#191893=CARTESIAN_POINT('Ctrl Pts',(10.3211590649999,11.6,1.33482139999999));
#191894=CARTESIAN_POINT('Ctrl Pts',(10.3199801189999,15.2,1.33480649299999));
#191895=CARTESIAN_POINT('Ctrl Pts',(10.3199801189999,11.6,1.33480649299999));
#191896=CARTESIAN_POINT('Ctrl Pts',(10.3188100709999,15.2,1.33479055299999));
#191897=CARTESIAN_POINT('Ctrl Pts',(10.3188100709999,11.6,1.33479055299999));
#191898=CARTESIAN_POINT('Ctrl Pts',(10.3176489429999,15.2,1.33477359499999));
#191899=CARTESIAN_POINT('Ctrl Pts',(10.3176489429999,11.6,1.33477359499999));
#191900=CARTESIAN_POINT('Ctrl Pts',(10.3164967599999,15.2,1.33475563599998));
#191901=CARTESIAN_POINT('Ctrl Pts',(10.3164967599999,11.6,1.33475563599998));
#191902=CARTESIAN_POINT('Ctrl Pts',(10.3153535459999,15.2,1.33473669599999));
#191903=CARTESIAN_POINT('Ctrl Pts',(10.3153535459999,11.6,1.33473669599998));
#191904=CARTESIAN_POINT('Ctrl Pts',(10.3142193239999,15.2,1.33471678699999));
#191905=CARTESIAN_POINT('Ctrl Pts',(10.3142193239999,11.6,1.33471678699998));
#191906=CARTESIAN_POINT('Ctrl Pts',(10.3130941179999,15.2,1.33469593099999));
#191907=CARTESIAN_POINT('Ctrl Pts',(10.3130941179999,11.6,1.33469593099999));
#191908=CARTESIAN_POINT('Ctrl Pts',(10.3119779519999,15.2,1.33467414199998));
#191909=CARTESIAN_POINT('Ctrl Pts',(10.3119779519999,11.6,1.33467414199998));
#191910=CARTESIAN_POINT('Ctrl Pts',(10.3108708509999,15.2,1.33465143799999));
#191911=CARTESIAN_POINT('Ctrl Pts',(10.3108708509999,11.6,1.33465143799999));
#191912=CARTESIAN_POINT('Ctrl Pts',(10.3097728379999,15.2,1.33462783699999));
#191913=CARTESIAN_POINT('Ctrl Pts',(10.3097728379999,11.6,1.33462783699999));
#191914=CARTESIAN_POINT('Ctrl Pts',(10.3086839379999,15.2,1.33460335699999));
#191915=CARTESIAN_POINT('Ctrl Pts',(10.3086839379999,11.6,1.33460335699999));
#191916=CARTESIAN_POINT('Ctrl Pts',(10.3076041749999,15.2,1.33457801399999));
#191917=CARTESIAN_POINT('Ctrl Pts',(10.3076041749999,11.6,1.33457801399999));
#191918=CARTESIAN_POINT('Ctrl Pts',(10.3065335739999,15.2,1.33455182699999));
#191919=CARTESIAN_POINT('Ctrl Pts',(10.3065335739999,11.6,1.33455182699999));
#191920=CARTESIAN_POINT('Ctrl Pts',(10.3054721599999,15.2,1.33452481299999));
#191921=CARTESIAN_POINT('Ctrl Pts',(10.3054721599999,11.6,1.33452481299999));
#191922=CARTESIAN_POINT('Ctrl Pts',(10.3044199559999,15.2,1.33449698899998));
#191923=CARTESIAN_POINT('Ctrl Pts',(10.3044199559999,11.6,1.33449698899998));
#191924=CARTESIAN_POINT('Ctrl Pts',(10.3033769899999,15.2,1.33446837399998));
#191925=CARTESIAN_POINT('Ctrl Pts',(10.3033769899999,11.6,1.33446837399998));
#191926=CARTESIAN_POINT('Ctrl Pts',(10.3023432839999,15.2,1.33443898699999));
#191927=CARTESIAN_POINT('Ctrl Pts',(10.3023432839999,11.6,1.33443898699999));
#191928=CARTESIAN_POINT('Ctrl Pts',(10.3013188639999,15.2,1.33440884399999));
#191929=CARTESIAN_POINT('Ctrl Pts',(10.3013188639999,11.6,1.33440884399999));
#191930=CARTESIAN_POINT('Ctrl Pts',(10.3003037569999,15.2,1.33437796599999));
#191931=CARTESIAN_POINT('Ctrl Pts',(10.3003037569999,11.6,1.33437796599999));
#191932=CARTESIAN_POINT('Ctrl Pts',(10.2992979849999,15.2,1.33434636899999));
#191933=CARTESIAN_POINT('Ctrl Pts',(10.2992979849999,11.6,1.33434636899999));
#191934=CARTESIAN_POINT('Ctrl Pts',(10.2983015759999,15.2,1.33431407099998));
#191935=CARTESIAN_POINT('Ctrl Pts',(10.2983015759999,11.6,1.33431407099998));
#191936=CARTESIAN_POINT('Ctrl Pts',(10.2973145539999,15.2,1.33428109299999));
#191937=CARTESIAN_POINT('Ctrl Pts',(10.2973145539999,11.6,1.33428109299999));
#191938=CARTESIAN_POINT('Ctrl Pts',(10.2963369469999,15.2,1.33424745299998));
#191939=CARTESIAN_POINT('Ctrl Pts',(10.2963369469999,11.6,1.33424745299998));
#191940=CARTESIAN_POINT('Ctrl Pts',(10.2953687779999,15.2,1.33421316799998));
#191941=CARTESIAN_POINT('Ctrl Pts',(10.2953687779999,11.6,1.33421316799998));
#191942=CARTESIAN_POINT('Ctrl Pts',(10.2944100739999,15.2,1.33417825799999));
#191943=CARTESIAN_POINT('Ctrl Pts',(10.2944100739999,11.6,1.33417825799999));
#191944=CARTESIAN_POINT('Ctrl Pts',(10.2934608629999,15.2,1.33414274199998));
#191945=CARTESIAN_POINT('Ctrl Pts',(10.2934608629999,11.6,1.33414274199998));
#191946=CARTESIAN_POINT('Ctrl Pts',(10.2925211679999,15.2,1.33410663999999));
#191947=CARTESIAN_POINT('Ctrl Pts',(10.2925211679999,11.6,1.33410663999999));
#191948=CARTESIAN_POINT('Ctrl Pts',(10.2915910169999,15.2,1.33406996999998));
#191949=CARTESIAN_POINT('Ctrl Pts',(10.2915910169999,11.6,1.33406996999998));
#191950=CARTESIAN_POINT('Ctrl Pts',(10.2906757369999,15.2,1.33403296599999));
#191951=CARTESIAN_POINT('Ctrl Pts',(10.2906757369999,11.6,1.33403296599999));
#191952=CARTESIAN_POINT('Ctrl Pts',(10.2899521419999,15.2,1.33400298799998));
#191953=CARTESIAN_POINT('Ctrl Pts',(10.2899521419999,11.6,1.33400298799998));
#191954=CARTESIAN_POINT('Ctrl Pts',(10.2894150039999,15.2,1.33398033399999));
#191955=CARTESIAN_POINT('Ctrl Pts',(10.2894150039999,11.6,1.33398033399999));
#191956=CARTESIAN_POINT('Ctrl Pts',(10.2890605209999,15.2,1.33396520799999));
#191957=CARTESIAN_POINT('Ctrl Pts',(10.2890605209999,11.6,1.33396520799998));
#191958=CARTESIAN_POINT('Ctrl Pts',(10.2888863229999,15.2,1.33395773199998));
#191959=CARTESIAN_POINT('Ctrl Pts',(10.2888863229999,11.6,1.33395773199998));
#191960=CARTESIAN_POINT('',(10.2888863229999,12.2,1.33395773199998));
#191961=CARTESIAN_POINT('',(10.2888863229999,15.2,1.33395773199998));
#191962=CARTESIAN_POINT('',(10.2888863229999,12.2,1.33395773199998));
#191963=CARTESIAN_POINT('Ctrl Pts',(11.4479048649999,12.2,1.09337742899998));
#191964=CARTESIAN_POINT('Ctrl Pts',(11.4471888789999,12.2,1.09364567099998));
#191965=CARTESIAN_POINT('Ctrl Pts',(11.4457572179999,12.2,1.09418172899999));
#191966=CARTESIAN_POINT('Ctrl Pts',(11.4436106639999,12.2,1.09498454299999));
#191967=CARTESIAN_POINT('Ctrl Pts',(11.4407504639999,12.2,1.09605241699999));
#191968=CARTESIAN_POINT('Ctrl Pts',(11.4371783349999,12.2,1.09738301699998));
#191969=CARTESIAN_POINT('Ctrl Pts',(11.4336093279999,12.2,1.09870937299998));
#191970=CARTESIAN_POINT('Ctrl Pts',(11.4300434449999,12.2,1.10003148899999));
#191971=CARTESIAN_POINT('Ctrl Pts',(11.4264806909999,12.2,1.10134936399998));
#191972=CARTESIAN_POINT('Ctrl Pts',(11.4229210689999,12.2,1.10266299899999));
#191973=CARTESIAN_POINT('Ctrl Pts',(11.4193645909999,12.2,1.10397239899998));
#191974=CARTESIAN_POINT('Ctrl Pts',(11.4158112619999,12.2,1.10527756499998));
#191975=CARTESIAN_POINT('Ctrl Pts',(11.4122610939999,12.2,1.10657849999999));
#191976=CARTESIAN_POINT('Ctrl Pts',(11.4087140989999,12.2,1.10787520999999));
#191977=CARTESIAN_POINT('Ctrl Pts',(11.4051702859999,12.2,1.10916769599998));
#191978=CARTESIAN_POINT('Ctrl Pts',(11.4016296639999,12.2,1.11045596299999));
#191979=CARTESIAN_POINT('Ctrl Pts',(11.3980922449999,12.2,1.11174001299998));
#191980=CARTESIAN_POINT('Ctrl Pts',(11.3945580339999,12.2,1.11301984899999));
#191981=CARTESIAN_POINT('Ctrl Pts',(11.3910270409999,12.2,1.11429547399998));
#191982=CARTESIAN_POINT('Ctrl Pts',(11.3874992709999,12.2,1.11556689099999));
#191983=CARTESIAN_POINT('Ctrl Pts',(11.3839747349999,12.2,1.11683410099999));
#191984=CARTESIAN_POINT('Ctrl Pts',(11.3804534399999,12.2,1.11809710599998));
#191985=CARTESIAN_POINT('Ctrl Pts',(11.3769353939999,12.2,1.11935591199999));
#191986=CARTESIAN_POINT('Ctrl Pts',(11.3734206059999,12.2,1.12061051999999));
#191987=CARTESIAN_POINT('Ctrl Pts',(11.3699090849999,12.2,1.12186093299998));
#191988=CARTESIAN_POINT('Ctrl Pts',(11.3664008399999,12.2,1.12310715499999));
#191989=CARTESIAN_POINT('Ctrl Pts',(11.3628958789999,12.2,1.12434918799998));
#191990=CARTESIAN_POINT('Ctrl Pts',(11.3593942139999,12.2,1.12558703499999));
#191991=CARTESIAN_POINT('Ctrl Pts',(11.3558958509999,12.2,1.12682069999999));
#191992=CARTESIAN_POINT('Ctrl Pts',(11.3524007989999,12.2,1.12805018499999));
#191993=CARTESIAN_POINT('Ctrl Pts',(11.3489090669999,12.2,1.12927549499998));
#191994=CARTESIAN_POINT('Ctrl Pts',(11.3454206639999,12.2,1.13049662999999));
#191995=CARTESIAN_POINT('Ctrl Pts',(11.3419355979999,12.2,1.13171359399999));
#191996=CARTESIAN_POINT('Ctrl Pts',(11.3384538779999,12.2,1.13292639099999));
#191997=CARTESIAN_POINT('Ctrl Pts',(11.3349755119999,12.2,1.13413502399998));
#191998=CARTESIAN_POINT('Ctrl Pts',(11.3315005099999,12.2,1.13533949399999));
#191999=CARTESIAN_POINT('Ctrl Pts',(11.3280288789999,12.2,1.13653980499999));
#192000=CARTESIAN_POINT('Ctrl Pts',(11.3245606299999,12.2,1.13773596199998));
#192001=CARTESIAN_POINT('Ctrl Pts',(11.3210957719999,12.2,1.13892796799998));
#192002=CARTESIAN_POINT('Ctrl Pts',(11.3176343119999,12.2,1.14011582299999));
#192003=CARTESIAN_POINT('Ctrl Pts',(11.3141762599999,12.2,1.14129953199999));
#192004=CARTESIAN_POINT('Ctrl Pts',(11.3107216239999,12.2,1.14247909899999));
#192005=CARTESIAN_POINT('Ctrl Pts',(11.3072704139999,12.2,1.14365452599999));
#192006=CARTESIAN_POINT('Ctrl Pts',(11.3038226389999,12.2,1.14482581599999));
#192007=CARTESIAN_POINT('Ctrl Pts',(11.3003783059999,12.2,1.14599297299999));
#192008=CARTESIAN_POINT('Ctrl Pts',(11.2969374249999,12.2,1.14715599999998));
#192009=CARTESIAN_POINT('Ctrl Pts',(11.2935000059999,12.2,1.14831489899998));
#192010=CARTESIAN_POINT('Ctrl Pts',(11.2900660559999,12.2,1.14946967499999));
#192011=CARTESIAN_POINT('Ctrl Pts',(11.2866355859999,12.2,1.15062032999999));
#192012=CARTESIAN_POINT('Ctrl Pts',(11.2832086039999,12.2,1.15176686799999));
#192013=CARTESIAN_POINT('Ctrl Pts',(11.2797851169999,12.2,1.15290929199999));
#192014=CARTESIAN_POINT('Ctrl Pts',(11.2763651379999,12.2,1.15404760499999));
#192015=CARTESIAN_POINT('Ctrl Pts',(11.2729486729999,12.2,1.15518180999999));
#192016=CARTESIAN_POINT('Ctrl Pts',(11.2695357319999,12.2,1.15631191099999));
#192017=CARTESIAN_POINT('Ctrl Pts',(11.2661263239999,12.2,1.15743791099999));
#192018=CARTESIAN_POINT('Ctrl Pts',(11.2627204589999,12.2,1.15855981299998));
#192019=CARTESIAN_POINT('Ctrl Pts',(11.2593181439999,12.2,1.15967762199999));
#192020=CARTESIAN_POINT('Ctrl Pts',(11.2559193889999,12.2,1.16079133899999));
#192021=CARTESIAN_POINT('Ctrl Pts',(11.2525242039999,12.2,1.16190096799999));
#192022=CARTESIAN_POINT('Ctrl Pts',(11.2491325969999,12.2,1.16300651299999));
#192023=CARTESIAN_POINT('Ctrl Pts',(11.2457445769999,12.2,1.16410797799999));
#192024=CARTESIAN_POINT('Ctrl Pts',(11.2423601539999,12.2,1.16520536499999));
#192025=CARTESIAN_POINT('Ctrl Pts',(11.2389793369999,12.2,1.16629867799999));
#192026=CARTESIAN_POINT('Ctrl Pts',(11.2356021349999,12.2,1.16738791999999));
#192027=CARTESIAN_POINT('Ctrl Pts',(11.2322285569999,12.2,1.16847309399999));
#192028=CARTESIAN_POINT('Ctrl Pts',(11.2288586119999,12.2,1.16955420599998));
#192029=CARTESIAN_POINT('Ctrl Pts',(11.2254923089999,12.2,1.17063125699998));
#192030=CARTESIAN_POINT('Ctrl Pts',(11.2221296589999,12.2,1.17170425099999));
#192031=CARTESIAN_POINT('Ctrl Pts',(11.2187706689999,12.2,1.17277319199999));
#192032=CARTESIAN_POINT('Ctrl Pts',(11.2154153489999,12.2,1.17383808299998));
#192033=CARTESIAN_POINT('Ctrl Pts',(11.2120637079999,12.2,1.17489892799998));
#192034=CARTESIAN_POINT('Ctrl Pts',(11.2087157559999,12.2,1.17595572999999));
#192035=CARTESIAN_POINT('Ctrl Pts',(11.2053715019999,12.2,1.17700849199998));
#192036=CARTESIAN_POINT('Ctrl Pts',(11.2020309559999,12.2,1.17805721999999));
#192037=CARTESIAN_POINT('Ctrl Pts',(11.1986941249999,12.2,1.17910191499998));
#192038=CARTESIAN_POINT('Ctrl Pts',(11.1953610209999,12.2,1.18014258099999));
#192039=CARTESIAN_POINT('Ctrl Pts',(11.1920316519999,12.2,1.18117922199998));
#192040=CARTESIAN_POINT('Ctrl Pts',(11.1887060269999,12.2,1.18221184299999));
#192041=CARTESIAN_POINT('Ctrl Pts',(11.1853841569999,12.2,1.18324044599999));
#192042=CARTESIAN_POINT('Ctrl Pts',(11.1820660499999,12.2,1.18426503499999));
#192043=CARTESIAN_POINT('Ctrl Pts',(11.1787517149999,12.2,1.18528561399998));
#192044=CARTESIAN_POINT('Ctrl Pts',(11.1754411629999,12.2,1.18630218499999));
#192045=CARTESIAN_POINT('Ctrl Pts',(11.1721344009999,12.2,1.18731475499999));
#192046=CARTESIAN_POINT('Ctrl Pts',(11.1688314409999,12.2,1.18832332399998));
#192047=CARTESIAN_POINT('Ctrl Pts',(11.1655322919999,12.2,1.18932789899999));
#192048=CARTESIAN_POINT('Ctrl Pts',(11.1622369629999,12.2,1.19032848099998));
#192049=CARTESIAN_POINT('Ctrl Pts',(11.1589454619999,12.2,1.19132507599998));
#192050=CARTESIAN_POINT('Ctrl Pts',(11.1556577999999,12.2,1.19231768599999));
#192051=CARTESIAN_POINT('Ctrl Pts',(11.1523739879999,12.2,1.19330631599999));
#192052=CARTESIAN_POINT('Ctrl Pts',(11.1490940329999,12.2,1.19429096899998));
#192053=CARTESIAN_POINT('Ctrl Pts',(11.1458179459999,12.2,1.19527164899999));
#192054=CARTESIAN_POINT('Ctrl Pts',(11.1425457349999,12.2,1.19624835999999));
#192055=CARTESIAN_POINT('Ctrl Pts',(11.1392774109999,12.2,1.19722110599998));
#192056=CARTESIAN_POINT('Ctrl Pts',(11.1360129839999,12.2,1.19818988999999));
#192057=CARTESIAN_POINT('Ctrl Pts',(11.1327524619999,12.2,1.19915471699999));
#192058=CARTESIAN_POINT('Ctrl Pts',(11.1294958549999,12.2,1.20011559099999));
#192059=CARTESIAN_POINT('Ctrl Pts',(11.1262431739999,12.2,1.20107251499999));
#192060=CARTESIAN_POINT('Ctrl Pts',(11.1229944269999,12.2,1.20202549299998));
#192061=CARTESIAN_POINT('Ctrl Pts',(11.1197496249999,12.2,1.20297452899999));
#192062=CARTESIAN_POINT('Ctrl Pts',(11.1165087779999,12.2,1.20391962699999));
#192063=CARTESIAN_POINT('Ctrl Pts',(11.1132718939999,12.2,1.20486079099999));
#192064=CARTESIAN_POINT('Ctrl Pts',(11.1100389819999,12.2,1.20579802499998));
#192065=CARTESIAN_POINT('Ctrl Pts',(11.1068100549999,12.2,1.20673133399999));
#192066=CARTESIAN_POINT('Ctrl Pts',(11.1035851209999,12.2,1.20766071999999));
#192067=CARTESIAN_POINT('Ctrl Pts',(11.1003641889999,12.2,1.20858618799998));
#192068=CARTESIAN_POINT('Ctrl Pts',(11.0971472699999,12.2,1.20950774199999));
#192069=CARTESIAN_POINT('Ctrl Pts',(11.0939343729999,12.2,1.21042538699998));
#192070=CARTESIAN_POINT('Ctrl Pts',(11.0907255089999,12.2,1.21133912599999));
#192071=CARTESIAN_POINT('Ctrl Pts',(11.0875206859999,12.2,1.21224896199998));
#192072=CARTESIAN_POINT('Ctrl Pts',(11.0843199139999,12.2,1.21315490199999));
#192073=CARTESIAN_POINT('Ctrl Pts',(11.0811232049999,12.2,1.21405694799999));
#192074=CARTESIAN_POINT('Ctrl Pts',(11.0779305669999,12.2,1.21495510399999));
#192075=CARTESIAN_POINT('Ctrl Pts',(11.0747420099999,12.2,1.21584937499998));
#192076=CARTESIAN_POINT('Ctrl Pts',(11.0715575449999,12.2,1.21673976599999));
#192077=CARTESIAN_POINT('Ctrl Pts',(11.0683771819999,12.2,1.21762627999999));
#192078=CARTESIAN_POINT('Ctrl Pts',(11.0652009289999,12.2,1.21850892099999));
#192079=CARTESIAN_POINT('Ctrl Pts',(11.0620287979999,12.2,1.21938769199998));
#192080=CARTESIAN_POINT('Ctrl Pts',(11.0588607969999,12.2,1.22026260099998));
#192081=CARTESIAN_POINT('Ctrl Pts',(11.0556969379999,12.2,1.22113364899999));
#192082=CARTESIAN_POINT('Ctrl Pts',(11.0525372299999,12.2,1.22200084099998));
#192083=CARTESIAN_POINT('Ctrl Pts',(11.0493816829999,12.2,1.22286418199999));
#192084=CARTESIAN_POINT('Ctrl Pts',(11.0462303079999,12.2,1.22372367599999));
#192085=CARTESIAN_POINT('Ctrl Pts',(11.0430831139999,12.2,1.22457932799998));
#192086=CARTESIAN_POINT('Ctrl Pts',(11.0399401109999,12.2,1.22543113999999));
#192087=CARTESIAN_POINT('Ctrl Pts',(11.0368013089999,12.2,1.22627911899999));
#192088=CARTESIAN_POINT('Ctrl Pts',(11.0336667189999,12.2,1.22712326699999));
#192089=CARTESIAN_POINT('Ctrl Pts',(11.0305363499999,12.2,1.22796359099999));
#192090=CARTESIAN_POINT('Ctrl Pts',(11.0274102129999,12.2,1.22880009299998));
#192091=CARTESIAN_POINT('Ctrl Pts',(11.0242883189999,12.2,1.22963277999999));
#192092=CARTESIAN_POINT('Ctrl Pts',(11.0211706759999,12.2,1.23046165299999));
#192093=CARTESIAN_POINT('Ctrl Pts',(11.0180572959999,12.2,1.23128671899998));
#192094=CARTESIAN_POINT('Ctrl Pts',(11.0149481889999,12.2,1.23210798199999));
#192095=CARTESIAN_POINT('Ctrl Pts',(11.0118433639999,12.2,1.23292544599999));
#192096=CARTESIAN_POINT('Ctrl Pts',(11.0087428319999,12.2,1.23373911599999));
#192097=CARTESIAN_POINT('Ctrl Pts',(11.0056466049999,12.2,1.23454899599999));
#192098=CARTESIAN_POINT('Ctrl Pts',(11.0025546899999,12.2,1.23535509099999));
#192099=CARTESIAN_POINT('Ctrl Pts',(10.9994670979999,12.2,1.23615740499998));
#192100=CARTESIAN_POINT('Ctrl Pts',(10.9963838419999,12.2,1.23695594399999));
#192101=CARTESIAN_POINT('Ctrl Pts',(10.9933049299999,12.2,1.23775071099999));
#192102=CARTESIAN_POINT('Ctrl Pts',(10.9902303719999,12.2,1.23854171099998));
#192103=CARTESIAN_POINT('Ctrl Pts',(10.9871601809999,12.2,1.23932894899998));
#192104=CARTESIAN_POINT('Ctrl Pts',(10.9840943639999,12.2,1.24011242999998));
#192105=CARTESIAN_POINT('Ctrl Pts',(10.9810329339999,12.2,1.24089215599998));
#192106=CARTESIAN_POINT('Ctrl Pts',(10.9779759009999,12.2,1.24166813599999));
#192107=CARTESIAN_POINT('Ctrl Pts',(10.9749232749999,12.2,1.24244037199999));
#192108=CARTESIAN_POINT('Ctrl Pts',(10.9718750649999,12.2,1.24320886799998));
#192109=CARTESIAN_POINT('Ctrl Pts',(10.9688312839999,12.2,1.24397363099999));
#192110=CARTESIAN_POINT('Ctrl Pts',(10.9657919419999,12.2,1.24473466399999));
#192111=CARTESIAN_POINT('Ctrl Pts',(10.9627570469999,12.2,1.24549197299999));
#192112=CARTESIAN_POINT('Ctrl Pts',(10.9597266129999,12.2,1.24624556199999));
#192113=CARTESIAN_POINT('Ctrl Pts',(10.9567006489999,12.2,1.24699543599998));
#192114=CARTESIAN_POINT('Ctrl Pts',(10.9536791659999,12.2,1.24774160099999));
#192115=CARTESIAN_POINT('Ctrl Pts',(10.9506621729999,12.2,1.24848405899999));
#192116=CARTESIAN_POINT('Ctrl Pts',(10.9476496829999,12.2,1.24922281699998));
#192117=CARTESIAN_POINT('Ctrl Pts',(10.9446417049999,12.2,1.24995787999998));
#192118=CARTESIAN_POINT('Ctrl Pts',(10.9416382509999,12.2,1.25068925199999));
#192119=CARTESIAN_POINT('Ctrl Pts',(10.9386393289999,12.2,1.25141693899999));
#192120=CARTESIAN_POINT('Ctrl Pts',(10.9356449539999,12.2,1.25214094399999));
#192121=CARTESIAN_POINT('Ctrl Pts',(10.9326551319999,12.2,1.25286127399999));
#192122=CARTESIAN_POINT('Ctrl Pts',(10.9296698779999,12.2,1.25357793199999));
#192123=CARTESIAN_POINT('Ctrl Pts',(10.9266891999999,12.2,1.25429092499999));
#192124=CARTESIAN_POINT('Ctrl Pts',(10.9237131089999,12.2,1.25500025699999));
#192125=CARTESIAN_POINT('Ctrl Pts',(10.9207416159999,12.2,1.25570593399999));
#192126=CARTESIAN_POINT('Ctrl Pts',(10.9177747329999,12.2,1.25640795999999));
#192127=CARTESIAN_POINT('Ctrl Pts',(10.9148124699999,12.2,1.25710633999998));
#192128=CARTESIAN_POINT('Ctrl Pts',(10.9118548369999,12.2,1.25780107899998));
#192129=CARTESIAN_POINT('Ctrl Pts',(10.9089018469999,12.2,1.25849218299999));
#192130=CARTESIAN_POINT('Ctrl Pts',(10.9059535079999,12.2,1.25917965599998));
#192131=CARTESIAN_POINT('Ctrl Pts',(10.9030098339999,12.2,1.25986350499999));
#192132=CARTESIAN_POINT('Ctrl Pts',(10.9000708339999,12.2,1.26054373299999));
#192133=CARTESIAN_POINT('Ctrl Pts',(10.8971365199999,12.2,1.26122034599998));
#192134=CARTESIAN_POINT('Ctrl Pts',(10.8942069009999,12.2,1.26189335099999));
#192135=CARTESIAN_POINT('Ctrl Pts',(10.8912819899999,12.2,1.26256274999998));
#192136=CARTESIAN_POINT('Ctrl Pts',(10.8883617979999,12.2,1.26322854999998));
#192137=CARTESIAN_POINT('Ctrl Pts',(10.8854463339999,12.2,1.26389075699999));
#192138=CARTESIAN_POINT('Ctrl Pts',(10.8825356119999,12.2,1.26454937599998));
#192139=CARTESIAN_POINT('Ctrl Pts',(10.8796296409999,12.2,1.26520441099998));
#192140=CARTESIAN_POINT('Ctrl Pts',(10.8767284329999,12.2,1.26585586799999));
#192141=CARTESIAN_POINT('Ctrl Pts',(10.8738319979999,12.2,1.26650375199999));
#192142=CARTESIAN_POINT('Ctrl Pts',(10.8709403489999,12.2,1.26714806999999));
#192143=CARTESIAN_POINT('Ctrl Pts',(10.8680534959999,12.2,1.26778882499998));
#192144=CARTESIAN_POINT('Ctrl Pts',(10.8651714489999,12.2,1.26842602399998));
#192145=CARTESIAN_POINT('Ctrl Pts',(10.8622942209999,12.2,1.26905967299999));
#192146=CARTESIAN_POINT('Ctrl Pts',(10.8594218239999,12.2,1.26968977599998));
#192147=CARTESIAN_POINT('Ctrl Pts',(10.8565542679999,12.2,1.27031633899998));
#192148=CARTESIAN_POINT('Ctrl Pts',(10.8536915629999,12.2,1.27093936699998));
#192149=CARTESIAN_POINT('Ctrl Pts',(10.8508337229999,12.2,1.27155886699999));
#192150=CARTESIAN_POINT('Ctrl Pts',(10.8479807569999,12.2,1.27217484299999));
#192151=CARTESIAN_POINT('Ctrl Pts',(10.8451326779999,12.2,1.27278730199999));
#192152=CARTESIAN_POINT('Ctrl Pts',(10.8422894959999,12.2,1.27339624799998));
#192153=CARTESIAN_POINT('Ctrl Pts',(10.8394512219999,12.2,1.27400168799999));
#192154=CARTESIAN_POINT('Ctrl Pts',(10.8366178699999,12.2,1.27460362699999));
#192155=CARTESIAN_POINT('Ctrl Pts',(10.8337894499999,12.2,1.27520206999999));
#192156=CARTESIAN_POINT('Ctrl Pts',(10.8309659719999,12.2,1.27579702399998));
#192157=CARTESIAN_POINT('Ctrl Pts',(10.8281474499999,12.2,1.27638849299998));
#192158=CARTESIAN_POINT('Ctrl Pts',(10.8253338939999,12.2,1.27697648499999));
#192159=CARTESIAN_POINT('Ctrl Pts',(10.8225253159999,12.2,1.27756100399999));
#192160=CARTESIAN_POINT('Ctrl Pts',(10.8197217269999,12.2,1.27814205699998));
#192161=CARTESIAN_POINT('Ctrl Pts',(10.8169231379999,12.2,1.27871964799999));
#192162=CARTESIAN_POINT('Ctrl Pts',(10.8141295629999,12.2,1.27929378499998));
#192163=CARTESIAN_POINT('Ctrl Pts',(10.8113410119999,12.2,1.27986447199998));
#192164=CARTESIAN_POINT('Ctrl Pts',(10.8085574969999,12.2,1.28043171599999));
#192165=CARTESIAN_POINT('Ctrl Pts',(10.8057790279999,12.2,1.28099552199998));
#192166=CARTESIAN_POINT('Ctrl Pts',(10.8030056189999,12.2,1.28155589599999));
#192167=CARTESIAN_POINT('Ctrl Pts',(10.8002372809999,12.2,1.28211284599999));
#192168=CARTESIAN_POINT('Ctrl Pts',(10.7974740259999,12.2,1.28266637499999));
#192169=CARTESIAN_POINT('Ctrl Pts',(10.7947158649999,12.2,1.28321648999998));
#192170=CARTESIAN_POINT('Ctrl Pts',(10.7919628099999,12.2,1.28376319699999));
#192171=CARTESIAN_POINT('Ctrl Pts',(10.7892148729999,12.2,1.28430650299999));
#192172=CARTESIAN_POINT('Ctrl Pts',(10.7864720659999,12.2,1.28484641299998));
#192173=CARTESIAN_POINT('Ctrl Pts',(10.7837344009999,12.2,1.28538293399998));
#192174=CARTESIAN_POINT('Ctrl Pts',(10.7810018879999,12.2,1.28591607099999));
#192175=CARTESIAN_POINT('Ctrl Pts',(10.7782745419999,12.2,1.28644583099998));
#192176=CARTESIAN_POINT('Ctrl Pts',(10.7755523729999,12.2,1.28697221799999));
#192177=CARTESIAN_POINT('Ctrl Pts',(10.7728353919999,12.2,1.28749524099999));
#192178=CARTESIAN_POINT('Ctrl Pts',(10.7701236149999,12.2,1.28801490499999));
#192179=CARTESIAN_POINT('Ctrl Pts',(10.7674170489999,12.2,1.28853121599999));
#192180=CARTESIAN_POINT('Ctrl Pts',(10.7647157089999,12.2,1.28904418099999));
#192181=CARTESIAN_POINT('Ctrl Pts',(10.7620196059999,12.2,1.28955380499999));
#192182=CARTESIAN_POINT('Ctrl Pts',(10.7593287539999,12.2,1.29006009499999));
#192183=CARTESIAN_POINT('Ctrl Pts',(10.7566431619999,12.2,1.29056305799998));
#192184=CARTESIAN_POINT('Ctrl Pts',(10.7539628449999,12.2,1.29106269999999));
#192185=CARTESIAN_POINT('Ctrl Pts',(10.7512878129999,12.2,1.29155902599999));
#192186=CARTESIAN_POINT('Ctrl Pts',(10.7486180789999,12.2,1.29205204399998));
#192187=CARTESIAN_POINT('Ctrl Pts',(10.7459536549999,12.2,1.29254175999999));
#192188=CARTESIAN_POINT('Ctrl Pts',(10.7432945539999,12.2,1.29302817899998));
#192189=CARTESIAN_POINT('Ctrl Pts',(10.7406407879999,12.2,1.29351130999999));
#192190=CARTESIAN_POINT('Ctrl Pts',(10.7379923689999,12.2,1.29399115799998));
#192191=CARTESIAN_POINT('Ctrl Pts',(10.7353493089999,12.2,1.29446772899998));
#192192=CARTESIAN_POINT('Ctrl Pts',(10.7327116219999,12.2,1.29494102999999));
#192193=CARTESIAN_POINT('Ctrl Pts',(10.7300793179999,12.2,1.29541106899998));
#192194=CARTESIAN_POINT('Ctrl Pts',(10.7274524109999,12.2,1.29587785099998));
#192195=CARTESIAN_POINT('Ctrl Pts',(10.7248309119999,12.2,1.29634138299998));
#192196=CARTESIAN_POINT('Ctrl Pts',(10.7222148359999,12.2,1.29680166999998));
#192197=CARTESIAN_POINT('Ctrl Pts',(10.7196041929999,12.2,1.29725872299999));
#192198=CARTESIAN_POINT('Ctrl Pts',(10.7169989959999,12.2,1.29771254499999));
#192199=CARTESIAN_POINT('Ctrl Pts',(10.7143992589999,12.2,1.29816314299998));
#192200=CARTESIAN_POINT('Ctrl Pts',(10.7118049929999,12.2,1.29861052499999));
#192201=CARTESIAN_POINT('Ctrl Pts',(10.7092162099999,12.2,1.29905469699999));
#192202=CARTESIAN_POINT('Ctrl Pts',(10.7066329249999,12.2,1.29949566599999));
#192203=CARTESIAN_POINT('Ctrl Pts',(10.7040551489999,12.2,1.29993343899999));
#192204=CARTESIAN_POINT('Ctrl Pts',(10.7014828959999,12.2,1.30036802199998));
#192205=CARTESIAN_POINT('Ctrl Pts',(10.6989161759999,12.2,1.30079942299998));
#192206=CARTESIAN_POINT('Ctrl Pts',(10.6963550049999,12.2,1.30122764799999));
#192207=CARTESIAN_POINT('Ctrl Pts',(10.6937993929999,12.2,1.30165270599999));
#192208=CARTESIAN_POINT('Ctrl Pts',(10.6912493539999,12.2,1.30207460099999));
#192209=CARTESIAN_POINT('Ctrl Pts',(10.6887049019999,12.2,1.30249334199998));
#192210=CARTESIAN_POINT('Ctrl Pts',(10.6861660479999,12.2,1.30290893499998));
#192211=CARTESIAN_POINT('Ctrl Pts',(10.6836328059999,12.2,1.30332138799998));
#192212=CARTESIAN_POINT('Ctrl Pts',(10.6811051889999,12.2,1.30373070699998));
#192213=CARTESIAN_POINT('Ctrl Pts',(10.6785832079999,12.2,1.30413689899999));
#192214=CARTESIAN_POINT('Ctrl Pts',(10.6760668779999,12.2,1.30453997299998));
#192215=CARTESIAN_POINT('Ctrl Pts',(10.6735562119999,12.2,1.30493993399998));
#192216=CARTESIAN_POINT('Ctrl Pts',(10.6710512209999,12.2,1.30533679099999));
#192217=CARTESIAN_POINT('Ctrl Pts',(10.6685519209999,12.2,1.30573054999998));
#192218=CARTESIAN_POINT('Ctrl Pts',(10.6660583229999,12.2,1.30612121799999));
#192219=CARTESIAN_POINT('Ctrl Pts',(10.6635704409999,12.2,1.30650880399998));
#192220=CARTESIAN_POINT('Ctrl Pts',(10.6610882879999,12.2,1.30689331299998));
#192221=CARTESIAN_POINT('Ctrl Pts',(10.6586118759999,12.2,1.30727475299999));
#192222=CARTESIAN_POINT('Ctrl Pts',(10.6561412199999,12.2,1.30765313299999));
#192223=CARTESIAN_POINT('Ctrl Pts',(10.6536763329999,12.2,1.30802845899999));
#192224=CARTESIAN_POINT('Ctrl Pts',(10.6512172259999,12.2,1.30840073799999));
#192225=CARTESIAN_POINT('Ctrl Pts',(10.6487639159999,12.2,1.30876997899998));
#192226=CARTESIAN_POINT('Ctrl Pts',(10.6463164129999,12.2,1.30913618899998));
#192227=CARTESIAN_POINT('Ctrl Pts',(10.6438747329999,12.2,1.30949937399999));
#192228=CARTESIAN_POINT('Ctrl Pts',(10.6414388879999,12.2,1.30985954199998));
#192229=CARTESIAN_POINT('Ctrl Pts',(10.6390088909999,12.2,1.31021670299999));
#192230=CARTESIAN_POINT('Ctrl Pts',(10.6365847569999,12.2,1.31057086099998));
#192231=CARTESIAN_POINT('Ctrl Pts',(10.6341664979999,12.2,1.31092202699998));
#192232=CARTESIAN_POINT('Ctrl Pts',(10.6317541279999,12.2,1.31127020699998));
#192233=CARTESIAN_POINT('Ctrl Pts',(10.6293476599999,12.2,1.31161540699999));
#192234=CARTESIAN_POINT('Ctrl Pts',(10.6269471099999,12.2,1.31195763899999));
#192235=CARTESIAN_POINT('Ctrl Pts',(10.6245524889999,12.2,1.31229690699998));
#192236=CARTESIAN_POINT('Ctrl Pts',(10.6221638119999,12.2,1.31263321999999));
#192237=CARTESIAN_POINT('Ctrl Pts',(10.6197810909999,12.2,1.31296658599998));
#192238=CARTESIAN_POINT('Ctrl Pts',(10.6174043419999,12.2,1.31329701299999));
#192239=CARTESIAN_POINT('Ctrl Pts',(10.6150335779999,12.2,1.31362450999998));
#192240=CARTESIAN_POINT('Ctrl Pts',(10.6126688119999,12.2,1.31394908099999));
#192241=CARTESIAN_POINT('Ctrl Pts',(10.6103100589999,12.2,1.31427073799999));
#192242=CARTESIAN_POINT('Ctrl Pts',(10.6079573329999,12.2,1.31458948699999));
#192243=CARTESIAN_POINT('Ctrl Pts',(10.6056106459999,12.2,1.31490533699999));
#192244=CARTESIAN_POINT('Ctrl Pts',(10.6032700129999,12.2,1.31521829699999));
#192245=CARTESIAN_POINT('Ctrl Pts',(10.6009354489999,12.2,1.31552837099999));
#192246=CARTESIAN_POINT('Ctrl Pts',(10.5986069669999,12.2,1.31583557099999));
#192247=CARTESIAN_POINT('Ctrl Pts',(10.5962845809999,12.2,1.31613990499998));
#192248=CARTESIAN_POINT('Ctrl Pts',(10.5935050499009,12.2,1.31650167378684));
#192249=CARTESIAN_POINT('Ctrl Pts',(10.5907347060494,12.2,1.31685916610655));
#192250=CARTESIAN_POINT('Ctrl Pts',(10.5879735759504,12.2,1.31721239989341));
#192251=CARTESIAN_POINT('Ctrl Pts',(10.5852216883489,12.2,1.31756139018143));
#192252=CARTESIAN_POINT('Ctrl Pts',(10.5824790749999,12.2,1.31790615499999));
#192253=CARTESIAN_POINT('Ctrl Pts',(10.5801997579999,12.2,1.31819064899998));
#192254=CARTESIAN_POINT('Ctrl Pts',(10.5779266509999,12.2,1.31847234299999));
#192255=CARTESIAN_POINT('Ctrl Pts',(10.5756597679999,12.2,1.31875124499999));
#192256=CARTESIAN_POINT('Ctrl Pts',(10.5733991249999,12.2,1.31902736299998));
#192257=CARTESIAN_POINT('Ctrl Pts',(10.5711447329999,12.2,1.31930070599998));
#192258=CARTESIAN_POINT('Ctrl Pts',(10.5688966099999,12.2,1.31957128299999));
#192259=CARTESIAN_POINT('Ctrl Pts',(10.5666547689999,12.2,1.31983910099999));
#192260=CARTESIAN_POINT('Ctrl Pts',(10.5644192249999,12.2,1.32010417099998));
#192261=CARTESIAN_POINT('Ctrl Pts',(10.5621899909999,12.2,1.32036649799999));
#192262=CARTESIAN_POINT('Ctrl Pts',(10.5599670829999,12.2,1.32062609399998));
#192263=CARTESIAN_POINT('Ctrl Pts',(10.5577505169999,12.2,1.32088296799999));
#192264=CARTESIAN_POINT('Ctrl Pts',(10.5555403039999,12.2,1.32113712699998));
#192265=CARTESIAN_POINT('Ctrl Pts',(10.5533364629999,12.2,1.32138857999998));
#192266=CARTESIAN_POINT('Ctrl Pts',(10.5511390059999,12.2,1.32163733699999));
#192267=CARTESIAN_POINT('Ctrl Pts',(10.5489479479999,12.2,1.32188340599999));
#192268=CARTESIAN_POINT('Ctrl Pts',(10.5467633059999,12.2,1.32212679499998));
#192269=CARTESIAN_POINT('Ctrl Pts',(10.5445850929999,12.2,1.32236751399998));
#192270=CARTESIAN_POINT('Ctrl Pts',(10.5424133229999,12.2,1.32260557299999));
#192271=CARTESIAN_POINT('Ctrl Pts',(10.5402480139999,12.2,1.32284097999999));
#192272=CARTESIAN_POINT('Ctrl Pts',(10.5380891789999,12.2,1.32307374399999));
#192273=CARTESIAN_POINT('Ctrl Pts',(10.5359368329999,12.2,1.32330387399998));
#192274=CARTESIAN_POINT('Ctrl Pts',(10.5337909929999,12.2,1.32353137899999));
#192275=CARTESIAN_POINT('Ctrl Pts',(10.5316516719999,12.2,1.32375626999998));
#192276=CARTESIAN_POINT('Ctrl Pts',(10.5295188859999,12.2,1.32397855399998));
#192277=CARTESIAN_POINT('Ctrl Pts',(10.5273926489999,12.2,1.32419824099999));
#192278=CARTESIAN_POINT('Ctrl Pts',(10.5252729789999,12.2,1.32441534099998));
#192279=CARTESIAN_POINT('Ctrl Pts',(10.5231598899999,12.2,1.32462986199998));
#192280=CARTESIAN_POINT('Ctrl Pts',(10.5210533959999,12.2,1.32484181499999));
#192281=CARTESIAN_POINT('Ctrl Pts',(10.5189535149999,12.2,1.32505120799999));
#192282=CARTESIAN_POINT('Ctrl Pts',(10.5168602599999,12.2,1.32525805099998));
#192283=CARTESIAN_POINT('Ctrl Pts',(10.5147736479999,12.2,1.32546235499999));
#192284=CARTESIAN_POINT('Ctrl Pts',(10.5126936939999,12.2,1.32566412699999));
#192285=CARTESIAN_POINT('Ctrl Pts',(10.5106204149999,12.2,1.32586337799999));
#192286=CARTESIAN_POINT('Ctrl Pts',(10.5085538239999,12.2,1.32606011699998));
#192287=CARTESIAN_POINT('Ctrl Pts',(10.5064939389999,12.2,1.32625435499999));
#192288=CARTESIAN_POINT('Ctrl Pts',(10.5044407749999,12.2,1.32644610099999));
#192289=CARTESIAN_POINT('Ctrl Pts',(10.5023943459999,12.2,1.32663536299999));
#192290=CARTESIAN_POINT('Ctrl Pts',(10.5003546709999,12.2,1.32682215399999));
#192291=CARTESIAN_POINT('Ctrl Pts',(10.4983217629999,12.2,1.32700648099998));
#192292=CARTESIAN_POINT('Ctrl Pts',(10.4962956399999,12.2,1.32718835599999));
#192293=CARTESIAN_POINT('Ctrl Pts',(10.4942763159999,12.2,1.32736778799998));
#192294=CARTESIAN_POINT('Ctrl Pts',(10.4922638099999,12.2,1.32754478599999));
#192295=CARTESIAN_POINT('Ctrl Pts',(10.4902581349999,12.2,1.32771936199998));
#192296=CARTESIAN_POINT('Ctrl Pts',(10.4882593079999,12.2,1.32789152599999));
#192297=CARTESIAN_POINT('Ctrl Pts',(10.4862673459999,12.2,1.32806128699999));
#192298=CARTESIAN_POINT('Ctrl Pts',(10.4842822649999,12.2,1.32822865399998));
#192299=CARTESIAN_POINT('Ctrl Pts',(10.4823040789999,12.2,1.32839363899999));
#192300=CARTESIAN_POINT('Ctrl Pts',(10.4803328079999,12.2,1.32855625199999));
#192301=CARTESIAN_POINT('Ctrl Pts',(10.4783684649999,12.2,1.32871650399998));
#192302=CARTESIAN_POINT('Ctrl Pts',(10.4764110689999,12.2,1.32887440299998));
#192303=CARTESIAN_POINT('Ctrl Pts',(10.4744606349999,12.2,1.32902996199999));
#192304=CARTESIAN_POINT('Ctrl Pts',(10.4725171799999,12.2,1.32918318999999));
#192305=CARTESIAN_POINT('Ctrl Pts',(10.4705807189999,12.2,1.32933409699998));
#192306=CARTESIAN_POINT('Ctrl Pts',(10.4686512709999,12.2,1.32948269499999));
#192307=CARTESIAN_POINT('Ctrl Pts',(10.4667288519999,12.2,1.32962899399999));
#192308=CARTESIAN_POINT('Ctrl Pts',(10.4648134769999,12.2,1.32977300399999));
#192309=CARTESIAN_POINT('Ctrl Pts',(10.4629051649999,12.2,1.32991473599999));
#192310=CARTESIAN_POINT('Ctrl Pts',(10.4610039309999,12.2,1.33005419999999));
#192311=CARTESIAN_POINT('Ctrl Pts',(10.4591097919999,12.2,1.33019140799998));
#192312=CARTESIAN_POINT('Ctrl Pts',(10.4572227669999,12.2,1.33032637099999));
#192313=CARTESIAN_POINT('Ctrl Pts',(10.4553428709999,12.2,1.33045909899999));
#192314=CARTESIAN_POINT('Ctrl Pts',(10.4534701199999,12.2,1.33058960299998));
#192315=CARTESIAN_POINT('Ctrl Pts',(10.4516045329999,12.2,1.33071789399999));
#192316=CARTESIAN_POINT('Ctrl Pts',(10.4497461279999,12.2,1.33084398299999));
#192317=CARTESIAN_POINT('Ctrl Pts',(10.4478949189999,12.2,1.33096787999999));
#192318=CARTESIAN_POINT('Ctrl Pts',(10.4460509249999,12.2,1.33108959799999));
#192319=CARTESIAN_POINT('Ctrl Pts',(10.4442141639999,12.2,1.33120914799999));
#192320=CARTESIAN_POINT('Ctrl Pts',(10.4423846519999,12.2,1.33132653899999));
#192321=CARTESIAN_POINT('Ctrl Pts',(10.4405624069999,12.2,1.33144178399998));
#192322=CARTESIAN_POINT('Ctrl Pts',(10.4387474469999,12.2,1.33155489399998));
#192323=CARTESIAN_POINT('Ctrl Pts',(10.4369397879999,12.2,1.33166588099999));
#192324=CARTESIAN_POINT('Ctrl Pts',(10.4351394479999,12.2,1.33177475499998));
#192325=CARTESIAN_POINT('Ctrl Pts',(10.4333464449999,12.2,1.33188152799999));
#192326=CARTESIAN_POINT('Ctrl Pts',(10.4315607969999,12.2,1.33198621299998));
#192327=CARTESIAN_POINT('Ctrl Pts',(10.4297825219999,12.2,1.33208881899999));
#192328=CARTESIAN_POINT('Ctrl Pts',(10.4280116349999,12.2,1.33218935899999));
#192329=CARTESIAN_POINT('Ctrl Pts',(10.4262481579999,12.2,1.33228784499998));
#192330=CARTESIAN_POINT('Ctrl Pts',(10.4244921049999,12.2,1.33238428799999));
#192331=CARTESIAN_POINT('Ctrl Pts',(10.4227434979999,12.2,1.33247869999999));
#192332=CARTESIAN_POINT('Ctrl Pts',(10.4210023509999,12.2,1.33257109199999));
#192333=CARTESIAN_POINT('Ctrl Pts',(10.4192686839999,12.2,1.33266147799999));
#192334=CARTESIAN_POINT('Ctrl Pts',(10.4175425149999,12.2,1.33274986699998));
#192335=CARTESIAN_POINT('Ctrl Pts',(10.4158238619999,12.2,1.33283627399999));
#192336=CARTESIAN_POINT('Ctrl Pts',(10.4141127429999,12.2,1.33292070899998));
#192337=CARTESIAN_POINT('Ctrl Pts',(10.4124091789999,12.2,1.33300318499999));
#192338=CARTESIAN_POINT('Ctrl Pts',(10.4107131829999,12.2,1.33308371299998));
#192339=CARTESIAN_POINT('Ctrl Pts',(10.4090247779999,12.2,1.33316230699998));
#192340=CARTESIAN_POINT('Ctrl Pts',(10.4073439809999,12.2,1.33323897699999));
#192341=CARTESIAN_POINT('Ctrl Pts',(10.4056708099999,12.2,1.33331373699999));
#192342=CARTESIAN_POINT('Ctrl Pts',(10.4040052849999,12.2,1.33338659999998));
#192343=CARTESIAN_POINT('Ctrl Pts',(10.4023474229999,12.2,1.33345757799999));
#192344=CARTESIAN_POINT('Ctrl Pts',(10.4006972429999,12.2,1.33352668099999));
#192345=CARTESIAN_POINT('Ctrl Pts',(10.3990547659999,12.2,1.33359392399999));
#192346=CARTESIAN_POINT('Ctrl Pts',(10.3974200079999,12.2,1.33365931999998));
#192347=CARTESIAN_POINT('Ctrl Pts',(10.3957929889999,12.2,1.33372287999999));
#192348=CARTESIAN_POINT('Ctrl Pts',(10.3941737289999,12.2,1.33378461799999));
#192349=CARTESIAN_POINT('Ctrl Pts',(10.3925622469999,12.2,1.33384454499998));
#192350=CARTESIAN_POINT('Ctrl Pts',(10.3909585599999,12.2,1.33390267699999));
#192351=CARTESIAN_POINT('Ctrl Pts',(10.3893626899999,12.2,1.33395902399998));
#192352=CARTESIAN_POINT('Ctrl Pts',(10.3877746539999,12.2,1.33401360099999));
#192353=CARTESIAN_POINT('Ctrl Pts',(10.3861944729999,12.2,1.33406641899999));
#192354=CARTESIAN_POINT('Ctrl Pts',(10.3846221649999,12.2,1.33411749199999));
#192355=CARTESIAN_POINT('Ctrl Pts',(10.3830577499999,12.2,1.33416683399998));
#192356=CARTESIAN_POINT('Ctrl Pts',(10.3815012489999,12.2,1.33421445799998));
#192357=CARTESIAN_POINT('Ctrl Pts',(10.3799526789999,12.2,1.33426037599999));
#192358=CARTESIAN_POINT('Ctrl Pts',(10.3784120619999,12.2,1.33430460199999));
#192359=CARTESIAN_POINT('Ctrl Pts',(10.3768794159999,12.2,1.33434714999999));
#192360=CARTESIAN_POINT('Ctrl Pts',(10.3753547629999,12.2,1.33438803399998));
#192361=CARTESIAN_POINT('Ctrl Pts',(10.3738381209999,12.2,1.33442726599998));
#192362=CARTESIAN_POINT('Ctrl Pts',(10.3723295099999,12.2,1.33446485899999));
#192363=CARTESIAN_POINT('Ctrl Pts',(10.3708289509999,12.2,1.33450082899999));
#192364=CARTESIAN_POINT('Ctrl Pts',(10.3693364639999,12.2,1.33453518899998));
#192365=CARTESIAN_POINT('Ctrl Pts',(10.3678520689999,12.2,1.33456795199999));
#192366=CARTESIAN_POINT('Ctrl Pts',(10.3663757859999,12.2,1.33459913299999));
#192367=CARTESIAN_POINT('Ctrl Pts',(10.3649076359999,12.2,1.33462874399998));
#192368=CARTESIAN_POINT('Ctrl Pts',(10.3634476389999,12.2,1.33465680099999));
#192369=CARTESIAN_POINT('Ctrl Pts',(10.3619958159999,12.2,1.33468331699999));
#192370=CARTESIAN_POINT('Ctrl Pts',(10.3605521859999,12.2,1.33470830799999));
#192371=CARTESIAN_POINT('Ctrl Pts',(10.3591167719999,12.2,1.33473178499999));
#192372=CARTESIAN_POINT('Ctrl Pts',(10.3576895929999,12.2,1.33475376599999));
#192373=CARTESIAN_POINT('Ctrl Pts',(10.3562706699999,12.2,1.33477426199998));
#192374=CARTESIAN_POINT('Ctrl Pts',(10.3548600249999,12.2,1.33479328899998));
#192375=CARTESIAN_POINT('Ctrl Pts',(10.3534576789999,12.2,1.33481086299998));
#192376=CARTESIAN_POINT('Ctrl Pts',(10.3520636509999,12.2,1.33482699499998));
#192377=CARTESIAN_POINT('Ctrl Pts',(10.3506779649999,12.2,1.33484170199999));
#192378=CARTESIAN_POINT('Ctrl Pts',(10.3493006389999,12.2,1.33485499899999));
#192379=CARTESIAN_POINT('Ctrl Pts',(10.3479316969999,12.2,1.33486689999998));
#192380=CARTESIAN_POINT('Ctrl Pts',(10.3465711599999,12.2,1.33487741899998));
#192381=CARTESIAN_POINT('Ctrl Pts',(10.3452190479999,12.2,1.33488657399999));
#192382=CARTESIAN_POINT('Ctrl Pts',(10.3438753839999,12.2,1.33489437599998));
#192383=CARTESIAN_POINT('Ctrl Pts',(10.3425401889999,12.2,1.33490084399998));
#192384=CARTESIAN_POINT('Ctrl Pts',(10.3412134849999,12.2,1.33490598999999));
#192385=CARTESIAN_POINT('Ctrl Pts',(10.3398952939999,12.2,1.33490982999998));
#192386=CARTESIAN_POINT('Ctrl Pts',(10.3385856379999,12.2,1.33491238099999));
#192387=CARTESIAN_POINT('Ctrl Pts',(10.3372845369999,12.2,1.33491365699999));
#192388=CARTESIAN_POINT('Ctrl Pts',(10.3359920159999,12.2,1.33491367299999));
#192389=CARTESIAN_POINT('Ctrl Pts',(10.3347080959999,12.2,1.33491244599998));
#192390=CARTESIAN_POINT('Ctrl Pts',(10.3334327989999,12.2,1.33490999099998));
#192391=CARTESIAN_POINT('Ctrl Pts',(10.3321661469999,12.2,1.33490632399999));
#192392=CARTESIAN_POINT('Ctrl Pts',(10.3309081639999,12.2,1.33490145999998));
#192393=CARTESIAN_POINT('Ctrl Pts',(10.3296588699999,12.2,1.33489541599999));
#192394=CARTESIAN_POINT('Ctrl Pts',(10.3284182899999,12.2,1.33488820699998));
#192395=CARTESIAN_POINT('Ctrl Pts',(10.3271864459999,12.2,1.33487984899999));
#192396=CARTESIAN_POINT('Ctrl Pts',(10.3259633609999,12.2,1.33487035899998));
#192397=CARTESIAN_POINT('Ctrl Pts',(10.3247490569999,12.2,1.33485975299998));
#192398=CARTESIAN_POINT('Ctrl Pts',(10.3235435579999,12.2,1.33484804699998));
#192399=CARTESIAN_POINT('Ctrl Pts',(10.3223468859999,12.2,1.33483525699999));
#192400=CARTESIAN_POINT('Ctrl Pts',(10.3211590649999,12.2,1.33482139999999));
#192401=CARTESIAN_POINT('Ctrl Pts',(10.3199801189999,12.2,1.33480649299999));
#192402=CARTESIAN_POINT('Ctrl Pts',(10.3188100709999,12.2,1.33479055299999));
#192403=CARTESIAN_POINT('Ctrl Pts',(10.3176489429999,12.2,1.33477359499999));
#192404=CARTESIAN_POINT('Ctrl Pts',(10.3164967599999,12.2,1.33475563599998));
#192405=CARTESIAN_POINT('Ctrl Pts',(10.3153535459999,12.2,1.33473669599999));
#192406=CARTESIAN_POINT('Ctrl Pts',(10.3142193239999,12.2,1.33471678699999));
#192407=CARTESIAN_POINT('Ctrl Pts',(10.3130941179999,12.2,1.33469593099999));
#192408=CARTESIAN_POINT('Ctrl Pts',(10.3119779519999,12.2,1.33467414199998));
#192409=CARTESIAN_POINT('Ctrl Pts',(10.3108708509999,12.2,1.33465143799999));
#192410=CARTESIAN_POINT('Ctrl Pts',(10.3097728379999,12.2,1.33462783699999));
#192411=CARTESIAN_POINT('Ctrl Pts',(10.3086839379999,12.2,1.33460335699999));
#192412=CARTESIAN_POINT('Ctrl Pts',(10.3076041749999,12.2,1.33457801399999));
#192413=CARTESIAN_POINT('Ctrl Pts',(10.3065335739999,12.2,1.33455182699999));
#192414=CARTESIAN_POINT('Ctrl Pts',(10.3054721599999,12.2,1.33452481299999));
#192415=CARTESIAN_POINT('Ctrl Pts',(10.3044199559999,12.2,1.33449698899998));
#192416=CARTESIAN_POINT('Ctrl Pts',(10.3033769899999,12.2,1.33446837399998));
#192417=CARTESIAN_POINT('Ctrl Pts',(10.3023432839999,12.2,1.33443898699999));
#192418=CARTESIAN_POINT('Ctrl Pts',(10.3013188639999,12.2,1.33440884399999));
#192419=CARTESIAN_POINT('Ctrl Pts',(10.3003037569999,12.2,1.33437796599999));
#192420=CARTESIAN_POINT('Ctrl Pts',(10.2992979849999,12.2,1.33434636899999));
#192421=CARTESIAN_POINT('Ctrl Pts',(10.2983015759999,12.2,1.33431407099998));
#192422=CARTESIAN_POINT('Ctrl Pts',(10.2973145539999,12.2,1.33428109299999));
#192423=CARTESIAN_POINT('Ctrl Pts',(10.2963369469999,12.2,1.33424745299998));
#192424=CARTESIAN_POINT('Ctrl Pts',(10.2953687779999,12.2,1.33421316799998));
#192425=CARTESIAN_POINT('Ctrl Pts',(10.2944100739999,12.2,1.33417825799999));
#192426=CARTESIAN_POINT('Ctrl Pts',(10.2934608629999,12.2,1.33414274199998));
#192427=CARTESIAN_POINT('Ctrl Pts',(10.2925211679999,12.2,1.33410663999999));
#192428=CARTESIAN_POINT('Ctrl Pts',(10.2915910169999,12.2,1.33406996999998));
#192429=CARTESIAN_POINT('Ctrl Pts',(10.2906757369999,12.2,1.33403296599999));
#192430=CARTESIAN_POINT('Ctrl Pts',(10.2899521419999,12.2,1.33400298799998));
#192431=CARTESIAN_POINT('Ctrl Pts',(10.2894150039999,12.2,1.33398033399999));
#192432=CARTESIAN_POINT('Ctrl Pts',(10.2890605199999,12.2,1.33396520799999));
#192433=CARTESIAN_POINT('Ctrl Pts',(10.2888863229999,12.2,1.33395773199998));
#192434=CARTESIAN_POINT('Ctrl Pts',(10.2888863229999,15.2,1.33395773199998));
#192435=CARTESIAN_POINT('Ctrl Pts',(10.2890605199999,15.2,1.33396520799999));
#192436=CARTESIAN_POINT('Ctrl Pts',(10.2894150039999,15.2,1.33398033399999));
#192437=CARTESIAN_POINT('Ctrl Pts',(10.2899521419999,15.2,1.33400298799998));
#192438=CARTESIAN_POINT('Ctrl Pts',(10.2906757369999,15.2,1.33403296599999));
#192439=CARTESIAN_POINT('Ctrl Pts',(10.2915910169999,15.2,1.33406996999998));
#192440=CARTESIAN_POINT('Ctrl Pts',(10.2925211679999,15.2,1.33410663999999));
#192441=CARTESIAN_POINT('Ctrl Pts',(10.2934608629999,15.2,1.33414274199998));
#192442=CARTESIAN_POINT('Ctrl Pts',(10.2944100739999,15.2,1.33417825799999));
#192443=CARTESIAN_POINT('Ctrl Pts',(10.2953687779999,15.2,1.33421316799998));
#192444=CARTESIAN_POINT('Ctrl Pts',(10.2963369469999,15.2,1.33424745299998));
#192445=CARTESIAN_POINT('Ctrl Pts',(10.2973145539999,15.2,1.33428109299999));
#192446=CARTESIAN_POINT('Ctrl Pts',(10.2983015759999,15.2,1.33431407099998));
#192447=CARTESIAN_POINT('Ctrl Pts',(10.2992979849999,15.2,1.33434636899999));
#192448=CARTESIAN_POINT('Ctrl Pts',(10.3003037569999,15.2,1.33437796599999));
#192449=CARTESIAN_POINT('Ctrl Pts',(10.3013188639999,15.2,1.33440884399999));
#192450=CARTESIAN_POINT('Ctrl Pts',(10.3023432839999,15.2,1.33443898699999));
#192451=CARTESIAN_POINT('Ctrl Pts',(10.3033769899999,15.2,1.33446837399998));
#192452=CARTESIAN_POINT('Ctrl Pts',(10.3044199559999,15.2,1.33449698899998));
#192453=CARTESIAN_POINT('Ctrl Pts',(10.3054721599999,15.2,1.33452481299999));
#192454=CARTESIAN_POINT('Ctrl Pts',(10.3065335739999,15.2,1.33455182699999));
#192455=CARTESIAN_POINT('Ctrl Pts',(10.3076041749999,15.2,1.33457801399999));
#192456=CARTESIAN_POINT('Ctrl Pts',(10.3086839379999,15.2,1.33460335699999));
#192457=CARTESIAN_POINT('Ctrl Pts',(10.3097728379999,15.2,1.33462783699999));
#192458=CARTESIAN_POINT('Ctrl Pts',(10.3108708509999,15.2,1.33465143799999));
#192459=CARTESIAN_POINT('Ctrl Pts',(10.3119779519999,15.2,1.33467414199998));
#192460=CARTESIAN_POINT('Ctrl Pts',(10.3130941179999,15.2,1.33469593099999));
#192461=CARTESIAN_POINT('Ctrl Pts',(10.3142193239999,15.2,1.33471678699999));
#192462=CARTESIAN_POINT('Ctrl Pts',(10.3153535459999,15.2,1.33473669599999));
#192463=CARTESIAN_POINT('Ctrl Pts',(10.3164967599999,15.2,1.33475563599998));
#192464=CARTESIAN_POINT('Ctrl Pts',(10.3176489429999,15.2,1.33477359499999));
#192465=CARTESIAN_POINT('Ctrl Pts',(10.3188100709999,15.2,1.33479055299999));
#192466=CARTESIAN_POINT('Ctrl Pts',(10.3199801189999,15.2,1.33480649299999));
#192467=CARTESIAN_POINT('Ctrl Pts',(10.3211590649999,15.2,1.33482139999999));
#192468=CARTESIAN_POINT('Ctrl Pts',(10.3223468859999,15.2,1.33483525699999));
#192469=CARTESIAN_POINT('Ctrl Pts',(10.3235435579999,15.2,1.33484804699998));
#192470=CARTESIAN_POINT('Ctrl Pts',(10.3247490569999,15.2,1.33485975299998));
#192471=CARTESIAN_POINT('Ctrl Pts',(10.3259633609999,15.2,1.33487035899998));
#192472=CARTESIAN_POINT('Ctrl Pts',(10.3271864459999,15.2,1.33487984899999));
#192473=CARTESIAN_POINT('Ctrl Pts',(10.3284182899999,15.2,1.33488820699998));
#192474=CARTESIAN_POINT('Ctrl Pts',(10.3296588699999,15.2,1.33489541599999));
#192475=CARTESIAN_POINT('Ctrl Pts',(10.3309081639999,15.2,1.33490145999998));
#192476=CARTESIAN_POINT('Ctrl Pts',(10.3321661469999,15.2,1.33490632399999));
#192477=CARTESIAN_POINT('Ctrl Pts',(10.3334327989999,15.2,1.33490999099998));
#192478=CARTESIAN_POINT('Ctrl Pts',(10.3347080959999,15.2,1.33491244599998));
#192479=CARTESIAN_POINT('Ctrl Pts',(10.3359920159999,15.2,1.33491367299999));
#192480=CARTESIAN_POINT('Ctrl Pts',(10.3372845369999,15.2,1.33491365699999));
#192481=CARTESIAN_POINT('Ctrl Pts',(10.3385856379999,15.2,1.33491238099999));
#192482=CARTESIAN_POINT('Ctrl Pts',(10.3398952939999,15.2,1.33490982999998));
#192483=CARTESIAN_POINT('Ctrl Pts',(10.3412134849999,15.2,1.33490598999999));
#192484=CARTESIAN_POINT('Ctrl Pts',(10.3425401889999,15.2,1.33490084399998));
#192485=CARTESIAN_POINT('Ctrl Pts',(10.3438753839999,15.2,1.33489437599998));
#192486=CARTESIAN_POINT('Ctrl Pts',(10.3452190479999,15.2,1.33488657399999));
#192487=CARTESIAN_POINT('Ctrl Pts',(10.3465711599999,15.2,1.33487741899998));
#192488=CARTESIAN_POINT('Ctrl Pts',(10.3479316969999,15.2,1.33486689999998));
#192489=CARTESIAN_POINT('Ctrl Pts',(10.3493006389999,15.2,1.33485499899999));
#192490=CARTESIAN_POINT('Ctrl Pts',(10.3506779649999,15.2,1.33484170199999));
#192491=CARTESIAN_POINT('Ctrl Pts',(10.3520636509999,15.2,1.33482699499998));
#192492=CARTESIAN_POINT('Ctrl Pts',(10.3534576789999,15.2,1.33481086299998));
#192493=CARTESIAN_POINT('Ctrl Pts',(10.3548600249999,15.2,1.33479328899998));
#192494=CARTESIAN_POINT('Ctrl Pts',(10.3562706699999,15.2,1.33477426199998));
#192495=CARTESIAN_POINT('Ctrl Pts',(10.3576895929999,15.2,1.33475376599999));
#192496=CARTESIAN_POINT('Ctrl Pts',(10.3591167719999,15.2,1.33473178499999));
#192497=CARTESIAN_POINT('Ctrl Pts',(10.3605521859999,15.2,1.33470830799999));
#192498=CARTESIAN_POINT('Ctrl Pts',(10.3619958159999,15.2,1.33468331699999));
#192499=CARTESIAN_POINT('Ctrl Pts',(10.3634476389999,15.2,1.33465680099999));
#192500=CARTESIAN_POINT('Ctrl Pts',(10.3649076359999,15.2,1.33462874399998));
#192501=CARTESIAN_POINT('Ctrl Pts',(10.3663757859999,15.2,1.33459913299999));
#192502=CARTESIAN_POINT('Ctrl Pts',(10.3678520689999,15.2,1.33456795199999));
#192503=CARTESIAN_POINT('Ctrl Pts',(10.3693364639999,15.2,1.33453518899998));
#192504=CARTESIAN_POINT('Ctrl Pts',(10.3708289509999,15.2,1.33450082899999));
#192505=CARTESIAN_POINT('Ctrl Pts',(10.3723295099999,15.2,1.33446485899999));
#192506=CARTESIAN_POINT('Ctrl Pts',(10.3738381209999,15.2,1.33442726599998));
#192507=CARTESIAN_POINT('Ctrl Pts',(10.3753547629999,15.2,1.33438803399998));
#192508=CARTESIAN_POINT('Ctrl Pts',(10.3768794159999,15.2,1.33434714999999));
#192509=CARTESIAN_POINT('Ctrl Pts',(10.3784120619999,15.2,1.33430460199999));
#192510=CARTESIAN_POINT('Ctrl Pts',(10.3799526789999,15.2,1.33426037599999));
#192511=CARTESIAN_POINT('Ctrl Pts',(10.3815012489999,15.2,1.33421445799998));
#192512=CARTESIAN_POINT('Ctrl Pts',(10.3830577499999,15.2,1.33416683399998));
#192513=CARTESIAN_POINT('Ctrl Pts',(10.3846221649999,15.2,1.33411749199999));
#192514=CARTESIAN_POINT('Ctrl Pts',(10.3861944729999,15.2,1.33406641899999));
#192515=CARTESIAN_POINT('Ctrl Pts',(10.3877746539999,15.2,1.33401360099999));
#192516=CARTESIAN_POINT('Ctrl Pts',(10.3893626899999,15.2,1.33395902399998));
#192517=CARTESIAN_POINT('Ctrl Pts',(10.3909585599999,15.2,1.33390267699999));
#192518=CARTESIAN_POINT('Ctrl Pts',(10.3925622469999,15.2,1.33384454499998));
#192519=CARTESIAN_POINT('Ctrl Pts',(10.3941737289999,15.2,1.33378461799999));
#192520=CARTESIAN_POINT('Ctrl Pts',(10.3957929889999,15.2,1.33372287999999));
#192521=CARTESIAN_POINT('Ctrl Pts',(10.3974200079999,15.2,1.33365931999998));
#192522=CARTESIAN_POINT('Ctrl Pts',(10.3990547659999,15.2,1.33359392399999));
#192523=CARTESIAN_POINT('Ctrl Pts',(10.4006972429999,15.2,1.33352668099999));
#192524=CARTESIAN_POINT('Ctrl Pts',(10.4023474229999,15.2,1.33345757799999));
#192525=CARTESIAN_POINT('Ctrl Pts',(10.4040052849999,15.2,1.33338659999998));
#192526=CARTESIAN_POINT('Ctrl Pts',(10.4056708099999,15.2,1.33331373699999));
#192527=CARTESIAN_POINT('Ctrl Pts',(10.4073439809999,15.2,1.33323897699999));
#192528=CARTESIAN_POINT('Ctrl Pts',(10.4090247779999,15.2,1.33316230699998));
#192529=CARTESIAN_POINT('Ctrl Pts',(10.4107131829999,15.2,1.33308371299998));
#192530=CARTESIAN_POINT('Ctrl Pts',(10.4124091789999,15.2,1.33300318499999));
#192531=CARTESIAN_POINT('Ctrl Pts',(10.4141127429999,15.2,1.33292070899998));
#192532=CARTESIAN_POINT('Ctrl Pts',(10.4158238619999,15.2,1.33283627399999));
#192533=CARTESIAN_POINT('Ctrl Pts',(10.4175425149999,15.2,1.33274986699998));
#192534=CARTESIAN_POINT('Ctrl Pts',(10.4192686839999,15.2,1.33266147799999));
#192535=CARTESIAN_POINT('Ctrl Pts',(10.4210023509999,15.2,1.33257109199999));
#192536=CARTESIAN_POINT('Ctrl Pts',(10.4227434979999,15.2,1.33247869999999));
#192537=CARTESIAN_POINT('Ctrl Pts',(10.4244921049999,15.2,1.33238428799999));
#192538=CARTESIAN_POINT('Ctrl Pts',(10.4262481579999,15.2,1.33228784499998));
#192539=CARTESIAN_POINT('Ctrl Pts',(10.4280116349999,15.2,1.33218935899999));
#192540=CARTESIAN_POINT('Ctrl Pts',(10.4297825219999,15.2,1.33208881899999));
#192541=CARTESIAN_POINT('Ctrl Pts',(10.4315607969999,15.2,1.33198621299998));
#192542=CARTESIAN_POINT('Ctrl Pts',(10.4333464449999,15.2,1.33188152799999));
#192543=CARTESIAN_POINT('Ctrl Pts',(10.4351394479999,15.2,1.33177475499998));
#192544=CARTESIAN_POINT('Ctrl Pts',(10.4369397879999,15.2,1.33166588099999));
#192545=CARTESIAN_POINT('Ctrl Pts',(10.4387474469999,15.2,1.33155489399998));
#192546=CARTESIAN_POINT('Ctrl Pts',(10.4405624069999,15.2,1.33144178399998));
#192547=CARTESIAN_POINT('Ctrl Pts',(10.4423846519999,15.2,1.33132653899999));
#192548=CARTESIAN_POINT('Ctrl Pts',(10.4442141639999,15.2,1.33120914799999));
#192549=CARTESIAN_POINT('Ctrl Pts',(10.4460509249999,15.2,1.33108959799999));
#192550=CARTESIAN_POINT('Ctrl Pts',(10.4478949189999,15.2,1.33096787999999));
#192551=CARTESIAN_POINT('Ctrl Pts',(10.4497461279999,15.2,1.33084398299999));
#192552=CARTESIAN_POINT('Ctrl Pts',(10.4516045329999,15.2,1.33071789399999));
#192553=CARTESIAN_POINT('Ctrl Pts',(10.4534701199999,15.2,1.33058960299998));
#192554=CARTESIAN_POINT('Ctrl Pts',(10.4553428709999,15.2,1.33045909899999));
#192555=CARTESIAN_POINT('Ctrl Pts',(10.4572227669999,15.2,1.33032637099999));
#192556=CARTESIAN_POINT('Ctrl Pts',(10.4591097919999,15.2,1.33019140799998));
#192557=CARTESIAN_POINT('Ctrl Pts',(10.4610039309999,15.2,1.33005419999999));
#192558=CARTESIAN_POINT('Ctrl Pts',(10.4629051649999,15.2,1.32991473599999));
#192559=CARTESIAN_POINT('Ctrl Pts',(10.4648134769999,15.2,1.32977300399999));
#192560=CARTESIAN_POINT('Ctrl Pts',(10.4667288519999,15.2,1.32962899399999));
#192561=CARTESIAN_POINT('Ctrl Pts',(10.4686512709999,15.2,1.32948269499999));
#192562=CARTESIAN_POINT('Ctrl Pts',(10.4705807189999,15.2,1.32933409699998));
#192563=CARTESIAN_POINT('Ctrl Pts',(10.4725171799999,15.2,1.32918318999999));
#192564=CARTESIAN_POINT('Ctrl Pts',(10.4744606349999,15.2,1.32902996199999));
#192565=CARTESIAN_POINT('Ctrl Pts',(10.4764110689999,15.2,1.32887440299998));
#192566=CARTESIAN_POINT('Ctrl Pts',(10.4783684649999,15.2,1.32871650399998));
#192567=CARTESIAN_POINT('Ctrl Pts',(10.4803328079999,15.2,1.32855625199999));
#192568=CARTESIAN_POINT('Ctrl Pts',(10.4823040789999,15.2,1.32839363899999));
#192569=CARTESIAN_POINT('Ctrl Pts',(10.4842822649999,15.2,1.32822865399998));
#192570=CARTESIAN_POINT('Ctrl Pts',(10.4862673459999,15.2,1.32806128699999));
#192571=CARTESIAN_POINT('Ctrl Pts',(10.4882593079999,15.2,1.32789152599999));
#192572=CARTESIAN_POINT('Ctrl Pts',(10.4902581349999,15.2,1.32771936199998));
#192573=CARTESIAN_POINT('Ctrl Pts',(10.4922638099999,15.2,1.32754478599999));
#192574=CARTESIAN_POINT('Ctrl Pts',(10.4942763159999,15.2,1.32736778799998));
#192575=CARTESIAN_POINT('Ctrl Pts',(10.4962956399999,15.2,1.32718835599999));
#192576=CARTESIAN_POINT('Ctrl Pts',(10.4983217629999,15.2,1.32700648099998));
#192577=CARTESIAN_POINT('Ctrl Pts',(10.5003546709999,15.2,1.32682215399999));
#192578=CARTESIAN_POINT('Ctrl Pts',(10.5023943459999,15.2,1.32663536299999));
#192579=CARTESIAN_POINT('Ctrl Pts',(10.5044407749999,15.2,1.32644610099999));
#192580=CARTESIAN_POINT('Ctrl Pts',(10.5064939389999,15.2,1.32625435499999));
#192581=CARTESIAN_POINT('Ctrl Pts',(10.5085538239999,15.2,1.32606011699998));
#192582=CARTESIAN_POINT('Ctrl Pts',(10.5106204149999,15.2,1.32586337799999));
#192583=CARTESIAN_POINT('Ctrl Pts',(10.5126936939999,15.2,1.32566412699999));
#192584=CARTESIAN_POINT('Ctrl Pts',(10.5147736479999,15.2,1.32546235499999));
#192585=CARTESIAN_POINT('Ctrl Pts',(10.5168602599999,15.2,1.32525805099998));
#192586=CARTESIAN_POINT('Ctrl Pts',(10.5189535149999,15.2,1.32505120799999));
#192587=CARTESIAN_POINT('Ctrl Pts',(10.5210533959999,15.2,1.32484181499999));
#192588=CARTESIAN_POINT('Ctrl Pts',(10.5231598899999,15.2,1.32462986199998));
#192589=CARTESIAN_POINT('Ctrl Pts',(10.5252729789999,15.2,1.32441534099998));
#192590=CARTESIAN_POINT('Ctrl Pts',(10.5273926489999,15.2,1.32419824099999));
#192591=CARTESIAN_POINT('Ctrl Pts',(10.5295188859999,15.2,1.32397855399998));
#192592=CARTESIAN_POINT('Ctrl Pts',(10.5316516719999,15.2,1.32375626999998));
#192593=CARTESIAN_POINT('Ctrl Pts',(10.5337909929999,15.2,1.32353137899999));
#192594=CARTESIAN_POINT('Ctrl Pts',(10.5359368329999,15.2,1.32330387399998));
#192595=CARTESIAN_POINT('Ctrl Pts',(10.5380891789999,15.2,1.32307374399999));
#192596=CARTESIAN_POINT('Ctrl Pts',(10.5402480139999,15.2,1.32284097999999));
#192597=CARTESIAN_POINT('Ctrl Pts',(10.5424133229999,15.2,1.32260557299999));
#192598=CARTESIAN_POINT('Ctrl Pts',(10.5445850929999,15.2,1.32236751399998));
#192599=CARTESIAN_POINT('Ctrl Pts',(10.5467633059999,15.2,1.32212679499998));
#192600=CARTESIAN_POINT('Ctrl Pts',(10.5489479479999,15.2,1.32188340599999));
#192601=CARTESIAN_POINT('Ctrl Pts',(10.5511390059999,15.2,1.32163733699999));
#192602=CARTESIAN_POINT('Ctrl Pts',(10.5533364629999,15.2,1.32138857999998));
#192603=CARTESIAN_POINT('Ctrl Pts',(10.5555403039999,15.2,1.32113712699998));
#192604=CARTESIAN_POINT('Ctrl Pts',(10.5577505169999,15.2,1.32088296799999));
#192605=CARTESIAN_POINT('Ctrl Pts',(10.5599670829999,15.2,1.32062609399998));
#192606=CARTESIAN_POINT('Ctrl Pts',(10.5621899909999,15.2,1.32036649799999));
#192607=CARTESIAN_POINT('Ctrl Pts',(10.5644192249999,15.2,1.32010417099998));
#192608=CARTESIAN_POINT('Ctrl Pts',(10.5666547689999,15.2,1.31983910099999));
#192609=CARTESIAN_POINT('Ctrl Pts',(10.5688966099999,15.2,1.31957128299999));
#192610=CARTESIAN_POINT('Ctrl Pts',(10.5711447329999,15.2,1.31930070599998));
#192611=CARTESIAN_POINT('Ctrl Pts',(10.5733991249999,15.2,1.31902736299998));
#192612=CARTESIAN_POINT('Ctrl Pts',(10.5756597679999,15.2,1.31875124499999));
#192613=CARTESIAN_POINT('Ctrl Pts',(10.5779266509999,15.2,1.31847234299999));
#192614=CARTESIAN_POINT('Ctrl Pts',(10.5801997579999,15.2,1.31819064899998));
#192615=CARTESIAN_POINT('Ctrl Pts',(10.5824790749999,15.2,1.31790615499999));
#192616=CARTESIAN_POINT('Ctrl Pts',(10.5852216883494,15.2,1.3175613901812));
#192617=CARTESIAN_POINT('Ctrl Pts',(10.5879735759502,15.2,1.31721239989353));
#192618=CARTESIAN_POINT('Ctrl Pts',(10.5907347060497,15.2,1.31685916610644));
#192619=CARTESIAN_POINT('Ctrl Pts',(10.5935050499004,15.2,1.31650167378707));
#192620=CARTESIAN_POINT('Ctrl Pts',(10.5962845809999,15.2,1.31613990499998));
#192621=CARTESIAN_POINT('Ctrl Pts',(10.5986069669999,15.2,1.31583557099999));
#192622=CARTESIAN_POINT('Ctrl Pts',(10.6009354489999,15.2,1.31552837099999));
#192623=CARTESIAN_POINT('Ctrl Pts',(10.6032700129999,15.2,1.31521829699999));
#192624=CARTESIAN_POINT('Ctrl Pts',(10.6056106459999,15.2,1.31490533699999));
#192625=CARTESIAN_POINT('Ctrl Pts',(10.6079573329999,15.2,1.31458948699999));
#192626=CARTESIAN_POINT('Ctrl Pts',(10.6103100589999,15.2,1.31427073799999));
#192627=CARTESIAN_POINT('Ctrl Pts',(10.6126688119999,15.2,1.31394908099999));
#192628=CARTESIAN_POINT('Ctrl Pts',(10.6150335779999,15.2,1.31362450999998));
#192629=CARTESIAN_POINT('Ctrl Pts',(10.6174043419999,15.2,1.31329701299999));
#192630=CARTESIAN_POINT('Ctrl Pts',(10.6197810909999,15.2,1.31296658599998));
#192631=CARTESIAN_POINT('Ctrl Pts',(10.6221638119999,15.2,1.31263321999999));
#192632=CARTESIAN_POINT('Ctrl Pts',(10.6245524889999,15.2,1.31229690699998));
#192633=CARTESIAN_POINT('Ctrl Pts',(10.6269471099999,15.2,1.31195763899999));
#192634=CARTESIAN_POINT('Ctrl Pts',(10.6293476599999,15.2,1.31161540699999));
#192635=CARTESIAN_POINT('Ctrl Pts',(10.6317541279999,15.2,1.31127020699998));
#192636=CARTESIAN_POINT('Ctrl Pts',(10.6341664979999,15.2,1.31092202699998));
#192637=CARTESIAN_POINT('Ctrl Pts',(10.6365847569999,15.2,1.31057086099998));
#192638=CARTESIAN_POINT('Ctrl Pts',(10.6390088909999,15.2,1.31021670299999));
#192639=CARTESIAN_POINT('Ctrl Pts',(10.6414388879999,15.2,1.30985954199998));
#192640=CARTESIAN_POINT('Ctrl Pts',(10.6438747329999,15.2,1.30949937399999));
#192641=CARTESIAN_POINT('Ctrl Pts',(10.6463164129999,15.2,1.30913618899998));
#192642=CARTESIAN_POINT('Ctrl Pts',(10.6487639159999,15.2,1.30876997899998));
#192643=CARTESIAN_POINT('Ctrl Pts',(10.6512172259999,15.2,1.30840073799999));
#192644=CARTESIAN_POINT('Ctrl Pts',(10.6536763329999,15.2,1.30802845899999));
#192645=CARTESIAN_POINT('Ctrl Pts',(10.6561412199999,15.2,1.30765313299999));
#192646=CARTESIAN_POINT('Ctrl Pts',(10.6586118759999,15.2,1.30727475299999));
#192647=CARTESIAN_POINT('Ctrl Pts',(10.6610882879999,15.2,1.30689331299998));
#192648=CARTESIAN_POINT('Ctrl Pts',(10.6635704409999,15.2,1.30650880399998));
#192649=CARTESIAN_POINT('Ctrl Pts',(10.6660583229999,15.2,1.30612121799999));
#192650=CARTESIAN_POINT('Ctrl Pts',(10.6685519209999,15.2,1.30573054999998));
#192651=CARTESIAN_POINT('Ctrl Pts',(10.6710512209999,15.2,1.30533679099999));
#192652=CARTESIAN_POINT('Ctrl Pts',(10.6735562119999,15.2,1.30493993399998));
#192653=CARTESIAN_POINT('Ctrl Pts',(10.6760668779999,15.2,1.30453997299998));
#192654=CARTESIAN_POINT('Ctrl Pts',(10.6785832079999,15.2,1.30413689899999));
#192655=CARTESIAN_POINT('Ctrl Pts',(10.6811051889999,15.2,1.30373070699998));
#192656=CARTESIAN_POINT('Ctrl Pts',(10.6836328059999,15.2,1.30332138799998));
#192657=CARTESIAN_POINT('Ctrl Pts',(10.6861660479999,15.2,1.30290893499998));
#192658=CARTESIAN_POINT('Ctrl Pts',(10.6887049019999,15.2,1.30249334199998));
#192659=CARTESIAN_POINT('Ctrl Pts',(10.6912493539999,15.2,1.30207460099999));
#192660=CARTESIAN_POINT('Ctrl Pts',(10.6937993929999,15.2,1.30165270599999));
#192661=CARTESIAN_POINT('Ctrl Pts',(10.6963550049999,15.2,1.30122764799999));
#192662=CARTESIAN_POINT('Ctrl Pts',(10.6989161759999,15.2,1.30079942299998));
#192663=CARTESIAN_POINT('Ctrl Pts',(10.7014828959999,15.2,1.30036802199998));
#192664=CARTESIAN_POINT('Ctrl Pts',(10.7040551489999,15.2,1.29993343899999));
#192665=CARTESIAN_POINT('Ctrl Pts',(10.7066329249999,15.2,1.29949566599999));
#192666=CARTESIAN_POINT('Ctrl Pts',(10.7092162099999,15.2,1.29905469699999));
#192667=CARTESIAN_POINT('Ctrl Pts',(10.7118049929999,15.2,1.29861052499999));
#192668=CARTESIAN_POINT('Ctrl Pts',(10.7143992589999,15.2,1.29816314299998));
#192669=CARTESIAN_POINT('Ctrl Pts',(10.7169989959999,15.2,1.29771254499999));
#192670=CARTESIAN_POINT('Ctrl Pts',(10.7196041929999,15.2,1.29725872299999));
#192671=CARTESIAN_POINT('Ctrl Pts',(10.7222148359999,15.2,1.29680166999998));
#192672=CARTESIAN_POINT('Ctrl Pts',(10.7248309119999,15.2,1.29634138299998));
#192673=CARTESIAN_POINT('Ctrl Pts',(10.7274524109999,15.2,1.29587785099998));
#192674=CARTESIAN_POINT('Ctrl Pts',(10.7300793179999,15.2,1.29541106899998));
#192675=CARTESIAN_POINT('Ctrl Pts',(10.7327116219999,15.2,1.29494102999999));
#192676=CARTESIAN_POINT('Ctrl Pts',(10.7353493089999,15.2,1.29446772899998));
#192677=CARTESIAN_POINT('Ctrl Pts',(10.7379923689999,15.2,1.29399115799998));
#192678=CARTESIAN_POINT('Ctrl Pts',(10.7406407879999,15.2,1.29351130999999));
#192679=CARTESIAN_POINT('Ctrl Pts',(10.7432945539999,15.2,1.29302817899998));
#192680=CARTESIAN_POINT('Ctrl Pts',(10.7459536549999,15.2,1.29254175999999));
#192681=CARTESIAN_POINT('Ctrl Pts',(10.7486180789999,15.2,1.29205204399998));
#192682=CARTESIAN_POINT('Ctrl Pts',(10.7512878129999,15.2,1.29155902599999));
#192683=CARTESIAN_POINT('Ctrl Pts',(10.7539628449999,15.2,1.29106269999999));
#192684=CARTESIAN_POINT('Ctrl Pts',(10.7566431619999,15.2,1.29056305799998));
#192685=CARTESIAN_POINT('Ctrl Pts',(10.7593287539999,15.2,1.29006009499999));
#192686=CARTESIAN_POINT('Ctrl Pts',(10.7620196059999,15.2,1.28955380499999));
#192687=CARTESIAN_POINT('Ctrl Pts',(10.7647157089999,15.2,1.28904418099999));
#192688=CARTESIAN_POINT('Ctrl Pts',(10.7674170489999,15.2,1.28853121599999));
#192689=CARTESIAN_POINT('Ctrl Pts',(10.7701236149999,15.2,1.28801490499999));
#192690=CARTESIAN_POINT('Ctrl Pts',(10.7728353919999,15.2,1.28749524099999));
#192691=CARTESIAN_POINT('Ctrl Pts',(10.7755523729999,15.2,1.28697221799999));
#192692=CARTESIAN_POINT('Ctrl Pts',(10.7782745419999,15.2,1.28644583099998));
#192693=CARTESIAN_POINT('Ctrl Pts',(10.7810018879999,15.2,1.28591607099999));
#192694=CARTESIAN_POINT('Ctrl Pts',(10.7837344009999,15.2,1.28538293399998));
#192695=CARTESIAN_POINT('Ctrl Pts',(10.7864720659999,15.2,1.28484641299998));
#192696=CARTESIAN_POINT('Ctrl Pts',(10.7892148729999,15.2,1.28430650299999));
#192697=CARTESIAN_POINT('Ctrl Pts',(10.7919628099999,15.2,1.28376319699999));
#192698=CARTESIAN_POINT('Ctrl Pts',(10.7947158649999,15.2,1.28321648999998));
#192699=CARTESIAN_POINT('Ctrl Pts',(10.7974740259999,15.2,1.28266637499999));
#192700=CARTESIAN_POINT('Ctrl Pts',(10.8002372809999,15.2,1.28211284599999));
#192701=CARTESIAN_POINT('Ctrl Pts',(10.8030056189999,15.2,1.28155589599999));
#192702=CARTESIAN_POINT('Ctrl Pts',(10.8057790279999,15.2,1.28099552199998));
#192703=CARTESIAN_POINT('Ctrl Pts',(10.8085574969999,15.2,1.28043171599999));
#192704=CARTESIAN_POINT('Ctrl Pts',(10.8113410119999,15.2,1.27986447199998));
#192705=CARTESIAN_POINT('Ctrl Pts',(10.8141295629999,15.2,1.27929378499998));
#192706=CARTESIAN_POINT('Ctrl Pts',(10.8169231379999,15.2,1.27871964799999));
#192707=CARTESIAN_POINT('Ctrl Pts',(10.8197217269999,15.2,1.27814205699998));
#192708=CARTESIAN_POINT('Ctrl Pts',(10.8225253159999,15.2,1.27756100399999));
#192709=CARTESIAN_POINT('Ctrl Pts',(10.8253338939999,15.2,1.27697648499999));
#192710=CARTESIAN_POINT('Ctrl Pts',(10.8281474499999,15.2,1.27638849299998));
#192711=CARTESIAN_POINT('Ctrl Pts',(10.8309659719999,15.2,1.27579702399998));
#192712=CARTESIAN_POINT('Ctrl Pts',(10.8337894499999,15.2,1.27520206999999));
#192713=CARTESIAN_POINT('Ctrl Pts',(10.8366178699999,15.2,1.27460362699999));
#192714=CARTESIAN_POINT('Ctrl Pts',(10.8394512219999,15.2,1.27400168799999));
#192715=CARTESIAN_POINT('Ctrl Pts',(10.8422894959999,15.2,1.27339624799998));
#192716=CARTESIAN_POINT('Ctrl Pts',(10.8451326779999,15.2,1.27278730199999));
#192717=CARTESIAN_POINT('Ctrl Pts',(10.8479807569999,15.2,1.27217484299999));
#192718=CARTESIAN_POINT('Ctrl Pts',(10.8508337229999,15.2,1.27155886699999));
#192719=CARTESIAN_POINT('Ctrl Pts',(10.8536915629999,15.2,1.27093936699998));
#192720=CARTESIAN_POINT('Ctrl Pts',(10.8565542679999,15.2,1.27031633899998));
#192721=CARTESIAN_POINT('Ctrl Pts',(10.8594218239999,15.2,1.26968977599998));
#192722=CARTESIAN_POINT('Ctrl Pts',(10.8622942209999,15.2,1.26905967299999));
#192723=CARTESIAN_POINT('Ctrl Pts',(10.8651714489999,15.2,1.26842602399998));
#192724=CARTESIAN_POINT('Ctrl Pts',(10.8680534959999,15.2,1.26778882499998));
#192725=CARTESIAN_POINT('Ctrl Pts',(10.8709403489999,15.2,1.26714806999999));
#192726=CARTESIAN_POINT('Ctrl Pts',(10.8738319979999,15.2,1.26650375199999));
#192727=CARTESIAN_POINT('Ctrl Pts',(10.8767284329999,15.2,1.26585586799999));
#192728=CARTESIAN_POINT('Ctrl Pts',(10.8796296409999,15.2,1.26520441099998));
#192729=CARTESIAN_POINT('Ctrl Pts',(10.8825356119999,15.2,1.26454937599998));
#192730=CARTESIAN_POINT('Ctrl Pts',(10.8854463339999,15.2,1.26389075699999));
#192731=CARTESIAN_POINT('Ctrl Pts',(10.8883617979999,15.2,1.26322854999998));
#192732=CARTESIAN_POINT('Ctrl Pts',(10.8912819899999,15.2,1.26256274999998));
#192733=CARTESIAN_POINT('Ctrl Pts',(10.8942069009999,15.2,1.26189335099999));
#192734=CARTESIAN_POINT('Ctrl Pts',(10.8971365199999,15.2,1.26122034599998));
#192735=CARTESIAN_POINT('Ctrl Pts',(10.9000708339999,15.2,1.26054373299999));
#192736=CARTESIAN_POINT('Ctrl Pts',(10.9030098339999,15.2,1.25986350499999));
#192737=CARTESIAN_POINT('Ctrl Pts',(10.9059535079999,15.2,1.25917965599998));
#192738=CARTESIAN_POINT('Ctrl Pts',(10.9089018469999,15.2,1.25849218299999));
#192739=CARTESIAN_POINT('Ctrl Pts',(10.9118548369999,15.2,1.25780107899998));
#192740=CARTESIAN_POINT('Ctrl Pts',(10.9148124699999,15.2,1.25710633999998));
#192741=CARTESIAN_POINT('Ctrl Pts',(10.9177747329999,15.2,1.25640795999999));
#192742=CARTESIAN_POINT('Ctrl Pts',(10.9207416159999,15.2,1.25570593399999));
#192743=CARTESIAN_POINT('Ctrl Pts',(10.9237131089999,15.2,1.25500025699999));
#192744=CARTESIAN_POINT('Ctrl Pts',(10.9266891999999,15.2,1.25429092499999));
#192745=CARTESIAN_POINT('Ctrl Pts',(10.9296698779999,15.2,1.25357793199999));
#192746=CARTESIAN_POINT('Ctrl Pts',(10.9326551319999,15.2,1.25286127399999));
#192747=CARTESIAN_POINT('Ctrl Pts',(10.9356449539999,15.2,1.25214094399999));
#192748=CARTESIAN_POINT('Ctrl Pts',(10.9386393289999,15.2,1.25141693899999));
#192749=CARTESIAN_POINT('Ctrl Pts',(10.9416382509999,15.2,1.25068925199999));
#192750=CARTESIAN_POINT('Ctrl Pts',(10.9446417049999,15.2,1.24995787999998));
#192751=CARTESIAN_POINT('Ctrl Pts',(10.9476496829999,15.2,1.24922281699998));
#192752=CARTESIAN_POINT('Ctrl Pts',(10.9506621729999,15.2,1.24848405899999));
#192753=CARTESIAN_POINT('Ctrl Pts',(10.9536791659999,15.2,1.24774160099999));
#192754=CARTESIAN_POINT('Ctrl Pts',(10.9567006489999,15.2,1.24699543599998));
#192755=CARTESIAN_POINT('Ctrl Pts',(10.9597266129999,15.2,1.24624556199999));
#192756=CARTESIAN_POINT('Ctrl Pts',(10.9627570469999,15.2,1.24549197299999));
#192757=CARTESIAN_POINT('Ctrl Pts',(10.9657919419999,15.2,1.24473466399999));
#192758=CARTESIAN_POINT('Ctrl Pts',(10.9688312839999,15.2,1.24397363099999));
#192759=CARTESIAN_POINT('Ctrl Pts',(10.9718750649999,15.2,1.24320886799998));
#192760=CARTESIAN_POINT('Ctrl Pts',(10.9749232749999,15.2,1.24244037199999));
#192761=CARTESIAN_POINT('Ctrl Pts',(10.9779759009999,15.2,1.24166813599999));
#192762=CARTESIAN_POINT('Ctrl Pts',(10.9810329339999,15.2,1.24089215599998));
#192763=CARTESIAN_POINT('Ctrl Pts',(10.9840943639999,15.2,1.24011242999998));
#192764=CARTESIAN_POINT('Ctrl Pts',(10.9871601809999,15.2,1.23932894899998));
#192765=CARTESIAN_POINT('Ctrl Pts',(10.9902303719999,15.2,1.23854171099998));
#192766=CARTESIAN_POINT('Ctrl Pts',(10.9933049299999,15.2,1.23775071099999));
#192767=CARTESIAN_POINT('Ctrl Pts',(10.9963838419999,15.2,1.23695594399999));
#192768=CARTESIAN_POINT('Ctrl Pts',(10.9994670979999,15.2,1.23615740499998));
#192769=CARTESIAN_POINT('Ctrl Pts',(11.0025546899999,15.2,1.23535509099999));
#192770=CARTESIAN_POINT('Ctrl Pts',(11.0056466049999,15.2,1.23454899599999));
#192771=CARTESIAN_POINT('Ctrl Pts',(11.0087428319999,15.2,1.23373911599999));
#192772=CARTESIAN_POINT('Ctrl Pts',(11.0118433639999,15.2,1.23292544599999));
#192773=CARTESIAN_POINT('Ctrl Pts',(11.0149481889999,15.2,1.23210798199999));
#192774=CARTESIAN_POINT('Ctrl Pts',(11.0180572959999,15.2,1.23128671899998));
#192775=CARTESIAN_POINT('Ctrl Pts',(11.0211706759999,15.2,1.23046165299999));
#192776=CARTESIAN_POINT('Ctrl Pts',(11.0242883189999,15.2,1.22963277999999));
#192777=CARTESIAN_POINT('Ctrl Pts',(11.0274102129999,15.2,1.22880009299998));
#192778=CARTESIAN_POINT('Ctrl Pts',(11.0305363499999,15.2,1.22796359099999));
#192779=CARTESIAN_POINT('Ctrl Pts',(11.0336667189999,15.2,1.22712326699999));
#192780=CARTESIAN_POINT('Ctrl Pts',(11.0368013089999,15.2,1.22627911899999));
#192781=CARTESIAN_POINT('Ctrl Pts',(11.0399401109999,15.2,1.22543113999999));
#192782=CARTESIAN_POINT('Ctrl Pts',(11.0430831139999,15.2,1.22457932799998));
#192783=CARTESIAN_POINT('Ctrl Pts',(11.0462303079999,15.2,1.22372367599999));
#192784=CARTESIAN_POINT('Ctrl Pts',(11.0493816829999,15.2,1.22286418199999));
#192785=CARTESIAN_POINT('Ctrl Pts',(11.0525372299999,15.2,1.22200084099998));
#192786=CARTESIAN_POINT('Ctrl Pts',(11.0556969379999,15.2,1.22113364899999));
#192787=CARTESIAN_POINT('Ctrl Pts',(11.0588607969999,15.2,1.22026260099998));
#192788=CARTESIAN_POINT('Ctrl Pts',(11.0620287979999,15.2,1.21938769199998));
#192789=CARTESIAN_POINT('Ctrl Pts',(11.0652009289999,15.2,1.21850892099999));
#192790=CARTESIAN_POINT('Ctrl Pts',(11.0683771819999,15.2,1.21762627999999));
#192791=CARTESIAN_POINT('Ctrl Pts',(11.0715575449999,15.2,1.21673976599999));
#192792=CARTESIAN_POINT('Ctrl Pts',(11.0747420099999,15.2,1.21584937499998));
#192793=CARTESIAN_POINT('Ctrl Pts',(11.0779305669999,15.2,1.21495510399999));
#192794=CARTESIAN_POINT('Ctrl Pts',(11.0811232049999,15.2,1.21405694799999));
#192795=CARTESIAN_POINT('Ctrl Pts',(11.0843199139999,15.2,1.21315490199999));
#192796=CARTESIAN_POINT('Ctrl Pts',(11.0875206859999,15.2,1.21224896199998));
#192797=CARTESIAN_POINT('Ctrl Pts',(11.0907255089999,15.2,1.21133912599999));
#192798=CARTESIAN_POINT('Ctrl Pts',(11.0939343729999,15.2,1.21042538699998));
#192799=CARTESIAN_POINT('Ctrl Pts',(11.0971472699999,15.2,1.20950774199999));
#192800=CARTESIAN_POINT('Ctrl Pts',(11.1003641889999,15.2,1.20858618799998));
#192801=CARTESIAN_POINT('Ctrl Pts',(11.1035851209999,15.2,1.20766071999999));
#192802=CARTESIAN_POINT('Ctrl Pts',(11.1068100549999,15.2,1.20673133399999));
#192803=CARTESIAN_POINT('Ctrl Pts',(11.1100389819999,15.2,1.20579802499998));
#192804=CARTESIAN_POINT('Ctrl Pts',(11.1132718939999,15.2,1.20486079099999));
#192805=CARTESIAN_POINT('Ctrl Pts',(11.1165087779999,15.2,1.20391962699999));
#192806=CARTESIAN_POINT('Ctrl Pts',(11.1197496249999,15.2,1.20297452899999));
#192807=CARTESIAN_POINT('Ctrl Pts',(11.1229944269999,15.2,1.20202549299998));
#192808=CARTESIAN_POINT('Ctrl Pts',(11.1262431739999,15.2,1.20107251499999));
#192809=CARTESIAN_POINT('Ctrl Pts',(11.1294958549999,15.2,1.20011559099999));
#192810=CARTESIAN_POINT('Ctrl Pts',(11.1327524619999,15.2,1.19915471699999));
#192811=CARTESIAN_POINT('Ctrl Pts',(11.1360129839999,15.2,1.19818988999999));
#192812=CARTESIAN_POINT('Ctrl Pts',(11.1392774109999,15.2,1.19722110599998));
#192813=CARTESIAN_POINT('Ctrl Pts',(11.1425457349999,15.2,1.19624835999999));
#192814=CARTESIAN_POINT('Ctrl Pts',(11.1458179459999,15.2,1.19527164899999));
#192815=CARTESIAN_POINT('Ctrl Pts',(11.1490940329999,15.2,1.19429096899998));
#192816=CARTESIAN_POINT('Ctrl Pts',(11.1523739879999,15.2,1.19330631599999));
#192817=CARTESIAN_POINT('Ctrl Pts',(11.1556577999999,15.2,1.19231768599999));
#192818=CARTESIAN_POINT('Ctrl Pts',(11.1589454619999,15.2,1.19132507599998));
#192819=CARTESIAN_POINT('Ctrl Pts',(11.1622369629999,15.2,1.19032848099998));
#192820=CARTESIAN_POINT('Ctrl Pts',(11.1655322919999,15.2,1.18932789899999));
#192821=CARTESIAN_POINT('Ctrl Pts',(11.1688314409999,15.2,1.18832332399998));
#192822=CARTESIAN_POINT('Ctrl Pts',(11.1721344009999,15.2,1.18731475499999));
#192823=CARTESIAN_POINT('Ctrl Pts',(11.1754411629999,15.2,1.18630218499999));
#192824=CARTESIAN_POINT('Ctrl Pts',(11.1787517149999,15.2,1.18528561399998));
#192825=CARTESIAN_POINT('Ctrl Pts',(11.1820660499999,15.2,1.18426503499999));
#192826=CARTESIAN_POINT('Ctrl Pts',(11.1853841569999,15.2,1.18324044599999));
#192827=CARTESIAN_POINT('Ctrl Pts',(11.1887060269999,15.2,1.18221184299999));
#192828=CARTESIAN_POINT('Ctrl Pts',(11.1920316519999,15.2,1.18117922199998));
#192829=CARTESIAN_POINT('Ctrl Pts',(11.1953610209999,15.2,1.18014258099999));
#192830=CARTESIAN_POINT('Ctrl Pts',(11.1986941249999,15.2,1.17910191499998));
#192831=CARTESIAN_POINT('Ctrl Pts',(11.2020309559999,15.2,1.17805721999999));
#192832=CARTESIAN_POINT('Ctrl Pts',(11.2053715019999,15.2,1.17700849199998));
#192833=CARTESIAN_POINT('Ctrl Pts',(11.2087157559999,15.2,1.17595572999999));
#192834=CARTESIAN_POINT('Ctrl Pts',(11.2120637079999,15.2,1.17489892799998));
#192835=CARTESIAN_POINT('Ctrl Pts',(11.2154153489999,15.2,1.17383808299998));
#192836=CARTESIAN_POINT('Ctrl Pts',(11.2187706689999,15.2,1.17277319199999));
#192837=CARTESIAN_POINT('Ctrl Pts',(11.2221296589999,15.2,1.17170425099999));
#192838=CARTESIAN_POINT('Ctrl Pts',(11.2254923089999,15.2,1.17063125699998));
#192839=CARTESIAN_POINT('Ctrl Pts',(11.2288586119999,15.2,1.16955420599998));
#192840=CARTESIAN_POINT('Ctrl Pts',(11.2322285569999,15.2,1.16847309399999));
#192841=CARTESIAN_POINT('Ctrl Pts',(11.2356021349999,15.2,1.16738791999999));
#192842=CARTESIAN_POINT('Ctrl Pts',(11.2389793369999,15.2,1.16629867799999));
#192843=CARTESIAN_POINT('Ctrl Pts',(11.2423601539999,15.2,1.16520536499999));
#192844=CARTESIAN_POINT('Ctrl Pts',(11.2457445769999,15.2,1.16410797799999));
#192845=CARTESIAN_POINT('Ctrl Pts',(11.2491325969999,15.2,1.16300651299999));
#192846=CARTESIAN_POINT('Ctrl Pts',(11.2525242039999,15.2,1.16190096799999));
#192847=CARTESIAN_POINT('Ctrl Pts',(11.2559193889999,15.2,1.16079133899999));
#192848=CARTESIAN_POINT('Ctrl Pts',(11.2593181439999,15.2,1.15967762199999));
#192849=CARTESIAN_POINT('Ctrl Pts',(11.2627204589999,15.2,1.15855981299998));
#192850=CARTESIAN_POINT('Ctrl Pts',(11.2661263239999,15.2,1.15743791099999));
#192851=CARTESIAN_POINT('Ctrl Pts',(11.2695357319999,15.2,1.15631191099999));
#192852=CARTESIAN_POINT('Ctrl Pts',(11.2729486729999,15.2,1.15518180999999));
#192853=CARTESIAN_POINT('Ctrl Pts',(11.2763651379999,15.2,1.15404760499999));
#192854=CARTESIAN_POINT('Ctrl Pts',(11.2797851169999,15.2,1.15290929199999));
#192855=CARTESIAN_POINT('Ctrl Pts',(11.2832086039999,15.2,1.15176686799999));
#192856=CARTESIAN_POINT('Ctrl Pts',(11.2866355859999,15.2,1.15062032999999));
#192857=CARTESIAN_POINT('Ctrl Pts',(11.2900660559999,15.2,1.14946967499999));
#192858=CARTESIAN_POINT('Ctrl Pts',(11.2935000059999,15.2,1.14831489899998));
#192859=CARTESIAN_POINT('Ctrl Pts',(11.2969374249999,15.2,1.14715599999998));
#192860=CARTESIAN_POINT('Ctrl Pts',(11.3003783059999,15.2,1.14599297299999));
#192861=CARTESIAN_POINT('Ctrl Pts',(11.3038226389999,15.2,1.14482581599999));
#192862=CARTESIAN_POINT('Ctrl Pts',(11.3072704139999,15.2,1.14365452599999));
#192863=CARTESIAN_POINT('Ctrl Pts',(11.3107216239999,15.2,1.14247909899999));
#192864=CARTESIAN_POINT('Ctrl Pts',(11.3141762599999,15.2,1.14129953199999));
#192865=CARTESIAN_POINT('Ctrl Pts',(11.3176343119999,15.2,1.14011582299999));
#192866=CARTESIAN_POINT('Ctrl Pts',(11.3210957719999,15.2,1.13892796799998));
#192867=CARTESIAN_POINT('Ctrl Pts',(11.3245606299999,15.2,1.13773596199998));
#192868=CARTESIAN_POINT('Ctrl Pts',(11.3280288789999,15.2,1.13653980499999));
#192869=CARTESIAN_POINT('Ctrl Pts',(11.3315005099999,15.2,1.13533949399999));
#192870=CARTESIAN_POINT('Ctrl Pts',(11.3349755119999,15.2,1.13413502399998));
#192871=CARTESIAN_POINT('Ctrl Pts',(11.3384538779999,15.2,1.13292639099999));
#192872=CARTESIAN_POINT('Ctrl Pts',(11.3419355979999,15.2,1.13171359399999));
#192873=CARTESIAN_POINT('Ctrl Pts',(11.3454206639999,15.2,1.13049662999999));
#192874=CARTESIAN_POINT('Ctrl Pts',(11.3489090669999,15.2,1.12927549499998));
#192875=CARTESIAN_POINT('Ctrl Pts',(11.3524007989999,15.2,1.12805018499999));
#192876=CARTESIAN_POINT('Ctrl Pts',(11.3558958509999,15.2,1.12682069999999));
#192877=CARTESIAN_POINT('Ctrl Pts',(11.3593942139999,15.2,1.12558703499999));
#192878=CARTESIAN_POINT('Ctrl Pts',(11.3628958789999,15.2,1.12434918799998));
#192879=CARTESIAN_POINT('Ctrl Pts',(11.3664008399999,15.2,1.12310715499999));
#192880=CARTESIAN_POINT('Ctrl Pts',(11.3699090849999,15.2,1.12186093299998));
#192881=CARTESIAN_POINT('Ctrl Pts',(11.3734206059999,15.2,1.12061051999999));
#192882=CARTESIAN_POINT('Ctrl Pts',(11.3769353939999,15.2,1.11935591199999));
#192883=CARTESIAN_POINT('Ctrl Pts',(11.3804534399999,15.2,1.11809710599998));
#192884=CARTESIAN_POINT('Ctrl Pts',(11.3839747349999,15.2,1.11683410099999));
#192885=CARTESIAN_POINT('Ctrl Pts',(11.3874992709999,15.2,1.11556689099999));
#192886=CARTESIAN_POINT('Ctrl Pts',(11.3910270409999,15.2,1.11429547399998));
#192887=CARTESIAN_POINT('Ctrl Pts',(11.3945580339999,15.2,1.11301984899999));
#192888=CARTESIAN_POINT('Ctrl Pts',(11.3980922449999,15.2,1.11174001299998));
#192889=CARTESIAN_POINT('Ctrl Pts',(11.4016296639999,15.2,1.11045596299999));
#192890=CARTESIAN_POINT('Ctrl Pts',(11.4051702859999,15.2,1.10916769599998));
#192891=CARTESIAN_POINT('Ctrl Pts',(11.4087140989999,15.2,1.10787520999999));
#192892=CARTESIAN_POINT('Ctrl Pts',(11.4122610939999,15.2,1.10657849999999));
#192893=CARTESIAN_POINT('Ctrl Pts',(11.4158112619999,15.2,1.10527756499998));
#192894=CARTESIAN_POINT('Ctrl Pts',(11.4193645909999,15.2,1.10397239899998));
#192895=CARTESIAN_POINT('Ctrl Pts',(11.4229210689999,15.2,1.10266299899999));
#192896=CARTESIAN_POINT('Ctrl Pts',(11.4264806909999,15.2,1.10134936399998));
#192897=CARTESIAN_POINT('Ctrl Pts',(11.4300434449999,15.2,1.10003148899999));
#192898=CARTESIAN_POINT('Ctrl Pts',(11.4336093279999,15.2,1.09870937299998));
#192899=CARTESIAN_POINT('Ctrl Pts',(11.4371783349999,15.2,1.09738301699998));
#192900=CARTESIAN_POINT('Ctrl Pts',(11.4407504639999,15.2,1.09605241699999));
#192901=CARTESIAN_POINT('Ctrl Pts',(11.4436106639999,15.2,1.09498454299999));
#192902=CARTESIAN_POINT('Ctrl Pts',(11.4457572179999,15.2,1.09418172899999));
#192903=CARTESIAN_POINT('Ctrl Pts',(11.4471888789999,15.2,1.09364567099998));
#192904=CARTESIAN_POINT('Ctrl Pts',(11.4479048649999,15.2,1.09337742899998));
#192905=CARTESIAN_POINT('Ctrl Pts',(10.3708900239999,15.2,0.292001928999985));
#192906=CARTESIAN_POINT('Ctrl Pts',(10.3708900239999,11.6,0.292001928999985));
#192907=CARTESIAN_POINT('Ctrl Pts',(10.3710632449999,15.2,0.292021795999986));
#192908=CARTESIAN_POINT('Ctrl Pts',(10.3710632449999,11.6,0.292021795999986));
#192909=CARTESIAN_POINT('Ctrl Pts',(10.3714157299999,15.2,0.292062309999985));
#192910=CARTESIAN_POINT('Ctrl Pts',(10.3714157299999,11.6,0.292062309999985));
#192911=CARTESIAN_POINT('Ctrl Pts',(10.3719497989999,15.2,0.292123961999984));
#192912=CARTESIAN_POINT('Ctrl Pts',(10.3719497989999,11.6,0.292123961999983));
#192913=CARTESIAN_POINT('Ctrl Pts',(10.3726691759999,15.2,0.292207547999985));
#192914=CARTESIAN_POINT('Ctrl Pts',(10.3726691759999,11.6,0.292207547999985));
#192915=CARTESIAN_POINT('Ctrl Pts',(10.3735789749999,15.2,0.292314179999984));
#192916=CARTESIAN_POINT('Ctrl Pts',(10.3735789749999,11.6,0.292314179999984));
#192917=CARTESIAN_POINT('Ctrl Pts',(10.3745034109999,15.2,0.292423468999985));
#192918=CARTESIAN_POINT('Ctrl Pts',(10.3745034109999,11.6,0.292423468999985));
#192919=CARTESIAN_POINT('Ctrl Pts',(10.3754371839999,15.2,0.292534811999987));
#192920=CARTESIAN_POINT('Ctrl Pts',(10.3754371839999,11.6,0.292534811999987));
#192921=CARTESIAN_POINT('Ctrl Pts',(10.3763802659999,15.2,0.292648223999983));
#192922=CARTESIAN_POINT('Ctrl Pts',(10.3763802659999,11.6,0.292648223999982));
#192923=CARTESIAN_POINT('Ctrl Pts',(10.3773326269999,15.2,0.292763717999982));
#192924=CARTESIAN_POINT('Ctrl Pts',(10.3773326269999,11.6,0.292763717999982));
#192925=CARTESIAN_POINT('Ctrl Pts',(10.3782942399999,15.2,0.292881309999986));
#192926=CARTESIAN_POINT('Ctrl Pts',(10.3782942399999,11.6,0.292881309999986));
#192927=CARTESIAN_POINT('Ctrl Pts',(10.3792650739999,15.2,0.293001014999987));
#192928=CARTESIAN_POINT('Ctrl Pts',(10.3792650739999,11.6,0.293001014999987));
#192929=CARTESIAN_POINT('Ctrl Pts',(10.3802451029999,15.2,0.293122846999987));
#192930=CARTESIAN_POINT('Ctrl Pts',(10.3802451029999,11.6,0.293122846999986));
#192931=CARTESIAN_POINT('Ctrl Pts',(10.3812342959999,15.2,0.293246819999986));
#192932=CARTESIAN_POINT('Ctrl Pts',(10.3812342959999,11.6,0.293246819999986));
#192933=CARTESIAN_POINT('Ctrl Pts',(10.3822326279999,15.2,0.293372949999986));
#192934=CARTESIAN_POINT('Ctrl Pts',(10.3822326279999,11.6,0.293372949999986));
#192935=CARTESIAN_POINT('Ctrl Pts',(10.3832400689999,15.2,0.293501248999988));
#192936=CARTESIAN_POINT('Ctrl Pts',(10.3832400689999,11.6,0.293501248999987));
#192937=CARTESIAN_POINT('Ctrl Pts',(10.3842565909999,15.2,0.293631731999984));
#192938=CARTESIAN_POINT('Ctrl Pts',(10.3842565909999,11.6,0.293631731999983));
#192939=CARTESIAN_POINT('Ctrl Pts',(10.3852821679999,15.2,0.293764413999984));
#192940=CARTESIAN_POINT('Ctrl Pts',(10.3852821679999,11.6,0.293764413999984));
#192941=CARTESIAN_POINT('Ctrl Pts',(10.3863167709999,15.2,0.293899307999985));
#192942=CARTESIAN_POINT('Ctrl Pts',(10.3863167709999,11.6,0.293899307999985));
#192943=CARTESIAN_POINT('Ctrl Pts',(10.3873603719999,15.2,0.294036427999984));
#192944=CARTESIAN_POINT('Ctrl Pts',(10.3873603719999,11.6,0.294036427999984));
#192945=CARTESIAN_POINT('Ctrl Pts',(10.3884129439999,15.2,0.294175786999986));
#192946=CARTESIAN_POINT('Ctrl Pts',(10.3884129439999,11.6,0.294175786999986));
#192947=CARTESIAN_POINT('Ctrl Pts',(10.3894744609999,15.2,0.294317400999984));
#192948=CARTESIAN_POINT('Ctrl Pts',(10.3894744609999,11.6,0.294317400999983));
#192949=CARTESIAN_POINT('Ctrl Pts',(10.3905448939999,15.2,0.294461282999983));
#192950=CARTESIAN_POINT('Ctrl Pts',(10.3905448939999,11.6,0.294461282999982));
#192951=CARTESIAN_POINT('Ctrl Pts',(10.3916242179999,15.2,0.294607444999984));
#192952=CARTESIAN_POINT('Ctrl Pts',(10.3916242179999,11.6,0.294607444999983));
#192953=CARTESIAN_POINT('Ctrl Pts',(10.3927124039999,15.2,0.294755900999988));
#192954=CARTESIAN_POINT('Ctrl Pts',(10.3927124039999,11.6,0.294755900999987));
#192955=CARTESIAN_POINT('Ctrl Pts',(10.3938094269999,15.2,0.294906666999988));
#192956=CARTESIAN_POINT('Ctrl Pts',(10.3938094269999,11.6,0.294906666999987));
#192957=CARTESIAN_POINT('Ctrl Pts',(10.3949152589999,15.2,0.295059752999984));
#192958=CARTESIAN_POINT('Ctrl Pts',(10.3949152589999,11.6,0.295059752999984));
#192959=CARTESIAN_POINT('Ctrl Pts',(10.3960298749999,15.2,0.295215173999988));
#192960=CARTESIAN_POINT('Ctrl Pts',(10.3960298749999,11.6,0.295215173999987));
#192961=CARTESIAN_POINT('Ctrl Pts',(10.3971532469999,15.2,0.295372941999985));
#192962=CARTESIAN_POINT('Ctrl Pts',(10.3971532469999,11.6,0.295372941999985));
#192963=CARTESIAN_POINT('Ctrl Pts',(10.3982853499999,15.2,0.295533071999987));
#192964=CARTESIAN_POINT('Ctrl Pts',(10.3982853499999,11.6,0.295533071999987));
#192965=CARTESIAN_POINT('Ctrl Pts',(10.3994261559999,15.2,0.295695575999986));
#192966=CARTESIAN_POINT('Ctrl Pts',(10.3994261559999,11.6,0.295695575999985));
#192967=CARTESIAN_POINT('Ctrl Pts',(10.4005756419999,15.2,0.295860467999987));
#192968=CARTESIAN_POINT('Ctrl Pts',(10.4005756419999,11.6,0.295860467999986));
#192969=CARTESIAN_POINT('Ctrl Pts',(10.4017337789999,15.2,0.296027758999986));
#192970=CARTESIAN_POINT('Ctrl Pts',(10.4017337789999,11.6,0.296027758999986));
#192971=CARTESIAN_POINT('Ctrl Pts',(10.4029005419999,15.2,0.296197463999985));
#192972=CARTESIAN_POINT('Ctrl Pts',(10.4029005419999,11.6,0.296197463999985));
#192973=CARTESIAN_POINT('Ctrl Pts',(10.4040759059999,15.2,0.296369593999986));
#192974=CARTESIAN_POINT('Ctrl Pts',(10.4040759059999,11.6,0.296369593999985));
#192975=CARTESIAN_POINT('Ctrl Pts',(10.4052598449999,15.2,0.296544161999983));
#192976=CARTESIAN_POINT('Ctrl Pts',(10.4052598449999,11.6,0.296544161999983));
#192977=CARTESIAN_POINT('Ctrl Pts',(10.4064523339999,15.2,0.296721180999988));
#192978=CARTESIAN_POINT('Ctrl Pts',(10.4064523339999,11.6,0.296721180999988));
#192979=CARTESIAN_POINT('Ctrl Pts',(10.4076533469999,15.2,0.296900664999988));
#192980=CARTESIAN_POINT('Ctrl Pts',(10.4076533469999,11.6,0.296900664999988));
#192981=CARTESIAN_POINT('Ctrl Pts',(10.4088628589999,15.2,0.297082624999985));
#192982=CARTESIAN_POINT('Ctrl Pts',(10.4088628589999,11.6,0.297082624999984));
#192983=CARTESIAN_POINT('Ctrl Pts',(10.4100808439999,15.2,0.297267072999983));
#192984=CARTESIAN_POINT('Ctrl Pts',(10.4100808439999,11.6,0.297267072999982));
#192985=CARTESIAN_POINT('Ctrl Pts',(10.4113072789999,15.2,0.297454021999983));
#192986=CARTESIAN_POINT('Ctrl Pts',(10.4113072789999,11.6,0.297454021999983));
#192987=CARTESIAN_POINT('Ctrl Pts',(10.4125421359999,15.2,0.297643483999988));
#192988=CARTESIAN_POINT('Ctrl Pts',(10.4125421359999,11.6,0.297643483999987));
#192989=CARTESIAN_POINT('Ctrl Pts',(10.4137853929999,15.2,0.297835471999988));
#192990=CARTESIAN_POINT('Ctrl Pts',(10.4137853929999,11.6,0.297835471999987));
#192991=CARTESIAN_POINT('Ctrl Pts',(10.4150370239999,15.2,0.298029997999985));
#192992=CARTESIAN_POINT('Ctrl Pts',(10.4150370239999,11.6,0.298029997999984));
#192993=CARTESIAN_POINT('Ctrl Pts',(10.4162970039999,15.2,0.298227073999984));
#192994=CARTESIAN_POINT('Ctrl Pts',(10.4162970039999,11.6,0.298227073999983));
#192995=CARTESIAN_POINT('Ctrl Pts',(10.4175653089999,15.2,0.298426710999986));
#192996=CARTESIAN_POINT('Ctrl Pts',(10.4175653089999,11.6,0.298426710999986));
#192997=CARTESIAN_POINT('Ctrl Pts',(10.4188419149999,15.2,0.298628921999988));
#192998=CARTESIAN_POINT('Ctrl Pts',(10.4188419149999,11.6,0.298628921999988));
#192999=CARTESIAN_POINT('Ctrl Pts',(10.4201267969999,15.2,0.298833718999987));
#193000=CARTESIAN_POINT('Ctrl Pts',(10.4201267969999,11.6,0.298833718999986));
#193001=CARTESIAN_POINT('Ctrl Pts',(10.4214199299999,15.2,0.299041113999987));
#193002=CARTESIAN_POINT('Ctrl Pts',(10.4214199299999,11.6,0.299041113999987));
#193003=CARTESIAN_POINT('Ctrl Pts',(10.4227212909999,15.2,0.299251117999986));
#193004=CARTESIAN_POINT('Ctrl Pts',(10.4227212909999,11.6,0.299251117999985));
#193005=CARTESIAN_POINT('Ctrl Pts',(10.4240308559999,15.2,0.299463742999984));
#193006=CARTESIAN_POINT('Ctrl Pts',(10.4240308559999,11.6,0.299463742999983));
#193007=CARTESIAN_POINT('Ctrl Pts',(10.4253486009999,15.2,0.299679001999986));
#193008=CARTESIAN_POINT('Ctrl Pts',(10.4253486009999,11.6,0.299679001999986));
#193009=CARTESIAN_POINT('Ctrl Pts',(10.4266745019999,15.2,0.299896902999985));
#193010=CARTESIAN_POINT('Ctrl Pts',(10.4266745019999,11.6,0.299896902999985));
#193011=CARTESIAN_POINT('Ctrl Pts',(10.4280085349999,15.2,0.300117460999987));
#193012=CARTESIAN_POINT('Ctrl Pts',(10.4280085349999,11.6,0.300117460999986));
#193013=CARTESIAN_POINT('Ctrl Pts',(10.4293506769999,15.2,0.300340685999987));
#193014=CARTESIAN_POINT('Ctrl Pts',(10.4293506769999,11.6,0.300340685999986));
#193015=CARTESIAN_POINT('Ctrl Pts',(10.4307009019999,15.2,0.300566589999987));
#193016=CARTESIAN_POINT('Ctrl Pts',(10.4307009019999,11.6,0.300566589999986));
#193017=CARTESIAN_POINT('Ctrl Pts',(10.4320591909999,15.2,0.300795183999987));
#193018=CARTESIAN_POINT('Ctrl Pts',(10.4320591909999,11.6,0.300795183999986));
#193019=CARTESIAN_POINT('Ctrl Pts',(10.4334255159999,15.2,0.301026479999984));
#193020=CARTESIAN_POINT('Ctrl Pts',(10.4334255159999,11.6,0.301026479999984));
#193021=CARTESIAN_POINT('Ctrl Pts',(10.4347998569999,15.2,0.301260487999984));
#193022=CARTESIAN_POINT('Ctrl Pts',(10.4347998569999,11.6,0.301260487999983));
#193023=CARTESIAN_POINT('Ctrl Pts',(10.4361821889999,15.2,0.301497219999987));
#193024=CARTESIAN_POINT('Ctrl Pts',(10.4361821889999,11.6,0.301497219999986));
#193025=CARTESIAN_POINT('Ctrl Pts',(10.4375724899999,15.2,0.301736685999985));
#193026=CARTESIAN_POINT('Ctrl Pts',(10.4375724899999,11.6,0.301736685999984));
#193027=CARTESIAN_POINT('Ctrl Pts',(10.4389707379999,15.2,0.301978897999984));
#193028=CARTESIAN_POINT('Ctrl Pts',(10.4389707379999,11.6,0.301978897999983));
#193029=CARTESIAN_POINT('Ctrl Pts',(10.4403769079999,15.2,0.302223867999984));
#193030=CARTESIAN_POINT('Ctrl Pts',(10.4403769079999,11.6,0.302223867999984));
#193031=CARTESIAN_POINT('Ctrl Pts',(10.4417909759999,15.2,0.302471604999983));
#193032=CARTESIAN_POINT('Ctrl Pts',(10.4417909759999,11.6,0.302471604999983));
#193033=CARTESIAN_POINT('Ctrl Pts',(10.4432129229999,15.2,0.302722120999985));
#193034=CARTESIAN_POINT('Ctrl Pts',(10.4432129229999,11.6,0.302722120999985));
#193035=CARTESIAN_POINT('Ctrl Pts',(10.4446427239999,15.2,0.302975425999983));
#193036=CARTESIAN_POINT('Ctrl Pts',(10.4446427239999,11.6,0.302975425999982));
#193037=CARTESIAN_POINT('Ctrl Pts',(10.4460803579999,15.2,0.303231530999986));
#193038=CARTESIAN_POINT('Ctrl Pts',(10.4460803579999,11.6,0.303231530999985));
#193039=CARTESIAN_POINT('Ctrl Pts',(10.4475257999999,15.2,0.303490447999986));
#193040=CARTESIAN_POINT('Ctrl Pts',(10.4475257999999,11.6,0.303490447999985));
#193041=CARTESIAN_POINT('Ctrl Pts',(10.4489790289999,15.2,0.303752186999984));
#193042=CARTESIAN_POINT('Ctrl Pts',(10.4489790289999,11.6,0.303752186999983));
#193043=CARTESIAN_POINT('Ctrl Pts',(10.4504400239999,15.2,0.304016756999985));
#193044=CARTESIAN_POINT('Ctrl Pts',(10.4504400239999,11.6,0.304016756999985));
#193045=CARTESIAN_POINT('Ctrl Pts',(10.4519087609999,15.2,0.304284169999987));
#193046=CARTESIAN_POINT('Ctrl Pts',(10.4519087609999,11.6,0.304284169999986));
#193047=CARTESIAN_POINT('Ctrl Pts',(10.4533852189999,15.2,0.304554435999984));
#193048=CARTESIAN_POINT('Ctrl Pts',(10.4533852189999,11.6,0.304554435999984));
#193049=CARTESIAN_POINT('Ctrl Pts',(10.4548693739999,15.2,0.304827565999983));
#193050=CARTESIAN_POINT('Ctrl Pts',(10.4548693739999,11.6,0.304827565999983));
#193051=CARTESIAN_POINT('Ctrl Pts',(10.4563612069999,15.2,0.305103569999985));
#193052=CARTESIAN_POINT('Ctrl Pts',(10.4563612069999,11.6,0.305103569999984));
#193053=CARTESIAN_POINT('Ctrl Pts',(10.4578606949999,15.2,0.305382457999985));
#193054=CARTESIAN_POINT('Ctrl Pts',(10.4578606949999,11.6,0.305382457999985));
#193055=CARTESIAN_POINT('Ctrl Pts',(10.4593678149999,15.2,0.305664240999985));
#193056=CARTESIAN_POINT('Ctrl Pts',(10.4593678149999,11.6,0.305664240999985));
#193057=CARTESIAN_POINT('Ctrl Pts',(10.4608825449999,15.2,0.305948927999986));
#193058=CARTESIAN_POINT('Ctrl Pts',(10.4608825449999,11.6,0.305948927999986));
#193059=CARTESIAN_POINT('Ctrl Pts',(10.4624048659999,15.2,0.306236530999984));
#193060=CARTESIAN_POINT('Ctrl Pts',(10.4624048659999,11.6,0.306236530999983));
#193061=CARTESIAN_POINT('Ctrl Pts',(10.4639347549999,15.2,0.306527058999984));
#193062=CARTESIAN_POINT('Ctrl Pts',(10.4639347549999,11.6,0.306527058999983));
#193063=CARTESIAN_POINT('Ctrl Pts',(10.4654721899999,15.2,0.306820520999986));
#193064=CARTESIAN_POINT('Ctrl Pts',(10.4654721899999,11.6,0.306820520999986));
#193065=CARTESIAN_POINT('Ctrl Pts',(10.4670171509999,15.2,0.307116928999989));
#193066=CARTESIAN_POINT('Ctrl Pts',(10.4670171509999,11.6,0.307116928999988));
#193067=CARTESIAN_POINT('Ctrl Pts',(10.4685696139999,15.2,0.307416291999987));
#193068=CARTESIAN_POINT('Ctrl Pts',(10.4685696139999,11.6,0.307416291999986));
#193069=CARTESIAN_POINT('Ctrl Pts',(10.4701295609999,15.2,0.307718619999986));
#193070=CARTESIAN_POINT('Ctrl Pts',(10.4701295609999,11.6,0.307718619999986));
#193071=CARTESIAN_POINT('Ctrl Pts',(10.4716969689999,15.2,0.308023921999983));
#193072=CARTESIAN_POINT('Ctrl Pts',(10.4716969689999,11.6,0.308023921999982));
#193073=CARTESIAN_POINT('Ctrl Pts',(10.4732718189999,15.2,0.308332208999986));
#193074=CARTESIAN_POINT('Ctrl Pts',(10.4732718189999,11.6,0.308332208999986));
#193075=CARTESIAN_POINT('Ctrl Pts',(10.4748540859999,15.2,0.308643490999985));
#193076=CARTESIAN_POINT('Ctrl Pts',(10.4748540859999,11.6,0.308643490999984));
#193077=CARTESIAN_POINT('Ctrl Pts',(10.4764437519999,15.2,0.308957776999983));
#193078=CARTESIAN_POINT('Ctrl Pts',(10.4764437519999,11.6,0.308957776999983));
#193079=CARTESIAN_POINT('Ctrl Pts',(10.4780407969999,15.2,0.309275076999986));
#193080=CARTESIAN_POINT('Ctrl Pts',(10.4780407969999,11.6,0.309275076999986));
#193081=CARTESIAN_POINT('Ctrl Pts',(10.4796451969999,15.2,0.309595398999987));
#193082=CARTESIAN_POINT('Ctrl Pts',(10.4796451969999,11.6,0.309595398999986));
#193083=CARTESIAN_POINT('Ctrl Pts',(10.4812569339999,15.2,0.309918754999985));
#193084=CARTESIAN_POINT('Ctrl Pts',(10.4812569339999,11.6,0.309918754999984));
#193085=CARTESIAN_POINT('Ctrl Pts',(10.4828759869999,15.2,0.310245152999986));
#193086=CARTESIAN_POINT('Ctrl Pts',(10.4828759869999,11.6,0.310245152999986));
#193087=CARTESIAN_POINT('Ctrl Pts',(10.4845023339999,15.2,0.310574602999987));
#193088=CARTESIAN_POINT('Ctrl Pts',(10.4845023339999,11.6,0.310574602999986));
#193089=CARTESIAN_POINT('Ctrl Pts',(10.4861359559999,15.2,0.310907112999987));
#193090=CARTESIAN_POINT('Ctrl Pts',(10.4861359559999,11.6,0.310907112999987));
#193091=CARTESIAN_POINT('Ctrl Pts',(10.4877768319999,15.2,0.311242694999985));
#193092=CARTESIAN_POINT('Ctrl Pts',(10.4877768319999,11.6,0.311242694999984));
#193093=CARTESIAN_POINT('Ctrl Pts',(10.4894249419999,15.2,0.311581356999984));
#193094=CARTESIAN_POINT('Ctrl Pts',(10.4894249419999,11.6,0.311581356999983));
#193095=CARTESIAN_POINT('Ctrl Pts',(10.4910802659999,15.2,0.311923107999985));
#193096=CARTESIAN_POINT('Ctrl Pts',(10.4910802659999,11.6,0.311923107999985));
#193097=CARTESIAN_POINT('Ctrl Pts',(10.4927427829999,15.2,0.312267955999985));
#193098=CARTESIAN_POINT('Ctrl Pts',(10.4927427829999,11.6,0.312267955999985));
#193099=CARTESIAN_POINT('Ctrl Pts',(10.4944124729999,15.2,0.312615912999985));
#193100=CARTESIAN_POINT('Ctrl Pts',(10.4944124729999,11.6,0.312615912999985));
#193101=CARTESIAN_POINT('Ctrl Pts',(10.4960893159999,15.2,0.312966985999985));
#193102=CARTESIAN_POINT('Ctrl Pts',(10.4960893159999,11.6,0.312966985999985));
#193103=CARTESIAN_POINT('Ctrl Pts',(10.4977732919999,15.2,0.313321184999986));
#193104=CARTESIAN_POINT('Ctrl Pts',(10.4977732919999,11.6,0.313321184999986));
#193105=CARTESIAN_POINT('Ctrl Pts',(10.4994643819999,15.2,0.313678519999985));
#193106=CARTESIAN_POINT('Ctrl Pts',(10.4994643819999,11.6,0.313678519999984));
#193107=CARTESIAN_POINT('Ctrl Pts',(10.5011625649999,15.2,0.314038996999986));
#193108=CARTESIAN_POINT('Ctrl Pts',(10.5011625649999,11.6,0.314038996999985));
#193109=CARTESIAN_POINT('Ctrl Pts',(10.5028678219999,15.2,0.314402627999986));
#193110=CARTESIAN_POINT('Ctrl Pts',(10.5028678219999,11.6,0.314402627999985));
#193111=CARTESIAN_POINT('Ctrl Pts',(10.5045801319999,15.2,0.314769419999985));
#193112=CARTESIAN_POINT('Ctrl Pts',(10.5045801319999,11.6,0.314769419999985));
#193113=CARTESIAN_POINT('Ctrl Pts',(10.5062994779999,15.2,0.315139381999985));
#193114=CARTESIAN_POINT('Ctrl Pts',(10.5062994779999,11.6,0.315139381999984));
#193115=CARTESIAN_POINT('Ctrl Pts',(10.5080258379999,15.2,0.315512523999986));
#193116=CARTESIAN_POINT('Ctrl Pts',(10.5080258379999,11.6,0.315512523999985));
#193117=CARTESIAN_POINT('Ctrl Pts',(10.5097591929999,15.2,0.315888853999984));
#193118=CARTESIAN_POINT('Ctrl Pts',(10.5097591929999,11.6,0.315888853999983));
#193119=CARTESIAN_POINT('Ctrl Pts',(10.5114995239999,15.2,0.316268379999984));
#193120=CARTESIAN_POINT('Ctrl Pts',(10.5114995239999,11.6,0.316268379999984));
#193121=CARTESIAN_POINT('Ctrl Pts',(10.5132468119999,15.2,0.316651112999988));
#193122=CARTESIAN_POINT('Ctrl Pts',(10.5132468119999,11.6,0.316651112999988));
#193123=CARTESIAN_POINT('Ctrl Pts',(10.5150010359999,15.2,0.317037058999983));
#193124=CARTESIAN_POINT('Ctrl Pts',(10.5150010359999,11.6,0.317037058999982));
#193125=CARTESIAN_POINT('Ctrl Pts',(10.5167621799999,15.2,0.317426227999986));
#193126=CARTESIAN_POINT('Ctrl Pts',(10.5167621799999,11.6,0.317426227999986));
#193127=CARTESIAN_POINT('Ctrl Pts',(10.5185302209999,15.2,0.317818628999986));
#193128=CARTESIAN_POINT('Ctrl Pts',(10.5185302209999,11.6,0.317818628999986));
#193129=CARTESIAN_POINT('Ctrl Pts',(10.5203051419999,15.2,0.318214267999988));
#193130=CARTESIAN_POINT('Ctrl Pts',(10.5203051419999,11.6,0.318214267999987));
#193131=CARTESIAN_POINT('Ctrl Pts',(10.5220869239999,15.2,0.318613156999987));
#193132=CARTESIAN_POINT('Ctrl Pts',(10.5220869239999,11.6,0.318613156999987));
#193133=CARTESIAN_POINT('Ctrl Pts',(10.5238755469999,15.2,0.319015301999985));
#193134=CARTESIAN_POINT('Ctrl Pts',(10.5238755469999,11.6,0.319015301999985));
#193135=CARTESIAN_POINT('Ctrl Pts',(10.5256709929999,15.2,0.319420711999987));
#193136=CARTESIAN_POINT('Ctrl Pts',(10.5256709929999,11.6,0.319420711999987));
#193137=CARTESIAN_POINT('Ctrl Pts',(10.5274732429999,15.2,0.319829395999989));
#193138=CARTESIAN_POINT('Ctrl Pts',(10.5274732429999,11.6,0.319829395999988));
#193139=CARTESIAN_POINT('Ctrl Pts',(10.5292822789999,15.2,0.320241360999987));
#193140=CARTESIAN_POINT('Ctrl Pts',(10.5292822789999,11.6,0.320241360999986));
#193141=CARTESIAN_POINT('Ctrl Pts',(10.5310980799999,15.2,0.320656615999986));
#193142=CARTESIAN_POINT('Ctrl Pts',(10.5310980799999,11.6,0.320656615999985));
#193143=CARTESIAN_POINT('Ctrl Pts',(10.5329206289999,15.2,0.321075169999983));
#193144=CARTESIAN_POINT('Ctrl Pts',(10.5329206289999,11.6,0.321075169999982));
#193145=CARTESIAN_POINT('Ctrl Pts',(10.5347499079999,15.2,0.321497028999986));
#193146=CARTESIAN_POINT('Ctrl Pts',(10.5347499079999,11.6,0.321497028999986));
#193147=CARTESIAN_POINT('Ctrl Pts',(10.5365858959999,15.2,0.321922202999985));
#193148=CARTESIAN_POINT('Ctrl Pts',(10.5365858959999,11.6,0.321922202999984));
#193149=CARTESIAN_POINT('Ctrl Pts',(10.5384285769999,15.2,0.322350700999987));
#193150=CARTESIAN_POINT('Ctrl Pts',(10.5384285769999,11.6,0.322350700999987));
#193151=CARTESIAN_POINT('Ctrl Pts',(10.5402779309999,15.2,0.322782526999985));
#193152=CARTESIAN_POINT('Ctrl Pts',(10.5402779309999,11.6,0.322782526999985));
#193153=CARTESIAN_POINT('Ctrl Pts',(10.5421339399999,15.2,0.323217693999984));
#193154=CARTESIAN_POINT('Ctrl Pts',(10.5421339399999,11.6,0.323217693999984));
#193155=CARTESIAN_POINT('Ctrl Pts',(10.5439965859999,15.2,0.323656206999985));
#193156=CARTESIAN_POINT('Ctrl Pts',(10.5439965859999,11.6,0.323656206999984));
#193157=CARTESIAN_POINT('Ctrl Pts',(10.5458658509999,15.2,0.324098074999988));
#193158=CARTESIAN_POINT('Ctrl Pts',(10.5458658509999,11.6,0.324098074999987));
#193159=CARTESIAN_POINT('Ctrl Pts',(10.5477417169999,15.2,0.324543303999985));
#193160=CARTESIAN_POINT('Ctrl Pts',(10.5477417169999,11.6,0.324543303999984));
#193161=CARTESIAN_POINT('Ctrl Pts',(10.5496241639999,15.2,0.324991904999985));
#193162=CARTESIAN_POINT('Ctrl Pts',(10.5496241639999,11.6,0.324991904999985));
#193163=CARTESIAN_POINT('Ctrl Pts',(10.5515131759999,15.2,0.325443883999985));
#193164=CARTESIAN_POINT('Ctrl Pts',(10.5515131759999,11.6,0.325443883999985));
#193165=CARTESIAN_POINT('Ctrl Pts',(10.5534087349999,15.2,0.325899248999986));
#193166=CARTESIAN_POINT('Ctrl Pts',(10.5534087349999,11.6,0.325899248999985));
#193167=CARTESIAN_POINT('Ctrl Pts',(10.5553108209999,15.2,0.326358006999987));
#193168=CARTESIAN_POINT('Ctrl Pts',(10.5553108209999,11.6,0.326358006999987));
#193169=CARTESIAN_POINT('Ctrl Pts',(10.5572194179999,15.2,0.326820166999986));
#193170=CARTESIAN_POINT('Ctrl Pts',(10.5572194179999,11.6,0.326820166999986));
#193171=CARTESIAN_POINT('Ctrl Pts',(10.5591345069999,15.2,0.327285735999983));
#193172=CARTESIAN_POINT('Ctrl Pts',(10.5591345069999,11.6,0.327285735999982));
#193173=CARTESIAN_POINT('Ctrl Pts',(10.5610560699999,15.2,0.327754721999987));
#193174=CARTESIAN_POINT('Ctrl Pts',(10.5610560699999,11.6,0.327754721999986));
#193175=CARTESIAN_POINT('Ctrl Pts',(10.5629840909999,15.2,0.328227131999985));
#193176=CARTESIAN_POINT('Ctrl Pts',(10.5629840909999,11.6,0.328227131999985));
#193177=CARTESIAN_POINT('Ctrl Pts',(10.5649185509999,15.2,0.328702973999988));
#193178=CARTESIAN_POINT('Ctrl Pts',(10.5649185509999,11.6,0.328702973999988));
#193179=CARTESIAN_POINT('Ctrl Pts',(10.5668594319999,15.2,0.329182255999987));
#193180=CARTESIAN_POINT('Ctrl Pts',(10.5668594319999,11.6,0.329182255999986));
#193181=CARTESIAN_POINT('Ctrl Pts',(10.5688067179999,15.2,0.329664984999987));
#193182=CARTESIAN_POINT('Ctrl Pts',(10.5688067179999,11.6,0.329664984999986));
#193183=CARTESIAN_POINT('Ctrl Pts',(10.5707603889999,15.2,0.330151168999984));
#193184=CARTESIAN_POINT('Ctrl Pts',(10.5707603889999,11.6,0.330151168999983));
#193185=CARTESIAN_POINT('Ctrl Pts',(10.5727204309999,15.2,0.330640813999987));
#193186=CARTESIAN_POINT('Ctrl Pts',(10.5727204309999,11.6,0.330640813999987));
#193187=CARTESIAN_POINT('Ctrl Pts',(10.5746868229999,15.2,0.331133928999985));
#193188=CARTESIAN_POINT('Ctrl Pts',(10.5746868229999,11.6,0.331133928999984));
#193189=CARTESIAN_POINT('Ctrl Pts',(10.5766595509999,15.2,0.331630518999986));
#193190=CARTESIAN_POINT('Ctrl Pts',(10.5766595509999,11.6,0.331630518999985));
#193191=CARTESIAN_POINT('Ctrl Pts',(10.5786385939999,15.2,0.332130593999986));
#193192=CARTESIAN_POINT('Ctrl Pts',(10.5786385939999,11.6,0.332130593999986));
#193193=CARTESIAN_POINT('Ctrl Pts',(10.5806239379999,15.2,0.332634160999987));
#193194=CARTESIAN_POINT('Ctrl Pts',(10.5806239379999,11.6,0.332634160999987));
#193195=CARTESIAN_POINT('Ctrl Pts',(10.5826155629999,15.2,0.333141224999984));
#193196=CARTESIAN_POINT('Ctrl Pts',(10.5826155629999,11.6,0.333141224999984));
#193197=CARTESIAN_POINT('Ctrl Pts',(10.5846134539999,15.2,0.333651795999987));
#193198=CARTESIAN_POINT('Ctrl Pts',(10.5846134539999,11.6,0.333651795999987));
#193199=CARTESIAN_POINT('Ctrl Pts',(10.5866175939999,15.2,0.334165879999984));
#193200=CARTESIAN_POINT('Ctrl Pts',(10.5866175939999,11.6,0.334165879999983));
#193201=CARTESIAN_POINT('Ctrl Pts',(10.5886279639999,15.2,0.334683481999987));
#193202=CARTESIAN_POINT('Ctrl Pts',(10.5886279639999,11.6,0.334683481999986));
#193203=CARTESIAN_POINT('Ctrl Pts',(10.5906445489999,15.2,0.335204612999984));
#193204=CARTESIAN_POINT('Ctrl Pts',(10.5906445489999,11.6,0.335204612999984));
#193205=CARTESIAN_POINT('Ctrl Pts',(10.5926673309999,15.2,0.335729276999985));
#193206=CARTESIAN_POINT('Ctrl Pts',(10.5926673309999,11.6,0.335729276999985));
#193207=CARTESIAN_POINT('Ctrl Pts',(10.5946962929999,15.2,0.336257483999987));
#193208=CARTESIAN_POINT('Ctrl Pts',(10.5946962929999,11.6,0.336257483999986));
#193209=CARTESIAN_POINT('Ctrl Pts',(10.5967314189999,15.2,0.336789236999984));
#193210=CARTESIAN_POINT('Ctrl Pts',(10.5967314189999,11.6,0.336789236999983));
#193211=CARTESIAN_POINT('Ctrl Pts',(10.5987726909999,15.2,0.337324546999986));
#193212=CARTESIAN_POINT('Ctrl Pts',(10.5987726909999,11.6,0.337324546999986));
#193213=CARTESIAN_POINT('Ctrl Pts',(10.6008200939999,15.2,0.337863417999986));
#193214=CARTESIAN_POINT('Ctrl Pts',(10.6008200939999,11.6,0.337863417999986));
#193215=CARTESIAN_POINT('Ctrl Pts',(10.6028736079999,15.2,0.338405857999984));
#193216=CARTESIAN_POINT('Ctrl Pts',(10.6028736079999,11.6,0.338405857999983));
#193217=CARTESIAN_POINT('Ctrl Pts',(10.6049332199999,15.2,0.338951874999989));
#193218=CARTESIAN_POINT('Ctrl Pts',(10.6049332199999,11.6,0.338951874999988));
#193219=CARTESIAN_POINT('Ctrl Pts',(10.6069989119999,15.2,0.339501473999988));
#193220=CARTESIAN_POINT('Ctrl Pts',(10.6069989119999,11.6,0.339501473999988));
#193221=CARTESIAN_POINT('Ctrl Pts',(10.6090706669999,15.2,0.340054661999982));
#193222=CARTESIAN_POINT('Ctrl Pts',(10.6090706669999,11.6,0.340054661999982));
#193223=CARTESIAN_POINT('Ctrl Pts',(10.6111484689999,15.2,0.340611447999986));
#193224=CARTESIAN_POINT('Ctrl Pts',(10.6111484689999,11.6,0.340611447999985));
#193225=CARTESIAN_POINT('Ctrl Pts',(10.6132323019999,15.2,0.341171835999985));
#193226=CARTESIAN_POINT('Ctrl Pts',(10.6132323019999,11.6,0.341171835999984));
#193227=CARTESIAN_POINT('Ctrl Pts',(10.6153221469999,15.2,0.341735832999985));
#193228=CARTESIAN_POINT('Ctrl Pts',(10.6153221469999,11.6,0.341735832999985));
#193229=CARTESIAN_POINT('Ctrl Pts',(10.6174179919999,15.2,0.342303447999988));
#193230=CARTESIAN_POINT('Ctrl Pts',(10.6174179919999,11.6,0.342303447999987));
#193231=CARTESIAN_POINT('Ctrl Pts',(10.6195198169999,15.2,0.342874684999988));
#193232=CARTESIAN_POINT('Ctrl Pts',(10.6195198169999,11.6,0.342874684999987));
#193233=CARTESIAN_POINT('Ctrl Pts',(10.6216276069999,15.2,0.343449551999986));
#193234=CARTESIAN_POINT('Ctrl Pts',(10.6216276069999,11.6,0.343449551999985));
#193235=CARTESIAN_POINT('Ctrl Pts',(10.6237413459999,15.2,0.344028055999988));
#193236=CARTESIAN_POINT('Ctrl Pts',(10.6237413459999,11.6,0.344028055999987));
#193237=CARTESIAN_POINT('Ctrl Pts',(10.6258610179999,15.2,0.344610201999984));
#193238=CARTESIAN_POINT('Ctrl Pts',(10.6258610179999,11.6,0.344610201999984));
#193239=CARTESIAN_POINT('Ctrl Pts',(10.6279866059999,15.2,0.345195998999985));
#193240=CARTESIAN_POINT('Ctrl Pts',(10.6279866059999,11.6,0.345195998999985));
#193241=CARTESIAN_POINT('Ctrl Pts',(10.6301180949999,15.2,0.345785449999987));
#193242=CARTESIAN_POINT('Ctrl Pts',(10.6301180949999,11.6,0.345785449999986));
#193243=CARTESIAN_POINT('Ctrl Pts',(10.6322554669999,15.2,0.346378564999985));
#193244=CARTESIAN_POINT('Ctrl Pts',(10.6322554669999,11.6,0.346378564999985));
#193245=CARTESIAN_POINT('Ctrl Pts',(10.6343987089999,15.2,0.346975346999985));
#193246=CARTESIAN_POINT('Ctrl Pts',(10.6343987089999,11.6,0.346975346999984));
#193247=CARTESIAN_POINT('Ctrl Pts',(10.6365478019999,15.2,0.347575804999987));
#193248=CARTESIAN_POINT('Ctrl Pts',(10.6365478019999,11.6,0.347575804999986));
#193249=CARTESIAN_POINT('Ctrl Pts',(10.6387027319999,15.2,0.348179944999987));
#193250=CARTESIAN_POINT('Ctrl Pts',(10.6387027319999,11.6,0.348179944999986));
#193251=CARTESIAN_POINT('Ctrl Pts',(10.6408634829999,15.2,0.348787772999986));
#193252=CARTESIAN_POINT('Ctrl Pts',(10.6408634829999,11.6,0.348787772999985));
#193253=CARTESIAN_POINT('Ctrl Pts',(10.6430300389999,15.2,0.349399293999983));
#193254=CARTESIAN_POINT('Ctrl Pts',(10.6430300389999,11.6,0.349399293999983));
#193255=CARTESIAN_POINT('Ctrl Pts',(10.6452023819999,15.2,0.350014516999986));
#193256=CARTESIAN_POINT('Ctrl Pts',(10.6452023819999,11.6,0.350014516999985));
#193257=CARTESIAN_POINT('Ctrl Pts',(10.6473805009999,15.2,0.350633446999984));
#193258=CARTESIAN_POINT('Ctrl Pts',(10.6473805009999,11.6,0.350633446999983));
#193259=CARTESIAN_POINT('Ctrl Pts',(10.6495643749999,15.2,0.351256088999987));
#193260=CARTESIAN_POINT('Ctrl Pts',(10.6495643749999,11.6,0.351256088999987));
#193261=CARTESIAN_POINT('Ctrl Pts',(10.6517539929999,15.2,0.351882449999987));
#193262=CARTESIAN_POINT('Ctrl Pts',(10.6517539929999,11.6,0.351882449999987));
#193263=CARTESIAN_POINT('Ctrl Pts',(10.6539493359999,15.2,0.352512536999985));
#193264=CARTESIAN_POINT('Ctrl Pts',(10.6539493359999,11.6,0.352512536999984));
#193265=CARTESIAN_POINT('Ctrl Pts',(10.6561503909999,15.2,0.353146354999985));
#193266=CARTESIAN_POINT('Ctrl Pts',(10.6561503909999,11.6,0.353146354999984));
#193267=CARTESIAN_POINT('Ctrl Pts',(10.6583571409999,15.2,0.353783909999983));
#193268=CARTESIAN_POINT('Ctrl Pts',(10.6583571409999,11.6,0.353783909999982));
#193269=CARTESIAN_POINT('Ctrl Pts',(10.6605695709999,15.2,0.354425208999984));
#193270=CARTESIAN_POINT('Ctrl Pts',(10.6605695709999,11.6,0.354425208999984));
#193271=CARTESIAN_POINT('Ctrl Pts',(10.6627876639999,15.2,0.355070257999985));
#193272=CARTESIAN_POINT('Ctrl Pts',(10.6627876639999,11.6,0.355070257999985));
#193273=CARTESIAN_POINT('Ctrl Pts',(10.6650114069999,15.2,0.355719062999986));
#193274=CARTESIAN_POINT('Ctrl Pts',(10.6650114069999,11.6,0.355719062999986));
#193275=CARTESIAN_POINT('Ctrl Pts',(10.6672407829999,15.2,0.356371629999988));
#193276=CARTESIAN_POINT('Ctrl Pts',(10.6672407829999,11.6,0.356371629999987));
#193277=CARTESIAN_POINT('Ctrl Pts',(10.6694757779999,15.2,0.357027963999985));
#193278=CARTESIAN_POINT('Ctrl Pts',(10.6694757779999,11.6,0.357027963999985));
#193279=CARTESIAN_POINT('Ctrl Pts',(10.6717163759999,15.2,0.357688071999984));
#193280=CARTESIAN_POINT('Ctrl Pts',(10.6717163759999,11.6,0.357688071999984));
#193281=CARTESIAN_POINT('Ctrl Pts',(10.6739625609999,15.2,0.358351958999985));
#193282=CARTESIAN_POINT('Ctrl Pts',(10.6739625609999,11.6,0.358351958999985));
#193283=CARTESIAN_POINT('Ctrl Pts',(10.6762143189999,15.2,0.359019631999988));
#193284=CARTESIAN_POINT('Ctrl Pts',(10.6762143189999,11.6,0.359019631999988));
#193285=CARTESIAN_POINT('Ctrl Pts',(10.6784716349999,15.2,0.359691095999985));
#193286=CARTESIAN_POINT('Ctrl Pts',(10.6784716349999,11.6,0.359691095999985));
#193287=CARTESIAN_POINT('Ctrl Pts',(10.6807344929999,15.2,0.360366356999986));
#193288=CARTESIAN_POINT('Ctrl Pts',(10.6807344929999,11.6,0.360366356999986));
#193289=CARTESIAN_POINT('Ctrl Pts',(10.6830028779999,15.2,0.361045420999986));
#193290=CARTESIAN_POINT('Ctrl Pts',(10.6830028779999,11.6,0.361045420999985));
#193291=CARTESIAN_POINT('Ctrl Pts',(10.6852767759999,15.2,0.361728292999985));
#193292=CARTESIAN_POINT('Ctrl Pts',(10.6852767759999,11.6,0.361728292999985));
#193293=CARTESIAN_POINT('Ctrl Pts',(10.6875561699999,15.2,0.362414979999985));
#193294=CARTESIAN_POINT('Ctrl Pts',(10.6875561699999,11.6,0.362414979999985));
#193295=CARTESIAN_POINT('Ctrl Pts',(10.6898410479999,15.2,0.363105487999986));
#193296=CARTESIAN_POINT('Ctrl Pts',(10.6898410479999,11.6,0.363105487999986));
#193297=CARTESIAN_POINT('Ctrl Pts',(10.6921313919999,15.2,0.363799819999984));
#193298=CARTESIAN_POINT('Ctrl Pts',(10.6921313919999,11.6,0.363799819999983));
#193299=CARTESIAN_POINT('Ctrl Pts',(10.6944271889999,15.2,0.364497984999983));
#193300=CARTESIAN_POINT('Ctrl Pts',(10.6944271889999,11.6,0.364497984999983));
#193301=CARTESIAN_POINT('Ctrl Pts',(10.6967284239999,15.2,0.365199985999984));
#193302=CARTESIAN_POINT('Ctrl Pts',(10.6967284239999,11.6,0.365199985999984));
#193303=CARTESIAN_POINT('Ctrl Pts',(10.6990350819999,15.2,0.365905829999988));
#193304=CARTESIAN_POINT('Ctrl Pts',(10.6990350819999,11.6,0.365905829999988));
#193305=CARTESIAN_POINT('Ctrl Pts',(10.7013471479999,15.2,0.366615522999982));
#193306=CARTESIAN_POINT('Ctrl Pts',(10.7013471479999,11.6,0.366615522999982));
#193307=CARTESIAN_POINT('Ctrl Pts',(10.7036646069999,15.2,0.367329069999984));
#193308=CARTESIAN_POINT('Ctrl Pts',(10.7036646069999,11.6,0.367329069999984));
#193309=CARTESIAN_POINT('Ctrl Pts',(10.7059874449999,15.2,0.368046474999986));
#193310=CARTESIAN_POINT('Ctrl Pts',(10.7059874449999,11.6,0.368046474999985));
#193311=CARTESIAN_POINT('Ctrl Pts',(10.7083156469999,15.2,0.368767745999987));
#193312=CARTESIAN_POINT('Ctrl Pts',(10.7083156469999,11.6,0.368767745999987));
#193313=CARTESIAN_POINT('Ctrl Pts',(10.7106491999999,15.2,0.369492886999985));
#193314=CARTESIAN_POINT('Ctrl Pts',(10.7106491999999,11.6,0.369492886999984));
#193315=CARTESIAN_POINT('Ctrl Pts',(10.7129880859999,15.2,0.370221903999983));
#193316=CARTESIAN_POINT('Ctrl Pts',(10.7129880859999,11.6,0.370221903999983));
#193317=CARTESIAN_POINT('Ctrl Pts',(10.7153322929999,15.2,0.370954801999983));
#193318=CARTESIAN_POINT('Ctrl Pts',(10.7153322929999,11.6,0.370954801999983));
#193319=CARTESIAN_POINT('Ctrl Pts',(10.7176818059999,15.2,0.371691585999985));
#193320=CARTESIAN_POINT('Ctrl Pts',(10.7176818059999,11.6,0.371691585999984));
#193321=CARTESIAN_POINT('Ctrl Pts',(10.7200366109999,15.2,0.372432262999984));
#193322=CARTESIAN_POINT('Ctrl Pts',(10.7200366109999,11.6,0.372432262999984));
#193323=CARTESIAN_POINT('Ctrl Pts',(10.7223966929999,15.2,0.373176837999987));
#193324=CARTESIAN_POINT('Ctrl Pts',(10.7223966929999,11.6,0.373176837999986));
#193325=CARTESIAN_POINT('Ctrl Pts',(10.7247620369999,15.2,0.373925313999983));
#193326=CARTESIAN_POINT('Ctrl Pts',(10.7247620369999,11.6,0.373925313999983));
#193327=CARTESIAN_POINT('Ctrl Pts',(10.7271326309999,15.2,0.374677699999988));
#193328=CARTESIAN_POINT('Ctrl Pts',(10.7271326309999,11.6,0.374677699999987));
#193329=CARTESIAN_POINT('Ctrl Pts',(10.7295084569999,15.2,0.375433997999988));
#193330=CARTESIAN_POINT('Ctrl Pts',(10.7295084569999,11.6,0.375433997999987));
#193331=CARTESIAN_POINT('Ctrl Pts',(10.7318895039999,15.2,0.376194214999988));
#193332=CARTESIAN_POINT('Ctrl Pts',(10.7318895039999,11.6,0.376194214999987));
#193333=CARTESIAN_POINT('Ctrl Pts',(10.7342757559999,15.2,0.376958354999988));
#193334=CARTESIAN_POINT('Ctrl Pts',(10.7342757559999,11.6,0.376958354999987));
#193335=CARTESIAN_POINT('Ctrl Pts',(10.7366671989999,15.2,0.377726424999985));
#193336=CARTESIAN_POINT('Ctrl Pts',(10.7366671989999,11.6,0.377726424999984));
#193337=CARTESIAN_POINT('Ctrl Pts',(10.7390638199999,15.2,0.378498429999983));
#193338=CARTESIAN_POINT('Ctrl Pts',(10.7390638199999,11.6,0.378498429999982));
#193339=CARTESIAN_POINT('Ctrl Pts',(10.7414656029999,15.2,0.379274372999987));
#193340=CARTESIAN_POINT('Ctrl Pts',(10.7414656029999,11.6,0.379274372999987));
#193341=CARTESIAN_POINT('Ctrl Pts',(10.7438725369999,15.2,0.380054260999985));
#193342=CARTESIAN_POINT('Ctrl Pts',(10.7438725369999,11.6,0.380054260999984));
#193343=CARTESIAN_POINT('Ctrl Pts',(10.7462846039999,15.2,0.380838097999985));
#193344=CARTESIAN_POINT('Ctrl Pts',(10.7462846039999,11.6,0.380838097999984));
#193345=CARTESIAN_POINT('Ctrl Pts',(10.7487017909999,15.2,0.381625889999988));
#193346=CARTESIAN_POINT('Ctrl Pts',(10.7487017909999,11.6,0.381625889999988));
#193347=CARTESIAN_POINT('Ctrl Pts',(10.7511240869999,15.2,0.382417640999986));
#193348=CARTESIAN_POINT('Ctrl Pts',(10.7511240869999,11.6,0.382417640999985));
#193349=CARTESIAN_POINT('Ctrl Pts',(10.7535514749999,15.2,0.383213357999987));
#193350=CARTESIAN_POINT('Ctrl Pts',(10.7535514749999,11.6,0.383213357999987));
#193351=CARTESIAN_POINT('Ctrl Pts',(10.7559839419999,15.2,0.384013043999989));
#193352=CARTESIAN_POINT('Ctrl Pts',(10.7559839419999,11.6,0.384013043999988));
#193353=CARTESIAN_POINT('Ctrl Pts',(10.7584214739999,15.2,0.384816704999986));
#193354=CARTESIAN_POINT('Ctrl Pts',(10.7584214739999,11.6,0.384816704999986));
#193355=CARTESIAN_POINT('Ctrl Pts',(10.7608640569999,15.2,0.385624345999984));
#193356=CARTESIAN_POINT('Ctrl Pts',(10.7608640569999,11.6,0.385624345999984));
#193357=CARTESIAN_POINT('Ctrl Pts',(10.7633116769999,15.2,0.386435971999983));
#193358=CARTESIAN_POINT('Ctrl Pts',(10.7633116769999,11.6,0.386435971999983));
#193359=CARTESIAN_POINT('Ctrl Pts',(10.7657643219999,15.2,0.387251585999984));
#193360=CARTESIAN_POINT('Ctrl Pts',(10.7657643219999,11.6,0.387251585999983));
#193361=CARTESIAN_POINT('Ctrl Pts',(10.7682219759999,15.2,0.388071195999986));
#193362=CARTESIAN_POINT('Ctrl Pts',(10.7682219759999,11.6,0.388071195999986));
#193363=CARTESIAN_POINT('Ctrl Pts',(10.7706846259999,15.2,0.388894804999986));
#193364=CARTESIAN_POINT('Ctrl Pts',(10.7706846259999,11.6,0.388894804999986));
#193365=CARTESIAN_POINT('Ctrl Pts',(10.7731522589999,15.2,0.389722418999985));
#193366=CARTESIAN_POINT('Ctrl Pts',(10.7731522589999,11.6,0.389722418999984));
#193367=CARTESIAN_POINT('Ctrl Pts',(10.7756248599999,15.2,0.390554039999986));
#193368=CARTESIAN_POINT('Ctrl Pts',(10.7756248599999,11.6,0.390554039999986));
#193369=CARTESIAN_POINT('Ctrl Pts',(10.7781024159999,15.2,0.391389675999987));
#193370=CARTESIAN_POINT('Ctrl Pts',(10.7781024159999,11.6,0.391389675999986));
#193371=CARTESIAN_POINT('Ctrl Pts',(10.7805849149999,15.2,0.392229330999987));
#193372=CARTESIAN_POINT('Ctrl Pts',(10.7805849149999,11.6,0.392229330999986));
#193373=CARTESIAN_POINT('Ctrl Pts',(10.7830723399999,15.2,0.393073009999987));
#193374=CARTESIAN_POINT('Ctrl Pts',(10.7830723399999,11.6,0.393073009999986));
#193375=CARTESIAN_POINT('Ctrl Pts',(10.7855646809999,15.2,0.393920716999983));
#193376=CARTESIAN_POINT('Ctrl Pts',(10.7855646809999,11.6,0.393920716999982));
#193377=CARTESIAN_POINT('Ctrl Pts',(10.7880619219999,15.2,0.394772455999988));
#193378=CARTESIAN_POINT('Ctrl Pts',(10.7880619219999,11.6,0.394772455999987));
#193379=CARTESIAN_POINT('Ctrl Pts',(10.7905640509999,15.2,0.395628232999985));
#193380=CARTESIAN_POINT('Ctrl Pts',(10.7905640509999,11.6,0.395628232999985));
#193381=CARTESIAN_POINT('Ctrl Pts',(10.7930710549999,15.2,0.396488051999988));
#193382=CARTESIAN_POINT('Ctrl Pts',(10.7930710549999,11.6,0.396488051999988));
#193383=CARTESIAN_POINT('Ctrl Pts',(10.7955829179999,15.2,0.397351917999984));
#193384=CARTESIAN_POINT('Ctrl Pts',(10.7955829179999,11.6,0.397351917999984));
#193385=CARTESIAN_POINT('Ctrl Pts',(10.7980996289999,15.2,0.398219834999987));
#193386=CARTESIAN_POINT('Ctrl Pts',(10.7980996289999,11.6,0.398219834999986));
#193387=CARTESIAN_POINT('Ctrl Pts',(10.8006211739999,15.2,0.399091808999987));
#193388=CARTESIAN_POINT('Ctrl Pts',(10.8006211739999,11.6,0.399091808999987));
#193389=CARTESIAN_POINT('Ctrl Pts',(10.8031475389999,15.2,0.399967843999987));
#193390=CARTESIAN_POINT('Ctrl Pts',(10.8031475389999,11.6,0.399967843999986));
#193391=CARTESIAN_POINT('Ctrl Pts',(10.8056787119999,15.2,0.400847942999984));
#193392=CARTESIAN_POINT('Ctrl Pts',(10.8056787119999,11.6,0.400847942999984));
#193393=CARTESIAN_POINT('Ctrl Pts',(10.8082146789999,15.2,0.401732112999986));
#193394=CARTESIAN_POINT('Ctrl Pts',(10.8082146789999,11.6,0.401732112999986));
#193395=CARTESIAN_POINT('Ctrl Pts',(10.8107554269999,15.2,0.402620356999983));
#193396=CARTESIAN_POINT('Ctrl Pts',(10.8107554269999,11.6,0.402620356999983));
#193397=CARTESIAN_POINT('Ctrl Pts',(10.8133009429999,15.2,0.403512679999984));
#193398=CARTESIAN_POINT('Ctrl Pts',(10.8133009429999,11.6,0.403512679999984));
#193399=CARTESIAN_POINT('Ctrl Pts',(10.8158512129999,15.2,0.404409085999986));
#193400=CARTESIAN_POINT('Ctrl Pts',(10.8158512129999,11.6,0.404409085999986));
#193401=CARTESIAN_POINT('Ctrl Pts',(10.8184062239999,15.2,0.405309579999984));
#193402=CARTESIAN_POINT('Ctrl Pts',(10.8184062239999,11.6,0.405309579999984));
#193403=CARTESIAN_POINT('Ctrl Pts',(10.8209659639999,15.2,0.406214165999987));
#193404=CARTESIAN_POINT('Ctrl Pts',(10.8209659639999,11.6,0.406214165999987));
#193405=CARTESIAN_POINT('Ctrl Pts',(10.8235304189999,15.2,0.407122848999983));
#193406=CARTESIAN_POINT('Ctrl Pts',(10.8235304189999,11.6,0.407122848999983));
#193407=CARTESIAN_POINT('Ctrl Pts',(10.8260995769999,15.2,0.408035632999986));
#193408=CARTESIAN_POINT('Ctrl Pts',(10.8260995769999,11.6,0.408035632999985));
#193409=CARTESIAN_POINT('Ctrl Pts',(10.8286734229999,15.2,0.408952522999986));
#193410=CARTESIAN_POINT('Ctrl Pts',(10.8286734229999,11.6,0.408952522999985));
#193411=CARTESIAN_POINT('Ctrl Pts',(10.8312519469999,15.2,0.409873522999984));
#193412=CARTESIAN_POINT('Ctrl Pts',(10.8312519469999,11.6,0.409873522999983));
#193413=CARTESIAN_POINT('Ctrl Pts',(10.8338351319999,15.2,0.410798634999985));
#193414=CARTESIAN_POINT('Ctrl Pts',(10.8338351319999,11.6,0.410798634999984));
#193415=CARTESIAN_POINT('Ctrl Pts',(10.8364229689999,15.2,0.411727866999985));
#193416=CARTESIAN_POINT('Ctrl Pts',(10.8364229689999,11.6,0.411727866999984));
#193417=CARTESIAN_POINT('Ctrl Pts',(10.8390154429999,15.2,0.412661221999984));
#193418=CARTESIAN_POINT('Ctrl Pts',(10.8390154429999,11.6,0.412661221999983));
#193419=CARTESIAN_POINT('Ctrl Pts',(10.8416125419999,15.2,0.413598703999987));
#193420=CARTESIAN_POINT('Ctrl Pts',(10.8416125419999,11.6,0.413598703999986));
#193421=CARTESIAN_POINT('Ctrl Pts',(10.8442142529999,15.2,0.414540315999985));
#193422=CARTESIAN_POINT('Ctrl Pts',(10.8442142529999,11.6,0.414540315999985));
#193423=CARTESIAN_POINT('Ctrl Pts',(10.8468205619999,15.2,0.415486064999988));
#193424=CARTESIAN_POINT('Ctrl Pts',(10.8468205619999,11.6,0.415486064999988));
#193425=CARTESIAN_POINT('Ctrl Pts',(10.8494314579999,15.2,0.416435953999983));
#193426=CARTESIAN_POINT('Ctrl Pts',(10.8494314579999,11.6,0.416435953999982));
#193427=CARTESIAN_POINT('Ctrl Pts',(10.8520469269999,15.2,0.417389984999983));
#193428=CARTESIAN_POINT('Ctrl Pts',(10.8520469269999,11.6,0.417389984999982));
#193429=CARTESIAN_POINT('Ctrl Pts',(10.8546669569999,15.2,0.418348164999984));
#193430=CARTESIAN_POINT('Ctrl Pts',(10.8546669569999,11.6,0.418348164999984));
#193431=CARTESIAN_POINT('Ctrl Pts',(10.8572915349999,15.2,0.419310497999987));
#193432=CARTESIAN_POINT('Ctrl Pts',(10.8572915349999,11.6,0.419310497999987));
#193433=CARTESIAN_POINT('Ctrl Pts',(10.8599206479999,15.2,0.420276986999983));
#193434=CARTESIAN_POINT('Ctrl Pts',(10.8599206479999,11.6,0.420276986999983));
#193435=CARTESIAN_POINT('Ctrl Pts',(10.8625542849999,15.2,0.421247635999986));
#193436=CARTESIAN_POINT('Ctrl Pts',(10.8625542849999,11.6,0.421247635999986));
#193437=CARTESIAN_POINT('Ctrl Pts',(10.8651924309999,15.2,0.422222449999987));
#193438=CARTESIAN_POINT('Ctrl Pts',(10.8651924309999,11.6,0.422222449999987));
#193439=CARTESIAN_POINT('Ctrl Pts',(10.8678350749999,15.2,0.423201432999987));
#193440=CARTESIAN_POINT('Ctrl Pts',(10.8678350749999,11.6,0.423201432999986));
#193441=CARTESIAN_POINT('Ctrl Pts',(10.8704822049999,15.2,0.424184587999985));
#193442=CARTESIAN_POINT('Ctrl Pts',(10.8704822049999,11.6,0.424184587999985));
#193443=CARTESIAN_POINT('Ctrl Pts',(10.8731338059999,15.2,0.425171920999983));
#193444=CARTESIAN_POINT('Ctrl Pts',(10.8731338059999,11.6,0.425171920999982));
#193445=CARTESIAN_POINT('Ctrl Pts',(10.8757898679999,15.2,0.426163433999989));
#193446=CARTESIAN_POINT('Ctrl Pts',(10.8757898679999,11.6,0.426163433999988));
#193447=CARTESIAN_POINT('Ctrl Pts',(10.8784503779999,15.2,0.427159131999986));
#193448=CARTESIAN_POINT('Ctrl Pts',(10.8784503779999,11.6,0.427159131999985));
#193449=CARTESIAN_POINT('Ctrl Pts',(10.8811153219999,15.2,0.428159017999987));
#193450=CARTESIAN_POINT('Ctrl Pts',(10.8811153219999,11.6,0.428159017999987));
#193451=CARTESIAN_POINT('Ctrl Pts',(10.8837846889999,15.2,0.429163097999985));
#193452=CARTESIAN_POINT('Ctrl Pts',(10.8837846889999,11.6,0.429163097999985));
#193453=CARTESIAN_POINT('Ctrl Pts',(10.8864584659999,15.2,0.430171373999984));
#193454=CARTESIAN_POINT('Ctrl Pts',(10.8864584659999,11.6,0.430171373999983));
#193455=CARTESIAN_POINT('Ctrl Pts',(10.8891366429999,15.2,0.431183849999983));
#193456=CARTESIAN_POINT('Ctrl Pts',(10.8891366429999,11.6,0.431183849999983));
#193457=CARTESIAN_POINT('Ctrl Pts',(10.8918192029999,15.2,0.432200530999989));
#193458=CARTESIAN_POINT('Ctrl Pts',(10.8918192029999,11.6,0.432200530999988));
#193459=CARTESIAN_POINT('Ctrl Pts',(10.8945061379999,15.2,0.433221420999987));
#193460=CARTESIAN_POINT('Ctrl Pts',(10.8945061379999,11.6,0.433221420999987));
#193461=CARTESIAN_POINT('Ctrl Pts',(10.8971974329999,15.2,0.434246522999988));
#193462=CARTESIAN_POINT('Ctrl Pts',(10.8971974329999,11.6,0.434246522999988));
#193463=CARTESIAN_POINT('Ctrl Pts',(10.8998930779999,15.2,0.435275839999987));
#193464=CARTESIAN_POINT('Ctrl Pts',(10.8998930779999,11.6,0.435275839999986));
#193465=CARTESIAN_POINT('Ctrl Pts',(10.9025930589999,15.2,0.436309378999984));
#193466=CARTESIAN_POINT('Ctrl Pts',(10.9025930589999,11.6,0.436309378999983));
#193467=CARTESIAN_POINT('Ctrl Pts',(10.9052973639999,15.2,0.437347140999984));
#193468=CARTESIAN_POINT('Ctrl Pts',(10.9052973639999,11.6,0.437347140999984));
#193469=CARTESIAN_POINT('Ctrl Pts',(10.9080059809999,15.2,0.438389129999983));
#193470=CARTESIAN_POINT('Ctrl Pts',(10.9080059809999,11.6,0.438389129999983));
#193471=CARTESIAN_POINT('Ctrl Pts',(10.9107188979999,15.2,0.439435350999986));
#193472=CARTESIAN_POINT('Ctrl Pts',(10.9107188979999,11.6,0.439435350999986));
#193473=CARTESIAN_POINT('Ctrl Pts',(10.9134361039999,15.2,0.440485805999984));
#193474=CARTESIAN_POINT('Ctrl Pts',(10.9134361039999,11.6,0.440485805999983));
#193475=CARTESIAN_POINT('Ctrl Pts',(10.9161575839999,15.2,0.441540500999986));
#193476=CARTESIAN_POINT('Ctrl Pts',(10.9161575839999,11.6,0.441540500999986));
#193477=CARTESIAN_POINT('Ctrl Pts',(10.9188833299999,15.2,0.442599438999984));
#193478=CARTESIAN_POINT('Ctrl Pts',(10.9188833299999,11.6,0.442599438999984));
#193479=CARTESIAN_POINT('Ctrl Pts',(10.9216133259999,15.2,0.443662621999987));
#193480=CARTESIAN_POINT('Ctrl Pts',(10.9216133259999,11.6,0.443662621999987));
#193481=CARTESIAN_POINT('Ctrl Pts',(10.9243475619999,15.2,0.444730056999987));
#193482=CARTESIAN_POINT('Ctrl Pts',(10.9243475619999,11.6,0.444730056999986));
#193483=CARTESIAN_POINT('Ctrl Pts',(10.9270860269999,15.2,0.445801742999983));
#193484=CARTESIAN_POINT('Ctrl Pts',(10.9270860269999,11.6,0.445801742999982));
#193485=CARTESIAN_POINT('Ctrl Pts',(10.9298287059999,15.2,0.446877687999985));
#193486=CARTESIAN_POINT('Ctrl Pts',(10.9298287059999,11.6,0.446877687999984));
#193487=CARTESIAN_POINT('Ctrl Pts',(10.9325755889999,15.2,0.447957893999984));
#193488=CARTESIAN_POINT('Ctrl Pts',(10.9325755889999,11.6,0.447957893999984));
#193489=CARTESIAN_POINT('Ctrl Pts',(10.9353266639999,15.2,0.449042364999985));
#193490=CARTESIAN_POINT('Ctrl Pts',(10.9353266639999,11.6,0.449042364999985));
#193491=CARTESIAN_POINT('Ctrl Pts',(10.9380819189999,15.2,0.450131101999984));
#193492=CARTESIAN_POINT('Ctrl Pts',(10.9380819189999,11.6,0.450131101999984));
#193493=CARTESIAN_POINT('Ctrl Pts',(10.9408413419999,15.2,0.451224112999986));
#193494=CARTESIAN_POINT('Ctrl Pts',(10.9408413419999,11.6,0.451224112999986));
#193495=CARTESIAN_POINT('Ctrl Pts',(10.9436049209999,15.2,0.452321397999986));
#193496=CARTESIAN_POINT('Ctrl Pts',(10.9436049209999,11.6,0.452321397999986));
#193497=CARTESIAN_POINT('Ctrl Pts',(10.9463726449999,15.2,0.453422962999985));
#193498=CARTESIAN_POINT('Ctrl Pts',(10.9463726449999,11.6,0.453422962999985));
#193499=CARTESIAN_POINT('Ctrl Pts',(10.9491445009999,15.2,0.454528808999988));
#193500=CARTESIAN_POINT('Ctrl Pts',(10.9491445009999,11.6,0.454528808999987));
#193501=CARTESIAN_POINT('Ctrl Pts',(10.9519204779999,15.2,0.455638941999985));
#193502=CARTESIAN_POINT('Ctrl Pts',(10.9519204779999,11.6,0.455638941999985));
#193503=CARTESIAN_POINT('Ctrl Pts',(10.9547005639999,15.2,0.456753363999987));
#193504=CARTESIAN_POINT('Ctrl Pts',(10.9547005639999,11.6,0.456753363999986));
#193505=CARTESIAN_POINT('Ctrl Pts',(10.9574847479999,15.2,0.457872078999984));
#193506=CARTESIAN_POINT('Ctrl Pts',(10.9574847479999,11.6,0.457872078999983));
#193507=CARTESIAN_POINT('Ctrl Pts',(10.9602730159999,15.2,0.458995089999985));
#193508=CARTESIAN_POINT('Ctrl Pts',(10.9602730159999,11.6,0.458995089999985));
#193509=CARTESIAN_POINT('Ctrl Pts',(10.9630653589999,15.2,0.460122401999987));
#193510=CARTESIAN_POINT('Ctrl Pts',(10.9630653589999,11.6,0.460122401999987));
#193511=CARTESIAN_POINT('Ctrl Pts',(10.9658617639999,15.2,0.461254016999986));
#193512=CARTESIAN_POINT('Ctrl Pts',(10.9658617639999,11.6,0.461254016999985));
#193513=CARTESIAN_POINT('Ctrl Pts',(10.9686622189999,15.2,0.462389937999985));
#193514=CARTESIAN_POINT('Ctrl Pts',(10.9686622189999,11.6,0.462389937999985));
#193515=CARTESIAN_POINT('Ctrl Pts',(10.9714667139999,15.2,0.463530168999986));
#193516=CARTESIAN_POINT('Ctrl Pts',(10.9714667139999,11.6,0.463530168999986));
#193517=CARTESIAN_POINT('Ctrl Pts',(10.9742752359999,15.2,0.464674713999984));
#193518=CARTESIAN_POINT('Ctrl Pts',(10.9742752359999,11.6,0.464674713999984));
#193519=CARTESIAN_POINT('Ctrl Pts',(10.9770877739999,15.2,0.465823574999984));
#193520=CARTESIAN_POINT('Ctrl Pts',(10.9770877739999,11.6,0.465823574999984));
#193521=CARTESIAN_POINT('Ctrl Pts',(10.9799043159999,15.2,0.466976757999986));
#193522=CARTESIAN_POINT('Ctrl Pts',(10.9799043159999,11.6,0.466976757999986));
#193523=CARTESIAN_POINT('Ctrl Pts',(10.9827248519999,15.2,0.468134262999986));
#193524=CARTESIAN_POINT('Ctrl Pts',(10.9827248519999,11.6,0.468134262999986));
#193525=CARTESIAN_POINT('Ctrl Pts',(10.9855493679999,15.2,0.469296094999985));
#193526=CARTESIAN_POINT('Ctrl Pts',(10.9855493679999,11.6,0.469296094999984));
#193527=CARTESIAN_POINT('Ctrl Pts',(10.9883778529999,15.2,0.470462257999986));
#193528=CARTESIAN_POINT('Ctrl Pts',(10.9883778529999,11.6,0.470462257999986));
#193529=CARTESIAN_POINT('Ctrl Pts',(10.9912102979999,15.2,0.471632752999986));
#193530=CARTESIAN_POINT('Ctrl Pts',(10.9912102979999,11.6,0.471632752999986));
#193531=CARTESIAN_POINT('Ctrl Pts',(10.9940466899999,15.2,0.472807584999986));
#193532=CARTESIAN_POINT('Ctrl Pts',(10.9940466899999,11.6,0.472807584999985));
#193533=CARTESIAN_POINT('Ctrl Pts',(10.9968870169999,15.2,0.473986756999984));
#193534=CARTESIAN_POINT('Ctrl Pts',(10.9968870169999,11.6,0.473986756999984));
#193535=CARTESIAN_POINT('Ctrl Pts',(10.9997312679999,15.2,0.475170272999983));
#193536=CARTESIAN_POINT('Ctrl Pts',(10.9997312679999,11.6,0.475170272999982));
#193537=CARTESIAN_POINT('Ctrl Pts',(11.0025794309999,15.2,0.476358134999986));
#193538=CARTESIAN_POINT('Ctrl Pts',(11.0025794309999,11.6,0.476358134999985));
#193539=CARTESIAN_POINT('Ctrl Pts',(11.0054314969999,15.2,0.477550345999984));
#193540=CARTESIAN_POINT('Ctrl Pts',(11.0054314969999,11.6,0.477550345999984));
#193541=CARTESIAN_POINT('Ctrl Pts',(11.0082874519999,15.2,0.478746909999987));
#193542=CARTESIAN_POINT('Ctrl Pts',(11.0082874519999,11.6,0.478746909999987));
#193543=CARTESIAN_POINT('Ctrl Pts',(11.0111472859999,15.2,0.479947829999983));
#193544=CARTESIAN_POINT('Ctrl Pts',(11.0111472859999,11.6,0.479947829999982));
#193545=CARTESIAN_POINT('Ctrl Pts',(11.0140109889999,15.2,0.481153109999983));
#193546=CARTESIAN_POINT('Ctrl Pts',(11.0140109889999,11.6,0.481153109999983));
#193547=CARTESIAN_POINT('Ctrl Pts',(11.0168785469999,15.2,0.482362750999985));
#193548=CARTESIAN_POINT('Ctrl Pts',(11.0168785469999,11.6,0.482362750999985));
#193549=CARTESIAN_POINT('Ctrl Pts',(11.0197499499999,15.2,0.483576758999984));
#193550=CARTESIAN_POINT('Ctrl Pts',(11.0197499499999,11.6,0.483576758999984));
#193551=CARTESIAN_POINT('Ctrl Pts',(11.0226251869999,15.2,0.484795133999985));
#193552=CARTESIAN_POINT('Ctrl Pts',(11.0226251869999,11.6,0.484795133999984));
#193553=CARTESIAN_POINT('Ctrl Pts',(11.0255042469999,15.2,0.486017880999987));
#193554=CARTESIAN_POINT('Ctrl Pts',(11.0255042469999,11.6,0.486017880999987));
#193555=CARTESIAN_POINT('Ctrl Pts',(11.0283871179999,15.2,0.487245001999987));
#193556=CARTESIAN_POINT('Ctrl Pts',(11.0283871179999,11.6,0.487245001999987));
#193557=CARTESIAN_POINT('Ctrl Pts',(11.0312737899999,15.2,0.488476501999986));
#193558=CARTESIAN_POINT('Ctrl Pts',(11.0312737899999,11.6,0.488476501999985));
#193559=CARTESIAN_POINT('Ctrl Pts',(11.0341642509999,15.2,0.489712382999983));
#193560=CARTESIAN_POINT('Ctrl Pts',(11.0341642509999,11.6,0.489712382999982));
#193561=CARTESIAN_POINT('Ctrl Pts',(11.0370584909999,15.2,0.490952646999983));
#193562=CARTESIAN_POINT('Ctrl Pts',(11.0370584909999,11.6,0.490952646999982));
#193563=CARTESIAN_POINT('Ctrl Pts',(11.0399564969999,15.2,0.492197297999986));
#193564=CARTESIAN_POINT('Ctrl Pts',(11.0399564969999,11.6,0.492197297999985));
#193565=CARTESIAN_POINT('Ctrl Pts',(11.0428582599999,15.2,0.493446338999988));
#193566=CARTESIAN_POINT('Ctrl Pts',(11.0428582599999,11.6,0.493446338999987));
#193567=CARTESIAN_POINT('Ctrl Pts',(11.0457637679999,15.2,0.494699771999985));
#193568=CARTESIAN_POINT('Ctrl Pts',(11.0457637679999,11.6,0.494699771999984));
#193569=CARTESIAN_POINT('Ctrl Pts',(11.0486730089999,15.2,0.495957601999986));
#193570=CARTESIAN_POINT('Ctrl Pts',(11.0486730089999,11.6,0.495957601999985));
#193571=CARTESIAN_POINT('Ctrl Pts',(11.0515859739999,15.2,0.497219829999986));
#193572=CARTESIAN_POINT('Ctrl Pts',(11.0515859739999,11.6,0.497219829999986));
#193573=CARTESIAN_POINT('Ctrl Pts',(11.0545026509999,15.2,0.498486459999987));
#193574=CARTESIAN_POINT('Ctrl Pts',(11.0545026509999,11.6,0.498486459999987));
#193575=CARTESIAN_POINT('Ctrl Pts',(11.0574230279999,15.2,0.499757494999984));
#193576=CARTESIAN_POINT('Ctrl Pts',(11.0574230279999,11.6,0.499757494999983));
#193577=CARTESIAN_POINT('Ctrl Pts',(11.0603470969999,15.2,0.501032936999986));
#193578=CARTESIAN_POINT('Ctrl Pts',(11.0603470969999,11.6,0.501032936999985));
#193579=CARTESIAN_POINT('Ctrl Pts',(11.0632748429999,15.2,0.502312789999984));
#193580=CARTESIAN_POINT('Ctrl Pts',(11.0632748429999,11.6,0.502312789999983));
#193581=CARTESIAN_POINT('Ctrl Pts',(11.0662062589999,15.2,0.503597055999983));
#193582=CARTESIAN_POINT('Ctrl Pts',(11.0662062589999,11.6,0.503597055999982));
#193583=CARTESIAN_POINT('Ctrl Pts',(11.0691413309999,15.2,0.504885737999987));
#193584=CARTESIAN_POINT('Ctrl Pts',(11.0691413309999,11.6,0.504885737999987));
#193585=CARTESIAN_POINT('Ctrl Pts',(11.0720800509999,15.2,0.506178839999984));
#193586=CARTESIAN_POINT('Ctrl Pts',(11.0720800509999,11.6,0.506178839999984));
#193587=CARTESIAN_POINT('Ctrl Pts',(11.0750224069999,15.2,0.507476362999988));
#193588=CARTESIAN_POINT('Ctrl Pts',(11.0750224069999,11.6,0.507476362999987));
#193589=CARTESIAN_POINT('Ctrl Pts',(11.0779683879999,15.2,0.508778310999984));
#193590=CARTESIAN_POINT('Ctrl Pts',(11.0779683879999,11.6,0.508778310999984));
#193591=CARTESIAN_POINT('Ctrl Pts',(11.0809179819999,15.2,0.510084686999988));
#193592=CARTESIAN_POINT('Ctrl Pts',(11.0809179819999,11.6,0.510084686999987));
#193593=CARTESIAN_POINT('Ctrl Pts',(11.0838711809999,15.2,0.511395492999984));
#193594=CARTESIAN_POINT('Ctrl Pts',(11.0838711809999,11.6,0.511395492999984));
#193595=CARTESIAN_POINT('Ctrl Pts',(11.0868279709999,15.2,0.512710731999988));
#193596=CARTESIAN_POINT('Ctrl Pts',(11.0868279709999,11.6,0.512710731999988));
#193597=CARTESIAN_POINT('Ctrl Pts',(11.0897883439999,15.2,0.514030406999986));
#193598=CARTESIAN_POINT('Ctrl Pts',(11.0897883439999,11.6,0.514030406999985));
#193599=CARTESIAN_POINT('Ctrl Pts',(11.0927522879999,15.2,0.515354519999986));
#193600=CARTESIAN_POINT('Ctrl Pts',(11.0927522879999,11.6,0.515354519999986));
#193601=CARTESIAN_POINT('Ctrl Pts',(11.0957197919999,15.2,0.516683075999986));
#193602=CARTESIAN_POINT('Ctrl Pts',(11.0957197919999,11.6,0.516683075999986));
#193603=CARTESIAN_POINT('Ctrl Pts',(11.0986908469999,15.2,0.518016075999985));
#193604=CARTESIAN_POINT('Ctrl Pts',(11.0986908469999,11.6,0.518016075999985));
#193605=CARTESIAN_POINT('Ctrl Pts',(11.1016654419999,15.2,0.519353521999988));
#193606=CARTESIAN_POINT('Ctrl Pts',(11.1016654419999,11.6,0.519353521999987));
#193607=CARTESIAN_POINT('Ctrl Pts',(11.1046435639999,15.2,0.520695417999986));
#193608=CARTESIAN_POINT('Ctrl Pts',(11.1046435639999,11.6,0.520695417999985));
#193609=CARTESIAN_POINT('Ctrl Pts',(11.1076252049999,15.2,0.522041765999983));
#193610=CARTESIAN_POINT('Ctrl Pts',(11.1076252049999,11.6,0.522041765999983));
#193611=CARTESIAN_POINT('Ctrl Pts',(11.1106103519999,15.2,0.523392568999985));
#193612=CARTESIAN_POINT('Ctrl Pts',(11.1106103519999,11.6,0.523392568999985));
#193613=CARTESIAN_POINT('Ctrl Pts',(11.1135989969999,15.2,0.524747829999987));
#193614=CARTESIAN_POINT('Ctrl Pts',(11.1135989969999,11.6,0.524747829999987));
#193615=CARTESIAN_POINT('Ctrl Pts',(11.1165911289999,15.2,0.526107550999986));
#193616=CARTESIAN_POINT('Ctrl Pts',(11.1165911289999,11.6,0.526107550999985));
#193617=CARTESIAN_POINT('Ctrl Pts',(11.1195867359999,15.2,0.527471733999985));
#193618=CARTESIAN_POINT('Ctrl Pts',(11.1195867359999,11.6,0.527471733999984));
#193619=CARTESIAN_POINT('Ctrl Pts',(11.1225858069999,15.2,0.528840383999984));
#193620=CARTESIAN_POINT('Ctrl Pts',(11.1225858069999,11.6,0.528840383999984));
#193621=CARTESIAN_POINT('Ctrl Pts',(11.1255883349999,15.2,0.530213501999985));
#193622=CARTESIAN_POINT('Ctrl Pts',(11.1255883349999,11.6,0.530213501999985));
#193623=CARTESIAN_POINT('Ctrl Pts',(11.1285943059999,15.2,0.531591089999988));
#193624=CARTESIAN_POINT('Ctrl Pts',(11.1285943059999,11.6,0.531591089999987));
#193625=CARTESIAN_POINT('Ctrl Pts',(11.1316037109999,15.2,0.532973150999982));
#193626=CARTESIAN_POINT('Ctrl Pts',(11.1316037109999,11.6,0.532973150999982));
#193627=CARTESIAN_POINT('Ctrl Pts',(11.1346165399999,15.2,0.534359688999988));
#193628=CARTESIAN_POINT('Ctrl Pts',(11.1346165399999,11.6,0.534359688999988));
#193629=CARTESIAN_POINT('Ctrl Pts',(11.1376327809999,15.2,0.535750703999986));
#193630=CARTESIAN_POINT('Ctrl Pts',(11.1376327809999,11.6,0.535750703999986));
#193631=CARTESIAN_POINT('Ctrl Pts',(11.1406524249999,15.2,0.537146200999987));
#193632=CARTESIAN_POINT('Ctrl Pts',(11.1406524249999,11.6,0.537146200999987));
#193633=CARTESIAN_POINT('Ctrl Pts',(11.1436754609999,15.2,0.538546180999986));
#193634=CARTESIAN_POINT('Ctrl Pts',(11.1436754609999,11.6,0.538546180999985));
#193635=CARTESIAN_POINT('Ctrl Pts',(11.1467018789999,15.2,0.539950646999987));
#193636=CARTESIAN_POINT('Ctrl Pts',(11.1467018789999,11.6,0.539950646999987));
#193637=CARTESIAN_POINT('Ctrl Pts',(11.1497316689999,15.2,0.541359601999982));
#193638=CARTESIAN_POINT('Ctrl Pts',(11.1497316689999,11.6,0.541359601999982));
#193639=CARTESIAN_POINT('Ctrl Pts',(11.1527648199999,15.2,0.542773047999985));
#193640=CARTESIAN_POINT('Ctrl Pts',(11.1527648199999,11.6,0.542773047999984));
#193641=CARTESIAN_POINT('Ctrl Pts',(11.1558013209999,15.2,0.544190986999986));
#193642=CARTESIAN_POINT('Ctrl Pts',(11.1558013209999,11.6,0.544190986999986));
#193643=CARTESIAN_POINT('Ctrl Pts',(11.1588411629999,15.2,0.545613420999986));
#193644=CARTESIAN_POINT('Ctrl Pts',(11.1588411629999,11.6,0.545613420999986));
#193645=CARTESIAN_POINT('Ctrl Pts',(11.1618843359999,15.2,0.547040353999986));
#193646=CARTESIAN_POINT('Ctrl Pts',(11.1618843359999,11.6,0.547040353999985));
#193647=CARTESIAN_POINT('Ctrl Pts',(11.1649308279999,15.2,0.548471788999985));
#193648=CARTESIAN_POINT('Ctrl Pts',(11.1649308279999,11.6,0.548471788999984));
#193649=CARTESIAN_POINT('Ctrl Pts',(11.1679806309999,15.2,0.549907724999983));
#193650=CARTESIAN_POINT('Ctrl Pts',(11.1679806309999,11.6,0.549907724999982));
#193651=CARTESIAN_POINT('Ctrl Pts',(11.1710337319999,15.2,0.551348167999985));
#193652=CARTESIAN_POINT('Ctrl Pts',(11.1710337319999,11.6,0.551348167999985));
#193653=CARTESIAN_POINT('Ctrl Pts',(11.1740901229999,15.2,0.552793118999984));
#193654=CARTESIAN_POINT('Ctrl Pts',(11.1740901229999,11.6,0.552793118999983));
#193655=CARTESIAN_POINT('Ctrl Pts',(11.1771497949999,15.2,0.554242579999986));
#193656=CARTESIAN_POINT('Ctrl Pts',(11.1771497949999,11.6,0.554242579999986));
#193657=CARTESIAN_POINT('Ctrl Pts',(11.1802127339999,15.2,0.555696553999985));
#193658=CARTESIAN_POINT('Ctrl Pts',(11.1802127339999,11.6,0.555696553999984));
#193659=CARTESIAN_POINT('Ctrl Pts',(11.1832789319999,15.2,0.557155042999984));
#193660=CARTESIAN_POINT('Ctrl Pts',(11.1832789319999,11.6,0.557155042999983));
#193661=CARTESIAN_POINT('Ctrl Pts',(11.1863483789999,15.2,0.558618048999988));
#193662=CARTESIAN_POINT('Ctrl Pts',(11.1863483789999,11.6,0.558618048999988));
#193663=CARTESIAN_POINT('Ctrl Pts',(11.1894210649999,15.2,0.560085574999984));
#193664=CARTESIAN_POINT('Ctrl Pts',(11.1894210649999,11.6,0.560085574999984));
#193665=CARTESIAN_POINT('Ctrl Pts',(11.1924969799999,15.2,0.561557623999986));
#193666=CARTESIAN_POINT('Ctrl Pts',(11.1924969799999,11.6,0.561557623999986));
#193667=CARTESIAN_POINT('Ctrl Pts',(11.1955761109999,15.2,0.563034195999985));
#193668=CARTESIAN_POINT('Ctrl Pts',(11.1955761109999,11.6,0.563034195999985));
#193669=CARTESIAN_POINT('Ctrl Pts',(11.1986584539999,15.2,0.564515295999986));
#193670=CARTESIAN_POINT('Ctrl Pts',(11.1986584539999,11.6,0.564515295999985));
#193671=CARTESIAN_POINT('Ctrl Pts',(11.2017439929999,15.2,0.566000923999983));
#193672=CARTESIAN_POINT('Ctrl Pts',(11.2017439929999,11.6,0.566000923999983));
#193673=CARTESIAN_POINT('Ctrl Pts',(11.2048327209999,15.2,0.567491083999982));
#193674=CARTESIAN_POINT('Ctrl Pts',(11.2048327209999,11.6,0.567491083999982));
#193675=CARTESIAN_POINT('Ctrl Pts',(11.2079246269999,15.2,0.568985776999984));
#193676=CARTESIAN_POINT('Ctrl Pts',(11.2079246269999,11.6,0.568985776999984));
#193677=CARTESIAN_POINT('Ctrl Pts',(11.2110197019999,15.2,0.570485004999988));
#193678=CARTESIAN_POINT('Ctrl Pts',(11.2110197019999,11.6,0.570485004999987));
#193679=CARTESIAN_POINT('Ctrl Pts',(11.2141179349999,15.2,0.571988772999985));
#193680=CARTESIAN_POINT('Ctrl Pts',(11.2141179349999,11.6,0.571988772999985));
#193681=CARTESIAN_POINT('Ctrl Pts',(11.2172193169999,15.2,0.573497079999985));
#193682=CARTESIAN_POINT('Ctrl Pts',(11.2172193169999,11.6,0.573497079999985));
#193683=CARTESIAN_POINT('Ctrl Pts',(11.2203238359999,15.2,0.575009928999983));
#193684=CARTESIAN_POINT('Ctrl Pts',(11.2203238359999,11.6,0.575009928999983));
#193685=CARTESIAN_POINT('Ctrl Pts',(11.2234314849999,15.2,0.576527321999984));
#193686=CARTESIAN_POINT('Ctrl Pts',(11.2234314849999,11.6,0.576527321999984));
#193687=CARTESIAN_POINT('Ctrl Pts',(11.2265422519999,15.2,0.578049263999985));
#193688=CARTESIAN_POINT('Ctrl Pts',(11.2265422519999,11.6,0.578049263999984));
#193689=CARTESIAN_POINT('Ctrl Pts',(11.2296561279999,15.2,0.579575753999984));
#193690=CARTESIAN_POINT('Ctrl Pts',(11.2296561279999,11.6,0.579575753999983));
#193691=CARTESIAN_POINT('Ctrl Pts',(11.2327731029999,15.2,0.581106793999986));
#193692=CARTESIAN_POINT('Ctrl Pts',(11.2327731029999,11.6,0.581106793999985));
#193693=CARTESIAN_POINT('Ctrl Pts',(11.2358931669999,15.2,0.582642387999983));
#193694=CARTESIAN_POINT('Ctrl Pts',(11.2358931669999,11.6,0.582642387999983));
#193695=CARTESIAN_POINT('Ctrl Pts',(11.2390163099999,15.2,0.584182537999984));
#193696=CARTESIAN_POINT('Ctrl Pts',(11.2390163099999,11.6,0.584182537999984));
#193697=CARTESIAN_POINT('Ctrl Pts',(11.2421425229999,15.2,0.585727244999985));
#193698=CARTESIAN_POINT('Ctrl Pts',(11.2421425229999,11.6,0.585727244999985));
#193699=CARTESIAN_POINT('Ctrl Pts',(11.2452717949999,15.2,0.587276511999986));
#193700=CARTESIAN_POINT('Ctrl Pts',(11.2452717949999,11.6,0.587276511999985));
#193701=CARTESIAN_POINT('Ctrl Pts',(11.2484041159999,15.2,0.588830339999986));
#193702=CARTESIAN_POINT('Ctrl Pts',(11.2484041159999,11.6,0.588830339999986));
#193703=CARTESIAN_POINT('Ctrl Pts',(11.2515394779999,15.2,0.590388731999987));
#193704=CARTESIAN_POINT('Ctrl Pts',(11.2515394779999,11.6,0.590388731999986));
#193705=CARTESIAN_POINT('Ctrl Pts',(11.2546778709999,15.2,0.591951689999988));
#193706=CARTESIAN_POINT('Ctrl Pts',(11.2546778709999,11.6,0.591951689999987));
#193707=CARTESIAN_POINT('Ctrl Pts',(11.2578192829999,15.2,0.593519215999985));
#193708=CARTESIAN_POINT('Ctrl Pts',(11.2578192829999,11.6,0.593519215999984));
#193709=CARTESIAN_POINT('Ctrl Pts',(11.2609637079999,15.2,0.595091311999987));
#193710=CARTESIAN_POINT('Ctrl Pts',(11.2609637079999,11.6,0.595091311999986));
#193711=CARTESIAN_POINT('Ctrl Pts',(11.2641111319999,15.2,0.596667980999985));
#193712=CARTESIAN_POINT('Ctrl Pts',(11.2641111319999,11.6,0.596667980999985));
#193713=CARTESIAN_POINT('Ctrl Pts',(11.2672615479999,15.2,0.598249222999985));
#193714=CARTESIAN_POINT('Ctrl Pts',(11.2672615479999,11.6,0.598249222999984));
#193715=CARTESIAN_POINT('Ctrl Pts',(11.2704149449999,15.2,0.599835040999985));
#193716=CARTESIAN_POINT('Ctrl Pts',(11.2704149449999,11.6,0.599835040999985));
#193717=CARTESIAN_POINT('Ctrl Pts',(11.2735713159999,15.2,0.601425437999983));
#193718=CARTESIAN_POINT('Ctrl Pts',(11.2735713159999,11.6,0.601425437999982));
#193719=CARTESIAN_POINT('Ctrl Pts',(11.2767306479999,15.2,0.603020413999986));
#193720=CARTESIAN_POINT('Ctrl Pts',(11.2767306479999,11.6,0.603020413999986));
#193721=CARTESIAN_POINT('Ctrl Pts',(11.2798929329999,15.2,0.604619971999987));
#193722=CARTESIAN_POINT('Ctrl Pts',(11.2798929329999,11.6,0.604619971999986));
#193723=CARTESIAN_POINT('Ctrl Pts',(11.2830581619999,15.2,0.606224114999985));
#193724=CARTESIAN_POINT('Ctrl Pts',(11.2830581619999,11.6,0.606224114999984));
#193725=CARTESIAN_POINT('Ctrl Pts',(11.2862263229999,15.2,0.607832843999985));
#193726=CARTESIAN_POINT('Ctrl Pts',(11.2862263229999,11.6,0.607832843999984));
#193727=CARTESIAN_POINT('Ctrl Pts',(11.2893974099999,15.2,0.609446159999987));
#193728=CARTESIAN_POINT('Ctrl Pts',(11.2893974099999,11.6,0.609446159999986));
#193729=CARTESIAN_POINT('Ctrl Pts',(11.2925714099999,15.2,0.611064066999987));
#193730=CARTESIAN_POINT('Ctrl Pts',(11.2925714099999,11.6,0.611064066999986));
#193731=CARTESIAN_POINT('Ctrl Pts',(11.2957483149999,15.2,0.612686564999985));
#193732=CARTESIAN_POINT('Ctrl Pts',(11.2957483149999,11.6,0.612686564999984));
#193733=CARTESIAN_POINT('Ctrl Pts',(11.2989281149999,15.2,0.614313657999985));
#193734=CARTESIAN_POINT('Ctrl Pts',(11.2989281149999,11.6,0.614313657999985));
#193735=CARTESIAN_POINT('Ctrl Pts',(11.3021108019999,15.2,0.615945344999984));
#193736=CARTESIAN_POINT('Ctrl Pts',(11.3021108019999,11.6,0.615945344999984));
#193737=CARTESIAN_POINT('Ctrl Pts',(11.3052963649999,15.2,0.617581629999986));
#193738=CARTESIAN_POINT('Ctrl Pts',(11.3052963649999,11.6,0.617581629999985));
#193739=CARTESIAN_POINT('Ctrl Pts',(11.3084847949999,15.2,0.619222514999986));
#193740=CARTESIAN_POINT('Ctrl Pts',(11.3084847949999,11.6,0.619222514999986));
#193741=CARTESIAN_POINT('Ctrl Pts',(11.3116760819999,15.2,0.620868000999986));
#193742=CARTESIAN_POINT('Ctrl Pts',(11.3116760819999,11.6,0.620868000999985));
#193743=CARTESIAN_POINT('Ctrl Pts',(11.3148702169999,15.2,0.622518089999984));
#193744=CARTESIAN_POINT('Ctrl Pts',(11.3148702169999,11.6,0.622518089999983));
#193745=CARTESIAN_POINT('Ctrl Pts',(11.3180671909999,15.2,0.624172784999986));
#193746=CARTESIAN_POINT('Ctrl Pts',(11.3180671909999,11.6,0.624172784999985));
#193747=CARTESIAN_POINT('Ctrl Pts',(11.3212669929999,15.2,0.625832085999987));
#193748=CARTESIAN_POINT('Ctrl Pts',(11.3212669929999,11.6,0.625832085999986));
#193749=CARTESIAN_POINT('Ctrl Pts',(11.3244696159999,15.2,0.627495995999983));
#193750=CARTESIAN_POINT('Ctrl Pts',(11.3244696159999,11.6,0.627495995999982));
#193751=CARTESIAN_POINT('Ctrl Pts',(11.3276750489999,15.2,0.629164515999987));
#193752=CARTESIAN_POINT('Ctrl Pts',(11.3276750489999,11.6,0.629164515999987));
#193753=CARTESIAN_POINT('Ctrl Pts',(11.3308832819999,15.2,0.630837647999982));
#193754=CARTESIAN_POINT('Ctrl Pts',(11.3308832819999,11.6,0.630837647999982));
#193755=CARTESIAN_POINT('Ctrl Pts',(11.3340943069999,15.2,0.632515394999986));
#193756=CARTESIAN_POINT('Ctrl Pts',(11.3340943069999,11.6,0.632515394999986));
#193757=CARTESIAN_POINT('Ctrl Pts',(11.3373081149999,15.2,0.634197756999986));
#193758=CARTESIAN_POINT('Ctrl Pts',(11.3373081149999,11.6,0.634197756999985));
#193759=CARTESIAN_POINT('Ctrl Pts',(11.3405246939999,15.2,0.635884737999985));
#193760=CARTESIAN_POINT('Ctrl Pts',(11.3405246939999,11.6,0.635884737999985));
#193761=CARTESIAN_POINT('Ctrl Pts',(11.3437440379999,15.2,0.637576336999985));
#193762=CARTESIAN_POINT('Ctrl Pts',(11.3437440379999,11.6,0.637576336999985));
#193763=CARTESIAN_POINT('Ctrl Pts',(11.3469661359999,15.2,0.639272557999986));
#193764=CARTESIAN_POINT('Ctrl Pts',(11.3469661359999,11.6,0.639272557999985));
#193765=CARTESIAN_POINT('Ctrl Pts',(11.3501909789999,15.2,0.640973401999982));
#193766=CARTESIAN_POINT('Ctrl Pts',(11.3501909789999,11.6,0.640973401999982));
#193767=CARTESIAN_POINT('Ctrl Pts',(11.3534185569999,15.2,0.642678869999984));
#193768=CARTESIAN_POINT('Ctrl Pts',(11.3534185569999,11.6,0.642678869999984));
#193769=CARTESIAN_POINT('Ctrl Pts',(11.3566488609999,15.2,0.644388963999987));
#193770=CARTESIAN_POINT('Ctrl Pts',(11.3566488609999,11.6,0.644388963999986));
#193771=CARTESIAN_POINT('Ctrl Pts',(11.3598818839999,15.2,0.646103686999986));
#193772=CARTESIAN_POINT('Ctrl Pts',(11.3598818839999,11.6,0.646103686999985));
#193773=CARTESIAN_POINT('Ctrl Pts',(11.3631176139999,15.2,0.647823038999986));
#193774=CARTESIAN_POINT('Ctrl Pts',(11.3631176139999,11.6,0.647823038999986));
#193775=CARTESIAN_POINT('Ctrl Pts',(11.3663560419999,15.2,0.649547022999983));
#193776=CARTESIAN_POINT('Ctrl Pts',(11.3663560419999,11.6,0.649547022999983));
#193777=CARTESIAN_POINT('Ctrl Pts',(11.3695971609999,15.2,0.651275639999986));
#193778=CARTESIAN_POINT('Ctrl Pts',(11.3695971609999,11.6,0.651275639999986));
#193779=CARTESIAN_POINT('Ctrl Pts',(11.3728409599999,15.2,0.653008890999986));
#193780=CARTESIAN_POINT('Ctrl Pts',(11.3728409599999,11.6,0.653008890999986));
#193781=CARTESIAN_POINT('Ctrl Pts',(11.3760874289999,15.2,0.654746779999984));
#193782=CARTESIAN_POINT('Ctrl Pts',(11.3760874289999,11.6,0.654746779999984));
#193783=CARTESIAN_POINT('Ctrl Pts',(11.3793365599999,15.2,0.656489305999983));
#193784=CARTESIAN_POINT('Ctrl Pts',(11.3793365599999,11.6,0.656489305999983));
#193785=CARTESIAN_POINT('Ctrl Pts',(11.3825883449999,15.2,0.658236471999984));
#193786=CARTESIAN_POINT('Ctrl Pts',(11.3825883449999,11.6,0.658236471999984));
#193787=CARTESIAN_POINT('Ctrl Pts',(11.3858427729999,15.2,0.659988279999983));
#193788=CARTESIAN_POINT('Ctrl Pts',(11.3858427729999,11.6,0.659988279999983));
#193789=CARTESIAN_POINT('Ctrl Pts',(11.3890998339999,15.2,0.661744729999985));
#193790=CARTESIAN_POINT('Ctrl Pts',(11.3890998339999,11.6,0.661744729999984));
#193791=CARTESIAN_POINT('Ctrl Pts',(11.3923595219999,15.2,0.663505825999984));
#193792=CARTESIAN_POINT('Ctrl Pts',(11.3923595219999,11.6,0.663505825999983));
#193793=CARTESIAN_POINT('Ctrl Pts',(11.3956218269999,15.2,0.665271566999985));
#193794=CARTESIAN_POINT('Ctrl Pts',(11.3956218269999,11.6,0.665271566999985));
#193795=CARTESIAN_POINT('Ctrl Pts',(11.3988867389999,15.2,0.667041954999985));
#193796=CARTESIAN_POINT('Ctrl Pts',(11.3988867389999,11.6,0.667041954999985));
#193797=CARTESIAN_POINT('Ctrl Pts',(11.4021542499999,15.2,0.668816992999983));
#193798=CARTESIAN_POINT('Ctrl Pts',(11.4021542499999,11.6,0.668816992999983));
#193799=CARTESIAN_POINT('Ctrl Pts',(11.4054243509999,15.2,0.670596681999989));
#193800=CARTESIAN_POINT('Ctrl Pts',(11.4054243509999,11.6,0.670596681999988));
#193801=CARTESIAN_POINT('Ctrl Pts',(11.4086970319999,15.2,0.672381023999984));
#193802=CARTESIAN_POINT('Ctrl Pts',(11.4086970319999,11.6,0.672381023999983));
#193803=CARTESIAN_POINT('Ctrl Pts',(11.4119722829999,15.2,0.674170018999987));
#193804=CARTESIAN_POINT('Ctrl Pts',(11.4119722829999,11.6,0.674170018999986));
#193805=CARTESIAN_POINT('Ctrl Pts',(11.4152500959999,15.2,0.675963670999984));
#193806=CARTESIAN_POINT('Ctrl Pts',(11.4152500959999,11.6,0.675963670999983));
#193807=CARTESIAN_POINT('Ctrl Pts',(11.4185304599999,15.2,0.677761978999989));
#193808=CARTESIAN_POINT('Ctrl Pts',(11.4185304599999,11.6,0.677761978999988));
#193809=CARTESIAN_POINT('Ctrl Pts',(11.4218133689999,15.2,0.679564945999989));
#193810=CARTESIAN_POINT('Ctrl Pts',(11.4218133689999,11.6,0.679564945999988));
#193811=CARTESIAN_POINT('Ctrl Pts',(11.4250988109999,15.2,0.681372573999983));
#193812=CARTESIAN_POINT('Ctrl Pts',(11.4250988109999,11.6,0.681372573999983));
#193813=CARTESIAN_POINT('Ctrl Pts',(11.4283867809999,15.2,0.683184862999986));
#193814=CARTESIAN_POINT('Ctrl Pts',(11.4283867809999,11.6,0.683184862999985));
#193815=CARTESIAN_POINT('Ctrl Pts',(11.4316772699999,15.2,0.685001813999988));
#193816=CARTESIAN_POINT('Ctrl Pts',(11.4316772699999,11.6,0.685001813999988));
#193817=CARTESIAN_POINT('Ctrl Pts',(11.4349702679999,15.2,0.686823429999985));
#193818=CARTESIAN_POINT('Ctrl Pts',(11.4349702679999,11.6,0.686823429999985));
#193819=CARTESIAN_POINT('Ctrl Pts',(11.4382657689999,15.2,0.688649711999982));
#193820=CARTESIAN_POINT('Ctrl Pts',(11.4382657689999,11.6,0.688649711999982));
#193821=CARTESIAN_POINT('Ctrl Pts',(11.4415637619999,15.2,0.690480658999988));
#193822=CARTESIAN_POINT('Ctrl Pts',(11.4415637619999,11.6,0.690480658999987));
#193823=CARTESIAN_POINT('Ctrl Pts',(11.4448642379999,15.2,0.692316276999985));
#193824=CARTESIAN_POINT('Ctrl Pts',(11.4448642379999,11.6,0.692316276999984));
#193825=CARTESIAN_POINT('Ctrl Pts',(11.4481671859999,15.2,0.694156563999986));
#193826=CARTESIAN_POINT('Ctrl Pts',(11.4481671859999,11.6,0.694156563999985));
#193827=CARTESIAN_POINT('Ctrl Pts',(11.4514725939999,15.2,0.696001523999983));
#193828=CARTESIAN_POINT('Ctrl Pts',(11.4514725939999,11.6,0.696001523999982));
#193829=CARTESIAN_POINT('Ctrl Pts',(11.4547804519999,15.2,0.697851158999985));
#193830=CARTESIAN_POINT('Ctrl Pts',(11.4547804519999,11.6,0.697851158999984));
#193831=CARTESIAN_POINT('Ctrl Pts',(11.4580907499999,15.2,0.699705468999987));
#193832=CARTESIAN_POINT('Ctrl Pts',(11.4580907499999,11.6,0.699705468999987));
#193833=CARTESIAN_POINT('Ctrl Pts',(11.4614034809999,15.2,0.701564455999986));
#193834=CARTESIAN_POINT('Ctrl Pts',(11.4614034809999,11.6,0.701564455999985));
#193835=CARTESIAN_POINT('Ctrl Pts',(11.4647186369999,15.2,0.703428121999985));
#193836=CARTESIAN_POINT('Ctrl Pts',(11.4647186369999,11.6,0.703428121999985));
#193837=CARTESIAN_POINT('Ctrl Pts',(11.4680362159999,15.2,0.705296463999985));
#193838=CARTESIAN_POINT('Ctrl Pts',(11.4680362159999,11.6,0.705296463999984));
#193839=CARTESIAN_POINT('Ctrl Pts',(11.4713562149999,15.2,0.707169484999985));
#193840=CARTESIAN_POINT('Ctrl Pts',(11.4713562149999,11.6,0.707169484999985));
#193841=CARTESIAN_POINT('Ctrl Pts',(11.4740141479999,15.2,0.708671645999988));
#193842=CARTESIAN_POINT('Ctrl Pts',(11.4740141479999,11.6,0.708671645999987));
#193843=CARTESIAN_POINT('Ctrl Pts',(11.4760086869999,15.2,0.709800371999982));
#193844=CARTESIAN_POINT('Ctrl Pts',(11.4760086869999,11.6,0.709800371999982));
#193845=CARTESIAN_POINT('Ctrl Pts',(11.4773388639999,15.2,0.710553791999988));
#193846=CARTESIAN_POINT('Ctrl Pts',(11.4773388639999,11.6,0.710553791999988));
#193847=CARTESIAN_POINT('Ctrl Pts',(11.4780040719999,15.2,0.710930734999984));
#193848=CARTESIAN_POINT('Ctrl Pts',(11.4780040719999,11.6,0.710930734999983));
#193849=CARTESIAN_POINT('Ctrl Pts',(10.3708900239999,15.2,0.292001928999985));
#193850=CARTESIAN_POINT('Ctrl Pts',(10.3726650375455,15.2,0.29220550820869));
#193851=CARTESIAN_POINT('Ctrl Pts',(10.3744962441107,15.2,0.292420934685804));
#193852=CARTESIAN_POINT('Ctrl Pts',(10.3763825855683,15.2,0.292648744500014));
#193853=CARTESIAN_POINT('Ctrl Pts',(10.3782780239178,15.2,0.2928776529283));
#193854=CARTESIAN_POINT('Ctrl Pts',(10.3802291370813,15.2,0.293119061022276));
#193855=CARTESIAN_POINT('Ctrl Pts',(10.3822349054607,15.2,0.293373492299609));
#193856=CARTESIAN_POINT('Ctrl Pts',(10.3845749682966,15.2,0.293670328755164));
#193857=CARTESIAN_POINT('Ctrl Pts',(10.38698942021,15.2,0.29398488688512));
#193858=CARTESIAN_POINT('Ctrl Pts',(10.3894766898008,15.2,0.294317967960511));
#193859=CARTESIAN_POINT('Ctrl Pts',(10.3916086354134,15.2,0.294603466058474));
#193860=CARTESIAN_POINT('Ctrl Pts',(10.3937940804213,15.2,0.294902569521762));
#193861=CARTESIAN_POINT('Ctrl Pts',(10.3960320642415,15.2,0.295215760805294));
#193862=CARTESIAN_POINT('Ctrl Pts',(10.39864304506,15.2,0.295581150593409));
#193863=CARTESIAN_POINT('Ctrl Pts',(10.4013255344682,15.2,0.295965719960752));
#193864=CARTESIAN_POINT('Ctrl Pts',(10.404078049501,15.2,0.296370203462173));
#193865=CARTESIAN_POINT('Ctrl Pts',(10.4064373483761,15.2,0.296716903646738));
#193866=CARTESIAN_POINT('Ctrl Pts',(10.4088480966947,15.2,0.297078237171211));
#193867=CARTESIAN_POINT('Ctrl Pts',(10.4113093847881,15.2,0.297454650294742));
#193868=CARTESIAN_POINT('Ctrl Pts',(10.4137706726579,15.2,0.297831063384081));
#193869=CARTESIAN_POINT('Ctrl Pts',(10.4162825002596,15.2,0.298222558514745));
#193870=CARTESIAN_POINT('Ctrl Pts',(10.4188439839998,15.2,0.298629568499958));
#193871=CARTESIAN_POINT('Ctrl Pts',(10.4214054677401,15.2,0.299036578485171));
#193872=CARTESIAN_POINT('Ctrl Pts',(10.4240166046342,15.2,0.299459106077529));
#193873=CARTESIAN_POINT('Ctrl Pts',(10.426676534751,15.2,0.299897567165915));
#193874=CARTESIAN_POINT('Ctrl Pts',(10.4293364651094,15.2,0.300336028294128));
#193875=CARTESIAN_POINT('Ctrl Pts',(10.4320451858385,15.2,0.3007904271745));
#193876=CARTESIAN_POINT('Ctrl Pts',(10.4348018550753,15.2,0.301261169034604));
#193877=CARTESIAN_POINT('Ctrl Pts',(10.4375585240618,15.2,0.301731910851949));
#193878=CARTESIAN_POINT('Ctrl Pts',(10.4403631424584,15.2,0.302218995524499));
#193879=CARTESIAN_POINT('Ctrl Pts',(10.4432148865345,15.2,0.302722818258519));
#193880=CARTESIAN_POINT('Ctrl Pts',(10.4460666306106,15.2,0.303226640992539));
#193881=CARTESIAN_POINT('Ctrl Pts',(10.4489654999236,15.2,0.303747202499338));
#193882=CARTESIAN_POINT('Ctrl Pts',(10.4519106910645,15.2,0.304284883229058));
#193883=CARTESIAN_POINT('Ctrl Pts',(10.454855882473,15.2,0.304822564007616));
#193884=CARTESIAN_POINT('Ctrl Pts',(10.457847395379,15.2,0.30537736525496));
#193885=CARTESIAN_POINT('Ctrl Pts',(10.4608844430476,15.2,0.305949657037339));
#193886=CARTESIAN_POINT('Ctrl Pts',(10.4639214904403,15.2,0.306521948767735));
#193887=CARTESIAN_POINT('Ctrl Pts',(10.4670040750655,15.2,0.307111731904449));
#193888=CARTESIAN_POINT('Ctrl Pts',(10.4701314264538,15.2,0.307719363549812));
#193889=CARTESIAN_POINT('Ctrl Pts',(10.4732587778421,15.2,0.308326995195175));
#193890=CARTESIAN_POINT('Ctrl Pts',(10.4764308974185,15.2,0.30895247778913));
#193891=CARTESIAN_POINT('Ctrl Pts',(10.4796470310498,15.2,0.309596157431617));
#193892=CARTESIAN_POINT('Ctrl Pts',(10.4828631649731,15.2,0.310239837132572));
#193893=CARTESIAN_POINT('Ctrl Pts',(10.4861233150853,15.2,0.310901714860778));
#193894=CARTESIAN_POINT('Ctrl Pts',(10.4894267458516,15.2,0.311582129315788));
#193895=CARTESIAN_POINT('Ctrl Pts',(10.4927301763179,15.2,0.312262543708994));
#193896=CARTESIAN_POINT('Ctrl Pts',(10.4960768859061,15.2,0.312961492114412));
#193897=CARTESIAN_POINT('Ctrl Pts',(10.4994661554514,15.2,0.313679305589152));
#193898=CARTESIAN_POINT('Ctrl Pts',(10.5045500597695,15.2,0.314756025801263));
#193899=CARTESIAN_POINT('Ctrl Pts',(10.5097297184083,15.2,0.315875189777522));
#193900=CARTESIAN_POINT('Ctrl Pts',(10.5150027656016,15.2,0.317037864666682));
#193901=CARTESIAN_POINT('Ctrl Pts',(10.5185181307164,15.2,0.317812981329863));
#193902=CARTESIAN_POINT('Ctrl Pts',(10.5220750012849,15.2,0.318607435192985));
#193903=CARTESIAN_POINT('Ctrl Pts',(10.5256726944004,15.2,0.319421530572026));
#193904=CARTESIAN_POINT('Ctrl Pts',(10.5292703871891,15.2,0.320235625877121));
#193905=CARTESIAN_POINT('Ctrl Pts',(10.5329089033351,15.2,0.321069360902435));
#193906=CARTESIAN_POINT('Ctrl Pts',(10.5365875692182,15.2,0.321923033958673));
#193907=CARTESIAN_POINT('Ctrl Pts',(10.5408793463046,15.2,0.322918985909312));
#193908=CARTESIAN_POINT('Ctrl Pts',(10.5452257733782,15.2,0.32394207156903));
#193909=CARTESIAN_POINT('Ctrl Pts',(10.5496258056443,15.2,0.324992749614784));
#193910=CARTESIAN_POINT('Ctrl Pts',(10.5533972616766,15.2,0.325893330750115));
#193911=CARTESIAN_POINT('Ctrl Pts',(10.5572081035156,15.2,0.326814180788589));
#193912=CARTESIAN_POINT('Ctrl Pts',(10.5610576844766,15.2,0.327755578008712));
#193913=CARTESIAN_POINT('Ctrl Pts',(10.5649072654377,15.2,0.328696975228835));
#193914=CARTESIAN_POINT('Ctrl Pts',(10.5687955874054,15.2,0.32965892028309));
#193915=CARTESIAN_POINT('Ctrl Pts',(10.5727220183444,15.2,0.330641681413143));
#193916=CARTESIAN_POINT('Ctrl Pts',(10.57664844964,15.2,0.331624442632464));
#193917=CARTESIAN_POINT('Ctrl Pts',(10.5806129884488,15.2,0.332628018379362));
#193918=CARTESIAN_POINT('Ctrl Pts',(10.5846150166694,15.2,0.333652674353308));
#193919=CARTESIAN_POINT('Ctrl Pts',(10.5879500396414,15.2,0.334506554191987));
#193920=CARTESIAN_POINT('Ctrl Pts',(10.5913110962726,15.2,0.335375069576351));
#193921=CARTESIAN_POINT('Ctrl Pts',(10.5946978335402,15.2,0.336258370451084));
#193922=CARTESIAN_POINT('Ctrl Pts',(10.598084571177,15.2,0.337141671422097));
#193923=CARTESIAN_POINT('Ctrl Pts',(10.6014969886578,15.2,0.33803975623175));
#193924=CARTESIAN_POINT('Ctrl Pts',(10.6049347395586,15.2,0.338952770397199));
#193925=CARTESIAN_POINT('Ctrl Pts',(10.6083724904593,15.2,0.339865784562648));
#193926=CARTESIAN_POINT('Ctrl Pts',(10.6118355735781,15.2,0.340793726400022));
#193927=CARTESIAN_POINT('Ctrl Pts',(10.6153236465284,15.2,0.341736737348865));
#193928=CARTESIAN_POINT('Ctrl Pts',(10.6195093342969,15.2,0.34286835054915));
#193929=CARTESIAN_POINT('Ctrl Pts',(10.6237310072045,15.2,0.344021663537506));
#193930=CARTESIAN_POINT('Ctrl Pts',(10.6279880816889,15.2,0.345196912686388));
#193931=CARTESIAN_POINT('Ctrl Pts',(10.6329546680074,15.2,0.34656803653329));
#193932=CARTESIAN_POINT('Ctrl Pts',(10.6379694394394,15.2,0.347969016672691));
#193933=CARTESIAN_POINT('Ctrl Pts',(10.6430314853886,15.2,0.349400219347995));
#193934=CARTESIAN_POINT('Ctrl Pts',(10.6466472327203,15.2,0.350422507036886));
#193935=CARTESIAN_POINT('Ctrl Pts',(10.6502871008117,15.2,0.351460214759748));
#193936=CARTESIAN_POINT('Ctrl Pts',(10.6539507637271,15.2,0.35251346968949));
#193937=CARTESIAN_POINT('Ctrl Pts',(10.6576144266425,15.2,0.353566724619232));
#193938=CARTESIAN_POINT('Ctrl Pts',(10.6613018846863,15.2,0.354635525991042));
#193939=CARTESIAN_POINT('Ctrl Pts',(10.6650128150323,15.2,0.355720003420784));
#193940=CARTESIAN_POINT('Ctrl Pts',(10.670950303505,15.2,0.35745516728473));
#193941=CARTESIAN_POINT('Ctrl Pts',(10.676947882173,15.2,0.359230456968549));
#193942=CARTESIAN_POINT('Ctrl Pts',(10.6830042559775,15.2,0.361046372942483));
#193943=CARTESIAN_POINT('Ctrl Pts',(10.6867894896568,15.2,0.362181320441656));
#193944=CARTESIAN_POINT('Ctrl Pts',(10.690597690334,15.2,0.363332138263453));
#193945=CARTESIAN_POINT('Ctrl Pts',(10.6944285482495,15.2,0.364498943957065));
#193946=CARTESIAN_POINT('Ctrl Pts',(10.6990255779986,15.2,0.365899110865708));
#193947=CARTESIAN_POINT('Ctrl Pts',(10.7036552325434,15.2,0.367322300760531));
#193948=CARTESIAN_POINT('Ctrl Pts',(10.7083169852164,15.2,0.368768713674277));
#193949=CARTESIAN_POINT('Ctrl Pts',(10.7122017784753,15.2,0.369974057571991));
#193950=CARTESIAN_POINT('Ctrl Pts',(10.7161088597494,15.2,0.37119552690207));
#193951=CARTESIAN_POINT('Ctrl Pts',(10.720037929736,15.2,0.37243323732139));
#193952=CARTESIAN_POINT('Ctrl Pts',(10.7239670001508,15.2,0.37367094787562));
#193953=CARTESIAN_POINT('Ctrl Pts',(10.7279180576654,15.2,0.374924897346244));
#193954=CARTESIAN_POINT('Ctrl Pts',(10.7318908047469,15.2,0.376195195608797));
#193955=CARTESIAN_POINT('Ctrl Pts',(10.7350690025854,15.2,0.377211434274224));
#193956=CARTESIAN_POINT('Ctrl Pts',(10.7382610807822,15.2,0.378238137886603));
#193957=CARTESIAN_POINT('Ctrl Pts',(10.7414668906937,15.2,0.379275359225652));
#193958=CARTESIAN_POINT('Ctrl Pts',(10.7462756051243,15.2,0.380831191092906));
#193959=CARTESIAN_POINT('Ctrl Pts',(10.7511152114962,15.2,0.382410689796956));
#193960=CARTESIAN_POINT('Ctrl Pts',(10.7559852079846,15.2,0.384014037654331));
#193961=CARTESIAN_POINT('Ctrl Pts',(10.7592318726051,15.2,0.385082936323006));
#193962=CARTESIAN_POINT('Ctrl Pts',(10.7624920433078,15.2,0.38616243504294));
#193963=CARTESIAN_POINT('Ctrl Pts',(10.7657655745426,15.2,0.387252585047496));
#193964=CARTESIAN_POINT('Ctrl Pts',(10.7690391053314,15.2,0.38834273490352));
#193965=CARTESIAN_POINT('Ctrl Pts',(10.7723259951077,15.2,0.389443538258318));
#193966=CARTESIAN_POINT('Ctrl Pts',(10.7756260982794,15.2,0.390555043555383));
#193967=CARTESIAN_POINT('Ctrl Pts',(10.7789262019008,15.2,0.391666549003891));
#193968=CARTESIAN_POINT('Ctrl Pts',(10.7822395196787,15.2,0.392788760491325));
#193969=CARTESIAN_POINT('Ctrl Pts',(10.7855659063053,15.2,0.393921725109331));
#193970=CARTESIAN_POINT('Ctrl Pts',(10.7888922924786,15.2,0.395054689572969));
#193971=CARTESIAN_POINT('Ctrl Pts',(10.7922317484244,15.2,0.396198408117783));
#193972=CARTESIAN_POINT('Ctrl Pts',(10.7955841294268,15.2,0.397352930577851));
#193973=CARTESIAN_POINT('Ctrl Pts',(10.798936510886,15.2,0.398507453195223));
#193974=CARTESIAN_POINT('Ctrl Pts',(10.8023018184777,15.2,0.399672780759046));
#193975=CARTESIAN_POINT('Ctrl Pts',(10.8056799105105,15.2,0.400848960717413));
#193976=CARTESIAN_POINT('Ctrl Pts',(10.8099025253214,15.2,0.402319185585244));
#193977=CARTESIAN_POINT('Ctrl Pts',(10.8141451158166,15.2,0.403806369147529));
#193978=CARTESIAN_POINT('Ctrl Pts',(10.8184074065121,15.2,0.405310603106756));
#193979=CARTESIAN_POINT('Ctrl Pts',(10.8218172387897,15.2,0.406513990175762));
#193980=CARTESIAN_POINT('Ctrl Pts',(10.8252396803287,15.2,0.407728290050905));
#193981=CARTESIAN_POINT('Ctrl Pts',(10.82867459188,15.2,0.40895355028295));
#193982=CARTESIAN_POINT('Ctrl Pts',(10.8321095038992,15.2,0.410178810681938));
#193983=CARTESIAN_POINT('Ctrl Pts',(10.8355568850952,15.2,0.411415028613229));
#193984=CARTESIAN_POINT('Ctrl Pts',(10.8390165992439,15.2,0.412662253742459));
#193985=CARTESIAN_POINT('Ctrl Pts',(10.8424763129213,15.2,0.413909478701755));
#193986=CARTESIAN_POINT('Ctrl Pts',(10.8459483590941,15.2,0.415167708938981));
#193987=CARTESIAN_POINT('Ctrl Pts',(10.8494326006969,15.2,0.416436989334086));
#193988=CARTESIAN_POINT('Ctrl Pts',(10.8529168427744,15.2,0.41770626990213));
#193989=CARTESIAN_POINT('Ctrl Pts',(10.8564132802198,15.2,0.418986601104559));
#193990=CARTESIAN_POINT('Ctrl Pts',(10.8599217789666,15.2,0.42027802700827));
#193991=CARTESIAN_POINT('Ctrl Pts',(10.8634302777133,15.2,0.421569452911981));
#193992=CARTESIAN_POINT('Ctrl Pts',(10.8669508372309,15.2,0.422871973497555));
#193993=CARTESIAN_POINT('Ctrl Pts',(10.8704833233691,15.2,0.424185632681398));
#193994=CARTESIAN_POINT('Ctrl Pts',(10.8748989303199,15.2,0.425827706392724));
#193995=CARTESIAN_POINT('Ctrl Pts',(10.8793331730265,15.2,0.427487183231485));
#193996=CARTESIAN_POINT('Ctrl Pts',(10.8837857909425,15.2,0.429164146797266));
#193997=CARTESIAN_POINT('Ctrl Pts',(10.8873478858576,15.2,0.430505717869237));
#193998=CARTESIAN_POINT('Ctrl Pts',(10.8909217425684,15.2,0.431858478925605));
#193999=CARTESIAN_POINT('Ctrl Pts',(10.8945072280416,15.2,0.433222473999939));
#194000=CARTESIAN_POINT('Ctrl Pts',(10.8980927135147,15.2,0.434586469074274));
#194001=CARTESIAN_POINT('Ctrl Pts',(10.9016898290587,15.2,0.435961696741592));
#194002=CARTESIAN_POINT('Ctrl Pts',(10.9052984425899,15.2,0.437348197984971));
#194003=CARTESIAN_POINT('Ctrl Pts',(10.9098092087663,15.2,0.43908132425583));
#194004=CARTESIAN_POINT('Ctrl Pts',(10.9143379425911,15.2,0.44083206546284));
#194005=CARTESIAN_POINT('Ctrl Pts',(10.9188843919552,15.2,0.442600500060302));
#194006=CARTESIAN_POINT('Ctrl Pts',(10.9225215520412,15.2,0.444015247969582));
#194007=CARTESIAN_POINT('Ctrl Pts',(10.926170050006,15.2,0.445441318854928));
#194008=CARTESIAN_POINT('Ctrl Pts',(10.9298297569832,15.2,0.446878753266602));
#194009=CARTESIAN_POINT('Ctrl Pts',(10.9334894639605,15.2,0.448316187678278));
#194010=CARTESIAN_POINT('Ctrl Pts',(10.9371603813529,15.2,0.449764984041275));
#194011=CARTESIAN_POINT('Ctrl Pts',(10.9408423816103,15.2,0.45122518178869));
#194012=CARTESIAN_POINT('Ctrl Pts',(10.9454448811794,15.2,0.45305042867453));
#194013=CARTESIAN_POINT('Ctrl Pts',(10.9500646984447,15.2,0.454893489216396));
#194014=CARTESIAN_POINT('Ctrl Pts',(10.9547015878684,15.2,0.456754436998201));
#194015=CARTESIAN_POINT('Ctrl Pts',(10.9584111000139,15.2,0.458243195467058));
#194016=CARTESIAN_POINT('Ctrl Pts',(10.9621315375354,15.2,0.45974340237033));
#194017=CARTESIAN_POINT('Ctrl Pts',(10.9658627765166,15.2,0.46125509350827));
#194018=CARTESIAN_POINT('Ctrl Pts',(10.9695940154977,15.2,0.462766784646209));
#194019=CARTESIAN_POINT('Ctrl Pts',(10.9733360566467,15.2,0.464289959282709));
#194020=CARTESIAN_POINT('Ctrl Pts',(10.9770887756301,15.2,0.465824655700869));
#194021=CARTESIAN_POINT('Ctrl Pts',(10.9817796741037,15.2,0.467743026119018));
#194022=CARTESIAN_POINT('Ctrl Pts',(10.9864872562776,15.2,0.469679397765223));
#194023=CARTESIAN_POINT('Ctrl Pts',(10.9912112853761,15.2,0.471633837488921));
#194024=CARTESIAN_POINT('Ctrl Pts',(10.994990508346,15.2,0.473197389140058));
#194025=CARTESIAN_POINT('Ctrl Pts',(10.9987802556102,15.2,0.474772506657516));
#194026=CARTESIAN_POINT('Ctrl Pts',(11.0025804067057,15.2,0.476359222257194));
#194027=CARTESIAN_POINT('Ctrl Pts',(11.0063805583189,15.2,0.477945938073063));
#194028=CARTESIAN_POINT('Ctrl Pts',(11.0101911138653,15.2,0.479544252743684));
#194029=CARTESIAN_POINT('Ctrl Pts',(11.014011953408,15.2,0.481154200554837));
#194030=CARTESIAN_POINT('Ctrl Pts',(11.0187880025759,15.2,0.483166635209101));
#194031=CARTESIAN_POINT('Ctrl Pts',(11.0235801178886,15.2,0.485197245672002));
#194032=CARTESIAN_POINT('Ctrl Pts',(11.0283880688621,15.2,0.487246096992937));
#194033=CARTESIAN_POINT('Ctrl Pts',(11.0331960193116,15.2,0.489294948090548));
#194034=CARTESIAN_POINT('Ctrl Pts',(11.0380198053124,15.2,0.491362041494871));
#194035=CARTESIAN_POINT('Ctrl Pts',(11.0428591956169,15.2,0.493447436752176));
#194036=CARTESIAN_POINT('Ctrl Pts',(11.047698586449,15.2,0.495532832236788));
#194037=CARTESIAN_POINT('Ctrl Pts',(11.0525535802363,15.2,0.497636531907216));
#194038=CARTESIAN_POINT('Ctrl Pts',(11.0574239503045,15.2,0.499758596489045));
#194039=CARTESIAN_POINT('Ctrl Pts',(11.0613202465714,15.2,0.50145624824703));
#194040=CARTESIAN_POINT('Ctrl Pts',(11.0652263825158,15.2,0.503165653263345));
#194041=CARTESIAN_POINT('Ctrl Pts',(11.0691422429692,15.2,0.504886842976115));
#194042=CARTESIAN_POINT('Ctrl Pts',(11.0730581028892,15.2,0.506608032454372));
#194043=CARTESIAN_POINT('Ctrl Pts',(11.0769836887681,15.2,0.508341006089075));
#194044=CARTESIAN_POINT('Ctrl Pts',(11.0809188825565,15.2,0.510085794223005));
#194045=CARTESIAN_POINT('Ctrl Pts',(11.0848540768811,15.2,0.511830582594661));
#194046=CARTESIAN_POINT('Ctrl Pts',(11.0887988802455,15.2,0.513587184286891));
#194047=CARTESIAN_POINT('Ctrl Pts',(11.0927531780166,15.2,0.515355630716602));
#194048=CARTESIAN_POINT('Ctrl Pts',(11.097696049961,15.2,0.517566188633265));
#194049=CARTESIAN_POINT('Ctrl Pts',(11.1026537596467,15.2,0.519795253490901));
#194050=CARTESIAN_POINT('Ctrl Pts',(11.1076260815443,15.2,0.522042879751165));
#194051=CARTESIAN_POINT('Ctrl Pts',(11.1135928676047,15.2,0.524740031165488));
#194052=CARTESIAN_POINT('Ctrl Pts',(11.1195806986001,15.2,0.527463913042928));
#194053=CARTESIAN_POINT('Ctrl Pts',(11.1255891954642,15.2,0.530214619358469));
#194054=CARTESIAN_POINT('Ctrl Pts',(11.1295948604041,15.2,0.5320484237354));
#194055=CARTESIAN_POINT('Ctrl Pts',(11.1336097096201,15.2,0.533894149516556));
#194056=CARTESIAN_POINT('Ctrl Pts',(11.1376336320623,15.2,0.535751824618584));
#194057=CARTESIAN_POINT('Ctrl Pts',(11.1426635348408,15.2,0.538073918369565));
#194058=CARTESIAN_POINT('Ctrl Pts',(11.1477076159057,15.2,0.540414683626949));
#194059=CARTESIAN_POINT('Ctrl Pts',(11.1527656581038,15.2,0.542774171523905));
#194060=CARTESIAN_POINT('Ctrl Pts',(11.1568120915315,15.2,0.544661761687159));
#194061=CARTESIAN_POINT('Ctrl Pts',(11.1608674602089,15.2,0.54656133336473));
#194062=CARTESIAN_POINT('Ctrl Pts',(11.1649316553761,15.2,0.548472914152112));
#194063=CARTESIAN_POINT('Ctrl Pts',(11.168995851097,15.2,0.550384495199946));
#194064=CARTESIAN_POINT('Ctrl Pts',(11.1730688724662,15.2,0.55230808468256));
#194065=CARTESIAN_POINT('Ctrl Pts',(11.1771506121337,15.2,0.554243708399956));
#194066=CARTESIAN_POINT('Ctrl Pts',(11.1822527864399,15.2,0.556663237914836));
#194067=CARTESIAN_POINT('Ctrl Pts',(11.1873685805938,15.2,0.559101570438957));
#194068=CARTESIAN_POINT('Ctrl Pts',(11.1924977846704,15.2,0.561558755076914));
#194069=CARTESIAN_POINT('Ctrl Pts',(11.1955753070045,15.2,0.563033065806122));
#194070=CARTESIAN_POINT('Ctrl Pts',(11.1986576579149,15.2,0.564514162982364));
#194071=CARTESIAN_POINT('Ctrl Pts',(11.2017447905532,15.2,0.566002057137232));
#194072=CARTESIAN_POINT('Ctrl Pts',(11.2058609672172,15.2,0.56798591592029));
#194073=CARTESIAN_POINT('Ctrl Pts',(11.2099856463879,15.2,0.569981857509243));
#194074=CARTESIAN_POINT('Ctrl Pts',(11.2141187215492,15.2,0.571989907454961));
#194075=CARTESIAN_POINT('Ctrl Pts',(11.2182517972736,15.2,0.573997957674276));
#194076=CARTESIAN_POINT('Ctrl Pts',(11.2223932680549,15.2,0.576018112850739));
#194077=CARTESIAN_POINT('Ctrl Pts',(11.2265430292444,15.2,0.578050401026323));
#194078=CARTESIAN_POINT('Ctrl Pts',(11.2296553498538,15.2,0.579574617019562));
#194079=CARTESIAN_POINT('Ctrl Pts',(11.2327723341463,15.2,0.581105654914132));
#194080=CARTESIAN_POINT('Ctrl Pts',(11.2358939367554,15.2,0.582643526990209));
#194081=CARTESIAN_POINT('Ctrl Pts',(11.2390155393645,15.2,0.584181399066286));
#194082=CARTESIAN_POINT('Ctrl Pts',(11.2421417612895,15.2,0.585726104487905));
#194083=CARTESIAN_POINT('Ctrl Pts',(11.2452725569254,15.2,0.587277652097601));
#194084=CARTESIAN_POINT('Ctrl Pts',(11.2494469514857,15.2,0.589346382431773));
#194085=CARTESIAN_POINT('Ctrl Pts',(11.2536294794081,15.2,0.591427276953513));
#194086=CARTESIAN_POINT('Ctrl Pts',(11.2578200365259,15.2,0.593520358679495));
#194087=CARTESIAN_POINT('Ctrl Pts',(11.2609629540788,15.2,0.59509016983139));
#194088=CARTESIAN_POINT('Ctrl Pts',(11.2641103876363,15.2,0.59666683680169));
#194089=CARTESIAN_POINT('Ctrl Pts',(11.2672622932861,15.2,0.598250367001377));
#194090=CARTESIAN_POINT('Ctrl Pts',(11.2714648339617,15.2,0.60036174050507));
#194091=CARTESIAN_POINT('Ctrl Pts',(11.2756753271309,15.2,0.602485317171043));
#194092=CARTESIAN_POINT('Ctrl Pts',(11.2798936682852,15.2,0.604621117884072));
#194093=CARTESIAN_POINT('Ctrl Pts',(11.2830574248694,15.2,0.606222968782597));
#194094=CARTESIAN_POINT('Ctrl Pts',(11.2862255958965,15.2,0.607831696166409));
#194095=CARTESIAN_POINT('Ctrl Pts',(11.2893981389832,15.2,0.609447308068814));
#194096=CARTESIAN_POINT('Ctrl Pts',(11.2925706814935,15.2,0.611062919677716));
#194097=CARTESIAN_POINT('Ctrl Pts',(11.2957475944786,15.2,0.612685416652924));
#194098=CARTESIAN_POINT('Ctrl Pts',(11.2989288370717,15.2,0.614314806719324));
#194099=CARTESIAN_POINT('Ctrl Pts',(11.3031704936699,15.2,0.616487326709188));
#194100=CARTESIAN_POINT('Ctrl Pts',(11.3074198466527,15.2,0.618672101302142));
#194101=CARTESIAN_POINT('Ctrl Pts',(11.3116767933039,15.2,0.62086915139906));
#194102=CARTESIAN_POINT('Ctrl Pts',(11.3148695040173,15.2,0.622516939345932));
#194103=CARTESIAN_POINT('Ctrl Pts',(11.3180664866986,15.2,0.624171632686409));
#194104=CARTESIAN_POINT('Ctrl Pts',(11.3212676989145,15.2,0.625833238595509));
#194105=CARTESIAN_POINT('Ctrl Pts',(11.3244689105487,15.2,0.62749484420275));
#194106=CARTESIAN_POINT('Ctrl Pts',(11.3276743522767,15.2,0.62916336240053));
#194107=CARTESIAN_POINT('Ctrl Pts',(11.3308839806126,15.2,0.63083880204916));
#194108=CARTESIAN_POINT('Ctrl Pts',(11.3340936089485,15.2,0.632514241697791));
#194109=CARTESIAN_POINT('Ctrl Pts',(11.337307424884,15.2,0.634196602661629));
#194110=CARTESIAN_POINT('Ctrl Pts',(11.3405253855591,15.2,0.635885892725854));
#194111=CARTESIAN_POINT('Ctrl Pts',(11.3448159995977,15.2,0.638138279375857));
#194112=CARTESIAN_POINT('Ctrl Pts',(11.3491139843876,15.2,0.640402984712273));
#194113=CARTESIAN_POINT('Ctrl Pts',(11.3534192378127,15.2,0.642680026135979));
#194114=CARTESIAN_POINT('Ctrl Pts',(11.3566481786147,15.2,0.644387807591567));
#194115=CARTESIAN_POINT('Ctrl Pts',(11.3598812104179,15.2,0.646102528940771));
#194116=CARTESIAN_POINT('Ctrl Pts',(11.3631182892223,15.2,0.647824197358602));
#194117=CARTESIAN_POINT('Ctrl Pts',(11.3685134191907,15.2,0.650693643991859));
#194118=CARTESIAN_POINT('Ctrl Pts',(11.3739197946772,15.2,0.653582388915906));
#194119=CARTESIAN_POINT('Ctrl Pts',(11.3793372227663,15.2,0.65649046561123));
#194120=CARTESIAN_POINT('Ctrl Pts',(11.3825876804465,15.2,0.658235312072198));
#194121=CARTESIAN_POINT('Ctrl Pts',(11.3858421171195,15.2,0.659987118460131));
#194122=CARTESIAN_POINT('Ctrl Pts',(11.3891004914269,15.2,0.661745891841689));
#194123=CARTESIAN_POINT('Ctrl Pts',(11.3945311144834,15.2,0.664677180384938));
#194124=CARTESIAN_POINT('Ctrl Pts',(11.3999726797678,15.2,0.667627819647947));
#194125=CARTESIAN_POINT('Ctrl Pts',(11.4054249967131,15.2,0.670597845621758));
#194126=CARTESIAN_POINT('Ctrl Pts',(11.4086963867614,15.2,0.672379861141297));
#194127=CARTESIAN_POINT('Ctrl Pts',(11.4119716465893,15.2,0.674168855272206));
#194128=CARTESIAN_POINT('Ctrl Pts',(11.415250734426,15.2,0.67596483538082));
#194129=CARTESIAN_POINT('Ctrl Pts',(11.4185298222628,15.2,0.677760815489433));
#194130=CARTESIAN_POINT('Ctrl Pts',(11.4218127380273,15.2,0.679563780979161));
#194131=CARTESIAN_POINT('Ctrl Pts',(11.4250994433249,15.2,0.681373739455673));
#194132=CARTESIAN_POINT('Ctrl Pts',(11.4283861486225,15.2,0.683183697932186));
#194133=CARTESIAN_POINT('Ctrl Pts',(11.4316766450363,15.2,0.685000647549539));
#194134=CARTESIAN_POINT('Ctrl Pts',(11.4349708937083,15.2,0.686824596483266));
#194135=CARTESIAN_POINT('Ctrl Pts',(11.4382651423802,15.2,0.688648545416993));
#194136=CARTESIAN_POINT('Ctrl Pts',(11.4415631447104,15.2,0.690479491583784));
#194137=CARTESIAN_POINT('Ctrl Pts',(11.4448648556318,15.2,0.692317444099715));
#194138=CARTESIAN_POINT('Ctrl Pts',(11.4481665665531,15.2,0.694155396615647));
#194139=CARTESIAN_POINT('Ctrl Pts',(11.4514719840484,15.2,0.696000354800605));
#194140=CARTESIAN_POINT('Ctrl Pts',(11.4547810613847,15.2,0.697852327408362));
#194141=CARTESIAN_POINT('Ctrl Pts',(11.4580901387211,15.2,0.69970430001612));
#194142=CARTESIAN_POINT('Ctrl Pts',(11.4614028748479,15.2,0.701563286711907));
#194143=CARTESIAN_POINT('Ctrl Pts',(11.4647192420186,15.2,0.703429290643153));
#194144=CARTESIAN_POINT('Ctrl Pts',(11.4691410653145,15.2,0.705917296110807));
#194145=CARTESIAN_POINT('Ctrl Pts',(11.4735693507915,15.2,0.7084177809819));
#194146=CARTESIAN_POINT('Ctrl Pts',(11.4780040719999,15.2,0.710930734999984));
#194147=CARTESIAN_POINT('Ctrl Pts',(10.3708900239999,12.2,0.292001928999985));
#194148=CARTESIAN_POINT('Ctrl Pts',(10.3726650375455,12.2,0.29220550820869));
#194149=CARTESIAN_POINT('Ctrl Pts',(10.3744962441107,12.2,0.292420934685804));
#194150=CARTESIAN_POINT('Ctrl Pts',(10.3763825855683,12.2,0.292648744500013));
#194151=CARTESIAN_POINT('Ctrl Pts',(10.3782780239178,12.2,0.2928776529283));
#194152=CARTESIAN_POINT('Ctrl Pts',(10.3802291370813,12.2,0.293119061022275));
#194153=CARTESIAN_POINT('Ctrl Pts',(10.3822349054607,12.2,0.293373492299608));
#194154=CARTESIAN_POINT('Ctrl Pts',(10.3845749682966,12.2,0.293670328755164));
#194155=CARTESIAN_POINT('Ctrl Pts',(10.38698942021,12.2,0.29398488688512));
#194156=CARTESIAN_POINT('Ctrl Pts',(10.3894766898008,12.2,0.29431796796051));
#194157=CARTESIAN_POINT('Ctrl Pts',(10.3916086354134,12.2,0.294603466058474));
#194158=CARTESIAN_POINT('Ctrl Pts',(10.3937940804213,12.2,0.294902569521762));
#194159=CARTESIAN_POINT('Ctrl Pts',(10.3960320642415,12.2,0.295215760805293));
#194160=CARTESIAN_POINT('Ctrl Pts',(10.39864304506,12.2,0.295581150593408));
#194161=CARTESIAN_POINT('Ctrl Pts',(10.4013255344682,12.2,0.295965719960751));
#194162=CARTESIAN_POINT('Ctrl Pts',(10.404078049501,12.2,0.296370203462172));
#194163=CARTESIAN_POINT('Ctrl Pts',(10.4064373483761,12.2,0.296716903646737));
#194164=CARTESIAN_POINT('Ctrl Pts',(10.4088480966947,12.2,0.29707823717121));
#194165=CARTESIAN_POINT('Ctrl Pts',(10.4113093847881,12.2,0.297454650294741));
#194166=CARTESIAN_POINT('Ctrl Pts',(10.4137706726579,12.2,0.297831063384081));
#194167=CARTESIAN_POINT('Ctrl Pts',(10.4162825002596,12.2,0.298222558514745));
#194168=CARTESIAN_POINT('Ctrl Pts',(10.4188439839998,12.2,0.298629568499958));
#194169=CARTESIAN_POINT('Ctrl Pts',(10.4214054677401,12.2,0.299036578485171));
#194170=CARTESIAN_POINT('Ctrl Pts',(10.4240166046342,12.2,0.299459106077528));
#194171=CARTESIAN_POINT('Ctrl Pts',(10.426676534751,12.2,0.299897567165915));
#194172=CARTESIAN_POINT('Ctrl Pts',(10.429779786715,12.2,0.300409105128917));
#194173=CARTESIAN_POINT('Ctrl Pts',(10.4329494469773,12.2,0.300942337035746));
#194174=CARTESIAN_POINT('Ctrl Pts',(10.4361841812499,12.2,0.301497903516621));
#194175=CARTESIAN_POINT('Ctrl Pts',(10.4389568104824,12.2,0.301974103332653));
#194176=CARTESIAN_POINT('Ctrl Pts',(10.4417772507362,12.2,0.302466714036415));
#194177=CARTESIAN_POINT('Ctrl Pts',(10.4446446819393,12.2,0.30297612595905));
#194178=CARTESIAN_POINT('Ctrl Pts',(10.4475121134028,12.2,0.303485537927957));
#194179=CARTESIAN_POINT('Ctrl Pts',(10.4504265340331,12.2,0.304011754270072));
#194180=CARTESIAN_POINT('Ctrl Pts',(10.4533871436142,12.2,0.304555152050855));
#194181=CARTESIAN_POINT('Ctrl Pts',(10.4563477529265,12.2,0.305098549782279));
#194182=CARTESIAN_POINT('Ctrl Pts',(10.4593545518565,12.2,0.30565912976856));
#194183=CARTESIAN_POINT('Ctrl Pts',(10.4624067580096,12.2,0.306237262250217));
#194184=CARTESIAN_POINT('Ctrl Pts',(10.4654589641627,12.2,0.306815394731874));
#194185=CARTESIAN_POINT('Ctrl Pts',(10.4685565750616,12.2,0.307411077481327));
#194186=CARTESIAN_POINT('Ctrl Pts',(10.4716988292788,12.2,0.308024668208254));
#194187=CARTESIAN_POINT('Ctrl Pts',(10.4748410837814,12.2,0.308638258990916));
#194188=CARTESIAN_POINT('Ctrl Pts',(10.478027976748,12.2,0.309269760050793));
#194189=CARTESIAN_POINT('Ctrl Pts',(10.4812587633437,12.2,0.309919515587448));
#194190=CARTESIAN_POINT('Ctrl Pts',(10.484489549646,12.2,0.310569271065084));
#194191=CARTESIAN_POINT('Ctrl Pts',(10.4877642267818,12.2,0.311237281638716));
#194192=CARTESIAN_POINT('Ctrl Pts',(10.4910820642597,12.2,0.311923882283599));
#194193=CARTESIAN_POINT('Ctrl Pts',(10.4943999017377,12.2,0.312610482928481));
#194194=CARTESIAN_POINT('Ctrl Pts',(10.4977608967567,12.2,0.3133156758627));
#194195=CARTESIAN_POINT('Ctrl Pts',(10.5011643332979,12.2,0.314039785418901));
#194196=CARTESIAN_POINT('Ctrl Pts',(10.5045677701482,12.2,0.314763895040875));
#194197=CARTESIAN_POINT('Ctrl Pts',(10.5080136477538,12.2,0.315506921331853));
#194198=CARTESIAN_POINT('Ctrl Pts',(10.5115012636134,12.2,0.316269181791375));
#194199=CARTESIAN_POINT('Ctrl Pts',(10.5149888791561,12.2,0.31703144218166));
#194200=CARTESIAN_POINT('Ctrl Pts',(10.5185182327559,12.2,0.317812935846945));
#194201=CARTESIAN_POINT('Ctrl Pts',(10.5220886344613,12.2,0.318613971068692));
#194202=CARTESIAN_POINT('Ctrl Pts',(10.5256590361667,12.2,0.319415006290438));
#194203=CARTESIAN_POINT('Ctrl Pts',(10.5292704866605,12.2,0.320235581935627));
#194204=CARTESIAN_POINT('Ctrl Pts',(10.532922311276,12.2,0.321075996237563));
#194205=CARTESIAN_POINT('Ctrl Pts',(10.5365741358916,12.2,0.321916410539499));
#194206=CARTESIAN_POINT('Ctrl Pts',(10.5402663324814,12.2,0.32277666341235));
#194207=CARTESIAN_POINT('Ctrl Pts',(10.5439982403431,12.2,0.323657045628992));
#194208=CARTESIAN_POINT('Ctrl Pts',(10.5477301485438,12.2,0.324537427925602));
#194209=CARTESIAN_POINT('Ctrl Pts',(10.55150176864,12.2,0.325437938149148));
#194210=CARTESIAN_POINT('Ctrl Pts',(10.5553124489327,12.2,0.32635885753356));
#194211=CARTESIAN_POINT('Ctrl Pts',(10.5597582420884,12.2,0.327433263356567));
#194212=CARTESIAN_POINT('Ctrl Pts',(10.5642572009667,12.2,0.328535448838623));
#194213=CARTESIAN_POINT('Ctrl Pts',(10.5688083138747,12.2,0.329665848627676));
#194214=CARTESIAN_POINT('Ctrl Pts',(10.5720591090114,12.2,0.330473277098718));
#194215=CARTESIAN_POINT('Ctrl Pts',(10.5753365152977,12.2,0.33129509770841));
#194216=CARTESIAN_POINT('Ctrl Pts',(10.5786401687678,12.2,0.332131466873889));
#194217=CARTESIAN_POINT('Ctrl Pts',(10.5819438222378,12.2,0.332967836039368));
#194218=CARTESIAN_POINT('Ctrl Pts',(10.5852737236279,12.2,0.333818752173959));
#194219=CARTESIAN_POINT('Ctrl Pts',(10.5886295173354,12.2,0.334684364091183));
#194220=CARTESIAN_POINT('Ctrl Pts',(10.5919853110429,12.2,0.335549976008407));
#194221=CARTESIAN_POINT('Ctrl Pts',(10.5953669967508,12.2,0.336430285558935));
#194222=CARTESIAN_POINT('Ctrl Pts',(10.5987742234855,12.2,0.337325437224829));
#194223=CARTESIAN_POINT('Ctrl Pts',(10.6021814502203,12.2,0.338220588890723));
#194224=CARTESIAN_POINT('Ctrl Pts',(10.6056142165808,12.2,0.339130582162553));
#194225=CARTESIAN_POINT('Ctrl Pts',(10.6090721785239,12.2,0.340055561397878));
#194226=CARTESIAN_POINT('Ctrl Pts',(10.612530140467,12.2,0.340980540633203));
#194227=CARTESIAN_POINT('Ctrl Pts',(10.6160132978765,12.2,0.341920504778467));
#194228=CARTESIAN_POINT('Ctrl Pts',(10.6195213082396,12.2,0.342875592491096));
#194229=CARTESIAN_POINT('Ctrl Pts',(10.6230293186027,12.2,0.343830680203724));
#194230=CARTESIAN_POINT('Ctrl Pts',(10.6265621837777,12.2,0.344800893372168));
#194231=CARTESIAN_POINT('Ctrl Pts',(10.6301195657916,12.2,0.345786365941613));
#194232=CARTESIAN_POINT('Ctrl Pts',(10.6336769478055,12.2,0.346771838511057));
#194233=CARTESIAN_POINT('Ctrl Pts',(10.6372588474132,12.2,0.347772571140291));
#194234=CARTESIAN_POINT('Ctrl Pts',(10.6408649342352,12.2,0.348788696283835));
#194235=CARTESIAN_POINT('Ctrl Pts',(10.6444710210572,12.2,0.349804821427379));
#194236=CARTESIAN_POINT('Ctrl Pts',(10.6481012925933,12.2,0.35083634071771));
#194237=CARTESIAN_POINT('Ctrl Pts',(10.651755424539,12.2,0.351883381551851));
#194238=CARTESIAN_POINT('Ctrl Pts',(10.6561403827145,12.2,0.353139830507171));
#194239=CARTESIAN_POINT('Ctrl Pts',(10.6605596987789,12.2,0.354418630552376));
#194240=CARTESIAN_POINT('Ctrl Pts',(10.6650128150323,12.2,0.355720003420783));
#194241=CARTESIAN_POINT('Ctrl Pts',(10.6702081175976,12.2,0.357238271846064));
#194242=CARTESIAN_POINT('Ctrl Pts',(10.6754494275741,12.2,0.35878726088698));
#194243=CARTESIAN_POINT('Ctrl Pts',(10.6807358750053,12.2,0.360367307815519));
#194244=CARTESIAN_POINT('Ctrl Pts',(10.684511908826,12.2,0.361495912746902));
#194245=CARTESIAN_POINT('Ctrl Pts',(10.6883109732599,12.2,0.3626403632751));
#194246=CARTESIAN_POINT('Ctrl Pts',(10.6921327554833,12.2,0.363800778275934));
#194247=CARTESIAN_POINT('Ctrl Pts',(10.6959545377067,12.2,0.364961193276767));
#194248=CARTESIAN_POINT('Ctrl Pts',(10.6997990398407,12.2,0.366137573777189));
#194249=CARTESIAN_POINT('Ctrl Pts',(10.7036659519946,12.2,0.367330034611361));
#194250=CARTESIAN_POINT('Ctrl Pts',(10.7075328641485,12.2,0.368522495445535));
#194251=CARTESIAN_POINT('Ctrl Pts',(10.711422188446,12.2,0.369731037763199));
#194252=CARTESIAN_POINT('Ctrl Pts',(10.7153336199624,12.2,0.37095577365884));
#194253=CARTESIAN_POINT('Ctrl Pts',(10.7192450514787,12.2,0.372180509554481));
#194254=CARTESIAN_POINT('Ctrl Pts',(10.7231785915877,12.2,0.373421440913062));
#194255=CARTESIAN_POINT('Ctrl Pts',(10.7271339395756,12.2,0.374678678206065));
#194256=CARTESIAN_POINT('Ctrl Pts',(10.7302982177072,12.2,0.375684467958244));
#194257=CARTESIAN_POINT('Ctrl Pts',(10.7334764524204,12.2,0.376700691622952));
#194258=CARTESIAN_POINT('Ctrl Pts',(10.7366684932141,12.2,0.377727408649442));
#194259=CARTESIAN_POINT('Ctrl Pts',(10.7398605344427,12.2,0.378754125815822));
#194260=CARTESIAN_POINT('Ctrl Pts',(10.743066382813,12.2,0.379791333552787));
#194261=CARTESIAN_POINT('Ctrl Pts',(10.7462858844838,12.2,0.380839086885371));
#194262=CARTESIAN_POINT('Ctrl Pts',(10.749505385716,12.2,0.381886840075198));
#194263=CARTESIAN_POINT('Ctrl Pts',(10.7527385438064,12.2,0.382945139131294));
#194264=CARTESIAN_POINT('Ctrl Pts',(10.7559852079846,12.2,0.384014037654331));
#194265=CARTESIAN_POINT('Ctrl Pts',(10.7592318726051,12.2,0.385082936323006));
#194266=CARTESIAN_POINT('Ctrl Pts',(10.7624920433078,12.2,0.38616243504294));
#194267=CARTESIAN_POINT('Ctrl Pts',(10.7657655745426,12.2,0.387252585047496));
#194268=CARTESIAN_POINT('Ctrl Pts',(10.7690391053314,12.2,0.388342734903519));
#194269=CARTESIAN_POINT('Ctrl Pts',(10.7723259951077,12.2,0.389443538258318));
#194270=CARTESIAN_POINT('Ctrl Pts',(10.7756260982794,12.2,0.390555043555382));
#194271=CARTESIAN_POINT('Ctrl Pts',(10.7789262019008,12.2,0.39166654900389));
#194272=CARTESIAN_POINT('Ctrl Pts',(10.7822395196787,12.2,0.392788760491324));
#194273=CARTESIAN_POINT('Ctrl Pts',(10.7855659063053,12.2,0.39392172510933));
#194274=CARTESIAN_POINT('Ctrl Pts',(10.7888922924786,12.2,0.395054689572968));
#194275=CARTESIAN_POINT('Ctrl Pts',(10.7922317484244,12.2,0.396198408117784));
#194276=CARTESIAN_POINT('Ctrl Pts',(10.7955841294268,12.2,0.397352930577852));
#194277=CARTESIAN_POINT('Ctrl Pts',(10.798936510886,12.2,0.398507453195224));
#194278=CARTESIAN_POINT('Ctrl Pts',(10.8023018184777,12.2,0.399672780759045));
#194279=CARTESIAN_POINT('Ctrl Pts',(10.8056799105105,12.2,0.400848960717412));
#194280=CARTESIAN_POINT('Ctrl Pts',(10.8090580020831,12.2,0.402025140515525));
#194281=CARTESIAN_POINT('Ctrl Pts',(10.8124488787035,12.2,0.403212174061467));
#194282=CARTESIAN_POINT('Ctrl Pts',(10.8158523977018,12.2,0.404410107795754));
#194283=CARTESIAN_POINT('Ctrl Pts',(10.8192559171637,12.2,0.405608041693259));
#194284=CARTESIAN_POINT('Ctrl Pts',(10.8226720809103,12.2,0.406816876258458));
#194285=CARTESIAN_POINT('Ctrl Pts',(10.8261007490416,12.2,0.408036659491605));
#194286=CARTESIAN_POINT('Ctrl Pts',(10.8295294171729,12.2,0.409256442724752));
#194287=CARTESIAN_POINT('Ctrl Pts',(10.8329705894834,12.2,0.410487172836951));
#194288=CARTESIAN_POINT('Ctrl Pts',(10.8364241288396,12.2,0.411728897961302));
#194289=CARTESIAN_POINT('Ctrl Pts',(10.8398776677252,12.2,0.412970622916468));
#194290=CARTESIAN_POINT('Ctrl Pts',(10.8433435737133,12.2,0.414223341143917));
#194291=CARTESIAN_POINT('Ctrl Pts',(10.8468217087225,12.2,0.41548709999075));
#194292=CARTESIAN_POINT('Ctrl Pts',(10.8502998442056,12.2,0.41675085900977));
#194293=CARTESIAN_POINT('Ctrl Pts',(10.8537902098138,12.2,0.418025655425087));
#194294=CARTESIAN_POINT('Ctrl Pts',(10.8572926693392,12.2,0.419311537218523));
#194295=CARTESIAN_POINT('Ctrl Pts',(10.8607951283875,12.2,0.420597418836759));
#194296=CARTESIAN_POINT('Ctrl Pts',(10.8643096819758,12.2,0.42189438352578));
#194297=CARTESIAN_POINT('Ctrl Pts',(10.8678361961867,12.2,0.423202475918111));
#194298=CARTESIAN_POINT('Ctrl Pts',(10.8713627108781,12.2,0.424510568488671));
#194299=CARTESIAN_POINT('Ctrl Pts',(10.8749011853905,12.2,0.425829789244775));
#194300=CARTESIAN_POINT('Ctrl Pts',(10.8784514870401,12.2,0.427160179218054));
#194301=CARTESIAN_POINT('Ctrl Pts',(10.8820017882061,12.2,0.428490569010066));
#194302=CARTESIAN_POINT('Ctrl Pts',(10.885563915548,12.2,0.429832129409109));
#194303=CARTESIAN_POINT('Ctrl Pts',(10.8891377385328,12.2,0.431184901131124));
#194304=CARTESIAN_POINT('Ctrl Pts',(10.8927115620046,12.2,0.432537673037453));
#194305=CARTESIAN_POINT('Ctrl Pts',(10.8962970795584,12.2,0.433901657709012));
#194306=CARTESIAN_POINT('Ctrl Pts',(10.8998941623107,12.2,0.435276895562474));
#194307=CARTESIAN_POINT('Ctrl Pts',(10.903491244573,12.2,0.436652133228559));
#194308=CARTESIAN_POINT('Ctrl Pts',(10.9070998892519,12.2,0.438038624931487));
#194309=CARTESIAN_POINT('Ctrl Pts',(10.9107199696913,12.2,0.439436409330509));
#194310=CARTESIAN_POINT('Ctrl Pts',(10.9152450706106,12.2,0.441183639972123));
#194311=CARTESIAN_POINT('Ctrl Pts',(10.9197880365582,12.2,0.442948518389949));
#194312=CARTESIAN_POINT('Ctrl Pts',(10.9243486189184,12.2,0.444731119708467));
#194313=CARTESIAN_POINT('Ctrl Pts',(10.9279970850054,12.2,0.446157200841003));
#194314=CARTESIAN_POINT('Ctrl Pts',(10.931656823766,12.2,0.447594625763789));
#194315=CARTESIAN_POINT('Ctrl Pts',(10.9353277093001,12.2,0.449043431676821));
#194316=CARTESIAN_POINT('Ctrl Pts',(10.938998594334,12.2,0.450492237392454));
#194317=CARTESIAN_POINT('Ctrl Pts',(10.9426806255991,12.2,0.451952425403687));
#194318=CARTESIAN_POINT('Ctrl Pts',(10.9463736774807,12.2,0.453424033078131));
#194319=CARTESIAN_POINT('Ctrl Pts',(10.9500667298655,12.2,0.454895640953082));
#194320=CARTESIAN_POINT('Ctrl Pts',(10.95377080242,12.2,0.456378668612243));
#194321=CARTESIAN_POINT('Ctrl Pts',(10.9574857693454,12.2,0.45787315313889));
#194322=CARTESIAN_POINT('Ctrl Pts',(10.9612007357646,12.2,0.459367637461913));
#194323=CARTESIAN_POINT('Ctrl Pts',(10.964926596615,12.2,0.460873580265958));
#194324=CARTESIAN_POINT('Ctrl Pts',(10.968663228364,12.2,0.462391015251845));
#194325=CARTESIAN_POINT('Ctrl Pts',(10.9723998606221,12.2,0.463908450444482));
#194326=CARTESIAN_POINT('Ctrl Pts',(10.9761472635951,12.2,0.465437379513202));
#194327=CARTESIAN_POINT('Ctrl Pts',(10.9799053144666,12.2,0.466977838541603));
#194328=CARTESIAN_POINT('Ctrl Pts',(10.9836633653381,12.2,0.468518297570005));
#194329=CARTESIAN_POINT('Ctrl Pts',(10.9874320618913,12.2,0.470070285624747));
#194330=CARTESIAN_POINT('Ctrl Pts',(10.9912112853761,12.2,0.471633837488919));
#194331=CARTESIAN_POINT('Ctrl Pts',(10.994990508346,12.2,0.473197389140057));
#194332=CARTESIAN_POINT('Ctrl Pts',(10.9987802556102,12.2,0.474772506657516));
#194333=CARTESIAN_POINT('Ctrl Pts',(11.0025804067057,12.2,0.476359222257194));
#194334=CARTESIAN_POINT('Ctrl Pts',(11.0063805583189,12.2,0.477945938073062));
#194335=CARTESIAN_POINT('Ctrl Pts',(11.0101911138653,12.2,0.479544252743683));
#194336=CARTESIAN_POINT('Ctrl Pts',(11.014011953408,12.2,0.481154200554837));
#194337=CARTESIAN_POINT('Ctrl Pts',(11.0187880025759,12.2,0.483166635209101));
#194338=CARTESIAN_POINT('Ctrl Pts',(11.0235801178886,12.2,0.485197245672001));
#194339=CARTESIAN_POINT('Ctrl Pts',(11.0283880688621,12.2,0.487246096992937));
#194340=CARTESIAN_POINT('Ctrl Pts',(11.0322344293265,12.2,0.48888517791569));
#194341=CARTESIAN_POINT('Ctrl Pts',(11.0360909250208,12.2,0.490535934007757));
#194342=CARTESIAN_POINT('Ctrl Pts',(11.0399574362223,12.2,0.492198395490474));
#194343=CARTESIAN_POINT('Ctrl Pts',(11.0438239479505,12.2,0.493860857199702));
#194344=CARTESIAN_POINT('Ctrl Pts',(11.0477004757558,12.2,0.495535024951953));
#194345=CARTESIAN_POINT('Ctrl Pts',(11.0515869026353,12.2,0.497220930767254));
#194346=CARTESIAN_POINT('Ctrl Pts',(11.0554733289853,12.2,0.49890683635285));
#194347=CARTESIAN_POINT('Ctrl Pts',(11.059369653609,12.2,0.500604480314707));
#194348=CARTESIAN_POINT('Ctrl Pts',(11.0632757601223,12.2,0.502313893118637));
#194349=CARTESIAN_POINT('Ctrl Pts',(11.0671818671679,12.2,0.504023306155474));
#194350=CARTESIAN_POINT('Ctrl Pts',(11.0710977566781,12.2,0.505744488255535));
#194351=CARTESIAN_POINT('Ctrl Pts',(11.0750233138113,12.2,0.507477469493138));
#194352=CARTESIAN_POINT('Ctrl Pts',(11.0789488704095,12.2,0.509210450494623));
#194353=CARTESIAN_POINT('Ctrl Pts',(11.0828840924951,12.2,0.510955231381379));
#194354=CARTESIAN_POINT('Ctrl Pts',(11.0868288663942,12.2,0.512711840848114));
#194355=CARTESIAN_POINT('Ctrl Pts',(11.0907736408308,12.2,0.514468450554187));
#194356=CARTESIAN_POINT('Ctrl Pts',(11.0947279667574,12.2,0.516236889897792));
#194357=CARTESIAN_POINT('Ctrl Pts',(11.0986917323074,12.2,0.518017187662257));
#194358=CARTESIAN_POINT('Ctrl Pts',(11.1026554973173,12.2,0.519797485184156));
#194359=CARTESIAN_POINT('Ctrl Pts',(11.10662869908,12.2,0.521589640343834));
#194360=CARTESIAN_POINT('Ctrl Pts',(11.1106112258971,12.2,0.523393683229892));
#194361=CARTESIAN_POINT('Ctrl Pts',(11.1145937532567,12.2,0.525197726361749));
#194362=CARTESIAN_POINT('Ctrl Pts',(11.1185856064668,12.2,0.527013655557412));
#194363=CARTESIAN_POINT('Ctrl Pts',(11.1225866715188,12.2,0.528841501157811));
#194364=CARTESIAN_POINT('Ctrl Pts',(11.1265877360256,12.2,0.530669346509165));
#194365=CARTESIAN_POINT('Ctrl Pts',(11.1305980138639,12.2,0.532509105863678));
#194366=CARTESIAN_POINT('Ctrl Pts',(11.1346173923677,12.2,0.534360807988857));
#194367=CARTESIAN_POINT('Ctrl Pts',(11.1386367714192,12.2,0.536212510366331));
#194368=CARTESIAN_POINT('Ctrl Pts',(11.1426652509226,12.2,0.538076154854329));
#194369=CARTESIAN_POINT('Ctrl Pts',(11.1467027219943,12.2,0.539951769242885));
#194370=CARTESIAN_POINT('Ctrl Pts',(11.1497308250231,12.2,0.541358479906526));
#194371=CARTESIAN_POINT('Ctrl Pts',(11.1527639856271,12.2,0.542771924060498));
#194372=CARTESIAN_POINT('Ctrl Pts',(11.1558021562388,12.2,0.544192110765316));
#194373=CARTESIAN_POINT('Ctrl Pts',(11.1588403268505,12.2,0.545612297470135));
#194374=CARTESIAN_POINT('Ctrl Pts',(11.1618835088623,12.2,0.547039228496462));
#194375=CARTESIAN_POINT('Ctrl Pts',(11.1649316553761,12.2,0.548472914152111));
#194376=CARTESIAN_POINT('Ctrl Pts',(11.1679798018899,12.2,0.54990659980776));
#194377=CARTESIAN_POINT('Ctrl Pts',(11.1710329121117,12.2,0.551347040037955));
#194378=CARTESIAN_POINT('Ctrl Pts',(11.1740909425416,12.2,0.552794246192785));
#194379=CARTESIAN_POINT('Ctrl Pts',(11.177148973527,12.2,0.554241452610524));
#194380=CARTESIAN_POINT('Ctrl Pts',(11.1802119228055,12.2,0.555695424655167));
#194381=CARTESIAN_POINT('Ctrl Pts',(11.1832797449187,12.2,0.557156172576721));
#194382=CARTESIAN_POINT('Ctrl Pts',(11.1863475664746,12.2,0.558616920232907));
#194383=CARTESIAN_POINT('Ctrl Pts',(11.1894202623362,12.2,0.560084444347706));
#194384=CARTESIAN_POINT('Ctrl Pts',(11.1924977846704,12.2,0.561558755076913));
#194385=CARTESIAN_POINT('Ctrl Pts',(11.1955753070045,12.2,0.563033065806121));
#194386=CARTESIAN_POINT('Ctrl Pts',(11.1986576579149,12.2,0.564514162982363));
#194387=CARTESIAN_POINT('Ctrl Pts',(11.2017447905532,12.2,0.566002057137232));
#194388=CARTESIAN_POINT('Ctrl Pts',(11.2058609672172,12.2,0.567985915920289));
#194389=CARTESIAN_POINT('Ctrl Pts',(11.2099856463879,12.2,0.569981857509243));
#194390=CARTESIAN_POINT('Ctrl Pts',(11.2141187215492,12.2,0.571989907454961));
#194391=CARTESIAN_POINT('Ctrl Pts',(11.217218528624,12.2,0.573495945256245));
#194392=CARTESIAN_POINT('Ctrl Pts',(11.2203230576252,12.2,0.575008791642777));
#194393=CARTESIAN_POINT('Ctrl Pts',(11.2234322652027,12.2,0.576528459531231));
#194394=CARTESIAN_POINT('Ctrl Pts',(11.2265414722154,12.2,0.578048127143612));
#194395=CARTESIAN_POINT('Ctrl Pts',(11.2296553571436,12.2,0.579574615508317));
#194396=CARTESIAN_POINT('Ctrl Pts',(11.2327738758533,12.2,0.581107932780002));
#194397=CARTESIAN_POINT('Ctrl Pts',(11.235892394563,12.2,0.582641250051688));
#194398=CARTESIAN_POINT('Ctrl Pts',(11.2390155465875,12.2,0.584181398040953));
#194399=CARTESIAN_POINT('Ctrl Pts',(11.2421432880992,12.2,0.585728385152007));
#194400=CARTESIAN_POINT('Ctrl Pts',(11.245271029611,12.2,0.587275372263061));
#194401=CARTESIAN_POINT('Ctrl Pts',(11.2484033592639,12.2,0.588829198389968));
#194402=CARTESIAN_POINT('Ctrl Pts',(11.2515402357332,12.2,0.590389873499935));
#194403=CARTESIAN_POINT('Ctrl Pts',(11.2546771122026,12.2,0.591950548609903));
#194404=CARTESIAN_POINT('Ctrl Pts',(11.2578185339551,12.2,0.593518072486248));
#194405=CARTESIAN_POINT('Ctrl Pts',(11.2609644574654,12.2,0.595092455053444));
#194406=CARTESIAN_POINT('Ctrl Pts',(11.2641103809757,12.2,0.59666683762064));
#194407=CARTESIAN_POINT('Ctrl Pts',(11.2672608046304,12.2,0.598248077771908));
#194408=CARTESIAN_POINT('Ctrl Pts',(11.2704156878396,12.2,0.599836185417745));
#194409=CARTESIAN_POINT('Ctrl Pts',(11.2735705710487,12.2,0.601424293063581));
#194410=CARTESIAN_POINT('Ctrl Pts',(11.2767299122758,12.2,0.603019267276549));
#194411=CARTESIAN_POINT('Ctrl Pts',(11.2798936682852,12.2,0.604621117884072));
#194412=CARTESIAN_POINT('Ctrl Pts',(11.2830574248694,12.2,0.606222968782597));
#194413=CARTESIAN_POINT('Ctrl Pts',(11.2862255958965,12.2,0.607831696166409));
#194414=CARTESIAN_POINT('Ctrl Pts',(11.2893981389832,12.2,0.609447308068814));
#194415=CARTESIAN_POINT('Ctrl Pts',(11.2936281954715,12.2,0.611601456782849));
#194416=CARTESIAN_POINT('Ctrl Pts',(11.2978660221283,12.2,0.613767846150855));
#194417=CARTESIAN_POINT('Ctrl Pts',(11.3021115206696,12.2,0.615946494305279));
#194418=CARTESIAN_POINT('Ctrl Pts',(11.3052956447202,12.2,0.617580480495307));
#194419=CARTESIAN_POINT('Ctrl Pts',(11.3084840831705,12.2,0.619221363751534));
#194420=CARTESIAN_POINT('Ctrl Pts',(11.3116767933039,12.2,0.62086915139906));
#194421=CARTESIAN_POINT('Ctrl Pts',(11.3148695040173,12.2,0.622516939345933));
#194422=CARTESIAN_POINT('Ctrl Pts',(11.3180664866986,12.2,0.624171632686409));
#194423=CARTESIAN_POINT('Ctrl Pts',(11.3212676989145,12.2,0.625833238595508));
#194424=CARTESIAN_POINT('Ctrl Pts',(11.3244689105487,12.2,0.627494844202749));
#194425=CARTESIAN_POINT('Ctrl Pts',(11.3276743522767,12.2,0.629163362400529));
#194426=CARTESIAN_POINT('Ctrl Pts',(11.3308839806126,12.2,0.63083880204916));
#194427=CARTESIAN_POINT('Ctrl Pts',(11.3340936089485,12.2,0.632514241697791));
#194428=CARTESIAN_POINT('Ctrl Pts',(11.337307424884,12.2,0.634196602661628));
#194429=CARTESIAN_POINT('Ctrl Pts',(11.3405253855591,12.2,0.635885892725853));
#194430=CARTESIAN_POINT('Ctrl Pts',(11.3437433462342,12.2,0.637575182790078));
#194431=CARTESIAN_POINT('Ctrl Pts',(11.3469654531671,12.2,0.639271401945137));
#194432=CARTESIAN_POINT('Ctrl Pts',(11.3501916627582,12.2,0.640974558008262));
#194433=CARTESIAN_POINT('Ctrl Pts',(11.3534178723494,12.2,0.642677714071387));
#194434=CARTESIAN_POINT('Ctrl Pts',(11.3566481849153,12.2,0.644387806525886));
#194435=CARTESIAN_POINT('Ctrl Pts',(11.3598825604224,12.2,0.646104844087896));
#194436=CARTESIAN_POINT('Ctrl Pts',(11.3631169359296,12.2,0.647821881649906));
#194437=CARTESIAN_POINT('Ctrl Pts',(11.3663553722123,12.2,0.649545863958999));
#194438=CARTESIAN_POINT('Ctrl Pts',(11.369597830381,12.2,0.651276798190114));
#194439=CARTESIAN_POINT('Ctrl Pts',(11.3728402885497,12.2,0.653007732421228));
#194440=CARTESIAN_POINT('Ctrl Pts',(11.3760867656766,12.2,0.654745619467243));
#194441=CARTESIAN_POINT('Ctrl Pts',(11.3793372227663,12.2,0.65649046561123));
#194442=CARTESIAN_POINT('Ctrl Pts',(11.3825876804465,12.2,0.658235312072197));
#194443=CARTESIAN_POINT('Ctrl Pts',(11.3858421171195,12.2,0.659987118460131));
#194444=CARTESIAN_POINT('Ctrl Pts',(11.3891004914269,12.2,0.661745891841688));
#194445=CARTESIAN_POINT('Ctrl Pts',(11.3934449895169,12.2,0.664090922484581));
#194446=CARTESIAN_POINT('Ctrl Pts',(11.3977964905477,12.2,0.666448337592532));
#194447=CARTESIAN_POINT('Ctrl Pts',(11.4021548971354,12.2,0.668818155564653));
#194448=CARTESIAN_POINT('Ctrl Pts',(11.4054237022246,12.2,0.670595519124467));
#194449=CARTESIAN_POINT('Ctrl Pts',(11.4086963915885,12.2,0.672379859213161));
#194450=CARTESIAN_POINT('Ctrl Pts',(11.411972922841,12.2,0.674171182861762));
#194451=CARTESIAN_POINT('Ctrl Pts',(11.4152494540936,12.2,0.675962506510362));
#194452=CARTESIAN_POINT('Ctrl Pts',(11.4185298269205,12.2,0.67776081332294));
#194453=CARTESIAN_POINT('Ctrl Pts',(11.4218140015923,12.2,0.679566110839722));
#194454=CARTESIAN_POINT('Ctrl Pts',(11.4261929015525,12.2,0.681973174414073));
#194455=CARTESIAN_POINT('Ctrl Pts',(11.4305785617466,12.2,0.684392664350729));
#194456=CARTESIAN_POINT('Ctrl Pts',(11.4349708937083,12.2,0.686824596483265));
#194457=CARTESIAN_POINT('Ctrl Pts',(11.4382651423802,12.2,0.688648545416993));
#194458=CARTESIAN_POINT('Ctrl Pts',(11.4415631447104,12.2,0.690479491583783));
#194459=CARTESIAN_POINT('Ctrl Pts',(11.4448648556318,12.2,0.692317444099715));
#194460=CARTESIAN_POINT('Ctrl Pts',(11.4481665665531,12.2,0.694155396615647));
#194461=CARTESIAN_POINT('Ctrl Pts',(11.4514719840484,12.2,0.696000354800609));
#194462=CARTESIAN_POINT('Ctrl Pts',(11.4547810613847,12.2,0.697852327408367));
#194463=CARTESIAN_POINT('Ctrl Pts',(11.4580901387211,12.2,0.699704300016125));
#194464=CARTESIAN_POINT('Ctrl Pts',(11.4614028748479,12.2,0.701563286711908));
#194465=CARTESIAN_POINT('Ctrl Pts',(11.4647192420186,12.2,0.703429290643153));
#194466=CARTESIAN_POINT('Ctrl Pts',(11.4691410653145,12.2,0.705917296110806));
#194467=CARTESIAN_POINT('Ctrl Pts',(11.4735693507915,12.2,0.7084177809819));
#194468=CARTESIAN_POINT('Ctrl Pts',(11.4780040719999,12.2,0.710930734999983));
#194469=CARTESIAN_POINT('Origin',(-5.66257110645729E-14,15.2,-1.77635683940025E-14));
#194470=CARTESIAN_POINT('',(10.2237731090076,15.2,1.76496130733463));
#194471=CARTESIAN_POINT('',(10.2237731090076,12.2,1.76496130733463));
#194472=CARTESIAN_POINT('',(10.2237731089999,15.2,1.76496130699999));
#194473=CARTESIAN_POINT('Origin',(-5.66257110645729E-14,12.2,-1.77635683940025E-14));
#194474=CARTESIAN_POINT('Origin',(-5.66257110645729E-14,15.2,-1.77635683940025E-14));
#194475=CARTESIAN_POINT('Origin',(-5.66257110645729E-14,15.2,-1.77635683940025E-14));
#194476=CARTESIAN_POINT('',(11.2599985479999,15.2,2.33718477899998));
#194477=CARTESIAN_POINT('',(11.1757778679999,15.2,2.71145515299998));
#194478=CARTESIAN_POINT('Origin',(-5.66257110645729E-14,15.2,-1.77635683940025E-14));
#194479=CARTESIAN_POINT('',(11.1757778679999,12.2,2.71145515299998));
#194480=CARTESIAN_POINT('',(11.1757778679999,15.2,2.71145515299998));
#194481=CARTESIAN_POINT('',(11.2599985479999,12.2,2.33718477899998));
#194482=CARTESIAN_POINT('Origin',(-5.66257110645729E-14,12.2,-1.77635683940025E-14));
#194483=CARTESIAN_POINT('',(11.2599985479999,15.2,2.33718477899998));
#194484=CARTESIAN_POINT('Ctrl Pts',(10.2237731089999,15.2,1.76496130799999));
#194485=CARTESIAN_POINT('Ctrl Pts',(10.2237731089999,11.6,1.76496130799999));
#194486=CARTESIAN_POINT('Ctrl Pts',(10.2239417409999,15.2,1.76500562399998));
#194487=CARTESIAN_POINT('Ctrl Pts',(10.2239417409999,11.6,1.76500562399998));
#194488=CARTESIAN_POINT('Ctrl Pts',(10.2242848729999,15.2,1.76509588899998));
#194489=CARTESIAN_POINT('Ctrl Pts',(10.2242848729999,11.6,1.76509588899998));
#194490=CARTESIAN_POINT('Ctrl Pts',(10.2248047309999,15.2,1.76523291899999));
#194491=CARTESIAN_POINT('Ctrl Pts',(10.2248047309999,11.6,1.76523291899999));
#194492=CARTESIAN_POINT('Ctrl Pts',(10.2255048889999,15.2,1.76541803299999));
#194493=CARTESIAN_POINT('Ctrl Pts',(10.2255048889999,11.6,1.76541803299999));
#194494=CARTESIAN_POINT('Ctrl Pts',(10.2263902529999,15.2,1.76565305799999));
#194495=CARTESIAN_POINT('Ctrl Pts',(10.2263902529999,11.6,1.76565305799999));
#194496=CARTESIAN_POINT('Ctrl Pts',(10.2272897259999,15.2,1.76589279499999));
#194497=CARTESIAN_POINT('Ctrl Pts',(10.2272897259999,11.6,1.76589279499999));
#194498=CARTESIAN_POINT('Ctrl Pts',(10.2281981499999,15.2,1.76613589499999));
#194499=CARTESIAN_POINT('Ctrl Pts',(10.2281981499999,11.6,1.76613589499999));
#194500=CARTESIAN_POINT('Ctrl Pts',(10.2291154919999,15.2,1.76638236599999));
#194501=CARTESIAN_POINT('Ctrl Pts',(10.2291154919999,11.6,1.76638236599999));
#194502=CARTESIAN_POINT('Ctrl Pts',(10.2300417219999,15.2,1.76663221999998));
#194503=CARTESIAN_POINT('Ctrl Pts',(10.2300417219999,11.6,1.76663221999998));
#194504=CARTESIAN_POINT('Ctrl Pts',(10.2309768119999,15.2,1.76688546699999));
#194505=CARTESIAN_POINT('Ctrl Pts',(10.2309768119999,11.6,1.76688546699999));
#194506=CARTESIAN_POINT('Ctrl Pts',(10.2319207289999,15.2,1.76714211799998));
#194507=CARTESIAN_POINT('Ctrl Pts',(10.2319207289999,11.6,1.76714211799998));
#194508=CARTESIAN_POINT('Ctrl Pts',(10.2328734439999,15.2,1.76740218199999));
#194509=CARTESIAN_POINT('Ctrl Pts',(10.2328734439999,11.6,1.76740218199999));
#194510=CARTESIAN_POINT('Ctrl Pts',(10.2338349259999,15.2,1.76766566999999));
#194511=CARTESIAN_POINT('Ctrl Pts',(10.2338349259999,11.6,1.76766566999999));
#194512=CARTESIAN_POINT('Ctrl Pts',(10.2348051459999,15.2,1.76793259399998));
#194513=CARTESIAN_POINT('Ctrl Pts',(10.2348051459999,11.6,1.76793259399998));
#194514=CARTESIAN_POINT('Ctrl Pts',(10.2357840739999,15.2,1.76820296099998));
#194515=CARTESIAN_POINT('Ctrl Pts',(10.2357840739999,11.6,1.76820296099998));
#194516=CARTESIAN_POINT('Ctrl Pts',(10.2367716789999,15.2,1.76847678099998));
#194517=CARTESIAN_POINT('Ctrl Pts',(10.2367716789999,11.6,1.76847678099998));
#194518=CARTESIAN_POINT('Ctrl Pts',(10.2377679339999,15.2,1.76875406799998));
#194519=CARTESIAN_POINT('Ctrl Pts',(10.2377679339999,11.6,1.76875406799998));
#194520=CARTESIAN_POINT('Ctrl Pts',(10.2387728089999,15.2,1.76903482699998));
#194521=CARTESIAN_POINT('Ctrl Pts',(10.2387728089999,11.6,1.76903482699998));
#194522=CARTESIAN_POINT('Ctrl Pts',(10.2397862729999,15.2,1.76931907099998));
#194523=CARTESIAN_POINT('Ctrl Pts',(10.2397862729999,11.6,1.76931907099998));
#194524=CARTESIAN_POINT('Ctrl Pts',(10.2408082999999,15.2,1.76960680999999));
#194525=CARTESIAN_POINT('Ctrl Pts',(10.2408082999999,11.6,1.76960680999999));
#194526=CARTESIAN_POINT('Ctrl Pts',(10.2418388579999,15.2,1.76989805099999));
#194527=CARTESIAN_POINT('Ctrl Pts',(10.2418388579999,11.6,1.76989805099998));
#194528=CARTESIAN_POINT('Ctrl Pts',(10.2428779189999,15.2,1.77019280699998));
#194529=CARTESIAN_POINT('Ctrl Pts',(10.2428779189999,11.6,1.77019280699998));
#194530=CARTESIAN_POINT('Ctrl Pts',(10.2439254559999,15.2,1.77049108599999));
#194531=CARTESIAN_POINT('Ctrl Pts',(10.2439254559999,11.6,1.77049108599999));
#194532=CARTESIAN_POINT('Ctrl Pts',(10.2449814379999,15.2,1.77079289599999));
#194533=CARTESIAN_POINT('Ctrl Pts',(10.2449814379999,11.6,1.77079289599999));
#194534=CARTESIAN_POINT('Ctrl Pts',(10.2460458399999,15.2,1.77109824999999));
#194535=CARTESIAN_POINT('Ctrl Pts',(10.2460458399999,11.6,1.77109824999999));
#194536=CARTESIAN_POINT('Ctrl Pts',(10.2471186289999,15.2,1.77140715399998));
#194537=CARTESIAN_POINT('Ctrl Pts',(10.2471186289999,11.6,1.77140715399998));
#194538=CARTESIAN_POINT('Ctrl Pts',(10.2481997809999,15.2,1.77171961899999));
#194539=CARTESIAN_POINT('Ctrl Pts',(10.2481997809999,11.6,1.77171961899999));
#194540=CARTESIAN_POINT('Ctrl Pts',(10.2492892659999,15.2,1.77203565399998));
#194541=CARTESIAN_POINT('Ctrl Pts',(10.2492892659999,11.6,1.77203565399998));
#194542=CARTESIAN_POINT('Ctrl Pts',(10.2503870569999,15.2,1.77235526999999));
#194543=CARTESIAN_POINT('Ctrl Pts',(10.2503870569999,11.6,1.77235526999999));
#194544=CARTESIAN_POINT('Ctrl Pts',(10.2514931249999,15.2,1.77267847299999));
#194545=CARTESIAN_POINT('Ctrl Pts',(10.2514931249999,11.6,1.77267847299999));
#194546=CARTESIAN_POINT('Ctrl Pts',(10.2526074429999,15.2,1.77300527499999));
#194547=CARTESIAN_POINT('Ctrl Pts',(10.2526074429999,11.6,1.77300527499999));
#194548=CARTESIAN_POINT('Ctrl Pts',(10.2537299839999,15.2,1.77333568399999));
#194549=CARTESIAN_POINT('Ctrl Pts',(10.2537299839999,11.6,1.77333568399999));
#194550=CARTESIAN_POINT('Ctrl Pts',(10.2548607199999,15.2,1.77366970799998));
#194551=CARTESIAN_POINT('Ctrl Pts',(10.2548607199999,11.6,1.77366970799998));
#194552=CARTESIAN_POINT('Ctrl Pts',(10.2559996249999,15.2,1.77400735799999));
#194553=CARTESIAN_POINT('Ctrl Pts',(10.2559996249999,11.6,1.77400735799999));
#194554=CARTESIAN_POINT('Ctrl Pts',(10.2571466689999,15.2,1.77434864199999));
#194555=CARTESIAN_POINT('Ctrl Pts',(10.2571466689999,11.6,1.77434864199998));
#194556=CARTESIAN_POINT('Ctrl Pts',(10.2583018279999,15.2,1.77469356899998));
#194557=CARTESIAN_POINT('Ctrl Pts',(10.2583018279999,11.6,1.77469356899998));
#194558=CARTESIAN_POINT('Ctrl Pts',(10.2594650729999,15.2,1.77504214699999));
#194559=CARTESIAN_POINT('Ctrl Pts',(10.2594650729999,11.6,1.77504214699999));
#194560=CARTESIAN_POINT('Ctrl Pts',(10.2606363769999,15.2,1.77539438599998));
#194561=CARTESIAN_POINT('Ctrl Pts',(10.2606363769999,11.6,1.77539438599998));
#194562=CARTESIAN_POINT('Ctrl Pts',(10.2618157169999,15.2,1.77575029399998));
#194563=CARTESIAN_POINT('Ctrl Pts',(10.2618157169999,11.6,1.77575029399998));
#194564=CARTESIAN_POINT('Ctrl Pts',(10.2630030619999,15.2,1.77610988099998));
#194565=CARTESIAN_POINT('Ctrl Pts',(10.2630030619999,11.6,1.77610988099998));
#194566=CARTESIAN_POINT('Ctrl Pts',(10.2641983869999,15.2,1.77647315299998));
#194567=CARTESIAN_POINT('Ctrl Pts',(10.2641983869999,11.6,1.77647315299998));
#194568=CARTESIAN_POINT('Ctrl Pts',(10.2654016659999,15.2,1.77684012099999));
#194569=CARTESIAN_POINT('Ctrl Pts',(10.2654016659999,11.6,1.77684012099998));
#194570=CARTESIAN_POINT('Ctrl Pts',(10.2666128729999,15.2,1.77721079199999));
#194571=CARTESIAN_POINT('Ctrl Pts',(10.2666128729999,11.6,1.77721079199999));
#194572=CARTESIAN_POINT('Ctrl Pts',(10.2678319819999,15.2,1.77758517599999));
#194573=CARTESIAN_POINT('Ctrl Pts',(10.2678319819999,11.6,1.77758517599999));
#194574=CARTESIAN_POINT('Ctrl Pts',(10.2690589659999,15.2,1.77796327999999));
#194575=CARTESIAN_POINT('Ctrl Pts',(10.2690589659999,11.6,1.77796327999999));
#194576=CARTESIAN_POINT('Ctrl Pts',(10.2702937999999,15.2,1.77834511299999));
#194577=CARTESIAN_POINT('Ctrl Pts',(10.2702937999999,11.6,1.77834511299999));
#194578=CARTESIAN_POINT('Ctrl Pts',(10.2715364579999,15.2,1.77873068299998));
#194579=CARTESIAN_POINT('Ctrl Pts',(10.2715364579999,11.6,1.77873068299998));
#194580=CARTESIAN_POINT('Ctrl Pts',(10.2727869139999,15.2,1.77911999899999));
#194581=CARTESIAN_POINT('Ctrl Pts',(10.2727869139999,11.6,1.77911999899999));
#194582=CARTESIAN_POINT('Ctrl Pts',(10.2740451429999,15.2,1.77951306799998));
#194583=CARTESIAN_POINT('Ctrl Pts',(10.2740451429999,11.6,1.77951306799998));
#194584=CARTESIAN_POINT('Ctrl Pts',(10.2753111179999,15.2,1.77990989899998));
#194585=CARTESIAN_POINT('Ctrl Pts',(10.2753111179999,11.6,1.77990989899998));
#194586=CARTESIAN_POINT('Ctrl Pts',(10.2765848159999,15.2,1.78031050099999));
#194587=CARTESIAN_POINT('Ctrl Pts',(10.2765848159999,11.6,1.78031050099999));
#194588=CARTESIAN_POINT('Ctrl Pts',(10.2778662099999,15.2,1.78071487999999));
#194589=CARTESIAN_POINT('Ctrl Pts',(10.2778662099999,11.6,1.78071487999999));
#194590=CARTESIAN_POINT('Ctrl Pts',(10.2791552759999,15.2,1.78112304599999));
#194591=CARTESIAN_POINT('Ctrl Pts',(10.2791552759999,11.6,1.78112304599999));
#194592=CARTESIAN_POINT('Ctrl Pts',(10.2804519869999,15.2,1.78153500599999));
#194593=CARTESIAN_POINT('Ctrl Pts',(10.2804519869999,11.6,1.78153500599999));
#194594=CARTESIAN_POINT('Ctrl Pts',(10.2817563209999,15.2,1.78195076799998));
#194595=CARTESIAN_POINT('Ctrl Pts',(10.2817563209999,11.6,1.78195076799998));
#194596=CARTESIAN_POINT('Ctrl Pts',(10.2830682509999,15.2,1.78237033999999));
#194597=CARTESIAN_POINT('Ctrl Pts',(10.2830682509999,11.6,1.78237033999999));
#194598=CARTESIAN_POINT('Ctrl Pts',(10.2843877529999,15.2,1.78279372899999));
#194599=CARTESIAN_POINT('Ctrl Pts',(10.2843877529999,11.6,1.78279372899999));
#194600=CARTESIAN_POINT('Ctrl Pts',(10.2857148029999,15.2,1.78322094399999));
#194601=CARTESIAN_POINT('Ctrl Pts',(10.2857148029999,11.6,1.78322094399999));
#194602=CARTESIAN_POINT('Ctrl Pts',(10.2870493749999,15.2,1.78365199299999));
#194603=CARTESIAN_POINT('Ctrl Pts',(10.2870493749999,11.6,1.78365199299999));
#194604=CARTESIAN_POINT('Ctrl Pts',(10.2883914449999,15.2,1.78408688299998));
#194605=CARTESIAN_POINT('Ctrl Pts',(10.2883914449999,11.6,1.78408688299998));
#194606=CARTESIAN_POINT('Ctrl Pts',(10.2897409889999,15.2,1.78452562099999));
#194607=CARTESIAN_POINT('Ctrl Pts',(10.2897409889999,11.6,1.78452562099999));
#194608=CARTESIAN_POINT('Ctrl Pts',(10.2910979839999,15.2,1.78496821599999));
#194609=CARTESIAN_POINT('Ctrl Pts',(10.2910979839999,11.6,1.78496821599999));
#194610=CARTESIAN_POINT('Ctrl Pts',(10.2924624019999,15.2,1.78541467399999));
#194611=CARTESIAN_POINT('Ctrl Pts',(10.2924624019999,11.6,1.78541467399999));
#194612=CARTESIAN_POINT('Ctrl Pts',(10.2938342229999,15.2,1.78586500399998));
#194613=CARTESIAN_POINT('Ctrl Pts',(10.2938342229999,11.6,1.78586500399998));
#194614=CARTESIAN_POINT('Ctrl Pts',(10.2952134229999,15.2,1.78631921299999));
#194615=CARTESIAN_POINT('Ctrl Pts',(10.2952134229999,11.6,1.78631921299999));
#194616=CARTESIAN_POINT('Ctrl Pts',(10.2965999749999,15.2,1.78677730799999));
#194617=CARTESIAN_POINT('Ctrl Pts',(10.2965999749999,11.6,1.78677730799999));
#194618=CARTESIAN_POINT('Ctrl Pts',(10.2979938569999,15.2,1.78723929699999));
#194619=CARTESIAN_POINT('Ctrl Pts',(10.2979938569999,11.6,1.78723929699998));
#194620=CARTESIAN_POINT('Ctrl Pts',(10.2993950459999,15.2,1.78770518799999));
#194621=CARTESIAN_POINT('Ctrl Pts',(10.2993950459999,11.6,1.78770518799999));
#194622=CARTESIAN_POINT('Ctrl Pts',(10.3008035169999,15.2,1.78817498699999));
#194623=CARTESIAN_POINT('Ctrl Pts',(10.3008035169999,11.6,1.78817498699999));
#194624=CARTESIAN_POINT('Ctrl Pts',(10.3022192479999,15.2,1.78864870099999));
#194625=CARTESIAN_POINT('Ctrl Pts',(10.3022192479999,11.6,1.78864870099999));
#194626=CARTESIAN_POINT('Ctrl Pts',(10.3036422139999,15.2,1.78912633799999));
#194627=CARTESIAN_POINT('Ctrl Pts',(10.3036422139999,11.6,1.78912633799999));
#194628=CARTESIAN_POINT('Ctrl Pts',(10.3050723929999,15.2,1.78960790499998));
#194629=CARTESIAN_POINT('Ctrl Pts',(10.3050723929999,11.6,1.78960790499998));
#194630=CARTESIAN_POINT('Ctrl Pts',(10.3065097609999,15.2,1.79009340899999));
#194631=CARTESIAN_POINT('Ctrl Pts',(10.3065097609999,11.6,1.79009340899999));
#194632=CARTESIAN_POINT('Ctrl Pts',(10.3079542959999,15.2,1.79058285899998));
#194633=CARTESIAN_POINT('Ctrl Pts',(10.3079542959999,11.6,1.79058285899998));
#194634=CARTESIAN_POINT('Ctrl Pts',(10.3094059739999,15.2,1.79107625799999));
#194635=CARTESIAN_POINT('Ctrl Pts',(10.3094059739999,11.6,1.79107625799999));
#194636=CARTESIAN_POINT('Ctrl Pts',(10.3108647719999,15.2,1.79157361699998));
#194637=CARTESIAN_POINT('Ctrl Pts',(10.3108647719999,11.6,1.79157361699998));
#194638=CARTESIAN_POINT('Ctrl Pts',(10.3123306679999,15.2,1.79207494199999));
#194639=CARTESIAN_POINT('Ctrl Pts',(10.3123306679999,11.6,1.79207494199999));
#194640=CARTESIAN_POINT('Ctrl Pts',(10.3138036379999,15.2,1.79258023699999));
#194641=CARTESIAN_POINT('Ctrl Pts',(10.3138036379999,11.6,1.79258023699999));
#194642=CARTESIAN_POINT('Ctrl Pts',(10.3152836599999,15.2,1.79308951299999));
#194643=CARTESIAN_POINT('Ctrl Pts',(10.3152836599999,11.6,1.79308951299999));
#194644=CARTESIAN_POINT('Ctrl Pts',(10.3167707109999,15.2,1.79360277499998));
#194645=CARTESIAN_POINT('Ctrl Pts',(10.3167707109999,11.6,1.79360277499998));
#194646=CARTESIAN_POINT('Ctrl Pts',(10.3182647709999,15.2,1.79412002899999));
#194647=CARTESIAN_POINT('Ctrl Pts',(10.3182647709999,11.6,1.79412002899999));
#194648=CARTESIAN_POINT('Ctrl Pts',(10.3197658129999,15.2,1.79464128299998));
#194649=CARTESIAN_POINT('Ctrl Pts',(10.3197658129999,11.6,1.79464128299998));
#194650=CARTESIAN_POINT('Ctrl Pts',(10.3212738189999,15.2,1.79516654399999));
#194651=CARTESIAN_POINT('Ctrl Pts',(10.3212738189999,11.6,1.79516654399999));
#194652=CARTESIAN_POINT('Ctrl Pts',(10.3227887639999,15.2,1.79569581799999));
#194653=CARTESIAN_POINT('Ctrl Pts',(10.3227887639999,11.6,1.79569581799999));
#194654=CARTESIAN_POINT('Ctrl Pts',(10.3243106259999,15.2,1.79622911099999));
#194655=CARTESIAN_POINT('Ctrl Pts',(10.3243106259999,11.6,1.79622911099999));
#194656=CARTESIAN_POINT('Ctrl Pts',(10.3258393839999,15.2,1.79676642999999));
#194657=CARTESIAN_POINT('Ctrl Pts',(10.3258393839999,11.6,1.79676642999999));
#194658=CARTESIAN_POINT('Ctrl Pts',(10.3273750169999,15.2,1.79730778399998));
#194659=CARTESIAN_POINT('Ctrl Pts',(10.3273750169999,11.6,1.79730778399998));
#194660=CARTESIAN_POINT('Ctrl Pts',(10.3289175009999,15.2,1.79785317599999));
#194661=CARTESIAN_POINT('Ctrl Pts',(10.3289175009999,11.6,1.79785317599999));
#194662=CARTESIAN_POINT('Ctrl Pts',(10.3304668139999,15.2,1.79840261399999));
#194663=CARTESIAN_POINT('Ctrl Pts',(10.3304668139999,11.6,1.79840261399998));
#194664=CARTESIAN_POINT('Ctrl Pts',(10.3320229349999,15.2,1.79895610499999));
#194665=CARTESIAN_POINT('Ctrl Pts',(10.3320229349999,11.6,1.79895610499999));
#194666=CARTESIAN_POINT('Ctrl Pts',(10.3335858439999,15.2,1.79951365499999));
#194667=CARTESIAN_POINT('Ctrl Pts',(10.3335858439999,11.6,1.79951365499999));
#194668=CARTESIAN_POINT('Ctrl Pts',(10.3351555169999,15.2,1.80007527099999));
#194669=CARTESIAN_POINT('Ctrl Pts',(10.3351555169999,11.6,1.80007527099999));
#194670=CARTESIAN_POINT('Ctrl Pts',(10.3367319329999,15.2,1.80064095699999));
#194671=CARTESIAN_POINT('Ctrl Pts',(10.3367319329999,11.6,1.80064095699999));
#194672=CARTESIAN_POINT('Ctrl Pts',(10.3383150709999,15.2,1.80121072199999));
#194673=CARTESIAN_POINT('Ctrl Pts',(10.3383150709999,11.6,1.80121072199999));
#194674=CARTESIAN_POINT('Ctrl Pts',(10.3399049089999,15.2,1.80178457099998));
#194675=CARTESIAN_POINT('Ctrl Pts',(10.3399049089999,11.6,1.80178457099998));
#194676=CARTESIAN_POINT('Ctrl Pts',(10.3415014269999,15.2,1.80236251099998));
#194677=CARTESIAN_POINT('Ctrl Pts',(10.3415014269999,11.6,1.80236251099998));
#194678=CARTESIAN_POINT('Ctrl Pts',(10.3431046029999,15.2,1.80294454799999));
#194679=CARTESIAN_POINT('Ctrl Pts',(10.3431046029999,11.6,1.80294454799998));
#194680=CARTESIAN_POINT('Ctrl Pts',(10.3447144149999,15.2,1.80353068699999));
#194681=CARTESIAN_POINT('Ctrl Pts',(10.3447144149999,11.6,1.80353068699999));
#194682=CARTESIAN_POINT('Ctrl Pts',(10.3463308429999,15.2,1.80412093599998));
#194683=CARTESIAN_POINT('Ctrl Pts',(10.3463308429999,11.6,1.80412093599998));
#194684=CARTESIAN_POINT('Ctrl Pts',(10.3479538659999,15.2,1.80471529999998));
#194685=CARTESIAN_POINT('Ctrl Pts',(10.3479538659999,11.6,1.80471529999998));
#194686=CARTESIAN_POINT('Ctrl Pts',(10.3495834629999,15.2,1.80531378499999));
#194687=CARTESIAN_POINT('Ctrl Pts',(10.3495834629999,11.6,1.80531378499999));
#194688=CARTESIAN_POINT('Ctrl Pts',(10.3512196119999,15.2,1.80591639799998));
#194689=CARTESIAN_POINT('Ctrl Pts',(10.3512196119999,11.6,1.80591639799998));
#194690=CARTESIAN_POINT('Ctrl Pts',(10.3528622949999,15.2,1.80652314399998));
#194691=CARTESIAN_POINT('Ctrl Pts',(10.3528622949999,11.6,1.80652314399998));
#194692=CARTESIAN_POINT('Ctrl Pts',(10.3545114879999,15.2,1.80713402899999));
#194693=CARTESIAN_POINT('Ctrl Pts',(10.3545114879999,11.6,1.80713402899999));
#194694=CARTESIAN_POINT('Ctrl Pts',(10.3561671729999,15.2,1.80774905899999));
#194695=CARTESIAN_POINT('Ctrl Pts',(10.3561671729999,11.6,1.80774905899999));
#194696=CARTESIAN_POINT('Ctrl Pts',(10.3578293269999,15.2,1.80836824099998));
#194697=CARTESIAN_POINT('Ctrl Pts',(10.3578293269999,11.6,1.80836824099998));
#194698=CARTESIAN_POINT('Ctrl Pts',(10.3594979319999,15.2,1.80899157899999));
#194699=CARTESIAN_POINT('Ctrl Pts',(10.3594979319999,11.6,1.80899157899999));
#194700=CARTESIAN_POINT('Ctrl Pts',(10.3611729669999,15.2,1.80961908099999));
#194701=CARTESIAN_POINT('Ctrl Pts',(10.3611729669999,11.6,1.80961908099999));
#194702=CARTESIAN_POINT('Ctrl Pts',(10.3628544089999,15.2,1.81025075099999));
#194703=CARTESIAN_POINT('Ctrl Pts',(10.3628544089999,11.6,1.81025075099999));
#194704=CARTESIAN_POINT('Ctrl Pts',(10.3645422419999,15.2,1.81088659599999));
#194705=CARTESIAN_POINT('Ctrl Pts',(10.3645422419999,11.6,1.81088659599998));
#194706=CARTESIAN_POINT('Ctrl Pts',(10.3662364429999,15.2,1.81152661999999));
#194707=CARTESIAN_POINT('Ctrl Pts',(10.3662364429999,11.6,1.81152661999999));
#194708=CARTESIAN_POINT('Ctrl Pts',(10.3679369919999,15.2,1.81217083099999));
#194709=CARTESIAN_POINT('Ctrl Pts',(10.3679369919999,11.6,1.81217083099999));
#194710=CARTESIAN_POINT('Ctrl Pts',(10.3696438709999,15.2,1.81281923299998));
#194711=CARTESIAN_POINT('Ctrl Pts',(10.3696438709999,11.6,1.81281923299998));
#194712=CARTESIAN_POINT('Ctrl Pts',(10.3713570579999,15.2,1.81347183299998));
#194713=CARTESIAN_POINT('Ctrl Pts',(10.3713570579999,11.6,1.81347183299998));
#194714=CARTESIAN_POINT('Ctrl Pts',(10.3730765319999,15.2,1.81412863499999));
#194715=CARTESIAN_POINT('Ctrl Pts',(10.3730765319999,11.6,1.81412863499998));
#194716=CARTESIAN_POINT('Ctrl Pts',(10.3748022759999,15.2,1.81478964499998));
#194717=CARTESIAN_POINT('Ctrl Pts',(10.3748022759999,11.6,1.81478964499998));
#194718=CARTESIAN_POINT('Ctrl Pts',(10.3765342689999,15.2,1.81545486999998));
#194719=CARTESIAN_POINT('Ctrl Pts',(10.3765342689999,11.6,1.81545486999998));
#194720=CARTESIAN_POINT('Ctrl Pts',(10.3782724909999,15.2,1.81612431399999));
#194721=CARTESIAN_POINT('Ctrl Pts',(10.3782724909999,11.6,1.81612431399999));
#194722=CARTESIAN_POINT('Ctrl Pts',(10.3800169229999,15.2,1.81679798299998));
#194723=CARTESIAN_POINT('Ctrl Pts',(10.3800169229999,11.6,1.81679798299998));
#194724=CARTESIAN_POINT('Ctrl Pts',(10.3817675449999,15.2,1.81747588299999));
#194725=CARTESIAN_POINT('Ctrl Pts',(10.3817675449999,11.6,1.81747588299999));
#194726=CARTESIAN_POINT('Ctrl Pts',(10.3835243379999,15.2,1.81815801799999));
#194727=CARTESIAN_POINT('Ctrl Pts',(10.3835243379999,11.6,1.81815801799999));
#194728=CARTESIAN_POINT('Ctrl Pts',(10.3852872809999,15.2,1.81884439299999));
#194729=CARTESIAN_POINT('Ctrl Pts',(10.3852872809999,11.6,1.81884439299999));
#194730=CARTESIAN_POINT('Ctrl Pts',(10.3870563549999,15.2,1.81953501599999));
#194731=CARTESIAN_POINT('Ctrl Pts',(10.3870563549999,11.6,1.81953501599999));
#194732=CARTESIAN_POINT('Ctrl Pts',(10.3888315429999,15.2,1.82022989099998));
#194733=CARTESIAN_POINT('Ctrl Pts',(10.3888315429999,11.6,1.82022989099998));
#194734=CARTESIAN_POINT('Ctrl Pts',(10.3906128229999,15.2,1.82092902299999));
#194735=CARTESIAN_POINT('Ctrl Pts',(10.3906128229999,11.6,1.82092902299999));
#194736=CARTESIAN_POINT('Ctrl Pts',(10.3924001779999,15.2,1.82163241699998));
#194737=CARTESIAN_POINT('Ctrl Pts',(10.3924001779999,11.6,1.82163241699998));
#194738=CARTESIAN_POINT('Ctrl Pts',(10.3941935869999,15.2,1.82234007799998));
#194739=CARTESIAN_POINT('Ctrl Pts',(10.3941935869999,11.6,1.82234007799998));
#194740=CARTESIAN_POINT('Ctrl Pts',(10.3959930309999,15.2,1.82305201299998));
#194741=CARTESIAN_POINT('Ctrl Pts',(10.3959930309999,11.6,1.82305201299998));
#194742=CARTESIAN_POINT('Ctrl Pts',(10.3977984929999,15.2,1.82376822499998));
#194743=CARTESIAN_POINT('Ctrl Pts',(10.3977984929999,11.6,1.82376822499998));
#194744=CARTESIAN_POINT('Ctrl Pts',(10.3996099509999,15.2,1.82448872199998));
#194745=CARTESIAN_POINT('Ctrl Pts',(10.3996099509999,11.6,1.82448872199998));
#194746=CARTESIAN_POINT('Ctrl Pts',(10.4014273889999,15.2,1.82521350599998));
#194747=CARTESIAN_POINT('Ctrl Pts',(10.4014273889999,11.6,1.82521350599998));
#194748=CARTESIAN_POINT('Ctrl Pts',(10.4032507859999,15.2,1.82594258299998));
#194749=CARTESIAN_POINT('Ctrl Pts',(10.4032507859999,11.6,1.82594258299998));
#194750=CARTESIAN_POINT('Ctrl Pts',(10.4050801249999,15.2,1.82667595899999));
#194751=CARTESIAN_POINT('Ctrl Pts',(10.4050801249999,11.6,1.82667595899999));
#194752=CARTESIAN_POINT('Ctrl Pts',(10.4069153869999,15.2,1.82741363799999));
#194753=CARTESIAN_POINT('Ctrl Pts',(10.4069153869999,11.6,1.82741363799999));
#194754=CARTESIAN_POINT('Ctrl Pts',(10.4087565519999,15.2,1.82815562599998));
#194755=CARTESIAN_POINT('Ctrl Pts',(10.4087565519999,11.6,1.82815562599998));
#194756=CARTESIAN_POINT('Ctrl Pts',(10.4106036029999,15.2,1.82890192799999));
#194757=CARTESIAN_POINT('Ctrl Pts',(10.4106036029999,11.6,1.82890192799999));
#194758=CARTESIAN_POINT('Ctrl Pts',(10.4124565199999,15.2,1.82965254699999));
#194759=CARTESIAN_POINT('Ctrl Pts',(10.4124565199999,11.6,1.82965254699999));
#194760=CARTESIAN_POINT('Ctrl Pts',(10.4143152849999,15.2,1.83040748999999));
#194761=CARTESIAN_POINT('Ctrl Pts',(10.4143152849999,11.6,1.83040748999999));
#194762=CARTESIAN_POINT('Ctrl Pts',(10.4161798809999,15.2,1.83116676099999));
#194763=CARTESIAN_POINT('Ctrl Pts',(10.4161798809999,11.6,1.83116676099999));
#194764=CARTESIAN_POINT('Ctrl Pts',(10.4180502869999,15.2,1.83193036499999));
#194765=CARTESIAN_POINT('Ctrl Pts',(10.4180502869999,11.6,1.83193036499999));
#194766=CARTESIAN_POINT('Ctrl Pts',(10.4199264869999,15.2,1.83269830799999));
#194767=CARTESIAN_POINT('Ctrl Pts',(10.4199264869999,11.6,1.83269830799999));
#194768=CARTESIAN_POINT('Ctrl Pts',(10.4218084619999,15.2,1.83347059299999));
#194769=CARTESIAN_POINT('Ctrl Pts',(10.4218084619999,11.6,1.83347059299999));
#194770=CARTESIAN_POINT('Ctrl Pts',(10.4236961939999,15.2,1.83424722499999));
#194771=CARTESIAN_POINT('Ctrl Pts',(10.4236961939999,11.6,1.83424722499998));
#194772=CARTESIAN_POINT('Ctrl Pts',(10.4255896649999,15.2,1.83502820899998));
#194773=CARTESIAN_POINT('Ctrl Pts',(10.4255896649999,11.6,1.83502820899998));
#194774=CARTESIAN_POINT('Ctrl Pts',(10.4274888559999,15.2,1.83581354999999));
#194775=CARTESIAN_POINT('Ctrl Pts',(10.4274888559999,11.6,1.83581354999998));
#194776=CARTESIAN_POINT('Ctrl Pts',(10.4293937499999,15.2,1.83660325299998));
#194777=CARTESIAN_POINT('Ctrl Pts',(10.4293937499999,11.6,1.83660325299998));
#194778=CARTESIAN_POINT('Ctrl Pts',(10.4313043289999,15.2,1.83739732299999));
#194779=CARTESIAN_POINT('Ctrl Pts',(10.4313043289999,11.6,1.83739732299998));
#194780=CARTESIAN_POINT('Ctrl Pts',(10.4332205739999,15.2,1.83819576399999));
#194781=CARTESIAN_POINT('Ctrl Pts',(10.4332205739999,11.6,1.83819576399999));
#194782=CARTESIAN_POINT('Ctrl Pts',(10.4351424679999,15.2,1.83899857999998));
#194783=CARTESIAN_POINT('Ctrl Pts',(10.4351424679999,11.6,1.83899857999998));
#194784=CARTESIAN_POINT('Ctrl Pts',(10.4370699929999,15.2,1.83980577599999));
#194785=CARTESIAN_POINT('Ctrl Pts',(10.4370699929999,11.6,1.83980577599998));
#194786=CARTESIAN_POINT('Ctrl Pts',(10.4390031319999,15.2,1.84061735699999));
#194787=CARTESIAN_POINT('Ctrl Pts',(10.4390031319999,11.6,1.84061735699998));
#194788=CARTESIAN_POINT('Ctrl Pts',(10.4409418659999,15.2,1.84143332699998));
#194789=CARTESIAN_POINT('Ctrl Pts',(10.4409418659999,11.6,1.84143332699998));
#194790=CARTESIAN_POINT('Ctrl Pts',(10.4428861799999,15.2,1.84225368999998));
#194791=CARTESIAN_POINT('Ctrl Pts',(10.4428861799999,11.6,1.84225368999998));
#194792=CARTESIAN_POINT('Ctrl Pts',(10.4448360519999,15.2,1.84307845199998));
#194793=CARTESIAN_POINT('Ctrl Pts',(10.4448360519999,11.6,1.84307845199998));
#194794=CARTESIAN_POINT('Ctrl Pts',(10.4467914679999,15.2,1.84390761799999));
#194795=CARTESIAN_POINT('Ctrl Pts',(10.4467914679999,11.6,1.84390761799999));
#194796=CARTESIAN_POINT('Ctrl Pts',(10.4487524099999,15.2,1.84474118999999));
#194797=CARTESIAN_POINT('Ctrl Pts',(10.4487524099999,11.6,1.84474118999999));
#194798=CARTESIAN_POINT('Ctrl Pts',(10.4507188599999,15.2,1.84557917299998));
#194799=CARTESIAN_POINT('Ctrl Pts',(10.4507188599999,11.6,1.84557917299998));
#194800=CARTESIAN_POINT('Ctrl Pts',(10.4526908009999,15.2,1.84642157199999));
#194801=CARTESIAN_POINT('Ctrl Pts',(10.4526908009999,11.6,1.84642157199999));
#194802=CARTESIAN_POINT('Ctrl Pts',(10.4546682149999,15.2,1.84726839199998));
#194803=CARTESIAN_POINT('Ctrl Pts',(10.4546682149999,11.6,1.84726839199998));
#194804=CARTESIAN_POINT('Ctrl Pts',(10.4566510849999,15.2,1.84811963699998));
#194805=CARTESIAN_POINT('Ctrl Pts',(10.4566510849999,11.6,1.84811963699998));
#194806=CARTESIAN_POINT('Ctrl Pts',(10.4586393939999,15.2,1.84897530999999));
#194807=CARTESIAN_POINT('Ctrl Pts',(10.4586393939999,11.6,1.84897530999998));
#194808=CARTESIAN_POINT('Ctrl Pts',(10.4606331249999,15.2,1.84983541599999));
#194809=CARTESIAN_POINT('Ctrl Pts',(10.4606331249999,11.6,1.84983541599998));
#194810=CARTESIAN_POINT('Ctrl Pts',(10.4626322619999,15.2,1.85069995999998));
#194811=CARTESIAN_POINT('Ctrl Pts',(10.4626322619999,11.6,1.85069995999998));
#194812=CARTESIAN_POINT('Ctrl Pts',(10.4646367859999,15.2,1.85156894599999));
#194813=CARTESIAN_POINT('Ctrl Pts',(10.4646367859999,11.6,1.85156894599999));
#194814=CARTESIAN_POINT('Ctrl Pts',(10.4666466809999,15.2,1.85244237799999));
#194815=CARTESIAN_POINT('Ctrl Pts',(10.4666466809999,11.6,1.85244237799999));
#194816=CARTESIAN_POINT('Ctrl Pts',(10.4686619289999,15.2,1.85332025999998));
#194817=CARTESIAN_POINT('Ctrl Pts',(10.4686619289999,11.6,1.85332025999998));
#194818=CARTESIAN_POINT('Ctrl Pts',(10.4706825139999,15.2,1.85420259599999));
#194819=CARTESIAN_POINT('Ctrl Pts',(10.4706825139999,11.6,1.85420259599998));
#194820=CARTESIAN_POINT('Ctrl Pts',(10.4727084189999,15.2,1.85508938999998));
#194821=CARTESIAN_POINT('Ctrl Pts',(10.4727084189999,11.6,1.85508938999998));
#194822=CARTESIAN_POINT('Ctrl Pts',(10.4747396279999,15.2,1.85598064699999));
#194823=CARTESIAN_POINT('Ctrl Pts',(10.4747396279999,11.6,1.85598064699999));
#194824=CARTESIAN_POINT('Ctrl Pts',(10.4767761229999,15.2,1.85687637099999));
#194825=CARTESIAN_POINT('Ctrl Pts',(10.4767761229999,11.6,1.85687637099999));
#194826=CARTESIAN_POINT('Ctrl Pts',(10.4788178879999,15.2,1.85777656499999));
#194827=CARTESIAN_POINT('Ctrl Pts',(10.4788178879999,11.6,1.85777656499999));
#194828=CARTESIAN_POINT('Ctrl Pts',(10.4808649049999,15.2,1.85868123499999));
#194829=CARTESIAN_POINT('Ctrl Pts',(10.4808649049999,11.6,1.85868123499999));
#194830=CARTESIAN_POINT('Ctrl Pts',(10.4829171589999,15.2,1.85959038199998));
#194831=CARTESIAN_POINT('Ctrl Pts',(10.4829171589999,11.6,1.85959038199998));
#194832=CARTESIAN_POINT('Ctrl Pts',(10.4849746339999,15.2,1.86050401299998));
#194833=CARTESIAN_POINT('Ctrl Pts',(10.4849746339999,11.6,1.86050401299998));
#194834=CARTESIAN_POINT('Ctrl Pts',(10.4870373119999,15.2,1.86142212899998));
#194835=CARTESIAN_POINT('Ctrl Pts',(10.4870373119999,11.6,1.86142212899998));
#194836=CARTESIAN_POINT('Ctrl Pts',(10.4891051769999,15.2,1.86234473799999));
#194837=CARTESIAN_POINT('Ctrl Pts',(10.4891051769999,11.6,1.86234473799999));
#194838=CARTESIAN_POINT('Ctrl Pts',(10.4911782119999,15.2,1.86327183999999));
#194839=CARTESIAN_POINT('Ctrl Pts',(10.4911782119999,11.6,1.86327183999999));
#194840=CARTESIAN_POINT('Ctrl Pts',(10.4932564019999,15.2,1.86420344099998));
#194841=CARTESIAN_POINT('Ctrl Pts',(10.4932564019999,11.6,1.86420344099998));
#194842=CARTESIAN_POINT('Ctrl Pts',(10.4953397299999,15.2,1.86513954399999));
#194843=CARTESIAN_POINT('Ctrl Pts',(10.4953397299999,11.6,1.86513954399999));
#194844=CARTESIAN_POINT('Ctrl Pts',(10.4974281779999,15.2,1.86608015299999));
#194845=CARTESIAN_POINT('Ctrl Pts',(10.4974281779999,11.6,1.86608015299999));
#194846=CARTESIAN_POINT('Ctrl Pts',(10.4995217329999,15.2,1.86702527299999));
#194847=CARTESIAN_POINT('Ctrl Pts',(10.4995217329999,11.6,1.86702527299999));
#194848=CARTESIAN_POINT('Ctrl Pts',(10.5016203769999,15.2,1.86797490599998));
#194849=CARTESIAN_POINT('Ctrl Pts',(10.5016203769999,11.6,1.86797490599998));
#194850=CARTESIAN_POINT('Ctrl Pts',(10.5037240939999,15.2,1.86892905699999));
#194851=CARTESIAN_POINT('Ctrl Pts',(10.5037240939999,11.6,1.86892905699999));
#194852=CARTESIAN_POINT('Ctrl Pts',(10.5058328669999,15.2,1.86988772999999));
#194853=CARTESIAN_POINT('Ctrl Pts',(10.5058328669999,11.6,1.86988772999999));
#194854=CARTESIAN_POINT('Ctrl Pts',(10.5079466819999,15.2,1.87085092699999));
#194855=CARTESIAN_POINT('Ctrl Pts',(10.5079466819999,11.6,1.87085092699998));
#194856=CARTESIAN_POINT('Ctrl Pts',(10.5100655219999,15.2,1.87181865399999));
#194857=CARTESIAN_POINT('Ctrl Pts',(10.5100655219999,11.6,1.87181865399999));
#194858=CARTESIAN_POINT('Ctrl Pts',(10.5121893699999,15.2,1.87279091299999));
#194859=CARTESIAN_POINT('Ctrl Pts',(10.5121893699999,11.6,1.87279091299999));
#194860=CARTESIAN_POINT('Ctrl Pts',(10.5143182119999,15.2,1.87376770899998));
#194861=CARTESIAN_POINT('Ctrl Pts',(10.5143182119999,11.6,1.87376770899998));
#194862=CARTESIAN_POINT('Ctrl Pts',(10.5164520309999,15.2,1.87474904399998));
#194863=CARTESIAN_POINT('Ctrl Pts',(10.5164520309999,11.6,1.87474904399998));
#194864=CARTESIAN_POINT('Ctrl Pts',(10.5185908099999,15.2,1.87573492299999));
#194865=CARTESIAN_POINT('Ctrl Pts',(10.5185908099999,11.6,1.87573492299998));
#194866=CARTESIAN_POINT('Ctrl Pts',(10.5207345359999,15.2,1.87672534899999));
#194867=CARTESIAN_POINT('Ctrl Pts',(10.5207345359999,11.6,1.87672534899999));
#194868=CARTESIAN_POINT('Ctrl Pts',(10.5228831919999,15.2,1.87772032599999));
#194869=CARTESIAN_POINT('Ctrl Pts',(10.5228831919999,11.6,1.87772032599998));
#194870=CARTESIAN_POINT('Ctrl Pts',(10.5250367609999,15.2,1.87871985699998));
#194871=CARTESIAN_POINT('Ctrl Pts',(10.5250367609999,11.6,1.87871985699998));
#194872=CARTESIAN_POINT('Ctrl Pts',(10.5271952289999,15.2,1.87972394599999));
#194873=CARTESIAN_POINT('Ctrl Pts',(10.5271952289999,11.6,1.87972394599999));
#194874=CARTESIAN_POINT('Ctrl Pts',(10.5293585799999,15.2,1.88073259699999));
#194875=CARTESIAN_POINT('Ctrl Pts',(10.5293585799999,11.6,1.88073259699999));
#194876=CARTESIAN_POINT('Ctrl Pts',(10.5315267989999,15.2,1.88174581299998));
#194877=CARTESIAN_POINT('Ctrl Pts',(10.5315267989999,11.6,1.88174581299998));
#194878=CARTESIAN_POINT('Ctrl Pts',(10.5336998689999,15.2,1.88276359699998));
#194879=CARTESIAN_POINT('Ctrl Pts',(10.5336998689999,11.6,1.88276359699998));
#194880=CARTESIAN_POINT('Ctrl Pts',(10.5358777749999,15.2,1.88378595299998));
#194881=CARTESIAN_POINT('Ctrl Pts',(10.5358777749999,11.6,1.88378595299998));
#194882=CARTESIAN_POINT('Ctrl Pts',(10.5380605019999,15.2,1.88481288399998));
#194883=CARTESIAN_POINT('Ctrl Pts',(10.5380605019999,11.6,1.88481288399998));
#194884=CARTESIAN_POINT('Ctrl Pts',(10.5402480349999,15.2,1.88584439399999));
#194885=CARTESIAN_POINT('Ctrl Pts',(10.5402480349999,11.6,1.88584439399999));
#194886=CARTESIAN_POINT('Ctrl Pts',(10.5424403579999,15.2,1.88688048699999));
#194887=CARTESIAN_POINT('Ctrl Pts',(10.5424403579999,11.6,1.88688048699999));
#194888=CARTESIAN_POINT('Ctrl Pts',(10.5446374549999,15.2,1.88792116499998));
#194889=CARTESIAN_POINT('Ctrl Pts',(10.5446374549999,11.6,1.88792116499998));
#194890=CARTESIAN_POINT('Ctrl Pts',(10.5468393119999,15.2,1.88896643199998));
#194891=CARTESIAN_POINT('Ctrl Pts',(10.5468393119999,11.6,1.88896643199998));
#194892=CARTESIAN_POINT('Ctrl Pts',(10.5490459129999,15.2,1.89001629099999));
#194893=CARTESIAN_POINT('Ctrl Pts',(10.5490459129999,11.6,1.89001629099998));
#194894=CARTESIAN_POINT('Ctrl Pts',(10.5512572439999,15.2,1.89107074599999));
#194895=CARTESIAN_POINT('Ctrl Pts',(10.5512572439999,11.6,1.89107074599998));
#194896=CARTESIAN_POINT('Ctrl Pts',(10.5534732879999,15.2,1.89212979899999));
#194897=CARTESIAN_POINT('Ctrl Pts',(10.5534732879999,11.6,1.89212979899999));
#194898=CARTESIAN_POINT('Ctrl Pts',(10.5556940319999,15.2,1.89319345599999));
#194899=CARTESIAN_POINT('Ctrl Pts',(10.5556940319999,11.6,1.89319345599999));
#194900=CARTESIAN_POINT('Ctrl Pts',(10.5579194589999,15.2,1.89426171699999));
#194901=CARTESIAN_POINT('Ctrl Pts',(10.5579194589999,11.6,1.89426171699999));
#194902=CARTESIAN_POINT('Ctrl Pts',(10.5601495539999,15.2,1.89533458699998));
#194903=CARTESIAN_POINT('Ctrl Pts',(10.5601495539999,11.6,1.89533458699998));
#194904=CARTESIAN_POINT('Ctrl Pts',(10.5623843029999,15.2,1.89641206899998));
#194905=CARTESIAN_POINT('Ctrl Pts',(10.5623843029999,11.6,1.89641206899998));
#194906=CARTESIAN_POINT('Ctrl Pts',(10.5646236909999,15.2,1.89749416699998));
#194907=CARTESIAN_POINT('Ctrl Pts',(10.5646236909999,11.6,1.89749416699998));
#194908=CARTESIAN_POINT('Ctrl Pts',(10.5668677029999,15.2,1.89858088199998));
#194909=CARTESIAN_POINT('Ctrl Pts',(10.5668677029999,11.6,1.89858088199998));
#194910=CARTESIAN_POINT('Ctrl Pts',(10.5691163239999,15.2,1.89967221899999));
#194911=CARTESIAN_POINT('Ctrl Pts',(10.5691163239999,11.6,1.89967221899999));
#194912=CARTESIAN_POINT('Ctrl Pts',(10.5713695389999,15.2,1.90076818199998));
#194913=CARTESIAN_POINT('Ctrl Pts',(10.5713695389999,11.6,1.90076818199998));
#194914=CARTESIAN_POINT('Ctrl Pts',(10.5736273329999,15.2,1.90186877199999));
#194915=CARTESIAN_POINT('Ctrl Pts',(10.5736273329999,11.6,1.90186877199999));
#194916=CARTESIAN_POINT('Ctrl Pts',(10.5758896919999,15.2,1.90297399199999));
#194917=CARTESIAN_POINT('Ctrl Pts',(10.5758896919999,11.6,1.90297399199999));
#194918=CARTESIAN_POINT('Ctrl Pts',(10.5781565999999,15.2,1.90408384699999));
#194919=CARTESIAN_POINT('Ctrl Pts',(10.5781565999999,11.6,1.90408384699999));
#194920=CARTESIAN_POINT('Ctrl Pts',(10.5804280449999,15.2,1.90519833799998));
#194921=CARTESIAN_POINT('Ctrl Pts',(10.5804280449999,11.6,1.90519833799998));
#194922=CARTESIAN_POINT('Ctrl Pts',(10.5827040089999,15.2,1.90631746999999));
#194923=CARTESIAN_POINT('Ctrl Pts',(10.5827040089999,11.6,1.90631746999998));
#194924=CARTESIAN_POINT('Ctrl Pts',(10.5849844789999,15.2,1.90744124499998));
#194925=CARTESIAN_POINT('Ctrl Pts',(10.5849844789999,11.6,1.90744124499998));
#194926=CARTESIAN_POINT('Ctrl Pts',(10.5872694409999,15.2,1.90856966699998));
#194927=CARTESIAN_POINT('Ctrl Pts',(10.5872694409999,11.6,1.90856966699998));
#194928=CARTESIAN_POINT('Ctrl Pts',(10.5895588789999,15.2,1.90970273699998));
#194929=CARTESIAN_POINT('Ctrl Pts',(10.5895588789999,11.6,1.90970273699998));
#194930=CARTESIAN_POINT('Ctrl Pts',(10.5918527799999,15.2,1.91084046099999));
#194931=CARTESIAN_POINT('Ctrl Pts',(10.5918527799999,11.6,1.91084046099998));
#194932=CARTESIAN_POINT('Ctrl Pts',(10.5941511279999,15.2,1.91198283799999));
#194933=CARTESIAN_POINT('Ctrl Pts',(10.5941511279999,11.6,1.91198283799999));
#194934=CARTESIAN_POINT('Ctrl Pts',(10.5964539099999,15.2,1.91312987399999));
#194935=CARTESIAN_POINT('Ctrl Pts',(10.5964539099999,11.6,1.91312987399999));
#194936=CARTESIAN_POINT('Ctrl Pts',(10.5987611109999,15.2,1.91428157099998));
#194937=CARTESIAN_POINT('Ctrl Pts',(10.5987611109999,11.6,1.91428157099998));
#194938=CARTESIAN_POINT('Ctrl Pts',(10.6010727169999,15.2,1.91543793199999));
#194939=CARTESIAN_POINT('Ctrl Pts',(10.6010727169999,11.6,1.91543793199999));
#194940=CARTESIAN_POINT('Ctrl Pts',(10.6033887129999,15.2,1.91659895999999));
#194941=CARTESIAN_POINT('Ctrl Pts',(10.6033887129999,11.6,1.91659895999999));
#194942=CARTESIAN_POINT('Ctrl Pts',(10.6057090859999,15.2,1.91776465699999));
#194943=CARTESIAN_POINT('Ctrl Pts',(10.6057090859999,11.6,1.91776465699998));
#194944=CARTESIAN_POINT('Ctrl Pts',(10.6080338189999,15.2,1.91893502699998));
#194945=CARTESIAN_POINT('Ctrl Pts',(10.6080338189999,11.6,1.91893502699998));
#194946=CARTESIAN_POINT('Ctrl Pts',(10.6103629009999,15.2,1.92011007299998));
#194947=CARTESIAN_POINT('Ctrl Pts',(10.6103629009999,11.6,1.92011007299998));
#194948=CARTESIAN_POINT('Ctrl Pts',(10.6126963159999,15.2,1.92128979699998));
#194949=CARTESIAN_POINT('Ctrl Pts',(10.6126963159999,11.6,1.92128979699998));
#194950=CARTESIAN_POINT('Ctrl Pts',(10.6150340509999,15.2,1.92247420199998));
#194951=CARTESIAN_POINT('Ctrl Pts',(10.6150340509999,11.6,1.92247420199998));
#194952=CARTESIAN_POINT('Ctrl Pts',(10.6173760899999,15.2,1.92366328999999));
#194953=CARTESIAN_POINT('Ctrl Pts',(10.6173760899999,11.6,1.92366328999999));
#194954=CARTESIAN_POINT('Ctrl Pts',(10.6197224209999,15.2,1.92485706499999));
#194955=CARTESIAN_POINT('Ctrl Pts',(10.6197224209999,11.6,1.92485706499998));
#194956=CARTESIAN_POINT('Ctrl Pts',(10.6220730289999,15.2,1.92605552899999));
#194957=CARTESIAN_POINT('Ctrl Pts',(10.6220730289999,11.6,1.92605552899999));
#194958=CARTESIAN_POINT('Ctrl Pts',(10.6244279009999,15.2,1.92725868499998));
#194959=CARTESIAN_POINT('Ctrl Pts',(10.6244279009999,11.6,1.92725868499998));
#194960=CARTESIAN_POINT('Ctrl Pts',(10.6267870199999,15.2,1.92846653699998));
#194961=CARTESIAN_POINT('Ctrl Pts',(10.6267870199999,11.6,1.92846653699998));
#194962=CARTESIAN_POINT('Ctrl Pts',(10.6291503759999,15.2,1.92967908499998));
#194963=CARTESIAN_POINT('Ctrl Pts',(10.6291503759999,11.6,1.92967908499998));
#194964=CARTESIAN_POINT('Ctrl Pts',(10.6315179529999,15.2,1.93089633399998));
#194965=CARTESIAN_POINT('Ctrl Pts',(10.6315179529999,11.6,1.93089633399998));
#194966=CARTESIAN_POINT('Ctrl Pts',(10.6338897369999,15.2,1.93211828599999));
#194967=CARTESIAN_POINT('Ctrl Pts',(10.6338897369999,11.6,1.93211828599999));
#194968=CARTESIAN_POINT('Ctrl Pts',(10.6362657159999,15.2,1.93334494299998));
#194969=CARTESIAN_POINT('Ctrl Pts',(10.6362657159999,11.6,1.93334494299998));
#194970=CARTESIAN_POINT('Ctrl Pts',(10.6386458729999,15.2,1.93457630799998));
#194971=CARTESIAN_POINT('Ctrl Pts',(10.6386458729999,11.6,1.93457630799998));
#194972=CARTESIAN_POINT('Ctrl Pts',(10.6410301979999,15.2,1.93581238299998));
#194973=CARTESIAN_POINT('Ctrl Pts',(10.6410301979999,11.6,1.93581238299998));
#194974=CARTESIAN_POINT('Ctrl Pts',(10.6434186729999,15.2,1.93705317299999));
#194975=CARTESIAN_POINT('Ctrl Pts',(10.6434186729999,11.6,1.93705317299999));
#194976=CARTESIAN_POINT('Ctrl Pts',(10.6458112889999,15.2,1.93829867799999));
#194977=CARTESIAN_POINT('Ctrl Pts',(10.6458112889999,11.6,1.93829867799999));
#194978=CARTESIAN_POINT('Ctrl Pts',(10.6482080289999,15.2,1.93954890099999));
#194979=CARTESIAN_POINT('Ctrl Pts',(10.6482080289999,11.6,1.93954890099999));
#194980=CARTESIAN_POINT('Ctrl Pts',(10.6506088799999,15.2,1.94080384499999));
#194981=CARTESIAN_POINT('Ctrl Pts',(10.6506088799999,11.6,1.94080384499998));
#194982=CARTESIAN_POINT('Ctrl Pts',(10.6530138299999,15.2,1.94206351299998));
#194983=CARTESIAN_POINT('Ctrl Pts',(10.6530138299999,11.6,1.94206351299998));
#194984=CARTESIAN_POINT('Ctrl Pts',(10.6554228629999,15.2,1.94332790599999));
#194985=CARTESIAN_POINT('Ctrl Pts',(10.6554228629999,11.6,1.94332790599998));
#194986=CARTESIAN_POINT('Ctrl Pts',(10.6578359679999,15.2,1.94459702899998));
#194987=CARTESIAN_POINT('Ctrl Pts',(10.6578359679999,11.6,1.94459702899998));
#194988=CARTESIAN_POINT('Ctrl Pts',(10.6602531299999,15.2,1.94587088299999));
#194989=CARTESIAN_POINT('Ctrl Pts',(10.6602531299999,11.6,1.94587088299999));
#194990=CARTESIAN_POINT('Ctrl Pts',(10.6626743349999,15.2,1.94714946999999));
#194991=CARTESIAN_POINT('Ctrl Pts',(10.6626743349999,11.6,1.94714946999999));
#194992=CARTESIAN_POINT('Ctrl Pts',(10.6650995699999,15.2,1.94843279199999));
#194993=CARTESIAN_POINT('Ctrl Pts',(10.6650995699999,11.6,1.94843279199999));
#194994=CARTESIAN_POINT('Ctrl Pts',(10.6675288229999,15.2,1.94972085299999));
#194995=CARTESIAN_POINT('Ctrl Pts',(10.6675288229999,11.6,1.94972085299998));
#194996=CARTESIAN_POINT('Ctrl Pts',(10.6699620789999,15.2,1.95101365499998));
#194997=CARTESIAN_POINT('Ctrl Pts',(10.6699620789999,11.6,1.95101365499998));
#194998=CARTESIAN_POINT('Ctrl Pts',(10.6723993259999,15.2,1.95231119999999));
#194999=CARTESIAN_POINT('Ctrl Pts',(10.6723993259999,11.6,1.95231119999998));
#195000=CARTESIAN_POINT('Ctrl Pts',(10.6748405499999,15.2,1.95361349199999));
#195001=CARTESIAN_POINT('Ctrl Pts',(10.6748405499999,11.6,1.95361349199999));
#195002=CARTESIAN_POINT('Ctrl Pts',(10.6772857359999,15.2,1.95492052999999));
#195003=CARTESIAN_POINT('Ctrl Pts',(10.6772857359999,11.6,1.95492052999999));
#195004=CARTESIAN_POINT('Ctrl Pts',(10.6797348739999,15.2,1.95623231899999));
#195005=CARTESIAN_POINT('Ctrl Pts',(10.6797348739999,11.6,1.95623231899999));
#195006=CARTESIAN_POINT('Ctrl Pts',(10.6821879489999,15.2,1.95754885999999));
#195007=CARTESIAN_POINT('Ctrl Pts',(10.6821879489999,11.6,1.95754885999999));
#195008=CARTESIAN_POINT('Ctrl Pts',(10.6846449469999,15.2,1.95887015699999));
#195009=CARTESIAN_POINT('Ctrl Pts',(10.6846449469999,11.6,1.95887015699999));
#195010=CARTESIAN_POINT('Ctrl Pts',(10.6871058569999,15.2,1.96019620999999));
#195011=CARTESIAN_POINT('Ctrl Pts',(10.6871058569999,11.6,1.96019620999999));
#195012=CARTESIAN_POINT('Ctrl Pts',(10.6895706639999,15.2,1.96152702399999));
#195013=CARTESIAN_POINT('Ctrl Pts',(10.6895706639999,11.6,1.96152702399999));
#195014=CARTESIAN_POINT('Ctrl Pts',(10.6920393549999,15.2,1.96286259899999));
#195015=CARTESIAN_POINT('Ctrl Pts',(10.6920393549999,11.6,1.96286259899999));
#195016=CARTESIAN_POINT('Ctrl Pts',(10.6945119189999,15.2,1.96420293799999));
#195017=CARTESIAN_POINT('Ctrl Pts',(10.6945119189999,11.6,1.96420293799999));
#195018=CARTESIAN_POINT('Ctrl Pts',(10.6969883409999,15.2,1.96554804299998));
#195019=CARTESIAN_POINT('Ctrl Pts',(10.6969883409999,11.6,1.96554804299998));
#195020=CARTESIAN_POINT('Ctrl Pts',(10.6994686089999,15.2,1.96689791799999));
#195021=CARTESIAN_POINT('Ctrl Pts',(10.6994686089999,11.6,1.96689791799999));
#195022=CARTESIAN_POINT('Ctrl Pts',(10.7019527089999,15.2,1.96825256199999));
#195023=CARTESIAN_POINT('Ctrl Pts',(10.7019527089999,11.6,1.96825256199999));
#195024=CARTESIAN_POINT('Ctrl Pts',(10.7044406279999,15.2,1.96961197999999));
#195025=CARTESIAN_POINT('Ctrl Pts',(10.7044406279999,11.6,1.96961197999999));
#195026=CARTESIAN_POINT('Ctrl Pts',(10.7069323549999,15.2,1.97097617399999));
#195027=CARTESIAN_POINT('Ctrl Pts',(10.7069323549999,11.6,1.97097617399998));
#195028=CARTESIAN_POINT('Ctrl Pts',(10.7094278759999,15.2,1.97234514399999));
#195029=CARTESIAN_POINT('Ctrl Pts',(10.7094278759999,11.6,1.97234514399998));
#195030=CARTESIAN_POINT('Ctrl Pts',(10.7119271769999,15.2,1.97371889399999));
#195031=CARTESIAN_POINT('Ctrl Pts',(10.7119271769999,11.6,1.97371889399998));
#195032=CARTESIAN_POINT('Ctrl Pts',(10.7144302479999,15.2,1.97509742499999));
#195033=CARTESIAN_POINT('Ctrl Pts',(10.7144302479999,11.6,1.97509742499998));
#195034=CARTESIAN_POINT('Ctrl Pts',(10.7169370719999,15.2,1.97648073999999));
#195035=CARTESIAN_POINT('Ctrl Pts',(10.7169370719999,11.6,1.97648073999999));
#195036=CARTESIAN_POINT('Ctrl Pts',(10.7194476399999,15.2,1.97786884199999));
#195037=CARTESIAN_POINT('Ctrl Pts',(10.7194476399999,11.6,1.97786884199999));
#195038=CARTESIAN_POINT('Ctrl Pts',(10.7219619379999,15.2,1.97926173099999));
#195039=CARTESIAN_POINT('Ctrl Pts',(10.7219619379999,11.6,1.97926173099999));
#195040=CARTESIAN_POINT('Ctrl Pts',(10.7244799519999,15.2,1.98065940999999));
#195041=CARTESIAN_POINT('Ctrl Pts',(10.7244799519999,11.6,1.98065940999998));
#195042=CARTESIAN_POINT('Ctrl Pts',(10.7270016709999,15.2,1.98206188099999));
#195043=CARTESIAN_POINT('Ctrl Pts',(10.7270016709999,11.6,1.98206188099999));
#195044=CARTESIAN_POINT('Ctrl Pts',(10.7295270829999,15.2,1.98346914599998));
#195045=CARTESIAN_POINT('Ctrl Pts',(10.7295270829999,11.6,1.98346914599998));
#195046=CARTESIAN_POINT('Ctrl Pts',(10.7320561729999,15.2,1.98488120799999));
#195047=CARTESIAN_POINT('Ctrl Pts',(10.7320561729999,11.6,1.98488120799999));
#195048=CARTESIAN_POINT('Ctrl Pts',(10.7345889299999,15.2,1.98629806799998));
#195049=CARTESIAN_POINT('Ctrl Pts',(10.7345889299999,11.6,1.98629806799998));
#195050=CARTESIAN_POINT('Ctrl Pts',(10.7371253409999,15.2,1.98771972799999));
#195051=CARTESIAN_POINT('Ctrl Pts',(10.7371253409999,11.6,1.98771972799999));
#195052=CARTESIAN_POINT('Ctrl Pts',(10.7396653929999,15.2,1.98914618999999));
#195053=CARTESIAN_POINT('Ctrl Pts',(10.7396653929999,11.6,1.98914618999999));
#195054=CARTESIAN_POINT('Ctrl Pts',(10.7422090749999,15.2,1.99057745699998));
#195055=CARTESIAN_POINT('Ctrl Pts',(10.7422090749999,11.6,1.99057745699998));
#195056=CARTESIAN_POINT('Ctrl Pts',(10.7447563729999,15.2,1.99201352999999));
#195057=CARTESIAN_POINT('Ctrl Pts',(10.7447563729999,11.6,1.99201352999998));
#195058=CARTESIAN_POINT('Ctrl Pts',(10.7473072759999,15.2,1.99345441099998));
#195059=CARTESIAN_POINT('Ctrl Pts',(10.7473072759999,11.6,1.99345441099998));
#195060=CARTESIAN_POINT('Ctrl Pts',(10.7498617699999,15.2,1.99490010199999));
#195061=CARTESIAN_POINT('Ctrl Pts',(10.7498617699999,11.6,1.99490010199999));
#195062=CARTESIAN_POINT('Ctrl Pts',(10.7524198429999,15.2,1.99635060499999));
#195063=CARTESIAN_POINT('Ctrl Pts',(10.7524198429999,11.6,1.99635060499999));
#195064=CARTESIAN_POINT('Ctrl Pts',(10.7549814829999,15.2,1.99780592199998));
#195065=CARTESIAN_POINT('Ctrl Pts',(10.7549814829999,11.6,1.99780592199998));
#195066=CARTESIAN_POINT('Ctrl Pts',(10.7575466779999,15.2,1.99926605499999));
#195067=CARTESIAN_POINT('Ctrl Pts',(10.7575466779999,11.6,1.99926605499999));
#195068=CARTESIAN_POINT('Ctrl Pts',(10.7601154139999,15.2,2.00073100599999));
#195069=CARTESIAN_POINT('Ctrl Pts',(10.7601154139999,11.6,2.00073100599999));
#195070=CARTESIAN_POINT('Ctrl Pts',(10.7626876819999,15.2,2.00220077599999));
#195071=CARTESIAN_POINT('Ctrl Pts',(10.7626876819999,11.6,2.00220077599999));
#195072=CARTESIAN_POINT('Ctrl Pts',(10.7652634659999,15.2,2.00367536799999));
#195073=CARTESIAN_POINT('Ctrl Pts',(10.7652634659999,11.6,2.00367536799999));
#195074=CARTESIAN_POINT('Ctrl Pts',(10.7678427559999,15.2,2.00515478299998));
#195075=CARTESIAN_POINT('Ctrl Pts',(10.7678427559999,11.6,2.00515478299998));
#195076=CARTESIAN_POINT('Ctrl Pts',(10.7704255389999,15.2,2.00663902299999));
#195077=CARTESIAN_POINT('Ctrl Pts',(10.7704255389999,11.6,2.00663902299999));
#195078=CARTESIAN_POINT('Ctrl Pts',(10.7730118039999,15.2,2.00812809099999));
#195079=CARTESIAN_POINT('Ctrl Pts',(10.7730118039999,11.6,2.00812809099999));
#195080=CARTESIAN_POINT('Ctrl Pts',(10.7756015359999,15.2,2.00962198699999));
#195081=CARTESIAN_POINT('Ctrl Pts',(10.7756015359999,11.6,2.00962198699999));
#195082=CARTESIAN_POINT('Ctrl Pts',(10.7781947259999,15.2,2.01112071299999));
#195083=CARTESIAN_POINT('Ctrl Pts',(10.7781947259999,11.6,2.01112071299998));
#195084=CARTESIAN_POINT('Ctrl Pts',(10.7807913609999,15.2,2.01262427099998));
#195085=CARTESIAN_POINT('Ctrl Pts',(10.7807913609999,11.6,2.01262427099998));
#195086=CARTESIAN_POINT('Ctrl Pts',(10.7833914279999,15.2,2.01413266499999));
#195087=CARTESIAN_POINT('Ctrl Pts',(10.7833914279999,11.6,2.01413266499999));
#195088=CARTESIAN_POINT('Ctrl Pts',(10.7859949149999,15.2,2.01564589299998));
#195089=CARTESIAN_POINT('Ctrl Pts',(10.7859949149999,11.6,2.01564589299998));
#195090=CARTESIAN_POINT('Ctrl Pts',(10.7886018119999,15.2,2.01716395899998));
#195091=CARTESIAN_POINT('Ctrl Pts',(10.7886018119999,11.6,2.01716395899998));
#195092=CARTESIAN_POINT('Ctrl Pts',(10.7912121039999,15.2,2.01868686499999));
#195093=CARTESIAN_POINT('Ctrl Pts',(10.7912121039999,11.6,2.01868686499999));
#195094=CARTESIAN_POINT('Ctrl Pts',(10.7938257809999,15.2,2.02021461199998));
#195095=CARTESIAN_POINT('Ctrl Pts',(10.7938257809999,11.6,2.02021461199998));
#195096=CARTESIAN_POINT('Ctrl Pts',(10.7964428309999,15.2,2.02174720099999));
#195097=CARTESIAN_POINT('Ctrl Pts',(10.7964428309999,11.6,2.02174720099999));
#195098=CARTESIAN_POINT('Ctrl Pts',(10.7990632409999,15.2,2.02328463499999));
#195099=CARTESIAN_POINT('Ctrl Pts',(10.7990632409999,11.6,2.02328463499999));
#195100=CARTESIAN_POINT('Ctrl Pts',(10.8016870009999,15.2,2.02482691399998));
#195101=CARTESIAN_POINT('Ctrl Pts',(10.8016870009999,11.6,2.02482691399998));
#195102=CARTESIAN_POINT('Ctrl Pts',(10.8043140959999,15.2,2.02637404199999));
#195103=CARTESIAN_POINT('Ctrl Pts',(10.8043140959999,11.6,2.02637404199998));
#195104=CARTESIAN_POINT('Ctrl Pts',(10.8069445179999,15.2,2.02792601899999));
#195105=CARTESIAN_POINT('Ctrl Pts',(10.8069445179999,11.6,2.02792601899999));
#195106=CARTESIAN_POINT('Ctrl Pts',(10.8095782509999,15.2,2.02948284699998));
#195107=CARTESIAN_POINT('Ctrl Pts',(10.8095782509999,11.6,2.02948284699998));
#195108=CARTESIAN_POINT('Ctrl Pts',(10.8122152859999,15.2,2.03104452799999));
#195109=CARTESIAN_POINT('Ctrl Pts',(10.8122152859999,11.6,2.03104452799999));
#195110=CARTESIAN_POINT('Ctrl Pts',(10.8148556109999,15.2,2.03261106299998));
#195111=CARTESIAN_POINT('Ctrl Pts',(10.8148556109999,11.6,2.03261106299998));
#195112=CARTESIAN_POINT('Ctrl Pts',(10.8174992139999,15.2,2.03418245299999));
#195113=CARTESIAN_POINT('Ctrl Pts',(10.8174992139999,11.6,2.03418245299999));
#195114=CARTESIAN_POINT('Ctrl Pts',(10.8201460829999,15.2,2.03575870199999));
#195115=CARTESIAN_POINT('Ctrl Pts',(10.8201460829999,11.6,2.03575870199999));
#195116=CARTESIAN_POINT('Ctrl Pts',(10.8227962069999,15.2,2.03733980899999));
#195117=CARTESIAN_POINT('Ctrl Pts',(10.8227962069999,11.6,2.03733980899999));
#195118=CARTESIAN_POINT('Ctrl Pts',(10.8254495719999,15.2,2.03892577599999));
#195119=CARTESIAN_POINT('Ctrl Pts',(10.8254495719999,11.6,2.03892577599999));
#195120=CARTESIAN_POINT('Ctrl Pts',(10.8281061699999,15.2,2.04051660499998));
#195121=CARTESIAN_POINT('Ctrl Pts',(10.8281061699999,11.6,2.04051660499998));
#195122=CARTESIAN_POINT('Ctrl Pts',(10.8307659859999,15.2,2.04211229899999));
#195123=CARTESIAN_POINT('Ctrl Pts',(10.8307659859999,11.6,2.04211229899998));
#195124=CARTESIAN_POINT('Ctrl Pts',(10.8334290109999,15.2,2.04371285799999));
#195125=CARTESIAN_POINT('Ctrl Pts',(10.8334290109999,11.6,2.04371285799999));
#195126=CARTESIAN_POINT('Ctrl Pts',(10.8360952309999,15.2,2.04531828299999));
#195127=CARTESIAN_POINT('Ctrl Pts',(10.8360952309999,11.6,2.04531828299999));
#195128=CARTESIAN_POINT('Ctrl Pts',(10.8387646369999,15.2,2.04692857699999));
#195129=CARTESIAN_POINT('Ctrl Pts',(10.8387646369999,11.6,2.04692857699999));
#195130=CARTESIAN_POINT('Ctrl Pts',(10.8414372149999,15.2,2.04854373999999));
#195131=CARTESIAN_POINT('Ctrl Pts',(10.8414372149999,11.6,2.04854373999999));
#195132=CARTESIAN_POINT('Ctrl Pts',(10.8441129549999,15.2,2.05016377399998));
#195133=CARTESIAN_POINT('Ctrl Pts',(10.8441129549999,11.6,2.05016377399998));
#195134=CARTESIAN_POINT('Ctrl Pts',(10.8467918459999,15.2,2.05178867999999));
#195135=CARTESIAN_POINT('Ctrl Pts',(10.8467918459999,11.6,2.05178867999999));
#195136=CARTESIAN_POINT('Ctrl Pts',(10.8494738749999,15.2,2.05341846099998));
#195137=CARTESIAN_POINT('Ctrl Pts',(10.8494738749999,11.6,2.05341846099998));
#195138=CARTESIAN_POINT('Ctrl Pts',(10.8521590309999,15.2,2.05505311699998));
#195139=CARTESIAN_POINT('Ctrl Pts',(10.8521590309999,11.6,2.05505311699998));
#195140=CARTESIAN_POINT('Ctrl Pts',(10.8548473029999,15.2,2.05669265099999));
#195141=CARTESIAN_POINT('Ctrl Pts',(10.8548473029999,11.6,2.05669265099999));
#195142=CARTESIAN_POINT('Ctrl Pts',(10.8575386799999,15.2,2.05833706299998));
#195143=CARTESIAN_POINT('Ctrl Pts',(10.8575386799999,11.6,2.05833706299998));
#195144=CARTESIAN_POINT('Ctrl Pts',(10.8602331499999,15.2,2.05998635399999));
#195145=CARTESIAN_POINT('Ctrl Pts',(10.8602331499999,11.6,2.05998635399998));
#195146=CARTESIAN_POINT('Ctrl Pts',(10.8629307009999,15.2,2.06164052599998));
#195147=CARTESIAN_POINT('Ctrl Pts',(10.8629307009999,11.6,2.06164052599998));
#195148=CARTESIAN_POINT('Ctrl Pts',(10.8656313229999,15.2,2.06329958099999));
#195149=CARTESIAN_POINT('Ctrl Pts',(10.8656313229999,11.6,2.06329958099999));
#195150=CARTESIAN_POINT('Ctrl Pts',(10.8683350049999,15.2,2.06496351899998));
#195151=CARTESIAN_POINT('Ctrl Pts',(10.8683350049999,11.6,2.06496351899998));
#195152=CARTESIAN_POINT('Ctrl Pts',(10.8710417329999,15.2,2.06663234299999));
#195153=CARTESIAN_POINT('Ctrl Pts',(10.8710417329999,11.6,2.06663234299999));
#195154=CARTESIAN_POINT('Ctrl Pts',(10.8737514979999,15.2,2.06830605399999));
#195155=CARTESIAN_POINT('Ctrl Pts',(10.8737514979999,11.6,2.06830605399999));
#195156=CARTESIAN_POINT('Ctrl Pts',(10.8764642889999,15.2,2.06998465199999));
#195157=CARTESIAN_POINT('Ctrl Pts',(10.8764642889999,11.6,2.06998465199998));
#195158=CARTESIAN_POINT('Ctrl Pts',(10.8791800939999,15.2,2.07166813999998));
#195159=CARTESIAN_POINT('Ctrl Pts',(10.8791800939999,11.6,2.07166813999998));
#195160=CARTESIAN_POINT('Ctrl Pts',(10.8818989019999,15.2,2.07335651799998));
#195161=CARTESIAN_POINT('Ctrl Pts',(10.8818989019999,11.6,2.07335651799998));
#195162=CARTESIAN_POINT('Ctrl Pts',(10.8846207019999,15.2,2.07504978699999));
#195163=CARTESIAN_POINT('Ctrl Pts',(10.8846207019999,11.6,2.07504978699998));
#195164=CARTESIAN_POINT('Ctrl Pts',(10.8873454819999,15.2,2.07674795099999));
#195165=CARTESIAN_POINT('Ctrl Pts',(10.8873454819999,11.6,2.07674795099999));
#195166=CARTESIAN_POINT('Ctrl Pts',(10.8900732309999,15.2,2.07845100799998));
#195167=CARTESIAN_POINT('Ctrl Pts',(10.8900732309999,11.6,2.07845100799998));
#195168=CARTESIAN_POINT('Ctrl Pts',(10.8928039389999,15.2,2.08015895999999));
#195169=CARTESIAN_POINT('Ctrl Pts',(10.8928039389999,11.6,2.08015895999999));
#195170=CARTESIAN_POINT('Ctrl Pts',(10.8955375949999,15.2,2.08187180999999));
#195171=CARTESIAN_POINT('Ctrl Pts',(10.8955375949999,11.6,2.08187180999999));
#195172=CARTESIAN_POINT('Ctrl Pts',(10.8982741869999,15.2,2.08358955799998));
#195173=CARTESIAN_POINT('Ctrl Pts',(10.8982741869999,11.6,2.08358955799998));
#195174=CARTESIAN_POINT('Ctrl Pts',(10.9010137039999,15.2,2.08531220599999));
#195175=CARTESIAN_POINT('Ctrl Pts',(10.9010137039999,11.6,2.08531220599998));
#195176=CARTESIAN_POINT('Ctrl Pts',(10.9037561339999,15.2,2.08703975299999));
#195177=CARTESIAN_POINT('Ctrl Pts',(10.9037561339999,11.6,2.08703975299999));
#195178=CARTESIAN_POINT('Ctrl Pts',(10.9065014689999,15.2,2.08877220199998));
#195179=CARTESIAN_POINT('Ctrl Pts',(10.9065014689999,11.6,2.08877220199998));
#195180=CARTESIAN_POINT('Ctrl Pts',(10.9092496959999,15.2,2.09050955499999));
#195181=CARTESIAN_POINT('Ctrl Pts',(10.9092496959999,11.6,2.09050955499999));
#195182=CARTESIAN_POINT('Ctrl Pts',(10.9120008039999,15.2,2.09225181199999));
#195183=CARTESIAN_POINT('Ctrl Pts',(10.9120008039999,11.6,2.09225181199999));
#195184=CARTESIAN_POINT('Ctrl Pts',(10.9147547819999,15.2,2.09399897299999));
#195185=CARTESIAN_POINT('Ctrl Pts',(10.9147547819999,11.6,2.09399897299999));
#195186=CARTESIAN_POINT('Ctrl Pts',(10.9175116189999,15.2,2.09575104199998));
#195187=CARTESIAN_POINT('Ctrl Pts',(10.9175116189999,11.6,2.09575104199998));
#195188=CARTESIAN_POINT('Ctrl Pts',(10.9202713059999,15.2,2.09750801799998));
#195189=CARTESIAN_POINT('Ctrl Pts',(10.9202713059999,11.6,2.09750801799998));
#195190=CARTESIAN_POINT('Ctrl Pts',(10.9230338299999,15.2,2.09926990299998));
#195191=CARTESIAN_POINT('Ctrl Pts',(10.9230338299999,11.6,2.09926990299998));
#195192=CARTESIAN_POINT('Ctrl Pts',(10.9257991809999,15.2,2.10103669699999));
#195193=CARTESIAN_POINT('Ctrl Pts',(10.9257991809999,11.6,2.10103669699999));
#195194=CARTESIAN_POINT('Ctrl Pts',(10.9285673489999,15.2,2.10280840299998));
#195195=CARTESIAN_POINT('Ctrl Pts',(10.9285673489999,11.6,2.10280840299998));
#195196=CARTESIAN_POINT('Ctrl Pts',(10.9313383209999,15.2,2.10458502099999));
#195197=CARTESIAN_POINT('Ctrl Pts',(10.9313383209999,11.6,2.10458502099998));
#195198=CARTESIAN_POINT('Ctrl Pts',(10.9341120879999,15.2,2.10636655199998));
#195199=CARTESIAN_POINT('Ctrl Pts',(10.9341120879999,11.6,2.10636655199998));
#195200=CARTESIAN_POINT('Ctrl Pts',(10.9368886379999,15.2,2.10815299699998));
#195201=CARTESIAN_POINT('Ctrl Pts',(10.9368886379999,11.6,2.10815299699998));
#195202=CARTESIAN_POINT('Ctrl Pts',(10.9396679609999,15.2,2.10994435799998));
#195203=CARTESIAN_POINT('Ctrl Pts',(10.9396679609999,11.6,2.10994435799998));
#195204=CARTESIAN_POINT('Ctrl Pts',(10.9424500479999,15.2,2.11174063499998));
#195205=CARTESIAN_POINT('Ctrl Pts',(10.9424500479999,11.6,2.11174063499998));
#195206=CARTESIAN_POINT('Ctrl Pts',(10.9452348849999,15.2,2.11354182899999));
#195207=CARTESIAN_POINT('Ctrl Pts',(10.9452348849999,11.6,2.11354182899999));
#195208=CARTESIAN_POINT('Ctrl Pts',(10.9480224639999,15.2,2.11534794299999));
#195209=CARTESIAN_POINT('Ctrl Pts',(10.9480224639999,11.6,2.11534794299999));
#195210=CARTESIAN_POINT('Ctrl Pts',(10.9508127719999,15.2,2.11715897599999));
#195211=CARTESIAN_POINT('Ctrl Pts',(10.9508127719999,11.6,2.11715897599999));
#195212=CARTESIAN_POINT('Ctrl Pts',(10.9536057999999,15.2,2.11897492899999));
#195213=CARTESIAN_POINT('Ctrl Pts',(10.9536057999999,11.6,2.11897492899999));
#195214=CARTESIAN_POINT('Ctrl Pts',(10.9564015379999,15.2,2.12079580299998));
#195215=CARTESIAN_POINT('Ctrl Pts',(10.9564015379999,11.6,2.12079580299998));
#195216=CARTESIAN_POINT('Ctrl Pts',(10.9591999729999,15.2,2.12262160099999));
#195217=CARTESIAN_POINT('Ctrl Pts',(10.9591999729999,11.6,2.12262160099998));
#195218=CARTESIAN_POINT('Ctrl Pts',(10.9620010959999,15.2,2.12445232199999));
#195219=CARTESIAN_POINT('Ctrl Pts',(10.9620010959999,11.6,2.12445232199999));
#195220=CARTESIAN_POINT('Ctrl Pts',(10.9648048959999,15.2,2.12628796699999));
#195221=CARTESIAN_POINT('Ctrl Pts',(10.9648048959999,11.6,2.12628796699999));
#195222=CARTESIAN_POINT('Ctrl Pts',(10.9676113639999,15.2,2.12812853899999));
#195223=CARTESIAN_POINT('Ctrl Pts',(10.9676113639999,11.6,2.12812853899999));
#195224=CARTESIAN_POINT('Ctrl Pts',(10.9704204879999,15.2,2.12997403599998));
#195225=CARTESIAN_POINT('Ctrl Pts',(10.9704204879999,11.6,2.12997403599998));
#195226=CARTESIAN_POINT('Ctrl Pts',(10.9732322569999,15.2,2.13182446099998));
#195227=CARTESIAN_POINT('Ctrl Pts',(10.9732322569999,11.6,2.13182446099998));
#195228=CARTESIAN_POINT('Ctrl Pts',(10.9760466609999,15.2,2.13367981399998));
#195229=CARTESIAN_POINT('Ctrl Pts',(10.9760466609999,11.6,2.13367981399998));
#195230=CARTESIAN_POINT('Ctrl Pts',(10.9788636899999,15.2,2.13554009799998));
#195231=CARTESIAN_POINT('Ctrl Pts',(10.9788636899999,11.6,2.13554009799998));
#195232=CARTESIAN_POINT('Ctrl Pts',(10.9816833339999,15.2,2.13740531099999));
#195233=CARTESIAN_POINT('Ctrl Pts',(10.9816833339999,11.6,2.13740531099999));
#195234=CARTESIAN_POINT('Ctrl Pts',(10.9845055819999,15.2,2.13927545499998));
#195235=CARTESIAN_POINT('Ctrl Pts',(10.9845055819999,11.6,2.13927545499998));
#195236=CARTESIAN_POINT('Ctrl Pts',(10.9873304239999,15.2,2.14115053199999));
#195237=CARTESIAN_POINT('Ctrl Pts',(10.9873304239999,11.6,2.14115053199999));
#195238=CARTESIAN_POINT('Ctrl Pts',(10.9901578469999,15.2,2.14303053999998));
#195239=CARTESIAN_POINT('Ctrl Pts',(10.9901578469999,11.6,2.14303053999998));
#195240=CARTESIAN_POINT('Ctrl Pts',(10.9929878449999,15.2,2.14491548299999));
#195241=CARTESIAN_POINT('Ctrl Pts',(10.9929878449999,11.6,2.14491548299998));
#195242=CARTESIAN_POINT('Ctrl Pts',(10.9958204049999,15.2,2.14680536099999));
#195243=CARTESIAN_POINT('Ctrl Pts',(10.9958204049999,11.6,2.14680536099999));
#195244=CARTESIAN_POINT('Ctrl Pts',(10.9986555149999,15.2,2.14870017399999));
#195245=CARTESIAN_POINT('Ctrl Pts',(10.9986555149999,11.6,2.14870017399999));
#195246=CARTESIAN_POINT('Ctrl Pts',(11.0014931689999,15.2,2.15059992399999));
#195247=CARTESIAN_POINT('Ctrl Pts',(11.0014931689999,11.6,2.15059992399999));
#195248=CARTESIAN_POINT('Ctrl Pts',(11.0043333539999,15.2,2.15250460999998));
#195249=CARTESIAN_POINT('Ctrl Pts',(11.0043333539999,11.6,2.15250460999998));
#195250=CARTESIAN_POINT('Ctrl Pts',(11.0071760609999,15.2,2.15441423599998));
#195251=CARTESIAN_POINT('Ctrl Pts',(11.0071760609999,11.6,2.15441423599998));
#195252=CARTESIAN_POINT('Ctrl Pts',(11.0100212779999,15.2,2.15632879999998));
#195253=CARTESIAN_POINT('Ctrl Pts',(11.0100212779999,11.6,2.15632879999998));
#195254=CARTESIAN_POINT('Ctrl Pts',(11.0128689959999,15.2,2.15824830299999));
#195255=CARTESIAN_POINT('Ctrl Pts',(11.0128689959999,11.6,2.15824830299999));
#195256=CARTESIAN_POINT('Ctrl Pts',(11.0157192049999,15.2,2.16017274699999));
#195257=CARTESIAN_POINT('Ctrl Pts',(11.0157192049999,11.6,2.16017274699999));
#195258=CARTESIAN_POINT('Ctrl Pts',(11.0185718939999,15.2,2.16210213199998));
#195259=CARTESIAN_POINT('Ctrl Pts',(11.0185718939999,11.6,2.16210213199998));
#195260=CARTESIAN_POINT('Ctrl Pts',(11.0214270539999,15.2,2.16403645899998));
#195261=CARTESIAN_POINT('Ctrl Pts',(11.0214270539999,11.6,2.16403645899998));
#195262=CARTESIAN_POINT('Ctrl Pts',(11.0242846729999,15.2,2.16597572899999));
#195263=CARTESIAN_POINT('Ctrl Pts',(11.0242846729999,11.6,2.16597572899999));
#195264=CARTESIAN_POINT('Ctrl Pts',(11.0271447429999,15.2,2.16791994299999));
#195265=CARTESIAN_POINT('Ctrl Pts',(11.0271447429999,11.6,2.16791994299998));
#195266=CARTESIAN_POINT('Ctrl Pts',(11.0300072519999,15.2,2.16986909999999));
#195267=CARTESIAN_POINT('Ctrl Pts',(11.0300072519999,11.6,2.16986909999999));
#195268=CARTESIAN_POINT('Ctrl Pts',(11.0328721909999,15.2,2.17182320299999));
#195269=CARTESIAN_POINT('Ctrl Pts',(11.0328721909999,11.6,2.17182320299999));
#195270=CARTESIAN_POINT('Ctrl Pts',(11.0357395489999,15.2,2.17378225199999));
#195271=CARTESIAN_POINT('Ctrl Pts',(11.0357395489999,11.6,2.17378225199999));
#195272=CARTESIAN_POINT('Ctrl Pts',(11.0386093189999,15.2,2.17574624799999));
#195273=CARTESIAN_POINT('Ctrl Pts',(11.0386093189999,11.6,2.17574624799999));
#195274=CARTESIAN_POINT('Ctrl Pts',(11.0414814859999,15.2,2.17771519099998));
#195275=CARTESIAN_POINT('Ctrl Pts',(11.0414814859999,11.6,2.17771519099998));
#195276=CARTESIAN_POINT('Ctrl Pts',(11.0443560429999,15.2,2.17968908099999));
#195277=CARTESIAN_POINT('Ctrl Pts',(11.0443560429999,11.6,2.17968908099999));
#195278=CARTESIAN_POINT('Ctrl Pts',(11.0472329809999,15.2,2.18166791999999));
#195279=CARTESIAN_POINT('Ctrl Pts',(11.0472329809999,11.6,2.18166791999999));
#195280=CARTESIAN_POINT('Ctrl Pts',(11.0501122879999,15.2,2.18365170899999));
#195281=CARTESIAN_POINT('Ctrl Pts',(11.0501122879999,11.6,2.18365170899998));
#195282=CARTESIAN_POINT('Ctrl Pts',(11.0529939539999,15.2,2.18564044699999));
#195283=CARTESIAN_POINT('Ctrl Pts',(11.0529939539999,11.6,2.18564044699999));
#195284=CARTESIAN_POINT('Ctrl Pts',(11.0558779689999,15.2,2.18763413699998));
#195285=CARTESIAN_POINT('Ctrl Pts',(11.0558779689999,11.6,2.18763413699998));
#195286=CARTESIAN_POINT('Ctrl Pts',(11.0587643239999,15.2,2.18963277699999));
#195287=CARTESIAN_POINT('Ctrl Pts',(11.0587643239999,11.6,2.18963277699999));
#195288=CARTESIAN_POINT('Ctrl Pts',(11.0616530089999,15.2,2.19163636999999));
#195289=CARTESIAN_POINT('Ctrl Pts',(11.0616530089999,11.6,2.19163636999998));
#195290=CARTESIAN_POINT('Ctrl Pts',(11.0645440139999,15.2,2.19364491499999));
#195291=CARTESIAN_POINT('Ctrl Pts',(11.0645440139999,11.6,2.19364491499999));
#195292=CARTESIAN_POINT('Ctrl Pts',(11.0674373299999,15.2,2.19565841299998));
#195293=CARTESIAN_POINT('Ctrl Pts',(11.0674373299999,11.6,2.19565841299998));
#195294=CARTESIAN_POINT('Ctrl Pts',(11.0703329449999,15.2,2.19767686499999));
#195295=CARTESIAN_POINT('Ctrl Pts',(11.0703329449999,11.6,2.19767686499999));
#195296=CARTESIAN_POINT('Ctrl Pts',(11.0732308509999,15.2,2.19970027199999));
#195297=CARTESIAN_POINT('Ctrl Pts',(11.0732308509999,11.6,2.19970027199999));
#195298=CARTESIAN_POINT('Ctrl Pts',(11.0761310369999,15.2,2.20172863399998));
#195299=CARTESIAN_POINT('Ctrl Pts',(11.0761310369999,11.6,2.20172863399998));
#195300=CARTESIAN_POINT('Ctrl Pts',(11.0790334939999,15.2,2.20376195199998));
#195301=CARTESIAN_POINT('Ctrl Pts',(11.0790334939999,11.6,2.20376195199998));
#195302=CARTESIAN_POINT('Ctrl Pts',(11.0819382109999,15.2,2.20580022499998));
#195303=CARTESIAN_POINT('Ctrl Pts',(11.0819382109999,11.6,2.20580022499998));
#195304=CARTESIAN_POINT('Ctrl Pts',(11.0848451789999,15.2,2.20784345599998));
#195305=CARTESIAN_POINT('Ctrl Pts',(11.0848451789999,11.6,2.20784345599998));
#195306=CARTESIAN_POINT('Ctrl Pts',(11.0877543899999,15.2,2.20989164299999));
#195307=CARTESIAN_POINT('Ctrl Pts',(11.0877543899999,11.6,2.20989164299999));
#195308=CARTESIAN_POINT('Ctrl Pts',(11.0906658309999,15.2,2.21194478999998));
#195309=CARTESIAN_POINT('Ctrl Pts',(11.0906658309999,11.6,2.21194478999998));
#195310=CARTESIAN_POINT('Ctrl Pts',(11.0935794949999,15.2,2.21400289499998));
#195311=CARTESIAN_POINT('Ctrl Pts',(11.0935794949999,11.6,2.21400289499998));
#195312=CARTESIAN_POINT('Ctrl Pts',(11.0964953709999,15.2,2.21606595799999));
#195313=CARTESIAN_POINT('Ctrl Pts',(11.0964953709999,11.6,2.21606595799999));
#195314=CARTESIAN_POINT('Ctrl Pts',(11.0994134489999,15.2,2.21813398099998));
#195315=CARTESIAN_POINT('Ctrl Pts',(11.0994134489999,11.6,2.21813398099998));
#195316=CARTESIAN_POINT('Ctrl Pts',(11.1023337189999,15.2,2.22020696299999));
#195317=CARTESIAN_POINT('Ctrl Pts',(11.1023337189999,11.6,2.22020696299999));
#195318=CARTESIAN_POINT('Ctrl Pts',(11.1052561719999,15.2,2.22228490799999));
#195319=CARTESIAN_POINT('Ctrl Pts',(11.1052561719999,11.6,2.22228490799999));
#195320=CARTESIAN_POINT('Ctrl Pts',(11.1081808009999,15.2,2.22436781199999));
#195321=CARTESIAN_POINT('Ctrl Pts',(11.1081808009999,11.6,2.22436781199999));
#195322=CARTESIAN_POINT('Ctrl Pts',(11.1111075909999,15.2,2.22645567899999));
#195323=CARTESIAN_POINT('Ctrl Pts',(11.1111075909999,11.6,2.22645567899999));
#195324=CARTESIAN_POINT('Ctrl Pts',(11.1140365369999,15.2,2.22854850799999));
#195325=CARTESIAN_POINT('Ctrl Pts',(11.1140365369999,11.6,2.22854850799999));
#195326=CARTESIAN_POINT('Ctrl Pts',(11.1169676269999,15.2,2.23064629899998));
#195327=CARTESIAN_POINT('Ctrl Pts',(11.1169676269999,11.6,2.23064629899998));
#195328=CARTESIAN_POINT('Ctrl Pts',(11.1199008519999,15.2,2.23274905299998));
#195329=CARTESIAN_POINT('Ctrl Pts',(11.1199008519999,11.6,2.23274905299998));
#195330=CARTESIAN_POINT('Ctrl Pts',(11.1228362039999,15.2,2.23485677099998));
#195331=CARTESIAN_POINT('Ctrl Pts',(11.1228362039999,11.6,2.23485677099998));
#195332=CARTESIAN_POINT('Ctrl Pts',(11.1257736699999,15.2,2.23696945299999));
#195333=CARTESIAN_POINT('Ctrl Pts',(11.1257736699999,11.6,2.23696945299999));
#195334=CARTESIAN_POINT('Ctrl Pts',(11.1287132429999,15.2,2.23908709899999));
#195335=CARTESIAN_POINT('Ctrl Pts',(11.1287132429999,11.6,2.23908709899999));
#195336=CARTESIAN_POINT('Ctrl Pts',(11.1316549139999,15.2,2.24120970899999));
#195337=CARTESIAN_POINT('Ctrl Pts',(11.1316549139999,11.6,2.24120970899999));
#195338=CARTESIAN_POINT('Ctrl Pts',(11.1345986719999,15.2,2.24333728499999));
#195339=CARTESIAN_POINT('Ctrl Pts',(11.1345986719999,11.6,2.24333728499999));
#195340=CARTESIAN_POINT('Ctrl Pts',(11.1375445069999,15.2,2.24546982699998));
#195341=CARTESIAN_POINT('Ctrl Pts',(11.1375445069999,11.6,2.24546982699998));
#195342=CARTESIAN_POINT('Ctrl Pts',(11.1404924099999,15.2,2.24760733499998));
#195343=CARTESIAN_POINT('Ctrl Pts',(11.1404924099999,11.6,2.24760733499998));
#195344=CARTESIAN_POINT('Ctrl Pts',(11.1434423739999,15.2,2.24974980999999));
#195345=CARTESIAN_POINT('Ctrl Pts',(11.1434423739999,11.6,2.24974980999999));
#195346=CARTESIAN_POINT('Ctrl Pts',(11.1463943869999,15.2,2.25189725099999));
#195347=CARTESIAN_POINT('Ctrl Pts',(11.1463943869999,11.6,2.25189725099999));
#195348=CARTESIAN_POINT('Ctrl Pts',(11.1493484399999,15.2,2.25404965899999));
#195349=CARTESIAN_POINT('Ctrl Pts',(11.1493484399999,11.6,2.25404965899999));
#195350=CARTESIAN_POINT('Ctrl Pts',(11.1523045239999,15.2,2.25620703599999));
#195351=CARTESIAN_POINT('Ctrl Pts',(11.1523045239999,11.6,2.25620703599999));
#195352=CARTESIAN_POINT('Ctrl Pts',(11.1552626289999,15.2,2.25836937999999));
#195353=CARTESIAN_POINT('Ctrl Pts',(11.1552626289999,11.6,2.25836937999999));
#195354=CARTESIAN_POINT('Ctrl Pts',(11.1582227479999,15.2,2.26053669299999));
#195355=CARTESIAN_POINT('Ctrl Pts',(11.1582227479999,11.6,2.26053669299999));
#195356=CARTESIAN_POINT('Ctrl Pts',(11.1611848689999,15.2,2.26270897399999));
#195357=CARTESIAN_POINT('Ctrl Pts',(11.1611848689999,11.6,2.26270897399999));
#195358=CARTESIAN_POINT('Ctrl Pts',(11.1641489819999,15.2,2.26488622499998));
#195359=CARTESIAN_POINT('Ctrl Pts',(11.1641489819999,11.6,2.26488622499998));
#195360=CARTESIAN_POINT('Ctrl Pts',(11.1671150809999,15.2,2.26706844399999));
#195361=CARTESIAN_POINT('Ctrl Pts',(11.1671150809999,11.6,2.26706844399999));
#195362=CARTESIAN_POINT('Ctrl Pts',(11.1700831519999,15.2,2.26925563399998));
#195363=CARTESIAN_POINT('Ctrl Pts',(11.1700831519999,11.6,2.26925563399998));
#195364=CARTESIAN_POINT('Ctrl Pts',(11.1730531909999,15.2,2.27144779399998));
#195365=CARTESIAN_POINT('Ctrl Pts',(11.1730531909999,11.6,2.27144779399998));
#195366=CARTESIAN_POINT('Ctrl Pts',(11.1760251839999,15.2,2.27364492299999));
#195367=CARTESIAN_POINT('Ctrl Pts',(11.1760251839999,11.6,2.27364492299999));
#195368=CARTESIAN_POINT('Ctrl Pts',(11.1789991259999,15.2,2.27584702399998));
#195369=CARTESIAN_POINT('Ctrl Pts',(11.1789991259999,11.6,2.27584702399998));
#195370=CARTESIAN_POINT('Ctrl Pts',(11.1819750049999,15.2,2.27805409499998));
#195371=CARTESIAN_POINT('Ctrl Pts',(11.1819750049999,11.6,2.27805409499998));
#195372=CARTESIAN_POINT('Ctrl Pts',(11.1849528119999,15.2,2.28026613799999));
#195373=CARTESIAN_POINT('Ctrl Pts',(11.1849528119999,11.6,2.28026613799999));
#195374=CARTESIAN_POINT('Ctrl Pts',(11.1879325399999,15.2,2.28248315199998));
#195375=CARTESIAN_POINT('Ctrl Pts',(11.1879325399999,11.6,2.28248315199998));
#195376=CARTESIAN_POINT('Ctrl Pts',(11.1909141789999,15.2,2.28470513899998));
#195377=CARTESIAN_POINT('Ctrl Pts',(11.1909141789999,11.6,2.28470513899998));
#195378=CARTESIAN_POINT('Ctrl Pts',(11.1938977179999,15.2,2.28693209699999));
#195379=CARTESIAN_POINT('Ctrl Pts',(11.1938977179999,11.6,2.28693209699998));
#195380=CARTESIAN_POINT('Ctrl Pts',(11.1968831489999,15.2,2.28916402699999));
#195381=CARTESIAN_POINT('Ctrl Pts',(11.1968831489999,11.6,2.28916402699999));
#195382=CARTESIAN_POINT('Ctrl Pts',(11.1998704629999,15.2,2.29140092999998));
#195383=CARTESIAN_POINT('Ctrl Pts',(11.1998704629999,11.6,2.29140092999998));
#195384=CARTESIAN_POINT('Ctrl Pts',(11.2028596489999,15.2,2.29364280599999));
#195385=CARTESIAN_POINT('Ctrl Pts',(11.2028596489999,11.6,2.29364280599999));
#195386=CARTESIAN_POINT('Ctrl Pts',(11.2058506979999,15.2,2.29588965499998));
#195387=CARTESIAN_POINT('Ctrl Pts',(11.2058506979999,11.6,2.29588965499998));
#195388=CARTESIAN_POINT('Ctrl Pts',(11.2088436019999,15.2,2.29814147699999));
#195389=CARTESIAN_POINT('Ctrl Pts',(11.2088436019999,11.6,2.29814147699999));
#195390=CARTESIAN_POINT('Ctrl Pts',(11.2118383509999,15.2,2.30039827199999));
#195391=CARTESIAN_POINT('Ctrl Pts',(11.2118383509999,11.6,2.30039827199999));
#195392=CARTESIAN_POINT('Ctrl Pts',(11.2148349389999,15.2,2.30266004199999));
#195393=CARTESIAN_POINT('Ctrl Pts',(11.2148349389999,11.6,2.30266004199999));
#195394=CARTESIAN_POINT('Ctrl Pts',(11.2178333559999,15.2,2.30492678499999));
#195395=CARTESIAN_POINT('Ctrl Pts',(11.2178333559999,11.6,2.30492678499999));
#195396=CARTESIAN_POINT('Ctrl Pts',(11.2208335929999,15.2,2.30719850199999));
#195397=CARTESIAN_POINT('Ctrl Pts',(11.2208335929999,11.6,2.30719850199998));
#195398=CARTESIAN_POINT('Ctrl Pts',(11.2238356439999,15.2,2.30947519299999));
#195399=CARTESIAN_POINT('Ctrl Pts',(11.2238356439999,11.6,2.30947519299999));
#195400=CARTESIAN_POINT('Ctrl Pts',(11.2268394979999,15.2,2.31175685899998));
#195401=CARTESIAN_POINT('Ctrl Pts',(11.2268394979999,11.6,2.31175685899998));
#195402=CARTESIAN_POINT('Ctrl Pts',(11.2298451429999,15.2,2.31404349899998));
#195403=CARTESIAN_POINT('Ctrl Pts',(11.2298451429999,11.6,2.31404349899998));
#195404=CARTESIAN_POINT('Ctrl Pts',(11.2328525719999,15.2,2.31633511299998));
#195405=CARTESIAN_POINT('Ctrl Pts',(11.2328525719999,11.6,2.31633511299998));
#195406=CARTESIAN_POINT('Ctrl Pts',(11.2358617709999,15.2,2.31863170299999));
#195407=CARTESIAN_POINT('Ctrl Pts',(11.2358617709999,11.6,2.31863170299999));
#195408=CARTESIAN_POINT('Ctrl Pts',(11.2388727289999,15.2,2.32093326799999));
#195409=CARTESIAN_POINT('Ctrl Pts',(11.2388727289999,11.6,2.32093326799998));
#195410=CARTESIAN_POINT('Ctrl Pts',(11.2418854369999,15.2,2.32323980799999));
#195411=CARTESIAN_POINT('Ctrl Pts',(11.2418854369999,11.6,2.32323980799999));
#195412=CARTESIAN_POINT('Ctrl Pts',(11.2448998869999,15.2,2.32555132399999));
#195413=CARTESIAN_POINT('Ctrl Pts',(11.2448998869999,11.6,2.32555132399999));
#195414=CARTESIAN_POINT('Ctrl Pts',(11.2479160729999,15.2,2.32786781599998));
#195415=CARTESIAN_POINT('Ctrl Pts',(11.2479160729999,11.6,2.32786781599998));
#195416=CARTESIAN_POINT('Ctrl Pts',(11.2509339899999,15.2,2.33018928199999));
#195417=CARTESIAN_POINT('Ctrl Pts',(11.2509339899999,11.6,2.33018928199999));
#195418=CARTESIAN_POINT('Ctrl Pts',(11.2539536379999,15.2,2.33251572499999));
#195419=CARTESIAN_POINT('Ctrl Pts',(11.2539536379999,11.6,2.33251572499999));
#195420=CARTESIAN_POINT('Ctrl Pts',(11.2563707379999,15.2,2.33438085799999));
#195421=CARTESIAN_POINT('Ctrl Pts',(11.2563707379999,11.6,2.33438085799999));
#195422=CARTESIAN_POINT('Ctrl Pts',(11.2581843409999,15.2,2.33578194799998));
#195423=CARTESIAN_POINT('Ctrl Pts',(11.2581843409999,11.6,2.33578194799998));
#195424=CARTESIAN_POINT('Ctrl Pts',(11.2593937549999,15.2,2.33671700299999));
#195425=CARTESIAN_POINT('Ctrl Pts',(11.2593937549999,11.6,2.33671700299999));
#195426=CARTESIAN_POINT('Ctrl Pts',(11.2599985479999,15.2,2.33718477899998));
#195427=CARTESIAN_POINT('Ctrl Pts',(11.2599985479999,11.6,2.33718477899998));
#195428=CARTESIAN_POINT('Ctrl Pts',(10.2237731089999,15.2,1.76496130799999));
#195429=CARTESIAN_POINT('Ctrl Pts',(10.2255010835344,15.2,1.76541541469069));
#195430=CARTESIAN_POINT('Ctrl Pts',(10.227282994496,15.2,1.76588926687173));
#195431=CARTESIAN_POINT('Ctrl Pts',(10.2291177138156,15.2,1.76638321167919));
#195432=CARTESIAN_POINT('Ctrl Pts',(10.2309612810791,15.2,1.76687953853818));
#195433=CARTESIAN_POINT('Ctrl Pts',(10.2328581800569,15.2,1.76739616235299));
#195434=CARTESIAN_POINT('Ctrl Pts',(10.2348073231802,15.2,1.76793345482698));
#195435=CARTESIAN_POINT('Ctrl Pts',(10.2367564661265,15.2,1.76847074725216));
#195436=CARTESIAN_POINT('Ctrl Pts',(10.2387578528578,15.2,1.76902870390431));
#195437=CARTESIAN_POINT('Ctrl Pts',(10.2408104327832,15.2,1.76960768554995));
#195438=CARTESIAN_POINT('Ctrl Pts',(10.2428630127086,15.2,1.77018666719558));
#195439=CARTESIAN_POINT('Ctrl Pts',(10.2449667829652,15.2,1.77078667349933));
#195440=CARTESIAN_POINT('Ctrl Pts',(10.2471207194916,15.2,1.77140804417322));
#195441=CARTESIAN_POINT('Ctrl Pts',(10.2492746562137,15.2,1.77202941490356));
#195442=CARTESIAN_POINT('Ctrl Pts',(10.251478760386,15.2,1.77267215322636));
#195443=CARTESIAN_POINT('Ctrl Pts',(10.2537320330121,15.2,1.77333658784738));
#195444=CARTESIAN_POINT('Ctrl Pts',(10.256360850769,15.2,1.77411176148137));
#195445=CARTESIAN_POINT('Ctrl Pts',(10.2590565910528,15.2,1.77491646793701));
#195446=CARTESIAN_POINT('Ctrl Pts',(10.261817718071,15.2,1.77575121364745));
#195447=CARTESIAN_POINT('Ctrl Pts',(10.2641843986488,15.2,1.77646671005425));
#195448=CARTESIAN_POINT('Ctrl Pts',(10.2665991148725,15.2,1.77720427386484));
#195449=CARTESIAN_POINT('Ctrl Pts',(10.2690609287599,15.2,1.77796421232445));
#195450=CARTESIAN_POINT('Ctrl Pts',(10.2715227424237,15.2,1.77872415071503));
#195451=CARTESIAN_POINT('Ctrl Pts',(10.2740316523571,15.2,1.77950646297585));
#195452=CARTESIAN_POINT('Ctrl Pts',(10.276586740026,15.2,1.78031144528365));
#195453=CARTESIAN_POINT('Ctrl Pts',(10.2791418276949,15.2,1.78111642759145));
#195454=CARTESIAN_POINT('Ctrl Pts',(10.281743092104,15.2,1.78194408006059));
#195455=CARTESIAN_POINT('Ctrl Pts',(10.2843896398392,15.2,1.78279468544535));
#195456=CARTESIAN_POINT('Ctrl Pts',(10.2870361878147,15.2,1.78364529090738));
#195457=CARTESIAN_POINT('Ctrl Pts',(10.2897280175293,15.2,1.78451885269724));
#195458=CARTESIAN_POINT('Ctrl Pts',(10.2924642530148,15.2,1.78541564208104));
#195459=CARTESIAN_POINT('Ctrl Pts',(10.2952004882518,15.2,1.78631243138337));
#195460=CARTESIAN_POINT('Ctrl Pts',(10.2979811341463,15.2,1.78723245159305));
#195461=CARTESIAN_POINT('Ctrl Pts',(10.300805332129,15.2,1.7881759658098));
#195462=CARTESIAN_POINT('Ctrl Pts',(10.3036295301116,15.2,1.78911948002654));
#195463=CARTESIAN_POINT('Ctrl Pts',(10.3064972817074,15.2,1.79008648852474));
#195464=CARTESIAN_POINT('Ctrl Pts',(10.3094077538498,15.2,1.79107724790438));
#195465=CARTESIAN_POINT('Ctrl Pts',(10.3123182259922,15.2,1.79206800728402));
#195466=CARTESIAN_POINT('Ctrl Pts',(10.3152714181101,15.2,1.79308251966779));
#195467=CARTESIAN_POINT('Ctrl Pts',(10.3182665162484,15.2,1.79412102887842));
#195468=CARTESIAN_POINT('Ctrl Pts',(10.3212616146588,15.2,1.79515953818338));
#195469=CARTESIAN_POINT('Ctrl Pts',(10.3242986165983,15.2,1.79622204662399));
#195470=CARTESIAN_POINT('Ctrl Pts',(10.3273767299345,15.2,1.79730879360094));
#195471=CARTESIAN_POINT('Ctrl Pts',(10.3304548429911,15.2,1.79839554047917));
#195472=CARTESIAN_POINT('Ctrl Pts',(10.3335740630194,15.2,1.79950652453049));
#195473=CARTESIAN_POINT('Ctrl Pts',(10.3367336133195,15.2,1.80064197665483));
#195474=CARTESIAN_POINT('Ctrl Pts',(10.3398931636196,15.2,1.80177742877918));
#195475=CARTESIAN_POINT('Ctrl Pts',(10.3430930440172,15.2,1.80293735075722));
#195476=CARTESIAN_POINT('Ctrl Pts',(10.3463324913968,15.2,1.80412196462916));
#195477=CARTESIAN_POINT('Ctrl Pts',(10.3495719390707,15.2,1.8053065786087));
#195478=CARTESIAN_POINT('Ctrl Pts',(10.3528509547067,15.2,1.8065158840573));
#195479=CARTESIAN_POINT('Ctrl Pts',(10.3561687904725,15.2,1.80775009704231));
#195480=CARTESIAN_POINT('Ctrl Pts',(10.359486625937,15.2,1.80898430991522));
#195481=CARTESIAN_POINT('Ctrl Pts',(10.3628432832897,15.2,1.81024343075692));
#195482=CARTESIAN_POINT('Ctrl Pts',(10.366238030015,15.2,1.81152766671603));
#195483=CARTESIAN_POINT('Ctrl Pts',(10.3696327767403,15.2,1.81281190267514));
#195484=CARTESIAN_POINT('Ctrl Pts',(10.3730656142586,15.2,1.81412125483802));
#195485=CARTESIAN_POINT('Ctrl Pts',(10.37653582588,15.2,1.81545592462113));
#195486=CARTESIAN_POINT('Ctrl Pts',(10.3800060378165,15.2,1.81679059452548));
#195487=CARTESIAN_POINT('Ctrl Pts',(10.3835136246788,15.2,1.81815058024617));
#195488=CARTESIAN_POINT('Ctrl Pts',(10.3870578838012,15.2,1.81953607914237));
#195489=CARTESIAN_POINT('Ctrl Pts',(10.3906021426016,15.2,1.82092157791272));
#195490=CARTESIAN_POINT('Ctrl Pts',(10.3941830753479,15.2,1.8223325864188));
#195491=CARTESIAN_POINT('Ctrl Pts',(10.3977999920499,15.2,1.82376929619994));
#195492=CARTESIAN_POINT('Ctrl Pts',(10.4014169087518,15.2,1.82520600598107));
#195493=CARTESIAN_POINT('Ctrl Pts',(10.4050698101533,15.2,1.82666841365391));
#195494=CARTESIAN_POINT('Ctrl Pts',(10.4087580231182,15.2,1.82815670433936));
#195495=CARTESIAN_POINT('Ctrl Pts',(10.4124462364181,15.2,1.82964499516));
#195496=CARTESIAN_POINT('Ctrl Pts',(10.416169759044,15.2,1.83115916493211));
#195497=CARTESIAN_POINT('Ctrl Pts',(10.4199279311679,15.2,1.8326993936845));
#195498=CARTESIAN_POINT('Ctrl Pts',(10.4230597411004,15.2,1.83398291757487));
#195499=CARTESIAN_POINT('Ctrl Pts',(10.4262156133916,15.2,1.83528453345442));
#195500=CARTESIAN_POINT('Ctrl Pts',(10.4293951716574,15.2,1.83660434491424));
#195501=CARTESIAN_POINT('Ctrl Pts',(10.4325747295767,15.2,1.8379241562302));
#195502=CARTESIAN_POINT('Ctrl Pts',(10.4357779722426,15.2,1.83926216116631));
#195503=CARTESIAN_POINT('Ctrl Pts',(10.4390045303612,15.2,1.84061845407254));
#195504=CARTESIAN_POINT('Ctrl Pts',(10.4422310888315,15.2,1.8419747471266));
#195505=CARTESIAN_POINT('Ctrl Pts',(10.4454809623459,15.2,1.8433493293748));
#195506=CARTESIAN_POINT('Ctrl Pts',(10.4487537865801,15.2,1.84474229256775));
#195507=CARTESIAN_POINT('Ctrl Pts',(10.4520266108144,15.2,1.84613525576069));
#195508=CARTESIAN_POINT('Ctrl Pts',(10.4553223845839,15.2,1.8475466014861));
#195509=CARTESIAN_POINT('Ctrl Pts',(10.4586407491231,15.2,1.84897641808402));
#195510=CARTESIAN_POINT('Ctrl Pts',(10.4619591136623,15.2,1.85040623468195));
#195511=CARTESIAN_POINT('Ctrl Pts',(10.4653000711479,15.2,1.8518545245162));
#195512=CARTESIAN_POINT('Ctrl Pts',(10.4686632630217,15.2,1.85332137340412));
#195513=CARTESIAN_POINT('Ctrl Pts',(10.4720264548956,15.2,1.85478822229204));
#195514=CARTESIAN_POINT('Ctrl Pts',(10.4754118847616,15.2,1.85627363004155));
#195515=CARTESIAN_POINT('Ctrl Pts',(10.4788192008022,15.2,1.85777768386002));
#195516=CARTESIAN_POINT('Ctrl Pts',(10.4835894433332,15.2,1.85988335923867));
#195517=CARTESIAN_POINT('Ctrl Pts',(10.4884025857108,15.2,1.86202557789432));
#195518=CARTESIAN_POINT('Ctrl Pts',(10.4932576867185,15.2,1.86420456661017));
#195519=CARTESIAN_POINT('Ctrl Pts',(10.4974192016519,15.2,1.86607227112682));
#195520=CARTESIAN_POINT('Ctrl Pts',(10.5016115419829,15.2,1.86796699033299));
#195521=CARTESIAN_POINT('Ctrl Pts',(10.5058341272449,15.2,1.86988886092864));
#195522=CARTESIAN_POINT('Ctrl Pts',(10.5093529484243,15.2,1.87149041981655));
#195523=CARTESIAN_POINT('Ctrl Pts',(10.5128927747652,15.2,1.87311083441943));
#195524=CARTESIAN_POINT('Ctrl Pts',(10.5164532710313,15.2,1.87475017998238));
#195525=CARTESIAN_POINT('Ctrl Pts',(10.5207258663954,15.2,1.87671739458644));
#195526=CARTESIAN_POINT('Ctrl Pts',(10.5250282293371,15.2,1.87871187060489));
#195527=CARTESIAN_POINT('Ctrl Pts',(10.5293597965111,15.2,1.88073373802956));
#195528=CARTESIAN_POINT('Ctrl Pts',(10.5329694359539,15.2,1.88241862761134));
#195529=CARTESIAN_POINT('Ctrl Pts',(10.5365993542464,15.2,1.88412253659281));
#195530=CARTESIAN_POINT('Ctrl Pts',(10.5402492320225,15.2,1.88584553950791));
#195531=CARTESIAN_POINT('Ctrl Pts',(10.5438991097986,15.2,1.887568542423));
#195532=CARTESIAN_POINT('Ctrl Pts',(10.5475689445887,15.2,1.88931063802));
#195533=CARTESIAN_POINT('Ctrl Pts',(10.551258421855,15.2,1.89107189532888));
#195534=CARTESIAN_POINT('Ctrl Pts',(10.5549478991213,15.2,1.89283315263777));
#195535=CARTESIAN_POINT('Ctrl Pts',(10.5586570170905,15.2,1.89461357251113));
#195536=CARTESIAN_POINT('Ctrl Pts',(10.5623854625062,15.2,1.89641322285736));
#195537=CARTESIAN_POINT('Ctrl Pts',(10.5661139079218,15.2,1.89821287320358));
#195538=CARTESIAN_POINT('Ctrl Pts',(10.5698616819046,15.2,1.90003175384195));
#195539=CARTESIAN_POINT('Ctrl Pts',(10.573628473987,15.2,1.9018699293965));
#195540=CARTESIAN_POINT('Ctrl Pts',(10.5766419078171,15.2,1.90334046992029));
#195541=CARTESIAN_POINT('Ctrl Pts',(10.5796675144474,15.2,1.90482335915971));
#195542=CARTESIAN_POINT('Ctrl Pts',(10.5827051359324,15.2,1.90631863098364));
#195543=CARTESIAN_POINT('Ctrl Pts',(10.5865021625817,15.2,1.9081877206617));
#195544=CARTESIAN_POINT('Ctrl Pts',(10.5903179639277,15.2,1.91007615824236));
#195545=CARTESIAN_POINT('Ctrl Pts',(10.5941522369848,15.2,1.91198400296616));
#195546=CARTESIAN_POINT('Ctrl Pts',(10.5972196551796,15.2,1.91351027862042));
#195547=CARTESIAN_POINT('Ctrl Pts',(10.6002988962174,15.2,1.9150489769342));
#195548=CARTESIAN_POINT('Ctrl Pts',(10.603389806964,15.2,1.91660012713992));
#195549=CARTESIAN_POINT('Ctrl Pts',(10.6064807181317,15.2,1.91815127755698));
#195550=CARTESIAN_POINT('Ctrl Pts',(10.6095832977116,15.2,1.91971488102687));
#195551=CARTESIAN_POINT('Ctrl Pts',(10.6126973964268,15.2,1.92129096747037));
#195552=CARTESIAN_POINT('Ctrl Pts',(10.6158114947177,15.2,1.92286705369913));
#195553=CARTESIAN_POINT('Ctrl Pts',(10.6189371099674,15.2,1.92445562162032));
#195554=CARTESIAN_POINT('Ctrl Pts',(10.6220740947102,15.2,1.9260567018775));
#195555=CARTESIAN_POINT('Ctrl Pts',(10.6267795724656,15.2,1.9284583225905));
#195556=CARTESIAN_POINT('Ctrl Pts',(10.6315106270658,15.2,1.93088809770698));
#195557=CARTESIAN_POINT('Ctrl Pts',(10.6362667610767,15.2,1.93334612025953));
#195558=CARTESIAN_POINT('Ctrl Pts',(10.6402302054377,15.2,1.93539447205175));
#195559=CARTESIAN_POINT('Ctrl Pts',(10.6442110659086,15.2,1.9374624416227));
#195560=CARTESIAN_POINT('Ctrl Pts',(10.6482090562353,15.2,1.93955008097688));
#195561=CARTESIAN_POINT('Ctrl Pts',(10.6514074490196,15.2,1.94122019273328));
#195562=CARTESIAN_POINT('Ctrl Pts',(10.6546168056938,15.2,1.9429028934992));
#195563=CARTESIAN_POINT('Ctrl Pts',(10.6578369822582,15.2,1.94459821175827));
#195564=CARTESIAN_POINT('Ctrl Pts',(10.6610571588226,15.2,1.94629353001733));
#195565=CARTESIAN_POINT('Ctrl Pts',(10.6642881529605,15.2,1.94800146288064));
#195566=CARTESIAN_POINT('Ctrl Pts',(10.6675298243049,15.2,1.94972203853126));
#195567=CARTESIAN_POINT('Ctrl Pts',(10.6715819128229,15.2,1.95187275774288));
#195568=CARTESIAN_POINT('Ctrl Pts',(10.6756506826844,15.2,1.9540432316316));
#195569=CARTESIAN_POINT('Ctrl Pts',(10.6797358577239,15.2,1.95623350673846));
#195570=CARTESIAN_POINT('Ctrl Pts',(10.6830039982898,15.2,1.95798572711043));
#195571=CARTESIAN_POINT('Ctrl Pts',(10.686282637504,15.2,1.95975062134473));
#195572=CARTESIAN_POINT('Ctrl Pts',(10.6895716350166,15.2,1.96152821427493));
#195573=CARTESIAN_POINT('Ctrl Pts',(10.6928606325291,15.2,1.96330580720514));
#195574=CARTESIAN_POINT('Ctrl Pts',(10.6961599902013,15.2,1.96509609760628));
#195575=CARTESIAN_POINT('Ctrl Pts',(10.6994695675494,15.2,1.96689911059474));
#195576=CARTESIAN_POINT('Ctrl Pts',(10.7036065385581,15.2,1.96915287646182));
#195577=CARTESIAN_POINT('Ctrl Pts',(10.7077594778936,15.2,1.97142652144045));
#195578=CARTESIAN_POINT('Ctrl Pts',(10.7119281188963,15.2,1.97372008896661));
#195579=CARTESIAN_POINT('Ctrl Pts',(10.7152630322437,15.2,1.97555494328754));
#195580=CARTESIAN_POINT('Ctrl Pts',(10.7186079935643,15.2,1.97740254944576));
#195581=CARTESIAN_POINT('Ctrl Pts',(10.7219628670249,15.2,1.9792629284916));
#195582=CARTESIAN_POINT('Ctrl Pts',(10.7253177404855,15.2,1.98112330753744));
#195583=CARTESIAN_POINT('Ctrl Pts',(10.7286825267667,15.2,1.98299645954587));
#195584=CARTESIAN_POINT('Ctrl Pts',(10.732057090285,15.2,1.98488240781663));
#195585=CARTESIAN_POINT('Ctrl Pts',(10.7362752939931,15.2,1.98723984276964));
#195586=CARTESIAN_POINT('Ctrl Pts',(10.7405087750363,15.2,1.98961727000487));
#195587=CARTESIAN_POINT('Ctrl Pts',(10.7447572736692,15.2,1.99201473168635));
#195588=CARTESIAN_POINT('Ctrl Pts',(10.7481560731312,15.2,1.99393270134512));
#195589=CARTESIAN_POINT('Ctrl Pts',(10.7515644829914,15.2,1.99586349233844));
#195590=CARTESIAN_POINT('Ctrl Pts',(10.7549823717332,15.2,1.99780712599993));
#195591=CARTESIAN_POINT('Ctrl Pts',(10.7584002604751,15.2,1.99975075966142));
#195592=CARTESIAN_POINT('Ctrl Pts',(10.7618276281264,15.2,2.00170723580496));
#195593=CARTESIAN_POINT('Ctrl Pts',(10.7652643430368,15.2,2.00367657408026));
#195594=CARTESIAN_POINT('Ctrl Pts',(10.768701057479,15.2,2.00564591208724));
#195595=CARTESIAN_POINT('Ctrl Pts',(10.7721471206199,15.2,2.0076281130971));
#195596=CARTESIAN_POINT('Ctrl Pts',(10.7756024004642,15.2,2.00962319449858));
#195597=CARTESIAN_POINT('Ctrl Pts',(10.7790576807793,15.2,2.01161827617189));
#195598=CARTESIAN_POINT('Ctrl Pts',(10.7825221798915,15.2,2.01362623970223));
#195599=CARTESIAN_POINT('Ctrl Pts',(10.7859957680262,15.2,2.01564710281369));
#195600=CARTESIAN_POINT('Ctrl Pts',(10.7903377529579,15.2,2.01817318156534));
#195601=CARTESIAN_POINT('Ctrl Pts',(10.7946939390982,15.2,2.02071941883954));
#195602=CARTESIAN_POINT('Ctrl Pts',(10.7990640790299,15.2,2.02328584661897));
#195603=CARTESIAN_POINT('Ctrl Pts',(10.8043082467573,15.2,2.02636555984238));
#195604=CARTESIAN_POINT('Ctrl Pts',(10.8095725046703,15.2,2.02947435145939));
#195605=CARTESIAN_POINT('Ctrl Pts',(10.8148564305023,15.2,2.03261227677636));
#195606=CARTESIAN_POINT('Ctrl Pts',(10.8183790475637,15.2,2.03470422689267));
#195607=CARTESIAN_POINT('Ctrl Pts',(10.8219104058475,15.2,2.03680912705869));
#195608=CARTESIAN_POINT('Ctrl Pts',(10.8254503796128,15.2,2.03892699116201));
#195609=CARTESIAN_POINT('Ctrl Pts',(10.8289903538604,15.2,2.04104485555388));
#195610=CARTESIAN_POINT('Ctrl Pts',(10.8325389445422,15.2,2.04317568727476));
#195611=CARTESIAN_POINT('Ctrl Pts',(10.8360960274582,15.2,2.04531950022493));
#195612=CARTESIAN_POINT('Ctrl Pts',(10.8396531103743,15.2,2.0474633131751));
#195613=CARTESIAN_POINT('Ctrl Pts',(10.843218685572,15.2,2.04962010746013));
#195614=CARTESIAN_POINT('Ctrl Pts',(10.8467926311009,15.2,2.0517898990797));
#195615=CARTESIAN_POINT('Ctrl Pts',(10.8512600622817,15.2,2.05450213816072));
#195616=CARTESIAN_POINT('Ctrl Pts',(10.8557405708641,15.2,2.05723468808047));
#195617=CARTESIAN_POINT('Ctrl Pts',(10.8602339196788,15.2,2.05998757388986));
#195618=CARTESIAN_POINT('Ctrl Pts',(10.8638285993184,15.2,2.06218988289744));
#195619=CARTESIAN_POINT('Ctrl Pts',(10.8674314978142,15.2,2.06440520789794));
#195620=CARTESIAN_POINT('Ctrl Pts',(10.8710424922332,15.2,2.0666335647416));
#195621=CARTESIAN_POINT('Ctrl Pts',(10.8746534866523,15.2,2.06886192158526));
#195622=CARTESIAN_POINT('Ctrl Pts',(10.8782725796639,15.2,2.07110330940823));
#195623=CARTESIAN_POINT('Ctrl Pts',(10.8818996505846,15.2,2.07335774114354));
#195624=CARTESIAN_POINT('Ctrl Pts',(10.8873402564715,15.2,2.07673938843934));
#195625=CARTESIAN_POINT('Ctrl Pts',(10.8927988116549,15.2,2.08015038720294));
#195626=CARTESIAN_POINT('Ctrl Pts',(10.8982749185401,15.2,2.08359078316256));
#195627=CARTESIAN_POINT('Ctrl Pts',(10.9019256562977,15.2,2.0858843803648));
#195628=CARTESIAN_POINT('Ctrl Pts',(10.9055841938399,15.2,2.08819104081164));
#195629=CARTESIAN_POINT('Ctrl Pts',(10.9092504156505,15.2,2.09051078062066));
#195630=CARTESIAN_POINT('Ctrl Pts',(10.9147497491157,15.2,2.0939903908083));
#195631=CARTESIAN_POINT('Ctrl Pts',(10.9202663680979,15.2,2.09749942469599));
#195632=CARTESIAN_POINT('Ctrl Pts',(10.9257998857603,15.2,2.10103792531731));
#195633=CARTESIAN_POINT('Ctrl Pts',(10.9294888970325,15.2,2.10339692541012));
#195634=CARTESIAN_POINT('Ctrl Pts',(10.933185416981,15.2,2.10576902187315));
#195635=CARTESIAN_POINT('Ctrl Pts',(10.9368893309555,15.2,2.1081542257884));
#195636=CARTESIAN_POINT('Ctrl Pts',(10.9405932454347,15.2,2.11053943002863));
#195637=CARTESIAN_POINT('Ctrl Pts',(10.9443045562731,15.2,2.11293774149825));
#195638=CARTESIAN_POINT('Ctrl Pts',(10.9480231465873,15.2,2.11534917296386));
#195639=CARTESIAN_POINT('Ctrl Pts',(10.9526713842268,15.2,2.11836346213159));
#195640=CARTESIAN_POINT('Ctrl Pts',(10.9573309977969,15.2,2.12139824793951));
#195641=CARTESIAN_POINT('Ctrl Pts',(10.9620017658088,15.2,2.12445355337135));
#195642=CARTESIAN_POINT('Ctrl Pts',(10.9666725338207,15.2,2.12750885880319));
#195643=CARTESIAN_POINT('Ctrl Pts',(10.9713544584184,15.2,2.13058468287549));
#195644=CARTESIAN_POINT('Ctrl Pts',(10.9760473178638,15.2,2.13368104711328));
#195645=CARTESIAN_POINT('Ctrl Pts',(10.9798016051131,15.2,2.13615813830101));
#195646=CARTESIAN_POINT('Ctrl Pts',(10.9835628936977,15.2,2.13864837468981));
#195647=CARTESIAN_POINT('Ctrl Pts',(10.9873310690003,15.2,2.14115176459541));
#195648=CARTESIAN_POINT('Ctrl Pts',(10.9901572006056,15.2,2.14302930710988));
#195649=CARTESIAN_POINT('Ctrl Pts',(10.9929872077135,15.2,2.14491424879229));
#195650=CARTESIAN_POINT('Ctrl Pts',(10.9958210420017,15.2,2.14680659440055));
#195651=CARTESIAN_POINT('Ctrl Pts',(10.9986548762898,15.2,2.14869894000881));
#195652=CARTESIAN_POINT('Ctrl Pts',(11.0014925388342,15.2,2.15059868852115));
#195653=CARTESIAN_POINT('Ctrl Pts',(11.0043339838555,15.2,2.15250584453418));
#195654=CARTESIAN_POINT('Ctrl Pts',(11.0071754293929,15.2,2.15441300089368));
#195655=CARTESIAN_POINT('Ctrl Pts',(11.0100206563231,15.2,2.1563275647886));
#195656=CARTESIAN_POINT('Ctrl Pts',(11.0128696193627,15.2,2.15824953865226));
#195657=CARTESIAN_POINT('Ctrl Pts',(11.0166682358861,15.2,2.16081216988856));
#195658=CARTESIAN_POINT('Ctrl Pts',(11.0204734941615,15.2,2.16338797565092));
#195659=CARTESIAN_POINT('Ctrl Pts',(11.024285285405,15.2,2.16597696477174));
#195660=CARTESIAN_POINT('Ctrl Pts',(11.0271441289675,15.2,2.16791870670055));
#195661=CARTESIAN_POINT('Ctrl Pts',(11.0300066474401,15.2,2.16986786306232));
#195662=CARTESIAN_POINT('Ctrl Pts',(11.0328727952288,15.2,2.17182443912979));
#195663=CARTESIAN_POINT('Ctrl Pts',(11.0357389430174,15.2,2.17378101519726));
#195664=CARTESIAN_POINT('Ctrl Pts',(11.0386087216284,15.2,2.17574501082614));
#195665=CARTESIAN_POINT('Ctrl Pts',(11.0414820828569,15.2,2.17771642733684));
#195666=CARTESIAN_POINT('Ctrl Pts',(11.0453132315094,15.2,2.18034498292319));
#195667=CARTESIAN_POINT('Ctrl Pts',(11.049150754771,15.2,2.18298673275803));
#195668=CARTESIAN_POINT('Ctrl Pts',(11.0529945412583,15.2,2.18564168495826));
#195669=CARTESIAN_POINT('Ctrl Pts',(11.0558773808618,15.2,2.18763289892758));
#195670=CARTESIAN_POINT('Ctrl Pts',(11.0587637445903,15.2,2.1896315388716));
#195671=CARTESIAN_POINT('Ctrl Pts',(11.0616535886933,15.2,2.19163760779806));
#195672=CARTESIAN_POINT('Ctrl Pts',(11.0645434327964,15.2,2.19364367672452));
#195673=CARTESIAN_POINT('Ctrl Pts',(11.0674367574171,15.2,2.19565717378234));
#195674=CARTESIAN_POINT('Ctrl Pts',(11.0703335171645,15.2,2.19767810335068));
#195675=CARTESIAN_POINT('Ctrl Pts',(11.0732302769119,15.2,2.19969903291901));
#195676=CARTESIAN_POINT('Ctrl Pts',(11.0761304723229,15.2,2.20172739483113));
#195677=CARTESIAN_POINT('Ctrl Pts',(11.0790340583836,15.2,2.20376319033947));
#195678=CARTESIAN_POINT('Ctrl Pts',(11.0819376449718,15.2,2.20579898621764));
#195679=CARTESIAN_POINT('Ctrl Pts',(11.0848446225943,15.2,2.20784221601461));
#195680=CARTESIAN_POINT('Ctrl Pts',(11.0877549481844,15.2,2.20989288339699));
#195681=CARTESIAN_POINT('Ctrl Pts',(11.0926054901296,15.2,2.2133106618709));
#195682=CARTESIAN_POINT('Ctrl Pts',(11.0974653306805,15.2,2.21674909830068));
#195683=CARTESIAN_POINT('Ctrl Pts',(11.1023342654034,15.2,2.22020820413573));
#195684=CARTESIAN_POINT('Ctrl Pts',(11.1052556261311,15.2,2.22228366756135));
#195685=CARTESIAN_POINT('Ctrl Pts',(11.1081802630752,15.2,2.22436657185321));
#195686=CARTESIAN_POINT('Ctrl Pts',(11.1111081302608,15.2,2.22645691973624));
#195687=CARTESIAN_POINT('Ctrl Pts',(11.1140359974464,15.2,2.22854726761927));
#195688=CARTESIAN_POINT('Ctrl Pts',(11.1169670961792,15.2,2.23064505801875));
#195689=CARTESIAN_POINT('Ctrl Pts',(11.1199013837109,15.2,2.23275029399352));
#195690=CARTESIAN_POINT('Ctrl Pts',(11.1228356712426,15.2,2.23485552996828));
#195691=CARTESIAN_POINT('Ctrl Pts',(11.1257731464074,15.2,2.23696821199878));
#195692=CARTESIAN_POINT('Ctrl Pts',(11.1287137674806,15.2,2.23908834001468));
#195693=CARTESIAN_POINT('Ctrl Pts',(11.1316543885538,15.2,2.24120846803057));
#195694=CARTESIAN_POINT('Ctrl Pts',(11.1345981554694,15.2,2.24333604331223));
#195695=CARTESIAN_POINT('Ctrl Pts',(11.1375450236954,15.2,2.24547106827567));
#195696=CARTESIAN_POINT('Ctrl Pts',(11.1404918919214,15.2,2.24760609323912));
#195697=CARTESIAN_POINT('Ctrl Pts',(11.1434418642139,15.2,2.24974856774373));
#195698=CARTESIAN_POINT('Ctrl Pts',(11.1463948963562,15.2,2.25189849228959));
#195699=CARTESIAN_POINT('Ctrl Pts',(11.1503322729035,15.2,2.25476505861112));
#195700=CARTESIAN_POINT('Ctrl Pts',(11.1542750895084,15.2,2.25764487213383));
#195701=CARTESIAN_POINT('Ctrl Pts',(11.1582232485193,15.2,2.26053793502691));
#195702=CARTESIAN_POINT('Ctrl Pts',(11.1611843675085,15.2,2.26270773199963));
#195703=CARTESIAN_POINT('Ctrl Pts',(11.1641484899249,15.2,2.26488498220077));
#195704=CARTESIAN_POINT('Ctrl Pts',(11.1671155740806,15.2,2.26706968671462));
#195705=CARTESIAN_POINT('Ctrl Pts',(11.1700826582362,15.2,2.26925439122848));
#195706=CARTESIAN_POINT('Ctrl Pts',(11.1730527041842,15.2,2.27144655075754));
#195707=CARTESIAN_POINT('Ctrl Pts',(11.1760256708676,15.2,2.27364616571863));
#195708=CARTESIAN_POINT('Ctrl Pts',(11.178998637551,15.2,2.27584578067973));
#195709=CARTESIAN_POINT('Ctrl Pts',(11.1819745248925,15.2,2.278052851832));
#195710=CARTESIAN_POINT('Ctrl Pts',(11.1849532915756,15.2,2.28026738029217));
#195711=CARTESIAN_POINT('Ctrl Pts',(11.188924980847,15.2,2.28322008517394));
#195712=CARTESIAN_POINT('Ctrl Pts',(11.192901790612,15.2,2.28618604801213));
#195713=CARTESIAN_POINT('Ctrl Pts',(11.196883619736,15.2,2.28916527024364));
#195714=CARTESIAN_POINT('Ctrl Pts',(11.1998699913077,15.2,2.29139968671431));
#195715=CARTESIAN_POINT('Ctrl Pts',(11.2028591860757,15.2,2.29364156281944));
#195716=CARTESIAN_POINT('Ctrl Pts',(11.2058511617305,15.2,2.29589089824789));
#195717=CARTESIAN_POINT('Ctrl Pts',(11.2088431373854,15.2,2.29814023367635));
#195718=CARTESIAN_POINT('Ctrl Pts',(11.2118378943324,15.2,2.30039702865285));
#195719=CARTESIAN_POINT('Ctrl Pts',(11.2148353959316,15.2,2.30266128502826));
#195720=CARTESIAN_POINT('Ctrl Pts',(11.2178328975308,15.2,2.30492554140367));
#195721=CARTESIAN_POINT('Ctrl Pts',(11.2208331426548,15.2,2.30719725782024));
#195722=CARTESIAN_POINT('Ctrl Pts',(11.223836094087,15.2,2.30947643623641));
#195723=CARTESIAN_POINT('Ctrl Pts',(11.2268390460647,15.2,2.31175561506664));
#195724=CARTESIAN_POINT('Ctrl Pts',(11.2298447017849,15.2,2.31404225509897));
#195725=CARTESIAN_POINT('Ctrl Pts',(11.2328530151807,15.2,2.31633635747505));
#195726=CARTESIAN_POINT('Ctrl Pts',(11.2358613280301,15.2,2.31863045943438));
#195727=CARTESIAN_POINT('Ctrl Pts',(11.2388722946416,15.2,2.32093202436442));
#195728=CARTESIAN_POINT('Ctrl Pts',(11.2418858730997,15.2,2.32324105243841));
#195729=CARTESIAN_POINT('Ctrl Pts',(11.2448994515577,15.2,2.32555008051241));
#195730=CARTESIAN_POINT('Ctrl Pts',(11.2479156408273,15.2,2.32786657206639));
#195731=CARTESIAN_POINT('Ctrl Pts',(11.2509344230443,15.2,2.33019052644606));
#195732=CARTESIAN_POINT('Ctrl Pts',(11.2539532052613,15.2,2.33251448082574));
#195733=CARTESIAN_POINT('Ctrl Pts',(11.2569745824506,15.2,2.3348458985751));
#195734=CARTESIAN_POINT('Ctrl Pts',(11.2599985479999,15.2,2.33718477899998));
#195735=CARTESIAN_POINT('Ctrl Pts',(10.2237731089999,12.2,1.76496130799999));
#195736=CARTESIAN_POINT('Ctrl Pts',(10.2255010835344,12.2,1.76541541469069));
#195737=CARTESIAN_POINT('Ctrl Pts',(10.227282994496,12.2,1.76588926687173));
#195738=CARTESIAN_POINT('Ctrl Pts',(10.2291177138156,12.2,1.76638321167919));
#195739=CARTESIAN_POINT('Ctrl Pts',(10.2309612810791,12.2,1.76687953853818));
#195740=CARTESIAN_POINT('Ctrl Pts',(10.2328581800569,12.2,1.76739616235299));
#195741=CARTESIAN_POINT('Ctrl Pts',(10.2348073231802,12.2,1.76793345482698));
#195742=CARTESIAN_POINT('Ctrl Pts',(10.2367564661264,12.2,1.76847074725216));
#195743=CARTESIAN_POINT('Ctrl Pts',(10.2387578528578,12.2,1.76902870390432));
#195744=CARTESIAN_POINT('Ctrl Pts',(10.2408104327832,12.2,1.76960768554995));
#195745=CARTESIAN_POINT('Ctrl Pts',(10.2428630127086,12.2,1.77018666719558));
#195746=CARTESIAN_POINT('Ctrl Pts',(10.2449667829652,12.2,1.77078667349933));
#195747=CARTESIAN_POINT('Ctrl Pts',(10.2471207194916,12.2,1.77140804417322));
#195748=CARTESIAN_POINT('Ctrl Pts',(10.2492746562137,12.2,1.77202941490356));
#195749=CARTESIAN_POINT('Ctrl Pts',(10.251478760386,12.2,1.77267215322635));
#195750=CARTESIAN_POINT('Ctrl Pts',(10.2537320330121,12.2,1.77333658784738));
#195751=CARTESIAN_POINT('Ctrl Pts',(10.256360850769,12.2,1.77411176148137));
#195752=CARTESIAN_POINT('Ctrl Pts',(10.2590565910528,12.2,1.77491646793701));
#195753=CARTESIAN_POINT('Ctrl Pts',(10.261817718071,12.2,1.77575121364745));
#195754=CARTESIAN_POINT('Ctrl Pts',(10.2641843986488,12.2,1.77646671005425));
#195755=CARTESIAN_POINT('Ctrl Pts',(10.2665991148725,12.2,1.77720427386484));
#195756=CARTESIAN_POINT('Ctrl Pts',(10.2690609287599,12.2,1.77796421232445));
#195757=CARTESIAN_POINT('Ctrl Pts',(10.2715227424237,12.2,1.77872415071503));
#195758=CARTESIAN_POINT('Ctrl Pts',(10.2740316523571,12.2,1.77950646297585));
#195759=CARTESIAN_POINT('Ctrl Pts',(10.276586740026,12.2,1.78031144528364));
#195760=CARTESIAN_POINT('Ctrl Pts',(10.2791418276949,12.2,1.78111642759144));
#195761=CARTESIAN_POINT('Ctrl Pts',(10.281743092104,12.2,1.78194408006059));
#195762=CARTESIAN_POINT('Ctrl Pts',(10.2843896398392,12.2,1.78279468544535));
#195763=CARTESIAN_POINT('Ctrl Pts',(10.2870361878147,12.2,1.78364529090738));
#195764=CARTESIAN_POINT('Ctrl Pts',(10.2897280175293,12.2,1.78451885269724));
#195765=CARTESIAN_POINT('Ctrl Pts',(10.2924642530148,12.2,1.78541564208103));
#195766=CARTESIAN_POINT('Ctrl Pts',(10.2952004882518,12.2,1.78631243138337));
#195767=CARTESIAN_POINT('Ctrl Pts',(10.2979811341463,12.2,1.78723245159305));
#195768=CARTESIAN_POINT('Ctrl Pts',(10.300805332129,12.2,1.7881759658098));
#195769=CARTESIAN_POINT('Ctrl Pts',(10.3036295301116,12.2,1.78911948002654));
#195770=CARTESIAN_POINT('Ctrl Pts',(10.3064972817074,12.2,1.79008648852474));
#195771=CARTESIAN_POINT('Ctrl Pts',(10.3094077538498,12.2,1.79107724790438));
#195772=CARTESIAN_POINT('Ctrl Pts',(10.3128033048588,12.2,1.79223313390729));
#195773=CARTESIAN_POINT('Ctrl Pts',(10.3162570022295,12.2,1.79342134934796));
#195774=CARTESIAN_POINT('Ctrl Pts',(10.3197675541057,12.2,1.79464228479875));
#195775=CARTESIAN_POINT('Ctrl Pts',(10.3227765984149,12.2,1.7956888008451));
#195776=CARTESIAN_POINT('Ctrl Pts',(10.3258274147873,12.2,1.79675935622287));
#195777=CARTESIAN_POINT('Ctrl Pts',(10.3289192080899,12.2,1.79785418743204));
#195778=CARTESIAN_POINT('Ctrl Pts',(10.3320110016733,12.2,1.79894901874066));
#195779=CARTESIAN_POINT('Ctrl Pts',(10.3351437736867,12.2,1.80006812807728));
#195780=CARTESIAN_POINT('Ctrl Pts',(10.3383167463624,12.2,1.80121174314127));
#195781=CARTESIAN_POINT('Ctrl Pts',(10.3414897187499,12.2,1.80235535810139));
#195782=CARTESIAN_POINT('Ctrl Pts',(10.3447028933688,12.2,1.80352348028232));
#195783=CARTESIAN_POINT('Ctrl Pts',(10.347955509669,12.2,1.80471633032339));
#195784=CARTESIAN_POINT('Ctrl Pts',(10.3512081259692,12.2,1.80590918036446));
#195785=CARTESIAN_POINT('Ctrl Pts',(10.3545001839163,12.2,1.8071267590119));
#195786=CARTESIAN_POINT('Ctrl Pts',(10.3578309395435,12.2,1.80836927996566));
#195787=CARTESIAN_POINT('Ctrl Pts',(10.3611616951708,12.2,1.80961180091942));
#195788=CARTESIAN_POINT('Ctrl Pts',(10.3645311495549,12.2,1.81087926476607));
#195789=CARTESIAN_POINT('Ctrl Pts',(10.3679385740951,12.2,1.81217187863405));
#195790=CARTESIAN_POINT('Ctrl Pts',(10.3713459989449,12.2,1.81346449261945));
#195791=CARTESIAN_POINT('Ctrl Pts',(10.3747913927401,12.2,1.81478225624894));
#195792=CARTESIAN_POINT('Ctrl Pts',(10.3782740436815,12.2,1.81612537032325));
#195793=CARTESIAN_POINT('Ctrl Pts',(10.3817566943066,12.2,1.81746848427556));
#195794=CARTESIAN_POINT('Ctrl Pts',(10.3852766014031,12.2,1.81883694746036));
#195795=CARTESIAN_POINT('Ctrl Pts',(10.3888330660399,12.2,1.82023095524931));
#195796=CARTESIAN_POINT('Ctrl Pts',(10.3923895306768,12.2,1.82162496303826));
#195797=CARTESIAN_POINT('Ctrl Pts',(10.3959825527803,12.2,1.82304451201334));
#195798=CARTESIAN_POINT('Ctrl Pts',(10.3996114455627,12.2,1.82448979362574));
#195799=CARTESIAN_POINT('Ctrl Pts',(10.4032403386747,12.2,1.82593507536942));
#195800=CARTESIAN_POINT('Ctrl Pts',(10.4069051046527,12.2,1.82740608543694));
#195801=CARTESIAN_POINT('Ctrl Pts',(10.4106050698746,12.2,1.82890300742815));
#195802=CARTESIAN_POINT('Ctrl Pts',(10.4136883740581,12.2,1.83015044235283));
#195803=CARTESIAN_POINT('Ctrl Pts',(10.4167961212353,12.2,1.83141586979413));
#195804=CARTESIAN_POINT('Ctrl Pts',(10.4199279311679,12.2,1.8326993936845));
#195805=CARTESIAN_POINT('Ctrl Pts',(10.4230597411004,12.2,1.83398291757487));
#195806=CARTESIAN_POINT('Ctrl Pts',(10.4262156133916,12.2,1.83528453345442));
#195807=CARTESIAN_POINT('Ctrl Pts',(10.4293951716574,12.2,1.83660434491424));
#195808=CARTESIAN_POINT('Ctrl Pts',(10.4325747295767,12.2,1.8379241562302));
#195809=CARTESIAN_POINT('Ctrl Pts',(10.4357779722426,12.2,1.83926216116631));
#195810=CARTESIAN_POINT('Ctrl Pts',(10.4390045303612,12.2,1.84061845407254));
#195811=CARTESIAN_POINT('Ctrl Pts',(10.4422310888315,12.2,1.8419747471266));
#195812=CARTESIAN_POINT('Ctrl Pts',(10.4454809623459,12.2,1.8433493293748));
#195813=CARTESIAN_POINT('Ctrl Pts',(10.4487537865801,12.2,1.84474229256775));
#195814=CARTESIAN_POINT('Ctrl Pts',(10.4520266108144,12.2,1.84613525576069));
#195815=CARTESIAN_POINT('Ctrl Pts',(10.4553223845839,12.2,1.8475466014861));
#195816=CARTESIAN_POINT('Ctrl Pts',(10.4586407491231,12.2,1.84897641808402));
#195817=CARTESIAN_POINT('Ctrl Pts',(10.4619591136623,12.2,1.85040623468195));
#195818=CARTESIAN_POINT('Ctrl Pts',(10.4653000711479,12.2,1.8518545245162));
#195819=CARTESIAN_POINT('Ctrl Pts',(10.4686632630217,12.2,1.85332137340412));
#195820=CARTESIAN_POINT('Ctrl Pts',(10.4720264548956,12.2,1.85478822229204));
#195821=CARTESIAN_POINT('Ctrl Pts',(10.4754118847616,12.2,1.85627363004155));
#195822=CARTESIAN_POINT('Ctrl Pts',(10.4788192008022,12.2,1.85777768386002));
#195823=CARTESIAN_POINT('Ctrl Pts',(10.4829079799022,12.2,1.85958254837661));
#195824=CARTESIAN_POINT('Ctrl Pts',(10.4870282781004,12.2,1.86141426084172));
#195825=CARTESIAN_POINT('Ctrl Pts',(10.4911795002807,12.2,1.86327296452234));
#195826=CARTESIAN_POINT('Ctrl Pts',(10.4946388522234,12.2,1.86482188431247));
#195827=CARTESIAN_POINT('Ctrl Pts',(10.4981196795769,12.2,1.86638954799397));
#195828=CARTESIAN_POINT('Ctrl Pts',(10.5016216447835,12.2,1.8679760352841));
#195829=CARTESIAN_POINT('Ctrl Pts',(10.5051236099901,12.2,1.86956252257423));
#195830=CARTESIAN_POINT('Ctrl Pts',(10.5086467117074,12.2,1.87116783397052));
#195831=CARTESIAN_POINT('Ctrl Pts',(10.5121906180636,12.2,1.87279204703646));
#195832=CARTESIAN_POINT('Ctrl Pts',(10.5157345244197,12.2,1.87441626010239));
#195833=CARTESIAN_POINT('Ctrl Pts',(10.5192992346944,12.2,1.87605937391457));
#195834=CARTESIAN_POINT('Ctrl Pts',(10.5228844200405,12.2,1.87772146439968));
#195835=CARTESIAN_POINT('Ctrl Pts',(10.5264696053867,12.2,1.8793835548848));
#195836=CARTESIAN_POINT('Ctrl Pts',(10.5300752665139,12.2,1.88106462272875));
#195837=CARTESIAN_POINT('Ctrl Pts',(10.5337010777629,12.2,1.88276473988053));
#195838=CARTESIAN_POINT('Ctrl Pts',(10.5373268890118,12.2,1.88446485703231));
#195839=CARTESIAN_POINT('Ctrl Pts',(10.540972851828,12.2,1.88618402414291));
#195840=CARTESIAN_POINT('Ctrl Pts',(10.5446386447436,12.2,1.88792231212803));
#195841=CARTESIAN_POINT('Ctrl Pts',(10.5483044376593,12.2,1.88966060011315));
#195842=CARTESIAN_POINT('Ctrl Pts',(10.55199006247,12.2,1.89141800835207));
#195843=CARTESIAN_POINT('Ctrl Pts',(10.5556952027645,12.2,1.89319460704064));
#195844=CARTESIAN_POINT('Ctrl Pts',(10.5594003430591,12.2,1.89497120572921));
#195845=CARTESIAN_POINT('Ctrl Pts',(10.5631249964999,12.2,1.89676699353326));
#195846=CARTESIAN_POINT('Ctrl Pts',(10.5668688552499,12.2,1.8985820374916));
#195847=CARTESIAN_POINT('Ctrl Pts',(10.5698639424131,12.2,1.9000340727374));
#195848=CARTESIAN_POINT('Ctrl Pts',(10.5728713198333,12.2,1.90149843387631));
#195849=CARTESIAN_POINT('Ctrl Pts',(10.5758908297769,12.2,1.90297515095805));
#195850=CARTESIAN_POINT('Ctrl Pts',(10.5796652165893,12.2,1.90482104700843));
#195851=CARTESIAN_POINT('Ctrl Pts',(10.5834585619572,12.2,1.90668625184932));
#195852=CARTESIAN_POINT('Ctrl Pts',(10.5872705595263,12.2,1.9085708287951));
#195853=CARTESIAN_POINT('Ctrl Pts',(10.5903201580802,12.2,1.91007849059822));
#195854=CARTESIAN_POINT('Ctrl Pts',(10.5933816942018,12.2,1.9115985502303));
#195855=CARTESIAN_POINT('Ctrl Pts',(10.5964550147582,12.2,1.91313103925827));
#195856=CARTESIAN_POINT('Ctrl Pts',(10.6002966652444,12.2,1.91504665043883));
#195857=CARTESIAN_POINT('Ctrl Pts',(10.604156728901,12.2,1.91698168230319));
#195858=CARTESIAN_POINT('Ctrl Pts',(10.6080349062104,12.2,1.91893619599267));
#195859=CARTESIAN_POINT('Ctrl Pts',(10.6111374478042,12.2,1.92049980681643));
#195860=CARTESIAN_POINT('Ctrl Pts',(10.6142515842205,12.2,1.92207588593802));
#195861=CARTESIAN_POINT('Ctrl Pts',(10.6173771624639,12.2,1.92366446147354));
#195862=CARTESIAN_POINT('Ctrl Pts',(10.620502741133,12.2,1.92525303722551));
#195863=CARTESIAN_POINT('Ctrl Pts',(10.6236397638061,12.2,1.92685411067588));
#195864=CARTESIAN_POINT('Ctrl Pts',(10.6267880791999,12.2,1.9284677110416));
#195865=CARTESIAN_POINT('Ctrl Pts',(10.6299363945937,12.2,1.93008131140732));
#195866=CARTESIAN_POINT('Ctrl Pts',(10.6330960050694,12.2,1.93170743855783));
#195867=CARTESIAN_POINT('Ctrl Pts',(10.6362667610767,12.2,1.93334612025953));
#195868=CARTESIAN_POINT('Ctrl Pts',(10.6402302054377,12.2,1.93539447205175));
#195869=CARTESIAN_POINT('Ctrl Pts',(10.6442110659086,12.2,1.93746244162271));
#195870=CARTESIAN_POINT('Ctrl Pts',(10.6482090562353,12.2,1.93955008097688));
#195871=CARTESIAN_POINT('Ctrl Pts',(10.6514074490196,12.2,1.94122019273328));
#195872=CARTESIAN_POINT('Ctrl Pts',(10.6546168056938,12.2,1.9429028934992));
#195873=CARTESIAN_POINT('Ctrl Pts',(10.6578369822582,12.2,1.94459821175826));
#195874=CARTESIAN_POINT('Ctrl Pts',(10.6610571588226,12.2,1.94629353001733));
#195875=CARTESIAN_POINT('Ctrl Pts',(10.6642881529605,12.2,1.94800146288064));
#195876=CARTESIAN_POINT('Ctrl Pts',(10.6675298243049,12.2,1.94972203853126));
#195877=CARTESIAN_POINT('Ctrl Pts',(10.6707714952077,12.2,1.95144261394744));
#195878=CARTESIAN_POINT('Ctrl Pts',(10.6740238429302,12.2,1.95317583285026));
#195879=CARTESIAN_POINT('Ctrl Pts',(10.677286723956,12.2,1.95492171771542));
#195880=CARTESIAN_POINT('Ctrl Pts',(10.6805496054264,12.2,1.95666760281846));
#195881=CARTESIAN_POINT('Ctrl Pts',(10.6838230218457,12.2,1.95842615545561));
#195882=CARTESIAN_POINT('Ctrl Pts',(10.6871068318035,12.2,1.96019740049788));
#195883=CARTESIAN_POINT('Ctrl Pts',(10.6903906413139,12.2,1.96196864529881));
#195884=CARTESIAN_POINT('Ctrl Pts',(10.6936848439284,12.2,1.96375258195922));
#195885=CARTESIAN_POINT('Ctrl Pts',(10.6969893022132,12.2,1.96554923531151));
#195886=CARTESIAN_POINT('Ctrl Pts',(10.7002937609482,12.2,1.9673458889086));
#195887=CARTESIAN_POINT('Ctrl Pts',(10.7036084731898,12.2,1.96915525855073));
#195888=CARTESIAN_POINT('Ctrl Pts',(10.7069333039824,12.2,1.97097736829774));
#195889=CARTESIAN_POINT('Ctrl Pts',(10.710258134322,12.2,1.97279947779648));
#195890=CARTESIAN_POINT('Ctrl Pts',(10.7135930812368,12.2,1.9746343252259));
#195891=CARTESIAN_POINT('Ctrl Pts',(10.7169380076849,12.2,1.97648193657401));
#195892=CARTESIAN_POINT('Ctrl Pts',(10.7202829345887,12.2,1.97832954817386));
#195893=CARTESIAN_POINT('Ctrl Pts',(10.723637841816,12.2,1.98018992194748));
#195894=CARTESIAN_POINT('Ctrl Pts',(10.7270025945001,12.2,1.98206307966152));
#195895=CARTESIAN_POINT('Ctrl Pts',(10.7303673467257,12.2,1.98393623712034));
#195896=CARTESIAN_POINT('Ctrl Pts',(10.7337419435507,12.2,1.98582218001653));
#195897=CARTESIAN_POINT('Ctrl Pts',(10.7371262507755,12.2,1.98772092823282));
#195898=CARTESIAN_POINT('Ctrl Pts',(10.7422027123046,12.2,1.99056905094533));
#195899=CARTESIAN_POINT('Ctrl Pts',(10.7473010240275,12.2,1.993445988323));
#195900=CARTESIAN_POINT('Ctrl Pts',(10.752420735308,12.2,1.99635180881668));
#195901=CARTESIAN_POINT('Ctrl Pts',(10.7558338756966,12.2,1.99828902221519));
#195902=CARTESIAN_POINT('Ctrl Pts',(10.7592565278284,12.2,2.00023907326201));
#195903=CARTESIAN_POINT('Ctrl Pts',(10.7626885607694,12.2,2.00220198132292));
#195904=CARTESIAN_POINT('Ctrl Pts',(10.7661205941781,12.2,2.00416488965128));
#195905=CARTESIAN_POINT('Ctrl Pts',(10.7695620076061,12.2,2.00614065531861));
#195906=CARTESIAN_POINT('Ctrl Pts',(10.7730126713007,12.2,2.00812929830524));
#195907=CARTESIAN_POINT('Ctrl Pts',(10.7764633345251,12.2,2.01011794102092));
#195908=CARTESIAN_POINT('Ctrl Pts',(10.7799232482395,12.2,2.01211945877313));
#195909=CARTESIAN_POINT('Ctrl Pts',(10.7833922827331,12.2,2.01413387338538));
#195910=CARTESIAN_POINT('Ctrl Pts',(10.7877285762045,12.2,2.01665189185654));
#195911=CARTESIAN_POINT('Ctrl Pts',(10.7920791223375,12.2,2.01919005935047));
#195912=CARTESIAN_POINT('Ctrl Pts',(10.7964436707396,12.2,2.02174841205774));
#195913=CARTESIAN_POINT('Ctrl Pts',(10.7999353096515,12.2,2.0237950943351));
#195914=CARTESIAN_POINT('Ctrl Pts',(10.8034359106256,12.2,2.0258546949168));
#195915=CARTESIAN_POINT('Ctrl Pts',(10.8069453460952,12.2,2.02792723191949));
#195916=CARTESIAN_POINT('Ctrl Pts',(10.8104547810867,12.2,2.0299997686398));
#195917=CARTESIAN_POINT('Ctrl Pts',(10.8139730500538,12.2,2.03208524130502));
#195918=CARTESIAN_POINT('Ctrl Pts',(10.8175000299965,12.2,2.03418366740384));
#195919=CARTESIAN_POINT('Ctrl Pts',(10.8210270104197,12.2,2.03628209378858));
#195920=CARTESIAN_POINT('Ctrl Pts',(10.8245626999794,12.2,2.03839347244877));
#195921=CARTESIAN_POINT('Ctrl Pts',(10.8281069748397,12.2,2.04051782139872));
#195922=CARTESIAN_POINT('Ctrl Pts',(10.8316512492172,12.2,2.04264217005924));
#195923=CARTESIAN_POINT('Ctrl Pts',(10.8352041084096,12.2,2.04477948931438));
#195924=CARTESIAN_POINT('Ctrl Pts',(10.838765429451,12.2,2.04692979391504));
#195925=CARTESIAN_POINT('Ctrl Pts',(10.8423267509775,12.2,2.04908009880867));
#195926=CARTESIAN_POINT('Ctrl Pts',(10.8458965344299,12.2,2.05124338814788));
#195927=CARTESIAN_POINT('Ctrl Pts',(10.8494746567524,12.2,2.05341967977642));
#195928=CARTESIAN_POINT('Ctrl Pts',(10.8530527785872,12.2,2.05559597110844));
#195929=CARTESIAN_POINT('Ctrl Pts',(10.8566392405291,12.2,2.05778526518234));
#195930=CARTESIAN_POINT('Ctrl Pts',(10.8602339196788,12.2,2.05998757388986));
#195931=CARTESIAN_POINT('Ctrl Pts',(10.8638285993184,12.2,2.06218988289744));
#195932=CARTESIAN_POINT('Ctrl Pts',(10.8674314978142,12.2,2.06440520789793));
#195933=CARTESIAN_POINT('Ctrl Pts',(10.8710424922332,12.2,2.06663356474159));
#195934=CARTESIAN_POINT('Ctrl Pts',(10.8746534866523,12.2,2.06886192158525));
#195935=CARTESIAN_POINT('Ctrl Pts',(10.8782725796639,12.2,2.07110330940823));
#195936=CARTESIAN_POINT('Ctrl Pts',(10.8818996505846,12.2,2.07335774114354));
#195937=CARTESIAN_POINT('Ctrl Pts',(10.8873402564715,12.2,2.07673938843934));
#195938=CARTESIAN_POINT('Ctrl Pts',(10.8927988116549,12.2,2.08015038720294));
#195939=CARTESIAN_POINT('Ctrl Pts',(10.8982749185401,12.2,2.08359078316256));
#195940=CARTESIAN_POINT('Ctrl Pts',(10.9019256562977,12.2,2.0858843803648));
#195941=CARTESIAN_POINT('Ctrl Pts',(10.9055841938399,12.2,2.08819104081164));
#195942=CARTESIAN_POINT('Ctrl Pts',(10.9092504156505,12.2,2.09051078062066));
#195943=CARTESIAN_POINT('Ctrl Pts',(10.9129166379606,12.2,2.09283052074575));
#195944=CARTESIAN_POINT('Ctrl Pts',(10.9165905423378,12.2,2.09516333765187));
#195945=CARTESIAN_POINT('Ctrl Pts',(10.9202720152774,12.2,2.09750924523487));
#195946=CARTESIAN_POINT('Ctrl Pts',(10.9239534877154,12.2,2.09985515249824));
#195947=CARTESIAN_POINT('Ctrl Pts',(10.9276425279235,12.2,2.10221414961292));
#195948=CARTESIAN_POINT('Ctrl Pts',(10.9313390191205,12.2,2.1045862488621));
#195949=CARTESIAN_POINT('Ctrl Pts',(10.9350355108212,12.2,2.10695834843448));
#195950=CARTESIAN_POINT('Ctrl Pts',(10.9387394539032,12.2,2.10934354991367));
#195951=CARTESIAN_POINT('Ctrl Pts',(10.9424507355499,12.2,2.11174186426659));
#195952=CARTESIAN_POINT('Ctrl Pts',(10.9461620171966,12.2,2.11414017861952));
#195953=CARTESIAN_POINT('Ctrl Pts',(10.9498806351581,12.2,2.116551607974));
#195954=CARTESIAN_POINT('Ctrl Pts',(10.9536064780841,12.2,2.11897615966302));
#195955=CARTESIAN_POINT('Ctrl Pts',(10.9564008600248,12.2,2.12079457326461));
#195956=CARTESIAN_POINT('Ctrl Pts',(10.9591993051035,12.2,2.12262037017885));
#195957=CARTESIAN_POINT('Ctrl Pts',(10.9620017658088,12.2,2.12445355337135));
#195958=CARTESIAN_POINT('Ctrl Pts',(10.9657383799129,12.2,2.12689779751701));
#195959=CARTESIAN_POINT('Ctrl Pts',(10.9694821348616,12.2,2.12935517419258));
#195960=CARTESIAN_POINT('Ctrl Pts',(10.9732329154434,12.2,2.13182569282309));
#195961=CARTESIAN_POINT('Ctrl Pts',(10.9760460010075,12.2,2.13367858188013));
#195962=CARTESIAN_POINT('Ctrl Pts',(10.9788630393713,12.2,2.13553886474498));
#195963=CARTESIAN_POINT('Ctrl Pts',(10.9816839843933,12.2,2.13740654334279));
#195964=CARTESIAN_POINT('Ctrl Pts',(10.9845049299278,12.2,2.13927422227989));
#195965=CARTESIAN_POINT('Ctrl Pts',(10.9873297811883,12.2,2.14114929818572));
#195966=CARTESIAN_POINT('Ctrl Pts',(10.9901584913082,12.2,2.14303177412699));
#195967=CARTESIAN_POINT('Ctrl Pts',(10.9939301039451,12.2,2.1455417414787));
#195968=CARTESIAN_POINT('Ctrl Pts',(10.9977085772952,12.2,2.14806486740242));
#195969=CARTESIAN_POINT('Ctrl Pts',(11.0014938017807,12.2,2.15060115803988));
#195970=CARTESIAN_POINT('Ctrl Pts',(11.0043327202737,12.2,2.15250337610436));
#195971=CARTESIAN_POINT('Ctrl Pts',(11.0071754363268,12.2,2.15441300099473));
#195972=CARTESIAN_POINT('Ctrl Pts',(11.0100219029314,12.2,2.15633003454943));
#195973=CARTESIAN_POINT('Ctrl Pts',(11.012868369536,12.2,2.15824706810413));
#195974=CARTESIAN_POINT('Ctrl Pts',(11.015718587582,12.2,2.16017151106667));
#195975=CARTESIAN_POINT('Ctrl Pts',(11.0185725111028,12.2,2.16210336707879));
#195976=CARTESIAN_POINT('Ctrl Pts',(11.021426435142,12.2,2.16403522344187));
#195977=CARTESIAN_POINT('Ctrl Pts',(11.0242840643573,12.2,2.16597449334039));
#195978=CARTESIAN_POINT('Ctrl Pts',(11.0271453533987,12.2,2.16792117920765));
#195979=CARTESIAN_POINT('Ctrl Pts',(11.0300066419202,12.2,2.16986786472126));
#195980=CARTESIAN_POINT('Ctrl Pts',(11.0328715893654,12.2,2.17182196655192));
#195981=CARTESIAN_POINT('Ctrl Pts',(11.0357401524883,12.2,2.17378348912119));
#195982=CARTESIAN_POINT('Ctrl Pts',(11.0386087156111,12.2,2.17574501169045));
#195983=CARTESIAN_POINT('Ctrl Pts',(11.0414808920176,12.2,2.17771395390331));
#195984=CARTESIAN_POINT('Ctrl Pts',(11.0443566385384,12.2,2.17969031845715));
#195985=CARTESIAN_POINT('Ctrl Pts',(11.0472323850593,12.2,2.18166668301098));
#195986=CARTESIAN_POINT('Ctrl Pts',(11.0501117016547,12.2,2.18365047098895));
#195987=CARTESIAN_POINT('Ctrl Pts',(11.0529945412583,12.2,2.18564168495826));
#195988=CARTESIAN_POINT('Ctrl Pts',(11.0558773808618,12.2,2.18763289892758));
#195989=CARTESIAN_POINT('Ctrl Pts',(11.0587637445903,12.2,2.1896315388716));
#195990=CARTESIAN_POINT('Ctrl Pts',(11.0616535886933,12.2,2.19163760779806));
#195991=CARTESIAN_POINT('Ctrl Pts',(11.0645434327964,12.2,2.19364367672452));
#195992=CARTESIAN_POINT('Ctrl Pts',(11.0674367574171,12.2,2.19565717378234));
#195993=CARTESIAN_POINT('Ctrl Pts',(11.0703335171645,12.2,2.19767810335068));
#195994=CARTESIAN_POINT('Ctrl Pts',(11.0732302769119,12.2,2.19969903291901));
#195995=CARTESIAN_POINT('Ctrl Pts',(11.0761304723229,12.2,2.20172739483113));
#195996=CARTESIAN_POINT('Ctrl Pts',(11.0790340583836,12.2,2.20376319033947));
#195997=CARTESIAN_POINT('Ctrl Pts',(11.0819376449718,12.2,2.20579898621764));
#195998=CARTESIAN_POINT('Ctrl Pts',(11.0848446225943,12.2,2.20784221601461));
#195999=CARTESIAN_POINT('Ctrl Pts',(11.0877549481844,12.2,2.20989288339698));
#196000=CARTESIAN_POINT('Ctrl Pts',(11.0916353814233,12.2,2.21262710595259));
#196001=CARTESIAN_POINT('Ctrl Pts',(11.0955217660643,12.2,2.21537455062593));
#196002=CARTESIAN_POINT('Ctrl Pts',(11.0994139966901,12.2,2.21813522056604));
#196003=CARTESIAN_POINT('Ctrl Pts',(11.1023331697921,12.2,2.22020572311515));
#196004=CARTESIAN_POINT('Ctrl Pts',(11.1052556321355,12.2,2.22228366670545));
#196005=CARTESIAN_POINT('Ctrl Pts',(11.1081813406955,12.2,2.22436905225366));
#196006=CARTESIAN_POINT('Ctrl Pts',(11.1111070497869,12.2,2.22645443818071));
#196007=CARTESIAN_POINT('Ctrl Pts',(11.1140360041792,12.2,2.22854726731821));
#196008=CARTESIAN_POINT('Ctrl Pts',(11.1169681613975,12.2,2.2306475402078));
#196009=CARTESIAN_POINT('Ctrl Pts',(11.119900318083,12.2,2.23274781271583));
#196010=CARTESIAN_POINT('Ctrl Pts',(11.1228356784281,12.2,2.23485553037956));
#196011=CARTESIAN_POINT('Ctrl Pts',(11.1257741973018,12.2,2.23697069440924));
#196012=CARTESIAN_POINT('Ctrl Pts',(11.1296922222889,12.2,2.2397909129874));
#196013=CARTESIAN_POINT('Ctrl Pts',(11.1336158662392,12.2,2.2426243684537));
#196014=CARTESIAN_POINT('Ctrl Pts',(11.1375450236954,12.2,2.24547106827567));
#196015=CARTESIAN_POINT('Ctrl Pts',(11.1404918919214,12.2,2.24760609323912));
#196016=CARTESIAN_POINT('Ctrl Pts',(11.1434418642139,12.2,2.24974856774373));
#196017=CARTESIAN_POINT('Ctrl Pts',(11.1463948963562,12.2,2.25189849228959));
#196018=CARTESIAN_POINT('Ctrl Pts',(11.1493479290349,12.2,2.25404841722602));
#196019=CARTESIAN_POINT('Ctrl Pts',(11.1523040214645,12.2,2.25620579383957));
#196020=CARTESIAN_POINT('Ctrl Pts',(11.1552631331034,12.2,2.25837062269688));
#196021=CARTESIAN_POINT('Ctrl Pts',(11.1582222442046,12.2,2.26053545116091));
#196022=CARTESIAN_POINT('Ctrl Pts',(11.1611843737996,12.2,2.26270773239117));
#196023=CARTESIAN_POINT('Ctrl Pts',(11.164149479007,12.2,2.2648874674634));
#196024=CARTESIAN_POINT('Ctrl Pts',(11.1671145842144,12.2,2.26706720253563));
#196025=CARTESIAN_POINT('Ctrl Pts',(11.1700826647982,12.2,2.26925439201835));
#196026=CARTESIAN_POINT('Ctrl Pts',(11.1730536798988,12.2,2.27144903652261));
#196027=CARTESIAN_POINT('Ctrl Pts',(11.1760246949995,12.2,2.27364368102686));
#196028=CARTESIAN_POINT('Ctrl Pts',(11.1789986447914,12.2,2.27584578101355));
#196029=CARTESIAN_POINT('Ctrl Pts',(11.1819754870166,12.2,2.27805533797493));
#196030=CARTESIAN_POINT('Ctrl Pts',(11.1849523292418,12.2,2.28026489493631));
#196031=CARTESIAN_POINT('Ctrl Pts',(11.1879320656002,12.2,2.28248190915573));
#196032=CARTESIAN_POINT('Ctrl Pts',(11.1909146536999,12.2,2.28470638153259));
#196033=CARTESIAN_POINT('Ctrl Pts',(11.1938972417996,12.2,2.28693085390945));
#196034=CARTESIAN_POINT('Ctrl Pts',(11.1968826812314,12.2,2.28916278328709));
#196035=CARTESIAN_POINT('Ctrl Pts',(11.1998709304385,12.2,2.29140217281674));
#196036=CARTESIAN_POINT('Ctrl Pts',(11.2028591796455,12.2,2.29364156234638));
#196037=CARTESIAN_POINT('Ctrl Pts',(11.2058502369064,12.2,2.29588841127475));
#196038=CARTESIAN_POINT('Ctrl Pts',(11.2088440626306,12.2,2.29814271977517));
#196039=CARTESIAN_POINT('Ctrl Pts',(11.2118378888987,12.2,2.30039702868511));
#196040=CARTESIAN_POINT('Ctrl Pts',(11.2148344848675,12.2,2.30265879861382));
#196041=CARTESIAN_POINT('Ctrl Pts',(11.2178338116788,12.2,2.3049280289863));
#196042=CARTESIAN_POINT('Ctrl Pts',(11.2208331379452,12.2,2.30719725894655));
#196043=CARTESIAN_POINT('Ctrl Pts',(11.2238351975198,12.2,2.30947394988138));
#196044=CARTESIAN_POINT('Ctrl Pts',(11.2268399461192,12.2,2.31175810275736));
#196045=CARTESIAN_POINT('Ctrl Pts',(11.2298446947185,12.2,2.31404225563335));
#196046=CARTESIAN_POINT('Ctrl Pts',(11.2328521331984,12.2,2.31633386937509));
#196047=CARTESIAN_POINT('Ctrl Pts',(11.2358622107693,12.2,2.31863294676036));
#196048=CARTESIAN_POINT('Ctrl Pts',(11.2398756473484,12.2,2.32169838313483));
#196049=CARTESIAN_POINT('Ctrl Pts',(11.2438937704077,12.2,2.32477708723464));
#196050=CARTESIAN_POINT('Ctrl Pts',(11.2479165051339,12.2,2.32786905903606));
#196051=CARTESIAN_POINT('Ctrl Pts',(11.2519392404082,12.2,2.33096103125876));
#196052=CARTESIAN_POINT('Ctrl Pts',(11.2559665935679,12.2,2.33406627148354));
#196053=CARTESIAN_POINT('Ctrl Pts',(11.2599985479999,12.2,2.33718477899998));
#196054=CARTESIAN_POINT('Ctrl Pts',(11.1757778679999,15.2,2.71145515299998));
#196055=CARTESIAN_POINT('Ctrl Pts',(11.1757778679999,11.6,2.71145515299998));
#196056=CARTESIAN_POINT('Ctrl Pts',(11.1750309949999,15.2,2.71161876799999));
#196057=CARTESIAN_POINT('Ctrl Pts',(11.1750309949999,11.6,2.71161876799999));
#196058=CARTESIAN_POINT('Ctrl Pts',(11.1735376169999,15.2,2.71194562399998));
#196059=CARTESIAN_POINT('Ctrl Pts',(11.1735376169999,11.6,2.71194562399998));
#196060=CARTESIAN_POINT('Ctrl Pts',(11.1712986599999,15.2,2.71243477999998));
#196061=CARTESIAN_POINT('Ctrl Pts',(11.1712986599999,11.6,2.71243477999998));
#196062=CARTESIAN_POINT('Ctrl Pts',(11.1683155989999,15.2,2.71308473599999));
#196063=CARTESIAN_POINT('Ctrl Pts',(11.1683155989999,11.6,2.71308473599999));
#196064=CARTESIAN_POINT('Ctrl Pts',(11.1645904639999,15.2,2.71389342499998));
#196065=CARTESIAN_POINT('Ctrl Pts',(11.1645904639999,11.6,2.71389342499998));
#196066=CARTESIAN_POINT('Ctrl Pts',(11.1608690239999,15.2,2.71469835899998));
#196067=CARTESIAN_POINT('Ctrl Pts',(11.1608690239999,11.6,2.71469835899998));
#196068=CARTESIAN_POINT('Ctrl Pts',(11.1571512799999,15.2,2.71549953899999));
#196069=CARTESIAN_POINT('Ctrl Pts',(11.1571512799999,11.6,2.71549953899999));
#196070=CARTESIAN_POINT('Ctrl Pts',(11.1534372359999,15.2,2.71629696699998));
#196071=CARTESIAN_POINT('Ctrl Pts',(11.1534372359999,11.6,2.71629696699998));
#196072=CARTESIAN_POINT('Ctrl Pts',(11.1497268969999,15.2,2.71709064499999));
#196073=CARTESIAN_POINT('Ctrl Pts',(11.1497268969999,11.6,2.71709064499999));
#196074=CARTESIAN_POINT('Ctrl Pts',(11.1460202709999,15.2,2.71788057599998));
#196075=CARTESIAN_POINT('Ctrl Pts',(11.1460202709999,11.6,2.71788057599998));
#196076=CARTESIAN_POINT('Ctrl Pts',(11.1423173659999,15.2,2.71866676499998));
#196077=CARTESIAN_POINT('Ctrl Pts',(11.1423173659999,11.6,2.71866676499998));
#196078=CARTESIAN_POINT('Ctrl Pts',(11.1386181909999,15.2,2.71944921899999));
#196079=CARTESIAN_POINT('Ctrl Pts',(11.1386181909999,11.6,2.71944921899998));
#196080=CARTESIAN_POINT('Ctrl Pts',(11.1349227589999,15.2,2.72022793899998));
#196081=CARTESIAN_POINT('Ctrl Pts',(11.1349227589999,11.6,2.72022793899998));
#196082=CARTESIAN_POINT('Ctrl Pts',(11.1312310749999,15.2,2.72100293299999));
#196083=CARTESIAN_POINT('Ctrl Pts',(11.1312310749999,11.6,2.72100293299999));
#196084=CARTESIAN_POINT('Ctrl Pts',(11.1275431529999,15.2,2.72177420499998));
#196085=CARTESIAN_POINT('Ctrl Pts',(11.1275431529999,11.6,2.72177420499998));
#196086=CARTESIAN_POINT('Ctrl Pts',(11.1238589999999,15.2,2.72254175699998));
#196087=CARTESIAN_POINT('Ctrl Pts',(11.1238589999999,11.6,2.72254175699998));
#196088=CARTESIAN_POINT('Ctrl Pts',(11.1201786229999,15.2,2.72330559599999));
#196089=CARTESIAN_POINT('Ctrl Pts',(11.1201786229999,11.6,2.72330559599998));
#196090=CARTESIAN_POINT('Ctrl Pts',(11.1165020289999,15.2,2.72406572399999));
#196091=CARTESIAN_POINT('Ctrl Pts',(11.1165020289999,11.6,2.72406572399999));
#196092=CARTESIAN_POINT('Ctrl Pts',(11.1128292269999,15.2,2.72482214499998));
#196093=CARTESIAN_POINT('Ctrl Pts',(11.1128292269999,11.6,2.72482214499998));
#196094=CARTESIAN_POINT('Ctrl Pts',(11.1091602219999,15.2,2.72557486299998));
#196095=CARTESIAN_POINT('Ctrl Pts',(11.1091602219999,11.6,2.72557486299998));
#196096=CARTESIAN_POINT('Ctrl Pts',(11.1054950239999,15.2,2.72632388099999));
#196097=CARTESIAN_POINT('Ctrl Pts',(11.1054950239999,11.6,2.72632388099999));
#196098=CARTESIAN_POINT('Ctrl Pts',(11.1018336399999,15.2,2.72706920299999));
#196099=CARTESIAN_POINT('Ctrl Pts',(11.1018336399999,11.6,2.72706920299999));
#196100=CARTESIAN_POINT('Ctrl Pts',(11.0981760779999,15.2,2.72781083499999));
#196101=CARTESIAN_POINT('Ctrl Pts',(11.0981760779999,11.6,2.72781083499999));
#196102=CARTESIAN_POINT('Ctrl Pts',(11.0945223469999,15.2,2.72854877899999));
#196103=CARTESIAN_POINT('Ctrl Pts',(11.0945223469999,11.6,2.72854877899999));
#196104=CARTESIAN_POINT('Ctrl Pts',(11.0908724549999,15.2,2.72928304099998));
#196105=CARTESIAN_POINT('Ctrl Pts',(11.0908724549999,11.6,2.72928304099998));
#196106=CARTESIAN_POINT('Ctrl Pts',(11.0872264109999,15.2,2.73001362299999));
#196107=CARTESIAN_POINT('Ctrl Pts',(11.0872264109999,11.6,2.73001362299999));
#196108=CARTESIAN_POINT('Ctrl Pts',(11.0835842229999,15.2,2.73074053299998));
#196109=CARTESIAN_POINT('Ctrl Pts',(11.0835842229999,11.6,2.73074053299998));
#196110=CARTESIAN_POINT('Ctrl Pts',(11.0799458989999,15.2,2.73146377099999));
#196111=CARTESIAN_POINT('Ctrl Pts',(11.0799458989999,11.6,2.73146377099999));
#196112=CARTESIAN_POINT('Ctrl Pts',(11.0763114489999,15.2,2.73218334499998));
#196113=CARTESIAN_POINT('Ctrl Pts',(11.0763114489999,11.6,2.73218334499998));
#196114=CARTESIAN_POINT('Ctrl Pts',(11.0726808779999,15.2,2.73289925699999));
#196115=CARTESIAN_POINT('Ctrl Pts',(11.0726808779999,11.6,2.73289925699999));
#196116=CARTESIAN_POINT('Ctrl Pts',(11.0690541959999,15.2,2.73361151099999));
#196117=CARTESIAN_POINT('Ctrl Pts',(11.0690541959999,11.6,2.73361151099999));
#196118=CARTESIAN_POINT('Ctrl Pts',(11.0654314099999,15.2,2.73432011199999));
#196119=CARTESIAN_POINT('Ctrl Pts',(11.0654314099999,11.6,2.73432011199999));
#196120=CARTESIAN_POINT('Ctrl Pts',(11.0618125299999,15.2,2.73502506399999));
#196121=CARTESIAN_POINT('Ctrl Pts',(11.0618125299999,11.6,2.73502506399998));
#196122=CARTESIAN_POINT('Ctrl Pts',(11.0581975619999,15.2,2.73572636999998));
#196123=CARTESIAN_POINT('Ctrl Pts',(11.0581975619999,11.6,2.73572636999998));
#196124=CARTESIAN_POINT('Ctrl Pts',(11.0545865169999,15.2,2.73642403699998));
#196125=CARTESIAN_POINT('Ctrl Pts',(11.0545865169999,11.6,2.73642403699998));
#196126=CARTESIAN_POINT('Ctrl Pts',(11.0509794009999,15.2,2.73711806699998));
#196127=CARTESIAN_POINT('Ctrl Pts',(11.0509794009999,11.6,2.73711806699998));
#196128=CARTESIAN_POINT('Ctrl Pts',(11.0473762219999,15.2,2.73780846599998));
#196129=CARTESIAN_POINT('Ctrl Pts',(11.0473762219999,11.6,2.73780846599998));
#196130=CARTESIAN_POINT('Ctrl Pts',(11.0437769909999,15.2,2.73849523599999));
#196131=CARTESIAN_POINT('Ctrl Pts',(11.0437769909999,11.6,2.73849523599999));
#196132=CARTESIAN_POINT('Ctrl Pts',(11.0401817149999,15.2,2.73917838399999));
#196133=CARTESIAN_POINT('Ctrl Pts',(11.0401817149999,11.6,2.73917838399999));
#196134=CARTESIAN_POINT('Ctrl Pts',(11.0365903999999,15.2,2.73985791299998));
#196135=CARTESIAN_POINT('Ctrl Pts',(11.0365903999999,11.6,2.73985791299998));
#196136=CARTESIAN_POINT('Ctrl Pts',(11.0330030589999,15.2,2.74053382799998));
#196137=CARTESIAN_POINT('Ctrl Pts',(11.0330030589999,11.6,2.74053382799998));
#196138=CARTESIAN_POINT('Ctrl Pts',(11.0294196959999,15.2,2.74120613199998));
#196139=CARTESIAN_POINT('Ctrl Pts',(11.0294196959999,11.6,2.74120613199998));
#196140=CARTESIAN_POINT('Ctrl Pts',(11.0258403219999,15.2,2.74187483099999));
#196141=CARTESIAN_POINT('Ctrl Pts',(11.0258403219999,11.6,2.74187483099999));
#196142=CARTESIAN_POINT('Ctrl Pts',(11.0222649439999,15.2,2.74253992799999));
#196143=CARTESIAN_POINT('Ctrl Pts',(11.0222649439999,11.6,2.74253992799998));
#196144=CARTESIAN_POINT('Ctrl Pts',(11.0186935709999,15.2,2.74320142899998));
#196145=CARTESIAN_POINT('Ctrl Pts',(11.0186935709999,11.6,2.74320142899998));
#196146=CARTESIAN_POINT('Ctrl Pts',(11.0151262099999,15.2,2.74385933599999));
#196147=CARTESIAN_POINT('Ctrl Pts',(11.0151262099999,11.6,2.74385933599999));
#196148=CARTESIAN_POINT('Ctrl Pts',(11.0115628719999,15.2,2.74451365599998));
#196149=CARTESIAN_POINT('Ctrl Pts',(11.0115628719999,11.6,2.74451365599998));
#196150=CARTESIAN_POINT('Ctrl Pts',(11.0080035629999,15.2,2.74516439199999));
#196151=CARTESIAN_POINT('Ctrl Pts',(11.0080035629999,11.6,2.74516439199999));
#196152=CARTESIAN_POINT('Ctrl Pts',(11.0044482939999,15.2,2.74581154899998));
#196153=CARTESIAN_POINT('Ctrl Pts',(11.0044482939999,11.6,2.74581154899998));
#196154=CARTESIAN_POINT('Ctrl Pts',(11.0008970699999,15.2,2.74645513199999));
#196155=CARTESIAN_POINT('Ctrl Pts',(11.0008970699999,11.6,2.74645513199999));
#196156=CARTESIAN_POINT('Ctrl Pts',(10.9973499019999,15.2,2.74709514499998));
#196157=CARTESIAN_POINT('Ctrl Pts',(10.9973499019999,11.6,2.74709514499998));
#196158=CARTESIAN_POINT('Ctrl Pts',(10.9938067979999,15.2,2.74773159199999));
#196159=CARTESIAN_POINT('Ctrl Pts',(10.9938067979999,11.6,2.74773159199999));
#196160=CARTESIAN_POINT('Ctrl Pts',(10.9902677649999,15.2,2.74836447799998));
#196161=CARTESIAN_POINT('Ctrl Pts',(10.9902677649999,11.6,2.74836447799998));
#196162=CARTESIAN_POINT('Ctrl Pts',(10.9867328139999,15.2,2.74899380799998));
#196163=CARTESIAN_POINT('Ctrl Pts',(10.9867328139999,11.6,2.74899380799998));
#196164=CARTESIAN_POINT('Ctrl Pts',(10.9832019509999,15.2,2.74961958599999));
#196165=CARTESIAN_POINT('Ctrl Pts',(10.9832019509999,11.6,2.74961958599999));
#196166=CARTESIAN_POINT('Ctrl Pts',(10.9796751869999,15.2,2.75024181699998));
#196167=CARTESIAN_POINT('Ctrl Pts',(10.9796751869999,11.6,2.75024181699998));
#196168=CARTESIAN_POINT('Ctrl Pts',(10.9761525279999,15.2,2.75086050399998));
#196169=CARTESIAN_POINT('Ctrl Pts',(10.9761525279999,11.6,2.75086050399998));
#196170=CARTESIAN_POINT('Ctrl Pts',(10.9726339839999,15.2,2.75147565399998));
#196171=CARTESIAN_POINT('Ctrl Pts',(10.9726339839999,11.6,2.75147565399998));
#196172=CARTESIAN_POINT('Ctrl Pts',(10.9691195629999,15.2,2.75208726999999));
#196173=CARTESIAN_POINT('Ctrl Pts',(10.9691195629999,11.6,2.75208726999998));
#196174=CARTESIAN_POINT('Ctrl Pts',(10.9656092739999,15.2,2.75269535799998));
#196175=CARTESIAN_POINT('Ctrl Pts',(10.9656092739999,11.6,2.75269535799998));
#196176=CARTESIAN_POINT('Ctrl Pts',(10.9621031259999,15.2,2.75329992099999));
#196177=CARTESIAN_POINT('Ctrl Pts',(10.9621031259999,11.6,2.75329992099999));
#196178=CARTESIAN_POINT('Ctrl Pts',(10.9586011259999,15.2,2.75390096599998));
#196179=CARTESIAN_POINT('Ctrl Pts',(10.9586011259999,11.6,2.75390096599998));
#196180=CARTESIAN_POINT('Ctrl Pts',(10.9551032829999,15.2,2.75449849499999));
#196181=CARTESIAN_POINT('Ctrl Pts',(10.9551032829999,11.6,2.75449849499999));
#196182=CARTESIAN_POINT('Ctrl Pts',(10.9516096059999,15.2,2.75509251399999));
#196183=CARTESIAN_POINT('Ctrl Pts',(10.9516096059999,11.6,2.75509251399999));
#196184=CARTESIAN_POINT('Ctrl Pts',(10.9481201049999,15.2,2.75568302799999));
#196185=CARTESIAN_POINT('Ctrl Pts',(10.9481201049999,11.6,2.75568302799999));
#196186=CARTESIAN_POINT('Ctrl Pts',(10.9446347859999,15.2,2.75627004099999));
#196187=CARTESIAN_POINT('Ctrl Pts',(10.9446347859999,11.6,2.75627004099999));
#196188=CARTESIAN_POINT('Ctrl Pts',(10.9411536579999,15.2,2.75685355899999));
#196189=CARTESIAN_POINT('Ctrl Pts',(10.9411536579999,11.6,2.75685355899998));
#196190=CARTESIAN_POINT('Ctrl Pts',(10.9376767319999,15.2,2.75743358499999));
#196191=CARTESIAN_POINT('Ctrl Pts',(10.9376767319999,11.6,2.75743358499999));
#196192=CARTESIAN_POINT('Ctrl Pts',(10.9342040149999,15.2,2.75801012499999));
#196193=CARTESIAN_POINT('Ctrl Pts',(10.9342040149999,11.6,2.75801012499999));
#196194=CARTESIAN_POINT('Ctrl Pts',(10.9307355149999,15.2,2.75858318399998));
#196195=CARTESIAN_POINT('Ctrl Pts',(10.9307355149999,11.6,2.75858318399998));
#196196=CARTESIAN_POINT('Ctrl Pts',(10.9272712419999,15.2,2.75915276599999));
#196197=CARTESIAN_POINT('Ctrl Pts',(10.9272712419999,11.6,2.75915276599999));
#196198=CARTESIAN_POINT('Ctrl Pts',(10.9238112039999,15.2,2.75971887599999));
#196199=CARTESIAN_POINT('Ctrl Pts',(10.9238112039999,11.6,2.75971887599999));
#196200=CARTESIAN_POINT('Ctrl Pts',(10.9203554099999,15.2,2.76028151899999));
#196201=CARTESIAN_POINT('Ctrl Pts',(10.9203554099999,11.6,2.76028151899998));
#196202=CARTESIAN_POINT('Ctrl Pts',(10.9169038679999,15.2,2.76084069999998));
#196203=CARTESIAN_POINT('Ctrl Pts',(10.9169038679999,11.6,2.76084069999998));
#196204=CARTESIAN_POINT('Ctrl Pts',(10.9134565879999,15.2,2.76139642399999));
#196205=CARTESIAN_POINT('Ctrl Pts',(10.9134565879999,11.6,2.76139642399999));
#196206=CARTESIAN_POINT('Ctrl Pts',(10.9100135769999,15.2,2.76194869599999));
#196207=CARTESIAN_POINT('Ctrl Pts',(10.9100135769999,11.6,2.76194869599998));
#196208=CARTESIAN_POINT('Ctrl Pts',(10.9065748449999,15.2,2.76249751999998));
#196209=CARTESIAN_POINT('Ctrl Pts',(10.9065748449999,11.6,2.76249751999998));
#196210=CARTESIAN_POINT('Ctrl Pts',(10.9031404009999,15.2,2.76304290199998));
#196211=CARTESIAN_POINT('Ctrl Pts',(10.9031404009999,11.6,2.76304290199998));
#196212=CARTESIAN_POINT('Ctrl Pts',(10.8997102529999,15.2,2.76358484599999));
#196213=CARTESIAN_POINT('Ctrl Pts',(10.8997102529999,11.6,2.76358484599999));
#196214=CARTESIAN_POINT('Ctrl Pts',(10.8962844109999,15.2,2.76412335799999));
#196215=CARTESIAN_POINT('Ctrl Pts',(10.8962844109999,11.6,2.76412335799999));
#196216=CARTESIAN_POINT('Ctrl Pts',(10.8928628809999,15.2,2.76465844099998));
#196217=CARTESIAN_POINT('Ctrl Pts',(10.8928628809999,11.6,2.76465844099998));
#196218=CARTESIAN_POINT('Ctrl Pts',(10.8894456749999,15.2,2.76519010299998));
#196219=CARTESIAN_POINT('Ctrl Pts',(10.8894456749999,11.6,2.76519010299998));
#196220=CARTESIAN_POINT('Ctrl Pts',(10.8860327999999,15.2,2.76571834699999));
#196221=CARTESIAN_POINT('Ctrl Pts',(10.8860327999999,11.6,2.76571834699999));
#196222=CARTESIAN_POINT('Ctrl Pts',(10.8826242649999,15.2,2.76624317899999));
#196223=CARTESIAN_POINT('Ctrl Pts',(10.8826242649999,11.6,2.76624317899999));
#196224=CARTESIAN_POINT('Ctrl Pts',(10.8792200789999,15.2,2.76676460199998));
#196225=CARTESIAN_POINT('Ctrl Pts',(10.8792200789999,11.6,2.76676460199998));
#196226=CARTESIAN_POINT('Ctrl Pts',(10.8758202519999,15.2,2.76728262299999));
#196227=CARTESIAN_POINT('Ctrl Pts',(10.8758202519999,11.6,2.76728262299999));
#196228=CARTESIAN_POINT('Ctrl Pts',(10.8724247909999,15.2,2.76779724699999));
#196229=CARTESIAN_POINT('Ctrl Pts',(10.8724247909999,11.6,2.76779724699999));
#196230=CARTESIAN_POINT('Ctrl Pts',(10.8690337059999,15.2,2.76830847799998));
#196231=CARTESIAN_POINT('Ctrl Pts',(10.8690337059999,11.6,2.76830847799998));
#196232=CARTESIAN_POINT('Ctrl Pts',(10.8656470049999,15.2,2.76881632399999));
#196233=CARTESIAN_POINT('Ctrl Pts',(10.8656470049999,11.6,2.76881632399998));
#196234=CARTESIAN_POINT('Ctrl Pts',(10.8622646979999,15.2,2.76932078499998));
#196235=CARTESIAN_POINT('Ctrl Pts',(10.8622646979999,11.6,2.76932078499998));
#196236=CARTESIAN_POINT('Ctrl Pts',(10.8588867929999,15.2,2.76982187099998));
#196237=CARTESIAN_POINT('Ctrl Pts',(10.8588867929999,11.6,2.76982187099998));
#196238=CARTESIAN_POINT('Ctrl Pts',(10.8555133009999,15.2,2.77031958499999));
#196239=CARTESIAN_POINT('Ctrl Pts',(10.8555133009999,11.6,2.77031958499998));
#196240=CARTESIAN_POINT('Ctrl Pts',(10.8521442279999,15.2,2.77081393199998));
#196241=CARTESIAN_POINT('Ctrl Pts',(10.8521442279999,11.6,2.77081393199998));
#196242=CARTESIAN_POINT('Ctrl Pts',(10.8487795839999,15.2,2.77130491799999));
#196243=CARTESIAN_POINT('Ctrl Pts',(10.8487795839999,11.6,2.77130491799999));
#196244=CARTESIAN_POINT('Ctrl Pts',(10.8454193789999,15.2,2.77179254799999));
#196245=CARTESIAN_POINT('Ctrl Pts',(10.8454193789999,11.6,2.77179254799999));
#196246=CARTESIAN_POINT('Ctrl Pts',(10.8420636209999,15.2,2.77227682699999));
#196247=CARTESIAN_POINT('Ctrl Pts',(10.8420636209999,11.6,2.77227682699999));
#196248=CARTESIAN_POINT('Ctrl Pts',(10.8387123189999,15.2,2.77275775999998));
#196249=CARTESIAN_POINT('Ctrl Pts',(10.8387123189999,11.6,2.77275775999998));
#196250=CARTESIAN_POINT('Ctrl Pts',(10.8353654819999,15.2,2.77323535299999));
#196251=CARTESIAN_POINT('Ctrl Pts',(10.8353654819999,11.6,2.77323535299998));
#196252=CARTESIAN_POINT('Ctrl Pts',(10.8320231199999,15.2,2.77370960999999));
#196253=CARTESIAN_POINT('Ctrl Pts',(10.8320231199999,11.6,2.77370960999999));
#196254=CARTESIAN_POINT('Ctrl Pts',(10.8286852409999,15.2,2.77418053799998));
#196255=CARTESIAN_POINT('Ctrl Pts',(10.8286852409999,11.6,2.77418053799998));
#196256=CARTESIAN_POINT('Ctrl Pts',(10.8253518549999,15.2,2.77464814099999));
#196257=CARTESIAN_POINT('Ctrl Pts',(10.8253518549999,11.6,2.77464814099999));
#196258=CARTESIAN_POINT('Ctrl Pts',(10.8220229679999,15.2,2.77511242599999));
#196259=CARTESIAN_POINT('Ctrl Pts',(10.8220229679999,11.6,2.77511242599999));
#196260=CARTESIAN_POINT('Ctrl Pts',(10.8186985939999,15.2,2.77557339599999));
#196261=CARTESIAN_POINT('Ctrl Pts',(10.8186985939999,11.6,2.77557339599999));
#196262=CARTESIAN_POINT('Ctrl Pts',(10.8153787389999,15.2,2.77603105699999));
#196263=CARTESIAN_POINT('Ctrl Pts',(10.8153787389999,11.6,2.77603105699999));
#196264=CARTESIAN_POINT('Ctrl Pts',(10.8120634119999,15.2,2.77648541599999));
#196265=CARTESIAN_POINT('Ctrl Pts',(10.8120634119999,11.6,2.77648541599999));
#196266=CARTESIAN_POINT('Ctrl Pts',(10.8087526239999,15.2,2.77693647799998));
#196267=CARTESIAN_POINT('Ctrl Pts',(10.8087526239999,11.6,2.77693647799998));
#196268=CARTESIAN_POINT('Ctrl Pts',(10.8054463819999,15.2,2.77738424699999));
#196269=CARTESIAN_POINT('Ctrl Pts',(10.8054463819999,11.6,2.77738424699999));
#196270=CARTESIAN_POINT('Ctrl Pts',(10.8021446959999,15.2,2.77782872899999));
#196271=CARTESIAN_POINT('Ctrl Pts',(10.8021446959999,11.6,2.77782872899999));
#196272=CARTESIAN_POINT('Ctrl Pts',(10.7988475759999,15.2,2.77826992999999));
#196273=CARTESIAN_POINT('Ctrl Pts',(10.7988475759999,11.6,2.77826992999999));
#196274=CARTESIAN_POINT('Ctrl Pts',(10.7955550299999,15.2,2.77870785499999));
#196275=CARTESIAN_POINT('Ctrl Pts',(10.7955550299999,11.6,2.77870785499999));
#196276=CARTESIAN_POINT('Ctrl Pts',(10.7922670679999,15.2,2.77914250999999));
#196277=CARTESIAN_POINT('Ctrl Pts',(10.7922670679999,11.6,2.77914250999999));
#196278=CARTESIAN_POINT('Ctrl Pts',(10.7889836979999,15.2,2.77957390099999));
#196279=CARTESIAN_POINT('Ctrl Pts',(10.7889836979999,11.6,2.77957390099999));
#196280=CARTESIAN_POINT('Ctrl Pts',(10.7857049309999,15.2,2.78000203199999));
#196281=CARTESIAN_POINT('Ctrl Pts',(10.7857049309999,11.6,2.78000203199999));
#196282=CARTESIAN_POINT('Ctrl Pts',(10.7824307749999,15.2,2.78042690799998));
#196283=CARTESIAN_POINT('Ctrl Pts',(10.7824307749999,11.6,2.78042690799998));
#196284=CARTESIAN_POINT('Ctrl Pts',(10.7791612379999,15.2,2.78084853699998));
#196285=CARTESIAN_POINT('Ctrl Pts',(10.7791612379999,11.6,2.78084853699998));
#196286=CARTESIAN_POINT('Ctrl Pts',(10.7758963329999,15.2,2.78126692399999));
#196287=CARTESIAN_POINT('Ctrl Pts',(10.7758963329999,11.6,2.78126692399999));
#196288=CARTESIAN_POINT('Ctrl Pts',(10.7726360659999,15.2,2.78168207299998));
#196289=CARTESIAN_POINT('Ctrl Pts',(10.7726360659999,11.6,2.78168207299998));
#196290=CARTESIAN_POINT('Ctrl Pts',(10.7693804469999,15.2,2.78209399099998));
#196291=CARTESIAN_POINT('Ctrl Pts',(10.7693804469999,11.6,2.78209399099998));
#196292=CARTESIAN_POINT('Ctrl Pts',(10.7661294859999,15.2,2.78250268399999));
#196293=CARTESIAN_POINT('Ctrl Pts',(10.7661294859999,11.6,2.78250268399999));
#196294=CARTESIAN_POINT('Ctrl Pts',(10.7628831919999,15.2,2.78290815599998));
#196295=CARTESIAN_POINT('Ctrl Pts',(10.7628831919999,11.6,2.78290815599998));
#196296=CARTESIAN_POINT('Ctrl Pts',(10.7596415739999,15.2,2.78331041399999));
#196297=CARTESIAN_POINT('Ctrl Pts',(10.7596415739999,11.6,2.78331041399999));
#196298=CARTESIAN_POINT('Ctrl Pts',(10.7564046409999,15.2,2.78370946299999));
#196299=CARTESIAN_POINT('Ctrl Pts',(10.7564046409999,11.6,2.78370946299999));
#196300=CARTESIAN_POINT('Ctrl Pts',(10.7531724039999,15.2,2.78410530999999));
#196301=CARTESIAN_POINT('Ctrl Pts',(10.7531724039999,11.6,2.78410530999999));
#196302=CARTESIAN_POINT('Ctrl Pts',(10.7499448709999,15.2,2.78449795899999));
#196303=CARTESIAN_POINT('Ctrl Pts',(10.7499448709999,11.6,2.78449795899998));
#196304=CARTESIAN_POINT('Ctrl Pts',(10.7467220519999,15.2,2.78488741599999));
#196305=CARTESIAN_POINT('Ctrl Pts',(10.7467220519999,11.6,2.78488741599999));
#196306=CARTESIAN_POINT('Ctrl Pts',(10.7435039549999,15.2,2.78527368799999));
#196307=CARTESIAN_POINT('Ctrl Pts',(10.7435039549999,11.6,2.78527368799998));
#196308=CARTESIAN_POINT('Ctrl Pts',(10.7402905919999,15.2,2.78565678199998));
#196309=CARTESIAN_POINT('Ctrl Pts',(10.7402905919999,11.6,2.78565678199998));
#196310=CARTESIAN_POINT('Ctrl Pts',(10.7370819699999,15.2,2.78603669899999));
#196311=CARTESIAN_POINT('Ctrl Pts',(10.7370819699999,11.6,2.78603669899999));
#196312=CARTESIAN_POINT('Ctrl Pts',(10.7338780989999,15.2,2.78641344999999));
#196313=CARTESIAN_POINT('Ctrl Pts',(10.7338780989999,11.6,2.78641344999999));
#196314=CARTESIAN_POINT('Ctrl Pts',(10.7306789899999,15.2,2.78678703799999));
#196315=CARTESIAN_POINT('Ctrl Pts',(10.7306789899999,11.6,2.78678703799999));
#196316=CARTESIAN_POINT('Ctrl Pts',(10.7274846509999,15.2,2.78715746999998));
#196317=CARTESIAN_POINT('Ctrl Pts',(10.7274846509999,11.6,2.78715746999998));
#196318=CARTESIAN_POINT('Ctrl Pts',(10.7242950909999,15.2,2.78752475099999));
#196319=CARTESIAN_POINT('Ctrl Pts',(10.7242950909999,11.6,2.78752475099999));
#196320=CARTESIAN_POINT('Ctrl Pts',(10.7211103209999,15.2,2.78788888599999));
#196321=CARTESIAN_POINT('Ctrl Pts',(10.7211103209999,11.6,2.78788888599998));
#196322=CARTESIAN_POINT('Ctrl Pts',(10.7179303499999,15.2,2.78824988399998));
#196323=CARTESIAN_POINT('Ctrl Pts',(10.7179303499999,11.6,2.78824988399998));
#196324=CARTESIAN_POINT('Ctrl Pts',(10.7147551869999,15.2,2.78860774899999));
#196325=CARTESIAN_POINT('Ctrl Pts',(10.7147551869999,11.6,2.78860774899999));
#196326=CARTESIAN_POINT('Ctrl Pts',(10.7115848429999,15.2,2.78896248699999));
#196327=CARTESIAN_POINT('Ctrl Pts',(10.7115848429999,11.6,2.78896248699999));
#196328=CARTESIAN_POINT('Ctrl Pts',(10.7084193239999,15.2,2.78931410399998));
#196329=CARTESIAN_POINT('Ctrl Pts',(10.7084193239999,11.6,2.78931410399998));
#196330=CARTESIAN_POINT('Ctrl Pts',(10.7052586439999,15.2,2.78966260699999));
#196331=CARTESIAN_POINT('Ctrl Pts',(10.7052586439999,11.6,2.78966260699998));
#196332=CARTESIAN_POINT('Ctrl Pts',(10.7021028099999,15.2,2.79000799999999));
#196333=CARTESIAN_POINT('Ctrl Pts',(10.7021028099999,11.6,2.79000799999999));
#196334=CARTESIAN_POINT('Ctrl Pts',(10.6989518329999,15.2,2.79035029099998));
#196335=CARTESIAN_POINT('Ctrl Pts',(10.6989518329999,11.6,2.79035029099998));
#196336=CARTESIAN_POINT('Ctrl Pts',(10.6958057219999,15.2,2.79068948499999));
#196337=CARTESIAN_POINT('Ctrl Pts',(10.6958057219999,11.6,2.79068948499999));
#196338=CARTESIAN_POINT('Ctrl Pts',(10.6926644859999,15.2,2.79102558999998));
#196339=CARTESIAN_POINT('Ctrl Pts',(10.6926644859999,11.6,2.79102558999998));
#196340=CARTESIAN_POINT('Ctrl Pts',(10.6895281349999,15.2,2.79135860899999));
#196341=CARTESIAN_POINT('Ctrl Pts',(10.6895281349999,11.6,2.79135860899998));
#196342=CARTESIAN_POINT('Ctrl Pts',(10.6863966799999,15.2,2.79168855099999));
#196343=CARTESIAN_POINT('Ctrl Pts',(10.6863966799999,11.6,2.79168855099999));
#196344=CARTESIAN_POINT('Ctrl Pts',(10.6832701279999,15.2,2.79201541999999));
#196345=CARTESIAN_POINT('Ctrl Pts',(10.6832701279999,11.6,2.79201541999999));
#196346=CARTESIAN_POINT('Ctrl Pts',(10.6801484919999,15.2,2.79233922399998));
#196347=CARTESIAN_POINT('Ctrl Pts',(10.6801484919999,11.6,2.79233922399998));
#196348=CARTESIAN_POINT('Ctrl Pts',(10.6770317779999,15.2,2.79265996699999));
#196349=CARTESIAN_POINT('Ctrl Pts',(10.6770317779999,11.6,2.79265996699999));
#196350=CARTESIAN_POINT('Ctrl Pts',(10.6739199989999,15.2,2.79297765699998));
#196351=CARTESIAN_POINT('Ctrl Pts',(10.6739199989999,11.6,2.79297765699998));
#196352=CARTESIAN_POINT('Ctrl Pts',(10.6708131629999,15.2,2.79329229999998));
#196353=CARTESIAN_POINT('Ctrl Pts',(10.6708131629999,11.6,2.79329229999998));
#196354=CARTESIAN_POINT('Ctrl Pts',(10.6677112809999,15.2,2.79360390199999));
#196355=CARTESIAN_POINT('Ctrl Pts',(10.6677112809999,11.6,2.79360390199999));
#196356=CARTESIAN_POINT('Ctrl Pts',(10.6646143609999,15.2,2.79391246899999));
#196357=CARTESIAN_POINT('Ctrl Pts',(10.6646143609999,11.6,2.79391246899999));
#196358=CARTESIAN_POINT('Ctrl Pts',(10.6615224159999,15.2,2.79421800799999));
#196359=CARTESIAN_POINT('Ctrl Pts',(10.6615224159999,11.6,2.79421800799999));
#196360=CARTESIAN_POINT('Ctrl Pts',(10.6584354509999,15.2,2.79452052399999));
#196361=CARTESIAN_POINT('Ctrl Pts',(10.6584354509999,11.6,2.79452052399999));
#196362=CARTESIAN_POINT('Ctrl Pts',(10.6553534799999,15.2,2.79482002499999));
#196363=CARTESIAN_POINT('Ctrl Pts',(10.6553534799999,11.6,2.79482002499999));
#196364=CARTESIAN_POINT('Ctrl Pts',(10.6522765109999,15.2,2.79511651699998));
#196365=CARTESIAN_POINT('Ctrl Pts',(10.6522765109999,11.6,2.79511651699998));
#196366=CARTESIAN_POINT('Ctrl Pts',(10.6492045549999,15.2,2.79541000599998));
#196367=CARTESIAN_POINT('Ctrl Pts',(10.6492045549999,11.6,2.79541000599998));
#196368=CARTESIAN_POINT('Ctrl Pts',(10.6461376199999,15.2,2.79570049699998));
#196369=CARTESIAN_POINT('Ctrl Pts',(10.6461376199999,11.6,2.79570049699998));
#196370=CARTESIAN_POINT('Ctrl Pts',(10.6430757179999,15.2,2.79598799899999));
#196371=CARTESIAN_POINT('Ctrl Pts',(10.6430757179999,11.6,2.79598799899999));
#196372=CARTESIAN_POINT('Ctrl Pts',(10.6400188569999,15.2,2.79627251799998));
#196373=CARTESIAN_POINT('Ctrl Pts',(10.6400188569999,11.6,2.79627251799998));
#196374=CARTESIAN_POINT('Ctrl Pts',(10.6369670479999,15.2,2.79655405899998));
#196375=CARTESIAN_POINT('Ctrl Pts',(10.6369670479999,11.6,2.79655405899998));
#196376=CARTESIAN_POINT('Ctrl Pts',(10.6339203009999,15.2,2.79683262899999));
#196377=CARTESIAN_POINT('Ctrl Pts',(10.6339203009999,11.6,2.79683262899999));
#196378=CARTESIAN_POINT('Ctrl Pts',(10.6308786259999,15.2,2.79710823499999));
#196379=CARTESIAN_POINT('Ctrl Pts',(10.6308786259999,11.6,2.79710823499998));
#196380=CARTESIAN_POINT('Ctrl Pts',(10.6278420329999,15.2,2.79738088399998));
#196381=CARTESIAN_POINT('Ctrl Pts',(10.6278420329999,11.6,2.79738088399998));
#196382=CARTESIAN_POINT('Ctrl Pts',(10.6248105309999,15.2,2.79765058099999));
#196383=CARTESIAN_POINT('Ctrl Pts',(10.6248105309999,11.6,2.79765058099999));
#196384=CARTESIAN_POINT('Ctrl Pts',(10.6217841319999,15.2,2.79791733399998));
#196385=CARTESIAN_POINT('Ctrl Pts',(10.6217841319999,11.6,2.79791733399998));
#196386=CARTESIAN_POINT('Ctrl Pts',(10.6187628439999,15.2,2.79818114899999));
#196387=CARTESIAN_POINT('Ctrl Pts',(10.6187628439999,11.6,2.79818114899999));
#196388=CARTESIAN_POINT('Ctrl Pts',(10.6157466779999,15.2,2.79844203299999));
#196389=CARTESIAN_POINT('Ctrl Pts',(10.6157466779999,11.6,2.79844203299999));
#196390=CARTESIAN_POINT('Ctrl Pts',(10.6127356429999,15.2,2.79869999199998));
#196391=CARTESIAN_POINT('Ctrl Pts',(10.6127356429999,11.6,2.79869999199998));
#196392=CARTESIAN_POINT('Ctrl Pts',(10.6097297519999,15.2,2.79895503299999));
#196393=CARTESIAN_POINT('Ctrl Pts',(10.6097297519999,11.6,2.79895503299999));
#196394=CARTESIAN_POINT('Ctrl Pts',(10.6067290119999,15.2,2.79920716299999));
#196395=CARTESIAN_POINT('Ctrl Pts',(10.6067290119999,11.6,2.79920716299999));
#196396=CARTESIAN_POINT('Ctrl Pts',(10.6037334349999,15.2,2.79945638899999));
#196397=CARTESIAN_POINT('Ctrl Pts',(10.6037334349999,11.6,2.79945638899999));
#196398=CARTESIAN_POINT('Ctrl Pts',(10.6007430289999,15.2,2.79970271699998));
#196399=CARTESIAN_POINT('Ctrl Pts',(10.6007430289999,11.6,2.79970271699998));
#196400=CARTESIAN_POINT('Ctrl Pts',(10.5977578069999,15.2,2.79994615399998));
#196401=CARTESIAN_POINT('Ctrl Pts',(10.5977578069999,11.6,2.79994615399998));
#196402=CARTESIAN_POINT('Ctrl Pts',(10.5947777769999,15.2,2.80018670699998));
#196403=CARTESIAN_POINT('Ctrl Pts',(10.5947777769999,11.6,2.80018670699998));
#196404=CARTESIAN_POINT('Ctrl Pts',(10.5918029509999,15.2,2.80042438199998));
#196405=CARTESIAN_POINT('Ctrl Pts',(10.5918029509999,11.6,2.80042438199998));
#196406=CARTESIAN_POINT('Ctrl Pts',(10.5888333369999,15.2,2.80065918699999));
#196407=CARTESIAN_POINT('Ctrl Pts',(10.5888333369999,11.6,2.80065918699999));
#196408=CARTESIAN_POINT('Ctrl Pts',(10.5858689469999,15.2,2.80089112799998));
#196409=CARTESIAN_POINT('Ctrl Pts',(10.5858689469999,11.6,2.80089112799998));
#196410=CARTESIAN_POINT('Ctrl Pts',(10.5829097899999,15.2,2.80112021299999));
#196411=CARTESIAN_POINT('Ctrl Pts',(10.5829097899999,11.6,2.80112021299999));
#196412=CARTESIAN_POINT('Ctrl Pts',(10.5799558779999,15.2,2.80134644699999));
#196413=CARTESIAN_POINT('Ctrl Pts',(10.5799558779999,11.6,2.80134644699999));
#196414=CARTESIAN_POINT('Ctrl Pts',(10.5770072199999,15.2,2.80156983799999));
#196415=CARTESIAN_POINT('Ctrl Pts',(10.5770072199999,11.6,2.80156983799999));
#196416=CARTESIAN_POINT('Ctrl Pts',(10.5740638259999,15.2,2.80179039399999));
#196417=CARTESIAN_POINT('Ctrl Pts',(10.5740638259999,11.6,2.80179039399999));
#196418=CARTESIAN_POINT('Ctrl Pts',(10.5711257059999,15.2,2.80200812099999));
#196419=CARTESIAN_POINT('Ctrl Pts',(10.5711257059999,11.6,2.80200812099999));
#196420=CARTESIAN_POINT('Ctrl Pts',(10.5681928729999,15.2,2.80222302499999));
#196421=CARTESIAN_POINT('Ctrl Pts',(10.5681928729999,11.6,2.80222302499999));
#196422=CARTESIAN_POINT('Ctrl Pts',(10.5652653349999,15.2,2.80243511499998));
#196423=CARTESIAN_POINT('Ctrl Pts',(10.5652653349999,11.6,2.80243511499998));
#196424=CARTESIAN_POINT('Ctrl Pts',(10.5623431029999,15.2,2.80264439699998));
#196425=CARTESIAN_POINT('Ctrl Pts',(10.5623431029999,11.6,2.80264439699998));
#196426=CARTESIAN_POINT('Ctrl Pts',(10.5594261859999,15.2,2.80285087799999));
#196427=CARTESIAN_POINT('Ctrl Pts',(10.5594261859999,11.6,2.80285087799999));
#196428=CARTESIAN_POINT('Ctrl Pts',(10.5565145969999,15.2,2.80305456499998));
#196429=CARTESIAN_POINT('Ctrl Pts',(10.5565145969999,11.6,2.80305456499998));
#196430=CARTESIAN_POINT('Ctrl Pts',(10.5536083449999,15.2,2.80325546599999));
#196431=CARTESIAN_POINT('Ctrl Pts',(10.5536083449999,11.6,2.80325546599998));
#196432=CARTESIAN_POINT('Ctrl Pts',(10.5507074409999,15.2,2.80345358699999));
#196433=CARTESIAN_POINT('Ctrl Pts',(10.5507074409999,11.6,2.80345358699999));
#196434=CARTESIAN_POINT('Ctrl Pts',(10.5478118939999,15.2,2.80364893599998));
#196435=CARTESIAN_POINT('Ctrl Pts',(10.5478118939999,11.6,2.80364893599998));
#196436=CARTESIAN_POINT('Ctrl Pts',(10.5449217159999,15.2,2.80384151899998));
#196437=CARTESIAN_POINT('Ctrl Pts',(10.5449217159999,11.6,2.80384151899998));
#196438=CARTESIAN_POINT('Ctrl Pts',(10.5420369179999,15.2,2.80403134499998));
#196439=CARTESIAN_POINT('Ctrl Pts',(10.5420369179999,11.6,2.80403134499998));
#196440=CARTESIAN_POINT('Ctrl Pts',(10.5391575079999,15.2,2.80421842099998));
#196441=CARTESIAN_POINT('Ctrl Pts',(10.5391575079999,11.6,2.80421842099998));
#196442=CARTESIAN_POINT('Ctrl Pts',(10.5362834999999,15.2,2.80440275299998));
#196443=CARTESIAN_POINT('Ctrl Pts',(10.5362834999999,11.6,2.80440275299998));
#196444=CARTESIAN_POINT('Ctrl Pts',(10.5334149019999,15.2,2.80458434899998));
#196445=CARTESIAN_POINT('Ctrl Pts',(10.5334149019999,11.6,2.80458434899998));
#196446=CARTESIAN_POINT('Ctrl Pts',(10.5305517249999,15.2,2.80476321599998));
#196447=CARTESIAN_POINT('Ctrl Pts',(10.5305517249999,11.6,2.80476321599998));
#196448=CARTESIAN_POINT('Ctrl Pts',(10.5276939799999,15.2,2.80493936099998));
#196449=CARTESIAN_POINT('Ctrl Pts',(10.5276939799999,11.6,2.80493936099998));
#196450=CARTESIAN_POINT('Ctrl Pts',(10.5248416769999,15.2,2.80511279299999));
#196451=CARTESIAN_POINT('Ctrl Pts',(10.5248416769999,11.6,2.80511279299999));
#196452=CARTESIAN_POINT('Ctrl Pts',(10.5219948289999,15.2,2.80528351899999));
#196453=CARTESIAN_POINT('Ctrl Pts',(10.5219948289999,11.6,2.80528351899999));
#196454=CARTESIAN_POINT('Ctrl Pts',(10.5191534429999,15.2,2.80545154499999));
#196455=CARTESIAN_POINT('Ctrl Pts',(10.5191534429999,11.6,2.80545154499999));
#196456=CARTESIAN_POINT('Ctrl Pts',(10.5163175329999,15.2,2.80561687899999));
#196457=CARTESIAN_POINT('Ctrl Pts',(10.5163175329999,11.6,2.80561687899999));
#196458=CARTESIAN_POINT('Ctrl Pts',(10.5134871079999,15.2,2.80577952899999));
#196459=CARTESIAN_POINT('Ctrl Pts',(10.5134871079999,11.6,2.80577952899998));
#196460=CARTESIAN_POINT('Ctrl Pts',(10.5106621789999,15.2,2.80593950299998));
#196461=CARTESIAN_POINT('Ctrl Pts',(10.5106621789999,11.6,2.80593950299998));
#196462=CARTESIAN_POINT('Ctrl Pts',(10.5078427569999,15.2,2.80609680699998));
#196463=CARTESIAN_POINT('Ctrl Pts',(10.5078427569999,11.6,2.80609680699998));
#196464=CARTESIAN_POINT('Ctrl Pts',(10.5050288509999,15.2,2.80625144999998));
#196465=CARTESIAN_POINT('Ctrl Pts',(10.5050288509999,11.6,2.80625144999998));
#196466=CARTESIAN_POINT('Ctrl Pts',(10.5022204749999,15.2,2.80640343899999));
#196467=CARTESIAN_POINT('Ctrl Pts',(10.5022204749999,11.6,2.80640343899999));
#196468=CARTESIAN_POINT('Ctrl Pts',(10.4994176369999,15.2,2.80655278099999));
#196469=CARTESIAN_POINT('Ctrl Pts',(10.4994176369999,11.6,2.80655278099999));
#196470=CARTESIAN_POINT('Ctrl Pts',(10.4966203499999,15.2,2.80669948499998));
#196471=CARTESIAN_POINT('Ctrl Pts',(10.4966203499999,11.6,2.80669948499998));
#196472=CARTESIAN_POINT('Ctrl Pts',(10.4938286229999,15.2,2.80684355699999));
#196473=CARTESIAN_POINT('Ctrl Pts',(10.4938286229999,11.6,2.80684355699999));
#196474=CARTESIAN_POINT('Ctrl Pts',(10.4910424679999,15.2,2.80698500599998));
#196475=CARTESIAN_POINT('Ctrl Pts',(10.4910424679999,11.6,2.80698500599998));
#196476=CARTESIAN_POINT('Ctrl Pts',(10.4882618969999,15.2,2.80712383899999));
#196477=CARTESIAN_POINT('Ctrl Pts',(10.4882618969999,11.6,2.80712383899999));
#196478=CARTESIAN_POINT('Ctrl Pts',(10.4854869179999,15.2,2.80726006499999));
#196479=CARTESIAN_POINT('Ctrl Pts',(10.4854869179999,11.6,2.80726006499999));
#196480=CARTESIAN_POINT('Ctrl Pts',(10.4827175439999,15.2,2.80739368999999));
#196481=CARTESIAN_POINT('Ctrl Pts',(10.4827175439999,11.6,2.80739368999999));
#196482=CARTESIAN_POINT('Ctrl Pts',(10.4799537849999,15.2,2.80752472299999));
#196483=CARTESIAN_POINT('Ctrl Pts',(10.4799537849999,11.6,2.80752472299999));
#196484=CARTESIAN_POINT('Ctrl Pts',(10.4771956519999,15.2,2.80765317099998));
#196485=CARTESIAN_POINT('Ctrl Pts',(10.4771956519999,11.6,2.80765317099998));
#196486=CARTESIAN_POINT('Ctrl Pts',(10.4744431569999,15.2,2.80777904299998));
#196487=CARTESIAN_POINT('Ctrl Pts',(10.4744431569999,11.6,2.80777904299998));
#196488=CARTESIAN_POINT('Ctrl Pts',(10.4716963109999,15.2,2.80790234499998));
#196489=CARTESIAN_POINT('Ctrl Pts',(10.4716963109999,11.6,2.80790234499998));
#196490=CARTESIAN_POINT('Ctrl Pts',(10.4689551229999,15.2,2.80802308599998));
#196491=CARTESIAN_POINT('Ctrl Pts',(10.4689551229999,11.6,2.80802308599998));
#196492=CARTESIAN_POINT('Ctrl Pts',(10.4662196059999,15.2,2.80814127499998));
#196493=CARTESIAN_POINT('Ctrl Pts',(10.4662196059999,11.6,2.80814127499998));
#196494=CARTESIAN_POINT('Ctrl Pts',(10.4634897709999,15.2,2.80825691999999));
#196495=CARTESIAN_POINT('Ctrl Pts',(10.4634897709999,11.6,2.80825691999999));
#196496=CARTESIAN_POINT('Ctrl Pts',(10.4607656289999,15.2,2.80837002599998));
#196497=CARTESIAN_POINT('Ctrl Pts',(10.4607656289999,11.6,2.80837002599998));
#196498=CARTESIAN_POINT('Ctrl Pts',(10.4580471909999,15.2,2.80848060399999));
#196499=CARTESIAN_POINT('Ctrl Pts',(10.4580471909999,11.6,2.80848060399999));
#196500=CARTESIAN_POINT('Ctrl Pts',(10.4553344669999,15.2,2.80858866099998));
#196501=CARTESIAN_POINT('Ctrl Pts',(10.4553344669999,11.6,2.80858866099998));
#196502=CARTESIAN_POINT('Ctrl Pts',(10.4526274699999,15.2,2.80869420399998));
#196503=CARTESIAN_POINT('Ctrl Pts',(10.4526274699999,11.6,2.80869420399998));
#196504=CARTESIAN_POINT('Ctrl Pts',(10.4499262109999,15.2,2.80879724399998));
#196505=CARTESIAN_POINT('Ctrl Pts',(10.4499262109999,11.6,2.80879724399998));
#196506=CARTESIAN_POINT('Ctrl Pts',(10.4472306989999,15.2,2.80889778599998));
#196507=CARTESIAN_POINT('Ctrl Pts',(10.4472306989999,11.6,2.80889778599998));
#196508=CARTESIAN_POINT('Ctrl Pts',(10.4445409479999,15.2,2.80899584099998));
#196509=CARTESIAN_POINT('Ctrl Pts',(10.4445409479999,11.6,2.80899584099998));
#196510=CARTESIAN_POINT('Ctrl Pts',(10.4418569669999,15.2,2.80909141499999));
#196511=CARTESIAN_POINT('Ctrl Pts',(10.4418569669999,11.6,2.80909141499999));
#196512=CARTESIAN_POINT('Ctrl Pts',(10.4391787699999,15.2,2.80918451599998));
#196513=CARTESIAN_POINT('Ctrl Pts',(10.4391787699999,11.6,2.80918451599998));
#196514=CARTESIAN_POINT('Ctrl Pts',(10.4365063659999,15.2,2.80927515599998));
#196515=CARTESIAN_POINT('Ctrl Pts',(10.4365063659999,11.6,2.80927515599998));
#196516=CARTESIAN_POINT('Ctrl Pts',(10.4338397659999,15.2,2.80936333799998));
#196517=CARTESIAN_POINT('Ctrl Pts',(10.4338397659999,11.6,2.80936333799998));
#196518=CARTESIAN_POINT('Ctrl Pts',(10.4311789839999,15.2,2.80944907299999));
#196519=CARTESIAN_POINT('Ctrl Pts',(10.4311789839999,11.6,2.80944907299999));
#196520=CARTESIAN_POINT('Ctrl Pts',(10.4285240289999,15.2,2.80953237099999));
#196521=CARTESIAN_POINT('Ctrl Pts',(10.4285240289999,11.6,2.80953237099998));
#196522=CARTESIAN_POINT('Ctrl Pts',(10.4258749129999,15.2,2.80961323599998));
#196523=CARTESIAN_POINT('Ctrl Pts',(10.4258749129999,11.6,2.80961323599998));
#196524=CARTESIAN_POINT('Ctrl Pts',(10.4232316479999,15.2,2.80969167999999));
#196525=CARTESIAN_POINT('Ctrl Pts',(10.4232316479999,11.6,2.80969167999999));
#196526=CARTESIAN_POINT('Ctrl Pts',(10.4205942449999,15.2,2.80976771199998));
#196527=CARTESIAN_POINT('Ctrl Pts',(10.4205942449999,11.6,2.80976771199998));
#196528=CARTESIAN_POINT('Ctrl Pts',(10.4179627159999,15.2,2.80984133699998));
#196529=CARTESIAN_POINT('Ctrl Pts',(10.4179627159999,11.6,2.80984133699998));
#196530=CARTESIAN_POINT('Ctrl Pts',(10.4153370719999,15.2,2.80991256599999));
#196531=CARTESIAN_POINT('Ctrl Pts',(10.4153370719999,11.6,2.80991256599999));
#196532=CARTESIAN_POINT('Ctrl Pts',(10.4127173239999,15.2,2.80998140599999));
#196533=CARTESIAN_POINT('Ctrl Pts',(10.4127173239999,11.6,2.80998140599999));
#196534=CARTESIAN_POINT('Ctrl Pts',(10.4101034849999,15.2,2.81004786799999));
#196535=CARTESIAN_POINT('Ctrl Pts',(10.4101034849999,11.6,2.81004786799999));
#196536=CARTESIAN_POINT('Ctrl Pts',(10.4074955649999,15.2,2.81011195799999));
#196537=CARTESIAN_POINT('Ctrl Pts',(10.4074955649999,11.6,2.81011195799999));
#196538=CARTESIAN_POINT('Ctrl Pts',(10.4048935769999,15.2,2.81017368599999));
#196539=CARTESIAN_POINT('Ctrl Pts',(10.4048935769999,11.6,2.81017368599999));
#196540=CARTESIAN_POINT('Ctrl Pts',(10.4022975309999,15.2,2.81023305999998));
#196541=CARTESIAN_POINT('Ctrl Pts',(10.4022975309999,11.6,2.81023305999998));
#196542=CARTESIAN_POINT('Ctrl Pts',(10.3997074399999,15.2,2.81029008999998));
#196543=CARTESIAN_POINT('Ctrl Pts',(10.3997074399999,11.6,2.81029008999998));
#196544=CARTESIAN_POINT('Ctrl Pts',(10.3971233149999,15.2,2.81034478199999));
#196545=CARTESIAN_POINT('Ctrl Pts',(10.3971233149999,11.6,2.81034478199999));
#196546=CARTESIAN_POINT('Ctrl Pts',(10.3945451689999,15.2,2.81039714699999));
#196547=CARTESIAN_POINT('Ctrl Pts',(10.3945451689999,11.6,2.81039714699999));
#196548=CARTESIAN_POINT('Ctrl Pts',(10.3919730119999,15.2,2.81044719399999));
#196549=CARTESIAN_POINT('Ctrl Pts',(10.3919730119999,11.6,2.81044719399999));
#196550=CARTESIAN_POINT('Ctrl Pts',(10.3894068559999,15.2,2.81049492999998));
#196551=CARTESIAN_POINT('Ctrl Pts',(10.3894068559999,11.6,2.81049492999998));
#196552=CARTESIAN_POINT('Ctrl Pts',(10.3868467139999,15.2,2.81054036599999));
#196553=CARTESIAN_POINT('Ctrl Pts',(10.3868467139999,11.6,2.81054036599999));
#196554=CARTESIAN_POINT('Ctrl Pts',(10.3842925959999,15.2,2.81058350899999));
#196555=CARTESIAN_POINT('Ctrl Pts',(10.3842925959999,11.6,2.81058350899999));
#196556=CARTESIAN_POINT('Ctrl Pts',(10.3817445159999,15.2,2.81062436799999));
#196557=CARTESIAN_POINT('Ctrl Pts',(10.3817445159999,11.6,2.81062436799999));
#196558=CARTESIAN_POINT('Ctrl Pts',(10.3792024839999,15.2,2.81066295399999));
#196559=CARTESIAN_POINT('Ctrl Pts',(10.3792024839999,11.6,2.81066295399999));
#196560=CARTESIAN_POINT('Ctrl Pts',(10.3766665119999,15.2,2.81069927299999));
#196561=CARTESIAN_POINT('Ctrl Pts',(10.3766665119999,11.6,2.81069927299999));
#196562=CARTESIAN_POINT('Ctrl Pts',(10.3741366129999,15.2,2.81073333699998));
#196563=CARTESIAN_POINT('Ctrl Pts',(10.3741366129999,11.6,2.81073333699998));
#196564=CARTESIAN_POINT('Ctrl Pts',(10.3716127979999,15.2,2.81076515299999));
#196565=CARTESIAN_POINT('Ctrl Pts',(10.3716127979999,11.6,2.81076515299999));
#196566=CARTESIAN_POINT('Ctrl Pts',(10.3690950799999,15.2,2.81079473099999));
#196567=CARTESIAN_POINT('Ctrl Pts',(10.3690950799999,11.6,2.81079473099999));
#196568=CARTESIAN_POINT('Ctrl Pts',(10.3665834699999,15.2,2.81082207899999));
#196569=CARTESIAN_POINT('Ctrl Pts',(10.3665834699999,11.6,2.81082207899999));
#196570=CARTESIAN_POINT('Ctrl Pts',(10.3640779799999,15.2,2.81084720699998));
#196571=CARTESIAN_POINT('Ctrl Pts',(10.3640779799999,11.6,2.81084720699998));
#196572=CARTESIAN_POINT('Ctrl Pts',(10.3615786239999,15.2,2.81087012399999));
#196573=CARTESIAN_POINT('Ctrl Pts',(10.3615786239999,11.6,2.81087012399999));
#196574=CARTESIAN_POINT('Ctrl Pts',(10.3590854099999,15.2,2.81089083999999));
#196575=CARTESIAN_POINT('Ctrl Pts',(10.3590854099999,11.6,2.81089083999999));
#196576=CARTESIAN_POINT('Ctrl Pts',(10.3565983529999,15.2,2.81090936199998));
#196577=CARTESIAN_POINT('Ctrl Pts',(10.3565983529999,11.6,2.81090936199998));
#196578=CARTESIAN_POINT('Ctrl Pts',(10.3541174659999,15.2,2.81092570199998));
#196579=CARTESIAN_POINT('Ctrl Pts',(10.3541174659999,11.6,2.81092570199998));
#196580=CARTESIAN_POINT('Ctrl Pts',(10.3516427589999,15.2,2.81093986799998));
#196581=CARTESIAN_POINT('Ctrl Pts',(10.3516427589999,11.6,2.81093986799998));
#196582=CARTESIAN_POINT('Ctrl Pts',(10.3491742439999,15.2,2.81095186899999));
#196583=CARTESIAN_POINT('Ctrl Pts',(10.3491742439999,11.6,2.81095186899999));
#196584=CARTESIAN_POINT('Ctrl Pts',(10.3467119339999,15.2,2.81096171499998));
#196585=CARTESIAN_POINT('Ctrl Pts',(10.3467119339999,11.6,2.81096171499998));
#196586=CARTESIAN_POINT('Ctrl Pts',(10.3442558419999,15.2,2.81096941599999));
#196587=CARTESIAN_POINT('Ctrl Pts',(10.3442558419999,11.6,2.81096941599999));
#196588=CARTESIAN_POINT('Ctrl Pts',(10.3418059809999,15.2,2.81097497899999));
#196589=CARTESIAN_POINT('Ctrl Pts',(10.3418059809999,11.6,2.81097497899999));
#196590=CARTESIAN_POINT('Ctrl Pts',(10.3393623599999,15.2,2.81097841599999));
#196591=CARTESIAN_POINT('Ctrl Pts',(10.3393623599999,11.6,2.81097841599998));
#196592=CARTESIAN_POINT('Ctrl Pts',(10.3369249929999,15.2,2.81097973599999));
#196593=CARTESIAN_POINT('Ctrl Pts',(10.3369249929999,11.6,2.81097973599999));
#196594=CARTESIAN_POINT('Ctrl Pts',(10.3344938929999,15.2,2.81097894699998));
#196595=CARTESIAN_POINT('Ctrl Pts',(10.3344938929999,11.6,2.81097894699998));
#196596=CARTESIAN_POINT('Ctrl Pts',(10.3320690709999,15.2,2.81097606099999));
#196597=CARTESIAN_POINT('Ctrl Pts',(10.3320690709999,11.6,2.81097606099999));
#196598=CARTESIAN_POINT('Ctrl Pts',(10.3296505419999,15.2,2.81097108499999));
#196599=CARTESIAN_POINT('Ctrl Pts',(10.3296505419999,11.6,2.81097108499999));
#196600=CARTESIAN_POINT('Ctrl Pts',(10.3272383149999,15.2,2.81096403199999));
#196601=CARTESIAN_POINT('Ctrl Pts',(10.3272383149999,11.6,2.81096403199999));
#196602=CARTESIAN_POINT('Ctrl Pts',(10.3248324049999,15.2,2.81095490799999));
#196603=CARTESIAN_POINT('Ctrl Pts',(10.3248324049999,11.6,2.81095490799998));
#196604=CARTESIAN_POINT('Ctrl Pts',(10.3224328229999,15.2,2.81094372499999));
#196605=CARTESIAN_POINT('Ctrl Pts',(10.3224328229999,11.6,2.81094372499999));
#196606=CARTESIAN_POINT('Ctrl Pts',(10.3200395829999,15.2,2.81093049299999));
#196607=CARTESIAN_POINT('Ctrl Pts',(10.3200395829999,11.6,2.81093049299999));
#196608=CARTESIAN_POINT('Ctrl Pts',(10.3176526949999,15.2,2.81091521999999));
#196609=CARTESIAN_POINT('Ctrl Pts',(10.3176526949999,11.6,2.81091521999999));
#196610=CARTESIAN_POINT('Ctrl Pts',(10.3152721739999,15.2,2.81089791699999));
#196611=CARTESIAN_POINT('Ctrl Pts',(10.3152721739999,11.6,2.81089791699999));
#196612=CARTESIAN_POINT('Ctrl Pts',(10.3128980319999,15.2,2.81087859499999));
#196613=CARTESIAN_POINT('Ctrl Pts',(10.3128980319999,11.6,2.81087859499999));
#196614=CARTESIAN_POINT('Ctrl Pts',(10.3105302809999,15.2,2.81085726199999));
#196615=CARTESIAN_POINT('Ctrl Pts',(10.3105302809999,11.6,2.81085726199999));
#196616=CARTESIAN_POINT('Ctrl Pts',(10.3081689339999,15.2,2.81083392699998));
#196617=CARTESIAN_POINT('Ctrl Pts',(10.3081689339999,11.6,2.81083392699998));
#196618=CARTESIAN_POINT('Ctrl Pts',(10.3058140039999,15.2,2.81080860299999));
#196619=CARTESIAN_POINT('Ctrl Pts',(10.3058140039999,11.6,2.81080860299999));
#196620=CARTESIAN_POINT('Ctrl Pts',(10.3034655029999,15.2,2.81078129899999));
#196621=CARTESIAN_POINT('Ctrl Pts',(10.3034655029999,11.6,2.81078129899999));
#196622=CARTESIAN_POINT('Ctrl Pts',(10.3011234449999,15.2,2.81075202499999));
#196623=CARTESIAN_POINT('Ctrl Pts',(10.3011234449999,11.6,2.81075202499998));
#196624=CARTESIAN_POINT('Ctrl Pts',(10.2987878399999,15.2,2.81072078899999));
#196625=CARTESIAN_POINT('Ctrl Pts',(10.2987878399999,11.6,2.81072078899999));
#196626=CARTESIAN_POINT('Ctrl Pts',(10.2964587039999,15.2,2.81068760399998));
#196627=CARTESIAN_POINT('Ctrl Pts',(10.2964587039999,11.6,2.81068760399998));
#196628=CARTESIAN_POINT('Ctrl Pts',(10.2941360499999,15.2,2.81065247899999));
#196629=CARTESIAN_POINT('Ctrl Pts',(10.2941360499999,11.6,2.81065247899999));
#196630=CARTESIAN_POINT('Ctrl Pts',(10.2918198869999,15.2,2.81061542499998));
#196631=CARTESIAN_POINT('Ctrl Pts',(10.2918198869999,11.6,2.81061542499998));
#196632=CARTESIAN_POINT('Ctrl Pts',(10.2895102319999,15.2,2.81057645199999));
#196633=CARTESIAN_POINT('Ctrl Pts',(10.2895102319999,11.6,2.81057645199999));
#196634=CARTESIAN_POINT('Ctrl Pts',(10.2872070959999,15.2,2.81053556799999));
#196635=CARTESIAN_POINT('Ctrl Pts',(10.2872070959999,11.6,2.81053556799999));
#196636=CARTESIAN_POINT('Ctrl Pts',(10.2849104899999,15.2,2.81049278699999));
#196637=CARTESIAN_POINT('Ctrl Pts',(10.2849104899999,11.6,2.81049278699999));
#196638=CARTESIAN_POINT('Ctrl Pts',(10.2826204319999,15.2,2.81044811699999));
#196639=CARTESIAN_POINT('Ctrl Pts',(10.2826204319999,11.6,2.81044811699999));
#196640=CARTESIAN_POINT('Ctrl Pts',(10.2803369309999,15.2,2.81040156799998));
#196641=CARTESIAN_POINT('Ctrl Pts',(10.2803369309999,11.6,2.81040156799998));
#196642=CARTESIAN_POINT('Ctrl Pts',(10.2780600009999,15.2,2.81035315199999));
#196643=CARTESIAN_POINT('Ctrl Pts',(10.2780600009999,11.6,2.81035315199999));
#196644=CARTESIAN_POINT('Ctrl Pts',(10.2757896559999,15.2,2.81030288099998));
#196645=CARTESIAN_POINT('Ctrl Pts',(10.2757896559999,11.6,2.81030288099998));
#196646=CARTESIAN_POINT('Ctrl Pts',(10.2735259089999,15.2,2.81025076199998));
#196647=CARTESIAN_POINT('Ctrl Pts',(10.2735259089999,11.6,2.81025076199998));
#196648=CARTESIAN_POINT('Ctrl Pts',(10.2712687709999,15.2,2.81019680599999));
#196649=CARTESIAN_POINT('Ctrl Pts',(10.2712687709999,11.6,2.81019680599999));
#196650=CARTESIAN_POINT('Ctrl Pts',(10.2690182579999,15.2,2.81014102599999));
#196651=CARTESIAN_POINT('Ctrl Pts',(10.2690182579999,11.6,2.81014102599999));
#196652=CARTESIAN_POINT('Ctrl Pts',(10.2667743819999,15.2,2.81008343199999));
#196653=CARTESIAN_POINT('Ctrl Pts',(10.2667743819999,11.6,2.81008343199999));
#196654=CARTESIAN_POINT('Ctrl Pts',(10.2645371559999,15.2,2.81002403399999));
#196655=CARTESIAN_POINT('Ctrl Pts',(10.2645371559999,11.6,2.81002403399999));
#196656=CARTESIAN_POINT('Ctrl Pts',(10.2623065929999,15.2,2.80996284199999));
#196657=CARTESIAN_POINT('Ctrl Pts',(10.2623065929999,11.6,2.80996284199999));
#196658=CARTESIAN_POINT('Ctrl Pts',(10.2600827069999,15.2,2.80989986699999));
#196659=CARTESIAN_POINT('Ctrl Pts',(10.2600827069999,11.6,2.80989986699998));
#196660=CARTESIAN_POINT('Ctrl Pts',(10.2578655119999,15.2,2.80983512099999));
#196661=CARTESIAN_POINT('Ctrl Pts',(10.2578655119999,11.6,2.80983512099999));
#196662=CARTESIAN_POINT('Ctrl Pts',(10.2556550209999,15.2,2.80976861599999));
#196663=CARTESIAN_POINT('Ctrl Pts',(10.2556550209999,11.6,2.80976861599999));
#196664=CARTESIAN_POINT('Ctrl Pts',(10.2534512459999,15.2,2.80970035899998));
#196665=CARTESIAN_POINT('Ctrl Pts',(10.2534512459999,11.6,2.80970035899998));
#196666=CARTESIAN_POINT('Ctrl Pts',(10.2512542019999,15.2,2.80963036499998));
#196667=CARTESIAN_POINT('Ctrl Pts',(10.2512542019999,11.6,2.80963036499998));
#196668=CARTESIAN_POINT('Ctrl Pts',(10.2490639019999,15.2,2.80955864199999));
#196669=CARTESIAN_POINT('Ctrl Pts',(10.2490639019999,11.6,2.80955864199999));
#196670=CARTESIAN_POINT('Ctrl Pts',(10.2468803589999,15.2,2.80948520299999));
#196671=CARTESIAN_POINT('Ctrl Pts',(10.2468803589999,11.6,2.80948520299999));
#196672=CARTESIAN_POINT('Ctrl Pts',(10.2447035879999,15.2,2.80941005799999));
#196673=CARTESIAN_POINT('Ctrl Pts',(10.2447035879999,11.6,2.80941005799999));
#196674=CARTESIAN_POINT('Ctrl Pts',(10.2425335999999,15.2,2.80933321799999));
#196675=CARTESIAN_POINT('Ctrl Pts',(10.2425335999999,11.6,2.80933321799999));
#196676=CARTESIAN_POINT('Ctrl Pts',(10.2403704109999,15.2,2.80925469399998));
#196677=CARTESIAN_POINT('Ctrl Pts',(10.2403704109999,11.6,2.80925469399998));
#196678=CARTESIAN_POINT('Ctrl Pts',(10.2382140349999,15.2,2.80917449999999));
#196679=CARTESIAN_POINT('Ctrl Pts',(10.2382140349999,11.6,2.80917449999999));
#196680=CARTESIAN_POINT('Ctrl Pts',(10.2360644839999,15.2,2.80909264399998));
#196681=CARTESIAN_POINT('Ctrl Pts',(10.2360644839999,11.6,2.80909264399998));
#196682=CARTESIAN_POINT('Ctrl Pts',(10.2339217719999,15.2,2.80900913799999));
#196683=CARTESIAN_POINT('Ctrl Pts',(10.2339217719999,11.6,2.80900913799999));
#196684=CARTESIAN_POINT('Ctrl Pts',(10.2317859129999,15.2,2.80892399399999));
#196685=CARTESIAN_POINT('Ctrl Pts',(10.2317859129999,11.6,2.80892399399999));
#196686=CARTESIAN_POINT('Ctrl Pts',(10.2296569209999,15.2,2.80883722299999));
#196687=CARTESIAN_POINT('Ctrl Pts',(10.2296569209999,11.6,2.80883722299999));
#196688=CARTESIAN_POINT('Ctrl Pts',(10.2275348109999,15.2,2.80874883799999));
#196689=CARTESIAN_POINT('Ctrl Pts',(10.2275348109999,11.6,2.80874883799999));
#196690=CARTESIAN_POINT('Ctrl Pts',(10.2254195939999,15.2,2.80865884799999));
#196691=CARTESIAN_POINT('Ctrl Pts',(10.2254195939999,11.6,2.80865884799999));
#196692=CARTESIAN_POINT('Ctrl Pts',(10.2233112869999,15.2,2.80856726499999));
#196693=CARTESIAN_POINT('Ctrl Pts',(10.2233112869999,11.6,2.80856726499999));
#196694=CARTESIAN_POINT('Ctrl Pts',(10.2212099009999,15.2,2.80847410299998));
#196695=CARTESIAN_POINT('Ctrl Pts',(10.2212099009999,11.6,2.80847410299998));
#196696=CARTESIAN_POINT('Ctrl Pts',(10.2191154529999,15.2,2.80837936999998));
#196697=CARTESIAN_POINT('Ctrl Pts',(10.2191154529999,11.6,2.80837936999998));
#196698=CARTESIAN_POINT('Ctrl Pts',(10.2170279549999,15.2,2.80828308099998));
#196699=CARTESIAN_POINT('Ctrl Pts',(10.2170279549999,11.6,2.80828308099998));
#196700=CARTESIAN_POINT('Ctrl Pts',(10.2149474219999,15.2,2.80818524499999));
#196701=CARTESIAN_POINT('Ctrl Pts',(10.2149474219999,11.6,2.80818524499999));
#196702=CARTESIAN_POINT('Ctrl Pts',(10.2128738679999,15.2,2.80808587499998));
#196703=CARTESIAN_POINT('Ctrl Pts',(10.2128738679999,11.6,2.80808587499998));
#196704=CARTESIAN_POINT('Ctrl Pts',(10.2108073059999,15.2,2.80798498399999));
#196705=CARTESIAN_POINT('Ctrl Pts',(10.2108073059999,11.6,2.80798498399999));
#196706=CARTESIAN_POINT('Ctrl Pts',(10.2087477509999,15.2,2.80788258099999));
#196707=CARTESIAN_POINT('Ctrl Pts',(10.2087477509999,11.6,2.80788258099999));
#196708=CARTESIAN_POINT('Ctrl Pts',(10.2066952179999,15.2,2.80777868099998));
#196709=CARTESIAN_POINT('Ctrl Pts',(10.2066952179999,11.6,2.80777868099998));
#196710=CARTESIAN_POINT('Ctrl Pts',(10.2046497199999,15.2,2.80767329399998));
#196711=CARTESIAN_POINT('Ctrl Pts',(10.2046497199999,11.6,2.80767329399998));
#196712=CARTESIAN_POINT('Ctrl Pts',(10.2026112719999,15.2,2.80756643299998));
#196713=CARTESIAN_POINT('Ctrl Pts',(10.2026112719999,11.6,2.80756643299998));
#196714=CARTESIAN_POINT('Ctrl Pts',(10.2005798889999,15.2,2.80745810899998));
#196715=CARTESIAN_POINT('Ctrl Pts',(10.2005798889999,11.6,2.80745810899998));
#196716=CARTESIAN_POINT('Ctrl Pts',(10.1985555829999,15.2,2.80734833399999));
#196717=CARTESIAN_POINT('Ctrl Pts',(10.1985555829999,11.6,2.80734833399999));
#196718=CARTESIAN_POINT('Ctrl Pts',(10.1965383709999,15.2,2.80723712199999));
#196719=CARTESIAN_POINT('Ctrl Pts',(10.1965383709999,11.6,2.80723712199999));
#196720=CARTESIAN_POINT('Ctrl Pts',(10.1945282669999,15.2,2.80712448399999));
#196721=CARTESIAN_POINT('Ctrl Pts',(10.1945282669999,11.6,2.80712448399999));
#196722=CARTESIAN_POINT('Ctrl Pts',(10.1925252829999,15.2,2.80701043199999));
#196723=CARTESIAN_POINT('Ctrl Pts',(10.1925252829999,11.6,2.80701043199999));
#196724=CARTESIAN_POINT('Ctrl Pts',(10.1905294369999,15.2,2.80689497899999));
#196725=CARTESIAN_POINT('Ctrl Pts',(10.1905294369999,11.6,2.80689497899999));
#196726=CARTESIAN_POINT('Ctrl Pts',(10.1885407419999,15.2,2.80677813699998));
#196727=CARTESIAN_POINT('Ctrl Pts',(10.1885407419999,11.6,2.80677813699998));
#196728=CARTESIAN_POINT('Ctrl Pts',(10.1865592119999,15.2,2.80665991699999));
#196729=CARTESIAN_POINT('Ctrl Pts',(10.1865592119999,11.6,2.80665991699998));
#196730=CARTESIAN_POINT('Ctrl Pts',(10.1845848629999,15.2,2.80654033399999));
#196731=CARTESIAN_POINT('Ctrl Pts',(10.1845848629999,11.6,2.80654033399998));
#196732=CARTESIAN_POINT('Ctrl Pts',(10.1826177079999,15.2,2.80641939899999));
#196733=CARTESIAN_POINT('Ctrl Pts',(10.1826177079999,11.6,2.80641939899999));
#196734=CARTESIAN_POINT('Ctrl Pts',(10.1806577639999,15.2,2.80629712499999));
#196735=CARTESIAN_POINT('Ctrl Pts',(10.1806577639999,11.6,2.80629712499999));
#196736=CARTESIAN_POINT('Ctrl Pts',(10.1787050449999,15.2,2.80617352499998));
#196737=CARTESIAN_POINT('Ctrl Pts',(10.1787050449999,11.6,2.80617352499998));
#196738=CARTESIAN_POINT('Ctrl Pts',(10.1767595639999,15.2,2.80604860999999));
#196739=CARTESIAN_POINT('Ctrl Pts',(10.1767595639999,11.6,2.80604860999999));
#196740=CARTESIAN_POINT('Ctrl Pts',(10.1748213379999,15.2,2.80592239499998));
#196741=CARTESIAN_POINT('Ctrl Pts',(10.1748213379999,11.6,2.80592239499998));
#196742=CARTESIAN_POINT('Ctrl Pts',(10.1728903809999,15.2,2.80579489099999));
#196743=CARTESIAN_POINT('Ctrl Pts',(10.1728903809999,11.6,2.80579489099999));
#196744=CARTESIAN_POINT('Ctrl Pts',(10.1709667089999,15.2,2.80566611099999));
#196745=CARTESIAN_POINT('Ctrl Pts',(10.1709667089999,11.6,2.80566611099999));
#196746=CARTESIAN_POINT('Ctrl Pts',(10.1690503349999,15.2,2.80553606899999));
#196747=CARTESIAN_POINT('Ctrl Pts',(10.1690503349999,11.6,2.80553606899998));
#196748=CARTESIAN_POINT('Ctrl Pts',(10.1671412759999,15.2,2.80540477799998));
#196749=CARTESIAN_POINT('Ctrl Pts',(10.1671412759999,11.6,2.80540477799998));
#196750=CARTESIAN_POINT('Ctrl Pts',(10.1652395459999,15.2,2.80527224899998));
#196751=CARTESIAN_POINT('Ctrl Pts',(10.1652395459999,11.6,2.80527224899998));
#196752=CARTESIAN_POINT('Ctrl Pts',(10.1633451609999,15.2,2.80513849699998));
#196753=CARTESIAN_POINT('Ctrl Pts',(10.1633451609999,11.6,2.80513849699998));
#196754=CARTESIAN_POINT('Ctrl Pts',(10.1614581339999,15.2,2.80500353399999));
#196755=CARTESIAN_POINT('Ctrl Pts',(10.1614581339999,11.6,2.80500353399999));
#196756=CARTESIAN_POINT('Ctrl Pts',(10.1595784839999,15.2,2.80486737399999));
#196757=CARTESIAN_POINT('Ctrl Pts',(10.1595784839999,11.6,2.80486737399999));
#196758=CARTESIAN_POINT('Ctrl Pts',(10.1577062229999,15.2,2.80473002899999));
#196759=CARTESIAN_POINT('Ctrl Pts',(10.1577062229999,11.6,2.80473002899999));
#196760=CARTESIAN_POINT('Ctrl Pts',(10.1558413669999,15.2,2.80459151299999));
#196761=CARTESIAN_POINT('Ctrl Pts',(10.1558413669999,11.6,2.80459151299999));
#196762=CARTESIAN_POINT('Ctrl Pts',(10.1539839329999,15.2,2.80445183999999));
#196763=CARTESIAN_POINT('Ctrl Pts',(10.1539839329999,11.6,2.80445183999999));
#196764=CARTESIAN_POINT('Ctrl Pts',(10.1521339339999,15.2,2.80431102199999));
#196765=CARTESIAN_POINT('Ctrl Pts',(10.1521339339999,11.6,2.80431102199999));
#196766=CARTESIAN_POINT('Ctrl Pts',(10.1502913879999,15.2,2.80416907399999));
#196767=CARTESIAN_POINT('Ctrl Pts',(10.1502913879999,11.6,2.80416907399999));
#196768=CARTESIAN_POINT('Ctrl Pts',(10.1484563089999,15.2,2.80402600799999));
#196769=CARTESIAN_POINT('Ctrl Pts',(10.1484563089999,11.6,2.80402600799999));
#196770=CARTESIAN_POINT('Ctrl Pts',(10.1466287129999,15.2,2.80388183699999));
#196771=CARTESIAN_POINT('Ctrl Pts',(10.1466287129999,11.6,2.80388183699999));
#196772=CARTESIAN_POINT('Ctrl Pts',(10.1448086139999,15.2,2.80373657799998));
#196773=CARTESIAN_POINT('Ctrl Pts',(10.1448086139999,11.6,2.80373657799998));
#196774=CARTESIAN_POINT('Ctrl Pts',(10.1429960289999,15.2,2.80359023999999));
#196775=CARTESIAN_POINT('Ctrl Pts',(10.1429960289999,11.6,2.80359023999999));
#196776=CARTESIAN_POINT('Ctrl Pts',(10.1411909749999,15.2,2.80344284099999));
#196777=CARTESIAN_POINT('Ctrl Pts',(10.1411909749999,11.6,2.80344284099999));
#196778=CARTESIAN_POINT('Ctrl Pts',(10.1393934659999,15.2,2.80329439199999));
#196779=CARTESIAN_POINT('Ctrl Pts',(10.1393934659999,11.6,2.80329439199999));
#196780=CARTESIAN_POINT('Ctrl Pts',(10.1376035179999,15.2,2.80314490699999));
#196781=CARTESIAN_POINT('Ctrl Pts',(10.1376035179999,11.6,2.80314490699999));
#196782=CARTESIAN_POINT('Ctrl Pts',(10.1358211459999,15.2,2.80299440199999));
#196783=CARTESIAN_POINT('Ctrl Pts',(10.1358211459999,11.6,2.80299440199998));
#196784=CARTESIAN_POINT('Ctrl Pts',(10.1340463689999,15.2,2.80284288899999));
#196785=CARTESIAN_POINT('Ctrl Pts',(10.1340463689999,11.6,2.80284288899999));
#196786=CARTESIAN_POINT('Ctrl Pts',(10.1322791999999,15.2,2.80269038199998));
#196787=CARTESIAN_POINT('Ctrl Pts',(10.1322791999999,11.6,2.80269038199998));
#196788=CARTESIAN_POINT('Ctrl Pts',(10.1305196549999,15.2,2.80253689599999));
#196789=CARTESIAN_POINT('Ctrl Pts',(10.1305196549999,11.6,2.80253689599998));
#196790=CARTESIAN_POINT('Ctrl Pts',(10.1287677519999,15.2,2.80238244599998));
#196791=CARTESIAN_POINT('Ctrl Pts',(10.1287677519999,11.6,2.80238244599998));
#196792=CARTESIAN_POINT('Ctrl Pts',(10.1270235059999,15.2,2.80222704299998));
#196793=CARTESIAN_POINT('Ctrl Pts',(10.1270235059999,11.6,2.80222704299998));
#196794=CARTESIAN_POINT('Ctrl Pts',(10.1252869329999,15.2,2.80207070399998));
#196795=CARTESIAN_POINT('Ctrl Pts',(10.1252869329999,11.6,2.80207070399998));
#196796=CARTESIAN_POINT('Ctrl Pts',(10.1235580499999,15.2,2.80191344299999));
#196797=CARTESIAN_POINT('Ctrl Pts',(10.1235580499999,11.6,2.80191344299999));
#196798=CARTESIAN_POINT('Ctrl Pts',(10.1218368709999,15.2,2.80175527399999));
#196799=CARTESIAN_POINT('Ctrl Pts',(10.1218368709999,11.6,2.80175527399999));
#196800=CARTESIAN_POINT('Ctrl Pts',(10.1201234149999,15.2,2.80159621099998));
#196801=CARTESIAN_POINT('Ctrl Pts',(10.1201234149999,11.6,2.80159621099998));
#196802=CARTESIAN_POINT('Ctrl Pts',(10.1184176969999,15.2,2.80143626899999));
#196803=CARTESIAN_POINT('Ctrl Pts',(10.1184176969999,11.6,2.80143626899999));
#196804=CARTESIAN_POINT('Ctrl Pts',(10.1167197329999,15.2,2.80127546199999));
#196805=CARTESIAN_POINT('Ctrl Pts',(10.1167197329999,11.6,2.80127546199999));
#196806=CARTESIAN_POINT('Ctrl Pts',(10.1150295409999,15.2,2.80111380599998));
#196807=CARTESIAN_POINT('Ctrl Pts',(10.1150295409999,11.6,2.80111380599998));
#196808=CARTESIAN_POINT('Ctrl Pts',(10.1133471369999,15.2,2.80095131499999));
#196809=CARTESIAN_POINT('Ctrl Pts',(10.1133471369999,11.6,2.80095131499999));
#196810=CARTESIAN_POINT('Ctrl Pts',(10.1116725359999,15.2,2.80078800299999));
#196811=CARTESIAN_POINT('Ctrl Pts',(10.1116725359999,11.6,2.80078800299999));
#196812=CARTESIAN_POINT('Ctrl Pts',(10.1100057559999,15.2,2.80062388499999));
#196813=CARTESIAN_POINT('Ctrl Pts',(10.1100057559999,11.6,2.80062388499999));
#196814=CARTESIAN_POINT('Ctrl Pts',(10.1083468139999,15.2,2.80045897699999));
#196815=CARTESIAN_POINT('Ctrl Pts',(10.1083468139999,11.6,2.80045897699999));
#196816=CARTESIAN_POINT('Ctrl Pts',(10.1066957249999,15.2,2.80029329299998));
#196817=CARTESIAN_POINT('Ctrl Pts',(10.1066957249999,11.6,2.80029329299998));
#196818=CARTESIAN_POINT('Ctrl Pts',(10.1050525089999,15.2,2.80012684799999));
#196819=CARTESIAN_POINT('Ctrl Pts',(10.1050525089999,11.6,2.80012684799999));
#196820=CARTESIAN_POINT('Ctrl Pts',(10.1034171789999,15.2,2.79995965799999));
#196821=CARTESIAN_POINT('Ctrl Pts',(10.1034171789999,11.6,2.79995965799999));
#196822=CARTESIAN_POINT('Ctrl Pts',(10.1017897539999,15.2,2.79979173799998));
#196823=CARTESIAN_POINT('Ctrl Pts',(10.1017897539999,11.6,2.79979173799998));
#196824=CARTESIAN_POINT('Ctrl Pts',(10.1001702509999,15.2,2.79962310199998));
#196825=CARTESIAN_POINT('Ctrl Pts',(10.1001702509999,11.6,2.79962310199998));
#196826=CARTESIAN_POINT('Ctrl Pts',(10.0985586869999,15.2,2.79945376699998));
#196827=CARTESIAN_POINT('Ctrl Pts',(10.0985586869999,11.6,2.79945376699998));
#196828=CARTESIAN_POINT('Ctrl Pts',(10.0969550769999,15.2,2.79928374699999));
#196829=CARTESIAN_POINT('Ctrl Pts',(10.0969550769999,11.6,2.79928374699998));
#196830=CARTESIAN_POINT('Ctrl Pts',(10.0953594409999,15.2,2.79911305799998));
#196831=CARTESIAN_POINT('Ctrl Pts',(10.0953594409999,11.6,2.79911305799998));
#196832=CARTESIAN_POINT('Ctrl Pts',(10.0937717949999,15.2,2.79894171599998));
#196833=CARTESIAN_POINT('Ctrl Pts',(10.0937717949999,11.6,2.79894171599998));
#196834=CARTESIAN_POINT('Ctrl Pts',(10.0921921569999,15.2,2.79876973499999));
#196835=CARTESIAN_POINT('Ctrl Pts',(10.0921921569999,11.6,2.79876973499999));
#196836=CARTESIAN_POINT('Ctrl Pts',(10.0906205419999,15.2,2.79859713299999));
#196837=CARTESIAN_POINT('Ctrl Pts',(10.0906205419999,11.6,2.79859713299999));
#196838=CARTESIAN_POINT('Ctrl Pts',(10.0890569699999,15.2,2.79842392399999));
#196839=CARTESIAN_POINT('Ctrl Pts',(10.0890569699999,11.6,2.79842392399999));
#196840=CARTESIAN_POINT('Ctrl Pts',(10.0875014559999,15.2,2.79825012399999));
#196841=CARTESIAN_POINT('Ctrl Pts',(10.0875014559999,11.6,2.79825012399999));
#196842=CARTESIAN_POINT('Ctrl Pts',(10.0859540199999,15.2,2.79807574899999));
#196843=CARTESIAN_POINT('Ctrl Pts',(10.0859540199999,11.6,2.79807574899999));
#196844=CARTESIAN_POINT('Ctrl Pts',(10.0844146779999,15.2,2.79790081599998));
#196845=CARTESIAN_POINT('Ctrl Pts',(10.0844146779999,11.6,2.79790081599998));
#196846=CARTESIAN_POINT('Ctrl Pts',(10.0828834479999,15.2,2.79772533899998));
#196847=CARTESIAN_POINT('Ctrl Pts',(10.0828834479999,11.6,2.79772533899998));
#196848=CARTESIAN_POINT('Ctrl Pts',(10.0813603479999,15.2,2.79754933599998));
#196849=CARTESIAN_POINT('Ctrl Pts',(10.0813603479999,11.6,2.79754933599998));
#196850=CARTESIAN_POINT('Ctrl Pts',(10.0798453939999,15.2,2.79737282199999));
#196851=CARTESIAN_POINT('Ctrl Pts',(10.0798453939999,11.6,2.79737282199999));
#196852=CARTESIAN_POINT('Ctrl Pts',(10.0783386059999,15.2,2.79719581399998));
#196853=CARTESIAN_POINT('Ctrl Pts',(10.0783386059999,11.6,2.79719581399998));
#196854=CARTESIAN_POINT('Ctrl Pts',(10.0768400009999,15.2,2.79701832799999));
#196855=CARTESIAN_POINT('Ctrl Pts',(10.0768400009999,11.6,2.79701832799999));
#196856=CARTESIAN_POINT('Ctrl Pts',(10.0753495959999,15.2,2.79684037999999));
#196857=CARTESIAN_POINT('Ctrl Pts',(10.0753495959999,11.6,2.79684037999999));
#196858=CARTESIAN_POINT('Ctrl Pts',(10.0738674099999,15.2,2.79666198699999));
#196859=CARTESIAN_POINT('Ctrl Pts',(10.0738674099999,11.6,2.79666198699999));
#196860=CARTESIAN_POINT('Ctrl Pts',(10.0723934619999,15.2,2.79648316499999));
#196861=CARTESIAN_POINT('Ctrl Pts',(10.0723934619999,11.6,2.79648316499999));
#196862=CARTESIAN_POINT('Ctrl Pts',(10.0709277689999,15.2,2.79630393099998));
#196863=CARTESIAN_POINT('Ctrl Pts',(10.0709277689999,11.6,2.79630393099998));
#196864=CARTESIAN_POINT('Ctrl Pts',(10.0694703469999,15.2,2.79612430099998));
#196865=CARTESIAN_POINT('Ctrl Pts',(10.0694703469999,11.6,2.79612430099998));
#196866=CARTESIAN_POINT('Ctrl Pts',(10.0680212179999,15.2,2.79594429399998));
#196867=CARTESIAN_POINT('Ctrl Pts',(10.0680212179999,11.6,2.79594429399998));
#196868=CARTESIAN_POINT('Ctrl Pts',(10.0665803979999,15.2,2.79576392499998));
#196869=CARTESIAN_POINT('Ctrl Pts',(10.0665803979999,11.6,2.79576392499998));
#196870=CARTESIAN_POINT('Ctrl Pts',(10.0651479059999,15.2,2.79558321099999));
#196871=CARTESIAN_POINT('Ctrl Pts',(10.0651479059999,11.6,2.79558321099999));
#196872=CARTESIAN_POINT('Ctrl Pts',(10.0637237609999,15.2,2.79540216899999));
#196873=CARTESIAN_POINT('Ctrl Pts',(10.0637237609999,11.6,2.79540216899999));
#196874=CARTESIAN_POINT('Ctrl Pts',(10.0623079809999,15.2,2.79522081599998));
#196875=CARTESIAN_POINT('Ctrl Pts',(10.0623079809999,11.6,2.79522081599998));
#196876=CARTESIAN_POINT('Ctrl Pts',(10.0609005839999,15.2,2.79503916999998));
#196877=CARTESIAN_POINT('Ctrl Pts',(10.0609005839999,11.6,2.79503916999998));
#196878=CARTESIAN_POINT('Ctrl Pts',(10.0595015889999,15.2,2.79485724899998));
#196879=CARTESIAN_POINT('Ctrl Pts',(10.0595015889999,11.6,2.79485724899998));
#196880=CARTESIAN_POINT('Ctrl Pts',(10.0581110159999,15.2,2.79467506799998));
#196881=CARTESIAN_POINT('Ctrl Pts',(10.0581110159999,11.6,2.79467506799998));
#196882=CARTESIAN_POINT('Ctrl Pts',(10.0567288819999,15.2,2.79449264599998));
#196883=CARTESIAN_POINT('Ctrl Pts',(10.0567288819999,11.6,2.79449264599998));
#196884=CARTESIAN_POINT('Ctrl Pts',(10.0553552059999,15.2,2.79430999899999));
#196885=CARTESIAN_POINT('Ctrl Pts',(10.0553552059999,11.6,2.79430999899999));
#196886=CARTESIAN_POINT('Ctrl Pts',(10.0539900079999,15.2,2.79412714599999));
#196887=CARTESIAN_POINT('Ctrl Pts',(10.0539900079999,11.6,2.79412714599999));
#196888=CARTESIAN_POINT('Ctrl Pts',(10.0526333059999,15.2,2.79394410499999));
#196889=CARTESIAN_POINT('Ctrl Pts',(10.0526333059999,11.6,2.79394410499999));
#196890=CARTESIAN_POINT('Ctrl Pts',(10.0512851199999,15.2,2.79376089299999));
#196891=CARTESIAN_POINT('Ctrl Pts',(10.0512851199999,11.6,2.79376089299999));
#196892=CARTESIAN_POINT('Ctrl Pts',(10.0499454679999,15.2,2.79357752799999));
#196893=CARTESIAN_POINT('Ctrl Pts',(10.0499454679999,11.6,2.79357752799999));
#196894=CARTESIAN_POINT('Ctrl Pts',(10.0486143699999,15.2,2.79339402899998));
#196895=CARTESIAN_POINT('Ctrl Pts',(10.0486143699999,11.6,2.79339402899998));
#196896=CARTESIAN_POINT('Ctrl Pts',(10.0472918449999,15.2,2.79321041199999));
#196897=CARTESIAN_POINT('Ctrl Pts',(10.0472918449999,11.6,2.79321041199999));
#196898=CARTESIAN_POINT('Ctrl Pts',(10.0459779129999,15.2,2.79302669599998));
#196899=CARTESIAN_POINT('Ctrl Pts',(10.0459779129999,11.6,2.79302669599998));
#196900=CARTESIAN_POINT('Ctrl Pts',(10.0446725919999,15.2,2.79284289899999));
#196901=CARTESIAN_POINT('Ctrl Pts',(10.0446725919999,11.6,2.79284289899999));
#196902=CARTESIAN_POINT('Ctrl Pts',(10.0433759029999,15.2,2.79265903999999));
#196903=CARTESIAN_POINT('Ctrl Pts',(10.0433759029999,11.6,2.79265903999998));
#196904=CARTESIAN_POINT('Ctrl Pts',(10.0420878649999,15.2,2.79247513699998));
#196905=CARTESIAN_POINT('Ctrl Pts',(10.0420878649999,11.6,2.79247513699998));
#196906=CARTESIAN_POINT('Ctrl Pts',(10.0408084969999,15.2,2.79229120899998));
#196907=CARTESIAN_POINT('Ctrl Pts',(10.0408084969999,11.6,2.79229120899998));
#196908=CARTESIAN_POINT('Ctrl Pts',(10.0395378199999,15.2,2.79210727399998));
#196909=CARTESIAN_POINT('Ctrl Pts',(10.0395378199999,11.6,2.79210727399998));
#196910=CARTESIAN_POINT('Ctrl Pts',(10.0382758529999,15.2,2.79192334999999));
#196911=CARTESIAN_POINT('Ctrl Pts',(10.0382758529999,11.6,2.79192334999998));
#196912=CARTESIAN_POINT('Ctrl Pts',(10.0370226159999,15.2,2.79173945599998));
#196913=CARTESIAN_POINT('Ctrl Pts',(10.0370226159999,11.6,2.79173945599998));
#196914=CARTESIAN_POINT('Ctrl Pts',(10.0357781289999,15.2,2.79155561199998));
#196915=CARTESIAN_POINT('Ctrl Pts',(10.0357781289999,11.6,2.79155561199998));
#196916=CARTESIAN_POINT('Ctrl Pts',(10.0345424119999,15.2,2.79137183599998));
#196917=CARTESIAN_POINT('Ctrl Pts',(10.0345424119999,11.6,2.79137183599998));
#196918=CARTESIAN_POINT('Ctrl Pts',(10.0333154849999,15.2,2.79118814799999));
#196919=CARTESIAN_POINT('Ctrl Pts',(10.0333154849999,11.6,2.79118814799999));
#196920=CARTESIAN_POINT('Ctrl Pts',(10.0320973689999,15.2,2.79100456599998));
#196921=CARTESIAN_POINT('Ctrl Pts',(10.0320973689999,11.6,2.79100456599998));
#196922=CARTESIAN_POINT('Ctrl Pts',(10.0308880829999,15.2,2.79082110899999));
#196923=CARTESIAN_POINT('Ctrl Pts',(10.0308880829999,11.6,2.79082110899999));
#196924=CARTESIAN_POINT('Ctrl Pts',(10.0296876489999,15.2,2.79063779799999));
#196925=CARTESIAN_POINT('Ctrl Pts',(10.0296876489999,11.6,2.79063779799999));
#196926=CARTESIAN_POINT('Ctrl Pts',(10.0284960859999,15.2,2.79045464999999));
#196927=CARTESIAN_POINT('Ctrl Pts',(10.0284960859999,11.6,2.79045464999999));
#196928=CARTESIAN_POINT('Ctrl Pts',(10.0273134139999,15.2,2.79027168599999));
#196929=CARTESIAN_POINT('Ctrl Pts',(10.0273134139999,11.6,2.79027168599998));
#196930=CARTESIAN_POINT('Ctrl Pts',(10.0261396569999,15.2,2.79008892699999));
#196931=CARTESIAN_POINT('Ctrl Pts',(10.0261396569999,11.6,2.79008892699998));
#196932=CARTESIAN_POINT('Ctrl Pts',(10.0249748309999,15.2,2.78990638999999));
#196933=CARTESIAN_POINT('Ctrl Pts',(10.0249748309999,11.6,2.78990638999998));
#196934=CARTESIAN_POINT('Ctrl Pts',(10.0238189609999,15.2,2.78972409599999));
#196935=CARTESIAN_POINT('Ctrl Pts',(10.0238189609999,11.6,2.78972409599999));
#196936=CARTESIAN_POINT('Ctrl Pts',(10.0226720649999,15.2,2.78954206499999));
#196937=CARTESIAN_POINT('Ctrl Pts',(10.0226720649999,11.6,2.78954206499999));
#196938=CARTESIAN_POINT('Ctrl Pts',(10.0215341659999,15.2,2.78936031699998));
#196939=CARTESIAN_POINT('Ctrl Pts',(10.0215341659999,11.6,2.78936031699998));
#196940=CARTESIAN_POINT('Ctrl Pts',(10.0204052839999,15.2,2.78917887199999));
#196941=CARTESIAN_POINT('Ctrl Pts',(10.0204052839999,11.6,2.78917887199999));
#196942=CARTESIAN_POINT('Ctrl Pts',(10.0192854389999,15.2,2.78899774999999));
#196943=CARTESIAN_POINT('Ctrl Pts',(10.0192854389999,11.6,2.78899774999999));
#196944=CARTESIAN_POINT('Ctrl Pts',(10.0181746539999,15.2,2.78881697199999));
#196945=CARTESIAN_POINT('Ctrl Pts',(10.0181746539999,11.6,2.78881697199999));
#196946=CARTESIAN_POINT('Ctrl Pts',(10.0170729509999,15.2,2.78863655799999));
#196947=CARTESIAN_POINT('Ctrl Pts',(10.0170729509999,11.6,2.78863655799999));
#196948=CARTESIAN_POINT('Ctrl Pts',(10.0159803479999,15.2,2.78845652899999));
#196949=CARTESIAN_POINT('Ctrl Pts',(10.0159803479999,11.6,2.78845652899999));
#196950=CARTESIAN_POINT('Ctrl Pts',(10.0148968709999,15.2,2.78827690399999));
#196951=CARTESIAN_POINT('Ctrl Pts',(10.0148968709999,11.6,2.78827690399999));
#196952=CARTESIAN_POINT('Ctrl Pts',(10.0138225379999,15.2,2.78809770699999));
#196953=CARTESIAN_POINT('Ctrl Pts',(10.0138225379999,11.6,2.78809770699999));
#196954=CARTESIAN_POINT('Ctrl Pts',(10.0127573729999,15.2,2.78791895599999));
#196955=CARTESIAN_POINT('Ctrl Pts',(10.0127573729999,11.6,2.78791895599999));
#196956=CARTESIAN_POINT('Ctrl Pts',(10.0117013959999,15.2,2.78774067199999));
#196957=CARTESIAN_POINT('Ctrl Pts',(10.0117013959999,11.6,2.78774067199999));
#196958=CARTESIAN_POINT('Ctrl Pts',(10.0106546299999,15.2,2.78756287699998));
#196959=CARTESIAN_POINT('Ctrl Pts',(10.0106546299999,11.6,2.78756287699998));
#196960=CARTESIAN_POINT('Ctrl Pts',(10.0096170959999,15.2,2.78738559299998));
#196961=CARTESIAN_POINT('Ctrl Pts',(10.0096170959999,11.6,2.78738559299998));
#196962=CARTESIAN_POINT('Ctrl Pts',(10.0085888169999,15.2,2.78720884099998));
#196963=CARTESIAN_POINT('Ctrl Pts',(10.0085888169999,11.6,2.78720884099998));
#196964=CARTESIAN_POINT('Ctrl Pts',(10.0075698159999,15.2,2.78703263999999));
#196965=CARTESIAN_POINT('Ctrl Pts',(10.0075698159999,11.6,2.78703263999999));
#196966=CARTESIAN_POINT('Ctrl Pts',(10.0065601129999,15.2,2.78685701499998));
#196967=CARTESIAN_POINT('Ctrl Pts',(10.0065601129999,11.6,2.78685701499998));
#196968=CARTESIAN_POINT('Ctrl Pts',(10.0055597309999,15.2,2.78668198499999));
#196969=CARTESIAN_POINT('Ctrl Pts',(10.0055597309999,11.6,2.78668198499999));
#196970=CARTESIAN_POINT('Ctrl Pts',(10.0045686949999,15.2,2.78650757299998));
#196971=CARTESIAN_POINT('Ctrl Pts',(10.0045686949999,11.6,2.78650757299998));
#196972=CARTESIAN_POINT('Ctrl Pts',(10.0035870229999,15.2,2.78633380099999));
#196973=CARTESIAN_POINT('Ctrl Pts',(10.0035870229999,11.6,2.78633380099999));
#196974=CARTESIAN_POINT('Ctrl Pts',(10.0026147409999,15.2,2.78616069099999));
#196975=CARTESIAN_POINT('Ctrl Pts',(10.0026147409999,11.6,2.78616069099999));
#196976=CARTESIAN_POINT('Ctrl Pts',(10.0016518709999,15.2,2.78598826499999));
#196977=CARTESIAN_POINT('Ctrl Pts',(10.0016518709999,11.6,2.78598826499999));
#196978=CARTESIAN_POINT('Ctrl Pts',(10.0006984369999,15.2,2.78581654399999));
#196979=CARTESIAN_POINT('Ctrl Pts',(10.0006984369999,11.6,2.78581654399999));
#196980=CARTESIAN_POINT('Ctrl Pts',(9.99975445999995,15.2,2.78564555199999));
#196981=CARTESIAN_POINT('Ctrl Pts',(9.99975445999995,11.6,2.78564555199999));
#196982=CARTESIAN_POINT('Ctrl Pts',(9.99881996399995,15.2,2.78547531199998));
#196983=CARTESIAN_POINT('Ctrl Pts',(9.99881996399995,11.6,2.78547531199998));
#196984=CARTESIAN_POINT('Ctrl Pts',(9.99789497199994,15.2,2.78530584299999));
#196985=CARTESIAN_POINT('Ctrl Pts',(9.99789497199994,11.6,2.78530584299999));
#196986=CARTESIAN_POINT('Ctrl Pts',(9.99697950699994,15.2,2.78513717199999));
#196987=CARTESIAN_POINT('Ctrl Pts',(9.99697950699994,11.6,2.78513717199999));
#196988=CARTESIAN_POINT('Ctrl Pts',(9.99607881099994,15.2,2.78497028699999));
#196989=CARTESIAN_POINT('Ctrl Pts',(9.99607881099994,11.6,2.78497028699999));
#196990=CARTESIAN_POINT('Ctrl Pts',(9.99536684599994,15.2,2.78483763599999));
#196991=CARTESIAN_POINT('Ctrl Pts',(9.99536684599994,11.6,2.78483763599999));
#196992=CARTESIAN_POINT('Ctrl Pts',(9.99483839999994,15.2,2.78473876999998));
#196993=CARTESIAN_POINT('Ctrl Pts',(9.99483839999994,11.6,2.78473876999998));
#196994=CARTESIAN_POINT('Ctrl Pts',(9.99448967699994,15.2,2.78467334899998));
#196995=CARTESIAN_POINT('Ctrl Pts',(9.99448967699994,11.6,2.78467334899998));
#196996=CARTESIAN_POINT('Ctrl Pts',(9.99431831699994,15.2,2.78464115899999));
#196997=CARTESIAN_POINT('Ctrl Pts',(9.99431831699994,11.6,2.78464115899998));
#196998=CARTESIAN_POINT('',(9.99431831699994,12.2,2.78464115899999));
#196999=CARTESIAN_POINT('',(9.99431831699994,15.2,2.78464115899999));
#197000=CARTESIAN_POINT('',(9.99431831699994,12.2,2.78464115899999));
#197001=CARTESIAN_POINT('Ctrl Pts',(11.1757778679999,12.2,2.71145515299998));
#197002=CARTESIAN_POINT('Ctrl Pts',(11.1750309949999,12.2,2.71161876799999));
#197003=CARTESIAN_POINT('Ctrl Pts',(11.1735376169999,12.2,2.71194562399998));
#197004=CARTESIAN_POINT('Ctrl Pts',(11.1712986599999,12.2,2.71243477999998));
#197005=CARTESIAN_POINT('Ctrl Pts',(11.1683155989999,12.2,2.71308473599999));
#197006=CARTESIAN_POINT('Ctrl Pts',(11.1645904639999,12.2,2.71389342499998));
#197007=CARTESIAN_POINT('Ctrl Pts',(11.1608690239999,12.2,2.71469835899998));
#197008=CARTESIAN_POINT('Ctrl Pts',(11.1571512799999,12.2,2.71549953899999));
#197009=CARTESIAN_POINT('Ctrl Pts',(11.1534372359999,12.2,2.71629696699998));
#197010=CARTESIAN_POINT('Ctrl Pts',(11.1497268969999,12.2,2.71709064499999));
#197011=CARTESIAN_POINT('Ctrl Pts',(11.1460202709999,12.2,2.71788057599998));
#197012=CARTESIAN_POINT('Ctrl Pts',(11.1423173659999,12.2,2.71866676499998));
#197013=CARTESIAN_POINT('Ctrl Pts',(11.1386181909999,12.2,2.71944921899999));
#197014=CARTESIAN_POINT('Ctrl Pts',(11.1349227589999,12.2,2.72022793899998));
#197015=CARTESIAN_POINT('Ctrl Pts',(11.1312310749999,12.2,2.72100293299999));
#197016=CARTESIAN_POINT('Ctrl Pts',(11.1275431529999,12.2,2.72177420499998));
#197017=CARTESIAN_POINT('Ctrl Pts',(11.1238589999999,12.2,2.72254175699998));
#197018=CARTESIAN_POINT('Ctrl Pts',(11.1201786229999,12.2,2.72330559599999));
#197019=CARTESIAN_POINT('Ctrl Pts',(11.1165020289999,12.2,2.72406572399999));
#197020=CARTESIAN_POINT('Ctrl Pts',(11.1128292269999,12.2,2.72482214499998));
#197021=CARTESIAN_POINT('Ctrl Pts',(11.1091602219999,12.2,2.72557486299998));
#197022=CARTESIAN_POINT('Ctrl Pts',(11.1054950239999,12.2,2.72632388099999));
#197023=CARTESIAN_POINT('Ctrl Pts',(11.1018336399999,12.2,2.72706920299999));
#197024=CARTESIAN_POINT('Ctrl Pts',(11.0981760779999,12.2,2.72781083499999));
#197025=CARTESIAN_POINT('Ctrl Pts',(11.0945223469999,12.2,2.72854877899999));
#197026=CARTESIAN_POINT('Ctrl Pts',(11.0908724549999,12.2,2.72928304099998));
#197027=CARTESIAN_POINT('Ctrl Pts',(11.0872264109999,12.2,2.73001362299999));
#197028=CARTESIAN_POINT('Ctrl Pts',(11.0835842229999,12.2,2.73074053299998));
#197029=CARTESIAN_POINT('Ctrl Pts',(11.0799458989999,12.2,2.73146377099999));
#197030=CARTESIAN_POINT('Ctrl Pts',(11.0763114489999,12.2,2.73218334499998));
#197031=CARTESIAN_POINT('Ctrl Pts',(11.0726808779999,12.2,2.73289925699999));
#197032=CARTESIAN_POINT('Ctrl Pts',(11.0690541959999,12.2,2.73361151099999));
#197033=CARTESIAN_POINT('Ctrl Pts',(11.0654314099999,12.2,2.73432011199999));
#197034=CARTESIAN_POINT('Ctrl Pts',(11.0618125299999,12.2,2.73502506399999));
#197035=CARTESIAN_POINT('Ctrl Pts',(11.0581975619999,12.2,2.73572636999998));
#197036=CARTESIAN_POINT('Ctrl Pts',(11.0545865169999,12.2,2.73642403699998));
#197037=CARTESIAN_POINT('Ctrl Pts',(11.0509794009999,12.2,2.73711806699998));
#197038=CARTESIAN_POINT('Ctrl Pts',(11.0473762219999,12.2,2.73780846599998));
#197039=CARTESIAN_POINT('Ctrl Pts',(11.0437769909999,12.2,2.73849523599999));
#197040=CARTESIAN_POINT('Ctrl Pts',(11.0401817149999,12.2,2.73917838399999));
#197041=CARTESIAN_POINT('Ctrl Pts',(11.0365903999999,12.2,2.73985791299998));
#197042=CARTESIAN_POINT('Ctrl Pts',(11.0330030589999,12.2,2.74053382799998));
#197043=CARTESIAN_POINT('Ctrl Pts',(11.0294196959999,12.2,2.74120613199998));
#197044=CARTESIAN_POINT('Ctrl Pts',(11.0258403219999,12.2,2.74187483099999));
#197045=CARTESIAN_POINT('Ctrl Pts',(11.0222649439999,12.2,2.74253992799999));
#197046=CARTESIAN_POINT('Ctrl Pts',(11.0186935709999,12.2,2.74320142899998));
#197047=CARTESIAN_POINT('Ctrl Pts',(11.0151262099999,12.2,2.74385933599999));
#197048=CARTESIAN_POINT('Ctrl Pts',(11.0115628719999,12.2,2.74451365599998));
#197049=CARTESIAN_POINT('Ctrl Pts',(11.0080035629999,12.2,2.74516439199999));
#197050=CARTESIAN_POINT('Ctrl Pts',(11.0044482939999,12.2,2.74581154899998));
#197051=CARTESIAN_POINT('Ctrl Pts',(11.0008970699999,12.2,2.74645513199999));
#197052=CARTESIAN_POINT('Ctrl Pts',(10.9973499019999,12.2,2.74709514499998));
#197053=CARTESIAN_POINT('Ctrl Pts',(10.9938067979999,12.2,2.74773159199999));
#197054=CARTESIAN_POINT('Ctrl Pts',(10.9902677649999,12.2,2.74836447799998));
#197055=CARTESIAN_POINT('Ctrl Pts',(10.9867328139999,12.2,2.74899380799998));
#197056=CARTESIAN_POINT('Ctrl Pts',(10.9832019509999,12.2,2.74961958599999));
#197057=CARTESIAN_POINT('Ctrl Pts',(10.9796751869999,12.2,2.75024181699998));
#197058=CARTESIAN_POINT('Ctrl Pts',(10.9761525279999,12.2,2.75086050399998));
#197059=CARTESIAN_POINT('Ctrl Pts',(10.9726339839999,12.2,2.75147565399998));
#197060=CARTESIAN_POINT('Ctrl Pts',(10.9691195629999,12.2,2.75208726999999));
#197061=CARTESIAN_POINT('Ctrl Pts',(10.9656092739999,12.2,2.75269535799998));
#197062=CARTESIAN_POINT('Ctrl Pts',(10.9621031259999,12.2,2.75329992099999));
#197063=CARTESIAN_POINT('Ctrl Pts',(10.9586011259999,12.2,2.75390096599998));
#197064=CARTESIAN_POINT('Ctrl Pts',(10.9551032829999,12.2,2.75449849499999));
#197065=CARTESIAN_POINT('Ctrl Pts',(10.9516096059999,12.2,2.75509251399999));
#197066=CARTESIAN_POINT('Ctrl Pts',(10.9481201049999,12.2,2.75568302799999));
#197067=CARTESIAN_POINT('Ctrl Pts',(10.9446347859999,12.2,2.75627004099999));
#197068=CARTESIAN_POINT('Ctrl Pts',(10.9411536579999,12.2,2.75685355899999));
#197069=CARTESIAN_POINT('Ctrl Pts',(10.9376767319999,12.2,2.75743358499999));
#197070=CARTESIAN_POINT('Ctrl Pts',(10.9342040149999,12.2,2.75801012499999));
#197071=CARTESIAN_POINT('Ctrl Pts',(10.9307355149999,12.2,2.75858318399998));
#197072=CARTESIAN_POINT('Ctrl Pts',(10.9272712419999,12.2,2.75915276599999));
#197073=CARTESIAN_POINT('Ctrl Pts',(10.9238112039999,12.2,2.75971887599999));
#197074=CARTESIAN_POINT('Ctrl Pts',(10.9203554099999,12.2,2.76028151899999));
#197075=CARTESIAN_POINT('Ctrl Pts',(10.9169038679999,12.2,2.76084069999998));
#197076=CARTESIAN_POINT('Ctrl Pts',(10.9134565879999,12.2,2.76139642399999));
#197077=CARTESIAN_POINT('Ctrl Pts',(10.9100135769999,12.2,2.76194869599999));
#197078=CARTESIAN_POINT('Ctrl Pts',(10.9065748449999,12.2,2.76249751999998));
#197079=CARTESIAN_POINT('Ctrl Pts',(10.9031404009999,12.2,2.76304290199998));
#197080=CARTESIAN_POINT('Ctrl Pts',(10.8997102529999,12.2,2.76358484599999));
#197081=CARTESIAN_POINT('Ctrl Pts',(10.8962844109999,12.2,2.76412335799999));
#197082=CARTESIAN_POINT('Ctrl Pts',(10.8928628809999,12.2,2.76465844099998));
#197083=CARTESIAN_POINT('Ctrl Pts',(10.8894456749999,12.2,2.76519010299998));
#197084=CARTESIAN_POINT('Ctrl Pts',(10.8860327999999,12.2,2.76571834699999));
#197085=CARTESIAN_POINT('Ctrl Pts',(10.8826242649999,12.2,2.76624317899999));
#197086=CARTESIAN_POINT('Ctrl Pts',(10.8792200789999,12.2,2.76676460199998));
#197087=CARTESIAN_POINT('Ctrl Pts',(10.8758202519999,12.2,2.76728262299999));
#197088=CARTESIAN_POINT('Ctrl Pts',(10.8724247909999,12.2,2.76779724699999));
#197089=CARTESIAN_POINT('Ctrl Pts',(10.8690337059999,12.2,2.76830847799998));
#197090=CARTESIAN_POINT('Ctrl Pts',(10.8656470049999,12.2,2.76881632399999));
#197091=CARTESIAN_POINT('Ctrl Pts',(10.8622646979999,12.2,2.76932078499998));
#197092=CARTESIAN_POINT('Ctrl Pts',(10.8588867929999,12.2,2.76982187099998));
#197093=CARTESIAN_POINT('Ctrl Pts',(10.8555133009999,12.2,2.77031958499999));
#197094=CARTESIAN_POINT('Ctrl Pts',(10.8521442279999,12.2,2.77081393199998));
#197095=CARTESIAN_POINT('Ctrl Pts',(10.8487795839999,12.2,2.77130491799999));
#197096=CARTESIAN_POINT('Ctrl Pts',(10.8454193789999,12.2,2.77179254799999));
#197097=CARTESIAN_POINT('Ctrl Pts',(10.8420636209999,12.2,2.77227682699999));
#197098=CARTESIAN_POINT('Ctrl Pts',(10.8387123189999,12.2,2.77275775999998));
#197099=CARTESIAN_POINT('Ctrl Pts',(10.8353654819999,12.2,2.77323535299999));
#197100=CARTESIAN_POINT('Ctrl Pts',(10.8320231199999,12.2,2.77370960999999));
#197101=CARTESIAN_POINT('Ctrl Pts',(10.8286852409999,12.2,2.77418053799998));
#197102=CARTESIAN_POINT('Ctrl Pts',(10.8253518549999,12.2,2.77464814099999));
#197103=CARTESIAN_POINT('Ctrl Pts',(10.8220229679999,12.2,2.77511242599999));
#197104=CARTESIAN_POINT('Ctrl Pts',(10.8186985939999,12.2,2.77557339599999));
#197105=CARTESIAN_POINT('Ctrl Pts',(10.8153787389999,12.2,2.77603105699999));
#197106=CARTESIAN_POINT('Ctrl Pts',(10.8120634119999,12.2,2.77648541599999));
#197107=CARTESIAN_POINT('Ctrl Pts',(10.8087526239999,12.2,2.77693647799998));
#197108=CARTESIAN_POINT('Ctrl Pts',(10.8054463819999,12.2,2.77738424699999));
#197109=CARTESIAN_POINT('Ctrl Pts',(10.8021446959999,12.2,2.77782872899999));
#197110=CARTESIAN_POINT('Ctrl Pts',(10.7988475759999,12.2,2.77826992999999));
#197111=CARTESIAN_POINT('Ctrl Pts',(10.7955550299999,12.2,2.77870785499999));
#197112=CARTESIAN_POINT('Ctrl Pts',(10.7922670679999,12.2,2.77914250999999));
#197113=CARTESIAN_POINT('Ctrl Pts',(10.7889836979999,12.2,2.77957390099999));
#197114=CARTESIAN_POINT('Ctrl Pts',(10.7857049309999,12.2,2.78000203199999));
#197115=CARTESIAN_POINT('Ctrl Pts',(10.7824307749999,12.2,2.78042690799998));
#197116=CARTESIAN_POINT('Ctrl Pts',(10.7791612379999,12.2,2.78084853699998));
#197117=CARTESIAN_POINT('Ctrl Pts',(10.7758963329999,12.2,2.78126692399999));
#197118=CARTESIAN_POINT('Ctrl Pts',(10.7726360659999,12.2,2.78168207299998));
#197119=CARTESIAN_POINT('Ctrl Pts',(10.7693804469999,12.2,2.78209399099998));
#197120=CARTESIAN_POINT('Ctrl Pts',(10.7661294859999,12.2,2.78250268399999));
#197121=CARTESIAN_POINT('Ctrl Pts',(10.7628831919999,12.2,2.78290815599998));
#197122=CARTESIAN_POINT('Ctrl Pts',(10.7596415739999,12.2,2.78331041399999));
#197123=CARTESIAN_POINT('Ctrl Pts',(10.7564046409999,12.2,2.78370946299999));
#197124=CARTESIAN_POINT('Ctrl Pts',(10.7531724039999,12.2,2.78410530999999));
#197125=CARTESIAN_POINT('Ctrl Pts',(10.7499448709999,12.2,2.78449795899999));
#197126=CARTESIAN_POINT('Ctrl Pts',(10.7467220519999,12.2,2.78488741599999));
#197127=CARTESIAN_POINT('Ctrl Pts',(10.7435039549999,12.2,2.78527368799999));
#197128=CARTESIAN_POINT('Ctrl Pts',(10.7402905919999,12.2,2.78565678199998));
#197129=CARTESIAN_POINT('Ctrl Pts',(10.7370819699999,12.2,2.78603669899999));
#197130=CARTESIAN_POINT('Ctrl Pts',(10.7338780989999,12.2,2.78641344999999));
#197131=CARTESIAN_POINT('Ctrl Pts',(10.7306789899999,12.2,2.78678703799999));
#197132=CARTESIAN_POINT('Ctrl Pts',(10.7274846509999,12.2,2.78715746999998));
#197133=CARTESIAN_POINT('Ctrl Pts',(10.7242950909999,12.2,2.78752475099999));
#197134=CARTESIAN_POINT('Ctrl Pts',(10.7211103209999,12.2,2.78788888599999));
#197135=CARTESIAN_POINT('Ctrl Pts',(10.7179303499999,12.2,2.78824988399998));
#197136=CARTESIAN_POINT('Ctrl Pts',(10.7147551869999,12.2,2.78860774899999));
#197137=CARTESIAN_POINT('Ctrl Pts',(10.7115848429999,12.2,2.78896248699999));
#197138=CARTESIAN_POINT('Ctrl Pts',(10.7084193239999,12.2,2.78931410399998));
#197139=CARTESIAN_POINT('Ctrl Pts',(10.7052586439999,12.2,2.78966260699999));
#197140=CARTESIAN_POINT('Ctrl Pts',(10.7021028099999,12.2,2.79000799999999));
#197141=CARTESIAN_POINT('Ctrl Pts',(10.6989518329999,12.2,2.79035029099998));
#197142=CARTESIAN_POINT('Ctrl Pts',(10.6958057219999,12.2,2.79068948499999));
#197143=CARTESIAN_POINT('Ctrl Pts',(10.6926644859999,12.2,2.79102558999998));
#197144=CARTESIAN_POINT('Ctrl Pts',(10.6895281349999,12.2,2.79135860899999));
#197145=CARTESIAN_POINT('Ctrl Pts',(10.6863966799999,12.2,2.79168855099999));
#197146=CARTESIAN_POINT('Ctrl Pts',(10.6832701279999,12.2,2.79201541999999));
#197147=CARTESIAN_POINT('Ctrl Pts',(10.6801484919999,12.2,2.79233922399998));
#197148=CARTESIAN_POINT('Ctrl Pts',(10.6770317779999,12.2,2.79265996699999));
#197149=CARTESIAN_POINT('Ctrl Pts',(10.6739199989999,12.2,2.79297765699998));
#197150=CARTESIAN_POINT('Ctrl Pts',(10.6708131629999,12.2,2.79329229999998));
#197151=CARTESIAN_POINT('Ctrl Pts',(10.6677112809999,12.2,2.79360390199999));
#197152=CARTESIAN_POINT('Ctrl Pts',(10.6646143609999,12.2,2.79391246899999));
#197153=CARTESIAN_POINT('Ctrl Pts',(10.6615224159999,12.2,2.79421800799999));
#197154=CARTESIAN_POINT('Ctrl Pts',(10.6584354509999,12.2,2.79452052399999));
#197155=CARTESIAN_POINT('Ctrl Pts',(10.6553534799999,12.2,2.79482002499999));
#197156=CARTESIAN_POINT('Ctrl Pts',(10.6522765109999,12.2,2.79511651699998));
#197157=CARTESIAN_POINT('Ctrl Pts',(10.6492045549999,12.2,2.79541000599998));
#197158=CARTESIAN_POINT('Ctrl Pts',(10.6461376199999,12.2,2.79570049699998));
#197159=CARTESIAN_POINT('Ctrl Pts',(10.6430757179999,12.2,2.79598799899999));
#197160=CARTESIAN_POINT('Ctrl Pts',(10.6400188569999,12.2,2.79627251799998));
#197161=CARTESIAN_POINT('Ctrl Pts',(10.6369670479999,12.2,2.79655405899998));
#197162=CARTESIAN_POINT('Ctrl Pts',(10.6339203009999,12.2,2.79683262899999));
#197163=CARTESIAN_POINT('Ctrl Pts',(10.6308786259999,12.2,2.79710823499999));
#197164=CARTESIAN_POINT('Ctrl Pts',(10.6278420329999,12.2,2.79738088399998));
#197165=CARTESIAN_POINT('Ctrl Pts',(10.6248105309999,12.2,2.79765058099999));
#197166=CARTESIAN_POINT('Ctrl Pts',(10.6217841319999,12.2,2.79791733399998));
#197167=CARTESIAN_POINT('Ctrl Pts',(10.6187628439999,12.2,2.79818114899999));
#197168=CARTESIAN_POINT('Ctrl Pts',(10.6157466779999,12.2,2.79844203299999));
#197169=CARTESIAN_POINT('Ctrl Pts',(10.6127356429999,12.2,2.79869999199998));
#197170=CARTESIAN_POINT('Ctrl Pts',(10.6097297519999,12.2,2.79895503299999));
#197171=CARTESIAN_POINT('Ctrl Pts',(10.6067290119999,12.2,2.79920716299999));
#197172=CARTESIAN_POINT('Ctrl Pts',(10.6037334349999,12.2,2.79945638899999));
#197173=CARTESIAN_POINT('Ctrl Pts',(10.6007430289999,12.2,2.79970271699998));
#197174=CARTESIAN_POINT('Ctrl Pts',(10.5977578069999,12.2,2.79994615399998));
#197175=CARTESIAN_POINT('Ctrl Pts',(10.5947777769999,12.2,2.80018670699998));
#197176=CARTESIAN_POINT('Ctrl Pts',(10.5918029509999,12.2,2.80042438199998));
#197177=CARTESIAN_POINT('Ctrl Pts',(10.5888333369999,12.2,2.80065918699999));
#197178=CARTESIAN_POINT('Ctrl Pts',(10.5858689469999,12.2,2.80089112799998));
#197179=CARTESIAN_POINT('Ctrl Pts',(10.5829097899999,12.2,2.80112021299999));
#197180=CARTESIAN_POINT('Ctrl Pts',(10.5799558779999,12.2,2.80134644699999));
#197181=CARTESIAN_POINT('Ctrl Pts',(10.5770072199999,12.2,2.80156983799999));
#197182=CARTESIAN_POINT('Ctrl Pts',(10.5740638259999,12.2,2.80179039399999));
#197183=CARTESIAN_POINT('Ctrl Pts',(10.5711257059999,12.2,2.80200812099999));
#197184=CARTESIAN_POINT('Ctrl Pts',(10.5681928729999,12.2,2.80222302499999));
#197185=CARTESIAN_POINT('Ctrl Pts',(10.5652653349999,12.2,2.80243511499998));
#197186=CARTESIAN_POINT('Ctrl Pts',(10.5623431029999,12.2,2.80264439699998));
#197187=CARTESIAN_POINT('Ctrl Pts',(10.5594261859999,12.2,2.80285087799999));
#197188=CARTESIAN_POINT('Ctrl Pts',(10.5565145969999,12.2,2.80305456499998));
#197189=CARTESIAN_POINT('Ctrl Pts',(10.5536083449999,12.2,2.80325546599999));
#197190=CARTESIAN_POINT('Ctrl Pts',(10.5507074409999,12.2,2.80345358699999));
#197191=CARTESIAN_POINT('Ctrl Pts',(10.5478118939999,12.2,2.80364893599998));
#197192=CARTESIAN_POINT('Ctrl Pts',(10.5449217159999,12.2,2.80384151899998));
#197193=CARTESIAN_POINT('Ctrl Pts',(10.5420369179999,12.2,2.80403134499998));
#197194=CARTESIAN_POINT('Ctrl Pts',(10.5391575079999,12.2,2.80421842099998));
#197195=CARTESIAN_POINT('Ctrl Pts',(10.5362834999999,12.2,2.80440275299998));
#197196=CARTESIAN_POINT('Ctrl Pts',(10.5334149019999,12.2,2.80458434899998));
#197197=CARTESIAN_POINT('Ctrl Pts',(10.5305517249999,12.2,2.80476321599998));
#197198=CARTESIAN_POINT('Ctrl Pts',(10.5276939799999,12.2,2.80493936099998));
#197199=CARTESIAN_POINT('Ctrl Pts',(10.5248416769999,12.2,2.80511279299999));
#197200=CARTESIAN_POINT('Ctrl Pts',(10.5219948289999,12.2,2.80528351899999));
#197201=CARTESIAN_POINT('Ctrl Pts',(10.5191534429999,12.2,2.80545154499999));
#197202=CARTESIAN_POINT('Ctrl Pts',(10.5163175329999,12.2,2.80561687899999));
#197203=CARTESIAN_POINT('Ctrl Pts',(10.5134871079999,12.2,2.80577952899999));
#197204=CARTESIAN_POINT('Ctrl Pts',(10.5106621789999,12.2,2.80593950299998));
#197205=CARTESIAN_POINT('Ctrl Pts',(10.5078427569999,12.2,2.80609680699998));
#197206=CARTESIAN_POINT('Ctrl Pts',(10.5050288509999,12.2,2.80625144999998));
#197207=CARTESIAN_POINT('Ctrl Pts',(10.5022204749999,12.2,2.80640343899999));
#197208=CARTESIAN_POINT('Ctrl Pts',(10.4994176369999,12.2,2.80655278099999));
#197209=CARTESIAN_POINT('Ctrl Pts',(10.4966203499999,12.2,2.80669948499998));
#197210=CARTESIAN_POINT('Ctrl Pts',(10.4938286229999,12.2,2.80684355699999));
#197211=CARTESIAN_POINT('Ctrl Pts',(10.4910424679999,12.2,2.80698500599998));
#197212=CARTESIAN_POINT('Ctrl Pts',(10.4882618969999,12.2,2.80712383899999));
#197213=CARTESIAN_POINT('Ctrl Pts',(10.4854869179999,12.2,2.80726006499999));
#197214=CARTESIAN_POINT('Ctrl Pts',(10.4827175439999,12.2,2.80739368999999));
#197215=CARTESIAN_POINT('Ctrl Pts',(10.4799537849999,12.2,2.80752472299999));
#197216=CARTESIAN_POINT('Ctrl Pts',(10.4771956519999,12.2,2.80765317099998));
#197217=CARTESIAN_POINT('Ctrl Pts',(10.4744431569999,12.2,2.80777904299998));
#197218=CARTESIAN_POINT('Ctrl Pts',(10.4716963109999,12.2,2.80790234499998));
#197219=CARTESIAN_POINT('Ctrl Pts',(10.4689551229999,12.2,2.80802308599998));
#197220=CARTESIAN_POINT('Ctrl Pts',(10.4662196059999,12.2,2.80814127499998));
#197221=CARTESIAN_POINT('Ctrl Pts',(10.4634897709999,12.2,2.80825691999999));
#197222=CARTESIAN_POINT('Ctrl Pts',(10.4607656289999,12.2,2.80837002599998));
#197223=CARTESIAN_POINT('Ctrl Pts',(10.4580471909999,12.2,2.80848060399999));
#197224=CARTESIAN_POINT('Ctrl Pts',(10.4553344669999,12.2,2.80858866099998));
#197225=CARTESIAN_POINT('Ctrl Pts',(10.4526274699999,12.2,2.80869420399998));
#197226=CARTESIAN_POINT('Ctrl Pts',(10.4499262109999,12.2,2.80879724399998));
#197227=CARTESIAN_POINT('Ctrl Pts',(10.4472306989999,12.2,2.80889778599998));
#197228=CARTESIAN_POINT('Ctrl Pts',(10.4445409479999,12.2,2.80899584099998));
#197229=CARTESIAN_POINT('Ctrl Pts',(10.4418569669999,12.2,2.80909141499999));
#197230=CARTESIAN_POINT('Ctrl Pts',(10.4391787699999,12.2,2.80918451599998));
#197231=CARTESIAN_POINT('Ctrl Pts',(10.4365063659999,12.2,2.80927515599998));
#197232=CARTESIAN_POINT('Ctrl Pts',(10.4338397659999,12.2,2.80936333799998));
#197233=CARTESIAN_POINT('Ctrl Pts',(10.4311789839999,12.2,2.80944907299999));
#197234=CARTESIAN_POINT('Ctrl Pts',(10.4285240289999,12.2,2.80953237099999));
#197235=CARTESIAN_POINT('Ctrl Pts',(10.4258749129999,12.2,2.80961323599998));
#197236=CARTESIAN_POINT('Ctrl Pts',(10.4232316479999,12.2,2.80969167999999));
#197237=CARTESIAN_POINT('Ctrl Pts',(10.4205942449999,12.2,2.80976771199998));
#197238=CARTESIAN_POINT('Ctrl Pts',(10.4179627159999,12.2,2.80984133699998));
#197239=CARTESIAN_POINT('Ctrl Pts',(10.4153370719999,12.2,2.80991256599999));
#197240=CARTESIAN_POINT('Ctrl Pts',(10.4127173239999,12.2,2.80998140599999));
#197241=CARTESIAN_POINT('Ctrl Pts',(10.4101034849999,12.2,2.81004786799999));
#197242=CARTESIAN_POINT('Ctrl Pts',(10.4074955649999,12.2,2.81011195799999));
#197243=CARTESIAN_POINT('Ctrl Pts',(10.4048935769999,12.2,2.81017368599999));
#197244=CARTESIAN_POINT('Ctrl Pts',(10.4022975309999,12.2,2.81023305999998));
#197245=CARTESIAN_POINT('Ctrl Pts',(10.3997074399999,12.2,2.81029008999998));
#197246=CARTESIAN_POINT('Ctrl Pts',(10.3971233149999,12.2,2.81034478199999));
#197247=CARTESIAN_POINT('Ctrl Pts',(10.3945451689999,12.2,2.81039714699999));
#197248=CARTESIAN_POINT('Ctrl Pts',(10.3919730119999,12.2,2.81044719399999));
#197249=CARTESIAN_POINT('Ctrl Pts',(10.3894068559999,12.2,2.81049492999998));
#197250=CARTESIAN_POINT('Ctrl Pts',(10.3868467139999,12.2,2.81054036599999));
#197251=CARTESIAN_POINT('Ctrl Pts',(10.3842925959999,12.2,2.81058350899999));
#197252=CARTESIAN_POINT('Ctrl Pts',(10.3817445159999,12.2,2.81062436799999));
#197253=CARTESIAN_POINT('Ctrl Pts',(10.3792024839999,12.2,2.81066295399999));
#197254=CARTESIAN_POINT('Ctrl Pts',(10.3766665119999,12.2,2.81069927299999));
#197255=CARTESIAN_POINT('Ctrl Pts',(10.3741366129999,12.2,2.81073333699998));
#197256=CARTESIAN_POINT('Ctrl Pts',(10.3716127979999,12.2,2.81076515299999));
#197257=CARTESIAN_POINT('Ctrl Pts',(10.3690950799999,12.2,2.81079473099999));
#197258=CARTESIAN_POINT('Ctrl Pts',(10.3665834699999,12.2,2.81082207899999));
#197259=CARTESIAN_POINT('Ctrl Pts',(10.3640779799999,12.2,2.81084720699998));
#197260=CARTESIAN_POINT('Ctrl Pts',(10.3615786239999,12.2,2.81087012399999));
#197261=CARTESIAN_POINT('Ctrl Pts',(10.3590854099999,12.2,2.81089083999999));
#197262=CARTESIAN_POINT('Ctrl Pts',(10.3565983529999,12.2,2.81090936199998));
#197263=CARTESIAN_POINT('Ctrl Pts',(10.3541174659999,12.2,2.81092570199998));
#197264=CARTESIAN_POINT('Ctrl Pts',(10.3516427589999,12.2,2.81093986799998));
#197265=CARTESIAN_POINT('Ctrl Pts',(10.3491742439999,12.2,2.81095186899999));
#197266=CARTESIAN_POINT('Ctrl Pts',(10.3467119339999,12.2,2.81096171499998));
#197267=CARTESIAN_POINT('Ctrl Pts',(10.3442558419999,12.2,2.81096941599999));
#197268=CARTESIAN_POINT('Ctrl Pts',(10.3418059809999,12.2,2.81097497899999));
#197269=CARTESIAN_POINT('Ctrl Pts',(10.3393623599999,12.2,2.81097841599999));
#197270=CARTESIAN_POINT('Ctrl Pts',(10.3369249929999,12.2,2.81097973599999));
#197271=CARTESIAN_POINT('Ctrl Pts',(10.3344938929999,12.2,2.81097894699998));
#197272=CARTESIAN_POINT('Ctrl Pts',(10.3320690709999,12.2,2.81097606099999));
#197273=CARTESIAN_POINT('Ctrl Pts',(10.3296505419999,12.2,2.81097108499999));
#197274=CARTESIAN_POINT('Ctrl Pts',(10.3272383149999,12.2,2.81096403199999));
#197275=CARTESIAN_POINT('Ctrl Pts',(10.3248324049999,12.2,2.81095490799999));
#197276=CARTESIAN_POINT('Ctrl Pts',(10.3224328229999,12.2,2.81094372499999));
#197277=CARTESIAN_POINT('Ctrl Pts',(10.3200395829999,12.2,2.81093049299999));
#197278=CARTESIAN_POINT('Ctrl Pts',(10.3176526949999,12.2,2.81091521999999));
#197279=CARTESIAN_POINT('Ctrl Pts',(10.3152721739999,12.2,2.81089791699999));
#197280=CARTESIAN_POINT('Ctrl Pts',(10.3128980319999,12.2,2.81087859499999));
#197281=CARTESIAN_POINT('Ctrl Pts',(10.3105302809999,12.2,2.81085726199999));
#197282=CARTESIAN_POINT('Ctrl Pts',(10.3081689339999,12.2,2.81083392699998));
#197283=CARTESIAN_POINT('Ctrl Pts',(10.3058140039999,12.2,2.81080860299999));
#197284=CARTESIAN_POINT('Ctrl Pts',(10.3034655029999,12.2,2.81078129899999));
#197285=CARTESIAN_POINT('Ctrl Pts',(10.3011234449999,12.2,2.81075202499999));
#197286=CARTESIAN_POINT('Ctrl Pts',(10.2987878399999,12.2,2.81072078899999));
#197287=CARTESIAN_POINT('Ctrl Pts',(10.2964587039999,12.2,2.81068760399998));
#197288=CARTESIAN_POINT('Ctrl Pts',(10.2941360499999,12.2,2.81065247899999));
#197289=CARTESIAN_POINT('Ctrl Pts',(10.2918198869999,12.2,2.81061542499998));
#197290=CARTESIAN_POINT('Ctrl Pts',(10.2895102319999,12.2,2.81057645199999));
#197291=CARTESIAN_POINT('Ctrl Pts',(10.2872070959999,12.2,2.81053556799999));
#197292=CARTESIAN_POINT('Ctrl Pts',(10.2849104899999,12.2,2.81049278699999));
#197293=CARTESIAN_POINT('Ctrl Pts',(10.2826204319999,12.2,2.81044811699999));
#197294=CARTESIAN_POINT('Ctrl Pts',(10.2803369309999,12.2,2.81040156799998));
#197295=CARTESIAN_POINT('Ctrl Pts',(10.2780600009999,12.2,2.81035315199999));
#197296=CARTESIAN_POINT('Ctrl Pts',(10.2757896559999,12.2,2.81030288099998));
#197297=CARTESIAN_POINT('Ctrl Pts',(10.2735259089999,12.2,2.81025076199998));
#197298=CARTESIAN_POINT('Ctrl Pts',(10.2712687709999,12.2,2.81019680599999));
#197299=CARTESIAN_POINT('Ctrl Pts',(10.2690182579999,12.2,2.81014102599999));
#197300=CARTESIAN_POINT('Ctrl Pts',(10.2667743819999,12.2,2.81008343199999));
#197301=CARTESIAN_POINT('Ctrl Pts',(10.2645371559999,12.2,2.81002403399999));
#197302=CARTESIAN_POINT('Ctrl Pts',(10.2623065929999,12.2,2.80996284199999));
#197303=CARTESIAN_POINT('Ctrl Pts',(10.2600827069999,12.2,2.80989986699999));
#197304=CARTESIAN_POINT('Ctrl Pts',(10.2578655119999,12.2,2.80983512099999));
#197305=CARTESIAN_POINT('Ctrl Pts',(10.2556550209999,12.2,2.80976861599999));
#197306=CARTESIAN_POINT('Ctrl Pts',(10.2534512459999,12.2,2.80970035899998));
#197307=CARTESIAN_POINT('Ctrl Pts',(10.2512542019999,12.2,2.80963036499998));
#197308=CARTESIAN_POINT('Ctrl Pts',(10.2490639019999,12.2,2.80955864199999));
#197309=CARTESIAN_POINT('Ctrl Pts',(10.2468803589999,12.2,2.80948520299999));
#197310=CARTESIAN_POINT('Ctrl Pts',(10.2447035879999,12.2,2.80941005799999));
#197311=CARTESIAN_POINT('Ctrl Pts',(10.2425335999999,12.2,2.80933321799999));
#197312=CARTESIAN_POINT('Ctrl Pts',(10.2403704109999,12.2,2.80925469399998));
#197313=CARTESIAN_POINT('Ctrl Pts',(10.2382140349999,12.2,2.80917449999999));
#197314=CARTESIAN_POINT('Ctrl Pts',(10.2360644839999,12.2,2.80909264399998));
#197315=CARTESIAN_POINT('Ctrl Pts',(10.2339217719999,12.2,2.80900913799999));
#197316=CARTESIAN_POINT('Ctrl Pts',(10.2317859129999,12.2,2.80892399399999));
#197317=CARTESIAN_POINT('Ctrl Pts',(10.2296569209999,12.2,2.80883722299999));
#197318=CARTESIAN_POINT('Ctrl Pts',(10.2275348109999,12.2,2.80874883799999));
#197319=CARTESIAN_POINT('Ctrl Pts',(10.2254195939999,12.2,2.80865884799999));
#197320=CARTESIAN_POINT('Ctrl Pts',(10.2233112869999,12.2,2.80856726499999));
#197321=CARTESIAN_POINT('Ctrl Pts',(10.2212099009999,12.2,2.80847410299998));
#197322=CARTESIAN_POINT('Ctrl Pts',(10.2191154529999,12.2,2.80837936999998));
#197323=CARTESIAN_POINT('Ctrl Pts',(10.2170279549999,12.2,2.80828308099998));
#197324=CARTESIAN_POINT('Ctrl Pts',(10.2149474219999,12.2,2.80818524499999));
#197325=CARTESIAN_POINT('Ctrl Pts',(10.2128738679999,12.2,2.80808587499998));
#197326=CARTESIAN_POINT('Ctrl Pts',(10.2108073059999,12.2,2.80798498399999));
#197327=CARTESIAN_POINT('Ctrl Pts',(10.2087477509999,12.2,2.80788258099999));
#197328=CARTESIAN_POINT('Ctrl Pts',(10.2066952179999,12.2,2.80777868099998));
#197329=CARTESIAN_POINT('Ctrl Pts',(10.2046497199999,12.2,2.80767329399998));
#197330=CARTESIAN_POINT('Ctrl Pts',(10.2026112719999,12.2,2.80756643299998));
#197331=CARTESIAN_POINT('Ctrl Pts',(10.2005798889999,12.2,2.80745810899998));
#197332=CARTESIAN_POINT('Ctrl Pts',(10.1985555829999,12.2,2.80734833399999));
#197333=CARTESIAN_POINT('Ctrl Pts',(10.1965383709999,12.2,2.80723712199999));
#197334=CARTESIAN_POINT('Ctrl Pts',(10.1945282669999,12.2,2.80712448399999));
#197335=CARTESIAN_POINT('Ctrl Pts',(10.1925252829999,12.2,2.80701043199999));
#197336=CARTESIAN_POINT('Ctrl Pts',(10.1905294369999,12.2,2.80689497899999));
#197337=CARTESIAN_POINT('Ctrl Pts',(10.1885407419999,12.2,2.80677813699998));
#197338=CARTESIAN_POINT('Ctrl Pts',(10.1865592119999,12.2,2.80665991699999));
#197339=CARTESIAN_POINT('Ctrl Pts',(10.1845848629999,12.2,2.80654033399999));
#197340=CARTESIAN_POINT('Ctrl Pts',(10.1826177079999,12.2,2.80641939899999));
#197341=CARTESIAN_POINT('Ctrl Pts',(10.1806577639999,12.2,2.80629712499999));
#197342=CARTESIAN_POINT('Ctrl Pts',(10.1787050449999,12.2,2.80617352499998));
#197343=CARTESIAN_POINT('Ctrl Pts',(10.1767595639999,12.2,2.80604860999999));
#197344=CARTESIAN_POINT('Ctrl Pts',(10.1748213379999,12.2,2.80592239499998));
#197345=CARTESIAN_POINT('Ctrl Pts',(10.1728903809999,12.2,2.80579489099999));
#197346=CARTESIAN_POINT('Ctrl Pts',(10.1709667089999,12.2,2.80566611099999));
#197347=CARTESIAN_POINT('Ctrl Pts',(10.1690503349999,12.2,2.80553606899999));
#197348=CARTESIAN_POINT('Ctrl Pts',(10.1671412759999,12.2,2.80540477799998));
#197349=CARTESIAN_POINT('Ctrl Pts',(10.1652395459999,12.2,2.80527224899998));
#197350=CARTESIAN_POINT('Ctrl Pts',(10.1633451609999,12.2,2.80513849699998));
#197351=CARTESIAN_POINT('Ctrl Pts',(10.1614581339999,12.2,2.80500353399999));
#197352=CARTESIAN_POINT('Ctrl Pts',(10.1595784839999,12.2,2.80486737399999));
#197353=CARTESIAN_POINT('Ctrl Pts',(10.1577062229999,12.2,2.80473002899999));
#197354=CARTESIAN_POINT('Ctrl Pts',(10.1558413669999,12.2,2.80459151299999));
#197355=CARTESIAN_POINT('Ctrl Pts',(10.1539839329999,12.2,2.80445183999999));
#197356=CARTESIAN_POINT('Ctrl Pts',(10.1521339339999,12.2,2.80431102199999));
#197357=CARTESIAN_POINT('Ctrl Pts',(10.1502913879999,12.2,2.80416907399999));
#197358=CARTESIAN_POINT('Ctrl Pts',(10.1484563089999,12.2,2.80402600799999));
#197359=CARTESIAN_POINT('Ctrl Pts',(10.1466287129999,12.2,2.80388183699999));
#197360=CARTESIAN_POINT('Ctrl Pts',(10.1448086139999,12.2,2.80373657799998));
#197361=CARTESIAN_POINT('Ctrl Pts',(10.1429960289999,12.2,2.80359023999999));
#197362=CARTESIAN_POINT('Ctrl Pts',(10.1411909749999,12.2,2.80344284099999));
#197363=CARTESIAN_POINT('Ctrl Pts',(10.1393934659999,12.2,2.80329439199999));
#197364=CARTESIAN_POINT('Ctrl Pts',(10.1376035179999,12.2,2.80314490699999));
#197365=CARTESIAN_POINT('Ctrl Pts',(10.1358211459999,12.2,2.80299440199999));
#197366=CARTESIAN_POINT('Ctrl Pts',(10.1340463689999,12.2,2.80284288899999));
#197367=CARTESIAN_POINT('Ctrl Pts',(10.1322791999999,12.2,2.80269038199998));
#197368=CARTESIAN_POINT('Ctrl Pts',(10.1305196549999,12.2,2.80253689599999));
#197369=CARTESIAN_POINT('Ctrl Pts',(10.1287677519999,12.2,2.80238244599998));
#197370=CARTESIAN_POINT('Ctrl Pts',(10.1270235059999,12.2,2.80222704299998));
#197371=CARTESIAN_POINT('Ctrl Pts',(10.1252869329999,12.2,2.80207070399998));
#197372=CARTESIAN_POINT('Ctrl Pts',(10.1235580499999,12.2,2.80191344299999));
#197373=CARTESIAN_POINT('Ctrl Pts',(10.1218368709999,12.2,2.80175527399999));
#197374=CARTESIAN_POINT('Ctrl Pts',(10.1201234149999,12.2,2.80159621099998));
#197375=CARTESIAN_POINT('Ctrl Pts',(10.1184176969999,12.2,2.80143626899999));
#197376=CARTESIAN_POINT('Ctrl Pts',(10.1167197329999,12.2,2.80127546199999));
#197377=CARTESIAN_POINT('Ctrl Pts',(10.1150295409999,12.2,2.80111380599998));
#197378=CARTESIAN_POINT('Ctrl Pts',(10.1133471369999,12.2,2.80095131499999));
#197379=CARTESIAN_POINT('Ctrl Pts',(10.1116725359999,12.2,2.80078800299999));
#197380=CARTESIAN_POINT('Ctrl Pts',(10.1100057559999,12.2,2.80062388499999));
#197381=CARTESIAN_POINT('Ctrl Pts',(10.1083468139999,12.2,2.80045897699999));
#197382=CARTESIAN_POINT('Ctrl Pts',(10.1066957249999,12.2,2.80029329299998));
#197383=CARTESIAN_POINT('Ctrl Pts',(10.1050525089999,12.2,2.80012684799999));
#197384=CARTESIAN_POINT('Ctrl Pts',(10.1034171789999,12.2,2.79995965799999));
#197385=CARTESIAN_POINT('Ctrl Pts',(10.1017897539999,12.2,2.79979173799998));
#197386=CARTESIAN_POINT('Ctrl Pts',(10.1001702509999,12.2,2.79962310199998));
#197387=CARTESIAN_POINT('Ctrl Pts',(10.0985586869999,12.2,2.79945376699998));
#197388=CARTESIAN_POINT('Ctrl Pts',(10.0969550769999,12.2,2.79928374699999));
#197389=CARTESIAN_POINT('Ctrl Pts',(10.0953594409999,12.2,2.79911305799998));
#197390=CARTESIAN_POINT('Ctrl Pts',(10.0937717949999,12.2,2.79894171599998));
#197391=CARTESIAN_POINT('Ctrl Pts',(10.0921921569999,12.2,2.79876973499999));
#197392=CARTESIAN_POINT('Ctrl Pts',(10.0906205419999,12.2,2.79859713299999));
#197393=CARTESIAN_POINT('Ctrl Pts',(10.0890569699999,12.2,2.79842392399999));
#197394=CARTESIAN_POINT('Ctrl Pts',(10.0875014559999,12.2,2.79825012399999));
#197395=CARTESIAN_POINT('Ctrl Pts',(10.0859540199999,12.2,2.79807574899999));
#197396=CARTESIAN_POINT('Ctrl Pts',(10.0844146779999,12.2,2.79790081599998));
#197397=CARTESIAN_POINT('Ctrl Pts',(10.0828834479999,12.2,2.79772533899998));
#197398=CARTESIAN_POINT('Ctrl Pts',(10.0813603479999,12.2,2.79754933599998));
#197399=CARTESIAN_POINT('Ctrl Pts',(10.0798453939999,12.2,2.79737282199999));
#197400=CARTESIAN_POINT('Ctrl Pts',(10.0783386059999,12.2,2.79719581399998));
#197401=CARTESIAN_POINT('Ctrl Pts',(10.0768400009999,12.2,2.79701832799999));
#197402=CARTESIAN_POINT('Ctrl Pts',(10.0753495959999,12.2,2.79684037999999));
#197403=CARTESIAN_POINT('Ctrl Pts',(10.0738674099999,12.2,2.79666198699999));
#197404=CARTESIAN_POINT('Ctrl Pts',(10.0723934619999,12.2,2.79648316499999));
#197405=CARTESIAN_POINT('Ctrl Pts',(10.0709277689999,12.2,2.79630393099998));
#197406=CARTESIAN_POINT('Ctrl Pts',(10.0694703469999,12.2,2.79612430099998));
#197407=CARTESIAN_POINT('Ctrl Pts',(10.0680212179999,12.2,2.79594429399998));
#197408=CARTESIAN_POINT('Ctrl Pts',(10.0665803979999,12.2,2.79576392499998));
#197409=CARTESIAN_POINT('Ctrl Pts',(10.0651479059999,12.2,2.79558321099999));
#197410=CARTESIAN_POINT('Ctrl Pts',(10.0637237609999,12.2,2.79540216899999));
#197411=CARTESIAN_POINT('Ctrl Pts',(10.0623079809999,12.2,2.79522081599998));
#197412=CARTESIAN_POINT('Ctrl Pts',(10.0609005839999,12.2,2.79503916999998));
#197413=CARTESIAN_POINT('Ctrl Pts',(10.0595015889999,12.2,2.79485724899998));
#197414=CARTESIAN_POINT('Ctrl Pts',(10.0581110159999,12.2,2.79467506799998));
#197415=CARTESIAN_POINT('Ctrl Pts',(10.0567288819999,12.2,2.79449264599998));
#197416=CARTESIAN_POINT('Ctrl Pts',(10.0553552059999,12.2,2.79430999899999));
#197417=CARTESIAN_POINT('Ctrl Pts',(10.0539900079999,12.2,2.79412714599999));
#197418=CARTESIAN_POINT('Ctrl Pts',(10.0526333059999,12.2,2.79394410499999));
#197419=CARTESIAN_POINT('Ctrl Pts',(10.0512851199999,12.2,2.79376089299999));
#197420=CARTESIAN_POINT('Ctrl Pts',(10.0499454679999,12.2,2.79357752799999));
#197421=CARTESIAN_POINT('Ctrl Pts',(10.0486143699999,12.2,2.79339402899998));
#197422=CARTESIAN_POINT('Ctrl Pts',(10.0472918449999,12.2,2.79321041199999));
#197423=CARTESIAN_POINT('Ctrl Pts',(10.0459779129999,12.2,2.79302669599998));
#197424=CARTESIAN_POINT('Ctrl Pts',(10.0446725919999,12.2,2.79284289899999));
#197425=CARTESIAN_POINT('Ctrl Pts',(10.0433759029999,12.2,2.79265903999999));
#197426=CARTESIAN_POINT('Ctrl Pts',(10.0420878649999,12.2,2.79247513699998));
#197427=CARTESIAN_POINT('Ctrl Pts',(10.0408084969999,12.2,2.79229120899998));
#197428=CARTESIAN_POINT('Ctrl Pts',(10.0395378199999,12.2,2.79210727399998));
#197429=CARTESIAN_POINT('Ctrl Pts',(10.0382758529999,12.2,2.79192334999999));
#197430=CARTESIAN_POINT('Ctrl Pts',(10.0370226159999,12.2,2.79173945599998));
#197431=CARTESIAN_POINT('Ctrl Pts',(10.0357781289999,12.2,2.79155561199998));
#197432=CARTESIAN_POINT('Ctrl Pts',(10.0345424119999,12.2,2.79137183599998));
#197433=CARTESIAN_POINT('Ctrl Pts',(10.0333154849999,12.2,2.79118814799999));
#197434=CARTESIAN_POINT('Ctrl Pts',(10.0320973689999,12.2,2.79100456599998));
#197435=CARTESIAN_POINT('Ctrl Pts',(10.0308880829999,12.2,2.79082110899999));
#197436=CARTESIAN_POINT('Ctrl Pts',(10.0296876489999,12.2,2.79063779799999));
#197437=CARTESIAN_POINT('Ctrl Pts',(10.0284960859999,12.2,2.79045464999999));
#197438=CARTESIAN_POINT('Ctrl Pts',(10.0273134139999,12.2,2.79027168599999));
#197439=CARTESIAN_POINT('Ctrl Pts',(10.0261396569999,12.2,2.79008892699999));
#197440=CARTESIAN_POINT('Ctrl Pts',(10.0249748309999,12.2,2.78990638999999));
#197441=CARTESIAN_POINT('Ctrl Pts',(10.0238189609999,12.2,2.78972409599999));
#197442=CARTESIAN_POINT('Ctrl Pts',(10.0226720649999,12.2,2.78954206499999));
#197443=CARTESIAN_POINT('Ctrl Pts',(10.0215341659999,12.2,2.78936031699998));
#197444=CARTESIAN_POINT('Ctrl Pts',(10.0204052839999,12.2,2.78917887199999));
#197445=CARTESIAN_POINT('Ctrl Pts',(10.0192854389999,12.2,2.78899774999999));
#197446=CARTESIAN_POINT('Ctrl Pts',(10.0181746539999,12.2,2.78881697199999));
#197447=CARTESIAN_POINT('Ctrl Pts',(10.0170729509999,12.2,2.78863655799999));
#197448=CARTESIAN_POINT('Ctrl Pts',(10.0159803479999,12.2,2.78845652899999));
#197449=CARTESIAN_POINT('Ctrl Pts',(10.0148968709999,12.2,2.78827690399999));
#197450=CARTESIAN_POINT('Ctrl Pts',(10.0138225379999,12.2,2.78809770699999));
#197451=CARTESIAN_POINT('Ctrl Pts',(10.0127573729999,12.2,2.78791895599999));
#197452=CARTESIAN_POINT('Ctrl Pts',(10.0117013959999,12.2,2.78774067199999));
#197453=CARTESIAN_POINT('Ctrl Pts',(10.0106546299999,12.2,2.78756287699998));
#197454=CARTESIAN_POINT('Ctrl Pts',(10.0096170959999,12.2,2.78738559299998));
#197455=CARTESIAN_POINT('Ctrl Pts',(10.0085888169999,12.2,2.78720884099998));
#197456=CARTESIAN_POINT('Ctrl Pts',(10.0075698159999,12.2,2.78703263999999));
#197457=CARTESIAN_POINT('Ctrl Pts',(10.0065601129999,12.2,2.78685701499998));
#197458=CARTESIAN_POINT('Ctrl Pts',(10.0055597309999,12.2,2.78668198499999));
#197459=CARTESIAN_POINT('Ctrl Pts',(10.0045686949999,12.2,2.78650757299998));
#197460=CARTESIAN_POINT('Ctrl Pts',(10.0035870229999,12.2,2.78633380099999));
#197461=CARTESIAN_POINT('Ctrl Pts',(10.0026147409999,12.2,2.78616069099999));
#197462=CARTESIAN_POINT('Ctrl Pts',(10.0016518709999,12.2,2.78598826499999));
#197463=CARTESIAN_POINT('Ctrl Pts',(10.0006984369999,12.2,2.78581654399999));
#197464=CARTESIAN_POINT('Ctrl Pts',(9.99975445999995,12.2,2.78564555199999));
#197465=CARTESIAN_POINT('Ctrl Pts',(9.99881996399995,12.2,2.78547531199998));
#197466=CARTESIAN_POINT('Ctrl Pts',(9.99789497199994,12.2,2.78530584299999));
#197467=CARTESIAN_POINT('Ctrl Pts',(9.99697950699994,12.2,2.78513717199999));
#197468=CARTESIAN_POINT('Ctrl Pts',(9.99607881099994,12.2,2.78497028699999));
#197469=CARTESIAN_POINT('Ctrl Pts',(9.99536684599994,12.2,2.78483763599999));
#197470=CARTESIAN_POINT('Ctrl Pts',(9.99483839899994,12.2,2.78473876899999));
#197471=CARTESIAN_POINT('Ctrl Pts',(9.99448967699994,12.2,2.78467334899998));
#197472=CARTESIAN_POINT('Ctrl Pts',(9.99431831699994,12.2,2.78464115899999));
#197473=CARTESIAN_POINT('Ctrl Pts',(9.99431831699994,15.2,2.78464115899999));
#197474=CARTESIAN_POINT('Ctrl Pts',(9.99448967699994,15.2,2.78467334899998));
#197475=CARTESIAN_POINT('Ctrl Pts',(9.99483839899994,15.2,2.78473876899999));
#197476=CARTESIAN_POINT('Ctrl Pts',(9.99536684599994,15.2,2.78483763599999));
#197477=CARTESIAN_POINT('Ctrl Pts',(9.99607881099994,15.2,2.78497028699999));
#197478=CARTESIAN_POINT('Ctrl Pts',(9.99697950699994,15.2,2.78513717199999));
#197479=CARTESIAN_POINT('Ctrl Pts',(9.99789497199994,15.2,2.78530584299999));
#197480=CARTESIAN_POINT('Ctrl Pts',(9.99881996399995,15.2,2.78547531199998));
#197481=CARTESIAN_POINT('Ctrl Pts',(9.99975445999995,15.2,2.78564555199999));
#197482=CARTESIAN_POINT('Ctrl Pts',(10.0006984369999,15.2,2.78581654399999));
#197483=CARTESIAN_POINT('Ctrl Pts',(10.0016518709999,15.2,2.78598826499999));
#197484=CARTESIAN_POINT('Ctrl Pts',(10.0026147409999,15.2,2.78616069099999));
#197485=CARTESIAN_POINT('Ctrl Pts',(10.0035870229999,15.2,2.78633380099999));
#197486=CARTESIAN_POINT('Ctrl Pts',(10.0045686949999,15.2,2.78650757299998));
#197487=CARTESIAN_POINT('Ctrl Pts',(10.0055597309999,15.2,2.78668198499999));
#197488=CARTESIAN_POINT('Ctrl Pts',(10.0065601129999,15.2,2.78685701499998));
#197489=CARTESIAN_POINT('Ctrl Pts',(10.0075698159999,15.2,2.78703263999999));
#197490=CARTESIAN_POINT('Ctrl Pts',(10.0085888169999,15.2,2.78720884099998));
#197491=CARTESIAN_POINT('Ctrl Pts',(10.0096170959999,15.2,2.78738559299998));
#197492=CARTESIAN_POINT('Ctrl Pts',(10.0106546299999,15.2,2.78756287699998));
#197493=CARTESIAN_POINT('Ctrl Pts',(10.0117013959999,15.2,2.78774067199999));
#197494=CARTESIAN_POINT('Ctrl Pts',(10.0127573729999,15.2,2.78791895599999));
#197495=CARTESIAN_POINT('Ctrl Pts',(10.0138225379999,15.2,2.78809770699999));
#197496=CARTESIAN_POINT('Ctrl Pts',(10.0148968709999,15.2,2.78827690399999));
#197497=CARTESIAN_POINT('Ctrl Pts',(10.0159803479999,15.2,2.78845652899999));
#197498=CARTESIAN_POINT('Ctrl Pts',(10.0170729509999,15.2,2.78863655799999));
#197499=CARTESIAN_POINT('Ctrl Pts',(10.0181746539999,15.2,2.78881697199999));
#197500=CARTESIAN_POINT('Ctrl Pts',(10.0192854389999,15.2,2.78899774999999));
#197501=CARTESIAN_POINT('Ctrl Pts',(10.0204052839999,15.2,2.78917887199999));
#197502=CARTESIAN_POINT('Ctrl Pts',(10.0215341659999,15.2,2.78936031699998));
#197503=CARTESIAN_POINT('Ctrl Pts',(10.0226720649999,15.2,2.78954206499999));
#197504=CARTESIAN_POINT('Ctrl Pts',(10.0238189609999,15.2,2.78972409599999));
#197505=CARTESIAN_POINT('Ctrl Pts',(10.0249748309999,15.2,2.78990638999999));
#197506=CARTESIAN_POINT('Ctrl Pts',(10.0261396569999,15.2,2.79008892699999));
#197507=CARTESIAN_POINT('Ctrl Pts',(10.0273134139999,15.2,2.79027168599999));
#197508=CARTESIAN_POINT('Ctrl Pts',(10.0284960859999,15.2,2.79045464999999));
#197509=CARTESIAN_POINT('Ctrl Pts',(10.0296876489999,15.2,2.79063779799999));
#197510=CARTESIAN_POINT('Ctrl Pts',(10.0308880829999,15.2,2.79082110899999));
#197511=CARTESIAN_POINT('Ctrl Pts',(10.0320973689999,15.2,2.79100456599998));
#197512=CARTESIAN_POINT('Ctrl Pts',(10.0333154849999,15.2,2.79118814799999));
#197513=CARTESIAN_POINT('Ctrl Pts',(10.0345424119999,15.2,2.79137183599998));
#197514=CARTESIAN_POINT('Ctrl Pts',(10.0357781289999,15.2,2.79155561199998));
#197515=CARTESIAN_POINT('Ctrl Pts',(10.0370226159999,15.2,2.79173945599998));
#197516=CARTESIAN_POINT('Ctrl Pts',(10.0382758529999,15.2,2.79192334999999));
#197517=CARTESIAN_POINT('Ctrl Pts',(10.0395378199999,15.2,2.79210727399998));
#197518=CARTESIAN_POINT('Ctrl Pts',(10.0408084969999,15.2,2.79229120899998));
#197519=CARTESIAN_POINT('Ctrl Pts',(10.0420878649999,15.2,2.79247513699998));
#197520=CARTESIAN_POINT('Ctrl Pts',(10.0433759029999,15.2,2.79265903999999));
#197521=CARTESIAN_POINT('Ctrl Pts',(10.0446725919999,15.2,2.79284289899999));
#197522=CARTESIAN_POINT('Ctrl Pts',(10.0459779129999,15.2,2.79302669599998));
#197523=CARTESIAN_POINT('Ctrl Pts',(10.0472918449999,15.2,2.79321041199999));
#197524=CARTESIAN_POINT('Ctrl Pts',(10.0486143699999,15.2,2.79339402899998));
#197525=CARTESIAN_POINT('Ctrl Pts',(10.0499454679999,15.2,2.79357752799999));
#197526=CARTESIAN_POINT('Ctrl Pts',(10.0512851199999,15.2,2.79376089299999));
#197527=CARTESIAN_POINT('Ctrl Pts',(10.0526333059999,15.2,2.79394410499999));
#197528=CARTESIAN_POINT('Ctrl Pts',(10.0539900079999,15.2,2.79412714599999));
#197529=CARTESIAN_POINT('Ctrl Pts',(10.0553552059999,15.2,2.79430999899999));
#197530=CARTESIAN_POINT('Ctrl Pts',(10.0567288819999,15.2,2.79449264599998));
#197531=CARTESIAN_POINT('Ctrl Pts',(10.0581110159999,15.2,2.79467506799998));
#197532=CARTESIAN_POINT('Ctrl Pts',(10.0595015889999,15.2,2.79485724899998));
#197533=CARTESIAN_POINT('Ctrl Pts',(10.0609005839999,15.2,2.79503916999998));
#197534=CARTESIAN_POINT('Ctrl Pts',(10.0623079809999,15.2,2.79522081599998));
#197535=CARTESIAN_POINT('Ctrl Pts',(10.0637237609999,15.2,2.79540216899999));
#197536=CARTESIAN_POINT('Ctrl Pts',(10.0651479059999,15.2,2.79558321099999));
#197537=CARTESIAN_POINT('Ctrl Pts',(10.0665803979999,15.2,2.79576392499998));
#197538=CARTESIAN_POINT('Ctrl Pts',(10.0680212179999,15.2,2.79594429399998));
#197539=CARTESIAN_POINT('Ctrl Pts',(10.0694703469999,15.2,2.79612430099998));
#197540=CARTESIAN_POINT('Ctrl Pts',(10.0709277689999,15.2,2.79630393099998));
#197541=CARTESIAN_POINT('Ctrl Pts',(10.0723934619999,15.2,2.79648316499999));
#197542=CARTESIAN_POINT('Ctrl Pts',(10.0738674099999,15.2,2.79666198699999));
#197543=CARTESIAN_POINT('Ctrl Pts',(10.0753495959999,15.2,2.79684037999999));
#197544=CARTESIAN_POINT('Ctrl Pts',(10.0768400009999,15.2,2.79701832799999));
#197545=CARTESIAN_POINT('Ctrl Pts',(10.0783386059999,15.2,2.79719581399998));
#197546=CARTESIAN_POINT('Ctrl Pts',(10.0798453939999,15.2,2.79737282199999));
#197547=CARTESIAN_POINT('Ctrl Pts',(10.0813603479999,15.2,2.79754933599998));
#197548=CARTESIAN_POINT('Ctrl Pts',(10.0828834479999,15.2,2.79772533899998));
#197549=CARTESIAN_POINT('Ctrl Pts',(10.0844146779999,15.2,2.79790081599998));
#197550=CARTESIAN_POINT('Ctrl Pts',(10.0859540199999,15.2,2.79807574899999));
#197551=CARTESIAN_POINT('Ctrl Pts',(10.0875014559999,15.2,2.79825012399999));
#197552=CARTESIAN_POINT('Ctrl Pts',(10.0890569699999,15.2,2.79842392399999));
#197553=CARTESIAN_POINT('Ctrl Pts',(10.0906205419999,15.2,2.79859713299999));
#197554=CARTESIAN_POINT('Ctrl Pts',(10.0921921569999,15.2,2.79876973499999));
#197555=CARTESIAN_POINT('Ctrl Pts',(10.0937717949999,15.2,2.79894171599998));
#197556=CARTESIAN_POINT('Ctrl Pts',(10.0953594409999,15.2,2.79911305799998));
#197557=CARTESIAN_POINT('Ctrl Pts',(10.0969550769999,15.2,2.79928374699999));
#197558=CARTESIAN_POINT('Ctrl Pts',(10.0985586869999,15.2,2.79945376699998));
#197559=CARTESIAN_POINT('Ctrl Pts',(10.1001702509999,15.2,2.79962310199998));
#197560=CARTESIAN_POINT('Ctrl Pts',(10.1017897539999,15.2,2.79979173799998));
#197561=CARTESIAN_POINT('Ctrl Pts',(10.1034171789999,15.2,2.79995965799999));
#197562=CARTESIAN_POINT('Ctrl Pts',(10.1050525089999,15.2,2.80012684799999));
#197563=CARTESIAN_POINT('Ctrl Pts',(10.1066957249999,15.2,2.80029329299998));
#197564=CARTESIAN_POINT('Ctrl Pts',(10.1083468139999,15.2,2.80045897699999));
#197565=CARTESIAN_POINT('Ctrl Pts',(10.1100057559999,15.2,2.80062388499999));
#197566=CARTESIAN_POINT('Ctrl Pts',(10.1116725359999,15.2,2.80078800299999));
#197567=CARTESIAN_POINT('Ctrl Pts',(10.1133471369999,15.2,2.80095131499999));
#197568=CARTESIAN_POINT('Ctrl Pts',(10.1150295409999,15.2,2.80111380599998));
#197569=CARTESIAN_POINT('Ctrl Pts',(10.1167197329999,15.2,2.80127546199999));
#197570=CARTESIAN_POINT('Ctrl Pts',(10.1184176969999,15.2,2.80143626899999));
#197571=CARTESIAN_POINT('Ctrl Pts',(10.1201234149999,15.2,2.80159621099998));
#197572=CARTESIAN_POINT('Ctrl Pts',(10.1218368709999,15.2,2.80175527399999));
#197573=CARTESIAN_POINT('Ctrl Pts',(10.1235580499999,15.2,2.80191344299999));
#197574=CARTESIAN_POINT('Ctrl Pts',(10.1252869329999,15.2,2.80207070399998));
#197575=CARTESIAN_POINT('Ctrl Pts',(10.1270235059999,15.2,2.80222704299998));
#197576=CARTESIAN_POINT('Ctrl Pts',(10.1287677519999,15.2,2.80238244599998));
#197577=CARTESIAN_POINT('Ctrl Pts',(10.1305196549999,15.2,2.80253689599999));
#197578=CARTESIAN_POINT('Ctrl Pts',(10.1322791999999,15.2,2.80269038199998));
#197579=CARTESIAN_POINT('Ctrl Pts',(10.1340463689999,15.2,2.80284288899999));
#197580=CARTESIAN_POINT('Ctrl Pts',(10.1358211459999,15.2,2.80299440199999));
#197581=CARTESIAN_POINT('Ctrl Pts',(10.1376035179999,15.2,2.80314490699999));
#197582=CARTESIAN_POINT('Ctrl Pts',(10.1393934659999,15.2,2.80329439199999));
#197583=CARTESIAN_POINT('Ctrl Pts',(10.1411909749999,15.2,2.80344284099999));
#197584=CARTESIAN_POINT('Ctrl Pts',(10.1429960289999,15.2,2.80359023999999));
#197585=CARTESIAN_POINT('Ctrl Pts',(10.1448086139999,15.2,2.80373657799998));
#197586=CARTESIAN_POINT('Ctrl Pts',(10.1466287129999,15.2,2.80388183699999));
#197587=CARTESIAN_POINT('Ctrl Pts',(10.1484563089999,15.2,2.80402600799999));
#197588=CARTESIAN_POINT('Ctrl Pts',(10.1502913879999,15.2,2.80416907399999));
#197589=CARTESIAN_POINT('Ctrl Pts',(10.1521339339999,15.2,2.80431102199999));
#197590=CARTESIAN_POINT('Ctrl Pts',(10.1539839329999,15.2,2.80445183999999));
#197591=CARTESIAN_POINT('Ctrl Pts',(10.1558413669999,15.2,2.80459151299999));
#197592=CARTESIAN_POINT('Ctrl Pts',(10.1577062229999,15.2,2.80473002899999));
#197593=CARTESIAN_POINT('Ctrl Pts',(10.1595784839999,15.2,2.80486737399999));
#197594=CARTESIAN_POINT('Ctrl Pts',(10.1614581339999,15.2,2.80500353399999));
#197595=CARTESIAN_POINT('Ctrl Pts',(10.1633451609999,15.2,2.80513849699998));
#197596=CARTESIAN_POINT('Ctrl Pts',(10.1652395459999,15.2,2.80527224899998));
#197597=CARTESIAN_POINT('Ctrl Pts',(10.1671412759999,15.2,2.80540477799998));
#197598=CARTESIAN_POINT('Ctrl Pts',(10.1690503349999,15.2,2.80553606899999));
#197599=CARTESIAN_POINT('Ctrl Pts',(10.1709667089999,15.2,2.80566611099999));
#197600=CARTESIAN_POINT('Ctrl Pts',(10.1728903809999,15.2,2.80579489099999));
#197601=CARTESIAN_POINT('Ctrl Pts',(10.1748213379999,15.2,2.80592239499998));
#197602=CARTESIAN_POINT('Ctrl Pts',(10.1767595639999,15.2,2.80604860999999));
#197603=CARTESIAN_POINT('Ctrl Pts',(10.1787050449999,15.2,2.80617352499998));
#197604=CARTESIAN_POINT('Ctrl Pts',(10.1806577639999,15.2,2.80629712499999));
#197605=CARTESIAN_POINT('Ctrl Pts',(10.1826177079999,15.2,2.80641939899999));
#197606=CARTESIAN_POINT('Ctrl Pts',(10.1845848629999,15.2,2.80654033399999));
#197607=CARTESIAN_POINT('Ctrl Pts',(10.1865592119999,15.2,2.80665991699999));
#197608=CARTESIAN_POINT('Ctrl Pts',(10.1885407419999,15.2,2.80677813699998));
#197609=CARTESIAN_POINT('Ctrl Pts',(10.1905294369999,15.2,2.80689497899999));
#197610=CARTESIAN_POINT('Ctrl Pts',(10.1925252829999,15.2,2.80701043199999));
#197611=CARTESIAN_POINT('Ctrl Pts',(10.1945282669999,15.2,2.80712448399999));
#197612=CARTESIAN_POINT('Ctrl Pts',(10.1965383709999,15.2,2.80723712199999));
#197613=CARTESIAN_POINT('Ctrl Pts',(10.1985555829999,15.2,2.80734833399999));
#197614=CARTESIAN_POINT('Ctrl Pts',(10.2005798889999,15.2,2.80745810899998));
#197615=CARTESIAN_POINT('Ctrl Pts',(10.2026112719999,15.2,2.80756643299998));
#197616=CARTESIAN_POINT('Ctrl Pts',(10.2046497199999,15.2,2.80767329399998));
#197617=CARTESIAN_POINT('Ctrl Pts',(10.2066952179999,15.2,2.80777868099998));
#197618=CARTESIAN_POINT('Ctrl Pts',(10.2087477509999,15.2,2.80788258099999));
#197619=CARTESIAN_POINT('Ctrl Pts',(10.2108073059999,15.2,2.80798498399999));
#197620=CARTESIAN_POINT('Ctrl Pts',(10.2128738679999,15.2,2.80808587499998));
#197621=CARTESIAN_POINT('Ctrl Pts',(10.2149474219999,15.2,2.80818524499999));
#197622=CARTESIAN_POINT('Ctrl Pts',(10.2170279549999,15.2,2.80828308099998));
#197623=CARTESIAN_POINT('Ctrl Pts',(10.2191154529999,15.2,2.80837936999998));
#197624=CARTESIAN_POINT('Ctrl Pts',(10.2212099009999,15.2,2.80847410299998));
#197625=CARTESIAN_POINT('Ctrl Pts',(10.2233112869999,15.2,2.80856726499999));
#197626=CARTESIAN_POINT('Ctrl Pts',(10.2254195939999,15.2,2.80865884799999));
#197627=CARTESIAN_POINT('Ctrl Pts',(10.2275348109999,15.2,2.80874883799999));
#197628=CARTESIAN_POINT('Ctrl Pts',(10.2296569209999,15.2,2.80883722299999));
#197629=CARTESIAN_POINT('Ctrl Pts',(10.2317859129999,15.2,2.80892399399999));
#197630=CARTESIAN_POINT('Ctrl Pts',(10.2339217719999,15.2,2.80900913799999));
#197631=CARTESIAN_POINT('Ctrl Pts',(10.2360644839999,15.2,2.80909264399998));
#197632=CARTESIAN_POINT('Ctrl Pts',(10.2382140349999,15.2,2.80917449999999));
#197633=CARTESIAN_POINT('Ctrl Pts',(10.2403704109999,15.2,2.80925469399998));
#197634=CARTESIAN_POINT('Ctrl Pts',(10.2425335999999,15.2,2.80933321799999));
#197635=CARTESIAN_POINT('Ctrl Pts',(10.2447035879999,15.2,2.80941005799999));
#197636=CARTESIAN_POINT('Ctrl Pts',(10.2468803589999,15.2,2.80948520299999));
#197637=CARTESIAN_POINT('Ctrl Pts',(10.2490639019999,15.2,2.80955864199999));
#197638=CARTESIAN_POINT('Ctrl Pts',(10.2512542019999,15.2,2.80963036499998));
#197639=CARTESIAN_POINT('Ctrl Pts',(10.2534512459999,15.2,2.80970035899998));
#197640=CARTESIAN_POINT('Ctrl Pts',(10.2556550209999,15.2,2.80976861599999));
#197641=CARTESIAN_POINT('Ctrl Pts',(10.2578655119999,15.2,2.80983512099999));
#197642=CARTESIAN_POINT('Ctrl Pts',(10.2600827069999,15.2,2.80989986699999));
#197643=CARTESIAN_POINT('Ctrl Pts',(10.2623065929999,15.2,2.80996284199999));
#197644=CARTESIAN_POINT('Ctrl Pts',(10.2645371559999,15.2,2.81002403399999));
#197645=CARTESIAN_POINT('Ctrl Pts',(10.2667743819999,15.2,2.81008343199999));
#197646=CARTESIAN_POINT('Ctrl Pts',(10.2690182579999,15.2,2.81014102599999));
#197647=CARTESIAN_POINT('Ctrl Pts',(10.2712687709999,15.2,2.81019680599999));
#197648=CARTESIAN_POINT('Ctrl Pts',(10.2735259089999,15.2,2.81025076199998));
#197649=CARTESIAN_POINT('Ctrl Pts',(10.2757896559999,15.2,2.81030288099998));
#197650=CARTESIAN_POINT('Ctrl Pts',(10.2780600009999,15.2,2.81035315199999));
#197651=CARTESIAN_POINT('Ctrl Pts',(10.2803369309999,15.2,2.81040156799998));
#197652=CARTESIAN_POINT('Ctrl Pts',(10.2826204319999,15.2,2.81044811699999));
#197653=CARTESIAN_POINT('Ctrl Pts',(10.2849104899999,15.2,2.81049278699999));
#197654=CARTESIAN_POINT('Ctrl Pts',(10.2872070959999,15.2,2.81053556799999));
#197655=CARTESIAN_POINT('Ctrl Pts',(10.2895102319999,15.2,2.81057645199999));
#197656=CARTESIAN_POINT('Ctrl Pts',(10.2918198869999,15.2,2.81061542499998));
#197657=CARTESIAN_POINT('Ctrl Pts',(10.2941360499999,15.2,2.81065247899999));
#197658=CARTESIAN_POINT('Ctrl Pts',(10.2964587039999,15.2,2.81068760399998));
#197659=CARTESIAN_POINT('Ctrl Pts',(10.2987878399999,15.2,2.81072078899999));
#197660=CARTESIAN_POINT('Ctrl Pts',(10.3011234449999,15.2,2.81075202499999));
#197661=CARTESIAN_POINT('Ctrl Pts',(10.3034655029999,15.2,2.81078129899999));
#197662=CARTESIAN_POINT('Ctrl Pts',(10.3058140039999,15.2,2.81080860299999));
#197663=CARTESIAN_POINT('Ctrl Pts',(10.3081689339999,15.2,2.81083392699998));
#197664=CARTESIAN_POINT('Ctrl Pts',(10.3105302809999,15.2,2.81085726199999));
#197665=CARTESIAN_POINT('Ctrl Pts',(10.3128980319999,15.2,2.81087859499999));
#197666=CARTESIAN_POINT('Ctrl Pts',(10.3152721739999,15.2,2.81089791699999));
#197667=CARTESIAN_POINT('Ctrl Pts',(10.3176526949999,15.2,2.81091521999999));
#197668=CARTESIAN_POINT('Ctrl Pts',(10.3200395829999,15.2,2.81093049299999));
#197669=CARTESIAN_POINT('Ctrl Pts',(10.3224328229999,15.2,2.81094372499999));
#197670=CARTESIAN_POINT('Ctrl Pts',(10.3248324049999,15.2,2.81095490799999));
#197671=CARTESIAN_POINT('Ctrl Pts',(10.3272383149999,15.2,2.81096403199999));
#197672=CARTESIAN_POINT('Ctrl Pts',(10.3296505419999,15.2,2.81097108499999));
#197673=CARTESIAN_POINT('Ctrl Pts',(10.3320690709999,15.2,2.81097606099999));
#197674=CARTESIAN_POINT('Ctrl Pts',(10.3344938929999,15.2,2.81097894699998));
#197675=CARTESIAN_POINT('Ctrl Pts',(10.3369249929999,15.2,2.81097973599999));
#197676=CARTESIAN_POINT('Ctrl Pts',(10.3393623599999,15.2,2.81097841599999));
#197677=CARTESIAN_POINT('Ctrl Pts',(10.3418059809999,15.2,2.81097497899999));
#197678=CARTESIAN_POINT('Ctrl Pts',(10.3442558419999,15.2,2.81096941599999));
#197679=CARTESIAN_POINT('Ctrl Pts',(10.3467119339999,15.2,2.81096171499998));
#197680=CARTESIAN_POINT('Ctrl Pts',(10.3491742439999,15.2,2.81095186899999));
#197681=CARTESIAN_POINT('Ctrl Pts',(10.3516427589999,15.2,2.81093986799998));
#197682=CARTESIAN_POINT('Ctrl Pts',(10.3541174659999,15.2,2.81092570199998));
#197683=CARTESIAN_POINT('Ctrl Pts',(10.3565983529999,15.2,2.81090936199998));
#197684=CARTESIAN_POINT('Ctrl Pts',(10.3590854099999,15.2,2.81089083999999));
#197685=CARTESIAN_POINT('Ctrl Pts',(10.3615786239999,15.2,2.81087012399999));
#197686=CARTESIAN_POINT('Ctrl Pts',(10.3640779799999,15.2,2.81084720699998));
#197687=CARTESIAN_POINT('Ctrl Pts',(10.3665834699999,15.2,2.81082207899999));
#197688=CARTESIAN_POINT('Ctrl Pts',(10.3690950799999,15.2,2.81079473099999));
#197689=CARTESIAN_POINT('Ctrl Pts',(10.3716127979999,15.2,2.81076515299999));
#197690=CARTESIAN_POINT('Ctrl Pts',(10.3741366129999,15.2,2.81073333699998));
#197691=CARTESIAN_POINT('Ctrl Pts',(10.3766665119999,15.2,2.81069927299999));
#197692=CARTESIAN_POINT('Ctrl Pts',(10.3792024839999,15.2,2.81066295399999));
#197693=CARTESIAN_POINT('Ctrl Pts',(10.3817445159999,15.2,2.81062436799999));
#197694=CARTESIAN_POINT('Ctrl Pts',(10.3842925959999,15.2,2.81058350899999));
#197695=CARTESIAN_POINT('Ctrl Pts',(10.3868467139999,15.2,2.81054036599999));
#197696=CARTESIAN_POINT('Ctrl Pts',(10.3894068559999,15.2,2.81049492999998));
#197697=CARTESIAN_POINT('Ctrl Pts',(10.3919730119999,15.2,2.81044719399999));
#197698=CARTESIAN_POINT('Ctrl Pts',(10.3945451689999,15.2,2.81039714699999));
#197699=CARTESIAN_POINT('Ctrl Pts',(10.3971233149999,15.2,2.81034478199999));
#197700=CARTESIAN_POINT('Ctrl Pts',(10.3997074399999,15.2,2.81029008999998));
#197701=CARTESIAN_POINT('Ctrl Pts',(10.4022975309999,15.2,2.81023305999998));
#197702=CARTESIAN_POINT('Ctrl Pts',(10.4048935769999,15.2,2.81017368599999));
#197703=CARTESIAN_POINT('Ctrl Pts',(10.4074955649999,15.2,2.81011195799999));
#197704=CARTESIAN_POINT('Ctrl Pts',(10.4101034849999,15.2,2.81004786799999));
#197705=CARTESIAN_POINT('Ctrl Pts',(10.4127173239999,15.2,2.80998140599999));
#197706=CARTESIAN_POINT('Ctrl Pts',(10.4153370719999,15.2,2.80991256599999));
#197707=CARTESIAN_POINT('Ctrl Pts',(10.4179627159999,15.2,2.80984133699998));
#197708=CARTESIAN_POINT('Ctrl Pts',(10.4205942449999,15.2,2.80976771199998));
#197709=CARTESIAN_POINT('Ctrl Pts',(10.4232316479999,15.2,2.80969167999999));
#197710=CARTESIAN_POINT('Ctrl Pts',(10.4258749129999,15.2,2.80961323599998));
#197711=CARTESIAN_POINT('Ctrl Pts',(10.4285240289999,15.2,2.80953237099999));
#197712=CARTESIAN_POINT('Ctrl Pts',(10.4311789839999,15.2,2.80944907299999));
#197713=CARTESIAN_POINT('Ctrl Pts',(10.4338397659999,15.2,2.80936333799998));
#197714=CARTESIAN_POINT('Ctrl Pts',(10.4365063659999,15.2,2.80927515599998));
#197715=CARTESIAN_POINT('Ctrl Pts',(10.4391787699999,15.2,2.80918451599998));
#197716=CARTESIAN_POINT('Ctrl Pts',(10.4418569669999,15.2,2.80909141499999));
#197717=CARTESIAN_POINT('Ctrl Pts',(10.4445409479999,15.2,2.80899584099998));
#197718=CARTESIAN_POINT('Ctrl Pts',(10.4472306989999,15.2,2.80889778599998));
#197719=CARTESIAN_POINT('Ctrl Pts',(10.4499262109999,15.2,2.80879724399998));
#197720=CARTESIAN_POINT('Ctrl Pts',(10.4526274699999,15.2,2.80869420399998));
#197721=CARTESIAN_POINT('Ctrl Pts',(10.4553344669999,15.2,2.80858866099998));
#197722=CARTESIAN_POINT('Ctrl Pts',(10.4580471909999,15.2,2.80848060399999));
#197723=CARTESIAN_POINT('Ctrl Pts',(10.4607656289999,15.2,2.80837002599998));
#197724=CARTESIAN_POINT('Ctrl Pts',(10.4634897709999,15.2,2.80825691999999));
#197725=CARTESIAN_POINT('Ctrl Pts',(10.4662196059999,15.2,2.80814127499998));
#197726=CARTESIAN_POINT('Ctrl Pts',(10.4689551229999,15.2,2.80802308599998));
#197727=CARTESIAN_POINT('Ctrl Pts',(10.4716963109999,15.2,2.80790234499998));
#197728=CARTESIAN_POINT('Ctrl Pts',(10.4744431569999,15.2,2.80777904299998));
#197729=CARTESIAN_POINT('Ctrl Pts',(10.4771956519999,15.2,2.80765317099998));
#197730=CARTESIAN_POINT('Ctrl Pts',(10.4799537849999,15.2,2.80752472299999));
#197731=CARTESIAN_POINT('Ctrl Pts',(10.4827175439999,15.2,2.80739368999999));
#197732=CARTESIAN_POINT('Ctrl Pts',(10.4854869179999,15.2,2.80726006499999));
#197733=CARTESIAN_POINT('Ctrl Pts',(10.4882618969999,15.2,2.80712383899999));
#197734=CARTESIAN_POINT('Ctrl Pts',(10.4910424679999,15.2,2.80698500599998));
#197735=CARTESIAN_POINT('Ctrl Pts',(10.4938286229999,15.2,2.80684355699999));
#197736=CARTESIAN_POINT('Ctrl Pts',(10.4966203499999,15.2,2.80669948499998));
#197737=CARTESIAN_POINT('Ctrl Pts',(10.4994176369999,15.2,2.80655278099999));
#197738=CARTESIAN_POINT('Ctrl Pts',(10.5022204749999,15.2,2.80640343899999));
#197739=CARTESIAN_POINT('Ctrl Pts',(10.5050288509999,15.2,2.80625144999998));
#197740=CARTESIAN_POINT('Ctrl Pts',(10.5078427569999,15.2,2.80609680699998));
#197741=CARTESIAN_POINT('Ctrl Pts',(10.5106621789999,15.2,2.80593950299998));
#197742=CARTESIAN_POINT('Ctrl Pts',(10.5134871079999,15.2,2.80577952899999));
#197743=CARTESIAN_POINT('Ctrl Pts',(10.5163175329999,15.2,2.80561687899999));
#197744=CARTESIAN_POINT('Ctrl Pts',(10.5191534429999,15.2,2.80545154499999));
#197745=CARTESIAN_POINT('Ctrl Pts',(10.5219948289999,15.2,2.80528351899999));
#197746=CARTESIAN_POINT('Ctrl Pts',(10.5248416769999,15.2,2.80511279299999));
#197747=CARTESIAN_POINT('Ctrl Pts',(10.5276939799999,15.2,2.80493936099998));
#197748=CARTESIAN_POINT('Ctrl Pts',(10.5305517249999,15.2,2.80476321599998));
#197749=CARTESIAN_POINT('Ctrl Pts',(10.5334149019999,15.2,2.80458434899998));
#197750=CARTESIAN_POINT('Ctrl Pts',(10.5362834999999,15.2,2.80440275299998));
#197751=CARTESIAN_POINT('Ctrl Pts',(10.5391575079999,15.2,2.80421842099998));
#197752=CARTESIAN_POINT('Ctrl Pts',(10.5420369179999,15.2,2.80403134499998));
#197753=CARTESIAN_POINT('Ctrl Pts',(10.5449217159999,15.2,2.80384151899998));
#197754=CARTESIAN_POINT('Ctrl Pts',(10.5478118939999,15.2,2.80364893599998));
#197755=CARTESIAN_POINT('Ctrl Pts',(10.5507074409999,15.2,2.80345358699999));
#197756=CARTESIAN_POINT('Ctrl Pts',(10.5536083449999,15.2,2.80325546599999));
#197757=CARTESIAN_POINT('Ctrl Pts',(10.5565145969999,15.2,2.80305456499998));
#197758=CARTESIAN_POINT('Ctrl Pts',(10.5594261859999,15.2,2.80285087799999));
#197759=CARTESIAN_POINT('Ctrl Pts',(10.5623431029999,15.2,2.80264439699998));
#197760=CARTESIAN_POINT('Ctrl Pts',(10.5652653349999,15.2,2.80243511499998));
#197761=CARTESIAN_POINT('Ctrl Pts',(10.5681928729999,15.2,2.80222302499999));
#197762=CARTESIAN_POINT('Ctrl Pts',(10.5711257059999,15.2,2.80200812099999));
#197763=CARTESIAN_POINT('Ctrl Pts',(10.5740638259999,15.2,2.80179039399999));
#197764=CARTESIAN_POINT('Ctrl Pts',(10.5770072199999,15.2,2.80156983799999));
#197765=CARTESIAN_POINT('Ctrl Pts',(10.5799558779999,15.2,2.80134644699999));
#197766=CARTESIAN_POINT('Ctrl Pts',(10.5829097899999,15.2,2.80112021299999));
#197767=CARTESIAN_POINT('Ctrl Pts',(10.5858689469999,15.2,2.80089112799998));
#197768=CARTESIAN_POINT('Ctrl Pts',(10.5888333369999,15.2,2.80065918699999));
#197769=CARTESIAN_POINT('Ctrl Pts',(10.5918029509999,15.2,2.80042438199998));
#197770=CARTESIAN_POINT('Ctrl Pts',(10.5947777769999,15.2,2.80018670699998));
#197771=CARTESIAN_POINT('Ctrl Pts',(10.5977578069999,15.2,2.79994615399998));
#197772=CARTESIAN_POINT('Ctrl Pts',(10.6007430289999,15.2,2.79970271699998));
#197773=CARTESIAN_POINT('Ctrl Pts',(10.6037334349999,15.2,2.79945638899999));
#197774=CARTESIAN_POINT('Ctrl Pts',(10.6067290119999,15.2,2.79920716299999));
#197775=CARTESIAN_POINT('Ctrl Pts',(10.6097297519999,15.2,2.79895503299999));
#197776=CARTESIAN_POINT('Ctrl Pts',(10.6127356429999,15.2,2.79869999199998));
#197777=CARTESIAN_POINT('Ctrl Pts',(10.6157466779999,15.2,2.79844203299999));
#197778=CARTESIAN_POINT('Ctrl Pts',(10.6187628439999,15.2,2.79818114899999));
#197779=CARTESIAN_POINT('Ctrl Pts',(10.6217841319999,15.2,2.79791733399998));
#197780=CARTESIAN_POINT('Ctrl Pts',(10.6248105309999,15.2,2.79765058099999));
#197781=CARTESIAN_POINT('Ctrl Pts',(10.6278420329999,15.2,2.79738088399998));
#197782=CARTESIAN_POINT('Ctrl Pts',(10.6308786259999,15.2,2.79710823499999));
#197783=CARTESIAN_POINT('Ctrl Pts',(10.6339203009999,15.2,2.79683262899999));
#197784=CARTESIAN_POINT('Ctrl Pts',(10.6369670479999,15.2,2.79655405899998));
#197785=CARTESIAN_POINT('Ctrl Pts',(10.6400188569999,15.2,2.79627251799998));
#197786=CARTESIAN_POINT('Ctrl Pts',(10.6430757179999,15.2,2.79598799899999));
#197787=CARTESIAN_POINT('Ctrl Pts',(10.6461376199999,15.2,2.79570049699998));
#197788=CARTESIAN_POINT('Ctrl Pts',(10.6492045549999,15.2,2.79541000599998));
#197789=CARTESIAN_POINT('Ctrl Pts',(10.6522765109999,15.2,2.79511651699998));
#197790=CARTESIAN_POINT('Ctrl Pts',(10.6553534799999,15.2,2.79482002499999));
#197791=CARTESIAN_POINT('Ctrl Pts',(10.6584354509999,15.2,2.79452052399999));
#197792=CARTESIAN_POINT('Ctrl Pts',(10.6615224159999,15.2,2.79421800799999));
#197793=CARTESIAN_POINT('Ctrl Pts',(10.6646143609999,15.2,2.79391246899999));
#197794=CARTESIAN_POINT('Ctrl Pts',(10.6677112809999,15.2,2.79360390199999));
#197795=CARTESIAN_POINT('Ctrl Pts',(10.6708131629999,15.2,2.79329229999998));
#197796=CARTESIAN_POINT('Ctrl Pts',(10.6739199989999,15.2,2.79297765699998));
#197797=CARTESIAN_POINT('Ctrl Pts',(10.6770317779999,15.2,2.79265996699999));
#197798=CARTESIAN_POINT('Ctrl Pts',(10.6801484919999,15.2,2.79233922399998));
#197799=CARTESIAN_POINT('Ctrl Pts',(10.6832701279999,15.2,2.79201541999999));
#197800=CARTESIAN_POINT('Ctrl Pts',(10.6863966799999,15.2,2.79168855099999));
#197801=CARTESIAN_POINT('Ctrl Pts',(10.6895281349999,15.2,2.79135860899999));
#197802=CARTESIAN_POINT('Ctrl Pts',(10.6926644859999,15.2,2.79102558999998));
#197803=CARTESIAN_POINT('Ctrl Pts',(10.6958057219999,15.2,2.79068948499999));
#197804=CARTESIAN_POINT('Ctrl Pts',(10.6989518329999,15.2,2.79035029099998));
#197805=CARTESIAN_POINT('Ctrl Pts',(10.7021028099999,15.2,2.79000799999999));
#197806=CARTESIAN_POINT('Ctrl Pts',(10.7052586439999,15.2,2.78966260699999));
#197807=CARTESIAN_POINT('Ctrl Pts',(10.7084193239999,15.2,2.78931410399998));
#197808=CARTESIAN_POINT('Ctrl Pts',(10.7115848429999,15.2,2.78896248699999));
#197809=CARTESIAN_POINT('Ctrl Pts',(10.7147551869999,15.2,2.78860774899999));
#197810=CARTESIAN_POINT('Ctrl Pts',(10.7179303499999,15.2,2.78824988399998));
#197811=CARTESIAN_POINT('Ctrl Pts',(10.7211103209999,15.2,2.78788888599999));
#197812=CARTESIAN_POINT('Ctrl Pts',(10.7242950909999,15.2,2.78752475099999));
#197813=CARTESIAN_POINT('Ctrl Pts',(10.7274846509999,15.2,2.78715746999998));
#197814=CARTESIAN_POINT('Ctrl Pts',(10.7306789899999,15.2,2.78678703799999));
#197815=CARTESIAN_POINT('Ctrl Pts',(10.7338780989999,15.2,2.78641344999999));
#197816=CARTESIAN_POINT('Ctrl Pts',(10.7370819699999,15.2,2.78603669899999));
#197817=CARTESIAN_POINT('Ctrl Pts',(10.7402905919999,15.2,2.78565678199998));
#197818=CARTESIAN_POINT('Ctrl Pts',(10.7435039549999,15.2,2.78527368799999));
#197819=CARTESIAN_POINT('Ctrl Pts',(10.7467220519999,15.2,2.78488741599999));
#197820=CARTESIAN_POINT('Ctrl Pts',(10.7499448709999,15.2,2.78449795899999));
#197821=CARTESIAN_POINT('Ctrl Pts',(10.7531724039999,15.2,2.78410530999999));
#197822=CARTESIAN_POINT('Ctrl Pts',(10.7564046409999,15.2,2.78370946299999));
#197823=CARTESIAN_POINT('Ctrl Pts',(10.7596415739999,15.2,2.78331041399999));
#197824=CARTESIAN_POINT('Ctrl Pts',(10.7628831919999,15.2,2.78290815599998));
#197825=CARTESIAN_POINT('Ctrl Pts',(10.7661294859999,15.2,2.78250268399999));
#197826=CARTESIAN_POINT('Ctrl Pts',(10.7693804469999,15.2,2.78209399099998));
#197827=CARTESIAN_POINT('Ctrl Pts',(10.7726360659999,15.2,2.78168207299998));
#197828=CARTESIAN_POINT('Ctrl Pts',(10.7758963329999,15.2,2.78126692399999));
#197829=CARTESIAN_POINT('Ctrl Pts',(10.7791612379999,15.2,2.78084853699998));
#197830=CARTESIAN_POINT('Ctrl Pts',(10.7824307749999,15.2,2.78042690799998));
#197831=CARTESIAN_POINT('Ctrl Pts',(10.7857049309999,15.2,2.78000203199999));
#197832=CARTESIAN_POINT('Ctrl Pts',(10.7889836979999,15.2,2.77957390099999));
#197833=CARTESIAN_POINT('Ctrl Pts',(10.7922670679999,15.2,2.77914250999999));
#197834=CARTESIAN_POINT('Ctrl Pts',(10.7955550299999,15.2,2.77870785499999));
#197835=CARTESIAN_POINT('Ctrl Pts',(10.7988475759999,15.2,2.77826992999999));
#197836=CARTESIAN_POINT('Ctrl Pts',(10.8021446959999,15.2,2.77782872899999));
#197837=CARTESIAN_POINT('Ctrl Pts',(10.8054463819999,15.2,2.77738424699999));
#197838=CARTESIAN_POINT('Ctrl Pts',(10.8087526239999,15.2,2.77693647799998));
#197839=CARTESIAN_POINT('Ctrl Pts',(10.8120634119999,15.2,2.77648541599999));
#197840=CARTESIAN_POINT('Ctrl Pts',(10.8153787389999,15.2,2.77603105699999));
#197841=CARTESIAN_POINT('Ctrl Pts',(10.8186985939999,15.2,2.77557339599999));
#197842=CARTESIAN_POINT('Ctrl Pts',(10.8220229679999,15.2,2.77511242599999));
#197843=CARTESIAN_POINT('Ctrl Pts',(10.8253518549999,15.2,2.77464814099999));
#197844=CARTESIAN_POINT('Ctrl Pts',(10.8286852409999,15.2,2.77418053799998));
#197845=CARTESIAN_POINT('Ctrl Pts',(10.8320231199999,15.2,2.77370960999999));
#197846=CARTESIAN_POINT('Ctrl Pts',(10.8353654819999,15.2,2.77323535299999));
#197847=CARTESIAN_POINT('Ctrl Pts',(10.8387123189999,15.2,2.77275775999998));
#197848=CARTESIAN_POINT('Ctrl Pts',(10.8420636209999,15.2,2.77227682699999));
#197849=CARTESIAN_POINT('Ctrl Pts',(10.8454193789999,15.2,2.77179254799999));
#197850=CARTESIAN_POINT('Ctrl Pts',(10.8487795839999,15.2,2.77130491799999));
#197851=CARTESIAN_POINT('Ctrl Pts',(10.8521442279999,15.2,2.77081393199998));
#197852=CARTESIAN_POINT('Ctrl Pts',(10.8555133009999,15.2,2.77031958499999));
#197853=CARTESIAN_POINT('Ctrl Pts',(10.8588867929999,15.2,2.76982187099998));
#197854=CARTESIAN_POINT('Ctrl Pts',(10.8622646979999,15.2,2.76932078499998));
#197855=CARTESIAN_POINT('Ctrl Pts',(10.8656470049999,15.2,2.76881632399999));
#197856=CARTESIAN_POINT('Ctrl Pts',(10.8690337059999,15.2,2.76830847799998));
#197857=CARTESIAN_POINT('Ctrl Pts',(10.8724247909999,15.2,2.76779724699999));
#197858=CARTESIAN_POINT('Ctrl Pts',(10.8758202519999,15.2,2.76728262299999));
#197859=CARTESIAN_POINT('Ctrl Pts',(10.8792200789999,15.2,2.76676460199998));
#197860=CARTESIAN_POINT('Ctrl Pts',(10.8826242649999,15.2,2.76624317899999));
#197861=CARTESIAN_POINT('Ctrl Pts',(10.8860327999999,15.2,2.76571834699999));
#197862=CARTESIAN_POINT('Ctrl Pts',(10.8894456749999,15.2,2.76519010299998));
#197863=CARTESIAN_POINT('Ctrl Pts',(10.8928628809999,15.2,2.76465844099998));
#197864=CARTESIAN_POINT('Ctrl Pts',(10.8962844109999,15.2,2.76412335799999));
#197865=CARTESIAN_POINT('Ctrl Pts',(10.8997102529999,15.2,2.76358484599999));
#197866=CARTESIAN_POINT('Ctrl Pts',(10.9031404009999,15.2,2.76304290199998));
#197867=CARTESIAN_POINT('Ctrl Pts',(10.9065748449999,15.2,2.76249751999998));
#197868=CARTESIAN_POINT('Ctrl Pts',(10.9100135769999,15.2,2.76194869599999));
#197869=CARTESIAN_POINT('Ctrl Pts',(10.9134565879999,15.2,2.76139642399999));
#197870=CARTESIAN_POINT('Ctrl Pts',(10.9169038679999,15.2,2.76084069999998));
#197871=CARTESIAN_POINT('Ctrl Pts',(10.9203554099999,15.2,2.76028151899999));
#197872=CARTESIAN_POINT('Ctrl Pts',(10.9238112039999,15.2,2.75971887599999));
#197873=CARTESIAN_POINT('Ctrl Pts',(10.9272712419999,15.2,2.75915276599999));
#197874=CARTESIAN_POINT('Ctrl Pts',(10.9307355149999,15.2,2.75858318399998));
#197875=CARTESIAN_POINT('Ctrl Pts',(10.9342040149999,15.2,2.75801012499999));
#197876=CARTESIAN_POINT('Ctrl Pts',(10.9376767319999,15.2,2.75743358499999));
#197877=CARTESIAN_POINT('Ctrl Pts',(10.9411536579999,15.2,2.75685355899999));
#197878=CARTESIAN_POINT('Ctrl Pts',(10.9446347859999,15.2,2.75627004099999));
#197879=CARTESIAN_POINT('Ctrl Pts',(10.9481201049999,15.2,2.75568302799999));
#197880=CARTESIAN_POINT('Ctrl Pts',(10.9516096059999,15.2,2.75509251399999));
#197881=CARTESIAN_POINT('Ctrl Pts',(10.9551032829999,15.2,2.75449849499999));
#197882=CARTESIAN_POINT('Ctrl Pts',(10.9586011259999,15.2,2.75390096599998));
#197883=CARTESIAN_POINT('Ctrl Pts',(10.9621031259999,15.2,2.75329992099999));
#197884=CARTESIAN_POINT('Ctrl Pts',(10.9656092739999,15.2,2.75269535799998));
#197885=CARTESIAN_POINT('Ctrl Pts',(10.9691195629999,15.2,2.75208726999999));
#197886=CARTESIAN_POINT('Ctrl Pts',(10.9726339839999,15.2,2.75147565399998));
#197887=CARTESIAN_POINT('Ctrl Pts',(10.9761525279999,15.2,2.75086050399998));
#197888=CARTESIAN_POINT('Ctrl Pts',(10.9796751869999,15.2,2.75024181699998));
#197889=CARTESIAN_POINT('Ctrl Pts',(10.9832019509999,15.2,2.74961958599999));
#197890=CARTESIAN_POINT('Ctrl Pts',(10.9867328139999,15.2,2.74899380799998));
#197891=CARTESIAN_POINT('Ctrl Pts',(10.9902677649999,15.2,2.74836447799998));
#197892=CARTESIAN_POINT('Ctrl Pts',(10.9938067979999,15.2,2.74773159199999));
#197893=CARTESIAN_POINT('Ctrl Pts',(10.9973499019999,15.2,2.74709514499998));
#197894=CARTESIAN_POINT('Ctrl Pts',(11.0008970699999,15.2,2.74645513199999));
#197895=CARTESIAN_POINT('Ctrl Pts',(11.0044482939999,15.2,2.74581154899998));
#197896=CARTESIAN_POINT('Ctrl Pts',(11.0080035629999,15.2,2.74516439199999));
#197897=CARTESIAN_POINT('Ctrl Pts',(11.0115628719999,15.2,2.74451365599998));
#197898=CARTESIAN_POINT('Ctrl Pts',(11.0151262099999,15.2,2.74385933599999));
#197899=CARTESIAN_POINT('Ctrl Pts',(11.0186935709999,15.2,2.74320142899998));
#197900=CARTESIAN_POINT('Ctrl Pts',(11.0222649439999,15.2,2.74253992799999));
#197901=CARTESIAN_POINT('Ctrl Pts',(11.0258403219999,15.2,2.74187483099999));
#197902=CARTESIAN_POINT('Ctrl Pts',(11.0294196959999,15.2,2.74120613199998));
#197903=CARTESIAN_POINT('Ctrl Pts',(11.0330030589999,15.2,2.74053382799998));
#197904=CARTESIAN_POINT('Ctrl Pts',(11.0365903999999,15.2,2.73985791299998));
#197905=CARTESIAN_POINT('Ctrl Pts',(11.0401817149999,15.2,2.73917838399999));
#197906=CARTESIAN_POINT('Ctrl Pts',(11.0437769909999,15.2,2.73849523599999));
#197907=CARTESIAN_POINT('Ctrl Pts',(11.0473762219999,15.2,2.73780846599998));
#197908=CARTESIAN_POINT('Ctrl Pts',(11.0509794009999,15.2,2.73711806699998));
#197909=CARTESIAN_POINT('Ctrl Pts',(11.0545865169999,15.2,2.73642403699998));
#197910=CARTESIAN_POINT('Ctrl Pts',(11.0581975619999,15.2,2.73572636999998));
#197911=CARTESIAN_POINT('Ctrl Pts',(11.0618125299999,15.2,2.73502506399999));
#197912=CARTESIAN_POINT('Ctrl Pts',(11.0654314099999,15.2,2.73432011199999));
#197913=CARTESIAN_POINT('Ctrl Pts',(11.0690541959999,15.2,2.73361151099999));
#197914=CARTESIAN_POINT('Ctrl Pts',(11.0726808779999,15.2,2.73289925699999));
#197915=CARTESIAN_POINT('Ctrl Pts',(11.0763114489999,15.2,2.73218334499998));
#197916=CARTESIAN_POINT('Ctrl Pts',(11.0799458989999,15.2,2.73146377099999));
#197917=CARTESIAN_POINT('Ctrl Pts',(11.0835842229999,15.2,2.73074053299998));
#197918=CARTESIAN_POINT('Ctrl Pts',(11.0872264109999,15.2,2.73001362299999));
#197919=CARTESIAN_POINT('Ctrl Pts',(11.0908724549999,15.2,2.72928304099998));
#197920=CARTESIAN_POINT('Ctrl Pts',(11.0945223469999,15.2,2.72854877899999));
#197921=CARTESIAN_POINT('Ctrl Pts',(11.0981760779999,15.2,2.72781083499999));
#197922=CARTESIAN_POINT('Ctrl Pts',(11.1018336399999,15.2,2.72706920299999));
#197923=CARTESIAN_POINT('Ctrl Pts',(11.1054950239999,15.2,2.72632388099999));
#197924=CARTESIAN_POINT('Ctrl Pts',(11.1091602219999,15.2,2.72557486299998));
#197925=CARTESIAN_POINT('Ctrl Pts',(11.1128292269999,15.2,2.72482214499998));
#197926=CARTESIAN_POINT('Ctrl Pts',(11.1165020289999,15.2,2.72406572399999));
#197927=CARTESIAN_POINT('Ctrl Pts',(11.1201786229999,15.2,2.72330559599999));
#197928=CARTESIAN_POINT('Ctrl Pts',(11.1238589999999,15.2,2.72254175699998));
#197929=CARTESIAN_POINT('Ctrl Pts',(11.1275431529999,15.2,2.72177420499998));
#197930=CARTESIAN_POINT('Ctrl Pts',(11.1312310749999,15.2,2.72100293299999));
#197931=CARTESIAN_POINT('Ctrl Pts',(11.1349227589999,15.2,2.72022793899998));
#197932=CARTESIAN_POINT('Ctrl Pts',(11.1386181909999,15.2,2.71944921899999));
#197933=CARTESIAN_POINT('Ctrl Pts',(11.1423173659999,15.2,2.71866676499998));
#197934=CARTESIAN_POINT('Ctrl Pts',(11.1460202709999,15.2,2.71788057599998));
#197935=CARTESIAN_POINT('Ctrl Pts',(11.1497268969999,15.2,2.71709064499999));
#197936=CARTESIAN_POINT('Ctrl Pts',(11.1534372359999,15.2,2.71629696699998));
#197937=CARTESIAN_POINT('Ctrl Pts',(11.1571512799999,15.2,2.71549953899999));
#197938=CARTESIAN_POINT('Ctrl Pts',(11.1608690239999,15.2,2.71469835899998));
#197939=CARTESIAN_POINT('Ctrl Pts',(11.1645904639999,15.2,2.71389342499998));
#197940=CARTESIAN_POINT('Ctrl Pts',(11.1683155989999,15.2,2.71308473599999));
#197941=CARTESIAN_POINT('Ctrl Pts',(11.1712986599999,15.2,2.71243477999998));
#197942=CARTESIAN_POINT('Ctrl Pts',(11.1735376169999,15.2,2.71194562399998));
#197943=CARTESIAN_POINT('Ctrl Pts',(11.1750309949999,15.2,2.71161876799999));
#197944=CARTESIAN_POINT('Ctrl Pts',(11.1757778679999,15.2,2.71145515299998));
#197945=CARTESIAN_POINT('Origin',(-5.66257110645729E-14,15.2,-1.77635683940025E-14));
#197946=CARTESIAN_POINT('',(9.86852965744612,15.2,3.20199116236993));
#197947=CARTESIAN_POINT('',(9.86852965744613,12.2,3.20199116236993));
#197948=CARTESIAN_POINT('',(9.86852965699994,15.2,3.20199116199999));
#197949=CARTESIAN_POINT('Origin',(-5.66257110645729E-14,12.2,-1.77635683940025E-14));
#197950=CARTESIAN_POINT('Origin',(-5.66257110645729E-14,15.2,-1.77635683940025E-14));
#197951=CARTESIAN_POINT('Origin',(-5.66257110645729E-14,15.2,-1.77635683940025E-14));
#197952=CARTESIAN_POINT('',(10.8127719249999,15.2,3.91586047999999));
#197953=CARTESIAN_POINT('',(10.6761442619999,15.2,4.27433546899999));
#197954=CARTESIAN_POINT('Origin',(-5.66257110645729E-14,15.2,-1.77635683940025E-14));
#197955=CARTESIAN_POINT('',(10.6761442619999,12.2,4.27433546899999));
#197956=CARTESIAN_POINT('',(10.6761442619999,15.2,4.27433546899999));
#197957=CARTESIAN_POINT('',(10.8127719249999,12.2,3.91586047999999));
#197958=CARTESIAN_POINT('Origin',(-5.66257110645729E-14,12.2,-1.77635683940025E-14));
#197959=CARTESIAN_POINT('',(10.8127719249999,15.2,3.91586047999999));
#197960=CARTESIAN_POINT('Ctrl Pts',(10.6761442619999,15.2,4.27433546899999));
#197961=CARTESIAN_POINT('Ctrl Pts',(10.6761442619999,11.6,4.27433546899999));
#197962=CARTESIAN_POINT('Ctrl Pts',(10.6753817049999,15.2,4.27439112799998));
#197963=CARTESIAN_POINT('Ctrl Pts',(10.6753817049999,11.6,4.27439112799998));
#197964=CARTESIAN_POINT('Ctrl Pts',(10.6738570129999,15.2,4.27450212599998));
#197965=CARTESIAN_POINT('Ctrl Pts',(10.6738570129999,11.6,4.27450212599998));
#197966=CARTESIAN_POINT('Ctrl Pts',(10.6715712299999,15.2,4.27466766699999));
#197967=CARTESIAN_POINT('Ctrl Pts',(10.6715712299999,11.6,4.27466766699998));
#197968=CARTESIAN_POINT('Ctrl Pts',(10.6685260339999,15.2,4.27488647299998));
#197969=CARTESIAN_POINT('Ctrl Pts',(10.6685260339999,11.6,4.27488647299998));
#197970=CARTESIAN_POINT('Ctrl Pts',(10.6647237269999,15.2,4.27515678899999));
#197971=CARTESIAN_POINT('Ctrl Pts',(10.6647237269999,11.6,4.27515678899999));
#197972=CARTESIAN_POINT('Ctrl Pts',(10.6609256119999,15.2,4.27542391299998));
#197973=CARTESIAN_POINT('Ctrl Pts',(10.6609256119999,11.6,4.27542391299998));
#197974=CARTESIAN_POINT('Ctrl Pts',(10.6571316899999,15.2,4.27568784899999));
#197975=CARTESIAN_POINT('Ctrl Pts',(10.6571316899999,11.6,4.27568784899999));
#197976=CARTESIAN_POINT('Ctrl Pts',(10.6533419639999,15.2,4.27594859599999));
#197977=CARTESIAN_POINT('Ctrl Pts',(10.6533419639999,11.6,4.27594859599999));
#197978=CARTESIAN_POINT('Ctrl Pts',(10.6495564379999,15.2,4.27620615899999));
#197979=CARTESIAN_POINT('Ctrl Pts',(10.6495564379999,11.6,4.27620615899999));
#197980=CARTESIAN_POINT('Ctrl Pts',(10.6457751209999,15.2,4.27646054299998));
#197981=CARTESIAN_POINT('Ctrl Pts',(10.6457751209999,11.6,4.27646054299998));
#197982=CARTESIAN_POINT('Ctrl Pts',(10.6419980199999,15.2,4.27671175199999));
#197983=CARTESIAN_POINT('Ctrl Pts',(10.6419980199999,11.6,4.27671175199999));
#197984=CARTESIAN_POINT('Ctrl Pts',(10.6382251429999,15.2,4.27695979399999));
#197985=CARTESIAN_POINT('Ctrl Pts',(10.6382251429999,11.6,4.27695979399999));
#197986=CARTESIAN_POINT('Ctrl Pts',(10.6344565009999,15.2,4.27720467299999));
#197987=CARTESIAN_POINT('Ctrl Pts',(10.6344565009999,11.6,4.27720467299998));
#197988=CARTESIAN_POINT('Ctrl Pts',(10.6306921009999,15.2,4.27744639699998));
#197989=CARTESIAN_POINT('Ctrl Pts',(10.6306921009999,11.6,4.27744639699998));
#197990=CARTESIAN_POINT('Ctrl Pts',(10.6269319529999,15.2,4.27768497199998));
#197991=CARTESIAN_POINT('Ctrl Pts',(10.6269319529999,11.6,4.27768497199998));
#197992=CARTESIAN_POINT('Ctrl Pts',(10.6231760649999,15.2,4.27792040299998));
#197993=CARTESIAN_POINT('Ctrl Pts',(10.6231760649999,11.6,4.27792040299998));
#197994=CARTESIAN_POINT('Ctrl Pts',(10.6194244419999,15.2,4.27815269399999));
#197995=CARTESIAN_POINT('Ctrl Pts',(10.6194244419999,11.6,4.27815269399998));
#197996=CARTESIAN_POINT('Ctrl Pts',(10.6156770939999,15.2,4.27838185099999));
#197997=CARTESIAN_POINT('Ctrl Pts',(10.6156770939999,11.6,4.27838185099999));
#197998=CARTESIAN_POINT('Ctrl Pts',(10.6119340259999,15.2,4.27860787899998));
#197999=CARTESIAN_POINT('Ctrl Pts',(10.6119340259999,11.6,4.27860787899998));
#198000=CARTESIAN_POINT('Ctrl Pts',(10.6081952429999,15.2,4.27883078099998));
#198001=CARTESIAN_POINT('Ctrl Pts',(10.6081952429999,11.6,4.27883078099998));
#198002=CARTESIAN_POINT('Ctrl Pts',(10.6044607549999,15.2,4.27905056299998));
#198003=CARTESIAN_POINT('Ctrl Pts',(10.6044607549999,11.6,4.27905056299998));
#198004=CARTESIAN_POINT('Ctrl Pts',(10.6007305679999,15.2,4.27926722899999));
#198005=CARTESIAN_POINT('Ctrl Pts',(10.6007305679999,11.6,4.27926722899999));
#198006=CARTESIAN_POINT('Ctrl Pts',(10.5970046899999,15.2,4.27948078699998));
#198007=CARTESIAN_POINT('Ctrl Pts',(10.5970046899999,11.6,4.27948078699998));
#198008=CARTESIAN_POINT('Ctrl Pts',(10.5932831279999,15.2,4.27969123999999));
#198009=CARTESIAN_POINT('Ctrl Pts',(10.5932831279999,11.6,4.27969123999999));
#198010=CARTESIAN_POINT('Ctrl Pts',(10.5895658899999,15.2,4.27989859399998));
#198011=CARTESIAN_POINT('Ctrl Pts',(10.5895658899999,11.6,4.27989859399998));
#198012=CARTESIAN_POINT('Ctrl Pts',(10.5858529849999,15.2,4.28010285499998));
#198013=CARTESIAN_POINT('Ctrl Pts',(10.5858529849999,11.6,4.28010285499998));
#198014=CARTESIAN_POINT('Ctrl Pts',(10.5821444189999,15.2,4.28030402799998));
#198015=CARTESIAN_POINT('Ctrl Pts',(10.5821444189999,11.6,4.28030402799998));
#198016=CARTESIAN_POINT('Ctrl Pts',(10.5784402009999,15.2,4.28050211799999));
#198017=CARTESIAN_POINT('Ctrl Pts',(10.5784402009999,11.6,4.28050211799999));
#198018=CARTESIAN_POINT('Ctrl Pts',(10.5747403369999,15.2,4.28069712999999));
#198019=CARTESIAN_POINT('Ctrl Pts',(10.5747403369999,11.6,4.28069712999999));
#198020=CARTESIAN_POINT('Ctrl Pts',(10.5710448359999,15.2,4.28088907099998));
#198021=CARTESIAN_POINT('Ctrl Pts',(10.5710448359999,11.6,4.28088907099998));
#198022=CARTESIAN_POINT('Ctrl Pts',(10.5673537039999,15.2,4.28107794499999));
#198023=CARTESIAN_POINT('Ctrl Pts',(10.5673537039999,11.6,4.28107794499999));
#198024=CARTESIAN_POINT('Ctrl Pts',(10.5636669489999,15.2,4.28126375699998));
#198025=CARTESIAN_POINT('Ctrl Pts',(10.5636669489999,11.6,4.28126375699998));
#198026=CARTESIAN_POINT('Ctrl Pts',(10.5599845779999,15.2,4.28144651299998));
#198027=CARTESIAN_POINT('Ctrl Pts',(10.5599845779999,11.6,4.28144651299998));
#198028=CARTESIAN_POINT('Ctrl Pts',(10.5563065999999,15.2,4.28162621899999));
#198029=CARTESIAN_POINT('Ctrl Pts',(10.5563065999999,11.6,4.28162621899998));
#198030=CARTESIAN_POINT('Ctrl Pts',(10.5526330209999,15.2,4.28180287899998));
#198031=CARTESIAN_POINT('Ctrl Pts',(10.5526330209999,11.6,4.28180287899998));
#198032=CARTESIAN_POINT('Ctrl Pts',(10.5489638489999,15.2,4.28197649899998));
#198033=CARTESIAN_POINT('Ctrl Pts',(10.5489638489999,11.6,4.28197649899998));
#198034=CARTESIAN_POINT('Ctrl Pts',(10.5452990929999,15.2,4.28214708399998));
#198035=CARTESIAN_POINT('Ctrl Pts',(10.5452990929999,11.6,4.28214708399998));
#198036=CARTESIAN_POINT('Ctrl Pts',(10.5416387579999,15.2,4.28231463999998));
#198037=CARTESIAN_POINT('Ctrl Pts',(10.5416387579999,11.6,4.28231463999998));
#198038=CARTESIAN_POINT('Ctrl Pts',(10.5379828539999,15.2,4.28247917299998));
#198039=CARTESIAN_POINT('Ctrl Pts',(10.5379828539999,11.6,4.28247917299998));
#198040=CARTESIAN_POINT('Ctrl Pts',(10.5343313879999,15.2,4.28264068899999));
#198041=CARTESIAN_POINT('Ctrl Pts',(10.5343313879999,11.6,4.28264068899998));
#198042=CARTESIAN_POINT('Ctrl Pts',(10.5306843669999,15.2,4.28279919099998));
#198043=CARTESIAN_POINT('Ctrl Pts',(10.5306843669999,11.6,4.28279919099998));
#198044=CARTESIAN_POINT('Ctrl Pts',(10.5270417989999,15.2,4.28295468699999));
#198045=CARTESIAN_POINT('Ctrl Pts',(10.5270417989999,11.6,4.28295468699999));
#198046=CARTESIAN_POINT('Ctrl Pts',(10.5234036919999,15.2,4.28310718099999));
#198047=CARTESIAN_POINT('Ctrl Pts',(10.5234036919999,11.6,4.28310718099999));
#198048=CARTESIAN_POINT('Ctrl Pts',(10.5197700539999,15.2,4.28325667899998));
#198049=CARTESIAN_POINT('Ctrl Pts',(10.5197700539999,11.6,4.28325667899998));
#198050=CARTESIAN_POINT('Ctrl Pts',(10.5161408899999,15.2,4.28340318599999));
#198051=CARTESIAN_POINT('Ctrl Pts',(10.5161408899999,11.6,4.28340318599999));
#198052=CARTESIAN_POINT('Ctrl Pts',(10.5125162099999,15.2,4.28354670899999));
#198053=CARTESIAN_POINT('Ctrl Pts',(10.5125162099999,11.6,4.28354670899999));
#198054=CARTESIAN_POINT('Ctrl Pts',(10.5088960219999,15.2,4.28368725399999));
#198055=CARTESIAN_POINT('Ctrl Pts',(10.5088960219999,11.6,4.28368725399999));
#198056=CARTESIAN_POINT('Ctrl Pts',(10.5052803329999,15.2,4.28382482399999));
#198057=CARTESIAN_POINT('Ctrl Pts',(10.5052803329999,11.6,4.28382482399999));
#198058=CARTESIAN_POINT('Ctrl Pts',(10.5016691499999,15.2,4.28395942599998));
#198059=CARTESIAN_POINT('Ctrl Pts',(10.5016691499999,11.6,4.28395942599998));
#198060=CARTESIAN_POINT('Ctrl Pts',(10.4980624809999,15.2,4.28409106699998));
#198061=CARTESIAN_POINT('Ctrl Pts',(10.4980624809999,11.6,4.28409106699998));
#198062=CARTESIAN_POINT('Ctrl Pts',(10.4944603349999,15.2,4.28421974999999));
#198063=CARTESIAN_POINT('Ctrl Pts',(10.4944603349999,11.6,4.28421974999999));
#198064=CARTESIAN_POINT('Ctrl Pts',(10.4908627189999,15.2,4.28434548299998));
#198065=CARTESIAN_POINT('Ctrl Pts',(10.4908627189999,11.6,4.28434548299998));
#198066=CARTESIAN_POINT('Ctrl Pts',(10.4872696399999,15.2,4.28446827099998));
#198067=CARTESIAN_POINT('Ctrl Pts',(10.4872696399999,11.6,4.28446827099998));
#198068=CARTESIAN_POINT('Ctrl Pts',(10.4836811069999,15.2,4.28458811899999));
#198069=CARTESIAN_POINT('Ctrl Pts',(10.4836811069999,11.6,4.28458811899999));
#198070=CARTESIAN_POINT('Ctrl Pts',(10.4800971249999,15.2,4.28470503199998));
#198071=CARTESIAN_POINT('Ctrl Pts',(10.4800971249999,11.6,4.28470503199998));
#198072=CARTESIAN_POINT('Ctrl Pts',(10.4765177049999,15.2,4.28481901899998));
#198073=CARTESIAN_POINT('Ctrl Pts',(10.4765177049999,11.6,4.28481901899998));
#198074=CARTESIAN_POINT('Ctrl Pts',(10.4729428539999,15.2,4.28493008299998));
#198075=CARTESIAN_POINT('Ctrl Pts',(10.4729428539999,11.6,4.28493008299998));
#198076=CARTESIAN_POINT('Ctrl Pts',(10.4693725789999,15.2,4.28503822999998));
#198077=CARTESIAN_POINT('Ctrl Pts',(10.4693725789999,11.6,4.28503822999998));
#198078=CARTESIAN_POINT('Ctrl Pts',(10.4658068879999,15.2,4.28514346699998));
#198079=CARTESIAN_POINT('Ctrl Pts',(10.4658068879999,11.6,4.28514346699998));
#198080=CARTESIAN_POINT('Ctrl Pts',(10.4622457879999,15.2,4.28524579899998));
#198081=CARTESIAN_POINT('Ctrl Pts',(10.4622457879999,11.6,4.28524579899998));
#198082=CARTESIAN_POINT('Ctrl Pts',(10.4586892889999,15.2,4.28534523199998));
#198083=CARTESIAN_POINT('Ctrl Pts',(10.4586892889999,11.6,4.28534523199998));
#198084=CARTESIAN_POINT('Ctrl Pts',(10.4551373969999,15.2,4.28544177099998));
#198085=CARTESIAN_POINT('Ctrl Pts',(10.4551373969999,11.6,4.28544177099998));
#198086=CARTESIAN_POINT('Ctrl Pts',(10.4515901199999,15.2,4.28553542399998));
#198087=CARTESIAN_POINT('Ctrl Pts',(10.4515901199999,11.6,4.28553542399998));
#198088=CARTESIAN_POINT('Ctrl Pts',(10.4480474659999,15.2,4.28562619399998));
#198089=CARTESIAN_POINT('Ctrl Pts',(10.4480474659999,11.6,4.28562619399998));
#198090=CARTESIAN_POINT('Ctrl Pts',(10.4445094429999,15.2,4.28571408999999));
#198091=CARTESIAN_POINT('Ctrl Pts',(10.4445094429999,11.6,4.28571408999998));
#198092=CARTESIAN_POINT('Ctrl Pts',(10.4409760589999,15.2,4.28579911599999));
#198093=CARTESIAN_POINT('Ctrl Pts',(10.4409760589999,11.6,4.28579911599999));
#198094=CARTESIAN_POINT('Ctrl Pts',(10.4374473219999,15.2,4.28588127799999));
#198095=CARTESIAN_POINT('Ctrl Pts',(10.4374473219999,11.6,4.28588127799998));
#198096=CARTESIAN_POINT('Ctrl Pts',(10.4339232389999,15.2,4.28596058199999));
#198097=CARTESIAN_POINT('Ctrl Pts',(10.4339232389999,11.6,4.28596058199999));
#198098=CARTESIAN_POINT('Ctrl Pts',(10.4304038179999,15.2,4.28603703499999));
#198099=CARTESIAN_POINT('Ctrl Pts',(10.4304038179999,11.6,4.28603703499998));
#198100=CARTESIAN_POINT('Ctrl Pts',(10.4268890689999,15.2,4.28611064199998));
#198101=CARTESIAN_POINT('Ctrl Pts',(10.4268890689999,11.6,4.28611064199998));
#198102=CARTESIAN_POINT('Ctrl Pts',(10.4233789969999,15.2,4.28618140899999));
#198103=CARTESIAN_POINT('Ctrl Pts',(10.4233789969999,11.6,4.28618140899999));
#198104=CARTESIAN_POINT('Ctrl Pts',(10.4198736109999,15.2,4.28624934199998));
#198105=CARTESIAN_POINT('Ctrl Pts',(10.4198736109999,11.6,4.28624934199998));
#198106=CARTESIAN_POINT('Ctrl Pts',(10.4163729199999,15.2,4.28631444799999));
#198107=CARTESIAN_POINT('Ctrl Pts',(10.4163729199999,11.6,4.28631444799999));
#198108=CARTESIAN_POINT('Ctrl Pts',(10.4128769299999,15.2,4.28637673099999));
#198109=CARTESIAN_POINT('Ctrl Pts',(10.4128769299999,11.6,4.28637673099998));
#198110=CARTESIAN_POINT('Ctrl Pts',(10.4093856499999,15.2,4.28643619999999));
#198111=CARTESIAN_POINT('Ctrl Pts',(10.4093856499999,11.6,4.28643619999998));
#198112=CARTESIAN_POINT('Ctrl Pts',(10.4058990889999,15.2,4.28649285799998));
#198113=CARTESIAN_POINT('Ctrl Pts',(10.4058990889999,11.6,4.28649285799998));
#198114=CARTESIAN_POINT('Ctrl Pts',(10.4024172519999,15.2,4.28654671399999));
#198115=CARTESIAN_POINT('Ctrl Pts',(10.4024172519999,11.6,4.28654671399998));
#198116=CARTESIAN_POINT('Ctrl Pts',(10.3989401499999,15.2,4.28659777199999));
#198117=CARTESIAN_POINT('Ctrl Pts',(10.3989401499999,11.6,4.28659777199999));
#198118=CARTESIAN_POINT('Ctrl Pts',(10.3954677879999,15.2,4.28664603899998));
#198119=CARTESIAN_POINT('Ctrl Pts',(10.3954677879999,11.6,4.28664603899998));
#198120=CARTESIAN_POINT('Ctrl Pts',(10.3920001779999,15.2,4.28669152099998));
#198121=CARTESIAN_POINT('Ctrl Pts',(10.3920001779999,11.6,4.28669152099998));
#198122=CARTESIAN_POINT('Ctrl Pts',(10.3885373239999,15.2,4.28673422399999));
#198123=CARTESIAN_POINT('Ctrl Pts',(10.3885373239999,11.6,4.28673422399999));
#198124=CARTESIAN_POINT('Ctrl Pts',(10.3850792369999,15.2,4.28677415499998));
#198125=CARTESIAN_POINT('Ctrl Pts',(10.3850792369999,11.6,4.28677415499998));
#198126=CARTESIAN_POINT('Ctrl Pts',(10.3816259229999,15.2,4.28681131999999));
#198127=CARTESIAN_POINT('Ctrl Pts',(10.3816259229999,11.6,4.28681131999998));
#198128=CARTESIAN_POINT('Ctrl Pts',(10.3781773909999,15.2,4.28684572399998));
#198129=CARTESIAN_POINT('Ctrl Pts',(10.3781773909999,11.6,4.28684572399998));
#198130=CARTESIAN_POINT('Ctrl Pts',(10.3747336489999,15.2,4.28687737299998));
#198131=CARTESIAN_POINT('Ctrl Pts',(10.3747336489999,11.6,4.28687737299998));
#198132=CARTESIAN_POINT('Ctrl Pts',(10.3712947049999,15.2,4.28690627599998));
#198133=CARTESIAN_POINT('Ctrl Pts',(10.3712947049999,11.6,4.28690627599998));
#198134=CARTESIAN_POINT('Ctrl Pts',(10.3678605659999,15.2,4.28693243699998));
#198135=CARTESIAN_POINT('Ctrl Pts',(10.3678605659999,11.6,4.28693243699998));
#198136=CARTESIAN_POINT('Ctrl Pts',(10.3644312409999,15.2,4.28695586399999));
#198137=CARTESIAN_POINT('Ctrl Pts',(10.3644312409999,11.6,4.28695586399999));
#198138=CARTESIAN_POINT('Ctrl Pts',(10.3610067379999,15.2,4.28697656099998));
#198139=CARTESIAN_POINT('Ctrl Pts',(10.3610067379999,11.6,4.28697656099998));
#198140=CARTESIAN_POINT('Ctrl Pts',(10.3575870659999,15.2,4.28699453699998));
#198141=CARTESIAN_POINT('Ctrl Pts',(10.3575870659999,11.6,4.28699453699998));
#198142=CARTESIAN_POINT('Ctrl Pts',(10.3541722309999,15.2,4.28700979599999));
#198143=CARTESIAN_POINT('Ctrl Pts',(10.3541722309999,11.6,4.28700979599998));
#198144=CARTESIAN_POINT('Ctrl Pts',(10.3507622439999,15.2,4.28702234599999));
#198145=CARTESIAN_POINT('Ctrl Pts',(10.3507622439999,11.6,4.28702234599999));
#198146=CARTESIAN_POINT('Ctrl Pts',(10.3473571099999,15.2,4.28703219199999));
#198147=CARTESIAN_POINT('Ctrl Pts',(10.3473571099999,11.6,4.28703219199999));
#198148=CARTESIAN_POINT('Ctrl Pts',(10.3439568399999,15.2,4.28703934199999));
#198149=CARTESIAN_POINT('Ctrl Pts',(10.3439568399999,11.6,4.28703934199999));
#198150=CARTESIAN_POINT('Ctrl Pts',(10.3405614389999,15.2,4.28704380099998));
#198151=CARTESIAN_POINT('Ctrl Pts',(10.3405614389999,11.6,4.28704380099998));
#198152=CARTESIAN_POINT('Ctrl Pts',(10.3371709179999,15.2,4.28704557699999));
#198153=CARTESIAN_POINT('Ctrl Pts',(10.3371709179999,11.6,4.28704557699999));
#198154=CARTESIAN_POINT('Ctrl Pts',(10.3337852839999,15.2,4.28704467399999));
#198155=CARTESIAN_POINT('Ctrl Pts',(10.3337852839999,11.6,4.28704467399999));
#198156=CARTESIAN_POINT('Ctrl Pts',(10.3304045439999,15.2,4.28704110199998));
#198157=CARTESIAN_POINT('Ctrl Pts',(10.3304045439999,11.6,4.28704110199998));
#198158=CARTESIAN_POINT('Ctrl Pts',(10.3270287089999,15.2,4.28703486399999));
#198159=CARTESIAN_POINT('Ctrl Pts',(10.3270287089999,11.6,4.28703486399998));
#198160=CARTESIAN_POINT('Ctrl Pts',(10.3236577839999,15.2,4.28702596899999));
#198161=CARTESIAN_POINT('Ctrl Pts',(10.3236577839999,11.6,4.28702596899999));
#198162=CARTESIAN_POINT('Ctrl Pts',(10.3202917799999,15.2,4.28701442299998));
#198163=CARTESIAN_POINT('Ctrl Pts',(10.3202917799999,11.6,4.28701442299998));
#198164=CARTESIAN_POINT('Ctrl Pts',(10.3169307029999,15.2,4.28700023099999));
#198165=CARTESIAN_POINT('Ctrl Pts',(10.3169307029999,11.6,4.28700023099999));
#198166=CARTESIAN_POINT('Ctrl Pts',(10.3135745629999,15.2,4.28698340099999));
#198167=CARTESIAN_POINT('Ctrl Pts',(10.3135745629999,11.6,4.28698340099999));
#198168=CARTESIAN_POINT('Ctrl Pts',(10.3102233669999,15.2,4.28696393999999));
#198169=CARTESIAN_POINT('Ctrl Pts',(10.3102233669999,11.6,4.28696393999999));
#198170=CARTESIAN_POINT('Ctrl Pts',(10.3068771239999,15.2,4.28694185499998));
#198171=CARTESIAN_POINT('Ctrl Pts',(10.3068771239999,11.6,4.28694185499998));
#198172=CARTESIAN_POINT('Ctrl Pts',(10.3035358409999,15.2,4.28691714999999));
#198173=CARTESIAN_POINT('Ctrl Pts',(10.3035358409999,11.6,4.28691714999999));
#198174=CARTESIAN_POINT('Ctrl Pts',(10.3001995279999,15.2,4.28688983399999));
#198175=CARTESIAN_POINT('Ctrl Pts',(10.3001995279999,11.6,4.28688983399999));
#198176=CARTESIAN_POINT('Ctrl Pts',(10.2968681929999,15.2,4.28685991399998));
#198177=CARTESIAN_POINT('Ctrl Pts',(10.2968681929999,11.6,4.28685991399998));
#198178=CARTESIAN_POINT('Ctrl Pts',(10.2935418419999,15.2,4.28682739499998));
#198179=CARTESIAN_POINT('Ctrl Pts',(10.2935418419999,11.6,4.28682739499998));
#198180=CARTESIAN_POINT('Ctrl Pts',(10.2902204869999,15.2,4.28679228399999));
#198181=CARTESIAN_POINT('Ctrl Pts',(10.2902204869999,11.6,4.28679228399999));
#198182=CARTESIAN_POINT('Ctrl Pts',(10.2869041329999,15.2,4.28675458899999));
#198183=CARTESIAN_POINT('Ctrl Pts',(10.2869041329999,11.6,4.28675458899998));
#198184=CARTESIAN_POINT('Ctrl Pts',(10.2835927899999,15.2,4.28671431599999));
#198185=CARTESIAN_POINT('Ctrl Pts',(10.2835927899999,11.6,4.28671431599999));
#198186=CARTESIAN_POINT('Ctrl Pts',(10.2802864669999,15.2,4.28667147199998));
#198187=CARTESIAN_POINT('Ctrl Pts',(10.2802864669999,11.6,4.28667147199998));
#198188=CARTESIAN_POINT('Ctrl Pts',(10.2769851699999,15.2,4.28662606299999));
#198189=CARTESIAN_POINT('Ctrl Pts',(10.2769851699999,11.6,4.28662606299999));
#198190=CARTESIAN_POINT('Ctrl Pts',(10.2736889099999,15.2,4.28657809699998));
#198191=CARTESIAN_POINT('Ctrl Pts',(10.2736889099999,11.6,4.28657809699998));
#198192=CARTESIAN_POINT('Ctrl Pts',(10.2703976929999,15.2,4.28652758099999));
#198193=CARTESIAN_POINT('Ctrl Pts',(10.2703976929999,11.6,4.28652758099999));
#198194=CARTESIAN_POINT('Ctrl Pts',(10.2671115289999,15.2,4.28647451899998));
#198195=CARTESIAN_POINT('Ctrl Pts',(10.2671115289999,11.6,4.28647451899998));
#198196=CARTESIAN_POINT('Ctrl Pts',(10.2638304259999,15.2,4.28641892199998));
#198197=CARTESIAN_POINT('Ctrl Pts',(10.2638304259999,11.6,4.28641892199998));
#198198=CARTESIAN_POINT('Ctrl Pts',(10.2605543909999,15.2,4.28636079499999));
#198199=CARTESIAN_POINT('Ctrl Pts',(10.2605543909999,11.6,4.28636079499999));
#198200=CARTESIAN_POINT('Ctrl Pts',(10.2572834349999,15.2,4.28630014399998));
#198201=CARTESIAN_POINT('Ctrl Pts',(10.2572834349999,11.6,4.28630014399998));
#198202=CARTESIAN_POINT('Ctrl Pts',(10.2540175649999,15.2,4.28623697799999));
#198203=CARTESIAN_POINT('Ctrl Pts',(10.2540175649999,11.6,4.28623697799999));
#198204=CARTESIAN_POINT('Ctrl Pts',(10.2507567889999,15.2,4.28617130199999));
#198205=CARTESIAN_POINT('Ctrl Pts',(10.2507567889999,11.6,4.28617130199999));
#198206=CARTESIAN_POINT('Ctrl Pts',(10.2475011169999,15.2,4.28610312399999));
#198207=CARTESIAN_POINT('Ctrl Pts',(10.2475011169999,11.6,4.28610312399999));
#198208=CARTESIAN_POINT('Ctrl Pts',(10.2442505549999,15.2,4.28603244999999));
#198209=CARTESIAN_POINT('Ctrl Pts',(10.2442505549999,11.6,4.28603244999999));
#198210=CARTESIAN_POINT('Ctrl Pts',(10.2410051139999,15.2,4.28595928999999));
#198211=CARTESIAN_POINT('Ctrl Pts',(10.2410051139999,11.6,4.28595928999999));
#198212=CARTESIAN_POINT('Ctrl Pts',(10.2377648009999,15.2,4.28588364599998));
#198213=CARTESIAN_POINT('Ctrl Pts',(10.2377648009999,11.6,4.28588364599998));
#198214=CARTESIAN_POINT('Ctrl Pts',(10.2345296249999,15.2,4.28580552999998));
#198215=CARTESIAN_POINT('Ctrl Pts',(10.2345296249999,11.6,4.28580552999998));
#198216=CARTESIAN_POINT('Ctrl Pts',(10.2312995949999,15.2,4.28572494799998));
#198217=CARTESIAN_POINT('Ctrl Pts',(10.2312995949999,11.6,4.28572494799998));
#198218=CARTESIAN_POINT('Ctrl Pts',(10.2280747169999,15.2,4.28564190499999));
#198219=CARTESIAN_POINT('Ctrl Pts',(10.2280747169999,11.6,4.28564190499999));
#198220=CARTESIAN_POINT('Ctrl Pts',(10.2248550039999,15.2,4.28555640899998));
#198221=CARTESIAN_POINT('Ctrl Pts',(10.2248550039999,11.6,4.28555640899998));
#198222=CARTESIAN_POINT('Ctrl Pts',(10.2216404599999,15.2,4.28546846799998));
#198223=CARTESIAN_POINT('Ctrl Pts',(10.2216404599999,11.6,4.28546846799998));
#198224=CARTESIAN_POINT('Ctrl Pts',(10.2184310959999,15.2,4.28537808899998));
#198225=CARTESIAN_POINT('Ctrl Pts',(10.2184310959999,11.6,4.28537808899998));
#198226=CARTESIAN_POINT('Ctrl Pts',(10.2152269199999,15.2,4.28528527899999));
#198227=CARTESIAN_POINT('Ctrl Pts',(10.2152269199999,11.6,4.28528527899999));
#198228=CARTESIAN_POINT('Ctrl Pts',(10.2120279409999,15.2,4.28519004499999));
#198229=CARTESIAN_POINT('Ctrl Pts',(10.2120279409999,11.6,4.28519004499999));
#198230=CARTESIAN_POINT('Ctrl Pts',(10.2088341669999,15.2,4.28509239499999));
#198231=CARTESIAN_POINT('Ctrl Pts',(10.2088341669999,11.6,4.28509239499998));
#198232=CARTESIAN_POINT('Ctrl Pts',(10.2056456079999,15.2,4.28499233499998));
#198233=CARTESIAN_POINT('Ctrl Pts',(10.2056456079999,11.6,4.28499233499998));
#198234=CARTESIAN_POINT('Ctrl Pts',(10.2024622709999,15.2,4.28488987299998));
#198235=CARTESIAN_POINT('Ctrl Pts',(10.2024622709999,11.6,4.28488987299998));
#198236=CARTESIAN_POINT('Ctrl Pts',(10.1992841639999,15.2,4.28478501599999));
#198237=CARTESIAN_POINT('Ctrl Pts',(10.1992841639999,11.6,4.28478501599999));
#198238=CARTESIAN_POINT('Ctrl Pts',(10.1961112979999,15.2,4.28467777199998));
#198239=CARTESIAN_POINT('Ctrl Pts',(10.1961112979999,11.6,4.28467777199998));
#198240=CARTESIAN_POINT('Ctrl Pts',(10.1929436789999,15.2,4.28456814899998));
#198241=CARTESIAN_POINT('Ctrl Pts',(10.1929436789999,11.6,4.28456814899998));
#198242=CARTESIAN_POINT('Ctrl Pts',(10.1897813189999,15.2,4.28445615199998));
#198243=CARTESIAN_POINT('Ctrl Pts',(10.1897813189999,11.6,4.28445615199998));
#198244=CARTESIAN_POINT('Ctrl Pts',(10.1866242239999,15.2,4.28434178999999));
#198245=CARTESIAN_POINT('Ctrl Pts',(10.1866242239999,11.6,4.28434178999998));
#198246=CARTESIAN_POINT('Ctrl Pts',(10.1834724029999,15.2,4.28422507099998));
#198247=CARTESIAN_POINT('Ctrl Pts',(10.1834724029999,11.6,4.28422507099998));
#198248=CARTESIAN_POINT('Ctrl Pts',(10.1803258649999,15.2,4.28410600199999));
#198249=CARTESIAN_POINT('Ctrl Pts',(10.1803258649999,11.6,4.28410600199999));
#198250=CARTESIAN_POINT('Ctrl Pts',(10.1771846189999,15.2,4.28398458999999));
#198251=CARTESIAN_POINT('Ctrl Pts',(10.1771846189999,11.6,4.28398458999998));
#198252=CARTESIAN_POINT('Ctrl Pts',(10.1740486739999,15.2,4.28386084199998));
#198253=CARTESIAN_POINT('Ctrl Pts',(10.1740486739999,11.6,4.28386084199998));
#198254=CARTESIAN_POINT('Ctrl Pts',(10.1709180389999,15.2,4.28373476599998));
#198255=CARTESIAN_POINT('Ctrl Pts',(10.1709180389999,11.6,4.28373476599998));
#198256=CARTESIAN_POINT('Ctrl Pts',(10.1677927209999,15.2,4.28360636999999));
#198257=CARTESIAN_POINT('Ctrl Pts',(10.1677927209999,11.6,4.28360636999999));
#198258=CARTESIAN_POINT('Ctrl Pts',(10.1646727299999,15.2,4.28347566199999));
#198259=CARTESIAN_POINT('Ctrl Pts',(10.1646727299999,11.6,4.28347566199999));
#198260=CARTESIAN_POINT('Ctrl Pts',(10.1615580749999,15.2,4.28334264799999));
#198261=CARTESIAN_POINT('Ctrl Pts',(10.1615580749999,11.6,4.28334264799999));
#198262=CARTESIAN_POINT('Ctrl Pts',(10.1584487639999,15.2,4.28320733699999));
#198263=CARTESIAN_POINT('Ctrl Pts',(10.1584487639999,11.6,4.28320733699999));
#198264=CARTESIAN_POINT('Ctrl Pts',(10.1553448059999,15.2,4.28306973499998));
#198265=CARTESIAN_POINT('Ctrl Pts',(10.1553448059999,11.6,4.28306973499998));
#198266=CARTESIAN_POINT('Ctrl Pts',(10.1522462099999,15.2,4.28292985199998));
#198267=CARTESIAN_POINT('Ctrl Pts',(10.1522462099999,11.6,4.28292985199998));
#198268=CARTESIAN_POINT('Ctrl Pts',(10.1491529859999,15.2,4.28278769499999));
#198269=CARTESIAN_POINT('Ctrl Pts',(10.1491529859999,11.6,4.28278769499998));
#198270=CARTESIAN_POINT('Ctrl Pts',(10.1460651409999,15.2,4.28264326999999));
#198271=CARTESIAN_POINT('Ctrl Pts',(10.1460651409999,11.6,4.28264326999999));
#198272=CARTESIAN_POINT('Ctrl Pts',(10.1429826849999,15.2,4.28249658699999));
#198273=CARTESIAN_POINT('Ctrl Pts',(10.1429826849999,11.6,4.28249658699999));
#198274=CARTESIAN_POINT('Ctrl Pts',(10.1399056249999,15.2,4.28234765099998));
#198275=CARTESIAN_POINT('Ctrl Pts',(10.1399056249999,11.6,4.28234765099998));
#198276=CARTESIAN_POINT('Ctrl Pts',(10.1368339729999,15.2,4.28219647199998));
#198277=CARTESIAN_POINT('Ctrl Pts',(10.1368339729999,11.6,4.28219647199998));
#198278=CARTESIAN_POINT('Ctrl Pts',(10.1337677349999,15.2,4.28204305799999));
#198279=CARTESIAN_POINT('Ctrl Pts',(10.1337677349999,11.6,4.28204305799999));
#198280=CARTESIAN_POINT('Ctrl Pts',(10.1307069219999,15.2,4.28188741599998));
#198281=CARTESIAN_POINT('Ctrl Pts',(10.1307069219999,11.6,4.28188741599998));
#198282=CARTESIAN_POINT('Ctrl Pts',(10.1276515429999,15.2,4.28172955299999));
#198283=CARTESIAN_POINT('Ctrl Pts',(10.1276515429999,11.6,4.28172955299999));
#198284=CARTESIAN_POINT('Ctrl Pts',(10.1246016049999,15.2,4.28156947899998));
#198285=CARTESIAN_POINT('Ctrl Pts',(10.1246016049999,11.6,4.28156947899998));
#198286=CARTESIAN_POINT('Ctrl Pts',(10.1215571169999,15.2,4.28140719999998));
#198287=CARTESIAN_POINT('Ctrl Pts',(10.1215571169999,11.6,4.28140719999998));
#198288=CARTESIAN_POINT('Ctrl Pts',(10.1185180899999,15.2,4.28124272399998));
#198289=CARTESIAN_POINT('Ctrl Pts',(10.1185180899999,11.6,4.28124272399998));
#198290=CARTESIAN_POINT('Ctrl Pts',(10.1154845319999,15.2,4.28107605999998));
#198291=CARTESIAN_POINT('Ctrl Pts',(10.1154845319999,11.6,4.28107605999998));
#198292=CARTESIAN_POINT('Ctrl Pts',(10.1124564509999,15.2,4.28090721599999));
#198293=CARTESIAN_POINT('Ctrl Pts',(10.1124564509999,11.6,4.28090721599998));
#198294=CARTESIAN_POINT('Ctrl Pts',(10.1094338579999,15.2,4.28073619999999));
#198295=CARTESIAN_POINT('Ctrl Pts',(10.1094338579999,11.6,4.28073619999999));
#198296=CARTESIAN_POINT('Ctrl Pts',(10.1064167609999,15.2,4.28056301899999));
#198297=CARTESIAN_POINT('Ctrl Pts',(10.1064167609999,11.6,4.28056301899998));
#198298=CARTESIAN_POINT('Ctrl Pts',(10.1034051679999,15.2,4.28038767999999));
#198299=CARTESIAN_POINT('Ctrl Pts',(10.1034051679999,11.6,4.28038767999999));
#198300=CARTESIAN_POINT('Ctrl Pts',(10.1003990899999,15.2,4.28021019499998));
#198301=CARTESIAN_POINT('Ctrl Pts',(10.1003990899999,11.6,4.28021019499998));
#198302=CARTESIAN_POINT('Ctrl Pts',(10.0973985339999,15.2,4.28003056799999));
#198303=CARTESIAN_POINT('Ctrl Pts',(10.0973985339999,11.6,4.28003056799999));
#198304=CARTESIAN_POINT('Ctrl Pts',(10.0944035109999,15.2,4.27984880999999));
#198305=CARTESIAN_POINT('Ctrl Pts',(10.0944035109999,11.6,4.27984880999999));
#198306=CARTESIAN_POINT('Ctrl Pts',(10.0914140299999,15.2,4.27966492799998));
#198307=CARTESIAN_POINT('Ctrl Pts',(10.0914140299999,11.6,4.27966492799998));
#198308=CARTESIAN_POINT('Ctrl Pts',(10.0884300979999,15.2,4.27947892899999));
#198309=CARTESIAN_POINT('Ctrl Pts',(10.0884300979999,11.6,4.27947892899999));
#198310=CARTESIAN_POINT('Ctrl Pts',(10.0854517259999,15.2,4.27929082399999));
#198311=CARTESIAN_POINT('Ctrl Pts',(10.0854517259999,11.6,4.27929082399999));
#198312=CARTESIAN_POINT('Ctrl Pts',(10.0824789229999,15.2,4.27910061799999));
#198313=CARTESIAN_POINT('Ctrl Pts',(10.0824789229999,11.6,4.27910061799999));
#198314=CARTESIAN_POINT('Ctrl Pts',(10.0795116959999,15.2,4.27890832199999));
#198315=CARTESIAN_POINT('Ctrl Pts',(10.0795116959999,11.6,4.27890832199999));
#198316=CARTESIAN_POINT('Ctrl Pts',(10.0765500579999,15.2,4.27871394299999));
#198317=CARTESIAN_POINT('Ctrl Pts',(10.0765500579999,11.6,4.27871394299998));
#198318=CARTESIAN_POINT('Ctrl Pts',(10.0735940149999,15.2,4.27851748899998));
#198319=CARTESIAN_POINT('Ctrl Pts',(10.0735940149999,11.6,4.27851748899998));
#198320=CARTESIAN_POINT('Ctrl Pts',(10.0706435779999,15.2,4.27831896899999));
#198321=CARTESIAN_POINT('Ctrl Pts',(10.0706435779999,11.6,4.27831896899998));
#198322=CARTESIAN_POINT('Ctrl Pts',(10.0676987549999,15.2,4.27811839099999));
#198323=CARTESIAN_POINT('Ctrl Pts',(10.0676987549999,11.6,4.27811839099998));
#198324=CARTESIAN_POINT('Ctrl Pts',(10.0647595569999,15.2,4.27791576399999));
#198325=CARTESIAN_POINT('Ctrl Pts',(10.0647595569999,11.6,4.27791576399999));
#198326=CARTESIAN_POINT('Ctrl Pts',(10.0618259909999,15.2,4.27771109499999));
#198327=CARTESIAN_POINT('Ctrl Pts',(10.0618259909999,11.6,4.27771109499999));
#198328=CARTESIAN_POINT('Ctrl Pts',(10.0588980669999,15.2,4.27750439399999));
#198329=CARTESIAN_POINT('Ctrl Pts',(10.0588980669999,11.6,4.27750439399999));
#198330=CARTESIAN_POINT('Ctrl Pts',(10.0559757949999,15.2,4.27729566799999));
#198331=CARTESIAN_POINT('Ctrl Pts',(10.0559757949999,11.6,4.27729566799999));
#198332=CARTESIAN_POINT('Ctrl Pts',(10.0530591839999,15.2,4.27708492699999));
#198333=CARTESIAN_POINT('Ctrl Pts',(10.0530591839999,11.6,4.27708492699998));
#198334=CARTESIAN_POINT('Ctrl Pts',(10.0501482429999,15.2,4.27687217799999));
#198335=CARTESIAN_POINT('Ctrl Pts',(10.0501482429999,11.6,4.27687217799999));
#198336=CARTESIAN_POINT('Ctrl Pts',(10.0472429809999,15.2,4.27665743099999));
#198337=CARTESIAN_POINT('Ctrl Pts',(10.0472429809999,11.6,4.27665743099999));
#198338=CARTESIAN_POINT('Ctrl Pts',(10.0443434079999,15.2,4.27644069399998));
#198339=CARTESIAN_POINT('Ctrl Pts',(10.0443434079999,11.6,4.27644069399998));
#198340=CARTESIAN_POINT('Ctrl Pts',(10.0414495329999,15.2,4.27622197499999));
#198341=CARTESIAN_POINT('Ctrl Pts',(10.0414495329999,11.6,4.27622197499998));
#198342=CARTESIAN_POINT('Ctrl Pts',(10.0385613659999,15.2,4.27600128499999));
#198343=CARTESIAN_POINT('Ctrl Pts',(10.0385613659999,11.6,4.27600128499999));
#198344=CARTESIAN_POINT('Ctrl Pts',(10.0356789149999,15.2,4.27577862799998));
#198345=CARTESIAN_POINT('Ctrl Pts',(10.0356789149999,11.6,4.27577862799998));
#198346=CARTESIAN_POINT('Ctrl Pts',(10.0328021909999,15.2,4.27555401699999));
#198347=CARTESIAN_POINT('Ctrl Pts',(10.0328021909999,11.6,4.27555401699998));
#198348=CARTESIAN_POINT('Ctrl Pts',(10.0299312019999,15.2,4.27532745799999));
#198349=CARTESIAN_POINT('Ctrl Pts',(10.0299312019999,11.6,4.27532745799999));
#198350=CARTESIAN_POINT('Ctrl Pts',(10.0270659569999,15.2,4.27509896199999));
#198351=CARTESIAN_POINT('Ctrl Pts',(10.0270659569999,11.6,4.27509896199999));
#198352=CARTESIAN_POINT('Ctrl Pts',(10.0242064689999,15.2,4.27486853499998));
#198353=CARTESIAN_POINT('Ctrl Pts',(10.0242064689999,11.6,4.27486853499998));
#198354=CARTESIAN_POINT('Ctrl Pts',(10.0213527429999,15.2,4.27463618899999));
#198355=CARTESIAN_POINT('Ctrl Pts',(10.0213527429999,11.6,4.27463618899999));
#198356=CARTESIAN_POINT('Ctrl Pts',(10.0185047909999,15.2,4.27440193099999));
#198357=CARTESIAN_POINT('Ctrl Pts',(10.0185047909999,11.6,4.27440193099999));
#198358=CARTESIAN_POINT('Ctrl Pts',(10.0156626229999,15.2,4.27416576999998));
#198359=CARTESIAN_POINT('Ctrl Pts',(10.0156626229999,11.6,4.27416576999998));
#198360=CARTESIAN_POINT('Ctrl Pts',(10.0128262459999,15.2,4.27392771499999));
#198361=CARTESIAN_POINT('Ctrl Pts',(10.0128262459999,11.6,4.27392771499999));
#198362=CARTESIAN_POINT('Ctrl Pts',(10.0099956719999,15.2,4.27368777399998));
#198363=CARTESIAN_POINT('Ctrl Pts',(10.0099956719999,11.6,4.27368777399998));
#198364=CARTESIAN_POINT('Ctrl Pts',(10.0071709079999,15.2,4.27344595699999));
#198365=CARTESIAN_POINT('Ctrl Pts',(10.0071709079999,11.6,4.27344595699999));
#198366=CARTESIAN_POINT('Ctrl Pts',(10.0043519659999,15.2,4.27320227299998));
#198367=CARTESIAN_POINT('Ctrl Pts',(10.0043519659999,11.6,4.27320227299998));
#198368=CARTESIAN_POINT('Ctrl Pts',(10.0015388549999,15.2,4.27295673099999));
#198369=CARTESIAN_POINT('Ctrl Pts',(10.0015388549999,11.6,4.27295673099999));
#198370=CARTESIAN_POINT('Ctrl Pts',(9.99873158399994,15.2,4.27270933899998));
#198371=CARTESIAN_POINT('Ctrl Pts',(9.99873158399994,11.6,4.27270933899998));
#198372=CARTESIAN_POINT('Ctrl Pts',(9.99593016199994,15.2,4.27246010699999));
#198373=CARTESIAN_POINT('Ctrl Pts',(9.99593016199994,11.6,4.27246010699999));
#198374=CARTESIAN_POINT('Ctrl Pts',(9.99313459899994,15.2,4.27220904299999));
#198375=CARTESIAN_POINT('Ctrl Pts',(9.99313459899994,11.6,4.27220904299999));
#198376=CARTESIAN_POINT('Ctrl Pts',(9.99034490599995,15.2,4.27195615799998));
#198377=CARTESIAN_POINT('Ctrl Pts',(9.99034490599995,11.6,4.27195615799998));
#198378=CARTESIAN_POINT('Ctrl Pts',(9.98756109199994,15.2,4.27170146099999));
#198379=CARTESIAN_POINT('Ctrl Pts',(9.98756109199994,11.6,4.27170146099999));
#198380=CARTESIAN_POINT('Ctrl Pts',(9.98478316599994,15.2,4.27144495899999));
#198381=CARTESIAN_POINT('Ctrl Pts',(9.98478316599994,11.6,4.27144495899998));
#198382=CARTESIAN_POINT('Ctrl Pts',(9.98201113799994,15.2,4.27118666199998));
#198383=CARTESIAN_POINT('Ctrl Pts',(9.98201113799994,11.6,4.27118666199998));
#198384=CARTESIAN_POINT('Ctrl Pts',(9.97924501799995,15.2,4.27092657899999));
#198385=CARTESIAN_POINT('Ctrl Pts',(9.97924501799995,11.6,4.27092657899998));
#198386=CARTESIAN_POINT('Ctrl Pts',(9.97648481499994,15.2,4.27066472199999));
#198387=CARTESIAN_POINT('Ctrl Pts',(9.97648481499994,11.6,4.27066472199999));
#198388=CARTESIAN_POINT('Ctrl Pts',(9.97373053899994,15.2,4.27040109699998));
#198389=CARTESIAN_POINT('Ctrl Pts',(9.97373053899994,11.6,4.27040109699998));
#198390=CARTESIAN_POINT('Ctrl Pts',(9.97098220099994,15.2,4.27013571499998));
#198391=CARTESIAN_POINT('Ctrl Pts',(9.97098220099994,11.6,4.27013571499998));
#198392=CARTESIAN_POINT('Ctrl Pts',(9.96823980799994,15.2,4.26986858399999));
#198393=CARTESIAN_POINT('Ctrl Pts',(9.96823980799994,11.6,4.26986858399999));
#198394=CARTESIAN_POINT('Ctrl Pts',(9.96550337299994,15.2,4.26959971399998));
#198395=CARTESIAN_POINT('Ctrl Pts',(9.96550337299994,11.6,4.26959971399998));
#198396=CARTESIAN_POINT('Ctrl Pts',(9.96277290299994,15.2,4.26932911599998));
#198397=CARTESIAN_POINT('Ctrl Pts',(9.96277290299994,11.6,4.26932911599998));
#198398=CARTESIAN_POINT('Ctrl Pts',(9.96004841099994,15.2,4.26905679799999));
#198399=CARTESIAN_POINT('Ctrl Pts',(9.96004841099994,11.6,4.26905679799999));
#198400=CARTESIAN_POINT('Ctrl Pts',(9.95732990299994,15.2,4.26878276699998));
#198401=CARTESIAN_POINT('Ctrl Pts',(9.95732990299994,11.6,4.26878276699998));
#198402=CARTESIAN_POINT('Ctrl Pts',(9.95461739199994,15.2,4.26850703699999));
#198403=CARTESIAN_POINT('Ctrl Pts',(9.95461739199994,11.6,4.26850703699999));
#198404=CARTESIAN_POINT('Ctrl Pts',(9.95191088699995,15.2,4.26822961499998));
#198405=CARTESIAN_POINT('Ctrl Pts',(9.95191088699995,11.6,4.26822961499998));
#198406=CARTESIAN_POINT('Ctrl Pts',(9.94921039699994,15.2,4.26795051099998));
#198407=CARTESIAN_POINT('Ctrl Pts',(9.94921039699994,11.6,4.26795051099998));
#198408=CARTESIAN_POINT('Ctrl Pts',(9.94651593299994,15.2,4.26766973499999));
#198409=CARTESIAN_POINT('Ctrl Pts',(9.94651593299994,11.6,4.26766973499999));
#198410=CARTESIAN_POINT('Ctrl Pts',(9.94382750299994,15.2,4.26738729599998));
#198411=CARTESIAN_POINT('Ctrl Pts',(9.94382750299994,11.6,4.26738729599998));
#198412=CARTESIAN_POINT('Ctrl Pts',(9.94114511999994,15.2,4.26710320399999));
#198413=CARTESIAN_POINT('Ctrl Pts',(9.94114511999994,11.6,4.26710320399999));
#198414=CARTESIAN_POINT('Ctrl Pts',(9.93846879199995,15.2,4.26681746899998));
#198415=CARTESIAN_POINT('Ctrl Pts',(9.93846879199995,11.6,4.26681746899998));
#198416=CARTESIAN_POINT('Ctrl Pts',(9.93579852899994,15.2,4.26653009999999));
#198417=CARTESIAN_POINT('Ctrl Pts',(9.93579852899994,11.6,4.26653009999998));
#198418=CARTESIAN_POINT('Ctrl Pts',(9.93313434199995,15.2,4.26624110699999));
#198419=CARTESIAN_POINT('Ctrl Pts',(9.93313434199995,11.6,4.26624110699999));
#198420=CARTESIAN_POINT('Ctrl Pts',(9.93047623999994,15.2,4.26595049999998));
#198421=CARTESIAN_POINT('Ctrl Pts',(9.93047623999994,11.6,4.26595049999998));
#198422=CARTESIAN_POINT('Ctrl Pts',(9.92782423299994,15.2,4.26565828799998));
#198423=CARTESIAN_POINT('Ctrl Pts',(9.92782423299994,11.6,4.26565828799998));
#198424=CARTESIAN_POINT('Ctrl Pts',(9.92517833199994,15.2,4.26536448199998));
#198425=CARTESIAN_POINT('Ctrl Pts',(9.92517833199994,11.6,4.26536448199998));
#198426=CARTESIAN_POINT('Ctrl Pts',(9.92253854699995,15.2,4.26506909199999));
#198427=CARTESIAN_POINT('Ctrl Pts',(9.92253854699995,11.6,4.26506909199999));
#198428=CARTESIAN_POINT('Ctrl Pts',(9.91990488599994,15.2,4.26477212699999));
#198429=CARTESIAN_POINT('Ctrl Pts',(9.91990488599994,11.6,4.26477212699999));
#198430=CARTESIAN_POINT('Ctrl Pts',(9.91727736199995,15.2,4.26447359699999));
#198431=CARTESIAN_POINT('Ctrl Pts',(9.91727736199995,11.6,4.26447359699999));
#198432=CARTESIAN_POINT('Ctrl Pts',(9.91465598399994,15.2,4.26417351199999));
#198433=CARTESIAN_POINT('Ctrl Pts',(9.91465598399994,11.6,4.26417351199999));
#198434=CARTESIAN_POINT('Ctrl Pts',(9.91204076099995,15.2,4.26387188299999));
#198435=CARTESIAN_POINT('Ctrl Pts',(9.91204076099995,11.6,4.26387188299999));
#198436=CARTESIAN_POINT('Ctrl Pts',(9.90943170599994,15.2,4.26356871799998));
#198437=CARTESIAN_POINT('Ctrl Pts',(9.90943170599994,11.6,4.26356871799998));
#198438=CARTESIAN_POINT('Ctrl Pts',(9.90682882599994,15.2,4.26326402999998));
#198439=CARTESIAN_POINT('Ctrl Pts',(9.90682882599994,11.6,4.26326402999998));
#198440=CARTESIAN_POINT('Ctrl Pts',(9.90423213299995,15.2,4.26295782599999));
#198441=CARTESIAN_POINT('Ctrl Pts',(9.90423213299995,11.6,4.26295782599999));
#198442=CARTESIAN_POINT('Ctrl Pts',(9.90164163699994,15.2,4.26265011899999));
#198443=CARTESIAN_POINT('Ctrl Pts',(9.90164163699994,11.6,4.26265011899999));
#198444=CARTESIAN_POINT('Ctrl Pts',(9.89905734899994,15.2,4.26234091699998));
#198445=CARTESIAN_POINT('Ctrl Pts',(9.89905734899994,11.6,4.26234091699998));
#198446=CARTESIAN_POINT('Ctrl Pts',(9.89647927699994,15.2,4.26203023099998));
#198447=CARTESIAN_POINT('Ctrl Pts',(9.89647927699994,11.6,4.26203023099998));
#198448=CARTESIAN_POINT('Ctrl Pts',(9.89390743399994,15.2,4.26171807099998));
#198449=CARTESIAN_POINT('Ctrl Pts',(9.89390743399994,11.6,4.26171807099998));
#198450=CARTESIAN_POINT('Ctrl Pts',(9.89134182899994,15.2,4.26140444699998));
#198451=CARTESIAN_POINT('Ctrl Pts',(9.89134182899994,11.6,4.26140444699998));
#198452=CARTESIAN_POINT('Ctrl Pts',(9.88878247099995,15.2,4.26108937099999));
#198453=CARTESIAN_POINT('Ctrl Pts',(9.88878247099995,11.6,4.26108937099999));
#198454=CARTESIAN_POINT('Ctrl Pts',(9.88622937299995,15.2,4.26077285299999));
#198455=CARTESIAN_POINT('Ctrl Pts',(9.88622937299995,11.6,4.26077285299998));
#198456=CARTESIAN_POINT('Ctrl Pts',(9.88368254299995,15.2,4.26045490099998));
#198457=CARTESIAN_POINT('Ctrl Pts',(9.88368254299995,11.6,4.26045490099998));
#198458=CARTESIAN_POINT('Ctrl Pts',(9.88114199299994,15.2,4.26013552799999));
#198459=CARTESIAN_POINT('Ctrl Pts',(9.88114199299994,11.6,4.26013552799999));
#198460=CARTESIAN_POINT('Ctrl Pts',(9.87860773299994,15.2,4.25981474199999));
#198461=CARTESIAN_POINT('Ctrl Pts',(9.87860773299994,11.6,4.25981474199998));
#198462=CARTESIAN_POINT('Ctrl Pts',(9.87607977299995,15.2,4.25949255699998));
#198463=CARTESIAN_POINT('Ctrl Pts',(9.87607977299995,11.6,4.25949255699998));
#198464=CARTESIAN_POINT('Ctrl Pts',(9.87355812499995,15.2,4.25916897999999));
#198465=CARTESIAN_POINT('Ctrl Pts',(9.87355812499995,11.6,4.25916897999999));
#198466=CARTESIAN_POINT('Ctrl Pts',(9.87104279699994,15.2,4.25884402399999));
#198467=CARTESIAN_POINT('Ctrl Pts',(9.87104279699994,11.6,4.25884402399998));
#198468=CARTESIAN_POINT('Ctrl Pts',(9.86853379999994,15.2,4.25851769899998));
#198469=CARTESIAN_POINT('Ctrl Pts',(9.86853379999994,11.6,4.25851769899998));
#198470=CARTESIAN_POINT('Ctrl Pts',(9.86603114699994,15.2,4.25819001399999));
#198471=CARTESIAN_POINT('Ctrl Pts',(9.86603114699994,11.6,4.25819001399999));
#198472=CARTESIAN_POINT('Ctrl Pts',(9.86353484599995,15.2,4.25786098199998));
#198473=CARTESIAN_POINT('Ctrl Pts',(9.86353484599995,11.6,4.25786098199998));
#198474=CARTESIAN_POINT('Ctrl Pts',(9.86104490799995,15.2,4.25753061299999));
#198475=CARTESIAN_POINT('Ctrl Pts',(9.86104490799995,11.6,4.25753061299999));
#198476=CARTESIAN_POINT('Ctrl Pts',(9.85856134499994,15.2,4.25719891699998));
#198477=CARTESIAN_POINT('Ctrl Pts',(9.85856134499994,11.6,4.25719891699998));
#198478=CARTESIAN_POINT('Ctrl Pts',(9.85608416599994,15.2,4.25686590499998));
#198479=CARTESIAN_POINT('Ctrl Pts',(9.85608416599994,11.6,4.25686590499998));
#198480=CARTESIAN_POINT('Ctrl Pts',(9.85361338199995,15.2,4.25653158799999));
#198481=CARTESIAN_POINT('Ctrl Pts',(9.85361338199995,11.6,4.25653158799999));
#198482=CARTESIAN_POINT('Ctrl Pts',(9.85114900399994,15.2,4.25619597799999));
#198483=CARTESIAN_POINT('Ctrl Pts',(9.85114900399994,11.6,4.25619597799999));
#198484=CARTESIAN_POINT('Ctrl Pts',(9.84869104299994,15.2,4.25585908399999));
#198485=CARTESIAN_POINT('Ctrl Pts',(9.84869104299994,11.6,4.25585908399999));
#198486=CARTESIAN_POINT('Ctrl Pts',(9.84623950799994,15.2,4.25552091799998));
#198487=CARTESIAN_POINT('Ctrl Pts',(9.84623950799994,11.6,4.25552091799998));
#198488=CARTESIAN_POINT('Ctrl Pts',(9.84379441199994,15.2,4.25518149099998));
#198489=CARTESIAN_POINT('Ctrl Pts',(9.84379441199994,11.6,4.25518149099998));
#198490=CARTESIAN_POINT('Ctrl Pts',(9.84135576399994,15.2,4.25484081399999));
#198491=CARTESIAN_POINT('Ctrl Pts',(9.84135576399994,11.6,4.25484081399999));
#198492=CARTESIAN_POINT('Ctrl Pts',(9.83892357499995,15.2,4.25449889699999));
#198493=CARTESIAN_POINT('Ctrl Pts',(9.83892357499995,11.6,4.25449889699998));
#198494=CARTESIAN_POINT('Ctrl Pts',(9.83649785699994,15.2,4.25415575299999));
#198495=CARTESIAN_POINT('Ctrl Pts',(9.83649785699994,11.6,4.25415575299999));
#198496=CARTESIAN_POINT('Ctrl Pts',(9.83407861999994,15.2,4.25381139099999));
#198497=CARTESIAN_POINT('Ctrl Pts',(9.83407861999994,11.6,4.25381139099999));
#198498=CARTESIAN_POINT('Ctrl Pts',(9.83166587499994,15.2,4.25346582299999));
#198499=CARTESIAN_POINT('Ctrl Pts',(9.83166587499994,11.6,4.25346582299999));
#198500=CARTESIAN_POINT('Ctrl Pts',(9.82925963199994,15.2,4.25311906199998));
#198501=CARTESIAN_POINT('Ctrl Pts',(9.82925963199994,11.6,4.25311906199998));
#198502=CARTESIAN_POINT('Ctrl Pts',(9.82685990299995,15.2,4.25277111699998));
#198503=CARTESIAN_POINT('Ctrl Pts',(9.82685990299995,11.6,4.25277111699998));
#198504=CARTESIAN_POINT('Ctrl Pts',(9.82446669799995,15.2,4.25242199999998));
#198505=CARTESIAN_POINT('Ctrl Pts',(9.82446669799995,11.6,4.25242199999998));
#198506=CARTESIAN_POINT('Ctrl Pts',(9.82208002799995,15.2,4.25207172099999));
#198507=CARTESIAN_POINT('Ctrl Pts',(9.82208002799995,11.6,4.25207172099998));
#198508=CARTESIAN_POINT('Ctrl Pts',(9.81969990499995,15.2,4.25172029499999));
#198509=CARTESIAN_POINT('Ctrl Pts',(9.81969990499995,11.6,4.25172029499999));
#198510=CARTESIAN_POINT('Ctrl Pts',(9.81732633899994,15.2,4.25136772899998));
#198511=CARTESIAN_POINT('Ctrl Pts',(9.81732633899994,11.6,4.25136772899998));
#198512=CARTESIAN_POINT('Ctrl Pts',(9.81495934099994,15.2,4.25101403799999));
#198513=CARTESIAN_POINT('Ctrl Pts',(9.81495934099994,11.6,4.25101403799999));
#198514=CARTESIAN_POINT('Ctrl Pts',(9.81259892299994,15.2,4.25065923199998));
#198515=CARTESIAN_POINT('Ctrl Pts',(9.81259892299994,11.6,4.25065923199998));
#198516=CARTESIAN_POINT('Ctrl Pts',(9.81024509399995,15.2,4.25030332099999));
#198517=CARTESIAN_POINT('Ctrl Pts',(9.81024509399995,11.6,4.25030332099999));
#198518=CARTESIAN_POINT('Ctrl Pts',(9.80789786799994,15.2,4.24994631899998));
#198519=CARTESIAN_POINT('Ctrl Pts',(9.80789786799994,11.6,4.24994631899998));
#198520=CARTESIAN_POINT('Ctrl Pts',(9.80555725299994,15.2,4.24958823699999));
#198521=CARTESIAN_POINT('Ctrl Pts',(9.80555725299994,11.6,4.24958823699999));
#198522=CARTESIAN_POINT('Ctrl Pts',(9.80322326199994,15.2,4.24922908599999));
#198523=CARTESIAN_POINT('Ctrl Pts',(9.80322326199994,11.6,4.24922908599999));
#198524=CARTESIAN_POINT('Ctrl Pts',(9.80089590499994,15.2,4.24886887799998));
#198525=CARTESIAN_POINT('Ctrl Pts',(9.80089590499994,11.6,4.24886887799998));
#198526=CARTESIAN_POINT('Ctrl Pts',(9.79857519499994,15.2,4.24850762499998));
#198527=CARTESIAN_POINT('Ctrl Pts',(9.79857519499994,11.6,4.24850762499998));
#198528=CARTESIAN_POINT('Ctrl Pts',(9.79626114099995,15.2,4.24814533899998));
#198529=CARTESIAN_POINT('Ctrl Pts',(9.79626114099995,11.6,4.24814533899998));
#198530=CARTESIAN_POINT('Ctrl Pts',(9.79395375499994,15.2,4.24778202999998));
#198531=CARTESIAN_POINT('Ctrl Pts',(9.79395375499994,11.6,4.24778202999998));
#198532=CARTESIAN_POINT('Ctrl Pts',(9.79165304999994,15.2,4.24741771299999));
#198533=CARTESIAN_POINT('Ctrl Pts',(9.79165304999994,11.6,4.24741771299998));
#198534=CARTESIAN_POINT('Ctrl Pts',(9.78935903399995,15.2,4.24705239699998));
#198535=CARTESIAN_POINT('Ctrl Pts',(9.78935903399995,11.6,4.24705239699998));
#198536=CARTESIAN_POINT('Ctrl Pts',(9.78707171999995,15.2,4.24668609599999));
#198537=CARTESIAN_POINT('Ctrl Pts',(9.78707171999995,11.6,4.24668609599998));
#198538=CARTESIAN_POINT('Ctrl Pts',(9.78479111999994,15.2,4.24631881999999));
#198539=CARTESIAN_POINT('Ctrl Pts',(9.78479111999994,11.6,4.24631881999998));
#198540=CARTESIAN_POINT('Ctrl Pts',(9.78251724499994,15.2,4.24595058299998));
#198541=CARTESIAN_POINT('Ctrl Pts',(9.78251724499994,11.6,4.24595058299998));
#198542=CARTESIAN_POINT('Ctrl Pts',(9.78025010499995,15.2,4.24558139499998));
#198543=CARTESIAN_POINT('Ctrl Pts',(9.78025010499995,11.6,4.24558139499998));
#198544=CARTESIAN_POINT('Ctrl Pts',(9.77798971299995,15.2,4.24521127099998));
#198545=CARTESIAN_POINT('Ctrl Pts',(9.77798971299995,11.6,4.24521127099998));
#198546=CARTESIAN_POINT('Ctrl Pts',(9.77573607899994,15.2,4.24484021999999));
#198547=CARTESIAN_POINT('Ctrl Pts',(9.77573607899994,11.6,4.24484021999999));
#198548=CARTESIAN_POINT('Ctrl Pts',(9.77348921599994,15.2,4.24446825699999));
#198549=CARTESIAN_POINT('Ctrl Pts',(9.77348921599994,11.6,4.24446825699999));
#198550=CARTESIAN_POINT('Ctrl Pts',(9.77124913399994,15.2,4.24409539199999));
#198551=CARTESIAN_POINT('Ctrl Pts',(9.77124913399994,11.6,4.24409539199999));
#198552=CARTESIAN_POINT('Ctrl Pts',(9.76901584499995,15.2,4.24372163899999));
#198553=CARTESIAN_POINT('Ctrl Pts',(9.76901584499995,11.6,4.24372163899999));
#198554=CARTESIAN_POINT('Ctrl Pts',(9.76678936099994,15.2,4.24334700899998));
#198555=CARTESIAN_POINT('Ctrl Pts',(9.76678936099994,11.6,4.24334700899998));
#198556=CARTESIAN_POINT('Ctrl Pts',(9.76456969299995,15.2,4.24297151599998));
#198557=CARTESIAN_POINT('Ctrl Pts',(9.76456969299995,11.6,4.24297151599998));
#198558=CARTESIAN_POINT('Ctrl Pts',(9.76235685299994,15.2,4.24259516999999));
#198559=CARTESIAN_POINT('Ctrl Pts',(9.76235685299994,11.6,4.24259516999999));
#198560=CARTESIAN_POINT('Ctrl Pts',(9.76015085199995,15.2,4.24221798599999));
#198561=CARTESIAN_POINT('Ctrl Pts',(9.76015085199995,11.6,4.24221798599999));
#198562=CARTESIAN_POINT('Ctrl Pts',(9.75795170099994,15.2,4.24183997499998));
#198563=CARTESIAN_POINT('Ctrl Pts',(9.75795170099994,11.6,4.24183997499998));
#198564=CARTESIAN_POINT('Ctrl Pts',(9.75575941399994,15.2,4.24146114999999));
#198565=CARTESIAN_POINT('Ctrl Pts',(9.75575941399994,11.6,4.24146114999999));
#198566=CARTESIAN_POINT('Ctrl Pts',(9.75357400199995,15.2,4.24108152299999));
#198567=CARTESIAN_POINT('Ctrl Pts',(9.75357400199995,11.6,4.24108152299999));
#198568=CARTESIAN_POINT('Ctrl Pts',(9.75139547399994,15.2,4.24070110799998));
#198569=CARTESIAN_POINT('Ctrl Pts',(9.75139547399994,11.6,4.24070110799998));
#198570=CARTESIAN_POINT('Ctrl Pts',(9.74922384499994,15.2,4.24031991699999));
#198571=CARTESIAN_POINT('Ctrl Pts',(9.74922384499994,11.6,4.24031991699999));
#198572=CARTESIAN_POINT('Ctrl Pts',(9.74705912399994,15.2,4.23993796299998));
#198573=CARTESIAN_POINT('Ctrl Pts',(9.74705912399994,11.6,4.23993796299998));
#198574=CARTESIAN_POINT('Ctrl Pts',(9.74490132599995,15.2,4.23955525799999));
#198575=CARTESIAN_POINT('Ctrl Pts',(9.74490132599995,11.6,4.23955525799998));
#198576=CARTESIAN_POINT('Ctrl Pts',(9.74275045999994,15.2,4.23917181499998));
#198577=CARTESIAN_POINT('Ctrl Pts',(9.74275045999994,11.6,4.23917181499998));
#198578=CARTESIAN_POINT('Ctrl Pts',(9.74060653799994,15.2,4.23878764799999));
#198579=CARTESIAN_POINT('Ctrl Pts',(9.74060653799994,11.6,4.23878764799999));
#198580=CARTESIAN_POINT('Ctrl Pts',(9.73846957399994,15.2,4.23840276899998));
#198581=CARTESIAN_POINT('Ctrl Pts',(9.73846957399994,11.6,4.23840276899998));
#198582=CARTESIAN_POINT('Ctrl Pts',(9.73633957899994,15.2,4.23801719199999));
#198583=CARTESIAN_POINT('Ctrl Pts',(9.73633957899994,11.6,4.23801719199999));
#198584=CARTESIAN_POINT('Ctrl Pts',(9.73421656399994,15.2,4.23763092799998));
#198585=CARTESIAN_POINT('Ctrl Pts',(9.73421656399994,11.6,4.23763092799998));
#198586=CARTESIAN_POINT('Ctrl Pts',(9.73210054099994,15.2,4.23724399299999));
#198587=CARTESIAN_POINT('Ctrl Pts',(9.73210054099994,11.6,4.23724399299999));
#198588=CARTESIAN_POINT('Ctrl Pts',(9.72999152299994,15.2,4.23685639699999));
#198589=CARTESIAN_POINT('Ctrl Pts',(9.72999152299994,11.6,4.23685639699999));
#198590=CARTESIAN_POINT('Ctrl Pts',(9.72788952199994,15.2,4.23646815499998));
#198591=CARTESIAN_POINT('Ctrl Pts',(9.72788952199994,11.6,4.23646815499998));
#198592=CARTESIAN_POINT('Ctrl Pts',(9.72579454899994,15.2,4.23607928199999));
#198593=CARTESIAN_POINT('Ctrl Pts',(9.72579454899994,11.6,4.23607928199999));
#198594=CARTESIAN_POINT('Ctrl Pts',(9.72370661699994,15.2,4.23568978799998));
#198595=CARTESIAN_POINT('Ctrl Pts',(9.72370661699994,11.6,4.23568978799998));
#198596=CARTESIAN_POINT('Ctrl Pts',(9.72162573699995,15.2,4.23529968699999));
#198597=CARTESIAN_POINT('Ctrl Pts',(9.72162573699995,11.6,4.23529968699999));
#198598=CARTESIAN_POINT('Ctrl Pts',(9.71955192299994,15.2,4.23490899299999));
#198599=CARTESIAN_POINT('Ctrl Pts',(9.71955192299994,11.6,4.23490899299999));
#198600=CARTESIAN_POINT('Ctrl Pts',(9.71748518499994,15.2,4.23451771999999));
#198601=CARTESIAN_POINT('Ctrl Pts',(9.71748518499994,11.6,4.23451771999999));
#198602=CARTESIAN_POINT('Ctrl Pts',(9.71542553799994,15.2,4.23412587999999));
#198603=CARTESIAN_POINT('Ctrl Pts',(9.71542553799994,11.6,4.23412587999999));
#198604=CARTESIAN_POINT('Ctrl Pts',(9.71337299099994,15.2,4.23373348899998));
#198605=CARTESIAN_POINT('Ctrl Pts',(9.71337299099994,11.6,4.23373348899998));
#198606=CARTESIAN_POINT('Ctrl Pts',(9.71132755699994,15.2,4.23334055899999));
#198607=CARTESIAN_POINT('Ctrl Pts',(9.71132755699994,11.6,4.23334055899998));
#198608=CARTESIAN_POINT('Ctrl Pts',(9.70928924999994,15.2,4.23294710199999));
#198609=CARTESIAN_POINT('Ctrl Pts',(9.70928924999994,11.6,4.23294710199999));
#198610=CARTESIAN_POINT('Ctrl Pts',(9.70725808099995,15.2,4.23255313599999));
#198611=CARTESIAN_POINT('Ctrl Pts',(9.70725808099995,11.6,4.23255313599998));
#198612=CARTESIAN_POINT('Ctrl Pts',(9.70523406399994,15.2,4.23215867099999));
#198613=CARTESIAN_POINT('Ctrl Pts',(9.70523406399994,11.6,4.23215867099999));
#198614=CARTESIAN_POINT('Ctrl Pts',(9.70321720799994,15.2,4.23176372099999));
#198615=CARTESIAN_POINT('Ctrl Pts',(9.70321720799994,11.6,4.23176372099998));
#198616=CARTESIAN_POINT('Ctrl Pts',(9.70120752899994,15.2,4.23136830299998));
#198617=CARTESIAN_POINT('Ctrl Pts',(9.70120752899994,11.6,4.23136830299998));
#198618=CARTESIAN_POINT('Ctrl Pts',(9.69920503699995,15.2,4.23097242699999));
#198619=CARTESIAN_POINT('Ctrl Pts',(9.69920503699995,11.6,4.23097242699999));
#198620=CARTESIAN_POINT('Ctrl Pts',(9.69720974699994,15.2,4.23057611099999));
#198621=CARTESIAN_POINT('Ctrl Pts',(9.69720974699994,11.6,4.23057611099999));
#198622=CARTESIAN_POINT('Ctrl Pts',(9.69522166799995,15.2,4.23017936499999));
#198623=CARTESIAN_POINT('Ctrl Pts',(9.69522166799995,11.6,4.23017936499999));
#198624=CARTESIAN_POINT('Ctrl Pts',(9.69324081599994,15.2,4.22978220499999));
#198625=CARTESIAN_POINT('Ctrl Pts',(9.69324081599994,11.6,4.22978220499999));
#198626=CARTESIAN_POINT('Ctrl Pts',(9.69126720099995,15.2,4.22938464599999));
#198627=CARTESIAN_POINT('Ctrl Pts',(9.69126720099995,11.6,4.22938464599999));
#198628=CARTESIAN_POINT('Ctrl Pts',(9.68930083599994,15.2,4.22898670099999));
#198629=CARTESIAN_POINT('Ctrl Pts',(9.68930083599994,11.6,4.22898670099999));
#198630=CARTESIAN_POINT('Ctrl Pts',(9.68734173699995,15.2,4.22858838399998));
#198631=CARTESIAN_POINT('Ctrl Pts',(9.68734173699995,11.6,4.22858838399998));
#198632=CARTESIAN_POINT('Ctrl Pts',(9.68538991099994,15.2,4.22818970999998));
#198633=CARTESIAN_POINT('Ctrl Pts',(9.68538991099994,11.6,4.22818970999998));
#198634=CARTESIAN_POINT('Ctrl Pts',(9.68344537499994,15.2,4.22779069299998));
#198635=CARTESIAN_POINT('Ctrl Pts',(9.68344537499994,11.6,4.22779069299998));
#198636=CARTESIAN_POINT('Ctrl Pts',(9.68150813999994,15.2,4.22739134799999));
#198637=CARTESIAN_POINT('Ctrl Pts',(9.68150813999994,11.6,4.22739134799999));
#198638=CARTESIAN_POINT('Ctrl Pts',(9.67957821999994,15.2,4.22699168799999));
#198639=CARTESIAN_POINT('Ctrl Pts',(9.67957821999994,11.6,4.22699168799998));
#198640=CARTESIAN_POINT('Ctrl Pts',(9.67765562599994,15.2,4.22659172999998));
#198641=CARTESIAN_POINT('Ctrl Pts',(9.67765562599994,11.6,4.22659172999998));
#198642=CARTESIAN_POINT('Ctrl Pts',(9.67574037299994,15.2,4.22619148699999));
#198643=CARTESIAN_POINT('Ctrl Pts',(9.67574037299994,11.6,4.22619148699999));
#198644=CARTESIAN_POINT('Ctrl Pts',(9.67383247099994,15.2,4.22579097199999));
#198645=CARTESIAN_POINT('Ctrl Pts',(9.67383247099994,11.6,4.22579097199998));
#198646=CARTESIAN_POINT('Ctrl Pts',(9.67193193599994,15.2,4.22539020399999));
#198647=CARTESIAN_POINT('Ctrl Pts',(9.67193193599994,11.6,4.22539020399998));
#198648=CARTESIAN_POINT('Ctrl Pts',(9.67003877899995,15.2,4.22498919399998));
#198649=CARTESIAN_POINT('Ctrl Pts',(9.67003877899995,11.6,4.22498919399998));
#198650=CARTESIAN_POINT('Ctrl Pts',(9.66815301399994,15.2,4.22458795799999));
#198651=CARTESIAN_POINT('Ctrl Pts',(9.66815301399994,11.6,4.22458795799999));
#198652=CARTESIAN_POINT('Ctrl Pts',(9.66627465299995,15.2,4.22418651099999));
#198653=CARTESIAN_POINT('Ctrl Pts',(9.66627465299995,11.6,4.22418651099999));
#198654=CARTESIAN_POINT('Ctrl Pts',(9.66440370999995,15.2,4.22378486799998));
#198655=CARTESIAN_POINT('Ctrl Pts',(9.66440370999995,11.6,4.22378486799998));
#198656=CARTESIAN_POINT('Ctrl Pts',(9.66254019799995,15.2,4.22338304499998));
#198657=CARTESIAN_POINT('Ctrl Pts',(9.66254019799995,11.6,4.22338304499998));
#198658=CARTESIAN_POINT('Ctrl Pts',(9.66068412999994,15.2,4.22298105399998));
#198659=CARTESIAN_POINT('Ctrl Pts',(9.66068412999994,11.6,4.22298105399998));
#198660=CARTESIAN_POINT('Ctrl Pts',(9.65883551799994,15.2,4.22257891399998));
#198661=CARTESIAN_POINT('Ctrl Pts',(9.65883551799994,11.6,4.22257891399998));
#198662=CARTESIAN_POINT('Ctrl Pts',(9.65699437699995,15.2,4.22217663699998));
#198663=CARTESIAN_POINT('Ctrl Pts',(9.65699437699995,11.6,4.22217663699998));
#198664=CARTESIAN_POINT('Ctrl Pts',(9.65516071899994,15.2,4.22177423999998));
#198665=CARTESIAN_POINT('Ctrl Pts',(9.65516071899994,11.6,4.22177423999998));
#198666=CARTESIAN_POINT('Ctrl Pts',(9.65333455799994,15.2,4.22137173699999));
#198667=CARTESIAN_POINT('Ctrl Pts',(9.65333455799994,11.6,4.22137173699999));
#198668=CARTESIAN_POINT('Ctrl Pts',(9.65151590799995,15.2,4.22096914499999));
#198669=CARTESIAN_POINT('Ctrl Pts',(9.65151590799995,11.6,4.22096914499999));
#198670=CARTESIAN_POINT('Ctrl Pts',(9.64970477999995,15.2,4.22056647799998));
#198671=CARTESIAN_POINT('Ctrl Pts',(9.64970477999995,11.6,4.22056647799998));
#198672=CARTESIAN_POINT('Ctrl Pts',(9.64790118899994,15.2,4.22016375299999));
#198673=CARTESIAN_POINT('Ctrl Pts',(9.64790118899994,11.6,4.22016375299999));
#198674=CARTESIAN_POINT('Ctrl Pts',(9.64610514899995,15.2,4.21976098399998));
#198675=CARTESIAN_POINT('Ctrl Pts',(9.64610514899995,11.6,4.21976098399998));
#198676=CARTESIAN_POINT('Ctrl Pts',(9.64431667199995,15.2,4.21935818699998));
#198677=CARTESIAN_POINT('Ctrl Pts',(9.64431667199995,11.6,4.21935818699998));
#198678=CARTESIAN_POINT('Ctrl Pts',(9.64253577199995,15.2,4.21895537799998));
#198679=CARTESIAN_POINT('Ctrl Pts',(9.64253577199995,11.6,4.21895537799998));
#198680=CARTESIAN_POINT('Ctrl Pts',(9.64076246299994,15.2,4.21855257399999));
#198681=CARTESIAN_POINT('Ctrl Pts',(9.64076246299994,11.6,4.21855257399999));
#198682=CARTESIAN_POINT('Ctrl Pts',(9.63899675899994,15.2,4.21814978799999));
#198683=CARTESIAN_POINT('Ctrl Pts',(9.63899675899994,11.6,4.21814978799999));
#198684=CARTESIAN_POINT('Ctrl Pts',(9.63723867199995,15.2,4.21774703799999));
#198685=CARTESIAN_POINT('Ctrl Pts',(9.63723867199995,11.6,4.21774703799999));
#198686=CARTESIAN_POINT('Ctrl Pts',(9.63548821799994,15.2,4.21734433899999));
#198687=CARTESIAN_POINT('Ctrl Pts',(9.63548821799994,11.6,4.21734433899999));
#198688=CARTESIAN_POINT('Ctrl Pts',(9.63374540699995,15.2,4.21694170799999));
#198689=CARTESIAN_POINT('Ctrl Pts',(9.63374540699995,11.6,4.21694170799999));
#198690=CARTESIAN_POINT('Ctrl Pts',(9.63201025599994,15.2,4.21653915999999));
#198691=CARTESIAN_POINT('Ctrl Pts',(9.63201025599994,11.6,4.21653915999998));
#198692=CARTESIAN_POINT('Ctrl Pts',(9.63028277899994,15.2,4.21613671099998));
#198693=CARTESIAN_POINT('Ctrl Pts',(9.63028277899994,11.6,4.21613671099998));
#198694=CARTESIAN_POINT('Ctrl Pts',(9.62856298699995,15.2,4.21573437799999));
#198695=CARTESIAN_POINT('Ctrl Pts',(9.62856298699995,11.6,4.21573437799999));
#198696=CARTESIAN_POINT('Ctrl Pts',(9.62685089699994,15.2,4.21533217699999));
#198697=CARTESIAN_POINT('Ctrl Pts',(9.62685089699994,11.6,4.21533217699999));
#198698=CARTESIAN_POINT('Ctrl Pts',(9.62514652099994,15.2,4.21493012499998));
#198699=CARTESIAN_POINT('Ctrl Pts',(9.62514652099994,11.6,4.21493012499998));
#198700=CARTESIAN_POINT('Ctrl Pts',(9.62344987299995,15.2,4.21452823799999));
#198701=CARTESIAN_POINT('Ctrl Pts',(9.62344987299995,11.6,4.21452823799999));
#198702=CARTESIAN_POINT('Ctrl Pts',(9.62176096699995,15.2,4.21412653099999));
#198703=CARTESIAN_POINT('Ctrl Pts',(9.62176096699995,11.6,4.21412653099999));
#198704=CARTESIAN_POINT('Ctrl Pts',(9.62007981799994,15.2,4.21372502199999));
#198705=CARTESIAN_POINT('Ctrl Pts',(9.62007981799994,11.6,4.21372502199999));
#198706=CARTESIAN_POINT('Ctrl Pts',(9.61840643899994,15.2,4.21332372799998));
#198707=CARTESIAN_POINT('Ctrl Pts',(9.61840643899994,11.6,4.21332372799998));
#198708=CARTESIAN_POINT('Ctrl Pts',(9.61674084499995,15.2,4.21292266499999));
#198709=CARTESIAN_POINT('Ctrl Pts',(9.61674084499995,11.6,4.21292266499999));
#198710=CARTESIAN_POINT('Ctrl Pts',(9.61508304999995,15.2,4.21252184999998));
#198711=CARTESIAN_POINT('Ctrl Pts',(9.61508304999995,11.6,4.21252184999998));
#198712=CARTESIAN_POINT('Ctrl Pts',(9.61343306699994,15.2,4.21212129899998));
#198713=CARTESIAN_POINT('Ctrl Pts',(9.61343306699994,11.6,4.21212129899998));
#198714=CARTESIAN_POINT('Ctrl Pts',(9.61179091199994,15.2,4.21172103099998));
#198715=CARTESIAN_POINT('Ctrl Pts',(9.61179091199994,11.6,4.21172103099998));
#198716=CARTESIAN_POINT('Ctrl Pts',(9.61015659699994,15.2,4.21132105999998));
#198717=CARTESIAN_POINT('Ctrl Pts',(9.61015659699994,11.6,4.21132105999998));
#198718=CARTESIAN_POINT('Ctrl Pts',(9.60853013999994,15.2,4.21092140599999));
#198719=CARTESIAN_POINT('Ctrl Pts',(9.60853013999994,11.6,4.21092140599998));
#198720=CARTESIAN_POINT('Ctrl Pts',(9.60691155199994,15.2,4.21052208399999));
#198721=CARTESIAN_POINT('Ctrl Pts',(9.60691155199994,11.6,4.21052208399998));
#198722=CARTESIAN_POINT('Ctrl Pts',(9.60530084799995,15.2,4.21012311199998));
#198723=CARTESIAN_POINT('Ctrl Pts',(9.60530084799995,11.6,4.21012311199998));
#198724=CARTESIAN_POINT('Ctrl Pts',(9.60369804399994,15.2,4.20972450799999));
#198725=CARTESIAN_POINT('Ctrl Pts',(9.60369804399994,11.6,4.20972450799999));
#198726=CARTESIAN_POINT('Ctrl Pts',(9.60210315399994,15.2,4.20932628799999));
#198727=CARTESIAN_POINT('Ctrl Pts',(9.60210315399994,11.6,4.20932628799999));
#198728=CARTESIAN_POINT('Ctrl Pts',(9.60051619099995,15.2,4.20892846999998));
#198729=CARTESIAN_POINT('Ctrl Pts',(9.60051619099995,11.6,4.20892846999998));
#198730=CARTESIAN_POINT('Ctrl Pts',(9.59893717199994,15.2,4.20853107199999));
#198731=CARTESIAN_POINT('Ctrl Pts',(9.59893717199994,11.6,4.20853107199999));
#198732=CARTESIAN_POINT('Ctrl Pts',(9.59736610999995,15.2,4.20813410999998));
#198733=CARTESIAN_POINT('Ctrl Pts',(9.59736610999995,11.6,4.20813410999998));
#198734=CARTESIAN_POINT('Ctrl Pts',(9.59580301899994,15.2,4.20773760399998));
#198735=CARTESIAN_POINT('Ctrl Pts',(9.59580301899994,11.6,4.20773760399998));
#198736=CARTESIAN_POINT('Ctrl Pts',(9.59424791599995,15.2,4.20734156899999));
#198737=CARTESIAN_POINT('Ctrl Pts',(9.59424791599995,11.6,4.20734156899999));
#198738=CARTESIAN_POINT('Ctrl Pts',(9.59270081499995,15.2,4.20694602499999));
#198739=CARTESIAN_POINT('Ctrl Pts',(9.59270081499995,11.6,4.20694602499999));
#198740=CARTESIAN_POINT('Ctrl Pts',(9.59116172899994,15.2,4.20655098899999));
#198741=CARTESIAN_POINT('Ctrl Pts',(9.59116172899994,11.6,4.20655098899999));
#198742=CARTESIAN_POINT('Ctrl Pts',(9.58963067599995,15.2,4.20615647899999));
#198743=CARTESIAN_POINT('Ctrl Pts',(9.58963067599995,11.6,4.20615647899999));
#198744=CARTESIAN_POINT('Ctrl Pts',(9.58810766899994,15.2,4.20576251499998));
#198745=CARTESIAN_POINT('Ctrl Pts',(9.58810766899994,11.6,4.20576251499998));
#198746=CARTESIAN_POINT('Ctrl Pts',(9.58659272199995,15.2,4.20536911099998));
#198747=CARTESIAN_POINT('Ctrl Pts',(9.58659272199995,11.6,4.20536911099998));
#198748=CARTESIAN_POINT('Ctrl Pts',(9.58508585299995,15.2,4.20497628799998));
#198749=CARTESIAN_POINT('Ctrl Pts',(9.58508585299995,11.6,4.20497628799998));
#198750=CARTESIAN_POINT('Ctrl Pts',(9.58358707499994,15.2,4.20458406399998));
#198751=CARTESIAN_POINT('Ctrl Pts',(9.58358707499994,11.6,4.20458406399998));
#198752=CARTESIAN_POINT('Ctrl Pts',(9.58209640399994,15.2,4.20419245699998));
#198753=CARTESIAN_POINT('Ctrl Pts',(9.58209640399994,11.6,4.20419245699998));
#198754=CARTESIAN_POINT('Ctrl Pts',(9.58061385399994,15.2,4.20380148499999));
#198755=CARTESIAN_POINT('Ctrl Pts',(9.58061385399994,11.6,4.20380148499999));
#198756=CARTESIAN_POINT('Ctrl Pts',(9.57913944099994,15.2,4.20341116699999));
#198757=CARTESIAN_POINT('Ctrl Pts',(9.57913944099994,11.6,4.20341116699999));
#198758=CARTESIAN_POINT('Ctrl Pts',(9.57767318099994,15.2,4.20302152199999));
#198759=CARTESIAN_POINT('Ctrl Pts',(9.57767318099994,11.6,4.20302152199999));
#198760=CARTESIAN_POINT('Ctrl Pts',(9.57621508799994,15.2,4.20263256899998));
#198761=CARTESIAN_POINT('Ctrl Pts',(9.57621508799994,11.6,4.20263256899998));
#198762=CARTESIAN_POINT('Ctrl Pts',(9.57476517899994,15.2,4.20224432599999));
#198763=CARTESIAN_POINT('Ctrl Pts',(9.57476517899994,11.6,4.20224432599999));
#198764=CARTESIAN_POINT('Ctrl Pts',(9.57332346799994,15.2,4.20185681099999));
#198765=CARTESIAN_POINT('Ctrl Pts',(9.57332346799994,11.6,4.20185681099999));
#198766=CARTESIAN_POINT('Ctrl Pts',(9.57188996999994,15.2,4.20147004499999));
#198767=CARTESIAN_POINT('Ctrl Pts',(9.57188996999994,11.6,4.20147004499999));
#198768=CARTESIAN_POINT('Ctrl Pts',(9.57046470299994,15.2,4.20108404499998));
#198769=CARTESIAN_POINT('Ctrl Pts',(9.57046470299994,11.6,4.20108404499998));
#198770=CARTESIAN_POINT('Ctrl Pts',(9.56904768099994,15.2,4.20069883199999));
#198771=CARTESIAN_POINT('Ctrl Pts',(9.56904768099994,11.6,4.20069883199999));
#198772=CARTESIAN_POINT('Ctrl Pts',(9.56763891899995,15.2,4.20031442499998));
#198773=CARTESIAN_POINT('Ctrl Pts',(9.56763891899995,11.6,4.20031442499998));
#198774=CARTESIAN_POINT('Ctrl Pts',(9.56623843399995,15.2,4.19993084099998));
#198775=CARTESIAN_POINT('Ctrl Pts',(9.56623843399995,11.6,4.19993084099998));
#198776=CARTESIAN_POINT('Ctrl Pts',(9.56484624099994,15.2,4.19954810099998));
#198777=CARTESIAN_POINT('Ctrl Pts',(9.56484624099994,11.6,4.19954810099998));
#198778=CARTESIAN_POINT('Ctrl Pts',(9.56346235699994,15.2,4.19916622499999));
#198779=CARTESIAN_POINT('Ctrl Pts',(9.56346235699994,11.6,4.19916622499999));
#198780=CARTESIAN_POINT('Ctrl Pts',(9.56208679599994,15.2,4.19878523199999));
#198781=CARTESIAN_POINT('Ctrl Pts',(9.56208679599994,11.6,4.19878523199999));
#198782=CARTESIAN_POINT('Ctrl Pts',(9.56071957599995,15.2,4.19840514199999));
#198783=CARTESIAN_POINT('Ctrl Pts',(9.56071957599995,11.6,4.19840514199999));
#198784=CARTESIAN_POINT('Ctrl Pts',(9.55936071099994,15.2,4.19802597299999));
#198785=CARTESIAN_POINT('Ctrl Pts',(9.55936071099994,11.6,4.19802597299998));
#198786=CARTESIAN_POINT('Ctrl Pts',(9.55801021799994,15.2,4.19764774799999));
#198787=CARTESIAN_POINT('Ctrl Pts',(9.55801021799994,11.6,4.19764774799999));
#198788=CARTESIAN_POINT('Ctrl Pts',(9.55666811299994,15.2,4.19727048399999));
#198789=CARTESIAN_POINT('Ctrl Pts',(9.55666811299994,11.6,4.19727048399999));
#198790=CARTESIAN_POINT('Ctrl Pts',(9.55533441299995,15.2,4.19689420199998));
#198791=CARTESIAN_POINT('Ctrl Pts',(9.55533441299995,11.6,4.19689420199998));
#198792=CARTESIAN_POINT('Ctrl Pts',(9.55400913299994,15.2,4.19651892299999));
#198793=CARTESIAN_POINT('Ctrl Pts',(9.55400913299994,11.6,4.19651892299999));
#198794=CARTESIAN_POINT('Ctrl Pts',(9.55269228999994,15.2,4.19614466599998));
#198795=CARTESIAN_POINT('Ctrl Pts',(9.55269228999994,11.6,4.19614466599998));
#198796=CARTESIAN_POINT('Ctrl Pts',(9.55138389999994,15.2,4.19577145199998));
#198797=CARTESIAN_POINT('Ctrl Pts',(9.55138389999994,11.6,4.19577145199998));
#198798=CARTESIAN_POINT('Ctrl Pts',(9.55008397999995,15.2,4.19539930199999));
#198799=CARTESIAN_POINT('Ctrl Pts',(9.55008397999995,11.6,4.19539930199999));
#198800=CARTESIAN_POINT('Ctrl Pts',(9.54879254499994,15.2,4.19502823399998));
#198801=CARTESIAN_POINT('Ctrl Pts',(9.54879254499994,11.6,4.19502823399998));
#198802=CARTESIAN_POINT('Ctrl Pts',(9.54750961299995,15.2,4.19465827199998));
#198803=CARTESIAN_POINT('Ctrl Pts',(9.54750961299995,11.6,4.19465827199998));
#198804=CARTESIAN_POINT('Ctrl Pts',(9.54623519999994,15.2,4.19428943299998));
#198805=CARTESIAN_POINT('Ctrl Pts',(9.54623519999994,11.6,4.19428943299998));
#198806=CARTESIAN_POINT('Ctrl Pts',(9.54496932299995,15.2,4.19392174099999));
#198807=CARTESIAN_POINT('Ctrl Pts',(9.54496932299995,11.6,4.19392174099999));
#198808=CARTESIAN_POINT('Ctrl Pts',(9.54371199799994,15.2,4.19355521499998));
#198809=CARTESIAN_POINT('Ctrl Pts',(9.54371199799994,11.6,4.19355521499998));
#198810=CARTESIAN_POINT('Ctrl Pts',(9.54246324199995,15.2,4.19318987699998));
#198811=CARTESIAN_POINT('Ctrl Pts',(9.54246324199995,11.6,4.19318987699998));
#198812=CARTESIAN_POINT('Ctrl Pts',(9.54122307199994,15.2,4.19282574899999));
#198813=CARTESIAN_POINT('Ctrl Pts',(9.54122307199994,11.6,4.19282574899999));
#198814=CARTESIAN_POINT('Ctrl Pts',(9.53999150599994,15.2,4.19246284899998));
#198815=CARTESIAN_POINT('Ctrl Pts',(9.53999150599994,11.6,4.19246284899998));
#198816=CARTESIAN_POINT('Ctrl Pts',(9.53876855799994,15.2,4.19210119999998));
#198817=CARTESIAN_POINT('Ctrl Pts',(9.53876855799994,11.6,4.19210119999998));
#198818=CARTESIAN_POINT('Ctrl Pts',(9.53755424799994,15.2,4.19174082399999));
#198819=CARTESIAN_POINT('Ctrl Pts',(9.53755424799994,11.6,4.19174082399999));
#198820=CARTESIAN_POINT('Ctrl Pts',(9.53634859199994,15.2,4.19138174299999));
#198821=CARTESIAN_POINT('Ctrl Pts',(9.53634859199994,11.6,4.19138174299999));
#198822=CARTESIAN_POINT('Ctrl Pts',(9.53515160699995,15.2,4.19102397699999));
#198823=CARTESIAN_POINT('Ctrl Pts',(9.53515160699995,11.6,4.19102397699999));
#198824=CARTESIAN_POINT('Ctrl Pts',(9.53396331099994,15.2,4.19066754699998));
#198825=CARTESIAN_POINT('Ctrl Pts',(9.53396331099994,11.6,4.19066754699998));
#198826=CARTESIAN_POINT('Ctrl Pts',(9.53278371899994,15.2,4.19031247799998));
#198827=CARTESIAN_POINT('Ctrl Pts',(9.53278371899994,11.6,4.19031247799998));
#198828=CARTESIAN_POINT('Ctrl Pts',(9.53161285099995,15.2,4.18995878899998));
#198829=CARTESIAN_POINT('Ctrl Pts',(9.53161285099995,11.6,4.18995878899998));
#198830=CARTESIAN_POINT('Ctrl Pts',(9.53045072299994,15.2,4.18960650399999));
#198831=CARTESIAN_POINT('Ctrl Pts',(9.53045072299994,11.6,4.18960650399998));
#198832=CARTESIAN_POINT('Ctrl Pts',(9.52929735299995,15.2,4.18925564399999));
#198833=CARTESIAN_POINT('Ctrl Pts',(9.52929735299995,11.6,4.18925564399998));
#198834=CARTESIAN_POINT('Ctrl Pts',(9.52815275799994,15.2,4.18890623099998));
#198835=CARTESIAN_POINT('Ctrl Pts',(9.52815275799994,11.6,4.18890623099998));
#198836=CARTESIAN_POINT('Ctrl Pts',(9.52701695699995,15.2,4.18855828699999));
#198837=CARTESIAN_POINT('Ctrl Pts',(9.52701695699995,11.6,4.18855828699999));
#198838=CARTESIAN_POINT('Ctrl Pts',(9.52588996599994,15.2,4.18821183699999));
#198839=CARTESIAN_POINT('Ctrl Pts',(9.52588996599994,11.6,4.18821183699999));
#198840=CARTESIAN_POINT('Ctrl Pts',(9.52477180299995,15.2,4.18786690099999));
#198841=CARTESIAN_POINT('Ctrl Pts',(9.52477180299995,11.6,4.18786690099999));
#198842=CARTESIAN_POINT('Ctrl Pts',(9.52366248699994,15.2,4.18752350299999));
#198843=CARTESIAN_POINT('Ctrl Pts',(9.52366248699994,11.6,4.18752350299999));
#198844=CARTESIAN_POINT('Ctrl Pts',(9.52256203499994,15.2,4.18718166499998));
#198845=CARTESIAN_POINT('Ctrl Pts',(9.52256203499994,11.6,4.18718166499998));
#198846=CARTESIAN_POINT('Ctrl Pts',(9.52147046599995,15.2,4.18684140999999));
#198847=CARTESIAN_POINT('Ctrl Pts',(9.52147046599995,11.6,4.18684140999999));
#198848=CARTESIAN_POINT('Ctrl Pts',(9.52038779599994,15.2,4.18650276199998));
#198849=CARTESIAN_POINT('Ctrl Pts',(9.52038779599994,11.6,4.18650276199998));
#198850=CARTESIAN_POINT('Ctrl Pts',(9.51931404499994,15.2,4.18616574199999));
#198851=CARTESIAN_POINT('Ctrl Pts',(9.51931404499994,11.6,4.18616574199999));
#198852=CARTESIAN_POINT('Ctrl Pts',(9.51824922999995,15.2,4.18583037599999));
#198853=CARTESIAN_POINT('Ctrl Pts',(9.51824922999995,11.6,4.18583037599999));
#198854=CARTESIAN_POINT('Ctrl Pts',(9.51719337099994,15.2,4.18549668499999));
#198855=CARTESIAN_POINT('Ctrl Pts',(9.51719337099994,11.6,4.18549668499998));
#198856=CARTESIAN_POINT('Ctrl Pts',(9.51614648399995,15.2,4.18516469399999));
#198857=CARTESIAN_POINT('Ctrl Pts',(9.51614648399995,11.6,4.18516469399999));
#198858=CARTESIAN_POINT('Ctrl Pts',(9.51510858899995,15.2,4.18483442699999));
#198859=CARTESIAN_POINT('Ctrl Pts',(9.51510858899995,11.6,4.18483442699999));
#198860=CARTESIAN_POINT('Ctrl Pts',(9.51407970499995,15.2,4.18450590599999));
#198861=CARTESIAN_POINT('Ctrl Pts',(9.51407970499995,11.6,4.18450590599999));
#198862=CARTESIAN_POINT('Ctrl Pts',(9.51305984899994,15.2,4.18417915699998));
#198863=CARTESIAN_POINT('Ctrl Pts',(9.51305984899994,11.6,4.18417915699998));
#198864=CARTESIAN_POINT('Ctrl Pts',(9.51204903999994,15.2,4.18385420099998));
#198865=CARTESIAN_POINT('Ctrl Pts',(9.51204903999994,11.6,4.18385420099998));
#198866=CARTESIAN_POINT('Ctrl Pts',(9.51104729599994,15.2,4.18353106499998));
#198867=CARTESIAN_POINT('Ctrl Pts',(9.51104729599994,11.6,4.18353106499998));
#198868=CARTESIAN_POINT('Ctrl Pts',(9.51005463899994,15.2,4.18320977199999));
#198869=CARTESIAN_POINT('Ctrl Pts',(9.51005463899994,11.6,4.18320977199999));
#198870=CARTESIAN_POINT('Ctrl Pts',(9.50907108499995,15.2,4.18289034599999));
#198871=CARTESIAN_POINT('Ctrl Pts',(9.50907108499995,11.6,4.18289034599999));
#198872=CARTESIAN_POINT('Ctrl Pts',(9.50809665399994,15.2,4.18257281199998));
#198873=CARTESIAN_POINT('Ctrl Pts',(9.50809665399994,11.6,4.18257281199998));
#198874=CARTESIAN_POINT('Ctrl Pts',(9.50713136399994,15.2,4.18225719599998));
#198875=CARTESIAN_POINT('Ctrl Pts',(9.50713136399994,11.6,4.18225719599998));
#198876=CARTESIAN_POINT('Ctrl Pts',(9.50617523599995,15.2,4.18194351999999));
#198877=CARTESIAN_POINT('Ctrl Pts',(9.50617523599995,11.6,4.18194351999999));
#198878=CARTESIAN_POINT('Ctrl Pts',(9.50522828699994,15.2,4.18163180999999));
#198879=CARTESIAN_POINT('Ctrl Pts',(9.50522828699994,11.6,4.18163180999999));
#198880=CARTESIAN_POINT('Ctrl Pts',(9.50429053899994,15.2,4.18132209199998));
#198881=CARTESIAN_POINT('Ctrl Pts',(9.50429053899994,11.6,4.18132209199998));
#198882=CARTESIAN_POINT('Ctrl Pts',(9.50336200799994,15.2,4.18101438999999));
#198883=CARTESIAN_POINT('Ctrl Pts',(9.50336200799994,11.6,4.18101438999999));
#198884=CARTESIAN_POINT('Ctrl Pts',(9.50244271599994,15.2,4.18070872899998));
#198885=CARTESIAN_POINT('Ctrl Pts',(9.50244271599994,11.6,4.18070872899998));
#198886=CARTESIAN_POINT('Ctrl Pts',(9.50153268199994,15.2,4.18040513599998));
#198887=CARTESIAN_POINT('Ctrl Pts',(9.50153268199994,11.6,4.18040513599998));
#198888=CARTESIAN_POINT('Ctrl Pts',(9.50063192599995,15.2,4.18010363499998));
#198889=CARTESIAN_POINT('Ctrl Pts',(9.50063192599995,11.6,4.18010363499998));
#198890=CARTESIAN_POINT('Ctrl Pts',(9.49974046599994,15.2,4.17980425199998));
#198891=CARTESIAN_POINT('Ctrl Pts',(9.49974046599994,11.6,4.17980425199998));
#198892=CARTESIAN_POINT('Ctrl Pts',(9.49885832399995,15.2,4.17950701299999));
#198893=CARTESIAN_POINT('Ctrl Pts',(9.49885832399995,11.6,4.17950701299999));
#198894=CARTESIAN_POINT('Ctrl Pts',(9.49799054499995,15.2,4.17921364399999));
#198895=CARTESIAN_POINT('Ctrl Pts',(9.49799054499995,11.6,4.17921364399999));
#198896=CARTESIAN_POINT('Ctrl Pts',(9.49730470599994,15.2,4.17898101999998));
#198897=CARTESIAN_POINT('Ctrl Pts',(9.49730470599994,11.6,4.17898101999998));
#198898=CARTESIAN_POINT('Ctrl Pts',(9.49679570899994,15.2,4.17880795499999));
#198899=CARTESIAN_POINT('Ctrl Pts',(9.49679570899994,11.6,4.17880795499998));
#198900=CARTESIAN_POINT('Ctrl Pts',(9.49645984599995,15.2,4.17869357199999));
#198901=CARTESIAN_POINT('Ctrl Pts',(9.49645984599995,11.6,4.17869357199999));
#198902=CARTESIAN_POINT('Ctrl Pts',(9.49629481099995,15.2,4.17863732199999));
#198903=CARTESIAN_POINT('Ctrl Pts',(9.49629481099995,11.6,4.17863732199999));
#198904=CARTESIAN_POINT('',(9.49629481052083,12.2,4.17863732208252));
#198905=CARTESIAN_POINT('',(9.49629481052083,15.2,4.17863732208252));
#198906=CARTESIAN_POINT('',(9.49629481099995,12.2,4.17863732199999));
#198907=CARTESIAN_POINT('Ctrl Pts',(10.6761442619999,12.2,4.27433546899999));
#198908=CARTESIAN_POINT('Ctrl Pts',(10.669789618948,12.2,4.27479929410106));
#198909=CARTESIAN_POINT('Ctrl Pts',(10.663452445214,12.2,4.27524981568719));
#198910=CARTESIAN_POINT('Ctrl Pts',(10.6571327390048,12.2,4.27568705180026));
#198911=CARTESIAN_POINT('Ctrl Pts',(10.653340915417,12.2,4.27594939345856));
#198912=CARTESIAN_POINT('Ctrl Pts',(10.6495553832665,12.2,4.27620695229114));
#198913=CARTESIAN_POINT('Ctrl Pts',(10.6457761750117,12.2,4.27645974928312));
#198914=CARTESIAN_POINT('Ctrl Pts',(10.6419969667568,12.2,4.2767125462751));
#198915=CARTESIAN_POINT('Ctrl Pts',(10.6382240820909,12.2,4.27696058213185));
#198916=CARTESIAN_POINT('Ctrl Pts',(10.6344575619356,12.2,4.27720388420675));
#198917=CARTESIAN_POINT('Ctrl Pts',(10.6306910417802,12.2,4.27744718628166));
#198918=CARTESIAN_POINT('Ctrl Pts',(10.6269308868494,12.2,4.27768575655688));
#198919=CARTESIAN_POINT('Ctrl Pts',(10.6231771321099,12.2,4.2779196179657));
#198920=CARTESIAN_POINT('Ctrl Pts',(10.618172125336,12.2,4.27823143320577));
#198921=CARTESIAN_POINT('Ctrl Pts',(10.6131784967851,12.2,4.27853487774393));
#198922=CARTESIAN_POINT('Ctrl Pts',(10.6081963167132,12.2,4.27883000098355));
#198923=CARTESIAN_POINT('Ctrl Pts',(10.6032141373201,12.2,4.27912512418296));
#198924=CARTESIAN_POINT('Ctrl Pts',(10.5982434084704,12.2,4.27941192655973));
#198925=CARTESIAN_POINT('Ctrl Pts',(10.5932842098191,12.2,4.27969046520447));
#198926=CARTESIAN_POINT('Ctrl Pts',(10.589564809986,12.2,4.27989936923547));
#198927=CARTESIAN_POINT('Ctrl Pts',(10.5858518970797,12.2,4.28010362534848));
#198928=CARTESIAN_POINT('Ctrl Pts',(10.5821455051669,12.2,4.28030325729353));
#198929=CARTESIAN_POINT('Ctrl Pts',(10.5784391139275,12.2,4.28050288920232));
#198930=CARTESIAN_POINT('Ctrl Pts',(10.574739243646,12.2,4.28069789641135));
#198931=CARTESIAN_POINT('Ctrl Pts',(10.5710459278641,12.2,4.28088830427903));
#198932=CARTESIAN_POINT('Ctrl Pts',(10.5661215070452,12.2,4.28114218142441));
#198933=CARTESIAN_POINT('Ctrl Pts',(10.5612087375452,12.2,4.28138787960012));
#198934=CARTESIAN_POINT('Ctrl Pts',(10.5563077004778,12.2,4.28162545748217));
#198935=CARTESIAN_POINT('Ctrl Pts',(10.5501814036427,12.2,4.28192242985899));
#198936=CARTESIAN_POINT('Ctrl Pts',(10.544073437927,12.2,4.28220671058151));
#198937=CARTESIAN_POINT('Ctrl Pts',(10.5379839638983,12.2,4.28247841870717));
#198938=CARTESIAN_POINT('Ctrl Pts',(10.5343302796138,12.2,4.28264144357664));
#198939=CARTESIAN_POINT('Ctrl Pts',(10.5306832517455,12.2,4.28279994107142));
#198940=CARTESIAN_POINT('Ctrl Pts',(10.5270429150435,12.2,4.28295393648311));
#198941=CARTESIAN_POINT('Ctrl Pts',(10.5234025776802,12.2,4.28310793192277));
#198942=CARTESIAN_POINT('Ctrl Pts',(10.5197689319688,12.2,4.28325742446116));
#198943=CARTESIAN_POINT('Ctrl Pts',(10.5161420101926,12.2,4.28340244002329));
#198944=CARTESIAN_POINT('Ctrl Pts',(10.5113061155891,12.2,4.28359579406223));
#198945=CARTESIAN_POINT('Ctrl Pts',(10.5064821785289,12.2,4.28378118984135));
#198946=CARTESIAN_POINT('Ctrl Pts',(10.5016702785115,12.2,4.28395868571656));
#198947=CARTESIAN_POINT('Ctrl Pts',(10.4980613533346,12.2,4.28409180762901));
#198948=CARTESIAN_POINT('Ctrl Pts',(10.4944592003619,12.2,4.28422048582386));
#198949=CARTESIAN_POINT('Ctrl Pts',(10.4908638536586,12.2,4.2843447467364));
#198950=CARTESIAN_POINT('Ctrl Pts',(10.4860700576187,12.2,4.28451042796816));
#198951=CARTESIAN_POINT('Ctrl Pts',(10.4812883603415,12.2,4.28466825377954));
#198952=CARTESIAN_POINT('Ctrl Pts',(10.4765188468601,12.2,4.28481828828721));
#198953=CARTESIAN_POINT('Ctrl Pts',(10.472941712074,12.2,4.28493081415774));
#198954=CARTESIAN_POINT('Ctrl Pts',(10.4693714304371,12.2,4.28503895580379));
#198955=CARTESIAN_POINT('Ctrl Pts',(10.4658080357749,12.2,4.28514274075835));
#198956=CARTESIAN_POINT('Ctrl Pts',(10.4622446411127,12.2,4.28524652571291));
#198957=CARTESIAN_POINT('Ctrl Pts',(10.4586881348419,12.2,4.28534595299265));
#198958=CARTESIAN_POINT('Ctrl Pts',(10.4551385511369,12.2,4.28544104944791));
#198959=CARTESIAN_POINT('Ctrl Pts',(10.4515889674319,12.2,4.28553614590316));
#198960=CARTESIAN_POINT('Ctrl Pts',(10.4480463063163,12.2,4.28562691108157));
#198961=CARTESIAN_POINT('Ctrl Pts',(10.444510603434,12.2,4.28571337249991));
#198962=CARTESIAN_POINT('Ctrl Pts',(10.4409749005517,12.2,4.28579983391826));
#198963=CARTESIAN_POINT('Ctrl Pts',(10.4374461564073,12.2,4.28588199021861));
#198964=CARTESIAN_POINT('Ctrl Pts',(10.4339244052843,12.2,4.28595986921637));
#198965=CARTESIAN_POINT('Ctrl Pts',(10.4304026535215,12.2,4.28603774822827));
#198966=CARTESIAN_POINT('Ctrl Pts',(10.426887896494,12.2,4.2861113499723));
#198967=CARTESIAN_POINT('Ctrl Pts',(10.4233801677352,12.2,4.28618070052346));
#198968=CARTESIAN_POINT('Ctrl Pts',(10.4198724396136,12.2,4.28625005106203));
#198969=CARTESIAN_POINT('Ctrl Pts',(10.4163717412417,12.2,4.28631515095916));
#198970=CARTESIAN_POINT('Ctrl Pts',(10.4128781071192,12.2,4.28637602745658));
#198971=CARTESIAN_POINT('Ctrl Pts',(10.4082199285008,12.2,4.28645719611612));
#198972=CARTESIAN_POINT('Ctrl Pts',(10.4035743106399,12.2,4.2865308568446));
#198973=CARTESIAN_POINT('Ctrl Pts',(10.3989413357306,12.2,4.28659707423203));
#198974=CARTESIAN_POINT('Ctrl Pts',(10.3954666043907,12.2,4.28664673727486));
#198975=CARTESIAN_POINT('Ctrl Pts',(10.3919989861295,12.2,4.28669221344194));
#198976=CARTESIAN_POINT('Ctrl Pts',(10.3885385164626,12.2,4.28673353098267));
#198977=CARTESIAN_POINT('Ctrl Pts',(10.3850780461671,12.2,4.28677484853091));
#198978=CARTESIAN_POINT('Ctrl Pts',(10.3816247245818,12.2,4.28681200815297));
#198979=CARTESIAN_POINT('Ctrl Pts',(10.3781785877486,12.2,4.28684503528221));
#198980=CARTESIAN_POINT('Ctrl Pts',(10.3735837396811,12.2,4.28688907144452));
#198981=CARTESIAN_POINT('Ctrl Pts',(10.3690016642314,12.2,4.28692576481891));
#198982=CARTESIAN_POINT('Ctrl Pts',(10.3644324468819,12.2,4.28695518153921));
#198983=CARTESIAN_POINT('Ctrl Pts',(10.3610055337141,12.2,4.28697724408043));
#198984=CARTESIAN_POINT('Ctrl Pts',(10.3575858539909,12.2,4.28699521367995));
#198985=CARTESIAN_POINT('Ctrl Pts',(10.3541734436102,12.2,4.28700911872228));
#198986=CARTESIAN_POINT('Ctrl Pts',(10.3507610332295,12.2,4.28702302376461));
#198987=CARTESIAN_POINT('Ctrl Pts',(10.3473558927515,12.2,4.28703286423174));
#198988=CARTESIAN_POINT('Ctrl Pts',(10.3439580580406,12.2,4.28703866927374));
#198989=CARTESIAN_POINT('Ctrl Pts',(10.3405602227125,12.2,4.2870444743168));
#198990=CARTESIAN_POINT('Ctrl Pts',(10.3371696935364,12.2,4.2870462436504));
#198991=CARTESIAN_POINT('Ctrl Pts',(10.3337865067957,12.2,4.28704400669119));
#198992=CARTESIAN_POINT('Ctrl Pts',(10.3304033206696,12.2,4.28704176973239));
#198993=CARTESIAN_POINT('Ctrl Pts',(10.3270274775098,12.2,4.28703552628214));
#198994=CARTESIAN_POINT('Ctrl Pts',(10.3236590138412,12.2,4.2870253062405));
#198995=CARTESIAN_POINT('Ctrl Pts',(10.3202905501726,12.2,4.28701508619885));
#198996=CARTESIAN_POINT('Ctrl Pts',(10.3169294662402,12.2,4.28700088816611));
#198997=CARTESIAN_POINT('Ctrl Pts',(10.3135757990135,12.2,4.28698274325));
#198998=CARTESIAN_POINT('Ctrl Pts',(10.3102221317868,12.2,4.28696459833389));
#198999=CARTESIAN_POINT('Ctrl Pts',(10.3068758806301,12.2,4.28694250706586));
#199000=CARTESIAN_POINT('Ctrl Pts',(10.3035370834863,12.2,4.28691649723337));
#199001=CARTESIAN_POINT('Ctrl Pts',(10.2990853535567,12.2,4.28688181745357));
#199002=CARTESIAN_POINT('Ctrl Pts',(10.2946468753079,12.2,4.28684017453431));
#199003=CARTESIAN_POINT('Ctrl Pts',(10.2902217365681,12.2,4.28679163797541));
#199004=CARTESIAN_POINT('Ctrl Pts',(10.2857965984312,12.2,4.28674310142312));
#199005=CARTESIAN_POINT('Ctrl Pts',(10.2813847995981,12.2,4.28668767290783));
#199006=CARTESIAN_POINT('Ctrl Pts',(10.2769864295679,12.2,4.2866254237467));
#199007=CARTESIAN_POINT('Ctrl Pts',(10.269289281266,12.2,4.28651648770412));
#199008=CARTESIAN_POINT('Ctrl Pts',(10.2616332568613,12.2,4.28638666492381));
#199009=CARTESIAN_POINT('Ctrl Pts',(10.254018838161,12.2,4.28623635051793));
#199010=CARTESIAN_POINT('Ctrl Pts',(10.2496677421842,12.2,4.28615045658007));
#199011=CARTESIAN_POINT('Ctrl Pts',(10.2453302314825,12.2,4.28605787097967));
#199012=CARTESIAN_POINT('Ctrl Pts',(10.2410063967235,12.2,4.28595866909956));
#199013=CARTESIAN_POINT('Ctrl Pts',(10.2366825613754,12.2,4.28585946720594));
#199014=CARTESIAN_POINT('Ctrl Pts',(10.2323724014811,12.2,4.28575365020103));
#199015=CARTESIAN_POINT('Ctrl Pts',(10.228076008172,12.2,4.28564129174993));
#199016=CARTESIAN_POINT('Ctrl Pts',(10.2237796154482,12.2,4.28552893331414));
#199017=CARTESIAN_POINT('Ctrl Pts',(10.2194969886475,12.2,4.28541003485126));
#199018=CARTESIAN_POINT('Ctrl Pts',(10.2152282199395,12.2,4.28528467302884));
#199019=CARTESIAN_POINT('Ctrl Pts',(10.2109594506499,12.2,4.28515931118933));
#199020=CARTESIAN_POINT('Ctrl Pts',(10.2067045403671,12.2,4.28502748609921));
#199021=CARTESIAN_POINT('Ctrl Pts',(10.2024635785249,12.2,4.28488927425835));
#199022=CARTESIAN_POINT('Ctrl Pts',(10.197162376511,12.2,4.28471650946668));
#199023=CARTESIAN_POINT('Ctrl Pts',(10.1918829712708,12.2,4.28453376720081));
#199024=CARTESIAN_POINT('Ctrl Pts',(10.186625542497,12.2,4.28434120074157));
#199025=CARTESIAN_POINT('Ctrl Pts',(10.1824195998218,12.2,4.28418714758678));
#199026=CARTESIAN_POINT('Ctrl Pts',(10.1782277209373,12.2,4.28402680845743));
#199027=CARTESIAN_POINT('Ctrl Pts',(10.1740500021663,12.2,4.28386026002723));
#199028=CARTESIAN_POINT('Ctrl Pts',(10.169872282826,12.2,4.28369371157435));
#199029=CARTESIAN_POINT('Ctrl Pts',(10.1657087209566,12.2,4.28352095623476));
#199030=CARTESIAN_POINT('Ctrl Pts',(10.1615594110082,12.2,4.28334207372501));
#199031=CARTESIAN_POINT('Ctrl Pts',(10.1574101010599,12.2,4.28316319121526));
#199032=CARTESIAN_POINT('Ctrl Pts',(10.1532750420465,12.2,4.2829781817909));
#199033=CARTESIAN_POINT('Ctrl Pts',(10.1491543301012,12.2,4.2827871280021));
#199034=CARTESIAN_POINT('Ctrl Pts',(10.141943085039,12.2,4.28245278391074));
#199035=CARTESIAN_POINT('Ctrl Pts',(10.1347757714352,12.2,4.28209992515461));
#199036=CARTESIAN_POINT('Ctrl Pts',(10.1276529035994,12.2,4.28172900023395));
#199037=CARTESIAN_POINT('Ctrl Pts',(10.1235826929322,12.2,4.28151704311167));
#199038=CARTESIAN_POINT('Ctrl Pts',(10.1195269927751,12.2,4.28129918610534));
#199039=CARTESIAN_POINT('Ctrl Pts',(10.1154859009447,12.2,4.28107551498167));
#199040=CARTESIAN_POINT('Ctrl Pts',(10.1114448096649,12.2,4.28085184388846));
#199041=CARTESIAN_POINT('Ctrl Pts',(10.1074183267127,12.2,4.28062235856309));
#199042=CARTESIAN_POINT('Ctrl Pts',(10.1034065473725,12.2,4.2803871434718));
#199043=CARTESIAN_POINT('Ctrl Pts',(10.0993947674857,12.2,4.28015192834845));
#199044=CARTESIAN_POINT('Ctrl Pts',(10.0953976918489,12.2,4.27991098513108));
#199045=CARTESIAN_POINT('Ctrl Pts',(10.0914154172805,12.2,4.27966439878317));
#199046=CARTESIAN_POINT('Ctrl Pts',(10.0874331432547,12.2,4.27941781246886));
#199047=CARTESIAN_POINT('Ctrl Pts',(10.0834656691273,12.2,4.27916558377884));
#199048=CARTESIAN_POINT('Ctrl Pts',(10.0795130938378,12.2,4.27890780130049));
#199049=CARTESIAN_POINT('Ctrl Pts',(10.0755605180098,12.2,4.278650018787));
#199050=CARTESIAN_POINT('Ctrl Pts',(10.071622841097,12.2,4.27838668119244));
#199051=CARTESIAN_POINT('Ctrl Pts',(10.0677001612165,12.2,4.27811787873334));
#199052=CARTESIAN_POINT('Ctrl Pts',(10.0637774813361,12.2,4.27784907627425));
#199053=CARTESIAN_POINT('Ctrl Pts',(10.0598697974907,12.2,4.2775748079173));
#199054=CARTESIAN_POINT('Ctrl Pts',(10.0559772096135,12.2,4.27729516417928));
#199055=CARTESIAN_POINT('Ctrl Pts',(10.0520846222666,12.2,4.27701552047937));
#199056=CARTESIAN_POINT('Ctrl Pts',(10.0482071298238,12.2,4.27673050144721));
#199057=CARTESIAN_POINT('Ctrl Pts',(10.0443448325109,12.2,4.2764401985252));
#199058=CARTESIAN_POINT('Ctrl Pts',(10.0404825346717,12.2,4.27614989556363));
#199059=CARTESIAN_POINT('Ctrl Pts',(10.0366354320612,12.2,4.27585430906497));
#199060=CARTESIAN_POINT('Ctrl Pts',(10.0328036241317,12.2,4.27555352999249));
#199061=CARTESIAN_POINT('Ctrl Pts',(10.0289718167243,12.2,4.275252750961));
#199062=CARTESIAN_POINT('Ctrl Pts',(10.0251553039288,12.2,4.27494677946073));
#199063=CARTESIAN_POINT('Ctrl Pts',(10.0213541867941,12.2,4.27463571104205));
#199064=CARTESIAN_POINT('Ctrl Pts',(10.0175530691415,12.2,4.27432464258099));
#199065=CARTESIAN_POINT('Ctrl Pts',(10.0137673486648,12.2,4.27400847592347));
#199066=CARTESIAN_POINT('Ctrl Pts',(10.0099971239946,12.2,4.27368730494504));
#199067=CARTESIAN_POINT('Ctrl Pts',(10.006226899838,12.2,4.27336613401037));
#199068=CARTESIAN_POINT('Ctrl Pts',(10.0024721738705,12.2,4.27303996064964));
#199069=CARTESIAN_POINT('Ctrl Pts',(9.99873304656404,12.2,4.27270887901036));
#199070=CARTESIAN_POINT('Ctrl Pts',(9.99499391874812,12.2,4.27237779732597));
#199071=CARTESIAN_POINT('Ctrl Pts',(9.99127038951741,12.2,4.27204180815487));
#199072=CARTESIAN_POINT('Ctrl Pts',(9.98756256370525,12.2,4.2717010097471));
#199073=CARTESIAN_POINT('Ctrl Pts',(9.98385473839828,12.2,4.27136021138576));
#199074=CARTESIAN_POINT('Ctrl Pts',(9.98016261534292,12.2,4.27101460046982));
#199075=CARTESIAN_POINT('Ctrl Pts',(9.97648629729176,12.2,4.27066428009248));
#199076=CARTESIAN_POINT('Ctrl Pts',(9.9728099787397,12.2,4.2703139596674));
#199077=CARTESIAN_POINT('Ctrl Pts',(9.9691494664219,12.2,4.26995892624324));
#199078=CARTESIAN_POINT('Ctrl Pts',(9.96550486400209,12.2,4.26959928194556));
#199079=CARTESIAN_POINT('Ctrl Pts',(9.96186026207885,12.2,4.26923963769688));
#199080=CARTESIAN_POINT('Ctrl Pts',(9.9582315701302,12.2,4.26887538111024));
#199081=CARTESIAN_POINT('Ctrl Pts',(9.95461889409056,12.2,4.26850661408529));
#199082=CARTESIAN_POINT('Ctrl Pts',(9.9510062175587,12.2,4.2681378470101));
#199083=CARTESIAN_POINT('Ctrl Pts',(9.94740955575046,12.2,4.26776456899428));
#199084=CARTESIAN_POINT('Ctrl Pts',(9.94382901470578,12.2,4.26738688274974));
#199085=CARTESIAN_POINT('Ctrl Pts',(9.94024847414895,12.2,4.26700919655667));
#199086=CARTESIAN_POINT('Ctrl Pts',(9.93668405516105,12.2,4.26662710246726));
#199087=CARTESIAN_POINT('Ctrl Pts',(9.93313586383835,12.2,4.26624070355484));
#199088=CARTESIAN_POINT('Ctrl Pts',(9.92958767203221,12.2,4.26585430458978));
#199089=CARTESIAN_POINT('Ctrl Pts',(9.92605570773315,12.2,4.26546360055764));
#199090=CARTESIAN_POINT('Ctrl Pts',(9.92254007804154,12.2,4.26506869825834));
#199091=CARTESIAN_POINT('Ctrl Pts',(9.91902444834994,12.2,4.26467379595904));
#199092=CARTESIAN_POINT('Ctrl Pts',(9.91552515345747,12.2,4.26427469383147));
#199093=CARTESIAN_POINT('Ctrl Pts',(9.91204230238044,12.2,4.26387149897574));
#199094=CARTESIAN_POINT('Ctrl Pts',(9.90855945177796,12.2,4.26346830417495));
#199095=CARTESIAN_POINT('Ctrl Pts',(9.90509304365537,12.2,4.26306101685463));
#199096=CARTESIAN_POINT('Ctrl Pts',(9.90164318897723,12.2,4.26264974527528));
#199097=CARTESIAN_POINT('Ctrl Pts',(9.89819333382905,12.2,4.2622384736399));
#199098=CARTESIAN_POINT('Ctrl Pts',(9.89476003118688,12.2,4.26182321604915));
#199099=CARTESIAN_POINT('Ctrl Pts',(9.8913433902246,12.2,4.2614040839148));
#199100=CARTESIAN_POINT('Ctrl Pts',(9.88792674972784,12.2,4.26098495183756));
#199101=CARTESIAN_POINT('Ctrl Pts',(9.88452677105669,12.2,4.26056194624416));
#199102=CARTESIAN_POINT('Ctrl Pts',(9.88114356577661,12.2,4.26013517483485));
#199103=CARTESIAN_POINT('Ctrl Pts',(9.87776036003559,12.2,4.2597084033674));
#199104=CARTESIAN_POINT('Ctrl Pts',(9.87439392829569,12.2,4.2592778680021));
#199105=CARTESIAN_POINT('Ctrl Pts',(9.87104437928059,12.2,4.25884368167864));
#199106=CARTESIAN_POINT('Ctrl Pts',(9.86769483072188,12.2,4.25840949541435));
#199107=CARTESIAN_POINT('Ctrl Pts',(9.86436216789282,12.2,4.25797165675806));
#199108=CARTESIAN_POINT('Ctrl Pts',(9.86104650199609,12.2,4.25753028129438));
#199109=CARTESIAN_POINT('Ctrl Pts',(9.85690191928636,12.2,4.25697856191967));
#199110=CARTESIAN_POINT('Ctrl Pts',(9.85278389494122,12.2,4.25642131443093));
#199111=CARTESIAN_POINT('Ctrl Pts',(9.84869264980094,12.2,4.25585876602842));
#199112=CARTESIAN_POINT('Ctrl Pts',(9.84460140466066,12.2,4.25529621762592));
#199113=CARTESIAN_POINT('Ctrl Pts',(9.84053693832048,12.2,4.25472836873623));
#199114=CARTESIAN_POINT('Ctrl Pts',(9.83649947726041,12.2,4.25415544852531));
#199115=CARTESIAN_POINT('Ctrl Pts',(9.83246201620035,12.2,4.25358252831439));
#199116=CARTESIAN_POINT('Ctrl Pts',(9.82845155932765,12.2,4.25300453780555));
#199117=CARTESIAN_POINT('Ctrl Pts',(9.8244683317582,12.2,4.25242170954166));
#199118=CARTESIAN_POINT('Ctrl Pts',(9.82048510418876,12.2,4.25183888127778));
#199119=CARTESIAN_POINT('Ctrl Pts',(9.81652910786098,12.2,4.25125121828333));
#199120=CARTESIAN_POINT('Ctrl Pts',(9.81260057029154,12.2,4.25065895578333));
#199121=CARTESIAN_POINT('Ctrl Pts',(9.8086720327221,12.2,4.25006669328333));
#199122=CARTESIAN_POINT('Ctrl Pts',(9.80477095437084,12.2,4.24946983258574));
#199123=CARTESIAN_POINT('Ctrl Pts',(9.80089756671443,12.2,4.24886861674967));
#199124=CARTESIAN_POINT('Ctrl Pts',(9.79702417905803,12.2,4.24826740091359));
#199125=CARTESIAN_POINT('Ctrl Pts',(9.79317848250446,12.2,4.24766182984364));
#199126=CARTESIAN_POINT('Ctrl Pts',(9.78936070924203,12.2,4.24705215067676));
#199127=CARTESIAN_POINT('Ctrl Pts',(9.78554293597961,12.2,4.24644247150988));
#199128=CARTESIAN_POINT('Ctrl Pts',(9.78175308901367,12.2,4.24582868342644));
#199129=CARTESIAN_POINT('Ctrl Pts',(9.77799140227903,12.2,4.24521103925958));
#199130=CARTESIAN_POINT('Ctrl Pts',(9.77422971554439,12.2,4.24459339509271));
#199131=CARTESIAN_POINT('Ctrl Pts',(9.77049618983077,12.2,4.2439718940089));
#199132=CARTESIAN_POINT('Ctrl Pts',(9.7667910645782,12.2,4.24334679314408));
#199133=CARTESIAN_POINT('Ctrl Pts',(9.76234491443666,12.2,4.24259667213356));
#199134=CARTESIAN_POINT('Ctrl Pts',(9.75793966089131,12.2,4.24184136578905));
#199135=CARTESIAN_POINT('Ctrl Pts',(9.75357572304987,12.2,4.24108132598333));
#199136=CARTESIAN_POINT('Ctrl Pts',(9.74993910804987,12.2,4.24044795945555));
#199137=CARTESIAN_POINT('Ctrl Pts',(9.74633118422521,12.2,4.23981130718033));
#199138=CARTESIAN_POINT('Ctrl Pts',(9.74275219601459,12.2,4.23917163398298));
#199139=CARTESIAN_POINT('Ctrl Pts',(9.73917320780397,12.2,4.23853196078562));
#199140=CARTESIAN_POINT('Ctrl Pts',(9.7356231577738,12.2,4.23788926851346));
#199141=CARTESIAN_POINT('Ctrl Pts',(9.73210229201145,12.2,4.23724382774943));
#199142=CARTESIAN_POINT('Ctrl Pts',(9.72858142624908,12.2,4.2365983869854));
#199143=CARTESIAN_POINT('Ctrl Pts',(9.7250897465721,12.2,4.23595019926311));
#199144=CARTESIAN_POINT('Ctrl Pts',(9.72162750324028,12.2,4.23529953870742));
#199145=CARTESIAN_POINT('Ctrl Pts',(9.71816525990848,12.2,4.23464887815174));
#199146=CARTESIAN_POINT('Ctrl Pts',(9.71473245426177,12.2,4.23399574767347));
#199147=CARTESIAN_POINT('Ctrl Pts',(9.71132933832993,12.2,4.23334042722391));
#199148=CARTESIAN_POINT('Ctrl Pts',(9.70792622239808,12.2,4.23268510677435));
#199149=CARTESIAN_POINT('Ctrl Pts',(9.70455279944898,12.2,4.23202759820278));
#199150=CARTESIAN_POINT('Ctrl Pts',(9.70120932535422,12.2,4.2313681884804));
#199151=CARTESIAN_POINT('Ctrl Pts',(9.69786585125945,12.2,4.23070877875803));
#199152=CARTESIAN_POINT('Ctrl Pts',(9.69455232774573,12.2,4.23004746754675));
#199153=CARTESIAN_POINT('Ctrl Pts',(9.69126901309542,12.2,4.22938454942161));
#199154=CARTESIAN_POINT('Ctrl Pts',(9.68732903565819,12.2,4.22858904770036));
#199155=CARTESIAN_POINT('Ctrl Pts',(9.68343256301487,12.2,4.2277912288941));
#199156=CARTESIAN_POINT('Ctrl Pts',(9.67958005132343,12.2,4.22699161342307));
#199157=CARTESIAN_POINT('Ctrl Pts',(9.675727539632,12.2,4.22619199795204));
#199158=CARTESIAN_POINT('Ctrl Pts',(9.67191898892038,12.2,4.22539058576451));
#199159=CARTESIAN_POINT('Ctrl Pts',(9.66815486522187,12.2,4.22458790529373));
#199160=CARTESIAN_POINT('Ctrl Pts',(9.66439074152335,12.2,4.22378522482295));
#199161=CARTESIAN_POINT('Ctrl Pts',(9.66067104486998,12.2,4.22298127845007));
#199162=CARTESIAN_POINT('Ctrl Pts',(9.6569962481671,12.2,4.22217660706269));
#199163=CARTESIAN_POINT('Ctrl Pts',(9.65270898512455,12.2,4.22123782372868));
#199164=CARTESIAN_POINT('Ctrl Pts',(9.64848283695619,12.2,4.22029805452518));
#199165=CARTESIAN_POINT('Ctrl Pts',(9.64431856644459,12.2,4.21935818405222));
#199166=CARTESIAN_POINT('Ctrl Pts',(9.64074919190563,12.2,4.21855258083149));
#199167=CARTESIAN_POINT('Ctrl Pts',(9.63722528164741,12.2,4.21774690523353));
#199168=CARTESIAN_POINT('Ctrl Pts',(9.63374732235397,12.2,4.21694172884608));
#199169=CARTESIAN_POINT('Ctrl Pts',(9.63026936274461,12.2,4.2161365523855));
#199170=CARTESIAN_POINT('Ctrl Pts',(9.62683736008971,12.2,4.21533187427494));
#199171=CARTESIAN_POINT('Ctrl Pts',(9.62345180832388,12.2,4.21452828298119));
#199172=CARTESIAN_POINT('Ctrl Pts',(9.62006625686557,12.2,4.21372469176044));
#199173=CARTESIAN_POINT('Ctrl Pts',(9.61672715953014,12.2,4.21292218593322));
#199174=CARTESIAN_POINT('Ctrl Pts',(9.61343502396803,12.2,4.21212136970868));
#199175=CARTESIAN_POINT('Ctrl Pts',(9.61014288840592,12.2,4.21132055348413));
#199176=CARTESIAN_POINT('Ctrl Pts',(9.60689771447714,12.2,4.21052142524137));
#199177=CARTESIAN_POINT('Ctrl Pts',(9.60370002284009,12.2,4.2097246041035));
#199178=CARTESIAN_POINT('Ctrl Pts',(9.60050233091258,12.2,4.20892778289326));
#199179=CARTESIAN_POINT('Ctrl Pts',(9.59735211823965,12.2,4.20813326764152));
#199180=CARTESIAN_POINT('Ctrl Pts',(9.59424991632266,12.2,4.20734169168185));
#199181=CARTESIAN_POINT('Ctrl Pts',(9.59063068117553,12.2,4.20641818650342));
#199182=CARTESIAN_POINT('Ctrl Pts',(9.58707678942903,12.2,4.20549868427875));
#199183=CARTESIAN_POINT('Ctrl Pts',(9.58358910205906,12.2,4.20458421833542));
#199184=CARTESIAN_POINT('Ctrl Pts',(9.58059965539281,12.2,4.20380039029244));
#199185=CARTESIAN_POINT('Ctrl Pts',(9.57765884608958,12.2,4.2030202627748));
#199186=CARTESIAN_POINT('Ctrl Pts',(9.57476722835081,12.2,4.20224450798272));
#199187=CARTESIAN_POINT('Ctrl Pts',(9.57187561087468,12.2,4.20146875326109));
#199188=CARTESIAN_POINT('Ctrl Pts',(9.56903318226246,12.2,4.20069737255097));
#199189=CARTESIAN_POINT('Ctrl Pts',(9.5662405070178,12.2,4.19993105199199));
#199190=CARTESIAN_POINT('Ctrl Pts',(9.56298238572992,12.2,4.19903701129344));
#199191=CARTESIAN_POINT('Ctrl Pts',(9.55979198352252,12.2,4.19814986238899));
#199192=CARTESIAN_POINT('Ctrl Pts',(9.55667021408757,12.2,4.19727072945893));
#199193=CARTESIAN_POINT('Ctrl Pts',(9.55399441185365,12.2,4.19651718698656));
#199194=CARTESIAN_POINT('Ctrl Pts',(9.5513690348193,12.2,4.19576953700177));
#199195=CARTESIAN_POINT('Ctrl Pts',(9.54879467073436,12.2,4.19502851044198));
#199196=CARTESIAN_POINT('Ctrl Pts',(9.54622030664942,12.2,4.19428748388219));
#199197=CARTESIAN_POINT('Ctrl Pts',(9.54369695648298,12.2,4.19355308067831));
#199198=CARTESIAN_POINT('Ctrl Pts',(9.54122522323595,12.2,4.19282605612088));
#199199=CARTESIAN_POINT('Ctrl Pts',(9.5387534897644,12.2,4.19209903149743));
#199200=CARTESIAN_POINT('Ctrl Pts',(9.53633337214024,12.2,4.19137938253835));
#199201=CARTESIAN_POINT('Ctrl Pts',(9.53396548681259,12.2,4.19066788713116));
#199202=CARTESIAN_POINT('Ctrl Pts',(9.53159760170003,12.2,4.18995639178861));
#199203=CARTESIAN_POINT('Ctrl Pts',(9.52928194860096,12.2,4.18925305068308));
#199204=CARTESIAN_POINT('Ctrl Pts',(9.52701915951651,12.2,4.1885586604583));
#199205=CARTESIAN_POINT('Ctrl Pts',(9.52475637043206,12.2,4.18786427023353));
#199206=CARTESIAN_POINT('Ctrl Pts',(9.52254644388275,12.2,4.18717883320012));
#199207=CARTESIAN_POINT('Ctrl Pts',(9.52039002593359,12.2,4.18650316910702));
#199208=CARTESIAN_POINT('Ctrl Pts',(9.51823360778857,12.2,4.18582750495255));
#199209=CARTESIAN_POINT('Ctrl Pts',(9.51613069890119,12.2,4.1851616150052));
#199210=CARTESIAN_POINT('Ctrl Pts',(9.51408196179321,12.2,4.18450634888688));
#199211=CARTESIAN_POINT('Ctrl Pts',(9.51203322487133,12.2,4.18385108282807));
#199212=CARTESIAN_POINT('Ctrl Pts',(9.5100386569622,12.2,4.1832064374462));
#199213=CARTESIAN_POINT('Ctrl Pts',(9.50809893927397,12.2,4.18257329146634));
#199214=CARTESIAN_POINT('Ctrl Pts',(9.50615922158575,12.2,4.18194014548649));
#199215=CARTESIAN_POINT('Ctrl Pts',(9.50427435329407,12.2,4.18131849573663));
#199216=CARTESIAN_POINT('Ctrl Pts',(9.50244503060811,12.2,4.18070924600822));
#199217=CARTESIAN_POINT('Ctrl Pts',(9.50031960011077,12.2,4.18000137857554));
#199218=CARTESIAN_POINT('Ctrl Pts',(9.49826915599089,12.2,4.17931025141339));
#199219=CARTESIAN_POINT('Ctrl Pts',(9.49629481099995,12.2,4.17863732199999));
#199220=CARTESIAN_POINT('Ctrl Pts',(9.49629481099995,15.2,4.17863732199999));
#199221=CARTESIAN_POINT('Ctrl Pts',(9.49798594157082,15.2,4.17921372151895));
#199222=CARTESIAN_POINT('Ctrl Pts',(9.49973290497691,15.2,4.17980347312964));
#199223=CARTESIAN_POINT('Ctrl Pts',(9.50153500128582,15.2,4.18040565895068));
#199224=CARTESIAN_POINT('Ctrl Pts',(9.50334578821404,15.2,4.18101074881613));
#199225=CARTESIAN_POINT('Ctrl Pts',(9.50521223961529,15.2,4.1816283930278));
#199226=CARTESIAN_POINT('Ctrl Pts',(9.50713365465252,15.2,4.1822576810942));
#199227=CARTESIAN_POINT('Ctrl Pts',(9.50905506951522,15.2,4.18288696910345));
#199228=CARTESIAN_POINT('Ctrl Pts',(9.51103144889862,15.2,4.18352790432364));
#199229=CARTESIAN_POINT('Ctrl Pts',(9.51306211074151,15.2,4.18417960529996));
#199230=CARTESIAN_POINT('Ctrl Pts',(9.5150927725844,15.2,4.18483130627629));
#199231=CARTESIAN_POINT('Ctrl Pts',(9.51717771587541,15.2,4.18549377330137));
#199232=CARTESIAN_POINT('Ctrl Pts',(9.5193162788181,15.2,4.18616615539328));
#199233=CARTESIAN_POINT('Ctrl Pts',(9.52145484195506,15.2,4.18683853754627));
#199234=CARTESIAN_POINT('Ctrl Pts',(9.52364702221027,15.2,4.18752083323704));
#199235=CARTESIAN_POINT('Ctrl Pts',(9.52589217325292,15.2,4.18821221560867));
#199236=CARTESIAN_POINT('Ctrl Pts',(9.5285115158301,15.2,4.18901882828137));
#199237=CARTESIAN_POINT('Ctrl Pts',(9.53120295425296,15.2,4.18983780925306));
#199238=CARTESIAN_POINT('Ctrl Pts',(9.53396548681259,15.2,4.19066788713116));
#199239=CARTESIAN_POINT('Ctrl Pts',(9.53633337214024,15.2,4.19137938253835));
#199240=CARTESIAN_POINT('Ctrl Pts',(9.53875348976439,15.2,4.19209903149742));
#199241=CARTESIAN_POINT('Ctrl Pts',(9.54122522323595,15.2,4.19282605612089));
#199242=CARTESIAN_POINT('Ctrl Pts',(9.54369695648298,15.2,4.19355308067831));
#199243=CARTESIAN_POINT('Ctrl Pts',(9.54622030664941,15.2,4.19428748388218));
#199244=CARTESIAN_POINT('Ctrl Pts',(9.54879467073436,15.2,4.19502851044198));
#199245=CARTESIAN_POINT('Ctrl Pts',(9.55136903481931,15.2,4.19576953700178));
#199246=CARTESIAN_POINT('Ctrl Pts',(9.55399441185365,15.2,4.19651718698656));
#199247=CARTESIAN_POINT('Ctrl Pts',(9.55667021408757,15.2,4.19727072945893));
#199248=CARTESIAN_POINT('Ctrl Pts',(9.55934601656456,15.2,4.19802427199975));
#199249=CARTESIAN_POINT('Ctrl Pts',(9.56207224395609,15.2,4.19878370428296));
#199250=CARTESIAN_POINT('Ctrl Pts',(9.56484831852746,15.2,4.19954831707499));
#199251=CARTESIAN_POINT('Ctrl Pts',(9.56901243000625,15.2,4.20069523615885));
#199252=CARTESIAN_POINT('Ctrl Pts',(9.57328869730923,15.2,4.20185380265907));
#199253=CARTESIAN_POINT('Ctrl Pts',(9.57767522277485,15.2,4.20302169499165));
#199254=CARTESIAN_POINT('Ctrl Pts',(9.58059957308527,15.2,4.20380028988003));
#199255=CARTESIAN_POINT('Ctrl Pts',(9.58357292771095,15.2,4.20458303238842));
#199256=CARTESIAN_POINT('Ctrl Pts',(9.58659474116599,15.2,4.20536925614893));
#199257=CARTESIAN_POINT('Ctrl Pts',(9.5896165548955,15.2,4.20615547998085));
#199258=CARTESIAN_POINT('Ctrl Pts',(9.59268682472488,15.2,4.20694518375132));
#199259=CARTESIAN_POINT('Ctrl Pts',(9.59580501631476,15.2,4.20773772187803));
#199260=CARTESIAN_POINT('Ctrl Pts',(9.59892320762139,15.2,4.20853025993276));
#199261=CARTESIAN_POINT('Ctrl Pts',(9.60208931759995,15.2,4.20932563084563));
#199262=CARTESIAN_POINT('Ctrl Pts',(9.60530282298319,15.2,4.21012320398331));
#199263=CARTESIAN_POINT('Ctrl Pts',(9.60905191279156,15.2,4.21105370602558));
#199264=CARTESIAN_POINT('Ctrl Pts',(9.61286551026422,15.2,4.21198720588282));
#199265=CARTESIAN_POINT('Ctrl Pts',(9.61674279506314,15.2,4.21292272706922));
#199266=CARTESIAN_POINT('Ctrl Pts',(9.62006618186113,15.2,4.21372460233024));
#199267=CARTESIAN_POINT('Ctrl Pts',(9.62343636180731,15.2,4.21452796402086));
#199268=CARTESIAN_POINT('Ctrl Pts',(9.62685282551652,15.2,4.21533221424165));
#199269=CARTESIAN_POINT('Ctrl Pts',(9.63026928922573,15.2,4.21613646446244));
#199270=CARTESIAN_POINT('Ctrl Pts',(9.63373204098209,15.2,4.21694160434445));
#199271=CARTESIAN_POINT('Ctrl Pts',(9.63724057986057,15.2,4.21774705068874));
#199272=CARTESIAN_POINT('Ctrl Pts',(9.64133387543126,15.2,4.21868673813918));
#199273=CARTESIAN_POINT('Ctrl Pts',(9.64548949482863,15.2,4.21962684247424));
#199274=CARTESIAN_POINT('Ctrl Pts',(9.64970666424153,15.2,4.22056646347498));
#199275=CARTESIAN_POINT('Ctrl Pts',(9.65332138069351,15.2,4.22137185286239));
#199276=CARTESIAN_POINT('Ctrl Pts',(9.65698131586871,15.2,4.22217688818619));
#199277=CARTESIAN_POINT('Ctrl Pts',(9.6606859936666,15.2,4.22298101661386));
#199278=CARTESIAN_POINT('Ctrl Pts',(9.66439067180099,15.2,4.22378514511458));
#199279=CARTESIAN_POINT('Ctrl Pts',(9.66814009081196,15.2,4.22458836783545));
#199280=CARTESIAN_POINT('Ctrl Pts',(9.67193378093839,15.2,4.22539014362905));
#199281=CARTESIAN_POINT('Ctrl Pts',(9.67572747072024,15.2,4.22619191934981));
#199282=CARTESIAN_POINT('Ctrl Pts',(9.67956543148328,15.2,4.22699225134241));
#199283=CARTESIAN_POINT('Ctrl Pts',(9.68344720027664,15.2,4.22779061098368));
#199284=CARTESIAN_POINT('Ctrl Pts',(9.68732896906999,15.2,4.22858897062496));
#199285=CARTESIAN_POINT('Ctrl Pts',(9.69125454579651,15.2,4.22938535806045));
#199286=CARTESIAN_POINT('Ctrl Pts',(9.69522347448375,15.2,4.23017926144838));
#199287=CARTESIAN_POINT('Ctrl Pts',(9.69853091517662,15.2,4.23084084762902));
#199288=CARTESIAN_POINT('Ctrl Pts',(9.70186846165916,15.2,4.2315007060513));
#199289=CARTESIAN_POINT('Ctrl Pts',(9.70523585408815,15.2,4.23215854973196));
#199290=CARTESIAN_POINT('Ctrl Pts',(9.70860324651715,15.2,4.23281639341262));
#199291=CARTESIAN_POINT('Ctrl Pts',(9.71200048621029,15.2,4.23347221832444));
#199292=CARTESIAN_POINT('Ctrl Pts',(9.71542731303134,15.2,4.2341257422163));
#199293=CARTESIAN_POINT('Ctrl Pts',(9.71953950506719,15.2,4.23490997085804));
#199294=CARTESIAN_POINT('Ctrl Pts',(9.72369430671445,15.2,4.23569088423493));
#199295=CARTESIAN_POINT('Ctrl Pts',(9.72789127855908,15.2,4.23646799712362));
#199296=CARTESIAN_POINT('Ctrl Pts',(9.73138875522334,15.2,4.23711559122106));
#199297=CARTESIAN_POINT('Ctrl Pts',(9.73491551802269,15.2,4.23776054943762));
#199298=CARTESIAN_POINT('Ctrl Pts',(9.7384713158372,15.2,4.23840259440045));
#199299=CARTESIAN_POINT('Ctrl Pts',(9.74273827344717,15.2,4.23917304839784));
#199300=CARTESIAN_POINT('Ctrl Pts',(9.74704704393414,15.2,4.23993931013349));
#199301=CARTESIAN_POINT('Ctrl Pts',(9.75139719917405,15.2,4.24070091409134));
#199302=CARTESIAN_POINT('Ctrl Pts',(9.75502232834309,15.2,4.24133558402163));
#199303=CARTESIAN_POINT('Ctrl Pts',(9.75867619725699,15.2,4.24196702068798));
#199304=CARTESIAN_POINT('Ctrl Pts',(9.76235856323153,15.2,4.2425949605488));
#199305=CARTESIAN_POINT('Ctrl Pts',(9.76677740224046,15.2,4.24334848835441));
#199306=CARTESIAN_POINT('Ctrl Pts',(9.77123727704875,15.2,4.24409698010938));
#199307=CARTESIAN_POINT('Ctrl Pts',(9.77573777197032,15.2,4.2448399919988));
#199308=CARTESIAN_POINT('Ctrl Pts',(9.77948818454122,15.2,4.24545916859582));
#199309=CARTESIAN_POINT('Ctrl Pts',(9.78326680533643,15.2,4.24607453982349));
#199310=CARTESIAN_POINT('Ctrl Pts',(9.78707339874066,15.2,4.24668585232328));
#199311=CARTESIAN_POINT('Ctrl Pts',(9.7908799921449,15.2,4.24729716482307));
#199312=CARTESIAN_POINT('Ctrl Pts',(9.79471455740344,15.2,4.2479044191346));
#199313=CARTESIAN_POINT('Ctrl Pts',(9.79857685947333,15.2,4.24850736680331));
#199314=CARTESIAN_POINT('Ctrl Pts',(9.80243916154321,15.2,4.24911031447202));
#199315=CARTESIAN_POINT('Ctrl Pts',(9.8063292009045,15.2,4.24970895587251));
#199316=CARTESIAN_POINT('Ctrl Pts',(9.8102467452123,15.2,4.2503030483027));
#199317=CARTESIAN_POINT('Ctrl Pts',(9.81416428952011,15.2,4.25089714073288));
#199318=CARTESIAN_POINT('Ctrl Pts',(9.81810933927836,15.2,4.25148668162132));
#199319=CARTESIAN_POINT('Ctrl Pts',(9.8220816652528,15.2,4.25207143425981));
#199320=CARTESIAN_POINT('Ctrl Pts',(9.82605399122725,15.2,4.25265618689831));
#199321=CARTESIAN_POINT('Ctrl Pts',(9.83005359330769,15.2,4.25323614965339));
#199322=CARTESIAN_POINT('Ctrl Pts',(9.83408024351824,15.2,4.25381108958353));
#199323=CARTESIAN_POINT('Ctrl Pts',(9.83810689328988,15.2,4.25438602945101));
#199324=CARTESIAN_POINT('Ctrl Pts',(9.84216059332423,15.2,4.2549559434317));
#199325=CARTESIAN_POINT('Ctrl Pts',(9.84624111718282,15.2,4.25552060267614));
#199326=CARTESIAN_POINT('Ctrl Pts',(9.85032164148619,15.2,4.25608526198213));
#199327=CARTESIAN_POINT('Ctrl Pts',(9.85442899020022,15.2,4.25664466612154));
#199328=CARTESIAN_POINT('Ctrl Pts',(9.85856294047583,15.2,4.25719858792754));
#199329=CARTESIAN_POINT('Ctrl Pts',(9.86435047095179,15.2,4.25797407846802));
#199330=CARTESIAN_POINT('Ctrl Pts',(9.87019014345699,15.2,4.25873882197897));
#199331=CARTESIAN_POINT('Ctrl Pts',(9.87608135096425,15.2,4.25949220904971));
#199332=CARTESIAN_POINT('Ctrl Pts',(9.88028935626106,15.2,4.26003034266327));
#199333=CARTESIAN_POINT('Ctrl Pts',(9.88452365741654,15.2,4.2605626834));
#199334=CARTESIAN_POINT('Ctrl Pts',(9.88878403595821,15.2,4.26108901048334));
#199335=CARTESIAN_POINT('Ctrl Pts',(9.89304441449987,15.2,4.26161533756667));
#199336=CARTESIAN_POINT('Ctrl Pts',(9.89733087027703,15.2,4.26213565575907));
#199337=CARTESIAN_POINT('Ctrl Pts',(9.90164318897723,15.2,4.26264974527528));
#199338=CARTESIAN_POINT('Ctrl Pts',(9.90509304365537,15.2,4.26306101685463));
#199339=CARTESIAN_POINT('Ctrl Pts',(9.90855945177796,15.2,4.26346830417495));
#199340=CARTESIAN_POINT('Ctrl Pts',(9.91204230238044,15.2,4.26387149897575));
#199341=CARTESIAN_POINT('Ctrl Pts',(9.91552515345746,15.2,4.26427469383147));
#199342=CARTESIAN_POINT('Ctrl Pts',(9.91902444834994,15.2,4.26467379595904));
#199343=CARTESIAN_POINT('Ctrl Pts',(9.92254007804154,15.2,4.26506869825834));
#199344=CARTESIAN_POINT('Ctrl Pts',(9.92693461491655,15.2,4.26556232610556));
#199345=CARTESIAN_POINT('Ctrl Pts',(9.93135467435427,15.2,4.26604939372033));
#199346=CARTESIAN_POINT('Ctrl Pts',(9.93580004798564,15.2,4.26652969400026));
#199347=CARTESIAN_POINT('Ctrl Pts',(9.93935634660001,15.2,4.2669139341928));
#199348=CARTESIAN_POINT('Ctrl Pts',(9.9429288464165,15.2,4.26729384361607));
#199349=CARTESIAN_POINT('Ctrl Pts',(9.94651744095482,15.2,4.26766931919694));
#199350=CARTESIAN_POINT('Ctrl Pts',(9.95010603598209,15.2,4.26804479482897));
#199351=CARTESIAN_POINT('Ctrl Pts',(9.9537107239081,15.2,4.26841583600502));
#199352=CARTESIAN_POINT('Ctrl Pts',(9.95733140221654,15.2,4.26878234219167));
#199353=CARTESIAN_POINT('Ctrl Pts',(9.96095208052498,15.2,4.26914884837832));
#199354=CARTESIAN_POINT('Ctrl Pts',(9.96458874695751,15.2,4.26951081646443));
#199355=CARTESIAN_POINT('Ctrl Pts',(9.96824129804708,15.2,4.26986814931676));
#199356=CARTESIAN_POINT('Ctrl Pts',(9.97189384863901,15.2,4.27022548212041));
#199357=CARTESIAN_POINT('Ctrl Pts',(9.97556228326243,15.2,4.27057817647662));
#199358=CARTESIAN_POINT('Ctrl Pts',(9.97924649725571,15.2,4.27092613544977));
#199359=CARTESIAN_POINT('Ctrl Pts',(9.98385176512377,15.2,4.27136108420176));
#199360=CARTESIAN_POINT('Ctrl Pts',(9.98848168787209,15.2,4.27178863162222));
#199361=CARTESIAN_POINT('Ctrl Pts',(9.99313606648321,15.2,4.27220858773334));
#199362=CARTESIAN_POINT('Ctrl Pts',(9.99779044509433,15.2,4.27262854384445));
#199363=CARTESIAN_POINT('Ctrl Pts',(10.002469276581,15.2,4.27304090733174));
#199364=CARTESIAN_POINT('Ctrl Pts',(10.0071723634774,15.2,4.27344549025022));
#199365=CARTESIAN_POINT('Ctrl Pts',(10.010934832687,15.2,4.27376915655855));
#199366=CARTESIAN_POINT('Ctrl Pts',(10.0147128242775,15.2,4.27408784355718));
#199367=CARTESIAN_POINT('Ctrl Pts',(10.0185062363547,15.2,4.27440145519873));
#199368=CARTESIAN_POINT('Ctrl Pts',(10.0232480018388,15.2,4.27479346978271));
#199369=CARTESIAN_POINT('Ctrl Pts',(10.0280138644809,15.2,4.27517755617239));
#199370=CARTESIAN_POINT('Ctrl Pts',(10.0328036241317,15.2,4.27555352999249));
#199371=CARTESIAN_POINT('Ctrl Pts',(10.0375933837825,15.2,4.2759295038126));
#199372=CARTESIAN_POINT('Ctrl Pts',(10.0424070412595,15.2,4.2762973645508));
#199373=CARTESIAN_POINT('Ctrl Pts',(10.0472444026801,15.2,4.27665693345824));
#199374=CARTESIAN_POINT('Ctrl Pts',(10.0511142920274,15.2,4.27694458859986));
#199375=CARTESIAN_POINT('Ctrl Pts',(10.0549993504859,15.2,4.27722693739397));
#199376=CARTESIAN_POINT('Ctrl Pts',(10.0588994803105,15.2,4.2775038877976));
#199377=CARTESIAN_POINT('Ctrl Pts',(10.0627996096038,15.2,4.27778083816349));
#199378=CARTESIAN_POINT('Ctrl Pts',(10.0667148089273,15.2,4.27805239009714));
#199379=CARTESIAN_POINT('Ctrl Pts',(10.0706449808823,15.2,4.27831845446484));
#199380=CARTESIAN_POINT('Ctrl Pts',(10.0745751533728,15.2,4.27858451886878));
#199381=CARTESIAN_POINT('Ctrl Pts',(10.0785202979298,15.2,4.27884509511848));
#199382=CARTESIAN_POINT('Ctrl Pts',(10.0824803170526,15.2,4.27910009546685));
#199383=CARTESIAN_POINT('Ctrl Pts',(10.0864403356358,15.2,4.27935509578047));
#199384=CARTESIAN_POINT('Ctrl Pts',(10.0904152277141,15.2,4.27960451975727));
#199385=CARTESIAN_POINT('Ctrl Pts',(10.0944048958309,15.2,4.27984827896015));
#199386=CARTESIAN_POINT('Ctrl Pts',(10.0983945644913,15.2,4.28009203819624));
#199387=CARTESIAN_POINT('Ctrl Pts',(10.1023990111947,15.2,4.2803301339179));
#199388=CARTESIAN_POINT('Ctrl Pts',(10.1064181370249,15.2,4.28056247954168));
#199389=CARTESIAN_POINT('Ctrl Pts',(10.1114420440388,15.2,4.28085291155556));
#199390=CARTESIAN_POINT('Ctrl Pts',(10.116488887711,15.2,4.28113435610556));
#199391=CARTESIAN_POINT('Ctrl Pts',(10.1215584822249,15.2,4.28140665075834));
#199392=CARTESIAN_POINT('Ctrl Pts',(10.1266280767388,15.2,4.28167894541112));
#199393=CARTESIAN_POINT('Ctrl Pts',(10.1317204193683,15.2,4.28194208678235));
#199394=CARTESIAN_POINT('Ctrl Pts',(10.1368353265443,15.2,4.28219591324181));
#199395=CARTESIAN_POINT('Ctrl Pts',(10.1409272519507,15.2,4.28239897439278));
#199396=CARTESIAN_POINT('Ctrl Pts',(10.1450336187173,15.2,4.28259607423933));
#199397=CARTESIAN_POINT('Ctrl Pts',(10.1491543301012,15.2,4.2827871280021));
#199398=CARTESIAN_POINT('Ctrl Pts',(10.1532750420465,15.2,4.28297818179091));
#199399=CARTESIAN_POINT('Ctrl Pts',(10.1574101010599,15.2,4.28316319121526));
#199400=CARTESIAN_POINT('Ctrl Pts',(10.1615594110082,15.2,4.28334207372501));
#199401=CARTESIAN_POINT('Ctrl Pts',(10.1677833753654,15.2,4.28361039746527));
#199402=CARTESIAN_POINT('Ctrl Pts',(10.1740394048079,15.2,4.28386493638929));
#199403=CARTESIAN_POINT('Ctrl Pts',(10.1803271873917,15.2,4.28410541622671));
#199404=CARTESIAN_POINT('Ctrl Pts',(10.1855670064019,15.2,4.28430581609852));
#199405=CARTESIAN_POINT('Ctrl Pts',(10.1908288732056,15.2,4.28449645561538));
#199406=CARTESIAN_POINT('Ctrl Pts',(10.1961126094545,15.2,4.28467717721313));
#199407=CARTESIAN_POINT('Ctrl Pts',(10.2003395986839,15.2,4.28482175449921));
#199408=CARTESIAN_POINT('Ctrl Pts',(10.2045805831178,15.2,4.28495998663174));
#199409=CARTESIAN_POINT('Ctrl Pts',(10.2088354710729,15.2,4.28509179252739));
#199410=CARTESIAN_POINT('Ctrl Pts',(10.2130903584481,15.2,4.28522359840509));
#199411=CARTESIAN_POINT('Ctrl Pts',(10.2173591502131,15.2,4.28534897926372));
#199412=CARTESIAN_POINT('Ctrl Pts',(10.2216417543535,15.2,4.28546785848272));
#199413=CARTESIAN_POINT('Ctrl Pts',(10.2259243590775,15.2,4.28558673771793));
#199414=CARTESIAN_POINT('Ctrl Pts',(10.2302207750916,15.2,4.28569911543937));
#199415=CARTESIAN_POINT('Ctrl Pts',(10.2345309118274,15.2,4.28580491350026));
#199416=CARTESIAN_POINT('Ctrl Pts',(10.2388410479759,15.2,4.28591071154674));
#199417=CARTESIAN_POINT('Ctrl Pts',(10.2431649057995,15.2,4.28600993291398));
#199418=CARTESIAN_POINT('Ctrl Pts',(10.2475023938324,15.2,4.28610250001821));
#199419=CARTESIAN_POINT('Ctrl Pts',(10.2518398824563,15.2,4.28619506713505));
#199420=CARTESIAN_POINT('Ctrl Pts',(10.2561910007951,15.2,4.28628097952041));
#199421=CARTESIAN_POINT('Ctrl Pts',(10.2605556607195,15.2,4.28636016402506));
#199422=CARTESIAN_POINT('Ctrl Pts',(10.2649203200493,15.2,4.28643934851893));
#199423=CARTESIAN_POINT('Ctrl Pts',(10.2692985199811,15.2,4.28651180541339));
#199424=CARTESIAN_POINT('Ctrl Pts',(10.2736901700652,15.2,4.28657745946427));
#199425=CARTESIAN_POINT('Ctrl Pts',(10.2802776460888,15.2,4.28667594055402));
#199426=CARTESIAN_POINT('Ctrl Pts',(10.286895386357,15.2,4.28675911825896));
#199427=CARTESIAN_POINT('Ctrl Pts',(10.293543091304,15.2,4.28682674701196));
#199428=CARTESIAN_POINT('Ctrl Pts',(10.3001907956471,15.2,4.28689437575882));
#199429=CARTESIAN_POINT('Ctrl Pts',(10.3068684645602,15.2,4.28694645341778));
#199430=CARTESIAN_POINT('Ctrl Pts',(10.3135757990135,15.2,4.28698274325));
#199431=CARTESIAN_POINT('Ctrl Pts',(10.3169294662402,15.2,4.28700088816611));
#199432=CARTESIAN_POINT('Ctrl Pts',(10.3202905501726,15.2,4.28701508619886));
#199433=CARTESIAN_POINT('Ctrl Pts',(10.3236590138412,15.2,4.2870253062405));
#199434=CARTESIAN_POINT('Ctrl Pts',(10.3270274775098,15.2,4.28703552628215));
#199435=CARTESIAN_POINT('Ctrl Pts',(10.3304033206696,15.2,4.28704176973239));
#199436=CARTESIAN_POINT('Ctrl Pts',(10.3337865067957,15.2,4.28704400669119));
#199437=CARTESIAN_POINT('Ctrl Pts',(10.3371696935364,15.2,4.2870462436504));
#199438=CARTESIAN_POINT('Ctrl Pts',(10.3405602227125,15.2,4.2870444743168));
#199439=CARTESIAN_POINT('Ctrl Pts',(10.3439580580406,15.2,4.28703866927374));
#199440=CARTESIAN_POINT('Ctrl Pts',(10.3473558927515,15.2,4.28703286423174));
#199441=CARTESIAN_POINT('Ctrl Pts',(10.3507610332295,15.2,4.28702302376461));
#199442=CARTESIAN_POINT('Ctrl Pts',(10.3541734436102,15.2,4.28700911872228));
#199443=CARTESIAN_POINT('Ctrl Pts',(10.3575858539909,15.2,4.28699521367995));
#199444=CARTESIAN_POINT('Ctrl Pts',(10.3610055337141,15.2,4.28697724408043));
#199445=CARTESIAN_POINT('Ctrl Pts',(10.3644324468819,15.2,4.28695518153921));
#199446=CARTESIAN_POINT('Ctrl Pts',(10.3678593600497,15.2,4.28693311899799));
#199447=CARTESIAN_POINT('Ctrl Pts',(10.3712935062416,15.2,4.28690696299891));
#199448=CARTESIAN_POINT('Ctrl Pts',(10.3747348484916,15.2,4.28687668645835));
#199449=CARTESIAN_POINT('Ctrl Pts',(10.3781761907415,15.2,4.28684640991778));
#199450=CARTESIAN_POINT('Ctrl Pts',(10.3816247301495,15.2,4.28681201195238));
#199451=CARTESIAN_POINT('Ctrl Pts',(10.3850804298983,15.2,4.28677346349581));
#199452=CARTESIAN_POINT('Ctrl Pts',(10.3885361296472,15.2,4.28673491503924));
#199453=CARTESIAN_POINT('Ctrl Pts',(10.3919989898822,15.2,4.2866922177592));
#199454=CARTESIAN_POINT('Ctrl Pts',(10.3954689752619,15.2,4.28664534275904));
#199455=CARTESIAN_POINT('Ctrl Pts',(10.3989389606417,15.2,4.28659846775889));
#199456=CARTESIAN_POINT('Ctrl Pts',(10.4024160710846,15.2,4.28654741500947));
#199457=CARTESIAN_POINT('Ctrl Pts',(10.4059002692903,15.2,4.28649215747039));
#199458=CARTESIAN_POINT('Ctrl Pts',(10.411707266511,15.2,4.28640006156857));
#199459=CARTESIAN_POINT('Ctrl Pts',(10.4175339539868,15.2,4.28629628475861));
#199460=CARTESIAN_POINT('Ctrl Pts',(10.4233801677352,15.2,4.28618070052346));
#199461=CARTESIAN_POINT('Ctrl Pts',(10.426887896494,15.2,4.2861113499723));
#199462=CARTESIAN_POINT('Ctrl Pts',(10.4304026535215,15.2,4.28603774822827));
#199463=CARTESIAN_POINT('Ctrl Pts',(10.4339244052843,15.2,4.28595986921637));
#199464=CARTESIAN_POINT('Ctrl Pts',(10.4374461564073,15.2,4.28588199021861));
#199465=CARTESIAN_POINT('Ctrl Pts',(10.4409749005517,15.2,4.28579983391826));
#199466=CARTESIAN_POINT('Ctrl Pts',(10.444510603434,15.2,4.28571337249991));
#199467=CARTESIAN_POINT('Ctrl Pts',(10.4480463063163,15.2,4.28562691108157));
#199468=CARTESIAN_POINT('Ctrl Pts',(10.4515889674319,15.2,4.28553614590317));
#199469=CARTESIAN_POINT('Ctrl Pts',(10.4551385511369,15.2,4.28544104944791));
#199470=CARTESIAN_POINT('Ctrl Pts',(10.4598713291953,15.2,4.28531425417999));
#199471=CARTESIAN_POINT('Ctrl Pts',(10.4646164147706,15.2,4.28517975916085));
#199472=CARTESIAN_POINT('Ctrl Pts',(10.4693737242137,15.2,4.2850375025066));
#199473=CARTESIAN_POINT('Ctrl Pts',(10.4753203615039,15.2,4.28485968167426));
#199474=CARTESIAN_POINT('Ctrl Pts',(10.4812860999909,15.2,4.28466973338657));
#199475=CARTESIAN_POINT('Ctrl Pts',(10.4872707756838,15.2,4.28446753602646));
#199476=CARTESIAN_POINT('Ctrl Pts',(10.4932554513767,15.2,4.28426533866635));
#199477=CARTESIAN_POINT('Ctrl Pts',(10.499259066218,15.2,4.28405089300899));
#199478=CARTESIAN_POINT('Ctrl Pts',(10.5052814588092,15.2,4.2838240820263));
#199479=CARTESIAN_POINT('Ctrl Pts',(10.5113038514004,15.2,4.28359727104361));
#199480=CARTESIAN_POINT('Ctrl Pts',(10.5173450222325,15.2,4.2833580927713));
#199481=CARTESIAN_POINT('Ctrl Pts',(10.5234048088287,15.2,4.28310643200807));
#199482=CARTESIAN_POINT('Ctrl Pts',(10.5270406806543,15.2,4.28295543555561));
#199483=CARTESIAN_POINT('Ctrl Pts',(10.5306832557212,15.2,4.28279994502846));
#199484=CARTESIAN_POINT('Ctrl Pts',(10.5343324984627,15.2,4.28263993557656));
#199485=CARTESIAN_POINT('Ctrl Pts',(10.5379817418672,15.2,4.28247992609559));
#199486=CARTESIAN_POINT('Ctrl Pts',(10.5416376536818,15.2,4.28231539773834));
#199487=CARTESIAN_POINT('Ctrl Pts',(10.54530019909,15.2,4.28214632671315));
#199488=CARTESIAN_POINT('Ctrl Pts',(10.5514044398845,15.2,4.28186454174283));
#199489=CARTESIAN_POINT('Ctrl Pts',(10.557527107662,15.2,4.281570133839));
#199490=CARTESIAN_POINT('Ctrl Pts',(10.5636680442133,15.2,4.28126299304019));
#199491=CARTESIAN_POINT('Ctrl Pts',(10.5673526070813,15.2,4.28107870851403));
#199492=CARTESIAN_POINT('Ctrl Pts',(10.5710437461177,15.2,4.28088983916992));
#199493=CARTESIAN_POINT('Ctrl Pts',(10.574741428531,15.2,4.28069636218284));
#199494=CARTESIAN_POINT('Ctrl Pts',(10.5784391102725,15.2,4.28050288523091));
#199495=CARTESIAN_POINT('Ctrl Pts',(10.5821433354387,15.2,4.28030480038755));
#199496=CARTESIAN_POINT('Ctrl Pts',(10.5858540701795,15.2,4.28010208297784));
#199497=CARTESIAN_POINT('Ctrl Pts',(10.5908017162758,15.2,4.27983179311051));
#199498=CARTESIAN_POINT('Ctrl Pts',(10.5957609355127,15.2,4.2795532686012));
#199499=CARTESIAN_POINT('Ctrl Pts',(10.6007316445204,15.2,4.27926645199992));
#199500=CARTESIAN_POINT('Ctrl Pts',(10.6044596764454,15.2,4.2790513395392));
#199501=CARTESIAN_POINT('Ctrl Pts',(10.6081941717378,15.2,4.27883156294015));
#199502=CARTESIAN_POINT('Ctrl Pts',(10.6119350964761,15.2,4.27860709757395));
#199503=CARTESIAN_POINT('Ctrl Pts',(10.6156760218939,15.2,4.27838263216697));
#199504=CARTESIAN_POINT('Ctrl Pts',(10.6194233766885,15.2,4.27815347941699));
#199505=CARTESIAN_POINT('Ctrl Pts',(10.6231771321099,15.2,4.2779196179657));
#199506=CARTESIAN_POINT('Ctrl Pts',(10.6269308868494,15.2,4.27768575655688));
#199507=CARTESIAN_POINT('Ctrl Pts',(10.6306910417802,15.2,4.27744718628166));
#199508=CARTESIAN_POINT('Ctrl Pts',(10.6344575619356,15.2,4.27720388420675));
#199509=CARTESIAN_POINT('Ctrl Pts',(10.6394795885813,15.2,4.27687948145495));
#199510=CARTESIAN_POINT('Ctrl Pts',(10.6445129285515,15.2,4.27654666277957));
#199511=CARTESIAN_POINT('Ctrl Pts',(10.6495574895013,15.2,4.27620536429116));
#199512=CARTESIAN_POINT('Ctrl Pts',(10.6533409103855,15.2,4.27594939041323));
#199513=CARTESIAN_POINT('Ctrl Pts',(10.6571306412445,15.2,4.27568864613094));
#199514=CARTESIAN_POINT('Ctrl Pts',(10.660926659439,15.2,4.27542311601623));
#199515=CARTESIAN_POINT('Ctrl Pts',(10.6659880174915,15.2,4.27506907583115));
#199516=CARTESIAN_POINT('Ctrl Pts',(10.6710605472813,15.2,4.27470652910107));
#199517=CARTESIAN_POINT('Ctrl Pts',(10.6761442619999,15.2,4.27433546899999));
#199518=CARTESIAN_POINT('Ctrl Pts',(9.86852965799994,15.2,3.20199116299998));
#199519=CARTESIAN_POINT('Ctrl Pts',(9.86852965799994,11.6,3.20199116299998));
#199520=CARTESIAN_POINT('Ctrl Pts',(9.86869026599994,15.2,3.20205902699998));
#199521=CARTESIAN_POINT('Ctrl Pts',(9.86869026599994,11.6,3.20205902699998));
#199522=CARTESIAN_POINT('Ctrl Pts',(9.86901705899994,15.2,3.20219720599999));
#199523=CARTESIAN_POINT('Ctrl Pts',(9.86901705899994,11.6,3.20219720599999));
#199524=CARTESIAN_POINT('Ctrl Pts',(9.86951212399994,15.2,3.20240682499998));
#199525=CARTESIAN_POINT('Ctrl Pts',(9.86951212399994,11.6,3.20240682499998));
#199526=CARTESIAN_POINT('Ctrl Pts',(9.87017881199994,15.2,3.20268969799999));
#199527=CARTESIAN_POINT('Ctrl Pts',(9.87017881199994,11.6,3.20268969799999));
#199528=CARTESIAN_POINT('Ctrl Pts',(9.87102171699994,15.2,3.20304833099998));
#199529=CARTESIAN_POINT('Ctrl Pts',(9.87102171699994,11.6,3.20304833099998));
#199530=CARTESIAN_POINT('Ctrl Pts',(9.87187791599995,15.2,3.20341363599999));
#199531=CARTESIAN_POINT('Ctrl Pts',(9.87187791599995,11.6,3.20341363599999));
#199532=CARTESIAN_POINT('Ctrl Pts',(9.87274249599994,15.2,3.20378354299999));
#199533=CARTESIAN_POINT('Ctrl Pts',(9.87274249599994,11.6,3.20378354299999));
#199534=CARTESIAN_POINT('Ctrl Pts',(9.87361542499994,15.2,3.20415805699999));
#199535=CARTESIAN_POINT('Ctrl Pts',(9.87361542499994,11.6,3.20415805699999));
#199536=CARTESIAN_POINT('Ctrl Pts',(9.87449666999994,15.2,3.20453718399998));
#199537=CARTESIAN_POINT('Ctrl Pts',(9.87449666999994,11.6,3.20453718399998));
#199538=CARTESIAN_POINT('Ctrl Pts',(9.87538619999994,15.2,3.20492093099999));
#199539=CARTESIAN_POINT('Ctrl Pts',(9.87538619999994,11.6,3.20492093099999));
#199540=CARTESIAN_POINT('Ctrl Pts',(9.87628398399995,15.2,3.20530930299999));
#199541=CARTESIAN_POINT('Ctrl Pts',(9.87628398399995,11.6,3.20530930299999));
#199542=CARTESIAN_POINT('Ctrl Pts',(9.87718998999994,15.2,3.20570230499998));
#199543=CARTESIAN_POINT('Ctrl Pts',(9.87718998999994,11.6,3.20570230499998));
#199544=CARTESIAN_POINT('Ctrl Pts',(9.87810418799994,15.2,3.20609994499998));
#199545=CARTESIAN_POINT('Ctrl Pts',(9.87810418799994,11.6,3.20609994499998));
#199546=CARTESIAN_POINT('Ctrl Pts',(9.87902654599995,15.2,3.20650222699999));
#199547=CARTESIAN_POINT('Ctrl Pts',(9.87902654599995,11.6,3.20650222699999));
#199548=CARTESIAN_POINT('Ctrl Pts',(9.87995703199994,15.2,3.20690915799998));
#199549=CARTESIAN_POINT('Ctrl Pts',(9.87995703199994,11.6,3.20690915799998));
#199550=CARTESIAN_POINT('Ctrl Pts',(9.88089561699995,15.2,3.20732074399999));
#199551=CARTESIAN_POINT('Ctrl Pts',(9.88089561699995,11.6,3.20732074399999));
#199552=CARTESIAN_POINT('Ctrl Pts',(9.88184226899994,15.2,3.20773698999999));
#199553=CARTESIAN_POINT('Ctrl Pts',(9.88184226899994,11.6,3.20773698999999));
#199554=CARTESIAN_POINT('Ctrl Pts',(9.88279695999994,15.2,3.20815789999998));
#199555=CARTESIAN_POINT('Ctrl Pts',(9.88279695999994,11.6,3.20815789999998));
#199556=CARTESIAN_POINT('Ctrl Pts',(9.88375965599994,15.2,3.20858348199998));
#199557=CARTESIAN_POINT('Ctrl Pts',(9.88375965599994,11.6,3.20858348199998));
#199558=CARTESIAN_POINT('Ctrl Pts',(9.88473033099995,15.2,3.20901374099999));
#199559=CARTESIAN_POINT('Ctrl Pts',(9.88473033099995,11.6,3.20901374099999));
#199560=CARTESIAN_POINT('Ctrl Pts',(9.88570895099994,15.2,3.20944868299998));
#199561=CARTESIAN_POINT('Ctrl Pts',(9.88570895099994,11.6,3.20944868299998));
#199562=CARTESIAN_POINT('Ctrl Pts',(9.88669548799994,15.2,3.20988831199998));
#199563=CARTESIAN_POINT('Ctrl Pts',(9.88669548799994,11.6,3.20988831199998));
#199564=CARTESIAN_POINT('Ctrl Pts',(9.88768991199995,15.2,3.21033263399999));
#199565=CARTESIAN_POINT('Ctrl Pts',(9.88768991199995,11.6,3.21033263399999));
#199566=CARTESIAN_POINT('Ctrl Pts',(9.88869219599994,15.2,3.21078165399998));
#199567=CARTESIAN_POINT('Ctrl Pts',(9.88869219599994,11.6,3.21078165399998));
#199568=CARTESIAN_POINT('Ctrl Pts',(9.88970230599995,15.2,3.21123537899999));
#199569=CARTESIAN_POINT('Ctrl Pts',(9.88970230599995,11.6,3.21123537899999));
#199570=CARTESIAN_POINT('Ctrl Pts',(9.89072021399994,15.2,3.21169381299999));
#199571=CARTESIAN_POINT('Ctrl Pts',(9.89072021399994,11.6,3.21169381299998));
#199572=CARTESIAN_POINT('Ctrl Pts',(9.89174589299994,15.2,3.21215696299999));
#199573=CARTESIAN_POINT('Ctrl Pts',(9.89174589299994,11.6,3.21215696299999));
#199574=CARTESIAN_POINT('Ctrl Pts',(9.89277931199994,15.2,3.21262483099999));
#199575=CARTESIAN_POINT('Ctrl Pts',(9.89277931199994,11.6,3.21262483099999));
#199576=CARTESIAN_POINT('Ctrl Pts',(9.89382044199995,15.2,3.21309742499999));
#199577=CARTESIAN_POINT('Ctrl Pts',(9.89382044199995,11.6,3.21309742499999));
#199578=CARTESIAN_POINT('Ctrl Pts',(9.89486925599994,15.2,3.21357474899998));
#199579=CARTESIAN_POINT('Ctrl Pts',(9.89486925599994,11.6,3.21357474899998));
#199580=CARTESIAN_POINT('Ctrl Pts',(9.89592572299994,15.2,3.21405680799998));
#199581=CARTESIAN_POINT('Ctrl Pts',(9.89592572299994,11.6,3.21405680799998));
#199582=CARTESIAN_POINT('Ctrl Pts',(9.89698981699994,15.2,3.21454360699998));
#199583=CARTESIAN_POINT('Ctrl Pts',(9.89698981699994,11.6,3.21454360699998));
#199584=CARTESIAN_POINT('Ctrl Pts',(9.89806150699994,15.2,3.21503515299998));
#199585=CARTESIAN_POINT('Ctrl Pts',(9.89806150699994,11.6,3.21503515299998));
#199586=CARTESIAN_POINT('Ctrl Pts',(9.89914076599995,15.2,3.21553144899998));
#199587=CARTESIAN_POINT('Ctrl Pts',(9.89914076599995,11.6,3.21553144899998));
#199588=CARTESIAN_POINT('Ctrl Pts',(9.90022756499994,15.2,3.21603250099999));
#199589=CARTESIAN_POINT('Ctrl Pts',(9.90022756499994,11.6,3.21603250099999));
#199590=CARTESIAN_POINT('Ctrl Pts',(9.90132187699994,15.2,3.21653831299999));
#199591=CARTESIAN_POINT('Ctrl Pts',(9.90132187699994,11.6,3.21653831299999));
#199592=CARTESIAN_POINT('Ctrl Pts',(9.90242367499994,15.2,3.21704888999999));
#199593=CARTESIAN_POINT('Ctrl Pts',(9.90242367499994,11.6,3.21704888999999));
#199594=CARTESIAN_POINT('Ctrl Pts',(9.90353292899995,15.2,3.21756423799999));
#199595=CARTESIAN_POINT('Ctrl Pts',(9.90353292899995,11.6,3.21756423799999));
#199596=CARTESIAN_POINT('Ctrl Pts',(9.90464961299995,15.2,3.21808436099998));
#199597=CARTESIAN_POINT('Ctrl Pts',(9.90464961299995,11.6,3.21808436099998));
#199598=CARTESIAN_POINT('Ctrl Pts',(9.90577369799994,15.2,3.21860926399999));
#199599=CARTESIAN_POINT('Ctrl Pts',(9.90577369799994,11.6,3.21860926399999));
#199600=CARTESIAN_POINT('Ctrl Pts',(9.90690515799994,15.2,3.21913895099998));
#199601=CARTESIAN_POINT('Ctrl Pts',(9.90690515799994,11.6,3.21913895099998));
#199602=CARTESIAN_POINT('Ctrl Pts',(9.90804396399995,15.2,3.21967342899999));
#199603=CARTESIAN_POINT('Ctrl Pts',(9.90804396399995,11.6,3.21967342899998));
#199604=CARTESIAN_POINT('Ctrl Pts',(9.90919009099994,15.2,3.22021269999999));
#199605=CARTESIAN_POINT('Ctrl Pts',(9.90919009099994,11.6,3.22021269999999));
#199606=CARTESIAN_POINT('Ctrl Pts',(9.91034350999995,15.2,3.22075676899999));
#199607=CARTESIAN_POINT('Ctrl Pts',(9.91034350999995,11.6,3.22075676899999));
#199608=CARTESIAN_POINT('Ctrl Pts',(9.91150419599995,15.2,3.22130564299999));
#199609=CARTESIAN_POINT('Ctrl Pts',(9.91150419599995,11.6,3.22130564299999));
#199610=CARTESIAN_POINT('Ctrl Pts',(9.91267211999994,15.2,3.22185932499998));
#199611=CARTESIAN_POINT('Ctrl Pts',(9.91267211999994,11.6,3.22185932499998));
#199612=CARTESIAN_POINT('Ctrl Pts',(9.91384725799995,15.2,3.22241781899999));
#199613=CARTESIAN_POINT('Ctrl Pts',(9.91384725799995,11.6,3.22241781899999));
#199614=CARTESIAN_POINT('Ctrl Pts',(9.91502957999994,15.2,3.22298113099999));
#199615=CARTESIAN_POINT('Ctrl Pts',(9.91502957999994,11.6,3.22298113099999));
#199616=CARTESIAN_POINT('Ctrl Pts',(9.91621906199994,15.2,3.22354926399999));
#199617=CARTESIAN_POINT('Ctrl Pts',(9.91621906199994,11.6,3.22354926399999));
#199618=CARTESIAN_POINT('Ctrl Pts',(9.91741567699994,15.2,3.22412222299998));
#199619=CARTESIAN_POINT('Ctrl Pts',(9.91741567699994,11.6,3.22412222299998));
#199620=CARTESIAN_POINT('Ctrl Pts',(9.91861939899995,15.2,3.22470001299998));
#199621=CARTESIAN_POINT('Ctrl Pts',(9.91861939899995,11.6,3.22470001299998));
#199622=CARTESIAN_POINT('Ctrl Pts',(9.91983020199994,15.2,3.22528263799998));
#199623=CARTESIAN_POINT('Ctrl Pts',(9.91983020199994,11.6,3.22528263799998));
#199624=CARTESIAN_POINT('Ctrl Pts',(9.92104805799995,15.2,3.22587010299999));
#199625=CARTESIAN_POINT('Ctrl Pts',(9.92104805799995,11.6,3.22587010299999));
#199626=CARTESIAN_POINT('Ctrl Pts',(9.92227294399994,15.2,3.22646241099999));
#199627=CARTESIAN_POINT('Ctrl Pts',(9.92227294399994,11.6,3.22646241099999));
#199628=CARTESIAN_POINT('Ctrl Pts',(9.92350483199995,15.2,3.22705956599999));
#199629=CARTESIAN_POINT('Ctrl Pts',(9.92350483199995,11.6,3.22705956599999));
#199630=CARTESIAN_POINT('Ctrl Pts',(9.92474369699995,15.2,3.22766157499998));
#199631=CARTESIAN_POINT('Ctrl Pts',(9.92474369699995,11.6,3.22766157499998));
#199632=CARTESIAN_POINT('Ctrl Pts',(9.92598951399994,15.2,3.22826843999999));
#199633=CARTESIAN_POINT('Ctrl Pts',(9.92598951399994,11.6,3.22826843999999));
#199634=CARTESIAN_POINT('Ctrl Pts',(9.92724225599994,15.2,3.22888016499999));
#199635=CARTESIAN_POINT('Ctrl Pts',(9.92724225599994,11.6,3.22888016499998));
#199636=CARTESIAN_POINT('Ctrl Pts',(9.92850189999994,15.2,3.22949675599999));
#199637=CARTESIAN_POINT('Ctrl Pts',(9.92850189999994,11.6,3.22949675599998));
#199638=CARTESIAN_POINT('Ctrl Pts',(9.92976841899995,15.2,3.23011821499998));
#199639=CARTESIAN_POINT('Ctrl Pts',(9.92976841899995,11.6,3.23011821499998));
#199640=CARTESIAN_POINT('Ctrl Pts',(9.93104178699994,15.2,3.23074454899999));
#199641=CARTESIAN_POINT('Ctrl Pts',(9.93104178699994,11.6,3.23074454899999));
#199642=CARTESIAN_POINT('Ctrl Pts',(9.93232198099994,15.2,3.23137575799999));
#199643=CARTESIAN_POINT('Ctrl Pts',(9.93232198099994,11.6,3.23137575799999));
#199644=CARTESIAN_POINT('Ctrl Pts',(9.93360897499995,15.2,3.23201184999999));
#199645=CARTESIAN_POINT('Ctrl Pts',(9.93360897499995,11.6,3.23201184999998));
#199646=CARTESIAN_POINT('Ctrl Pts',(9.93490274399995,15.2,3.23265282699998));
#199647=CARTESIAN_POINT('Ctrl Pts',(9.93490274399995,11.6,3.23265282699998));
#199648=CARTESIAN_POINT('Ctrl Pts',(9.93620326399995,15.2,3.23329869199998));
#199649=CARTESIAN_POINT('Ctrl Pts',(9.93620326399995,11.6,3.23329869199998));
#199650=CARTESIAN_POINT('Ctrl Pts',(9.93751050999995,15.2,3.23394945199999));
#199651=CARTESIAN_POINT('Ctrl Pts',(9.93751050999995,11.6,3.23394945199999));
#199652=CARTESIAN_POINT('Ctrl Pts',(9.93882445599995,15.2,3.23460510899999));
#199653=CARTESIAN_POINT('Ctrl Pts',(9.93882445599995,11.6,3.23460510899999));
#199654=CARTESIAN_POINT('Ctrl Pts',(9.94014507999994,15.2,3.23526566699999));
#199655=CARTESIAN_POINT('Ctrl Pts',(9.94014507999994,11.6,3.23526566699999));
#199656=CARTESIAN_POINT('Ctrl Pts',(9.94147235499995,15.2,3.23593112999998));
#199657=CARTESIAN_POINT('Ctrl Pts',(9.94147235499995,11.6,3.23593112999998));
#199658=CARTESIAN_POINT('Ctrl Pts',(9.94280625999994,15.2,3.23660150199998));
#199659=CARTESIAN_POINT('Ctrl Pts',(9.94280625999994,11.6,3.23660150199998));
#199660=CARTESIAN_POINT('Ctrl Pts',(9.94414676699994,15.2,3.23727678699999));
#199661=CARTESIAN_POINT('Ctrl Pts',(9.94414676699994,11.6,3.23727678699999));
#199662=CARTESIAN_POINT('Ctrl Pts',(9.94549385499995,15.2,3.23795698799999));
#199663=CARTESIAN_POINT('Ctrl Pts',(9.94549385499995,11.6,3.23795698799999));
#199664=CARTESIAN_POINT('Ctrl Pts',(9.94684749899994,15.2,3.23864210899998));
#199665=CARTESIAN_POINT('Ctrl Pts',(9.94684749899994,11.6,3.23864210899998));
#199666=CARTESIAN_POINT('Ctrl Pts',(9.94820767499995,15.2,3.23933215499999));
#199667=CARTESIAN_POINT('Ctrl Pts',(9.94820767499995,11.6,3.23933215499998));
#199668=CARTESIAN_POINT('Ctrl Pts',(9.94957435799994,15.2,3.24002712799999));
#199669=CARTESIAN_POINT('Ctrl Pts',(9.94957435799994,11.6,3.24002712799999));
#199670=CARTESIAN_POINT('Ctrl Pts',(9.95094752599995,15.2,3.24072703399998));
#199671=CARTESIAN_POINT('Ctrl Pts',(9.95094752599995,11.6,3.24072703399998));
#199672=CARTESIAN_POINT('Ctrl Pts',(9.95232715499995,15.2,3.24143187399999));
#199673=CARTESIAN_POINT('Ctrl Pts',(9.95232715499995,11.6,3.24143187399999));
#199674=CARTESIAN_POINT('Ctrl Pts',(9.95371322099994,15.2,3.24214165199999));
#199675=CARTESIAN_POINT('Ctrl Pts',(9.95371322099994,11.6,3.24214165199999));
#199676=CARTESIAN_POINT('Ctrl Pts',(9.95510570199994,15.2,3.24285637299998));
#199677=CARTESIAN_POINT('Ctrl Pts',(9.95510570199994,11.6,3.24285637299998));
#199678=CARTESIAN_POINT('Ctrl Pts',(9.95650457299995,15.2,3.24357603999999));
#199679=CARTESIAN_POINT('Ctrl Pts',(9.95650457299995,11.6,3.24357603999999));
#199680=CARTESIAN_POINT('Ctrl Pts',(9.95790981099995,15.2,3.24430065599999));
#199681=CARTESIAN_POINT('Ctrl Pts',(9.95790981099995,11.6,3.24430065599999));
#199682=CARTESIAN_POINT('Ctrl Pts',(9.95932139299994,15.2,3.24503022499999));
#199683=CARTESIAN_POINT('Ctrl Pts',(9.95932139299994,11.6,3.24503022499999));
#199684=CARTESIAN_POINT('Ctrl Pts',(9.96073929699994,15.2,3.24576475099998));
#199685=CARTESIAN_POINT('Ctrl Pts',(9.96073929699994,11.6,3.24576475099998));
#199686=CARTESIAN_POINT('Ctrl Pts',(9.96216349899995,15.2,3.24650423599999));
#199687=CARTESIAN_POINT('Ctrl Pts',(9.96216349899995,11.6,3.24650423599999));
#199688=CARTESIAN_POINT('Ctrl Pts',(9.96359397499995,15.2,3.24724868599999));
#199689=CARTESIAN_POINT('Ctrl Pts',(9.96359397499995,11.6,3.24724868599999));
#199690=CARTESIAN_POINT('Ctrl Pts',(9.96503070399994,15.2,3.24799810099999));
#199691=CARTESIAN_POINT('Ctrl Pts',(9.96503070399994,11.6,3.24799810099999));
#199692=CARTESIAN_POINT('Ctrl Pts',(9.96647366299995,15.2,3.24875248699998));
#199693=CARTESIAN_POINT('Ctrl Pts',(9.96647366299995,11.6,3.24875248699998));
#199694=CARTESIAN_POINT('Ctrl Pts',(9.96792282999994,15.2,3.24951184599998));
#199695=CARTESIAN_POINT('Ctrl Pts',(9.96792282999994,11.6,3.24951184599998));
#199696=CARTESIAN_POINT('Ctrl Pts',(9.96937817999994,15.2,3.25027618299998));
#199697=CARTESIAN_POINT('Ctrl Pts',(9.96937817999994,11.6,3.25027618299998));
#199698=CARTESIAN_POINT('Ctrl Pts',(9.97083969299995,15.2,3.25104549899999));
#199699=CARTESIAN_POINT('Ctrl Pts',(9.97083969299995,11.6,3.25104549899999));
#199700=CARTESIAN_POINT('Ctrl Pts',(9.97230734499994,15.2,3.25181979899998));
#199701=CARTESIAN_POINT('Ctrl Pts',(9.97230734499994,11.6,3.25181979899998));
#199702=CARTESIAN_POINT('Ctrl Pts',(9.97378111499994,15.2,3.25259908499999));
#199703=CARTESIAN_POINT('Ctrl Pts',(9.97378111499994,11.6,3.25259908499999));
#199704=CARTESIAN_POINT('Ctrl Pts',(9.97526097999994,15.2,3.25338336199999));
#199705=CARTESIAN_POINT('Ctrl Pts',(9.97526097999994,11.6,3.25338336199999));
#199706=CARTESIAN_POINT('Ctrl Pts',(9.97674691799994,15.2,3.25417263099999));
#199707=CARTESIAN_POINT('Ctrl Pts',(9.97674691799994,11.6,3.25417263099998));
#199708=CARTESIAN_POINT('Ctrl Pts',(9.97823890599994,15.2,3.25496689699998));
#199709=CARTESIAN_POINT('Ctrl Pts',(9.97823890599994,11.6,3.25496689699998));
#199710=CARTESIAN_POINT('Ctrl Pts',(9.97973692499994,15.2,3.25576616199999));
#199711=CARTESIAN_POINT('Ctrl Pts',(9.97973692499994,11.6,3.25576616199999));
#199712=CARTESIAN_POINT('Ctrl Pts',(9.98124094999995,15.2,3.25657042999998));
#199713=CARTESIAN_POINT('Ctrl Pts',(9.98124094999995,11.6,3.25657042999998));
#199714=CARTESIAN_POINT('Ctrl Pts',(9.98275095899994,15.2,3.25737970399998));
#199715=CARTESIAN_POINT('Ctrl Pts',(9.98275095899994,11.6,3.25737970399998));
#199716=CARTESIAN_POINT('Ctrl Pts',(9.98426693399994,15.2,3.25819398599998));
#199717=CARTESIAN_POINT('Ctrl Pts',(9.98426693399994,11.6,3.25819398599998));
#199718=CARTESIAN_POINT('Ctrl Pts',(9.98578884999995,15.2,3.25901328099999));
#199719=CARTESIAN_POINT('Ctrl Pts',(9.98578884999995,11.6,3.25901328099999));
#199720=CARTESIAN_POINT('Ctrl Pts',(9.98731668699994,15.2,3.25983759099999));
#199721=CARTESIAN_POINT('Ctrl Pts',(9.98731668699994,11.6,3.25983759099999));
#199722=CARTESIAN_POINT('Ctrl Pts',(9.98885042199994,15.2,3.26066691799999));
#199723=CARTESIAN_POINT('Ctrl Pts',(9.98885042199994,11.6,3.26066691799999));
#199724=CARTESIAN_POINT('Ctrl Pts',(9.99039003499995,15.2,3.26150126599998));
#199725=CARTESIAN_POINT('Ctrl Pts',(9.99039003499995,11.6,3.26150126599998));
#199726=CARTESIAN_POINT('Ctrl Pts',(9.99193550399994,15.2,3.26234063799999));
#199727=CARTESIAN_POINT('Ctrl Pts',(9.99193550399994,11.6,3.26234063799998));
#199728=CARTESIAN_POINT('Ctrl Pts',(9.99348680799995,15.2,3.26318503599998));
#199729=CARTESIAN_POINT('Ctrl Pts',(9.99348680799995,11.6,3.26318503599998));
#199730=CARTESIAN_POINT('Ctrl Pts',(9.99504392599994,15.2,3.26403446499998));
#199731=CARTESIAN_POINT('Ctrl Pts',(9.99504392599994,11.6,3.26403446499998));
#199732=CARTESIAN_POINT('Ctrl Pts',(9.99660683599994,15.2,3.26488892599999));
#199733=CARTESIAN_POINT('Ctrl Pts',(9.99660683599994,11.6,3.26488892599999));
#199734=CARTESIAN_POINT('Ctrl Pts',(9.99817551899995,15.2,3.26574842299999));
#199735=CARTESIAN_POINT('Ctrl Pts',(9.99817551899995,11.6,3.26574842299999));
#199736=CARTESIAN_POINT('Ctrl Pts',(9.99974995099995,15.2,3.26661295799998));
#199737=CARTESIAN_POINT('Ctrl Pts',(9.99974995099995,11.6,3.26661295799998));
#199738=CARTESIAN_POINT('Ctrl Pts',(10.0013301129999,15.2,3.26748253399998));
#199739=CARTESIAN_POINT('Ctrl Pts',(10.0013301129999,11.6,3.26748253399998));
#199740=CARTESIAN_POINT('Ctrl Pts',(10.0029159849999,15.2,3.26835715499998));
#199741=CARTESIAN_POINT('Ctrl Pts',(10.0029159849999,11.6,3.26835715499998));
#199742=CARTESIAN_POINT('Ctrl Pts',(10.0045075449999,15.2,3.26923682199999));
#199743=CARTESIAN_POINT('Ctrl Pts',(10.0045075449999,11.6,3.26923682199999));
#199744=CARTESIAN_POINT('Ctrl Pts',(10.0061047719999,15.2,3.27012153799998));
#199745=CARTESIAN_POINT('Ctrl Pts',(10.0061047719999,11.6,3.27012153799998));
#199746=CARTESIAN_POINT('Ctrl Pts',(10.0077076459999,15.2,3.27101130699998));
#199747=CARTESIAN_POINT('Ctrl Pts',(10.0077076459999,11.6,3.27101130699998));
#199748=CARTESIAN_POINT('Ctrl Pts',(10.0093161469999,15.2,3.27190612999999));
#199749=CARTESIAN_POINT('Ctrl Pts',(10.0093161469999,11.6,3.27190612999999));
#199750=CARTESIAN_POINT('Ctrl Pts',(10.0109302539999,15.2,3.27280601199998));
#199751=CARTESIAN_POINT('Ctrl Pts',(10.0109302539999,11.6,3.27280601199998));
#199752=CARTESIAN_POINT('Ctrl Pts',(10.0125499459999,15.2,3.27371095399998));
#199753=CARTESIAN_POINT('Ctrl Pts',(10.0125499459999,11.6,3.27371095399998));
#199754=CARTESIAN_POINT('Ctrl Pts',(10.0141752039999,15.2,3.27462095899998));
#199755=CARTESIAN_POINT('Ctrl Pts',(10.0141752039999,11.6,3.27462095899998));
#199756=CARTESIAN_POINT('Ctrl Pts',(10.0158060069999,15.2,3.27553602899999));
#199757=CARTESIAN_POINT('Ctrl Pts',(10.0158060069999,11.6,3.27553602899999));
#199758=CARTESIAN_POINT('Ctrl Pts',(10.0174423339999,15.2,3.27645616799998));
#199759=CARTESIAN_POINT('Ctrl Pts',(10.0174423339999,11.6,3.27645616799998));
#199760=CARTESIAN_POINT('Ctrl Pts',(10.0190841679999,15.2,3.27738137699999));
#199761=CARTESIAN_POINT('Ctrl Pts',(10.0190841679999,11.6,3.27738137699999));
#199762=CARTESIAN_POINT('Ctrl Pts',(10.0207314849999,15.2,3.27831165999999));
#199763=CARTESIAN_POINT('Ctrl Pts',(10.0207314849999,11.6,3.27831165999999));
#199764=CARTESIAN_POINT('Ctrl Pts',(10.0223842669999,15.2,3.27924701899998));
#199765=CARTESIAN_POINT('Ctrl Pts',(10.0223842669999,11.6,3.27924701899998));
#199766=CARTESIAN_POINT('Ctrl Pts',(10.0240424949999,15.2,3.28018745599999));
#199767=CARTESIAN_POINT('Ctrl Pts',(10.0240424949999,11.6,3.28018745599999));
#199768=CARTESIAN_POINT('Ctrl Pts',(10.0257061469999,15.2,3.28113297399998));
#199769=CARTESIAN_POINT('Ctrl Pts',(10.0257061469999,11.6,3.28113297399998));
#199770=CARTESIAN_POINT('Ctrl Pts',(10.0273752059999,15.2,3.28208357499998));
#199771=CARTESIAN_POINT('Ctrl Pts',(10.0273752059999,11.6,3.28208357499998));
#199772=CARTESIAN_POINT('Ctrl Pts',(10.0290496499999,15.2,3.28303926299998));
#199773=CARTESIAN_POINT('Ctrl Pts',(10.0290496499999,11.6,3.28303926299998));
#199774=CARTESIAN_POINT('Ctrl Pts',(10.0307294589999,15.2,3.28400003799998));
#199775=CARTESIAN_POINT('Ctrl Pts',(10.0307294589999,11.6,3.28400003799998));
#199776=CARTESIAN_POINT('Ctrl Pts',(10.0324146159999,15.2,3.28496590599999));
#199777=CARTESIAN_POINT('Ctrl Pts',(10.0324146159999,11.6,3.28496590599999));
#199778=CARTESIAN_POINT('Ctrl Pts',(10.0341050999999,15.2,3.28593686499998));
#199779=CARTESIAN_POINT('Ctrl Pts',(10.0341050999999,11.6,3.28593686499998));
#199780=CARTESIAN_POINT('Ctrl Pts',(10.0358008909999,15.2,3.28691291999998));
#199781=CARTESIAN_POINT('Ctrl Pts',(10.0358008909999,11.6,3.28691291999998));
#199782=CARTESIAN_POINT('Ctrl Pts',(10.0375019699999,15.2,3.28789407399999));
#199783=CARTESIAN_POINT('Ctrl Pts',(10.0375019699999,11.6,3.28789407399999));
#199784=CARTESIAN_POINT('Ctrl Pts',(10.0392083189999,15.2,3.28888032699999));
#199785=CARTESIAN_POINT('Ctrl Pts',(10.0392083189999,11.6,3.28888032699999));
#199786=CARTESIAN_POINT('Ctrl Pts',(10.0409199179999,15.2,3.28987168299999));
#199787=CARTESIAN_POINT('Ctrl Pts',(10.0409199179999,11.6,3.28987168299999));
#199788=CARTESIAN_POINT('Ctrl Pts',(10.0426367469999,15.2,3.29086814299998));
#199789=CARTESIAN_POINT('Ctrl Pts',(10.0426367469999,11.6,3.29086814299998));
#199790=CARTESIAN_POINT('Ctrl Pts',(10.0443587869999,15.2,3.29186971099999));
#199791=CARTESIAN_POINT('Ctrl Pts',(10.0443587869999,11.6,3.29186971099999));
#199792=CARTESIAN_POINT('Ctrl Pts',(10.0460860199999,15.2,3.29287638799999));
#199793=CARTESIAN_POINT('Ctrl Pts',(10.0460860199999,11.6,3.29287638799999));
#199794=CARTESIAN_POINT('Ctrl Pts',(10.0478184259999,15.2,3.29388817699999));
#199795=CARTESIAN_POINT('Ctrl Pts',(10.0478184259999,11.6,3.29388817699999));
#199796=CARTESIAN_POINT('Ctrl Pts',(10.0495559859999,15.2,3.29490507899998));
#199797=CARTESIAN_POINT('Ctrl Pts',(10.0495559859999,11.6,3.29490507899998));
#199798=CARTESIAN_POINT('Ctrl Pts',(10.0512986829999,15.2,3.29592709799999));
#199799=CARTESIAN_POINT('Ctrl Pts',(10.0512986829999,11.6,3.29592709799999));
#199800=CARTESIAN_POINT('Ctrl Pts',(10.0530464969999,15.2,3.29695423399999));
#199801=CARTESIAN_POINT('Ctrl Pts',(10.0530464969999,11.6,3.29695423399999));
#199802=CARTESIAN_POINT('Ctrl Pts',(10.0547994079999,15.2,3.29798649099998));
#199803=CARTESIAN_POINT('Ctrl Pts',(10.0547994079999,11.6,3.29798649099998));
#199804=CARTESIAN_POINT('Ctrl Pts',(10.0565573989999,15.2,3.29902387099998));
#199805=CARTESIAN_POINT('Ctrl Pts',(10.0565573989999,11.6,3.29902387099998));
#199806=CARTESIAN_POINT('Ctrl Pts',(10.0583204519999,15.2,3.30006637499999));
#199807=CARTESIAN_POINT('Ctrl Pts',(10.0583204519999,11.6,3.30006637499999));
#199808=CARTESIAN_POINT('Ctrl Pts',(10.0600885459999,15.2,3.30111400599999));
#199809=CARTESIAN_POINT('Ctrl Pts',(10.0600885459999,11.6,3.30111400599999));
#199810=CARTESIAN_POINT('Ctrl Pts',(10.0618616649999,15.2,3.30216676499998));
#199811=CARTESIAN_POINT('Ctrl Pts',(10.0618616649999,11.6,3.30216676499998));
#199812=CARTESIAN_POINT('Ctrl Pts',(10.0636397889999,15.2,3.30322465599998));
#199813=CARTESIAN_POINT('Ctrl Pts',(10.0636397889999,11.6,3.30322465599998));
#199814=CARTESIAN_POINT('Ctrl Pts',(10.0654228989999,15.2,3.30428767999998));
#199815=CARTESIAN_POINT('Ctrl Pts',(10.0654228989999,11.6,3.30428767999998));
#199816=CARTESIAN_POINT('Ctrl Pts',(10.0672109789999,15.2,3.30535583799998));
#199817=CARTESIAN_POINT('Ctrl Pts',(10.0672109789999,11.6,3.30535583799998));
#199818=CARTESIAN_POINT('Ctrl Pts',(10.0690040089999,15.2,3.30642913399998));
#199819=CARTESIAN_POINT('Ctrl Pts',(10.0690040089999,11.6,3.30642913399998));
#199820=CARTESIAN_POINT('Ctrl Pts',(10.0708019709999,15.2,3.30750756799999));
#199821=CARTESIAN_POINT('Ctrl Pts',(10.0708019709999,11.6,3.30750756799999));
#199822=CARTESIAN_POINT('Ctrl Pts',(10.0726048469999,15.2,3.30859114399999));
#199823=CARTESIAN_POINT('Ctrl Pts',(10.0726048469999,11.6,3.30859114399999));
#199824=CARTESIAN_POINT('Ctrl Pts',(10.0744126189999,15.2,3.30967986199998));
#199825=CARTESIAN_POINT('Ctrl Pts',(10.0744126189999,11.6,3.30967986199998));
#199826=CARTESIAN_POINT('Ctrl Pts',(10.0762252689999,15.2,3.31077372499998));
#199827=CARTESIAN_POINT('Ctrl Pts',(10.0762252689999,11.6,3.31077372499998));
#199828=CARTESIAN_POINT('Ctrl Pts',(10.0780427799999,15.2,3.31187273499999));
#199829=CARTESIAN_POINT('Ctrl Pts',(10.0780427799999,11.6,3.31187273499999));
#199830=CARTESIAN_POINT('Ctrl Pts',(10.0798651319999,15.2,3.31297689299999));
#199831=CARTESIAN_POINT('Ctrl Pts',(10.0798651319999,11.6,3.31297689299999));
#199832=CARTESIAN_POINT('Ctrl Pts',(10.0816923089999,15.2,3.31408620199999));
#199833=CARTESIAN_POINT('Ctrl Pts',(10.0816923089999,11.6,3.31408620199999));
#199834=CARTESIAN_POINT('Ctrl Pts',(10.0835242919999,15.2,3.31520066399998));
#199835=CARTESIAN_POINT('Ctrl Pts',(10.0835242919999,11.6,3.31520066399998));
#199836=CARTESIAN_POINT('Ctrl Pts',(10.0853610639999,15.2,3.31632027999999));
#199837=CARTESIAN_POINT('Ctrl Pts',(10.0853610639999,11.6,3.31632027999999));
#199838=CARTESIAN_POINT('Ctrl Pts',(10.0872026069999,15.2,3.31744505199998));
#199839=CARTESIAN_POINT('Ctrl Pts',(10.0872026069999,11.6,3.31744505199998));
#199840=CARTESIAN_POINT('Ctrl Pts',(10.0890489029999,15.2,3.31857498099998));
#199841=CARTESIAN_POINT('Ctrl Pts',(10.0890489029999,11.6,3.31857498099998));
#199842=CARTESIAN_POINT('Ctrl Pts',(10.0908999359999,15.2,3.31971007099998));
#199843=CARTESIAN_POINT('Ctrl Pts',(10.0908999359999,11.6,3.31971007099998));
#199844=CARTESIAN_POINT('Ctrl Pts',(10.0927556859999,15.2,3.32085032099998));
#199845=CARTESIAN_POINT('Ctrl Pts',(10.0927556859999,11.6,3.32085032099998));
#199846=CARTESIAN_POINT('Ctrl Pts',(10.0946161369999,15.2,3.32199573599999));
#199847=CARTESIAN_POINT('Ctrl Pts',(10.0946161369999,11.6,3.32199573599999));
#199848=CARTESIAN_POINT('Ctrl Pts',(10.0964812719999,15.2,3.32314631499998));
#199849=CARTESIAN_POINT('Ctrl Pts',(10.0964812719999,11.6,3.32314631499998));
#199850=CARTESIAN_POINT('Ctrl Pts',(10.0983510719999,15.2,3.32430206099998));
#199851=CARTESIAN_POINT('Ctrl Pts',(10.0983510719999,11.6,3.32430206099998));
#199852=CARTESIAN_POINT('Ctrl Pts',(10.1002255209999,15.2,3.32546297599999));
#199853=CARTESIAN_POINT('Ctrl Pts',(10.1002255209999,11.6,3.32546297599999));
#199854=CARTESIAN_POINT('Ctrl Pts',(10.1021046009999,15.2,3.32662905999998));
#199855=CARTESIAN_POINT('Ctrl Pts',(10.1021046009999,11.6,3.32662905999998));
#199856=CARTESIAN_POINT('Ctrl Pts',(10.1039882969999,15.2,3.32780031599999));
#199857=CARTESIAN_POINT('Ctrl Pts',(10.1039882969999,11.6,3.32780031599999));
#199858=CARTESIAN_POINT('Ctrl Pts',(10.1058765879999,15.2,3.32897674599998));
#199859=CARTESIAN_POINT('Ctrl Pts',(10.1058765879999,11.6,3.32897674599998));
#199860=CARTESIAN_POINT('Ctrl Pts',(10.1077694589999,15.2,3.33015835099999));
#199861=CARTESIAN_POINT('Ctrl Pts',(10.1077694589999,11.6,3.33015835099999));
#199862=CARTESIAN_POINT('Ctrl Pts',(10.1096668939999,15.2,3.33134513399998));
#199863=CARTESIAN_POINT('Ctrl Pts',(10.1096668939999,11.6,3.33134513399998));
#199864=CARTESIAN_POINT('Ctrl Pts',(10.1115688739999,15.2,3.33253709299999));
#199865=CARTESIAN_POINT('Ctrl Pts',(10.1115688739999,11.6,3.33253709299999));
#199866=CARTESIAN_POINT('Ctrl Pts',(10.1134753829999,15.2,3.33373423299999));
#199867=CARTESIAN_POINT('Ctrl Pts',(10.1134753829999,11.6,3.33373423299999));
#199868=CARTESIAN_POINT('Ctrl Pts',(10.1153864039999,15.2,3.33493655599998));
#199869=CARTESIAN_POINT('Ctrl Pts',(10.1153864039999,11.6,3.33493655599998));
#199870=CARTESIAN_POINT('Ctrl Pts',(10.1173019199999,15.2,3.33614405999998));
#199871=CARTESIAN_POINT('Ctrl Pts',(10.1173019199999,11.6,3.33614405999998));
#199872=CARTESIAN_POINT('Ctrl Pts',(10.1192219139999,15.2,3.33735674999998));
#199873=CARTESIAN_POINT('Ctrl Pts',(10.1192219139999,11.6,3.33735674999998));
#199874=CARTESIAN_POINT('Ctrl Pts',(10.1211463699999,15.2,3.33857462599998));
#199875=CARTESIAN_POINT('Ctrl Pts',(10.1211463699999,11.6,3.33857462599998));
#199876=CARTESIAN_POINT('Ctrl Pts',(10.1230752719999,15.2,3.33979768899999));
#199877=CARTESIAN_POINT('Ctrl Pts',(10.1230752719999,11.6,3.33979768899999));
#199878=CARTESIAN_POINT('Ctrl Pts',(10.1250086009999,15.2,3.34102594199998));
#199879=CARTESIAN_POINT('Ctrl Pts',(10.1250086009999,11.6,3.34102594199998));
#199880=CARTESIAN_POINT('Ctrl Pts',(10.1269463409999,15.2,3.34225938499999));
#199881=CARTESIAN_POINT('Ctrl Pts',(10.1269463409999,11.6,3.34225938499999));
#199882=CARTESIAN_POINT('Ctrl Pts',(10.1288884769999,15.2,3.34349802099998));
#199883=CARTESIAN_POINT('Ctrl Pts',(10.1288884769999,11.6,3.34349802099998));
#199884=CARTESIAN_POINT('Ctrl Pts',(10.1308349909999,15.2,3.34474184999999));
#199885=CARTESIAN_POINT('Ctrl Pts',(10.1308349909999,11.6,3.34474184999999));
#199886=CARTESIAN_POINT('Ctrl Pts',(10.1327858669999,15.2,3.34599087499999));
#199887=CARTESIAN_POINT('Ctrl Pts',(10.1327858669999,11.6,3.34599087499999));
#199888=CARTESIAN_POINT('Ctrl Pts',(10.1347410889999,15.2,3.34724509499999));
#199889=CARTESIAN_POINT('Ctrl Pts',(10.1347410889999,11.6,3.34724509499999));
#199890=CARTESIAN_POINT('Ctrl Pts',(10.1367006399999,15.2,3.34850451399999));
#199891=CARTESIAN_POINT('Ctrl Pts',(10.1367006399999,11.6,3.34850451399999));
#199892=CARTESIAN_POINT('Ctrl Pts',(10.1386645039999,15.2,3.34976913299998));
#199893=CARTESIAN_POINT('Ctrl Pts',(10.1386645039999,11.6,3.34976913299998));
#199894=CARTESIAN_POINT('Ctrl Pts',(10.1406326639999,15.2,3.35103894999998));
#199895=CARTESIAN_POINT('Ctrl Pts',(10.1406326639999,11.6,3.35103894999998));
#199896=CARTESIAN_POINT('Ctrl Pts',(10.1426051049999,15.2,3.35231397199999));
#199897=CARTESIAN_POINT('Ctrl Pts',(10.1426051049999,11.6,3.35231397199998));
#199898=CARTESIAN_POINT('Ctrl Pts',(10.1445818109999,15.2,3.35359419599998));
#199899=CARTESIAN_POINT('Ctrl Pts',(10.1445818109999,11.6,3.35359419599998));
#199900=CARTESIAN_POINT('Ctrl Pts',(10.1465627639999,15.2,3.35487962499998));
#199901=CARTESIAN_POINT('Ctrl Pts',(10.1465627639999,11.6,3.35487962499998));
#199902=CARTESIAN_POINT('Ctrl Pts',(10.1485479489999,15.2,3.35617025999999));
#199903=CARTESIAN_POINT('Ctrl Pts',(10.1485479489999,11.6,3.35617025999999));
#199904=CARTESIAN_POINT('Ctrl Pts',(10.1505373509999,15.2,3.35746610199998));
#199905=CARTESIAN_POINT('Ctrl Pts',(10.1505373509999,11.6,3.35746610199998));
#199906=CARTESIAN_POINT('Ctrl Pts',(10.1525309519999,15.2,3.35876715399999));
#199907=CARTESIAN_POINT('Ctrl Pts',(10.1525309519999,11.6,3.35876715399999));
#199908=CARTESIAN_POINT('Ctrl Pts',(10.1545287359999,15.2,3.36007341499998));
#199909=CARTESIAN_POINT('Ctrl Pts',(10.1545287359999,11.6,3.36007341499998));
#199910=CARTESIAN_POINT('Ctrl Pts',(10.1565306899999,15.2,3.36138488699999));
#199911=CARTESIAN_POINT('Ctrl Pts',(10.1565306899999,11.6,3.36138488699999));
#199912=CARTESIAN_POINT('Ctrl Pts',(10.1585367949999,15.2,3.36270157099998));
#199913=CARTESIAN_POINT('Ctrl Pts',(10.1585367949999,11.6,3.36270157099998));
#199914=CARTESIAN_POINT('Ctrl Pts',(10.1605470379999,15.2,3.36402346999999));
#199915=CARTESIAN_POINT('Ctrl Pts',(10.1605470379999,11.6,3.36402346999999));
#199916=CARTESIAN_POINT('Ctrl Pts',(10.1625613999999,15.2,3.36535058299999));
#199917=CARTESIAN_POINT('Ctrl Pts',(10.1625613999999,11.6,3.36535058299999));
#199918=CARTESIAN_POINT('Ctrl Pts',(10.1645798679999,15.2,3.36668291199998));
#199919=CARTESIAN_POINT('Ctrl Pts',(10.1645798679999,11.6,3.36668291199998));
#199920=CARTESIAN_POINT('Ctrl Pts',(10.1666024249999,15.2,3.36802045899999));
#199921=CARTESIAN_POINT('Ctrl Pts',(10.1666024249999,11.6,3.36802045899999));
#199922=CARTESIAN_POINT('Ctrl Pts',(10.1686290549999,15.2,3.36936322399998));
#199923=CARTESIAN_POINT('Ctrl Pts',(10.1686290549999,11.6,3.36936322399998));
#199924=CARTESIAN_POINT('Ctrl Pts',(10.1706597439999,15.2,3.37071120799998));
#199925=CARTESIAN_POINT('Ctrl Pts',(10.1706597439999,11.6,3.37071120799998));
#199926=CARTESIAN_POINT('Ctrl Pts',(10.1726944739999,15.2,3.37206441399999));
#199927=CARTESIAN_POINT('Ctrl Pts',(10.1726944739999,11.6,3.37206441399999));
#199928=CARTESIAN_POINT('Ctrl Pts',(10.1747332319999,15.2,3.37342283999998));
#199929=CARTESIAN_POINT('Ctrl Pts',(10.1747332319999,11.6,3.37342283999998));
#199930=CARTESIAN_POINT('Ctrl Pts',(10.1767759999999,15.2,3.37478648999999));
#199931=CARTESIAN_POINT('Ctrl Pts',(10.1767759999999,11.6,3.37478648999999));
#199932=CARTESIAN_POINT('Ctrl Pts',(10.1788227659999,15.2,3.37615536499998));
#199933=CARTESIAN_POINT('Ctrl Pts',(10.1788227659999,11.6,3.37615536499998));
#199934=CARTESIAN_POINT('Ctrl Pts',(10.1808735109999,15.2,3.37752946399998));
#199935=CARTESIAN_POINT('Ctrl Pts',(10.1808735109999,11.6,3.37752946399998));
#199936=CARTESIAN_POINT('Ctrl Pts',(10.1829282219999,15.2,3.37890878899999));
#199937=CARTESIAN_POINT('Ctrl Pts',(10.1829282219999,11.6,3.37890878899999));
#199938=CARTESIAN_POINT('Ctrl Pts',(10.1849868839999,15.2,3.38029334299998));
#199939=CARTESIAN_POINT('Ctrl Pts',(10.1849868839999,11.6,3.38029334299998));
#199940=CARTESIAN_POINT('Ctrl Pts',(10.1870494789999,15.2,3.38168312399999));
#199941=CARTESIAN_POINT('Ctrl Pts',(10.1870494789999,11.6,3.38168312399999));
#199942=CARTESIAN_POINT('Ctrl Pts',(10.1891159949999,15.2,3.38307813399998));
#199943=CARTESIAN_POINT('Ctrl Pts',(10.1891159949999,11.6,3.38307813399998));
#199944=CARTESIAN_POINT('Ctrl Pts',(10.1911864149999,15.2,3.38447837499999));
#199945=CARTESIAN_POINT('Ctrl Pts',(10.1911864149999,11.6,3.38447837499999));
#199946=CARTESIAN_POINT('Ctrl Pts',(10.1932607229999,15.2,3.38588384799999));
#199947=CARTESIAN_POINT('Ctrl Pts',(10.1932607229999,11.6,3.38588384799999));
#199948=CARTESIAN_POINT('Ctrl Pts',(10.1953389059999,15.2,3.38729455299998));
#199949=CARTESIAN_POINT('Ctrl Pts',(10.1953389059999,11.6,3.38729455299998));
#199950=CARTESIAN_POINT('Ctrl Pts',(10.1974209479999,15.2,3.38871049099998));
#199951=CARTESIAN_POINT('Ctrl Pts',(10.1974209479999,11.6,3.38871049099998));
#199952=CARTESIAN_POINT('Ctrl Pts',(10.1995068349999,15.2,3.39013166499999));
#199953=CARTESIAN_POINT('Ctrl Pts',(10.1995068349999,11.6,3.39013166499999));
#199954=CARTESIAN_POINT('Ctrl Pts',(10.2015965499999,15.2,3.39155807199998));
#199955=CARTESIAN_POINT('Ctrl Pts',(10.2015965499999,11.6,3.39155807199998));
#199956=CARTESIAN_POINT('Ctrl Pts',(10.2036900789999,15.2,3.39298971699999));
#199957=CARTESIAN_POINT('Ctrl Pts',(10.2036900789999,11.6,3.39298971699999));
#199958=CARTESIAN_POINT('Ctrl Pts',(10.2057874069999,15.2,3.39442659799998));
#199959=CARTESIAN_POINT('Ctrl Pts',(10.2057874069999,11.6,3.39442659799998));
#199960=CARTESIAN_POINT('Ctrl Pts',(10.2078885199999,15.2,3.39586871799998));
#199961=CARTESIAN_POINT('Ctrl Pts',(10.2078885199999,11.6,3.39586871799998));
#199962=CARTESIAN_POINT('Ctrl Pts',(10.2099934029999,15.2,3.39731607599998));
#199963=CARTESIAN_POINT('Ctrl Pts',(10.2099934029999,11.6,3.39731607599998));
#199964=CARTESIAN_POINT('Ctrl Pts',(10.2121020399999,15.2,3.39876867499999));
#199965=CARTESIAN_POINT('Ctrl Pts',(10.2121020399999,11.6,3.39876867499999));
#199966=CARTESIAN_POINT('Ctrl Pts',(10.2142144169999,15.2,3.40022651399998));
#199967=CARTESIAN_POINT('Ctrl Pts',(10.2142144169999,11.6,3.40022651399998));
#199968=CARTESIAN_POINT('Ctrl Pts',(10.2163305199999,15.2,3.40168959499999));
#199969=CARTESIAN_POINT('Ctrl Pts',(10.2163305199999,11.6,3.40168959499999));
#199970=CARTESIAN_POINT('Ctrl Pts',(10.2184503329999,15.2,3.40315791799998));
#199971=CARTESIAN_POINT('Ctrl Pts',(10.2184503329999,11.6,3.40315791799998));
#199972=CARTESIAN_POINT('Ctrl Pts',(10.2205738429999,15.2,3.40463148499998));
#199973=CARTESIAN_POINT('Ctrl Pts',(10.2205738429999,11.6,3.40463148499998));
#199974=CARTESIAN_POINT('Ctrl Pts',(10.2227010339999,15.2,3.40611029599999));
#199975=CARTESIAN_POINT('Ctrl Pts',(10.2227010339999,11.6,3.40611029599999));
#199976=CARTESIAN_POINT('Ctrl Pts',(10.2248318919999,15.2,3.40759435099999));
#199977=CARTESIAN_POINT('Ctrl Pts',(10.2248318919999,11.6,3.40759435099999));
#199978=CARTESIAN_POINT('Ctrl Pts',(10.2269664019999,15.2,3.40908365299998));
#199979=CARTESIAN_POINT('Ctrl Pts',(10.2269664019999,11.6,3.40908365299998));
#199980=CARTESIAN_POINT('Ctrl Pts',(10.2291045509999,15.2,3.41057820099999));
#199981=CARTESIAN_POINT('Ctrl Pts',(10.2291045509999,11.6,3.41057820099999));
#199982=CARTESIAN_POINT('Ctrl Pts',(10.2312463229999,15.2,3.41207799699998));
#199983=CARTESIAN_POINT('Ctrl Pts',(10.2312463229999,11.6,3.41207799699998));
#199984=CARTESIAN_POINT('Ctrl Pts',(10.2333917049999,15.2,3.41358303999999));
#199985=CARTESIAN_POINT('Ctrl Pts',(10.2333917049999,11.6,3.41358303999999));
#199986=CARTESIAN_POINT('Ctrl Pts',(10.2355406799999,15.2,3.41509333299998));
#199987=CARTESIAN_POINT('Ctrl Pts',(10.2355406799999,11.6,3.41509333299998));
#199988=CARTESIAN_POINT('Ctrl Pts',(10.2376932379999,15.2,3.41660887399998));
#199989=CARTESIAN_POINT('Ctrl Pts',(10.2376932379999,11.6,3.41660887399998));
#199990=CARTESIAN_POINT('Ctrl Pts',(10.2398493599999,15.2,3.41812966599999));
#199991=CARTESIAN_POINT('Ctrl Pts',(10.2398493599999,11.6,3.41812966599999));
#199992=CARTESIAN_POINT('Ctrl Pts',(10.2420090349999,15.2,3.41965570899998));
#199993=CARTESIAN_POINT('Ctrl Pts',(10.2420090349999,11.6,3.41965570899998));
#199994=CARTESIAN_POINT('Ctrl Pts',(10.2441722479999,15.2,3.42118700399999));
#199995=CARTESIAN_POINT('Ctrl Pts',(10.2441722479999,11.6,3.42118700399999));
#199996=CARTESIAN_POINT('Ctrl Pts',(10.2463389839999,15.2,3.42272355099999));
#199997=CARTESIAN_POINT('Ctrl Pts',(10.2463389839999,11.6,3.42272355099999));
#199998=CARTESIAN_POINT('Ctrl Pts',(10.2485092299999,15.2,3.42426535099998));
#199999=CARTESIAN_POINT('Ctrl Pts',(10.2485092299999,11.6,3.42426535099998));
#200000=CARTESIAN_POINT('Ctrl Pts',(10.2506829709999,15.2,3.42581240499998));
#200001=CARTESIAN_POINT('Ctrl Pts',(10.2506829709999,11.6,3.42581240499998));
#200002=CARTESIAN_POINT('Ctrl Pts',(10.2528601939999,15.2,3.42736471399999));
#200003=CARTESIAN_POINT('Ctrl Pts',(10.2528601939999,11.6,3.42736471399998));
#200004=CARTESIAN_POINT('Ctrl Pts',(10.2550408839999,15.2,3.42892227699998));
#200005=CARTESIAN_POINT('Ctrl Pts',(10.2550408839999,11.6,3.42892227699998));
#200006=CARTESIAN_POINT('Ctrl Pts',(10.2572250269999,15.2,3.43048509599999));
#200007=CARTESIAN_POINT('Ctrl Pts',(10.2572250269999,11.6,3.43048509599999));
#200008=CARTESIAN_POINT('Ctrl Pts',(10.2594126089999,15.2,3.43205317199998));
#200009=CARTESIAN_POINT('Ctrl Pts',(10.2594126089999,11.6,3.43205317199998));
#200010=CARTESIAN_POINT('Ctrl Pts',(10.2616036169999,15.2,3.43362650399998));
#200011=CARTESIAN_POINT('Ctrl Pts',(10.2616036169999,11.6,3.43362650399998));
#200012=CARTESIAN_POINT('Ctrl Pts',(10.2637980359999,15.2,3.43520509299999));
#200013=CARTESIAN_POINT('Ctrl Pts',(10.2637980359999,11.6,3.43520509299999));
#200014=CARTESIAN_POINT('Ctrl Pts',(10.2659958539999,15.2,3.43678894099998));
#200015=CARTESIAN_POINT('Ctrl Pts',(10.2659958539999,11.6,3.43678894099998));
#200016=CARTESIAN_POINT('Ctrl Pts',(10.2681970539999,15.2,3.43837804599998));
#200017=CARTESIAN_POINT('Ctrl Pts',(10.2681970539999,11.6,3.43837804599998));
#200018=CARTESIAN_POINT('Ctrl Pts',(10.2704016259999,15.2,3.43997241199999));
#200019=CARTESIAN_POINT('Ctrl Pts',(10.2704016259999,11.6,3.43997241199998));
#200020=CARTESIAN_POINT('Ctrl Pts',(10.2726095529999,15.2,3.44157203699999));
#200021=CARTESIAN_POINT('Ctrl Pts',(10.2726095529999,11.6,3.44157203699999));
#200022=CARTESIAN_POINT('Ctrl Pts',(10.2748208229999,15.2,3.44317692199999));
#200023=CARTESIAN_POINT('Ctrl Pts',(10.2748208229999,11.6,3.44317692199999));
#200024=CARTESIAN_POINT('Ctrl Pts',(10.2770354219999,15.2,3.44478706899999));
#200025=CARTESIAN_POINT('Ctrl Pts',(10.2770354219999,11.6,3.44478706899999));
#200026=CARTESIAN_POINT('Ctrl Pts',(10.2792533369999,15.2,3.44640247699999));
#200027=CARTESIAN_POINT('Ctrl Pts',(10.2792533369999,11.6,3.44640247699999));
#200028=CARTESIAN_POINT('Ctrl Pts',(10.2814745529999,15.2,3.44802314599999));
#200029=CARTESIAN_POINT('Ctrl Pts',(10.2814745529999,11.6,3.44802314599999));
#200030=CARTESIAN_POINT('Ctrl Pts',(10.2836990579999,15.2,3.44964907699998));
#200031=CARTESIAN_POINT('Ctrl Pts',(10.2836990579999,11.6,3.44964907699998));
#200032=CARTESIAN_POINT('Ctrl Pts',(10.2859268359999,15.2,3.45128027099998));
#200033=CARTESIAN_POINT('Ctrl Pts',(10.2859268359999,11.6,3.45128027099998));
#200034=CARTESIAN_POINT('Ctrl Pts',(10.2881578759999,15.2,3.45291672899998));
#200035=CARTESIAN_POINT('Ctrl Pts',(10.2881578759999,11.6,3.45291672899998));
#200036=CARTESIAN_POINT('Ctrl Pts',(10.2903921639999,15.2,3.45455845099998));
#200037=CARTESIAN_POINT('Ctrl Pts',(10.2903921639999,11.6,3.45455845099998));
#200038=CARTESIAN_POINT('Ctrl Pts',(10.2926296859999,15.2,3.45620543599999));
#200039=CARTESIAN_POINT('Ctrl Pts',(10.2926296859999,11.6,3.45620543599999));
#200040=CARTESIAN_POINT('Ctrl Pts',(10.2948704289999,15.2,3.45785768599999));
#200041=CARTESIAN_POINT('Ctrl Pts',(10.2948704289999,11.6,3.45785768599998));
#200042=CARTESIAN_POINT('Ctrl Pts',(10.2971143779999,15.2,3.45951520099998));
#200043=CARTESIAN_POINT('Ctrl Pts',(10.2971143779999,11.6,3.45951520099998));
#200044=CARTESIAN_POINT('Ctrl Pts',(10.2993615219999,15.2,3.46117798099999));
#200045=CARTESIAN_POINT('Ctrl Pts',(10.2993615219999,11.6,3.46117798099998));
#200046=CARTESIAN_POINT('Ctrl Pts',(10.3016118469999,15.2,3.46284602699999));
#200047=CARTESIAN_POINT('Ctrl Pts',(10.3016118469999,11.6,3.46284602699999));
#200048=CARTESIAN_POINT('Ctrl Pts',(10.3038653379999,15.2,3.46451933999998));
#200049=CARTESIAN_POINT('Ctrl Pts',(10.3038653379999,11.6,3.46451933999998));
#200050=CARTESIAN_POINT('Ctrl Pts',(10.3061219849999,15.2,3.46619791899998));
#200051=CARTESIAN_POINT('Ctrl Pts',(10.3061219849999,11.6,3.46619791899998));
#200052=CARTESIAN_POINT('Ctrl Pts',(10.3083817719999,15.2,3.46788176399999));
#200053=CARTESIAN_POINT('Ctrl Pts',(10.3083817719999,11.6,3.46788176399999));
#200054=CARTESIAN_POINT('Ctrl Pts',(10.3106446869999,15.2,3.46957087799999));
#200055=CARTESIAN_POINT('Ctrl Pts',(10.3106446869999,11.6,3.46957087799999));
#200056=CARTESIAN_POINT('Ctrl Pts',(10.3129107159999,15.2,3.47126525799998));
#200057=CARTESIAN_POINT('Ctrl Pts',(10.3129107159999,11.6,3.47126525799998));
#200058=CARTESIAN_POINT('Ctrl Pts',(10.3151798469999,15.2,3.47296490699998));
#200059=CARTESIAN_POINT('Ctrl Pts',(10.3151798469999,11.6,3.47296490699998));
#200060=CARTESIAN_POINT('Ctrl Pts',(10.3174520669999,15.2,3.47466982499999));
#200061=CARTESIAN_POINT('Ctrl Pts',(10.3174520669999,11.6,3.47466982499998));
#200062=CARTESIAN_POINT('Ctrl Pts',(10.3197273619999,15.2,3.47638000999999));
#200063=CARTESIAN_POINT('Ctrl Pts',(10.3197273619999,11.6,3.47638000999999));
#200064=CARTESIAN_POINT('Ctrl Pts',(10.3220057189999,15.2,3.47809546499998));
#200065=CARTESIAN_POINT('Ctrl Pts',(10.3220057189999,11.6,3.47809546499998));
#200066=CARTESIAN_POINT('Ctrl Pts',(10.3242871249999,15.2,3.47981618899999));
#200067=CARTESIAN_POINT('Ctrl Pts',(10.3242871249999,11.6,3.47981618899999));
#200068=CARTESIAN_POINT('Ctrl Pts',(10.3265715679999,15.2,3.48154218199999));
#200069=CARTESIAN_POINT('Ctrl Pts',(10.3265715679999,11.6,3.48154218199999));
#200070=CARTESIAN_POINT('Ctrl Pts',(10.3288590349999,15.2,3.48327344499998));
#200071=CARTESIAN_POINT('Ctrl Pts',(10.3288590349999,11.6,3.48327344499998));
#200072=CARTESIAN_POINT('Ctrl Pts',(10.3311495119999,15.2,3.48500997899999));
#200073=CARTESIAN_POINT('Ctrl Pts',(10.3311495119999,11.6,3.48500997899999));
#200074=CARTESIAN_POINT('Ctrl Pts',(10.3334429859999,15.2,3.48675178299998));
#200075=CARTESIAN_POINT('Ctrl Pts',(10.3334429859999,11.6,3.48675178299998));
#200076=CARTESIAN_POINT('Ctrl Pts',(10.3357394449999,15.2,3.48849885599999));
#200077=CARTESIAN_POINT('Ctrl Pts',(10.3357394449999,11.6,3.48849885599999));
#200078=CARTESIAN_POINT('Ctrl Pts',(10.3380388769999,15.2,3.49025120199999));
#200079=CARTESIAN_POINT('Ctrl Pts',(10.3380388769999,11.6,3.49025120199998));
#200080=CARTESIAN_POINT('Ctrl Pts',(10.3403412679999,15.2,3.49200881799998));
#200081=CARTESIAN_POINT('Ctrl Pts',(10.3403412679999,11.6,3.49200881799998));
#200082=CARTESIAN_POINT('Ctrl Pts',(10.3426466049999,15.2,3.49377170499999));
#200083=CARTESIAN_POINT('Ctrl Pts',(10.3426466049999,11.6,3.49377170499999));
#200084=CARTESIAN_POINT('Ctrl Pts',(10.3449548749999,15.2,3.49553986399999));
#200085=CARTESIAN_POINT('Ctrl Pts',(10.3449548749999,11.6,3.49553986399999));
#200086=CARTESIAN_POINT('Ctrl Pts',(10.3472660669999,15.2,3.49731329399999));
#200087=CARTESIAN_POINT('Ctrl Pts',(10.3472660669999,11.6,3.49731329399999));
#200088=CARTESIAN_POINT('Ctrl Pts',(10.3495801669999,15.2,3.49909199599999));
#200089=CARTESIAN_POINT('Ctrl Pts',(10.3495801669999,11.6,3.49909199599999));
#200090=CARTESIAN_POINT('Ctrl Pts',(10.3518971629999,15.2,3.50087596999998));
#200091=CARTESIAN_POINT('Ctrl Pts',(10.3518971629999,11.6,3.50087596999998));
#200092=CARTESIAN_POINT('Ctrl Pts',(10.3542170419999,15.2,3.50266521699999));
#200093=CARTESIAN_POINT('Ctrl Pts',(10.3542170419999,11.6,3.50266521699999));
#200094=CARTESIAN_POINT('Ctrl Pts',(10.3565397919999,15.2,3.50445973499999));
#200095=CARTESIAN_POINT('Ctrl Pts',(10.3565397919999,11.6,3.50445973499998));
#200096=CARTESIAN_POINT('Ctrl Pts',(10.3588653989999,15.2,3.50625952599999));
#200097=CARTESIAN_POINT('Ctrl Pts',(10.3588653989999,11.6,3.50625952599999));
#200098=CARTESIAN_POINT('Ctrl Pts',(10.3611938519999,15.2,3.50806458899999));
#200099=CARTESIAN_POINT('Ctrl Pts',(10.3611938519999,11.6,3.50806458899999));
#200100=CARTESIAN_POINT('Ctrl Pts',(10.3635251379999,15.2,3.50987492599998));
#200101=CARTESIAN_POINT('Ctrl Pts',(10.3635251379999,11.6,3.50987492599998));
#200102=CARTESIAN_POINT('Ctrl Pts',(10.3658592459999,15.2,3.51169053399998));
#200103=CARTESIAN_POINT('Ctrl Pts',(10.3658592459999,11.6,3.51169053399998));
#200104=CARTESIAN_POINT('Ctrl Pts',(10.3681961589999,15.2,3.51351141599999));
#200105=CARTESIAN_POINT('Ctrl Pts',(10.3681961589999,11.6,3.51351141599999));
#200106=CARTESIAN_POINT('Ctrl Pts',(10.3705358699999,15.2,3.51533757099999));
#200107=CARTESIAN_POINT('Ctrl Pts',(10.3705358699999,11.6,3.51533757099999));
#200108=CARTESIAN_POINT('Ctrl Pts',(10.3728783639999,15.2,3.51716899899999));
#200109=CARTESIAN_POINT('Ctrl Pts',(10.3728783639999,11.6,3.51716899899999));
#200110=CARTESIAN_POINT('Ctrl Pts',(10.3752236289999,15.2,3.51900569999999));
#200111=CARTESIAN_POINT('Ctrl Pts',(10.3752236289999,11.6,3.51900569999999));
#200112=CARTESIAN_POINT('Ctrl Pts',(10.3775716529999,15.2,3.52084767399998));
#200113=CARTESIAN_POINT('Ctrl Pts',(10.3775716529999,11.6,3.52084767399998));
#200114=CARTESIAN_POINT('Ctrl Pts',(10.3799224219999,15.2,3.52269492299998));
#200115=CARTESIAN_POINT('Ctrl Pts',(10.3799224219999,11.6,3.52269492299998));
#200116=CARTESIAN_POINT('Ctrl Pts',(10.3822759259999,15.2,3.52454744299998));
#200117=CARTESIAN_POINT('Ctrl Pts',(10.3822759259999,11.6,3.52454744299998));
#200118=CARTESIAN_POINT('Ctrl Pts',(10.3846321519999,15.2,3.52640523799998));
#200119=CARTESIAN_POINT('Ctrl Pts',(10.3846321519999,11.6,3.52640523799998));
#200120=CARTESIAN_POINT('Ctrl Pts',(10.3869910869999,15.2,3.52826830499998));
#200121=CARTESIAN_POINT('Ctrl Pts',(10.3869910869999,11.6,3.52826830499998));
#200122=CARTESIAN_POINT('Ctrl Pts',(10.3893527199999,15.2,3.53013664599998));
#200123=CARTESIAN_POINT('Ctrl Pts',(10.3893527199999,11.6,3.53013664599998));
#200124=CARTESIAN_POINT('Ctrl Pts',(10.3917170389999,15.2,3.53201026099998));
#200125=CARTESIAN_POINT('Ctrl Pts',(10.3917170389999,11.6,3.53201026099998));
#200126=CARTESIAN_POINT('Ctrl Pts',(10.3940840299999,15.2,3.53388914899998));
#200127=CARTESIAN_POINT('Ctrl Pts',(10.3940840299999,11.6,3.53388914899998));
#200128=CARTESIAN_POINT('Ctrl Pts',(10.3964536819999,15.2,3.53577330999999));
#200129=CARTESIAN_POINT('Ctrl Pts',(10.3964536819999,11.6,3.53577330999999));
#200130=CARTESIAN_POINT('Ctrl Pts',(10.3988259839999,15.2,3.53766274499999));
#200131=CARTESIAN_POINT('Ctrl Pts',(10.3988259839999,11.6,3.53766274499998));
#200132=CARTESIAN_POINT('Ctrl Pts',(10.4012009229999,15.2,3.53955745299999));
#200133=CARTESIAN_POINT('Ctrl Pts',(10.4012009229999,11.6,3.53955745299999));
#200134=CARTESIAN_POINT('Ctrl Pts',(10.4035784859999,15.2,3.54145743499998));
#200135=CARTESIAN_POINT('Ctrl Pts',(10.4035784859999,11.6,3.54145743499998));
#200136=CARTESIAN_POINT('Ctrl Pts',(10.4059586629999,15.2,3.54336268899999));
#200137=CARTESIAN_POINT('Ctrl Pts',(10.4059586629999,11.6,3.54336268899999));
#200138=CARTESIAN_POINT('Ctrl Pts',(10.4083414399999,15.2,3.54527321699998));
#200139=CARTESIAN_POINT('Ctrl Pts',(10.4083414399999,11.6,3.54527321699998));
#200140=CARTESIAN_POINT('Ctrl Pts',(10.4107268069999,15.2,3.54718901799998));
#200141=CARTESIAN_POINT('Ctrl Pts',(10.4107268069999,11.6,3.54718901799998));
#200142=CARTESIAN_POINT('Ctrl Pts',(10.4131147519999,15.2,3.54911009199999));
#200143=CARTESIAN_POINT('Ctrl Pts',(10.4131147519999,11.6,3.54911009199998));
#200144=CARTESIAN_POINT('Ctrl Pts',(10.4155052599999,15.2,3.55103643999998));
#200145=CARTESIAN_POINT('Ctrl Pts',(10.4155052599999,11.6,3.55103643999998));
#200146=CARTESIAN_POINT('Ctrl Pts',(10.4178983229999,15.2,3.55296805999998));
#200147=CARTESIAN_POINT('Ctrl Pts',(10.4178983229999,11.6,3.55296805999998));
#200148=CARTESIAN_POINT('Ctrl Pts',(10.4202939269999,15.2,3.55490495299998));
#200149=CARTESIAN_POINT('Ctrl Pts',(10.4202939269999,11.6,3.55490495299998));
#200150=CARTESIAN_POINT('Ctrl Pts',(10.4226920599999,15.2,3.55684711799999));
#200151=CARTESIAN_POINT('Ctrl Pts',(10.4226920599999,11.6,3.55684711799999));
#200152=CARTESIAN_POINT('Ctrl Pts',(10.4250927119999,15.2,3.55879455599998));
#200153=CARTESIAN_POINT('Ctrl Pts',(10.4250927119999,11.6,3.55879455599998));
#200154=CARTESIAN_POINT('Ctrl Pts',(10.4274958709999,15.2,3.56074726699998));
#200155=CARTESIAN_POINT('Ctrl Pts',(10.4274958709999,11.6,3.56074726699998));
#200156=CARTESIAN_POINT('Ctrl Pts',(10.4299015229999,15.2,3.56270524999999));
#200157=CARTESIAN_POINT('Ctrl Pts',(10.4299015229999,11.6,3.56270524999999));
#200158=CARTESIAN_POINT('Ctrl Pts',(10.4323096579999,15.2,3.56466850499999));
#200159=CARTESIAN_POINT('Ctrl Pts',(10.4323096579999,11.6,3.56466850499999));
#200160=CARTESIAN_POINT('Ctrl Pts',(10.4347202649999,15.2,3.56663703199998));
#200161=CARTESIAN_POINT('Ctrl Pts',(10.4347202649999,11.6,3.56663703199998));
#200162=CARTESIAN_POINT('Ctrl Pts',(10.4371333319999,15.2,3.56861083099999));
#200163=CARTESIAN_POINT('Ctrl Pts',(10.4371333319999,11.6,3.56861083099999));
#200164=CARTESIAN_POINT('Ctrl Pts',(10.4395488449999,15.2,3.57058990199998));
#200165=CARTESIAN_POINT('Ctrl Pts',(10.4395488449999,11.6,3.57058990199998));
#200166=CARTESIAN_POINT('Ctrl Pts',(10.4419667949999,15.2,3.57257424399998));
#200167=CARTESIAN_POINT('Ctrl Pts',(10.4419667949999,11.6,3.57257424399998));
#200168=CARTESIAN_POINT('Ctrl Pts',(10.4443871699999,15.2,3.57456385699999));
#200169=CARTESIAN_POINT('Ctrl Pts',(10.4443871699999,11.6,3.57456385699999));
#200170=CARTESIAN_POINT('Ctrl Pts',(10.4468099579999,15.2,3.57655874199998));
#200171=CARTESIAN_POINT('Ctrl Pts',(10.4468099579999,11.6,3.57655874199998));
#200172=CARTESIAN_POINT('Ctrl Pts',(10.4492351469999,15.2,3.57855889799998));
#200173=CARTESIAN_POINT('Ctrl Pts',(10.4492351469999,11.6,3.57855889799998));
#200174=CARTESIAN_POINT('Ctrl Pts',(10.4516627269999,15.2,3.58056432399999));
#200175=CARTESIAN_POINT('Ctrl Pts',(10.4516627269999,11.6,3.58056432399999));
#200176=CARTESIAN_POINT('Ctrl Pts',(10.4540926849999,15.2,3.58257501999999));
#200177=CARTESIAN_POINT('Ctrl Pts',(10.4540926849999,11.6,3.58257501999999));
#200178=CARTESIAN_POINT('Ctrl Pts',(10.4565250109999,15.2,3.58459098699999));
#200179=CARTESIAN_POINT('Ctrl Pts',(10.4565250109999,11.6,3.58459098699999));
#200180=CARTESIAN_POINT('Ctrl Pts',(10.4589596909999,15.2,3.58661222399999));
#200181=CARTESIAN_POINT('Ctrl Pts',(10.4589596909999,11.6,3.58661222399998));
#200182=CARTESIAN_POINT('Ctrl Pts',(10.4613967169999,15.2,3.58863873099998));
#200183=CARTESIAN_POINT('Ctrl Pts',(10.4613967169999,11.6,3.58863873099998));
#200184=CARTESIAN_POINT('Ctrl Pts',(10.4638360759999,15.2,3.59067050699998));
#200185=CARTESIAN_POINT('Ctrl Pts',(10.4638360759999,11.6,3.59067050699998));
#200186=CARTESIAN_POINT('Ctrl Pts',(10.4662777559999,15.2,3.59270755199999));
#200187=CARTESIAN_POINT('Ctrl Pts',(10.4662777559999,11.6,3.59270755199999));
#200188=CARTESIAN_POINT('Ctrl Pts',(10.4687217459999,15.2,3.59474986699999));
#200189=CARTESIAN_POINT('Ctrl Pts',(10.4687217459999,11.6,3.59474986699999));
#200190=CARTESIAN_POINT('Ctrl Pts',(10.4711680339999,15.2,3.59679744999998));
#200191=CARTESIAN_POINT('Ctrl Pts',(10.4711680339999,11.6,3.59679744999998));
#200192=CARTESIAN_POINT('Ctrl Pts',(10.4736166109999,15.2,3.59885030099999));
#200193=CARTESIAN_POINT('Ctrl Pts',(10.4736166109999,11.6,3.59885030099999));
#200194=CARTESIAN_POINT('Ctrl Pts',(10.4760674639999,15.2,3.60090842099999));
#200195=CARTESIAN_POINT('Ctrl Pts',(10.4760674639999,11.6,3.60090842099999));
#200196=CARTESIAN_POINT('Ctrl Pts',(10.4785205819999,15.2,3.60297180799999));
#200197=CARTESIAN_POINT('Ctrl Pts',(10.4785205819999,11.6,3.60297180799999));
#200198=CARTESIAN_POINT('Ctrl Pts',(10.4809759539999,15.2,3.60504046299998));
#200199=CARTESIAN_POINT('Ctrl Pts',(10.4809759539999,11.6,3.60504046299998));
#200200=CARTESIAN_POINT('Ctrl Pts',(10.4834335689999,15.2,3.60711438399999));
#200201=CARTESIAN_POINT('Ctrl Pts',(10.4834335689999,11.6,3.60711438399999));
#200202=CARTESIAN_POINT('Ctrl Pts',(10.4858934149999,15.2,3.60919357299998));
#200203=CARTESIAN_POINT('Ctrl Pts',(10.4858934149999,11.6,3.60919357299998));
#200204=CARTESIAN_POINT('Ctrl Pts',(10.4883554829999,15.2,3.61127802799999));
#200205=CARTESIAN_POINT('Ctrl Pts',(10.4883554829999,11.6,3.61127802799999));
#200206=CARTESIAN_POINT('Ctrl Pts',(10.4908197579999,15.2,3.61336774899998));
#200207=CARTESIAN_POINT('Ctrl Pts',(10.4908197579999,11.6,3.61336774899998));
#200208=CARTESIAN_POINT('Ctrl Pts',(10.4932862329999,15.2,3.61546273599998));
#200209=CARTESIAN_POINT('Ctrl Pts',(10.4932862329999,11.6,3.61546273599998));
#200210=CARTESIAN_POINT('Ctrl Pts',(10.4957548949999,15.2,3.61756298899999));
#200211=CARTESIAN_POINT('Ctrl Pts',(10.4957548949999,11.6,3.61756298899999));
#200212=CARTESIAN_POINT('Ctrl Pts',(10.4982257319999,15.2,3.61966850599998));
#200213=CARTESIAN_POINT('Ctrl Pts',(10.4982257319999,11.6,3.61966850599998));
#200214=CARTESIAN_POINT('Ctrl Pts',(10.5006987339999,15.2,3.62177928899998));
#200215=CARTESIAN_POINT('Ctrl Pts',(10.5006987339999,11.6,3.62177928899998));
#200216=CARTESIAN_POINT('Ctrl Pts',(10.5031738909999,15.2,3.62389533499999));
#200217=CARTESIAN_POINT('Ctrl Pts',(10.5031738909999,11.6,3.62389533499999));
#200218=CARTESIAN_POINT('Ctrl Pts',(10.5056511899999,15.2,3.62601664499999));
#200219=CARTESIAN_POINT('Ctrl Pts',(10.5056511899999,11.6,3.62601664499999));
#200220=CARTESIAN_POINT('Ctrl Pts',(10.5081306219999,15.2,3.62814321899998));
#200221=CARTESIAN_POINT('Ctrl Pts',(10.5081306219999,11.6,3.62814321899998));
#200222=CARTESIAN_POINT('Ctrl Pts',(10.5106121749999,15.2,3.63027505599998));
#200223=CARTESIAN_POINT('Ctrl Pts',(10.5106121749999,11.6,3.63027505599998));
#200224=CARTESIAN_POINT('Ctrl Pts',(10.5130958379999,15.2,3.63241215499999));
#200225=CARTESIAN_POINT('Ctrl Pts',(10.5130958379999,11.6,3.63241215499999));
#200226=CARTESIAN_POINT('Ctrl Pts',(10.5155816019999,15.2,3.63455451599999));
#200227=CARTESIAN_POINT('Ctrl Pts',(10.5155816019999,11.6,3.63455451599999));
#200228=CARTESIAN_POINT('Ctrl Pts',(10.5180694529999,15.2,3.63670213999999));
#200229=CARTESIAN_POINT('Ctrl Pts',(10.5180694529999,11.6,3.63670213999999));
#200230=CARTESIAN_POINT('Ctrl Pts',(10.5205593819999,15.2,3.63885502499999));
#200231=CARTESIAN_POINT('Ctrl Pts',(10.5205593819999,11.6,3.63885502499999));
#200232=CARTESIAN_POINT('Ctrl Pts',(10.5230513769999,15.2,3.64101317099998));
#200233=CARTESIAN_POINT('Ctrl Pts',(10.5230513769999,11.6,3.64101317099998));
#200234=CARTESIAN_POINT('Ctrl Pts',(10.5255454289999,15.2,3.64317657699999));
#200235=CARTESIAN_POINT('Ctrl Pts',(10.5255454289999,11.6,3.64317657699999));
#200236=CARTESIAN_POINT('Ctrl Pts',(10.5280415259999,15.2,3.64534524299999));
#200237=CARTESIAN_POINT('Ctrl Pts',(10.5280415259999,11.6,3.64534524299999));
#200238=CARTESIAN_POINT('Ctrl Pts',(10.5305396569999,15.2,3.64751916899999));
#200239=CARTESIAN_POINT('Ctrl Pts',(10.5305396569999,11.6,3.64751916899999));
#200240=CARTESIAN_POINT('Ctrl Pts',(10.5330398119999,15.2,3.64969835299998));
#200241=CARTESIAN_POINT('Ctrl Pts',(10.5330398119999,11.6,3.64969835299998));
#200242=CARTESIAN_POINT('Ctrl Pts',(10.5355419799999,15.2,3.65188279699999));
#200243=CARTESIAN_POINT('Ctrl Pts',(10.5355419799999,11.6,3.65188279699999));
#200244=CARTESIAN_POINT('Ctrl Pts',(10.5380461509999,15.2,3.65407249799999));
#200245=CARTESIAN_POINT('Ctrl Pts',(10.5380461509999,11.6,3.65407249799999));
#200246=CARTESIAN_POINT('Ctrl Pts',(10.5405523129999,15.2,3.65626745699998));
#200247=CARTESIAN_POINT('Ctrl Pts',(10.5405523129999,11.6,3.65626745699998));
#200248=CARTESIAN_POINT('Ctrl Pts',(10.5430604559999,15.2,3.65846767299999));
#200249=CARTESIAN_POINT('Ctrl Pts',(10.5430604559999,11.6,3.65846767299998));
#200250=CARTESIAN_POINT('Ctrl Pts',(10.5455705689999,15.2,3.66067314599999));
#200251=CARTESIAN_POINT('Ctrl Pts',(10.5455705689999,11.6,3.66067314599999));
#200252=CARTESIAN_POINT('Ctrl Pts',(10.5480826419999,15.2,3.66288387299999));
#200253=CARTESIAN_POINT('Ctrl Pts',(10.5480826419999,11.6,3.66288387299999));
#200254=CARTESIAN_POINT('Ctrl Pts',(10.5505966639999,15.2,3.66509985799999));
#200255=CARTESIAN_POINT('Ctrl Pts',(10.5505966639999,11.6,3.66509985799999));
#200256=CARTESIAN_POINT('Ctrl Pts',(10.5531126259999,15.2,3.66732109599998));
#200257=CARTESIAN_POINT('Ctrl Pts',(10.5531126259999,11.6,3.66732109599998));
#200258=CARTESIAN_POINT('Ctrl Pts',(10.5556305149999,15.2,3.66954758899999));
#200259=CARTESIAN_POINT('Ctrl Pts',(10.5556305149999,11.6,3.66954758899999));
#200260=CARTESIAN_POINT('Ctrl Pts',(10.5581503209999,15.2,3.67177933599999));
#200261=CARTESIAN_POINT('Ctrl Pts',(10.5581503209999,11.6,3.67177933599999));
#200262=CARTESIAN_POINT('Ctrl Pts',(10.5606720349999,15.2,3.67401633699998));
#200263=CARTESIAN_POINT('Ctrl Pts',(10.5606720349999,11.6,3.67401633699998));
#200264=CARTESIAN_POINT('Ctrl Pts',(10.5631956449999,15.2,3.67625858999999));
#200265=CARTESIAN_POINT('Ctrl Pts',(10.5631956449999,11.6,3.67625858999999));
#200266=CARTESIAN_POINT('Ctrl Pts',(10.5657211419999,15.2,3.67850609499998));
#200267=CARTESIAN_POINT('Ctrl Pts',(10.5657211419999,11.6,3.67850609499998));
#200268=CARTESIAN_POINT('Ctrl Pts',(10.5682485129999,15.2,3.68075884999998));
#200269=CARTESIAN_POINT('Ctrl Pts',(10.5682485129999,11.6,3.68075884999998));
#200270=CARTESIAN_POINT('Ctrl Pts',(10.5707777509999,15.2,3.68301685799998));
#200271=CARTESIAN_POINT('Ctrl Pts',(10.5707777509999,11.6,3.68301685799998));
#200272=CARTESIAN_POINT('Ctrl Pts',(10.5733088419999,15.2,3.68528011699999));
#200273=CARTESIAN_POINT('Ctrl Pts',(10.5733088419999,11.6,3.68528011699999));
#200274=CARTESIAN_POINT('Ctrl Pts',(10.5758417789999,15.2,3.68754862399998));
#200275=CARTESIAN_POINT('Ctrl Pts',(10.5758417789999,11.6,3.68754862399998));
#200276=CARTESIAN_POINT('Ctrl Pts',(10.5783765499999,15.2,3.68982238099999));
#200277=CARTESIAN_POINT('Ctrl Pts',(10.5783765499999,11.6,3.68982238099999));
#200278=CARTESIAN_POINT('Ctrl Pts',(10.5809131429999,15.2,3.69210138599998));
#200279=CARTESIAN_POINT('Ctrl Pts',(10.5809131429999,11.6,3.69210138599998));
#200280=CARTESIAN_POINT('Ctrl Pts',(10.5834515509999,15.2,3.69438563899998));
#200281=CARTESIAN_POINT('Ctrl Pts',(10.5834515509999,11.6,3.69438563899998));
#200282=CARTESIAN_POINT('Ctrl Pts',(10.5859917629999,15.2,3.69667513899999));
#200283=CARTESIAN_POINT('Ctrl Pts',(10.5859917629999,11.6,3.69667513899999));
#200284=CARTESIAN_POINT('Ctrl Pts',(10.5885337649999,15.2,3.69896988599999));
#200285=CARTESIAN_POINT('Ctrl Pts',(10.5885337649999,11.6,3.69896988599999));
#200286=CARTESIAN_POINT('Ctrl Pts',(10.5910775529999,15.2,3.70126987899998));
#200287=CARTESIAN_POINT('Ctrl Pts',(10.5910775529999,11.6,3.70126987899998));
#200288=CARTESIAN_POINT('Ctrl Pts',(10.5936231109999,15.2,3.70357511699999));
#200289=CARTESIAN_POINT('Ctrl Pts',(10.5936231109999,11.6,3.70357511699999));
#200290=CARTESIAN_POINT('Ctrl Pts',(10.5961704319999,15.2,3.70588559899999));
#200291=CARTESIAN_POINT('Ctrl Pts',(10.5961704319999,11.6,3.70588559899998));
#200292=CARTESIAN_POINT('Ctrl Pts',(10.5987195039999,15.2,3.70820132699999));
#200293=CARTESIAN_POINT('Ctrl Pts',(10.5987195039999,11.6,3.70820132699999));
#200294=CARTESIAN_POINT('Ctrl Pts',(10.6012703189999,15.2,3.71052229699998));
#200295=CARTESIAN_POINT('Ctrl Pts',(10.6012703189999,11.6,3.71052229699998));
#200296=CARTESIAN_POINT('Ctrl Pts',(10.6038228649999,15.2,3.71284850999999));
#200297=CARTESIAN_POINT('Ctrl Pts',(10.6038228649999,11.6,3.71284850999999));
#200298=CARTESIAN_POINT('Ctrl Pts',(10.6063771329999,15.2,3.71517996499998));
#200299=CARTESIAN_POINT('Ctrl Pts',(10.6063771329999,11.6,3.71517996499998));
#200300=CARTESIAN_POINT('Ctrl Pts',(10.6089331119999,15.2,3.71751665999999));
#200301=CARTESIAN_POINT('Ctrl Pts',(10.6089331119999,11.6,3.71751665999999));
#200302=CARTESIAN_POINT('Ctrl Pts',(10.6114907919999,15.2,3.71985859599998));
#200303=CARTESIAN_POINT('Ctrl Pts',(10.6114907919999,11.6,3.71985859599998));
#200304=CARTESIAN_POINT('Ctrl Pts',(10.6140501629999,15.2,3.72220577299998));
#200305=CARTESIAN_POINT('Ctrl Pts',(10.6140501629999,11.6,3.72220577299998));
#200306=CARTESIAN_POINT('Ctrl Pts',(10.6166112159999,15.2,3.72455818799998));
#200307=CARTESIAN_POINT('Ctrl Pts',(10.6166112159999,11.6,3.72455818799998));
#200308=CARTESIAN_POINT('Ctrl Pts',(10.6191739399999,15.2,3.72691584199998));
#200309=CARTESIAN_POINT('Ctrl Pts',(10.6191739399999,11.6,3.72691584199998));
#200310=CARTESIAN_POINT('Ctrl Pts',(10.6217383239999,15.2,3.72927873299999));
#200311=CARTESIAN_POINT('Ctrl Pts',(10.6217383239999,11.6,3.72927873299999));
#200312=CARTESIAN_POINT('Ctrl Pts',(10.6243043599999,15.2,3.73164686199999));
#200313=CARTESIAN_POINT('Ctrl Pts',(10.6243043599999,11.6,3.73164686199999));
#200314=CARTESIAN_POINT('Ctrl Pts',(10.6268720369999,15.2,3.73402022499998));
#200315=CARTESIAN_POINT('Ctrl Pts',(10.6268720369999,11.6,3.73402022499998));
#200316=CARTESIAN_POINT('Ctrl Pts',(10.6294413449999,15.2,3.73639882599999));
#200317=CARTESIAN_POINT('Ctrl Pts',(10.6294413449999,11.6,3.73639882599999));
#200318=CARTESIAN_POINT('Ctrl Pts',(10.6320122749999,15.2,3.73878265999998));
#200319=CARTESIAN_POINT('Ctrl Pts',(10.6320122749999,11.6,3.73878265999998));
#200320=CARTESIAN_POINT('Ctrl Pts',(10.6345848139999,15.2,3.74117172899999));
#200321=CARTESIAN_POINT('Ctrl Pts',(10.6345848139999,11.6,3.74117172899999));
#200322=CARTESIAN_POINT('Ctrl Pts',(10.6371589569999,15.2,3.74356603099999));
#200323=CARTESIAN_POINT('Ctrl Pts',(10.6371589569999,11.6,3.74356603099999));
#200324=CARTESIAN_POINT('Ctrl Pts',(10.6397346889999,15.2,3.74596556499998));
#200325=CARTESIAN_POINT('Ctrl Pts',(10.6397346889999,11.6,3.74596556499998));
#200326=CARTESIAN_POINT('Ctrl Pts',(10.6423120039999,15.2,3.74837032999999));
#200327=CARTESIAN_POINT('Ctrl Pts',(10.6423120039999,11.6,3.74837032999999));
#200328=CARTESIAN_POINT('Ctrl Pts',(10.6448908909999,15.2,3.75078032599999));
#200329=CARTESIAN_POINT('Ctrl Pts',(10.6448908909999,11.6,3.75078032599998));
#200330=CARTESIAN_POINT('Ctrl Pts',(10.6474713389999,15.2,3.75319555299999));
#200331=CARTESIAN_POINT('Ctrl Pts',(10.6474713389999,11.6,3.75319555299999));
#200332=CARTESIAN_POINT('Ctrl Pts',(10.6500533389999,15.2,3.75561600899999));
#200333=CARTESIAN_POINT('Ctrl Pts',(10.6500533389999,11.6,3.75561600899999));
#200334=CARTESIAN_POINT('Ctrl Pts',(10.6526368819999,15.2,3.75804169199998));
#200335=CARTESIAN_POINT('Ctrl Pts',(10.6526368819999,11.6,3.75804169199998));
#200336=CARTESIAN_POINT('Ctrl Pts',(10.6552219569999,15.2,3.76047260399999));
#200337=CARTESIAN_POINT('Ctrl Pts',(10.6552219569999,11.6,3.76047260399999));
#200338=CARTESIAN_POINT('Ctrl Pts',(10.6578085549999,15.2,3.76290874199999));
#200339=CARTESIAN_POINT('Ctrl Pts',(10.6578085549999,11.6,3.76290874199999));
#200340=CARTESIAN_POINT('Ctrl Pts',(10.6603966649999,15.2,3.76535010599999));
#200341=CARTESIAN_POINT('Ctrl Pts',(10.6603966649999,11.6,3.76535010599999));
#200342=CARTESIAN_POINT('Ctrl Pts',(10.6629862789999,15.2,3.76779669499999));
#200343=CARTESIAN_POINT('Ctrl Pts',(10.6629862789999,11.6,3.76779669499999));
#200344=CARTESIAN_POINT('Ctrl Pts',(10.6655773879999,15.2,3.77024850899998));
#200345=CARTESIAN_POINT('Ctrl Pts',(10.6655773879999,11.6,3.77024850899998));
#200346=CARTESIAN_POINT('Ctrl Pts',(10.6681699789999,15.2,3.77270554599999));
#200347=CARTESIAN_POINT('Ctrl Pts',(10.6681699789999,11.6,3.77270554599999));
#200348=CARTESIAN_POINT('Ctrl Pts',(10.6707640449999,15.2,3.77516780499998));
#200349=CARTESIAN_POINT('Ctrl Pts',(10.6707640449999,11.6,3.77516780499998));
#200350=CARTESIAN_POINT('Ctrl Pts',(10.6733595749999,15.2,3.77763528599999));
#200351=CARTESIAN_POINT('Ctrl Pts',(10.6733595749999,11.6,3.77763528599999));
#200352=CARTESIAN_POINT('Ctrl Pts',(10.6759565599999,15.2,3.78010798799998));
#200353=CARTESIAN_POINT('Ctrl Pts',(10.6759565599999,11.6,3.78010798799998));
#200354=CARTESIAN_POINT('Ctrl Pts',(10.6785549909999,15.2,3.78258590999998));
#200355=CARTESIAN_POINT('Ctrl Pts',(10.6785549909999,11.6,3.78258590999998));
#200356=CARTESIAN_POINT('Ctrl Pts',(10.6811548569999,15.2,3.78506904999998));
#200357=CARTESIAN_POINT('Ctrl Pts',(10.6811548569999,11.6,3.78506904999998));
#200358=CARTESIAN_POINT('Ctrl Pts',(10.6837561499999,15.2,3.78755740899998));
#200359=CARTESIAN_POINT('Ctrl Pts',(10.6837561499999,11.6,3.78755740899998));
#200360=CARTESIAN_POINT('Ctrl Pts',(10.6863588589999,15.2,3.79005098599999));
#200361=CARTESIAN_POINT('Ctrl Pts',(10.6863588589999,11.6,3.79005098599999));
#200362=CARTESIAN_POINT('Ctrl Pts',(10.6889629749999,15.2,3.79254977899999));
#200363=CARTESIAN_POINT('Ctrl Pts',(10.6889629749999,11.6,3.79254977899999));
#200364=CARTESIAN_POINT('Ctrl Pts',(10.6915684889999,15.2,3.79505378599998));
#200365=CARTESIAN_POINT('Ctrl Pts',(10.6915684889999,11.6,3.79505378599998));
#200366=CARTESIAN_POINT('Ctrl Pts',(10.6941753909999,15.2,3.79756300999999));
#200367=CARTESIAN_POINT('Ctrl Pts',(10.6941753909999,11.6,3.79756300999999));
#200368=CARTESIAN_POINT('Ctrl Pts',(10.6967836699999,15.2,3.80007744599999));
#200369=CARTESIAN_POINT('Ctrl Pts',(10.6967836699999,11.6,3.80007744599998));
#200370=CARTESIAN_POINT('Ctrl Pts',(10.6993933199999,15.2,3.80259709499998));
#200371=CARTESIAN_POINT('Ctrl Pts',(10.6993933199999,11.6,3.80259709499998));
#200372=CARTESIAN_POINT('Ctrl Pts',(10.7020043289999,15.2,3.80512195599999));
#200373=CARTESIAN_POINT('Ctrl Pts',(10.7020043289999,11.6,3.80512195599999));
#200374=CARTESIAN_POINT('Ctrl Pts',(10.7046166879999,15.2,3.80765202799999));
#200375=CARTESIAN_POINT('Ctrl Pts',(10.7046166879999,11.6,3.80765202799999));
#200376=CARTESIAN_POINT('Ctrl Pts',(10.7072303869999,15.2,3.81018730899999));
#200377=CARTESIAN_POINT('Ctrl Pts',(10.7072303869999,11.6,3.81018730899999));
#200378=CARTESIAN_POINT('Ctrl Pts',(10.7098454179999,15.2,3.81272779999998));
#200379=CARTESIAN_POINT('Ctrl Pts',(10.7098454179999,11.6,3.81272779999998));
#200380=CARTESIAN_POINT('Ctrl Pts',(10.7124617709999,15.2,3.81527349799998));
#200381=CARTESIAN_POINT('Ctrl Pts',(10.7124617709999,11.6,3.81527349799998));
#200382=CARTESIAN_POINT('Ctrl Pts',(10.7150794359999,15.2,3.81782440399999));
#200383=CARTESIAN_POINT('Ctrl Pts',(10.7150794359999,11.6,3.81782440399998));
#200384=CARTESIAN_POINT('Ctrl Pts',(10.7176984049999,15.2,3.82038051699999));
#200385=CARTESIAN_POINT('Ctrl Pts',(10.7176984049999,11.6,3.82038051699999));
#200386=CARTESIAN_POINT('Ctrl Pts',(10.7203186669999,15.2,3.82294183299998));
#200387=CARTESIAN_POINT('Ctrl Pts',(10.7203186669999,11.6,3.82294183299998));
#200388=CARTESIAN_POINT('Ctrl Pts',(10.7229402149999,15.2,3.82550835499998));
#200389=CARTESIAN_POINT('Ctrl Pts',(10.7229402149999,11.6,3.82550835499998));
#200390=CARTESIAN_POINT('Ctrl Pts',(10.7255630379999,15.2,3.82808007899998));
#200391=CARTESIAN_POINT('Ctrl Pts',(10.7255630379999,11.6,3.82808007899998));
#200392=CARTESIAN_POINT('Ctrl Pts',(10.7281871259999,15.2,3.83065700599998));
#200393=CARTESIAN_POINT('Ctrl Pts',(10.7281871259999,11.6,3.83065700599998));
#200394=CARTESIAN_POINT('Ctrl Pts',(10.7308124709999,15.2,3.83323913299999));
#200395=CARTESIAN_POINT('Ctrl Pts',(10.7308124709999,11.6,3.83323913299999));
#200396=CARTESIAN_POINT('Ctrl Pts',(10.7334390639999,15.2,3.83582646099998));
#200397=CARTESIAN_POINT('Ctrl Pts',(10.7334390639999,11.6,3.83582646099998));
#200398=CARTESIAN_POINT('Ctrl Pts',(10.7360668939999,15.2,3.83841898799999));
#200399=CARTESIAN_POINT('Ctrl Pts',(10.7360668939999,11.6,3.83841898799999));
#200400=CARTESIAN_POINT('Ctrl Pts',(10.7386959529999,15.2,3.84101671299998));
#200401=CARTESIAN_POINT('Ctrl Pts',(10.7386959529999,11.6,3.84101671299998));
#200402=CARTESIAN_POINT('Ctrl Pts',(10.7413262329999,15.2,3.84361963599999));
#200403=CARTESIAN_POINT('Ctrl Pts',(10.7413262329999,11.6,3.84361963599999));
#200404=CARTESIAN_POINT('Ctrl Pts',(10.7439577219999,15.2,3.84622775399999));
#200405=CARTESIAN_POINT('Ctrl Pts',(10.7439577219999,11.6,3.84622775399999));
#200406=CARTESIAN_POINT('Ctrl Pts',(10.7465904139999,15.2,3.84884106799999));
#200407=CARTESIAN_POINT('Ctrl Pts',(10.7465904139999,11.6,3.84884106799999));
#200408=CARTESIAN_POINT('Ctrl Pts',(10.7492242979999,15.2,3.85145957599998));
#200409=CARTESIAN_POINT('Ctrl Pts',(10.7492242979999,11.6,3.85145957599998));
#200410=CARTESIAN_POINT('Ctrl Pts',(10.7518593659999,15.2,3.85408327699999));
#200411=CARTESIAN_POINT('Ctrl Pts',(10.7518593659999,11.6,3.85408327699999));
#200412=CARTESIAN_POINT('Ctrl Pts',(10.7544956079999,15.2,3.85671216899999));
#200413=CARTESIAN_POINT('Ctrl Pts',(10.7544956079999,11.6,3.85671216899999));
#200414=CARTESIAN_POINT('Ctrl Pts',(10.7571330149999,15.2,3.85934625299999));
#200415=CARTESIAN_POINT('Ctrl Pts',(10.7571330149999,11.6,3.85934625299999));
#200416=CARTESIAN_POINT('Ctrl Pts',(10.7597715779999,15.2,3.86198552599998));
#200417=CARTESIAN_POINT('Ctrl Pts',(10.7597715779999,11.6,3.86198552599998));
#200418=CARTESIAN_POINT('Ctrl Pts',(10.7624112859999,15.2,3.86462998899999));
#200419=CARTESIAN_POINT('Ctrl Pts',(10.7624112859999,11.6,3.86462998899999));
#200420=CARTESIAN_POINT('Ctrl Pts',(10.7650521309999,15.2,3.86727963899999));
#200421=CARTESIAN_POINT('Ctrl Pts',(10.7650521309999,11.6,3.86727963899998));
#200422=CARTESIAN_POINT('Ctrl Pts',(10.7676941039999,15.2,3.86993447499999));
#200423=CARTESIAN_POINT('Ctrl Pts',(10.7676941039999,11.6,3.86993447499999));
#200424=CARTESIAN_POINT('Ctrl Pts',(10.7703371949999,15.2,3.87259449799998));
#200425=CARTESIAN_POINT('Ctrl Pts',(10.7703371949999,11.6,3.87259449799998));
#200426=CARTESIAN_POINT('Ctrl Pts',(10.7729813979999,15.2,3.87525970399999));
#200427=CARTESIAN_POINT('Ctrl Pts',(10.7729813979999,11.6,3.87525970399999));
#200428=CARTESIAN_POINT('Ctrl Pts',(10.7756267029999,15.2,3.87793009399999));
#200429=CARTESIAN_POINT('Ctrl Pts',(10.7756267029999,11.6,3.87793009399999));
#200430=CARTESIAN_POINT('Ctrl Pts',(10.7782731039999,15.2,3.88060566599999));
#200431=CARTESIAN_POINT('Ctrl Pts',(10.7782731039999,11.6,3.88060566599999));
#200432=CARTESIAN_POINT('Ctrl Pts',(10.7809205909999,15.2,3.88328641999999));
#200433=CARTESIAN_POINT('Ctrl Pts',(10.7809205909999,11.6,3.88328641999998));
#200434=CARTESIAN_POINT('Ctrl Pts',(10.7835691559999,15.2,3.88597235399998));
#200435=CARTESIAN_POINT('Ctrl Pts',(10.7835691559999,11.6,3.88597235399998));
#200436=CARTESIAN_POINT('Ctrl Pts',(10.7862187859999,15.2,3.88866346799999));
#200437=CARTESIAN_POINT('Ctrl Pts',(10.7862187859999,11.6,3.88866346799999));
#200438=CARTESIAN_POINT('Ctrl Pts',(10.7888694719999,15.2,3.89135975899999));
#200439=CARTESIAN_POINT('Ctrl Pts',(10.7888694719999,11.6,3.89135975899999));
#200440=CARTESIAN_POINT('Ctrl Pts',(10.7915212029999,15.2,3.89406122599999));
#200441=CARTESIAN_POINT('Ctrl Pts',(10.7915212029999,11.6,3.89406122599999));
#200442=CARTESIAN_POINT('Ctrl Pts',(10.7941739669999,15.2,3.89676786899999));
#200443=CARTESIAN_POINT('Ctrl Pts',(10.7941739669999,11.6,3.89676786899999));
#200444=CARTESIAN_POINT('Ctrl Pts',(10.7968277549999,15.2,3.89947968499998));
#200445=CARTESIAN_POINT('Ctrl Pts',(10.7968277549999,11.6,3.89947968499998));
#200446=CARTESIAN_POINT('Ctrl Pts',(10.7994825589999,15.2,3.90219667399998));
#200447=CARTESIAN_POINT('Ctrl Pts',(10.7994825589999,11.6,3.90219667399998));
#200448=CARTESIAN_POINT('Ctrl Pts',(10.8021383729999,15.2,3.90491883499998));
#200449=CARTESIAN_POINT('Ctrl Pts',(10.8021383729999,11.6,3.90491883499998));
#200450=CARTESIAN_POINT('Ctrl Pts',(10.8047951939999,15.2,3.90764616699999));
#200451=CARTESIAN_POINT('Ctrl Pts',(10.8047951939999,11.6,3.90764616699998));
#200452=CARTESIAN_POINT('Ctrl Pts',(10.8074530179999,15.2,3.91037866999999));
#200453=CARTESIAN_POINT('Ctrl Pts',(10.8074530179999,11.6,3.91037866999999));
#200454=CARTESIAN_POINT('Ctrl Pts',(10.8095800799999,15.2,3.91256880899999));
#200455=CARTESIAN_POINT('Ctrl Pts',(10.8095800799999,11.6,3.91256880899999));
#200456=CARTESIAN_POINT('Ctrl Pts',(10.8111758269999,15.2,3.91421373899998));
#200457=CARTESIAN_POINT('Ctrl Pts',(10.8111758269999,11.6,3.91421373899998));
#200458=CARTESIAN_POINT('Ctrl Pts',(10.8122398589999,15.2,3.91531139399999));
#200459=CARTESIAN_POINT('Ctrl Pts',(10.8122398589999,11.6,3.91531139399999));
#200460=CARTESIAN_POINT('Ctrl Pts',(10.8127719249999,15.2,3.91586047999999));
#200461=CARTESIAN_POINT('Ctrl Pts',(10.8127719249999,11.6,3.91586047999999));
#200462=CARTESIAN_POINT('Ctrl Pts',(9.86852965799994,15.2,3.20199116299998));
#200463=CARTESIAN_POINT('Ctrl Pts',(9.87017542602826,15.2,3.2026865729514));
#200464=CARTESIAN_POINT('Ctrl Pts',(9.87187175395476,15.2,3.20340918505387));
#200465=CARTESIAN_POINT('Ctrl Pts',(9.87361750382533,15.2,3.20415921017613));
#200466=CARTESIAN_POINT('Ctrl Pts',(9.8753716725842,15.2,3.20491285229864));
#200467=CARTESIAN_POINT('Ctrl Pts',(9.87717573909119,15.2,3.20569417515048));
#200468=CARTESIAN_POINT('Ctrl Pts',(9.87902857820422,15.2,3.20650338931996));
#200469=CARTESIAN_POINT('Ctrl Pts',(9.88088141714894,15.2,3.20731260341592));
#200470=CARTESIAN_POINT('Ctrl Pts',(9.88278302753734,15.2,3.20814970993136));
#200471=CARTESIAN_POINT('Ctrl Pts',(9.88473231729986,15.2,3.20901491173327));
#200472=CARTESIAN_POINT('Ctrl Pts',(9.88668160706237,15.2,3.20988011353517));
#200473=CARTESIAN_POINT('Ctrl Pts',(9.88867857432713,15.2,3.21077340710827));
#200474=CARTESIAN_POINT('Ctrl Pts',(9.89072215651895,15.2,3.21169499186919));
#200475=CARTESIAN_POINT('Ctrl Pts',(9.8927657388964,15.2,3.21261657671382));
#200476=CARTESIAN_POINT('Ctrl Pts',(9.89485593697986,15.2,3.21356644793465));
#200477=CARTESIAN_POINT('Ctrl Pts',(9.89699171626601,15.2,3.21454479382325));
#200478=CARTESIAN_POINT('Ctrl Pts',(9.89948345847554,15.2,3.21568619722663));
#200479=CARTESIAN_POINT('Ctrl Pts',(9.90203723794068,15.2,3.21686635803255));
#200480=CARTESIAN_POINT('Ctrl Pts',(9.90465146305821,15.2,3.21808555589058));
#200481=CARTESIAN_POINT('Ctrl Pts',(9.90689222770636,15.2,3.21913058274808));
#200482=CARTESIAN_POINT('Ctrl Pts',(9.90917740008215,15.2,3.22020428848307));
#200483=CARTESIAN_POINT('Ctrl Pts',(9.91150600579537,15.2,3.22130684512845));
#200484=CARTESIAN_POINT('Ctrl Pts',(9.91383461129706,15.2,3.22240940167369));
#200485=CARTESIAN_POINT('Ctrl Pts',(9.91620664881097,15.2,3.22354080604563));
#200486=CARTESIAN_POINT('Ctrl Pts',(9.9186211692343,15.2,3.22470122175879));
#200487=CARTESIAN_POINT('Ctrl Pts',(9.92103568965765,15.2,3.22586163747197));
#200488=CARTESIAN_POINT('Ctrl Pts',(9.92349269040646,15.2,3.22705106416252));
#200489=CARTESIAN_POINT('Ctrl Pts',(9.92599124514721,15.2,3.22826965495031));
#200490=CARTESIAN_POINT('Ctrl Pts',(9.9284898001149,15.2,3.22948824584879));
#200491=CARTESIAN_POINT('Ctrl Pts',(9.93102990997944,15.2,3.23073600190922));
#200492=CARTESIAN_POINT('Ctrl Pts',(9.93361066903952,15.2,3.23201307139747));
#200493=CARTESIAN_POINT('Ctrl Pts',(9.93619142786518,15.2,3.23329014076973));
#200494=CARTESIAN_POINT('Ctrl Pts',(9.93881283676505,15.2,3.23459652170345));
#200495=CARTESIAN_POINT('Ctrl Pts',(9.94147401258674,15.2,3.23593235732286));
#200496=CARTESIAN_POINT('Ctrl Pts',(9.94413518840844,15.2,3.23726819294227));
#200497=CARTESIAN_POINT('Ctrl Pts',(9.94683613201863,15.2,3.23863348160101));
#200498=CARTESIAN_POINT('Ctrl Pts',(9.94957597908405,15.2,3.24002836113237));
#200499=CARTESIAN_POINT('Ctrl Pts',(9.95231582614947,15.2,3.24142324066374));
#200500=CARTESIAN_POINT('Ctrl Pts',(9.95509458055612,15.2,3.24284770847963));
#200501=CARTESIAN_POINT('Ctrl Pts',(9.95791139670119,15.2,3.24430189409144));
#200502=CARTESIAN_POINT('Ctrl Pts',(9.96072821310213,15.2,3.24575607983533));
#200503=CARTESIAN_POINT('Ctrl Pts',(9.96358309289007,15.2,3.24723998469043));
#200504=CARTESIAN_POINT('Ctrl Pts',(9.96647521513266,15.2,3.24875373035756));
#200505=CARTESIAN_POINT('Ctrl Pts',(9.96936733711254,15.2,3.25026747588719));
#200506=CARTESIAN_POINT('Ctrl Pts',(9.97229669893939,15.2,3.25181106350611));
#200507=CARTESIAN_POINT('Ctrl Pts',(9.97526249808007,15.2,3.25338460994764));
#200508=CARTESIAN_POINT('Ctrl Pts',(9.97822829722075,15.2,3.25495815638917));
#200509=CARTESIAN_POINT('Ctrl Pts',(9.98123053182321,15.2,3.25656166152494));
#200510=CARTESIAN_POINT('Ctrl Pts',(9.98426841896043,15.2,3.25819523904688));
#200511=CARTESIAN_POINT('Ctrl Pts',(9.98730630637357,15.2,3.2598288167172));
#200512=CARTESIAN_POINT('Ctrl Pts',(9.9903798430735,15.2,3.2614924662154));
#200513=CARTESIAN_POINT('Ctrl Pts',(9.9934882616611,15.2,3.26318629380904));
#200514=CARTESIAN_POINT('Ctrl Pts',(9.99659667996637,15.2,3.26488012124881));
#200515=CARTESIAN_POINT('Ctrl Pts',(9.9997399786912,15.2,3.2666041282383));
#200516=CARTESIAN_POINT('Ctrl Pts',(10.0029174070068,15.2,3.2683584165158));
#200517=CARTESIAN_POINT('Ctrl Pts',(10.0066244069007,15.2,3.27040508627912));
#200518=CARTESIAN_POINT('Ctrl Pts',(10.0103778566166,15.2,3.27249297058149));
#200519=CARTESIAN_POINT('Ctrl Pts',(10.0141765904275,15.2,3.27462222536619));
#200520=CARTESIAN_POINT('Ctrl Pts',(10.0174326478106,15.2,3.27644730080122));
#200521=CARTESIAN_POINT('Ctrl Pts',(10.0207219743957,15.2,3.27830277088412));
#200522=CARTESIAN_POINT('Ctrl Pts',(10.02404385104,15.2,3.28018872624074));
#200523=CARTESIAN_POINT('Ctrl Pts',(10.0273657276843,15.2,3.28207468159738));
#200524=CARTESIAN_POINT('Ctrl Pts',(10.0307201547644,15.2,3.28399112417722));
#200525=CARTESIAN_POINT('Ctrl Pts',(10.0341064263891,15.2,3.28593813877105));
#200526=CARTESIAN_POINT('Ctrl Pts',(10.0374926983215,15.2,3.28788515354173));
#200527=CARTESIAN_POINT('Ctrl Pts',(10.0409108153715,15.2,3.28986274291605));
#200528=CARTESIAN_POINT('Ctrl Pts',(10.044360085567,15.2,3.29187098846095));
#200529=CARTESIAN_POINT('Ctrl Pts',(10.0472344772399,15.2,3.29354452632382));
#200530=CARTESIAN_POINT('Ctrl Pts',(10.0501305033909,15.2,3.29523935320601));
#200531=CARTESIAN_POINT('Ctrl Pts',(10.0530477716565,15.2,3.29695551445775));
#200532=CARTESIAN_POINT('Ctrl Pts',(10.0559650399221,15.2,3.29867167570949));
#200533=CARTESIAN_POINT('Ctrl Pts',(10.0589035501853,15.2,3.30040917285603));
#200534=CARTESIAN_POINT('Ctrl Pts',(10.0618629166453,15.2,3.302168048205));
#200535=CARTESIAN_POINT('Ctrl Pts',(10.0654141562683,15.2,3.30427869854707));
#200536=CARTESIAN_POINT('Ctrl Pts',(10.0689954263267,15.2,3.30642013547104));
#200537=CARTESIAN_POINT('Ctrl Pts',(10.0726060711968,15.2,3.30859242964345));
#200538=CARTESIAN_POINT('Ctrl Pts',(10.0756149420312,15.2,3.3104026748529));
#200539=CARTESIAN_POINT('Ctrl Pts',(10.078644213215,15.2,3.31223434765347));
#200540=CARTESIAN_POINT('Ctrl Pts',(10.0816935107161,15.2,3.31408749036292));
#200541=CARTESIAN_POINT('Ctrl Pts',(10.0847428082172,15.2,3.31594063307238));
#200542=CARTESIAN_POINT('Ctrl Pts',(10.0878121321529,15.2,3.31781524422945));
#200543=CARTESIAN_POINT('Ctrl Pts',(10.0909011156419,15.2,3.31971136127012));
#200544=CARTESIAN_POINT('Ctrl Pts',(10.0939900991309,15.2,3.32160747831078));
#200545=CARTESIAN_POINT('Ctrl Pts',(10.0970987406408,15.2,3.32352510248517));
#200546=CARTESIAN_POINT('Ctrl Pts',(10.100226679184,15.2,3.32546426852858));
#200547=CARTESIAN_POINT('Ctrl Pts',(10.1033546177273,15.2,3.327403434572));
#200548=CARTESIAN_POINT('Ctrl Pts',(10.1065018539514,15.2,3.32936414310745));
#200549=CARTESIAN_POINT('Ctrl Pts',(10.109668030689,15.2,3.33134642831755));
#200550=CARTESIAN_POINT('Ctrl Pts',(10.1128342070816,15.2,3.33332871331159));
#200551=CARTESIAN_POINT('Ctrl Pts',(10.1160193233205,15.2,3.33533257472978));
#200552=CARTESIAN_POINT('Ctrl Pts',(10.1192230290809,15.2,3.33735804624334));
#200553=CARTESIAN_POINT('Ctrl Pts',(10.1224267351904,15.2,3.33938351797768));
#200554=CARTESIAN_POINT('Ctrl Pts',(10.1256490317887,15.2,3.34143059796446));
#200555=CARTESIAN_POINT('Ctrl Pts',(10.1288895710927,15.2,3.34349931900435));
#200556=CARTESIAN_POINT('Ctrl Pts',(10.1321301103968,15.2,3.34556804004424));
#200557=CARTESIAN_POINT('Ctrl Pts',(10.1353888930293,15.2,3.3476584018786));
#200558=CARTESIAN_POINT('Ctrl Pts',(10.1386655776363,15.2,3.34977043232983));
#200559=CARTESIAN_POINT('Ctrl Pts',(10.1419422622431,15.2,3.35188246278107));
#200560=CARTESIAN_POINT('Ctrl Pts',(10.1452368494678,15.2,3.35401616384925));
#200561=CARTESIAN_POINT('Ctrl Pts',(10.1485490030083,15.2,3.35617156162571));
#200562=CARTESIAN_POINT('Ctrl Pts',(10.1518611565488,15.2,3.35832695940218));
#200563=CARTESIAN_POINT('Ctrl Pts',(10.1551908747876,15.2,3.36050405526851));
#200564=CARTESIAN_POINT('Ctrl Pts',(10.1585378292311,15.2,3.36270287457292));
#200565=CARTESIAN_POINT('Ctrl Pts',(10.1618847836746,15.2,3.36490169387733));
#200566=CARTESIAN_POINT('Ctrl Pts',(10.165248972552,15.2,3.36712223751011));
#200567=CARTESIAN_POINT('Ctrl Pts',(10.1686300694955,15.2,3.36936452862008));
#200568=CARTESIAN_POINT('Ctrl Pts',(10.1720111664391,15.2,3.37160681973005));
#200569=CARTESIAN_POINT('Ctrl Pts',(10.1754091705048,15.2,3.37387085927725));
#200570=CARTESIAN_POINT('Ctrl Pts',(10.178823760798,15.2,3.37615667102369));
#200571=CARTESIAN_POINT('Ctrl Pts',(10.1822383510913,15.2,3.37844248277012));
#200572=CARTESIAN_POINT('Ctrl Pts',(10.1856695266332,15.2,3.38075006569993));
#200573=CARTESIAN_POINT('Ctrl Pts',(10.1891169710082,15.2,3.38307944174159));
#200574=CARTESIAN_POINT('Ctrl Pts',(10.1918749266585,15.2,3.38494294267648));
#200575=CARTESIAN_POINT('Ctrl Pts',(10.1946432919156,15.2,3.38682039215467));
#200576=CARTESIAN_POINT('Ctrl Pts',(10.1974219096792,15.2,3.38871180025918));
#200577=CARTESIAN_POINT('Ctrl Pts',(10.2002005270642,15.2,3.39060320810599));
#200578=CARTESIAN_POINT('Ctrl Pts',(10.2029893944002,15.2,3.39250857375242));
#200579=CARTESIAN_POINT('Ctrl Pts',(10.2057883532397,15.2,3.39442790771529));
#200580=CARTESIAN_POINT('Ctrl Pts',(10.2085873124604,15.2,3.39634724193967));
#200581=CARTESIAN_POINT('Ctrl Pts',(10.2113963637895,15.2,3.39828054458298));
#200582=CARTESIAN_POINT('Ctrl Pts',(10.2142153489442,15.2,3.40022782480165));
#200583=CARTESIAN_POINT('Ctrl Pts',(10.2170343337147,15.2,3.40217510475501));
#200584=CARTESIAN_POINT('Ctrl Pts',(10.2198632530201,15.2,3.4041363628593));
#200585=CARTESIAN_POINT('Ctrl Pts',(10.2227019505096,15.2,3.40611160686359));
#200586=CARTESIAN_POINT('Ctrl Pts',(10.2255406483859,15.2,3.408086851137));
#200587=CARTESIAN_POINT('Ctrl Pts',(10.228389124582,15.2,3.41007608275244));
#200588=CARTESIAN_POINT('Ctrl Pts',(10.2312472258814,15.2,3.41207930907402));
#200589=CARTESIAN_POINT('Ctrl Pts',(10.2341053267913,15.2,3.41408253512266));
#200590=CARTESIAN_POINT('Ctrl Pts',(10.2369730516617,15.2,3.41609975537043));
#200591=CARTESIAN_POINT('Ctrl Pts',(10.2398502479815,15.2,3.41813097859234));
#200592=CARTESIAN_POINT('Ctrl Pts',(10.2427274446932,15.2,3.42016220209101));
#200593=CARTESIAN_POINT('Ctrl Pts',(10.2456141140672,15.2,3.42220742844416));
#200594=CARTESIAN_POINT('Ctrl Pts',(10.2485101040034,15.2,3.4242666646684));
#200595=CARTESIAN_POINT('Ctrl Pts',(10.251406093545,15.2,3.42632590061207));
#200596=CARTESIAN_POINT('Ctrl Pts',(10.2543114045955,15.2,3.4283991466647));
#200597=CARTESIAN_POINT('Ctrl Pts',(10.2572258863354,15.2,3.43048640993047));
#200598=CARTESIAN_POINT('Ctrl Pts',(10.2601403684724,15.2,3.43257367348062));
#200599=CARTESIAN_POINT('Ctrl Pts',(10.263064022471,15.2,3.43467495324568));
#200600=CARTESIAN_POINT('Ctrl Pts',(10.2659966997981,15.2,3.43679025547299));
#200601=CARTESIAN_POINT('Ctrl Pts',(10.2689293767256,15.2,3.43890555741208));
#200602=CARTESIAN_POINT('Ctrl Pts',(10.2718710771846,15.2,3.44103488257895));
#200603=CARTESIAN_POINT('Ctrl Pts',(10.2748216547758,15.2,3.4431782371245));
#200604=CARTESIAN_POINT('Ctrl Pts',(10.277772232769,15.2,3.44532159196209));
#200605=CARTESIAN_POINT('Ctrl Pts',(10.2807316889517,15.2,3.44747897584539));
#200606=CARTESIAN_POINT('Ctrl Pts',(10.2836998762936,15.2,3.44965039275141));
#200607=CARTESIAN_POINT('Ctrl Pts',(10.2866680632311,15.2,3.45182180936158));
#200608=CARTESIAN_POINT('Ctrl Pts',(10.2896449825456,15.2,3.45400726194379));
#200609=CARTESIAN_POINT('Ctrl Pts',(10.2926304907451,15.2,3.45620675187366));
#200610=CARTESIAN_POINT('Ctrl Pts',(10.2963623762996,15.2,3.45895611451075));
#200611=CARTESIAN_POINT('Ctrl Pts',(10.3001076799316,15.2,3.46172741288083));
#200612=CARTESIAN_POINT('Ctrl Pts',(10.3038661264583,15.2,3.46452065614291));
#200613=CARTESIAN_POINT('Ctrl Pts',(10.3068728838435,15.2,3.46675525087436));
#200614=CARTESIAN_POINT('Ctrl Pts',(10.309888052704,15.2,3.46900388892616));
#200615=CARTESIAN_POINT('Ctrl Pts',(10.3129114914936,15.2,3.47126657522648));
#200616=CARTESIAN_POINT('Ctrl Pts',(10.3159349298714,15.2,3.4735292612185));
#200617=CARTESIAN_POINT('Ctrl Pts',(10.3189666403995,15.2,3.475805996128));
#200618=CARTESIAN_POINT('Ctrl Pts',(10.3220064807612,15.2,3.47809678188373));
#200619=CARTESIAN_POINT('Ctrl Pts',(10.3258062815241,15.2,3.48096026431247));
#200620=CARTESIAN_POINT('Ctrl Pts',(10.3296187892507,15.2,3.48384570220479));
#200621=CARTESIAN_POINT('Ctrl Pts',(10.3334437317496,15.2,3.48675309991132));
#200622=CARTESIAN_POINT('Ctrl Pts',(10.3365036859155,15.2,3.4890790182033));
#200623=CARTESIAN_POINT('Ctrl Pts',(10.3395716014204,15.2,3.49141899217916));
#200624=CARTESIAN_POINT('Ctrl Pts',(10.3426473382687,15.2,3.49377302298487));
#200625=CARTESIAN_POINT('Ctrl Pts',(10.3464920091195,15.2,3.49671556133164));
#200626=CARTESIAN_POINT('Ctrl Pts',(10.3503489042913,15.2,3.49968006414424));
#200627=CARTESIAN_POINT('Ctrl Pts',(10.3542177599863,15.2,3.50266653497871));
#200628=CARTESIAN_POINT('Ctrl Pts',(10.3573128442894,15.2,3.50505571145097));
#200629=CARTESIAN_POINT('Ctrl Pts',(10.3604155820853,15.2,3.50745894693709));
#200630=CARTESIAN_POINT('Ctrl Pts',(10.3635258429414,15.2,3.50987624340471));
#200631=CARTESIAN_POINT('Ctrl Pts',(10.3666361042213,15.2,3.51229354020169));
#200632=CARTESIAN_POINT('Ctrl Pts',(10.3697538852342,15.2,3.51472489777383));
#200633=CARTESIAN_POINT('Ctrl Pts',(10.372879056752,15.2,3.5171703172516));
#200634=CARTESIAN_POINT('Ctrl Pts',(10.3767855209365,15.2,3.52022709143221));
#200635=CARTESIAN_POINT('Ctrl Pts',(10.3807035303564,15.2,3.52330583797949));
#200636=CARTESIAN_POINT('Ctrl Pts',(10.3846328295236,15.2,3.52640655624451));
#200637=CARTESIAN_POINT('Ctrl Pts',(10.3877762686004,15.2,3.52888713065374));
#200638=CARTESIAN_POINT('Ctrl Pts',(10.3909269342147,15.2,3.53138176766572));
#200639=CARTESIAN_POINT('Ctrl Pts',(10.3940846947336,15.2,3.5338904668481));
#200640=CARTESIAN_POINT('Ctrl Pts',(10.3972424556828,15.2,3.53639916637228));
#200641=CARTESIAN_POINT('Ctrl Pts',(10.4004073139604,15.2,3.53892192889499));
#200642=CARTESIAN_POINT('Ctrl Pts',(10.4035791394666,15.2,3.54145875303326));
#200643=CARTESIAN_POINT('Ctrl Pts',(10.4067509649728,15.2,3.54399557717152));
#200644=CARTESIAN_POINT('Ctrl Pts',(10.4099297590992,15.2,3.54654646280864));
#200645=CARTESIAN_POINT('Ctrl Pts',(10.4131153933291,15.2,3.54911141089431));
#200646=CARTESIAN_POINT('Ctrl Pts',(10.4163010271249,15.2,3.55167635863051));
#200647=CARTESIAN_POINT('Ctrl Pts',(10.4194935012003,15.2,3.55425536771787));
#200648=CARTESIAN_POINT('Ctrl Pts',(10.4226926897311,15.2,3.55684843623983));
#200649=CARTESIAN_POINT('Ctrl Pts',(10.4258918786977,15.2,3.55944150511511));
#200650=CARTESIAN_POINT('Ctrl Pts',(10.4290977829522,15.2,3.56204863528421));
#200651=CARTESIAN_POINT('Ctrl Pts',(10.4323102765168,15.2,3.5646698234285));
#200652=CARTESIAN_POINT('Ctrl Pts',(10.4355227696438,15.2,3.56729101121566));
#200653=CARTESIAN_POINT('Ctrl Pts',(10.4387418525837,15.2,3.56992625837041));
#200654=CARTESIAN_POINT('Ctrl Pts',(10.4419674009863,15.2,3.57257556154181));
#200655=CARTESIAN_POINT('Ctrl Pts',(10.4451929498283,15.2,3.57522486507418));
#200656=CARTESIAN_POINT('Ctrl Pts',(10.4484249642672,15.2,3.57788822689373));
#200657=CARTESIAN_POINT('Ctrl Pts',(10.4516633219949,15.2,3.58056564189685));
#200658=CARTESIAN_POINT('Ctrl Pts',(10.4549016792813,15.2,3.58324305653518));
#200659=CARTESIAN_POINT('Ctrl Pts',(10.4581463783143,15.2,3.58593452631486));
#200660=CARTESIAN_POINT('Ctrl Pts',(10.4613972999926,15.2,3.58864004803722));
#200661=CARTESIAN_POINT('Ctrl Pts',(10.4646482221138,15.2,3.59134557012821));
#200662=CARTESIAN_POINT('Ctrl Pts',(10.4679053641941,15.2,3.59406514435976));
#200663=CARTESIAN_POINT('Ctrl Pts',(10.4711686064834,15.2,3.59679876723187));
#200664=CARTESIAN_POINT('Ctrl Pts',(10.4744318483282,15.2,3.59953238973153));
#200665=CARTESIAN_POINT('Ctrl Pts',(10.4777011909821,15.2,3.60228006188829));
#200666=CARTESIAN_POINT('Ctrl Pts',(10.4809765142663,15.2,3.60504177913259));
#200667=CARTESIAN_POINT('Ctrl Pts',(10.4850706687063,15.2,3.60849392597017));
#200668=CARTESIAN_POINT('Ctrl Pts',(10.4891741670593,15.2,3.61196801906145));
#200669=CARTESIAN_POINT('Ctrl Pts',(10.4932867794893,15.2,3.61546405225475));
#200670=CARTESIAN_POINT('Ctrl Pts',(10.4965768696127,15.2,3.61826087896182));
#200671=CARTESIAN_POINT('Ctrl Pts',(10.4998727905118,15.2,3.62107174701222));
#200672=CARTESIAN_POINT('Ctrl Pts',(10.5031744268032,15.2,3.62389665122267));
#200673=CARTESIAN_POINT('Ctrl Pts',(10.5064760626448,15.2,3.62672155504822));
#200674=CARTESIAN_POINT('Ctrl Pts',(10.5097834127778,15.2,3.62956049679738));
#200675=CARTESIAN_POINT('Ctrl Pts',(10.5130963627276,15.2,3.63241347009436));
#200676=CARTESIAN_POINT('Ctrl Pts',(10.5164093131287,15.2,3.63526644378005));
#200677=CARTESIAN_POINT('Ctrl Pts',(10.5197278611485,15.2,3.63813345147489));
#200678=CARTESIAN_POINT('Ctrl Pts',(10.5230518914967,15.2,3.64101448624392));
#200679=CARTESIAN_POINT('Ctrl Pts',(10.5272069292055,15.2,3.64461577950895));
#200680=CARTESIAN_POINT('Ctrl Pts',(10.5313705333668,15.2,3.64823899082619));
#200681=CARTESIAN_POINT('Ctrl Pts',(10.5355424810062,15.2,3.65188411152179));
#200682=CARTESIAN_POINT('Ctrl Pts',(10.5388800388448,15.2,3.65480020783988));
#200683=CARTESIAN_POINT('Ctrl Pts',(10.5422229357793,15.2,3.65773032583704));
#200684=CARTESIAN_POINT('Ctrl Pts',(10.5455710585058,15.2,3.66067445913113));
#200685=CARTESIAN_POINT('Ctrl Pts',(10.5480821506647,15.2,3.66288255920198));
#200686=CARTESIAN_POINT('Ctrl Pts',(10.5505961827764,15.2,3.66509854378035));
#200687=CARTESIAN_POINT('Ctrl Pts',(10.5531131072262,15.2,3.66732240924013));
#200688=CARTESIAN_POINT('Ctrl Pts',(10.5556300321333,15.2,3.66954627510392));
#200689=CARTESIAN_POINT('Ctrl Pts',(10.5581498480828,15.2,3.67177802326162));
#200690=CARTESIAN_POINT('Ctrl Pts',(10.5606725095749,15.2,3.67401765050484));
#200691=CARTESIAN_POINT('Ctrl Pts',(10.5631951706086,15.2,3.6762572773412));
#200692=CARTESIAN_POINT('Ctrl Pts',(10.5657206764339,15.2,3.67850478199383));
#200693=CARTESIAN_POINT('Ctrl Pts',(10.5682489799672,15.2,3.68076016345423));
#200694=CARTESIAN_POINT('Ctrl Pts',(10.5707772835006,15.2,3.68301554491463));
#200695=CARTESIAN_POINT('Ctrl Pts',(10.5733083845828,15.2,3.68527880454083));
#200696=CARTESIAN_POINT('Ctrl Pts',(10.5758422375022,15.2,3.68754993646866));
#200697=CARTESIAN_POINT('Ctrl Pts',(10.5783760904217,15.2,3.68982106839649));
#200698=CARTESIAN_POINT('Ctrl Pts',(10.580912693095,15.2,3.6921000743706));
#200699=CARTESIAN_POINT('Ctrl Pts',(10.5834520019726,15.2,3.69438695075619));
#200700=CARTESIAN_POINT('Ctrl Pts',(10.5859913108502,15.2,3.69667382714178));
#200701=CARTESIAN_POINT('Ctrl Pts',(10.5885333233486,15.2,3.69896857466676));
#200702=CARTESIAN_POINT('Ctrl Pts',(10.5910779952976,15.2,3.70127118999908));
#200703=CARTESIAN_POINT('Ctrl Pts',(10.5944708915378,15.2,3.70434134405438));
#200704=CARTESIAN_POINT('Ctrl Pts',(10.5978685123674,15.2,3.70742548581691));
#200705=CARTESIAN_POINT('Ctrl Pts',(10.6012707520531,15.2,3.71052360798667));
#200706=CARTESIAN_POINT('Ctrl Pts',(10.6046729912753,15.2,3.7136217297343));
#200707=CARTESIAN_POINT('Ctrl Pts',(10.6080798480943,15.2,3.71673383070532));
#200708=CARTESIAN_POINT('Ctrl Pts',(10.6114912142633,15.2,3.71985990577139));
#200709=CARTESIAN_POINT('Ctrl Pts',(10.614902580897,15.2,3.72298598126339));
#200710=CARTESIAN_POINT('Ctrl Pts',(10.6183184581234,15.2,3.72612602937675));
#200711=CARTESIAN_POINT('Ctrl Pts',(10.6217387372546,15.2,3.72928004271624));
#200712=CARTESIAN_POINT('Ctrl Pts',(10.6243039463699,15.2,3.73164555250598));
#200713=CARTESIAN_POINT('Ctrl Pts',(10.6268716324766,15.2,3.73401891701978));
#200714=CARTESIAN_POINT('Ctrl Pts',(10.6294417504666,15.2,3.73640013430827));
#200715=CARTESIAN_POINT('Ctrl Pts',(10.6328685747645,15.2,3.73957509098132));
#200716=CARTESIAN_POINT('Ctrl Pts',(10.6362997213601,15.2,3.74276400716153));
#200717=CARTESIAN_POINT('Ctrl Pts',(10.6397350852699,15.2,3.74596687328194));
#200718=CARTESIAN_POINT('Ctrl Pts',(10.6431704487117,15.2,3.74916973896596));
#200719=CARTESIAN_POINT('Ctrl Pts',(10.6466100307746,15.2,3.75238655669723));
#200720=CARTESIAN_POINT('Ctrl Pts',(10.6500537247309,15.2,3.75561731578107));
#200721=CARTESIAN_POINT('Ctrl Pts',(10.6526364953155,15.2,3.75804038520399));
#200722=CARTESIAN_POINT('Ctrl Pts',(10.6552215796288,15.2,3.76047129735686));
#200723=CARTESIAN_POINT('Ctrl Pts',(10.6578089327429,15.2,3.76291004822591));
#200724=CARTESIAN_POINT('Ctrl Pts',(10.6603962858571,15.2,3.76534879909495));
#200725=CARTESIAN_POINT('Ctrl Pts',(10.6629859089127,15.2,3.76779538893845));
#200726=CARTESIAN_POINT('Ctrl Pts',(10.6655777579849,15.2,3.77024981422321));
#200727=CARTESIAN_POINT('Ctrl Pts',(10.668169607528,15.2,3.77270423995386));
#200728=CARTESIAN_POINT('Ctrl Pts',(10.6707636821883,15.2,3.7751665000117));
#200729=CARTESIAN_POINT('Ctrl Pts',(10.6733599393159,15.2,3.77763659178842));
#200730=CARTESIAN_POINT('Ctrl Pts',(10.6768216147,15.2,3.78093004674283));
#200731=CARTESIAN_POINT('Ctrl Pts',(10.6802871704613,15.2,3.78423742299263));
#200732=CARTESIAN_POINT('Ctrl Pts',(10.683756503733,15.2,3.78755871322021));
#200733=CARTESIAN_POINT('Ctrl Pts',(10.686358503805,15.2,3.79004968100403));
#200734=CARTESIAN_POINT('Ctrl Pts',(10.6889626283271,15.2,3.79254847424846));
#200735=CARTESIAN_POINT('Ctrl Pts',(10.6915688354874,15.2,3.79505508969837));
#200736=CARTESIAN_POINT('Ctrl Pts',(10.6941750426476,15.2,3.79756170514828));
#200737=CARTESIAN_POINT('Ctrl Pts',(10.696783330676,15.2,3.80007614262613));
#200738=CARTESIAN_POINT('Ctrl Pts',(10.6993936592059,15.2,3.80259839745008));
#200739=CARTESIAN_POINT('Ctrl Pts',(10.70200398821,15.2,3.80512065273224));
#200740=CARTESIAN_POINT('Ctrl Pts',(10.704616355923,15.2,3.80765072573329));
#200741=CARTESIAN_POINT('Ctrl Pts',(10.7072307205532,15.2,3.81018861201987));
#200742=CARTESIAN_POINT('Ctrl Pts',(10.7098450847085,15.2,3.81272649784541));
#200743=CARTESIAN_POINT('Ctrl Pts',(10.712461446147,15.2,3.81527219680382));
#200744=CARTESIAN_POINT('Ctrl Pts',(10.7150797622604,15.2,3.81782570600339));
#200745=CARTESIAN_POINT('Ctrl Pts',(10.7176980783737,15.2,3.82037921520297));
#200746=CARTESIAN_POINT('Ctrl Pts',(10.720318349219,15.2,3.82294053275057));
#200747=CARTESIAN_POINT('Ctrl Pts',(10.7229405337606,15.2,3.82550965554393));
#200748=CARTESIAN_POINT('Ctrl Pts',(10.7255627183023,15.2,3.82807877833729));
#200749=CARTESIAN_POINT('Ctrl Pts',(10.7281868148977,15.2,3.83065570584646));
#200750=CARTESIAN_POINT('Ctrl Pts',(10.7308127829809,15.2,3.83324043322259));
#200751=CARTESIAN_POINT('Ctrl Pts',(10.7343140740765,15.2,3.83668673670379));
#200752=CARTESIAN_POINT('Ctrl Pts',(10.737818690682,15.2,3.84014690793831));
#200753=CARTESIAN_POINT('Ctrl Pts',(10.7413265358735,15.2,3.84362093535128));
#200754=CARTESIAN_POINT('Ctrl Pts',(10.744834380587,15.2,3.84709496229092));
#200755=CARTESIAN_POINT('Ctrl Pts',(10.7483454538974,15.2,3.85058284616485));
#200756=CARTESIAN_POINT('Ctrl Pts',(10.751859659221,15.2,3.8540845744888));
#200757=CARTESIAN_POINT('Ctrl Pts',(10.7553738650234,15.2,3.85758630328985));
#200758=CARTESIAN_POINT('Ctrl Pts',(10.7588912026622,15.2,3.86110187746449));
#200759=CARTESIAN_POINT('Ctrl Pts',(10.7624115707524,15.2,3.86463128627882));
#200760=CARTESIAN_POINT('Ctrl Pts',(10.7650518465803,15.2,3.86727834264912));
#200761=CARTESIAN_POINT('Ctrl Pts',(10.7676938270174,15.2,3.86993317980302));
#200762=CARTESIAN_POINT('Ctrl Pts',(10.7703374732548,15.2,3.87259579408196));
#200763=CARTESIAN_POINT('Ctrl Pts',(10.7729811194922,15.2,3.87525840836091));
#200764=CARTESIAN_POINT('Ctrl Pts',(10.7756264323628,15.2,3.87792879866391));
#200765=CARTESIAN_POINT('Ctrl Pts',(10.7782733755166,15.2,3.88060696148326));
#200766=CARTESIAN_POINT('Ctrl Pts',(10.7809203186704,15.2,3.88328512430262));
#200767=CARTESIAN_POINT('Ctrl Pts',(10.7835688926242,15.2,3.88597105973833));
#200768=CARTESIAN_POINT('Ctrl Pts',(10.7862190496944,15.2,3.88866476197311));
#200769=CARTESIAN_POINT('Ctrl Pts',(10.7897525927757,15.2,3.89225636527905));
#200770=CARTESIAN_POINT('Ctrl Pts',(10.7932889486047,15.2,3.89586177510982));
#200771=CARTESIAN_POINT('Ctrl Pts',(10.7968280095302,15.2,3.89948097876684));
#200772=CARTESIAN_POINT('Ctrl Pts',(10.7994823049832,15.2,3.90219538126305));
#200773=CARTESIAN_POINT('Ctrl Pts',(10.8021381228242,15.2,3.90491754265944));
#200774=CARTESIAN_POINT('Ctrl Pts',(10.8047954450759,15.2,3.90764746004429));
#200775=CARTESIAN_POINT('Ctrl Pts',(10.8074527673276,15.2,3.91037737742914));
#200776=CARTESIAN_POINT('Ctrl Pts',(10.8101115945167,15.2,3.91311504950123));
#200777=CARTESIAN_POINT('Ctrl Pts',(10.8127719249999,15.2,3.91586047999999));
#200778=CARTESIAN_POINT('Ctrl Pts',(9.86852965799994,12.2,3.20199116299998));
#200779=CARTESIAN_POINT('Ctrl Pts',(9.87017542602826,12.2,3.2026865729514));
#200780=CARTESIAN_POINT('Ctrl Pts',(9.87187175395476,12.2,3.20340918505387));
#200781=CARTESIAN_POINT('Ctrl Pts',(9.87361750382533,12.2,3.20415921017613));
#200782=CARTESIAN_POINT('Ctrl Pts',(9.8753716725842,12.2,3.20491285229865));
#200783=CARTESIAN_POINT('Ctrl Pts',(9.87717573909119,12.2,3.20569417515048));
#200784=CARTESIAN_POINT('Ctrl Pts',(9.87902857820422,12.2,3.20650338931995));
#200785=CARTESIAN_POINT('Ctrl Pts',(9.88088141714894,12.2,3.20731260341592));
#200786=CARTESIAN_POINT('Ctrl Pts',(9.88278302753734,12.2,3.20814970993136));
#200787=CARTESIAN_POINT('Ctrl Pts',(9.88473231729986,12.2,3.20901491173327));
#200788=CARTESIAN_POINT('Ctrl Pts',(9.88668160706237,12.2,3.20988011353516));
#200789=CARTESIAN_POINT('Ctrl Pts',(9.88867857432713,12.2,3.21077340710827));
#200790=CARTESIAN_POINT('Ctrl Pts',(9.89072215651895,12.2,3.21169499186919));
#200791=CARTESIAN_POINT('Ctrl Pts',(9.8927657388964,12.2,3.21261657671382));
#200792=CARTESIAN_POINT('Ctrl Pts',(9.89485593697986,12.2,3.21356644793466));
#200793=CARTESIAN_POINT('Ctrl Pts',(9.89699171626601,12.2,3.21454479382324));
#200794=CARTESIAN_POINT('Ctrl Pts',(9.89912749535818,12.2,3.21552313962297));
#200795=CARTESIAN_POINT('Ctrl Pts',(9.90130885312988,12.2,3.2165299600416));
#200796=CARTESIAN_POINT('Ctrl Pts',(9.90353478647588,12.2,3.21756543175874));
#200797=CARTESIAN_POINT('Ctrl Pts',(9.90576071982188,12.2,3.21860090347588));
#200798=CARTESIAN_POINT('Ctrl Pts',(9.90803122617659,12.2,3.21966502636479));
#200799=CARTESIAN_POINT('Ctrl Pts',(9.9103453265906,12.2,3.22075797015716));
#200800=CARTESIAN_POINT('Ctrl Pts',(9.91265942721481,12.2,3.22185091404879));
#200801=CARTESIAN_POINT('Ctrl Pts',(9.91501712121113,12.2,3.22297268105235));
#200802=CARTESIAN_POINT('Ctrl Pts',(9.91741745401152,12.2,3.22412343086704));
#200803=CARTESIAN_POINT('Ctrl Pts',(9.91981778659389,12.2,3.2252741805772));
#200804=CARTESIAN_POINT('Ctrl Pts',(9.9222607575406,12.2,3.22645391462526));
#200805=CARTESIAN_POINT('Ctrl Pts',(9.9247454351188,12.2,3.22766278908261));
#200806=CARTESIAN_POINT('Ctrl Pts',(9.92723011269699,12.2,3.22887166353995));
#200807=CARTESIAN_POINT('Ctrl Pts',(9.92975649721356,12.2,3.23010967684499));
#200808=CARTESIAN_POINT('Ctrl Pts',(9.93232368086846,12.2,3.23137697863099));
#200809=CARTESIAN_POINT('Ctrl Pts',(9.93489086452338,12.2,3.23264428041699));
#200810=CARTESIAN_POINT('Ctrl Pts',(9.93749884761017,12.2,3.23394087148892));
#200811=CARTESIAN_POINT('Ctrl Pts',(9.94014674251127,12.2,3.2352668931054));
#200812=CARTESIAN_POINT('Ctrl Pts',(9.94279463765287,12.2,3.23659291484234));
#200813=CARTESIAN_POINT('Ctrl Pts',(9.94548244668999,12.2,3.23794836711543));
#200814=CARTESIAN_POINT('Ctrl Pts',(9.94820930192366,12.2,3.23933338685888));
#200815=CARTESIAN_POINT('Ctrl Pts',(9.95093615690962,12.2,3.24071840647652));
#200816=CARTESIAN_POINT('Ctrl Pts',(9.95370205967116,12.2,3.24213299372027));
#200817=CARTESIAN_POINT('Ctrl Pts',(9.9565061647486,12.2,3.24357727725761));
#200818=CARTESIAN_POINT('Ctrl Pts',(9.95931026982602,12.2,3.24502156079496));
#200819=CARTESIAN_POINT('Ctrl Pts',(9.96215257705149,12.2,3.2464955419427));
#200820=CARTESIAN_POINT('Ctrl Pts',(9.96503226119433,12.2,3.24799934355269));
#200821=CARTESIAN_POINT('Ctrl Pts',(9.96791194559875,12.2,3.24950314529928));
#200822=CARTESIAN_POINT('Ctrl Pts',(9.97082900750678,12.2,3.25103676921541));
#200823=CARTESIAN_POINT('Ctrl Pts',(9.97378263891934,12.2,3.25260033280194));
#200824=CARTESIAN_POINT('Ctrl Pts',(9.97673627006362,12.2,3.25416389624644));
#200825=CARTESIAN_POINT('Ctrl Pts',(9.97972647011979,12.2,3.25575739949255));
#200826=CARTESIAN_POINT('Ctrl Pts',(9.98275245044018,12.2,3.25738095602419));
#200827=CARTESIAN_POINT('Ctrl Pts',(9.98577843076056,12.2,3.25900451255585));
#200828=CARTESIAN_POINT('Ctrl Pts',(9.98884019302724,12.2,3.2606581238213));
#200829=CARTESIAN_POINT('Ctrl Pts',(9.99193696241234,12.2,3.26234189434141));
#200830=CARTESIAN_POINT('Ctrl Pts',(9.99503373207875,12.2,3.26402566501445));
#200831=CARTESIAN_POINT('Ctrl Pts',(9.99816550995689,12.2,3.26573959779312));
#200832=CARTESIAN_POINT('Ctrl Pts',(10.0013315407896,12.2,3.26748379539373));
#200833=CARTESIAN_POINT('Ctrl Pts',(10.0044975713347,12.2,3.26922799283592));
#200834=CARTESIAN_POINT('Ctrl Pts',(10.0076978547174,12.2,3.27100245274884));
#200835=CARTESIAN_POINT('Ctrl Pts',(10.0109316502666,12.2,3.27280727701659));
#200836=CARTESIAN_POINT('Ctrl Pts',(10.0141654458157,12.2,3.27461210128435));
#200837=CARTESIAN_POINT('Ctrl Pts',(10.0174327549627,12.2,3.27644728646254));
#200838=CARTESIAN_POINT('Ctrl Pts',(10.0207328509224,12.2,3.27831292881953));
#200839=CARTESIAN_POINT('Ctrl Pts',(10.0240329471819,12.2,3.28017857134599));
#200840=CARTESIAN_POINT('Ctrl Pts',(10.0273658333144,12.2,3.28207466795285));
#200841=CARTESIAN_POINT('Ctrl Pts',(10.0307307963333,12.2,3.28400131139327));
#200842=CARTESIAN_POINT('Ctrl Pts',(10.0340957590466,12.2,3.28592795465869));
#200843=CARTESIAN_POINT('Ctrl Pts',(10.0374928008687,12.2,3.2878851426723));
#200844=CARTESIAN_POINT('Ctrl Pts',(10.0409212255098,12.2,3.28987295902584));
#200845=CARTESIAN_POINT('Ctrl Pts',(10.0443496501508,12.2,3.29186077537937));
#200846=CARTESIAN_POINT('Ctrl Pts',(10.0478094545213,12.2,3.29387922191417));
#200847=CARTESIAN_POINT('Ctrl Pts',(10.0512999620598,12.2,3.29592837717172));
#200848=CARTESIAN_POINT('Ctrl Pts',(10.0542087184476,12.2,3.29763600661505));
#200849=CARTESIAN_POINT('Ctrl Pts',(10.0571387936914,12.2,3.29936496256449));
#200850=CARTESIAN_POINT('Ctrl Pts',(10.0600898020237,12.2,3.30111528791059));
#200851=CARTESIAN_POINT('Ctrl Pts',(10.0630408103559,12.2,3.30286561325669));
#200852=CARTESIAN_POINT('Ctrl Pts',(10.0660127511514,12.2,3.30463730991309));
#200853=CARTESIAN_POINT('Ctrl Pts',(10.0690052419983,12.2,3.30643041853229));
#200854=CARTESIAN_POINT('Ctrl Pts',(10.0719977328451,12.2,3.30822352715149));
#200855=CARTESIAN_POINT('Ctrl Pts',(10.0750107736166,12.2,3.31003804840549));
#200856=CARTESIAN_POINT('Ctrl Pts',(10.0780439902832,12.2,3.3118740220166));
#200857=CARTESIAN_POINT('Ctrl Pts',(10.0810772069499,12.2,3.31370999562771));
#200858=CARTESIAN_POINT('Ctrl Pts',(10.0841305984486,12.2,3.31556742342013));
#200859=CARTESIAN_POINT('Ctrl Pts',(10.0872037952682,12.2,3.31744634127596));
#200860=CARTESIAN_POINT('Ctrl Pts',(10.0902769920878,12.2,3.31932525913178));
#200861=CARTESIAN_POINT('Ctrl Pts',(10.0933699950748,12.2,3.32122566901908));
#200862=CARTESIAN_POINT('Ctrl Pts',(10.0964824384786,12.2,3.32314760686743));
#200863=CARTESIAN_POINT('Ctrl Pts',(10.0995948818824,12.2,3.32506954471577));
#200864=CARTESIAN_POINT('Ctrl Pts',(10.1027267670162,12.2,3.32701301044966));
#200865=CARTESIAN_POINT('Ctrl Pts',(10.1058777331978,12.2,3.32897803989524));
#200866=CARTESIAN_POINT('Ctrl Pts',(10.1090286993793,12.2,3.33094306934082));
#200867=CARTESIAN_POINT('Ctrl Pts',(10.1121987494873,12.2,3.33292966206464));
#200868=CARTESIAN_POINT('Ctrl Pts',(10.1153875281201,12.2,3.33493785154146));
#200869=CARTESIAN_POINT('Ctrl Pts',(10.118576306753,12.2,3.33694604101829));
#200870=CARTESIAN_POINT('Ctrl Pts',(10.1217838154981,12.2,3.33897582624982));
#200871=CARTESIAN_POINT('Ctrl Pts',(10.1250097041802,12.2,3.34102723979325));
#200872=CARTESIAN_POINT('Ctrl Pts',(10.1282355928622,12.2,3.3430786533367));
#200873=CARTESIAN_POINT('Ctrl Pts',(10.1314798631418,12.2,3.34515169548326));
#200874=CARTESIAN_POINT('Ctrl Pts',(10.1347421716849,12.2,3.34724639499893));
#200875=CARTESIAN_POINT('Ctrl Pts',(10.1380044798725,12.2,3.34934109428628));
#200876=CARTESIAN_POINT('Ctrl Pts',(10.1412848258294,12.2,3.35145745274398));
#200877=CARTESIAN_POINT('Ctrl Pts',(10.1445828723435,12.2,3.35359549695362));
#200878=CARTESIAN_POINT('Ctrl Pts',(10.1478809192171,12.2,3.35573354139629));
#200879=CARTESIAN_POINT('Ctrl Pts',(10.1511966652375,12.2,3.35789327308303));
#200880=CARTESIAN_POINT('Ctrl Pts',(10.1545297780139,12.2,3.36007471745627));
#200881=CARTESIAN_POINT('Ctrl Pts',(10.1578628907903,12.2,3.36225616182951));
#200882=CARTESIAN_POINT('Ctrl Pts',(10.1612133712775,12.2,3.3644593193885));
#200883=CARTESIAN_POINT('Ctrl Pts',(10.1645808898178,12.2,3.36668421619226));
#200884=CARTESIAN_POINT('Ctrl Pts',(10.167948408358,12.2,3.36890911299601));
#200885=CARTESIAN_POINT('Ctrl Pts',(10.171332964403,12.2,3.37115574858598));
#200886=CARTESIAN_POINT('Ctrl Pts',(10.1747342341551,12.2,3.37342414571168));
#200887=CARTESIAN_POINT('Ctrl Pts',(10.1781355039072,12.2,3.37569254283738));
#200888=CARTESIAN_POINT('Ctrl Pts',(10.1815534883263,12.2,3.37798270380001));
#200889=CARTESIAN_POINT('Ctrl Pts',(10.1849878670754,12.2,3.38029464963219));
#200890=CARTESIAN_POINT('Ctrl Pts',(10.1884222458245,12.2,3.38260659546438));
#200891=CARTESIAN_POINT('Ctrl Pts',(10.1918730184574,12.2,3.38494032500271));
#200892=CARTESIAN_POINT('Ctrl Pts',(10.1953398705399,12.2,3.38729586111267));
#200893=CARTESIAN_POINT('Ctrl Pts',(10.1981133523571,12.2,3.38918029010334));
#200894=CARTESIAN_POINT('Ctrl Pts',(10.2008971258154,12.2,3.39107867539597));
#200895=CARTESIAN_POINT('Ctrl Pts',(10.2036910291637,12.2,3.39299102631917));
#200896=CARTESIAN_POINT('Ctrl Pts',(10.2064849321313,12.2,3.3949033769818));
#200897=CARTESIAN_POINT('Ctrl Pts',(10.2092889672229,12.2,3.39682969297042));
#200898=CARTESIAN_POINT('Ctrl Pts',(10.2121029747699,12.2,3.39876998486644));
#200899=CARTESIAN_POINT('Ctrl Pts',(10.2149169827004,12.2,3.40071027702682));
#200900=CARTESIAN_POINT('Ctrl Pts',(10.2177409643432,12.2,3.40266454405278));
#200901=CARTESIAN_POINT('Ctrl Pts',(10.2205747634983,12.2,3.40463279616097));
#200902=CARTESIAN_POINT('Ctrl Pts',(10.2234085622673,12.2,3.40660104800098));
#200903=CARTESIAN_POINT('Ctrl Pts',(10.2262521773969,12.2,3.40858328336113));
#200904=CARTESIAN_POINT('Ctrl Pts',(10.2291054563609,12.2,3.41057951268534));
#200905=CARTESIAN_POINT('Ctrl Pts',(10.2319587357137,12.2,3.41257574228154));
#200906=CARTESIAN_POINT('Ctrl Pts',(10.2348216774777,12.2,3.41458596461265));
#200907=CARTESIAN_POINT('Ctrl Pts',(10.2376941293015,12.2,3.41661018689054));
#200908=CARTESIAN_POINT('Ctrl Pts',(10.2405665807339,12.2,3.41863440889263));
#200909=CARTESIAN_POINT('Ctrl Pts',(10.2434485414701,12.2,3.42067263263917));
#200910=CARTESIAN_POINT('Ctrl Pts',(10.2463398610105,12.2,3.4227248639144));
#200911=CARTESIAN_POINT('Ctrl Pts',(10.2492311809449,12.2,3.42477709546924));
#200912=CARTESIAN_POINT('Ctrl Pts',(10.252131859969,12.2,3.42684333603682));
#200913=CARTESIAN_POINT('Ctrl Pts',(10.2550417472519,12.2,3.42892359099302));
#200914=CARTESIAN_POINT('Ctrl Pts',(10.2579516341384,12.2,3.43100384566577));
#200915=CARTESIAN_POINT('Ctrl Pts',(10.2608707290809,12.2,3.43309811621235));
#200916=CARTESIAN_POINT('Ctrl Pts',(10.2637988852295,12.2,3.43520640737189));
#200917=CARTESIAN_POINT('Ctrl Pts',(10.266727041777,12.2,3.43731469881869));
#200918=CARTESIAN_POINT('Ctrl Pts',(10.2696642586838,12.2,3.43943701172515));
#200919=CARTESIAN_POINT('Ctrl Pts',(10.2726103887332,12.2,3.44157335200826));
#200920=CARTESIAN_POINT('Ctrl Pts',(10.2755565187827,12.2,3.44370969229137));
#200921=CARTESIAN_POINT('Ctrl Pts',(10.2785115630943,12.2,3.44586006162332));
#200922=CARTESIAN_POINT('Ctrl Pts',(10.2814753757012,12.2,3.44802446185382));
#200923=CARTESIAN_POINT('Ctrl Pts',(10.2844391879042,12.2,3.45018886178941));
#200924=CARTESIAN_POINT('Ctrl Pts',(10.2874117675698,12.2,3.45236729555388));
#200925=CARTESIAN_POINT('Ctrl Pts',(10.2903929725062,12.2,3.45455976677344));
#200926=CARTESIAN_POINT('Ctrl Pts',(10.2933741778489,12.2,3.45675223829172));
#200927=CARTESIAN_POINT('Ctrl Pts',(10.296364006512,12.2,3.45895874696276));
#200928=CARTESIAN_POINT('Ctrl Pts',(10.2993623177318,12.2,3.461179297863));
#200929=CARTESIAN_POINT('Ctrl Pts',(10.3023606285431,12.2,3.46339984846069));
#200930=CARTESIAN_POINT('Ctrl Pts',(10.3053674207616,12.2,3.46563444186764));
#200931=CARTESIAN_POINT('Ctrl Pts',(10.3083825537368,12.2,3.46788308101624));
#200932=CARTESIAN_POINT('Ctrl Pts',(10.3113976871228,12.2,3.4701317204712));
#200933=CARTESIAN_POINT('Ctrl Pts',(10.3144211607142,12.2,3.47239440649412));
#200934=CARTESIAN_POINT('Ctrl Pts',(10.3174528361982,12.2,3.47467114212204));
#200935=CARTESIAN_POINT('Ctrl Pts',(10.3204845112692,12.2,3.47694787743977));
#200936=CARTESIAN_POINT('Ctrl Pts',(10.3235243854922,12.2,3.47923866205654));
#200937=CARTESIAN_POINT('Ctrl Pts',(10.3265723237425,12.2,3.48154349931164));
#200938=CARTESIAN_POINT('Ctrl Pts',(10.329620262408,12.2,3.48384833688077));
#200939=CARTESIAN_POINT('Ctrl Pts',(10.3326762624274,12.2,3.48616722819883));
#200940=CARTESIAN_POINT('Ctrl Pts',(10.3357401884838,12.2,3.48850017438245));
#200941=CARTESIAN_POINT('Ctrl Pts',(10.3388041141227,12.2,3.49083312024821));
#200942=CARTESIAN_POINT('Ctrl Pts',(10.3418759651823,12.2,3.49318012216704));
#200943=CARTESIAN_POINT('Ctrl Pts',(10.3449556050281,12.2,3.49554118142408));
#200944=CARTESIAN_POINT('Ctrl Pts',(10.3480352452935,12.2,3.4979022410028));
#200945=CARTESIAN_POINT('Ctrl Pts',(10.3511226752616,12.2,3.50027735818093));
#200946=CARTESIAN_POINT('Ctrl Pts',(10.3542177599863,12.2,3.50266653497871));
#200947=CARTESIAN_POINT('Ctrl Pts',(10.3573128442894,12.2,3.50505571145097));
#200948=CARTESIAN_POINT('Ctrl Pts',(10.3604155820853,12.2,3.50745894693709));
#200949=CARTESIAN_POINT('Ctrl Pts',(10.3635258429414,12.2,3.50987624340471));
#200950=CARTESIAN_POINT('Ctrl Pts',(10.3666361042213,12.2,3.51229354020168));
#200951=CARTESIAN_POINT('Ctrl Pts',(10.3697538852342,12.2,3.51472489777384));
#200952=CARTESIAN_POINT('Ctrl Pts',(10.372879056752,12.2,3.5171703172516));
#200953=CARTESIAN_POINT('Ctrl Pts',(10.3760042278441,12.2,3.51961573639617));
#200954=CARTESIAN_POINT('Ctrl Pts',(10.3791367876884,12.2,3.52207521810194));
#200955=CARTESIAN_POINT('Ctrl Pts',(10.3822766059866,12.2,3.52454876128718));
#200956=CARTESIAN_POINT('Ctrl Pts',(10.3854164247125,12.2,3.52702230480944));
#200957=CARTESIAN_POINT('Ctrl Pts',(10.3885635015752,12.2,3.5295099105108));
#200958=CARTESIAN_POINT('Ctrl Pts',(10.3917177070249,12.2,3.53201157925826));
#200959=CARTESIAN_POINT('Ctrl Pts',(10.3956604636221,12.2,3.53513866502214));
#200960=CARTESIAN_POINT('Ctrl Pts',(10.3996143577999,12.2,3.53828772303325));
#200961=CARTESIAN_POINT('Ctrl Pts',(10.4035791394666,12.2,3.54145875303325));
#200962=CARTESIAN_POINT('Ctrl Pts',(10.4067509649728,12.2,3.54399557717152));
#200963=CARTESIAN_POINT('Ctrl Pts',(10.4099297590992,12.2,3.54654646280864));
#200964=CARTESIAN_POINT('Ctrl Pts',(10.4131153933291,12.2,3.54911141089431));
#200965=CARTESIAN_POINT('Ctrl Pts',(10.4163010271249,12.2,3.55167635863051));
#200966=CARTESIAN_POINT('Ctrl Pts',(10.4194935012003,12.2,3.55425536771786));
#200967=CARTESIAN_POINT('Ctrl Pts',(10.4226926897311,12.2,3.55684843623983));
#200968=CARTESIAN_POINT('Ctrl Pts',(10.4258918786977,12.2,3.55944150511511));
#200969=CARTESIAN_POINT('Ctrl Pts',(10.4290977829522,12.2,3.56204863528421));
#200970=CARTESIAN_POINT('Ctrl Pts',(10.4323102765168,12.2,3.5646698234285));
#200971=CARTESIAN_POINT('Ctrl Pts',(10.4355227696438,12.2,3.56729101121566));
#200972=CARTESIAN_POINT('Ctrl Pts',(10.4387418525837,12.2,3.56992625837041));
#200973=CARTESIAN_POINT('Ctrl Pts',(10.4419674009863,12.2,3.57257556154181));
#200974=CARTESIAN_POINT('Ctrl Pts',(10.4451929498283,12.2,3.57522486507418));
#200975=CARTESIAN_POINT('Ctrl Pts',(10.4484249642672,12.2,3.57788822689373));
#200976=CARTESIAN_POINT('Ctrl Pts',(10.4516633219949,12.2,3.58056564189685));
#200977=CARTESIAN_POINT('Ctrl Pts',(10.4549016792813,12.2,3.58324305653518));
#200978=CARTESIAN_POINT('Ctrl Pts',(10.4581463783143,12.2,3.58593452631486));
#200979=CARTESIAN_POINT('Ctrl Pts',(10.4613972999926,12.2,3.58864004803722));
#200980=CARTESIAN_POINT('Ctrl Pts',(10.4646482221138,12.2,3.59134557012821));
#200981=CARTESIAN_POINT('Ctrl Pts',(10.4679053641941,12.2,3.59406514435976));
#200982=CARTESIAN_POINT('Ctrl Pts',(10.4711686064834,12.2,3.59679876723187));
#200983=CARTESIAN_POINT('Ctrl Pts',(10.4744318483282,12.2,3.59953238973153));
#200984=CARTESIAN_POINT('Ctrl Pts',(10.4777011909821,12.2,3.60228006188829));
#200985=CARTESIAN_POINT('Ctrl Pts',(10.4809765142663,12.2,3.60504177913259));
#200986=CARTESIAN_POINT('Ctrl Pts',(10.4850706687063,12.2,3.60849392597017));
#200987=CARTESIAN_POINT('Ctrl Pts',(10.4891741670593,12.2,3.61196801906145));
#200988=CARTESIAN_POINT('Ctrl Pts',(10.4932867794893,12.2,3.61546405225475));
#200989=CARTESIAN_POINT('Ctrl Pts',(10.4965768696127,12.2,3.61826087896182));
#200990=CARTESIAN_POINT('Ctrl Pts',(10.4998727905118,12.2,3.62107174701222));
#200991=CARTESIAN_POINT('Ctrl Pts',(10.5031744268032,12.2,3.62389665122267));
#200992=CARTESIAN_POINT('Ctrl Pts',(10.5064760626448,12.2,3.62672155504822));
#200993=CARTESIAN_POINT('Ctrl Pts',(10.5097834127778,12.2,3.62956049679738));
#200994=CARTESIAN_POINT('Ctrl Pts',(10.5130963627276,12.2,3.63241347009436));
#200995=CARTESIAN_POINT('Ctrl Pts',(10.5164093131287,12.2,3.63526644378005));
#200996=CARTESIAN_POINT('Ctrl Pts',(10.5197278611485,12.2,3.63813345147488));
#200997=CARTESIAN_POINT('Ctrl Pts',(10.5230518914967,12.2,3.64101448624392));
#200998=CARTESIAN_POINT('Ctrl Pts',(10.5272069292055,12.2,3.64461577950895));
#200999=CARTESIAN_POINT('Ctrl Pts',(10.5313705333668,12.2,3.64823899082619));
#201000=CARTESIAN_POINT('Ctrl Pts',(10.5355424810062,12.2,3.65188411152179));
#201001=CARTESIAN_POINT('Ctrl Pts',(10.5388800388448,12.2,3.65480020783988));
#201002=CARTESIAN_POINT('Ctrl Pts',(10.5422229357793,12.2,3.65773032583704));
#201003=CARTESIAN_POINT('Ctrl Pts',(10.5455710585058,12.2,3.66067445913113));
#201004=CARTESIAN_POINT('Ctrl Pts',(10.5480821506647,12.2,3.66288255920198));
#201005=CARTESIAN_POINT('Ctrl Pts',(10.5505961827764,12.2,3.66509854378035));
#201006=CARTESIAN_POINT('Ctrl Pts',(10.5531131072262,12.2,3.66732240924013));
#201007=CARTESIAN_POINT('Ctrl Pts',(10.5556300321333,12.2,3.66954627510392));
#201008=CARTESIAN_POINT('Ctrl Pts',(10.5581498480828,12.2,3.67177802326162));
#201009=CARTESIAN_POINT('Ctrl Pts',(10.5606725095749,12.2,3.67401765050484));
#201010=CARTESIAN_POINT('Ctrl Pts',(10.5631951706086,12.2,3.6762572773412));
#201011=CARTESIAN_POINT('Ctrl Pts',(10.5657206764339,12.2,3.67850478199383));
#201012=CARTESIAN_POINT('Ctrl Pts',(10.5682489799672,12.2,3.68076016345423));
#201013=CARTESIAN_POINT('Ctrl Pts',(10.5707772835006,12.2,3.68301554491463));
#201014=CARTESIAN_POINT('Ctrl Pts',(10.5733083845828,12.2,3.68527880454083));
#201015=CARTESIAN_POINT('Ctrl Pts',(10.5758422375022,12.2,3.68754993646866));
#201016=CARTESIAN_POINT('Ctrl Pts',(10.5792207079081,12.2,3.6905781122349));
#201017=CARTESIAN_POINT('Ctrl Pts',(10.5826040686401,12.2,3.6936202858821));
#201018=CARTESIAN_POINT('Ctrl Pts',(10.5859922100293,12.2,3.69667645024192));
#201019=CARTESIAN_POINT('Ctrl Pts',(10.5885333166482,12.2,3.69896857403229));
#201020=CARTESIAN_POINT('Ctrl Pts',(10.5910771131846,12.2,3.70126856814991));
#201021=CARTESIAN_POINT('Ctrl Pts',(10.5936235522634,12.2,3.70357642852805));
#201022=CARTESIAN_POINT('Ctrl Pts',(10.5970188035974,12.2,3.70665357500014));
#201023=CARTESIAN_POINT('Ctrl Pts',(10.6004187539281,12.2,3.70974470865931));
#201024=CARTESIAN_POINT('Ctrl Pts',(10.603823295205,12.2,3.71284982023789));
#201025=CARTESIAN_POINT('Ctrl Pts',(10.6063767012787,12.2,3.71517865402759));
#201026=CARTESIAN_POINT('Ctrl Pts',(10.6089326895204,12.2,3.71751534936536));
#201027=CARTESIAN_POINT('Ctrl Pts',(10.6114912142633,12.2,3.71985990577139));
#201028=CARTESIAN_POINT('Ctrl Pts',(10.6140497390062,12.2,3.72220446217743));
#201029=CARTESIAN_POINT('Ctrl Pts',(10.6166108013512,12.2,3.72455687838889));
#201030=CARTESIAN_POINT('Ctrl Pts',(10.6191743544661,12.2,3.72691715076039));
#201031=CARTESIAN_POINT('Ctrl Pts',(10.6217379080466,12.2,3.72927742356068));
#201032=CARTESIAN_POINT('Ctrl Pts',(10.6243039532362,12.2,3.73164555263819));
#201033=CARTESIAN_POINT('Ctrl Pts',(10.6268724453182,12.2,3.7340215349429));
#201034=CARTESIAN_POINT('Ctrl Pts',(10.6294409369336,12.2,3.73639751681597));
#201035=CARTESIAN_POINT('Ctrl Pts',(10.6320118751237,12.2,3.73878135223031));
#201036=CARTESIAN_POINT('Ctrl Pts',(10.6345852151971,12.2,3.74117303751909));
#201037=CARTESIAN_POINT('Ctrl Pts',(10.6371585552705,12.2,3.74356472280788));
#201038=CARTESIAN_POINT('Ctrl Pts',(10.6397342970009,12.2,3.74596425732862));
#201039=CARTESIAN_POINT('Ctrl Pts',(10.6423123970023,12.2,3.74837163775212));
#201040=CARTESIAN_POINT('Ctrl Pts',(10.6448904970036,12.2,3.75077901817562));
#201041=CARTESIAN_POINT('Ctrl Pts',(10.6474709541464,12.2,3.75319424635814));
#201042=CARTESIAN_POINT('Ctrl Pts',(10.6500537247309,12.2,3.75561731578107));
#201043=CARTESIAN_POINT('Ctrl Pts',(10.6526364953155,12.2,3.75804038520399));
#201044=CARTESIAN_POINT('Ctrl Pts',(10.6552215796288,12.2,3.76047129735686));
#201045=CARTESIAN_POINT('Ctrl Pts',(10.6578089327429,12.2,3.76291004822591));
#201046=CARTESIAN_POINT('Ctrl Pts',(10.6603962858571,12.2,3.76534879909495));
#201047=CARTESIAN_POINT('Ctrl Pts',(10.6629859089127,12.2,3.76779538893845));
#201048=CARTESIAN_POINT('Ctrl Pts',(10.6655777579849,12.2,3.77024981422321));
#201049=CARTESIAN_POINT('Ctrl Pts',(10.668169607528,12.2,3.77270423995386));
#201050=CARTESIAN_POINT('Ctrl Pts',(10.6707636821883,12.2,3.7751665000117));
#201051=CARTESIAN_POINT('Ctrl Pts',(10.6733599393159,12.2,3.77763659178842));
#201052=CARTESIAN_POINT('Ctrl Pts',(10.6759561959719,12.2,3.78010668311641));
#201053=CARTESIAN_POINT('Ctrl Pts',(10.6785546353944,12.2,3.78258460559397));
#201054=CARTESIAN_POINT('Ctrl Pts',(10.6811552140084,12.2,3.78507035500434));
#201055=CARTESIAN_POINT('Ctrl Pts',(10.6837557926225,12.2,3.78755610441471));
#201056=CARTESIAN_POINT('Ctrl Pts',(10.6863585103684,12.2,3.79004968258171));
#201057=CARTESIAN_POINT('Ctrl Pts',(10.688963324494,12.2,3.79255108254387));
#201058=CARTESIAN_POINT('Ctrl Pts',(10.6915681386195,12.2,3.79505248250604));
#201059=CARTESIAN_POINT('Ctrl Pts',(10.6941750490305,12.2,3.79756170681105));
#201060=CARTESIAN_POINT('Ctrl Pts',(10.6967840126976,12.2,3.80007874923098));
#201061=CARTESIAN_POINT('Ctrl Pts',(10.6993929763646,12.2,3.80259579165091));
#201062=CARTESIAN_POINT('Ctrl Pts',(10.7020039945769,12.2,3.80512065363337));
#201063=CARTESIAN_POINT('Ctrl Pts',(10.7046170227318,12.2,3.807653329999));
#201064=CARTESIAN_POINT('Ctrl Pts',(10.7072300508867,12.2,3.81018600636464));
#201065=CARTESIAN_POINT('Ctrl Pts',(10.7098450902914,12.2,3.8127264975214));
#201066=CARTESIAN_POINT('Ctrl Pts',(10.7124620984461,12.2,3.81527479942774));
#201067=CARTESIAN_POINT('Ctrl Pts',(10.7150791070762,12.2,3.81782310179702));
#201068=CARTESIAN_POINT('Ctrl Pts',(10.7176980844068,12.2,3.82037921566852));
#201069=CARTESIAN_POINT('Ctrl Pts',(10.720318989038,12.2,3.82294313500054));
#201070=CARTESIAN_POINT('Ctrl Pts',(10.722939893193,12.2,3.82550705386679));
#201071=CARTESIAN_POINT('Ctrl Pts',(10.7255627249218,12.2,3.82807877957969));
#201072=CARTESIAN_POINT('Ctrl Pts',(10.7281874407494,12.2,3.83065830653241));
#201073=CARTESIAN_POINT('Ctrl Pts',(10.7308121565771,12.2,3.83323783348514));
#201074=CARTESIAN_POINT('Ctrl Pts',(10.7334387577985,12.2,3.83582516192653));
#201075=CARTESIAN_POINT('Ctrl Pts',(10.7360672015365,12.2,3.83842028779126));
#201076=CARTESIAN_POINT('Ctrl Pts',(10.739571793028,12.2,3.84188045545376));
#201077=CARTESIAN_POINT('Ctrl Pts',(10.7430796621271,12.2,3.84535448505789));
#201078=CARTESIAN_POINT('Ctrl Pts',(10.7465907114509,12.2,3.848842365938));
#201079=CARTESIAN_POINT('Ctrl Pts',(10.7492239990417,12.2,3.85145827719211));
#201080=CARTESIAN_POINT('Ctrl Pts',(10.7518590756913,12.2,3.85408197924009));
#201081=CARTESIAN_POINT('Ctrl Pts',(10.7544958998248,12.2,3.85671346754028));
#201082=CARTESIAN_POINT('Ctrl Pts',(10.7571327234792,12.2,3.8593449553624));
#201083=CARTESIAN_POINT('Ctrl Pts',(10.7597712949246,12.2,3.86198422990851));
#201084=CARTESIAN_POINT('Ctrl Pts',(10.7624115707524,12.2,3.86463128627882));
#201085=CARTESIAN_POINT('Ctrl Pts',(10.7650518465803,12.2,3.86727834264912));
#201086=CARTESIAN_POINT('Ctrl Pts',(10.7676938270174,12.2,3.86993317980302));
#201087=CARTESIAN_POINT('Ctrl Pts',(10.7703374732548,12.2,3.87259579408196));
#201088=CARTESIAN_POINT('Ctrl Pts',(10.7729811194922,12.2,3.8752584083609));
#201089=CARTESIAN_POINT('Ctrl Pts',(10.7756264323628,12.2,3.87792879866391));
#201090=CARTESIAN_POINT('Ctrl Pts',(10.7782733755166,12.2,3.88060696148326));
#201091=CARTESIAN_POINT('Ctrl Pts',(10.7809203186704,12.2,3.88328512430262));
#201092=CARTESIAN_POINT('Ctrl Pts',(10.7835688926242,12.2,3.88597105973833));
#201093=CARTESIAN_POINT('Ctrl Pts',(10.7862190496944,12.2,3.88866476197311));
#201094=CARTESIAN_POINT('Ctrl Pts',(10.7888692067647,12.2,3.89135846420789));
#201095=CARTESIAN_POINT('Ctrl Pts',(10.7915209471673,12.2,3.89405993233984));
#201096=CARTESIAN_POINT('Ctrl Pts',(10.7941742224949,12.2,3.89676916175084));
#201097=CARTESIAN_POINT('Ctrl Pts',(10.7968274978226,12.2,3.89947839116184));
#201098=CARTESIAN_POINT('Ctrl Pts',(10.7994823070509,12.2,3.902195380806));
#201099=CARTESIAN_POINT('Ctrl Pts',(10.8021386241625,12.2,3.90492012716428));
#201100=CARTESIAN_POINT('Ctrl Pts',(10.8056803806331,12.2,3.90855312263864));
#201101=CARTESIAN_POINT('Ctrl Pts',(10.8092248173667,12.2,3.91219990566914));
#201102=CARTESIAN_POINT('Ctrl Pts',(10.8127719249999,12.2,3.91586047999999));
#201103=CARTESIAN_POINT('Origin',(-5.66257110645729E-14,15.2,-1.77635683940025E-14));
#201104=CARTESIAN_POINT('',(9.31239139999994,15.2,4.57383771099998));
#201105=CARTESIAN_POINT('',(9.31239139999994,12.2,4.57383771099998));
#201106=CARTESIAN_POINT('',(9.31239139999994,15.2,4.57383771099998));
#201107=CARTESIAN_POINT('Origin',(-5.66257110645729E-14,12.2,-1.77635683940025E-14));
#201108=CARTESIAN_POINT('Origin',(-5.66257110645729E-14,15.2,-1.77635683940025E-14));
#201109=CARTESIAN_POINT('Origin',(-5.66257110645729E-14,15.2,-1.77635683940025E-14));
#201110=CARTESIAN_POINT('',(10.1454284469999,15.2,5.41482055399998));
#201111=CARTESIAN_POINT('',(9.95917514599994,15.2,5.75020264099999));
#201112=CARTESIAN_POINT('Origin',(-5.66257110645729E-14,15.2,-1.77635683940025E-14));
#201113=CARTESIAN_POINT('',(9.95917514599994,12.2,5.75020264099999));
#201114=CARTESIAN_POINT('',(9.95917514599994,15.2,5.75020264099999));
#201115=CARTESIAN_POINT('',(10.1454284469999,12.2,5.41482055399998));
#201116=CARTESIAN_POINT('Origin',(-5.66257110645729E-14,12.2,-1.77635683940025E-14));
#201117=CARTESIAN_POINT('',(10.1454284469999,15.2,5.41482055399998));
#201118=CARTESIAN_POINT('Ctrl Pts',(9.31239140099994,15.2,4.57383771099998));
#201119=CARTESIAN_POINT('Ctrl Pts',(9.31239140099994,11.6,4.57383771099998));
#201120=CARTESIAN_POINT('Ctrl Pts',(9.31254071599994,15.2,4.57392774199998));
#201121=CARTESIAN_POINT('Ctrl Pts',(9.31254071599994,11.6,4.57392774199998));
#201122=CARTESIAN_POINT('Ctrl Pts',(9.31284451699995,15.2,4.57411102199998));
#201123=CARTESIAN_POINT('Ctrl Pts',(9.31284451699995,11.6,4.57411102199998));
#201124=CARTESIAN_POINT('Ctrl Pts',(9.31330471199994,15.2,4.57438896299998));
#201125=CARTESIAN_POINT('Ctrl Pts',(9.31330471199994,11.6,4.57438896299998));
#201126=CARTESIAN_POINT('Ctrl Pts',(9.31392435699994,15.2,4.57476383599998));
#201127=CARTESIAN_POINT('Ctrl Pts',(9.31392435699994,11.6,4.57476383599998));
#201128=CARTESIAN_POINT('Ctrl Pts',(9.31470764299995,15.2,4.57523877599999));
#201129=CARTESIAN_POINT('Ctrl Pts',(9.31470764299995,11.6,4.57523877599998));
#201130=CARTESIAN_POINT('Ctrl Pts',(9.31550313899994,15.2,4.57572221299999));
#201131=CARTESIAN_POINT('Ctrl Pts',(9.31550313899994,11.6,4.57572221299999));
#201132=CARTESIAN_POINT('Ctrl Pts',(9.31630627599995,15.2,4.57621139699998));
#201133=CARTESIAN_POINT('Ctrl Pts',(9.31630627599995,11.6,4.57621139699998));
#201134=CARTESIAN_POINT('Ctrl Pts',(9.31711701999994,15.2,4.57670632999999));
#201135=CARTESIAN_POINT('Ctrl Pts',(9.31711701999994,11.6,4.57670632999999));
#201136=CARTESIAN_POINT('Ctrl Pts',(9.31793533999994,15.2,4.57720701299999));
#201137=CARTESIAN_POINT('Ctrl Pts',(9.31793533999994,11.6,4.57720701299999));
#201138=CARTESIAN_POINT('Ctrl Pts',(9.31876120399994,15.2,4.57771344699999));
#201139=CARTESIAN_POINT('Ctrl Pts',(9.31876120399994,11.6,4.57771344699999));
#201140=CARTESIAN_POINT('Ctrl Pts',(9.31959457899995,15.2,4.57822563399999));
#201141=CARTESIAN_POINT('Ctrl Pts',(9.31959457899995,11.6,4.57822563399999));
#201142=CARTESIAN_POINT('Ctrl Pts',(9.32043543399995,15.2,4.57874357399999));
#201143=CARTESIAN_POINT('Ctrl Pts',(9.32043543399995,11.6,4.57874357399999));
#201144=CARTESIAN_POINT('Ctrl Pts',(9.32128373599994,15.2,4.57926727099998));
#201145=CARTESIAN_POINT('Ctrl Pts',(9.32128373599994,11.6,4.57926727099998));
#201146=CARTESIAN_POINT('Ctrl Pts',(9.32213945299995,15.2,4.57979672299999));
#201147=CARTESIAN_POINT('Ctrl Pts',(9.32213945299995,11.6,4.57979672299999));
#201148=CARTESIAN_POINT('Ctrl Pts',(9.32300255699994,15.2,4.58033193499999));
#201149=CARTESIAN_POINT('Ctrl Pts',(9.32300255699994,11.6,4.58033193499999));
#201150=CARTESIAN_POINT('Ctrl Pts',(9.32387301399995,15.2,4.58087290499999));
#201151=CARTESIAN_POINT('Ctrl Pts',(9.32387301399995,11.6,4.58087290499999));
#201152=CARTESIAN_POINT('Ctrl Pts',(9.32475079199994,15.2,4.58141963599999));
#201153=CARTESIAN_POINT('Ctrl Pts',(9.32475079199994,11.6,4.58141963599999));
#201154=CARTESIAN_POINT('Ctrl Pts',(9.32563586399995,15.2,4.58197212999998));
#201155=CARTESIAN_POINT('Ctrl Pts',(9.32563586399995,11.6,4.58197212999998));
#201156=CARTESIAN_POINT('Ctrl Pts',(9.32652819499994,15.2,4.58253038599998));
#201157=CARTESIAN_POINT('Ctrl Pts',(9.32652819499994,11.6,4.58253038599998));
#201158=CARTESIAN_POINT('Ctrl Pts',(9.32742775699994,15.2,4.58309440699999));
#201159=CARTESIAN_POINT('Ctrl Pts',(9.32742775699994,11.6,4.58309440699998));
#201160=CARTESIAN_POINT('Ctrl Pts',(9.32833451799995,15.2,4.58366419299999));
#201161=CARTESIAN_POINT('Ctrl Pts',(9.32833451799995,11.6,4.58366419299998));
#201162=CARTESIAN_POINT('Ctrl Pts',(9.32924844799994,15.2,4.58423974599998));
#201163=CARTESIAN_POINT('Ctrl Pts',(9.32924844799994,11.6,4.58423974599998));
#201164=CARTESIAN_POINT('Ctrl Pts',(9.33016951599994,15.2,4.58482106699999));
#201165=CARTESIAN_POINT('Ctrl Pts',(9.33016951599994,11.6,4.58482106699999));
#201166=CARTESIAN_POINT('Ctrl Pts',(9.33109769499995,15.2,4.58540815699998));
#201167=CARTESIAN_POINT('Ctrl Pts',(9.33109769499995,11.6,4.58540815699998));
#201168=CARTESIAN_POINT('Ctrl Pts',(9.33203295199995,15.2,4.58600101799998));
#201169=CARTESIAN_POINT('Ctrl Pts',(9.33203295199995,11.6,4.58600101799998));
#201170=CARTESIAN_POINT('Ctrl Pts',(9.33297525899994,15.2,4.58659964899999));
#201171=CARTESIAN_POINT('Ctrl Pts',(9.33297525899994,11.6,4.58659964899999));
#201172=CARTESIAN_POINT('Ctrl Pts',(9.33392458399994,15.2,4.58720405299999));
#201173=CARTESIAN_POINT('Ctrl Pts',(9.33392458399994,11.6,4.58720405299999));
#201174=CARTESIAN_POINT('Ctrl Pts',(9.33488089999994,15.2,4.58781422999999));
#201175=CARTESIAN_POINT('Ctrl Pts',(9.33488089999994,11.6,4.58781422999999));
#201176=CARTESIAN_POINT('Ctrl Pts',(9.33584417599995,15.2,4.58843018099999));
#201177=CARTESIAN_POINT('Ctrl Pts',(9.33584417599995,11.6,4.58843018099999));
#201178=CARTESIAN_POINT('Ctrl Pts',(9.33681438399995,15.2,4.58905190899999));
#201179=CARTESIAN_POINT('Ctrl Pts',(9.33681438399995,11.6,4.58905190899999));
#201180=CARTESIAN_POINT('Ctrl Pts',(9.33779149399994,15.2,4.58967941299999));
#201181=CARTESIAN_POINT('Ctrl Pts',(9.33779149399994,11.6,4.58967941299999));
#201182=CARTESIAN_POINT('Ctrl Pts',(9.33877547699994,15.2,4.59031269399999));
#201183=CARTESIAN_POINT('Ctrl Pts',(9.33877547699994,11.6,4.59031269399999));
#201184=CARTESIAN_POINT('Ctrl Pts',(9.33976630399994,15.2,4.59095175399998));
#201185=CARTESIAN_POINT('Ctrl Pts',(9.33976630399994,11.6,4.59095175399998));
#201186=CARTESIAN_POINT('Ctrl Pts',(9.34076394799994,15.2,4.59159659299999));
#201187=CARTESIAN_POINT('Ctrl Pts',(9.34076394799994,11.6,4.59159659299999));
#201188=CARTESIAN_POINT('Ctrl Pts',(9.34176837799994,15.2,4.59224721199998));
#201189=CARTESIAN_POINT('Ctrl Pts',(9.34176837799994,11.6,4.59224721199998));
#201190=CARTESIAN_POINT('Ctrl Pts',(9.34277956799994,15.2,4.59290361199999));
#201191=CARTESIAN_POINT('Ctrl Pts',(9.34277956799994,11.6,4.59290361199999));
#201192=CARTESIAN_POINT('Ctrl Pts',(9.34379748799994,15.2,4.59356579499998));
#201193=CARTESIAN_POINT('Ctrl Pts',(9.34379748799994,11.6,4.59356579499998));
#201194=CARTESIAN_POINT('Ctrl Pts',(9.34482210899995,15.2,4.59423375999998));
#201195=CARTESIAN_POINT('Ctrl Pts',(9.34482210899995,11.6,4.59423375999998));
#201196=CARTESIAN_POINT('Ctrl Pts',(9.34585340499994,15.2,4.59490750999999));
#201197=CARTESIAN_POINT('Ctrl Pts',(9.34585340499994,11.6,4.59490750999999));
#201198=CARTESIAN_POINT('Ctrl Pts',(9.34689134699994,15.2,4.59558704399999));
#201199=CARTESIAN_POINT('Ctrl Pts',(9.34689134699994,11.6,4.59558704399999));
#201200=CARTESIAN_POINT('Ctrl Pts',(9.34793590799995,15.2,4.59627236399999));
#201201=CARTESIAN_POINT('Ctrl Pts',(9.34793590799995,11.6,4.59627236399999));
#201202=CARTESIAN_POINT('Ctrl Pts',(9.34898705999995,15.2,4.59696346999999));
#201203=CARTESIAN_POINT('Ctrl Pts',(9.34898705999995,11.6,4.59696346999999));
#201204=CARTESIAN_POINT('Ctrl Pts',(9.35004477499995,15.2,4.59766036199999));
#201205=CARTESIAN_POINT('Ctrl Pts',(9.35004477499995,11.6,4.59766036199999));
#201206=CARTESIAN_POINT('Ctrl Pts',(9.35110902499994,15.2,4.59836304399998));
#201207=CARTESIAN_POINT('Ctrl Pts',(9.35110902499994,11.6,4.59836304399998));
#201208=CARTESIAN_POINT('Ctrl Pts',(9.35217978299994,15.2,4.59907151299999));
#201209=CARTESIAN_POINT('Ctrl Pts',(9.35217978299994,11.6,4.59907151299999));
#201210=CARTESIAN_POINT('Ctrl Pts',(9.35325702299994,15.2,4.59978577299999));
#201211=CARTESIAN_POINT('Ctrl Pts',(9.35325702299994,11.6,4.59978577299999));
#201212=CARTESIAN_POINT('Ctrl Pts',(9.35434071699994,15.2,4.60050582099999));
#201213=CARTESIAN_POINT('Ctrl Pts',(9.35434071699994,11.6,4.60050582099999));
#201214=CARTESIAN_POINT('Ctrl Pts',(9.35543083699995,15.2,4.60123166099999));
#201215=CARTESIAN_POINT('Ctrl Pts',(9.35543083699995,11.6,4.60123166099999));
#201216=CARTESIAN_POINT('Ctrl Pts',(9.35652735799994,15.2,4.60196329299999));
#201217=CARTESIAN_POINT('Ctrl Pts',(9.35652735799994,11.6,4.60196329299999));
#201218=CARTESIAN_POINT('Ctrl Pts',(9.35763025299994,15.2,4.60270071599999));
#201219=CARTESIAN_POINT('Ctrl Pts',(9.35763025299994,11.6,4.60270071599999));
#201220=CARTESIAN_POINT('Ctrl Pts',(9.35873949399994,15.2,4.60344393199998));
#201221=CARTESIAN_POINT('Ctrl Pts',(9.35873949399994,11.6,4.60344393199998));
#201222=CARTESIAN_POINT('Ctrl Pts',(9.35985505599995,15.2,4.60419294199998));
#201223=CARTESIAN_POINT('Ctrl Pts',(9.35985505599995,11.6,4.60419294199998));
#201224=CARTESIAN_POINT('Ctrl Pts',(9.36097691199994,15.2,4.60494774699999));
#201225=CARTESIAN_POINT('Ctrl Pts',(9.36097691199994,11.6,4.60494774699998));
#201226=CARTESIAN_POINT('Ctrl Pts',(9.36210503599994,15.2,4.60570834399999));
#201227=CARTESIAN_POINT('Ctrl Pts',(9.36210503599994,11.6,4.60570834399998));
#201228=CARTESIAN_POINT('Ctrl Pts',(9.36323940099994,15.2,4.60647473799998));
#201229=CARTESIAN_POINT('Ctrl Pts',(9.36323940099994,11.6,4.60647473799998));
#201230=CARTESIAN_POINT('Ctrl Pts',(9.36437998199994,15.2,4.60724692899999));
#201231=CARTESIAN_POINT('Ctrl Pts',(9.36437998199994,11.6,4.60724692899999));
#201232=CARTESIAN_POINT('Ctrl Pts',(9.36552675199994,15.2,4.60802491399999));
#201233=CARTESIAN_POINT('Ctrl Pts',(9.36552675199994,11.6,4.60802491399999));
#201234=CARTESIAN_POINT('Ctrl Pts',(9.36667968599994,15.2,4.60880869699999));
#201235=CARTESIAN_POINT('Ctrl Pts',(9.36667968599994,11.6,4.60880869699999));
#201236=CARTESIAN_POINT('Ctrl Pts',(9.36783875799994,15.2,4.60959827699998));
#201237=CARTESIAN_POINT('Ctrl Pts',(9.36783875799994,11.6,4.60959827699998));
#201238=CARTESIAN_POINT('Ctrl Pts',(9.36900394199995,15.2,4.61039365599999));
#201239=CARTESIAN_POINT('Ctrl Pts',(9.36900394199995,11.6,4.61039365599999));
#201240=CARTESIAN_POINT('Ctrl Pts',(9.37017521299994,15.2,4.61119483299999));
#201241=CARTESIAN_POINT('Ctrl Pts',(9.37017521299994,11.6,4.61119483299999));
#201242=CARTESIAN_POINT('Ctrl Pts',(9.37135254599994,15.2,4.61200180799998));
#201243=CARTESIAN_POINT('Ctrl Pts',(9.37135254599994,11.6,4.61200180799998));
#201244=CARTESIAN_POINT('Ctrl Pts',(9.37253591499994,15.2,4.61281458399998));
#201245=CARTESIAN_POINT('Ctrl Pts',(9.37253591499994,11.6,4.61281458399998));
#201246=CARTESIAN_POINT('Ctrl Pts',(9.37372529599994,15.2,4.61363315899998));
#201247=CARTESIAN_POINT('Ctrl Pts',(9.37372529599994,11.6,4.61363315899998));
#201248=CARTESIAN_POINT('Ctrl Pts',(9.37492066099994,15.2,4.61445753499999));
#201249=CARTESIAN_POINT('Ctrl Pts',(9.37492066099994,11.6,4.61445753499999));
#201250=CARTESIAN_POINT('Ctrl Pts',(9.37612198799994,15.2,4.61528771099999));
#201251=CARTESIAN_POINT('Ctrl Pts',(9.37612198799994,11.6,4.61528771099999));
#201252=CARTESIAN_POINT('Ctrl Pts',(9.37732925099995,15.2,4.61612368799998));
#201253=CARTESIAN_POINT('Ctrl Pts',(9.37732925099995,11.6,4.61612368799998));
#201254=CARTESIAN_POINT('Ctrl Pts',(9.37854242599995,15.2,4.61696546699999));
#201255=CARTESIAN_POINT('Ctrl Pts',(9.37854242599995,11.6,4.61696546699999));
#201256=CARTESIAN_POINT('Ctrl Pts',(9.37976148599994,15.2,4.61781304799998));
#201257=CARTESIAN_POINT('Ctrl Pts',(9.37976148599994,11.6,4.61781304799998));
#201258=CARTESIAN_POINT('Ctrl Pts',(9.38098640899995,15.2,4.61866643099999));
#201259=CARTESIAN_POINT('Ctrl Pts',(9.38098640899995,11.6,4.61866643099999));
#201260=CARTESIAN_POINT('Ctrl Pts',(9.38221716999994,15.2,4.61952561599999));
#201261=CARTESIAN_POINT('Ctrl Pts',(9.38221716999994,11.6,4.61952561599999));
#201262=CARTESIAN_POINT('Ctrl Pts',(9.38345374299994,15.2,4.62039060399999));
#201263=CARTESIAN_POINT('Ctrl Pts',(9.38345374299994,11.6,4.62039060399999));
#201264=CARTESIAN_POINT('Ctrl Pts',(9.38469610599994,15.2,4.62126139599999));
#201265=CARTESIAN_POINT('Ctrl Pts',(9.38469610599994,11.6,4.62126139599999));
#201266=CARTESIAN_POINT('Ctrl Pts',(9.38594423299994,15.2,4.62213799099998));
#201267=CARTESIAN_POINT('Ctrl Pts',(9.38594423299994,11.6,4.62213799099998));
#201268=CARTESIAN_POINT('Ctrl Pts',(9.38719809999995,15.2,4.62302038999999));
#201269=CARTESIAN_POINT('Ctrl Pts',(9.38719809999995,11.6,4.62302038999999));
#201270=CARTESIAN_POINT('Ctrl Pts',(9.38845768499995,15.2,4.62390859299998));
#201271=CARTESIAN_POINT('Ctrl Pts',(9.38845768499995,11.6,4.62390859299998));
#201272=CARTESIAN_POINT('Ctrl Pts',(9.38972296199994,15.2,4.62480259999998));
#201273=CARTESIAN_POINT('Ctrl Pts',(9.38972296199994,11.6,4.62480259999998));
#201274=CARTESIAN_POINT('Ctrl Pts',(9.39099390899995,15.2,4.62570241299999));
#201275=CARTESIAN_POINT('Ctrl Pts',(9.39099390899995,11.6,4.62570241299998));
#201276=CARTESIAN_POINT('Ctrl Pts',(9.39227049999994,15.2,4.62660802899999));
#201277=CARTESIAN_POINT('Ctrl Pts',(9.39227049999994,11.6,4.62660802899998));
#201278=CARTESIAN_POINT('Ctrl Pts',(9.39355271299994,15.2,4.62751945099999));
#201279=CARTESIAN_POINT('Ctrl Pts',(9.39355271299994,11.6,4.62751945099999));
#201280=CARTESIAN_POINT('Ctrl Pts',(9.39484052399994,15.2,4.62843667799999));
#201281=CARTESIAN_POINT('Ctrl Pts',(9.39484052399994,11.6,4.62843667799999));
#201282=CARTESIAN_POINT('Ctrl Pts',(9.39613390999994,15.2,4.62935970999999));
#201283=CARTESIAN_POINT('Ctrl Pts',(9.39613390999994,11.6,4.62935970999998));
#201284=CARTESIAN_POINT('Ctrl Pts',(9.39743284699994,15.2,4.63028854799998));
#201285=CARTESIAN_POINT('Ctrl Pts',(9.39743284699994,11.6,4.63028854799998));
#201286=CARTESIAN_POINT('Ctrl Pts',(9.39873731199994,15.2,4.63122319099998));
#201287=CARTESIAN_POINT('Ctrl Pts',(9.39873731199994,11.6,4.63122319099998));
#201288=CARTESIAN_POINT('Ctrl Pts',(9.40004728399994,15.2,4.63216364099999));
#201289=CARTESIAN_POINT('Ctrl Pts',(9.40004728399994,11.6,4.63216364099999));
#201290=CARTESIAN_POINT('Ctrl Pts',(9.40136273499995,15.2,4.63310989699998));
#201291=CARTESIAN_POINT('Ctrl Pts',(9.40136273499995,11.6,4.63310989699998));
#201292=CARTESIAN_POINT('Ctrl Pts',(9.40268364699994,15.2,4.63406195899999));
#201293=CARTESIAN_POINT('Ctrl Pts',(9.40268364699994,11.6,4.63406195899999));
#201294=CARTESIAN_POINT('Ctrl Pts',(9.40400999399994,15.2,4.63501982699999));
#201295=CARTESIAN_POINT('Ctrl Pts',(9.40400999399994,11.6,4.63501982699999));
#201296=CARTESIAN_POINT('Ctrl Pts',(9.40534175499995,15.2,4.63598350099999));
#201297=CARTESIAN_POINT('Ctrl Pts',(9.40534175499995,11.6,4.63598350099998));
#201298=CARTESIAN_POINT('Ctrl Pts',(9.40667890599994,15.2,4.63695298199998));
#201299=CARTESIAN_POINT('Ctrl Pts',(9.40667890599994,11.6,4.63695298199998));
#201300=CARTESIAN_POINT('Ctrl Pts',(9.40802142599994,15.2,4.63792826899999));
#201301=CARTESIAN_POINT('Ctrl Pts',(9.40802142599994,11.6,4.63792826899999));
#201302=CARTESIAN_POINT('Ctrl Pts',(9.40936929099994,15.2,4.63890936299999));
#201303=CARTESIAN_POINT('Ctrl Pts',(9.40936929099994,11.6,4.63890936299998));
#201304=CARTESIAN_POINT('Ctrl Pts',(9.41072247899994,15.2,4.63989626299998));
#201305=CARTESIAN_POINT('Ctrl Pts',(9.41072247899994,11.6,4.63989626299998));
#201306=CARTESIAN_POINT('Ctrl Pts',(9.41208096699994,15.2,4.64088896999999));
#201307=CARTESIAN_POINT('Ctrl Pts',(9.41208096699994,11.6,4.64088896999998));
#201308=CARTESIAN_POINT('Ctrl Pts',(9.41344473399995,15.2,4.64188748299998));
#201309=CARTESIAN_POINT('Ctrl Pts',(9.41344473399995,11.6,4.64188748299998));
#201310=CARTESIAN_POINT('Ctrl Pts',(9.41481375699994,15.2,4.64289180399999));
#201311=CARTESIAN_POINT('Ctrl Pts',(9.41481375699994,11.6,4.64289180399999));
#201312=CARTESIAN_POINT('Ctrl Pts',(9.41618801399994,15.2,4.64390192999999));
#201313=CARTESIAN_POINT('Ctrl Pts',(9.41618801399994,11.6,4.64390192999998));
#201314=CARTESIAN_POINT('Ctrl Pts',(9.41756748299994,15.2,4.64491786399999));
#201315=CARTESIAN_POINT('Ctrl Pts',(9.41756748299994,11.6,4.64491786399999));
#201316=CARTESIAN_POINT('Ctrl Pts',(9.41895214199995,15.2,4.64593960399998));
#201317=CARTESIAN_POINT('Ctrl Pts',(9.41895214199995,11.6,4.64593960399998));
#201318=CARTESIAN_POINT('Ctrl Pts',(9.42034196999994,15.2,4.64696714999998));
#201319=CARTESIAN_POINT('Ctrl Pts',(9.42034196999994,11.6,4.64696714999998));
#201320=CARTESIAN_POINT('Ctrl Pts',(9.42173694299994,15.2,4.64800050299999));
#201321=CARTESIAN_POINT('Ctrl Pts',(9.42173694299994,11.6,4.64800050299999));
#201322=CARTESIAN_POINT('Ctrl Pts',(9.42313704199995,15.2,4.64903966199999));
#201323=CARTESIAN_POINT('Ctrl Pts',(9.42313704199995,11.6,4.64903966199999));
#201324=CARTESIAN_POINT('Ctrl Pts',(9.42454224399994,15.2,4.65008462799998));
#201325=CARTESIAN_POINT('Ctrl Pts',(9.42454224399994,11.6,4.65008462799998));
#201326=CARTESIAN_POINT('Ctrl Pts',(9.42595252799994,15.2,4.65113539899999));
#201327=CARTESIAN_POINT('Ctrl Pts',(9.42595252799994,11.6,4.65113539899999));
#201328=CARTESIAN_POINT('Ctrl Pts',(9.42736787099994,15.2,4.65219197699999));
#201329=CARTESIAN_POINT('Ctrl Pts',(9.42736787099994,11.6,4.65219197699999));
#201330=CARTESIAN_POINT('Ctrl Pts',(9.42878825299994,15.2,4.65325436099998));
#201331=CARTESIAN_POINT('Ctrl Pts',(9.42878825299994,11.6,4.65325436099998));
#201332=CARTESIAN_POINT('Ctrl Pts',(9.43021365299994,15.2,4.65432254999998));
#201333=CARTESIAN_POINT('Ctrl Pts',(9.43021365299994,11.6,4.65432254999998));
#201334=CARTESIAN_POINT('Ctrl Pts',(9.43164404899994,15.2,4.65539654499998));
#201335=CARTESIAN_POINT('Ctrl Pts',(9.43164404899994,11.6,4.65539654499998));
#201336=CARTESIAN_POINT('Ctrl Pts',(9.43307941999995,15.2,4.65647634499998));
#201337=CARTESIAN_POINT('Ctrl Pts',(9.43307941999995,11.6,4.65647634499998));
#201338=CARTESIAN_POINT('Ctrl Pts',(9.43451974499995,15.2,4.65756195099999));
#201339=CARTESIAN_POINT('Ctrl Pts',(9.43451974499995,11.6,4.65756195099999));
#201340=CARTESIAN_POINT('Ctrl Pts',(9.43596500299994,15.2,4.65865336199998));
#201341=CARTESIAN_POINT('Ctrl Pts',(9.43596500299994,11.6,4.65865336199998));
#201342=CARTESIAN_POINT('Ctrl Pts',(9.43741517299994,15.2,4.65975057799999));
#201343=CARTESIAN_POINT('Ctrl Pts',(9.43741517299994,11.6,4.65975057799999));
#201344=CARTESIAN_POINT('Ctrl Pts',(9.43887023499994,15.2,4.66085359799998));
#201345=CARTESIAN_POINT('Ctrl Pts',(9.43887023499994,11.6,4.66085359799998));
#201346=CARTESIAN_POINT('Ctrl Pts',(9.44033016699995,15.2,4.66196242299999));
#201347=CARTESIAN_POINT('Ctrl Pts',(9.44033016699995,11.6,4.66196242299999));
#201348=CARTESIAN_POINT('Ctrl Pts',(9.44179494899995,15.2,4.66307705199998));
#201349=CARTESIAN_POINT('Ctrl Pts',(9.44179494899995,11.6,4.66307705199998));
#201350=CARTESIAN_POINT('Ctrl Pts',(9.44326455999994,15.2,4.66419748599999));
#201351=CARTESIAN_POINT('Ctrl Pts',(9.44326455999994,11.6,4.66419748599998));
#201352=CARTESIAN_POINT('Ctrl Pts',(9.44473897999995,15.2,4.66532372299999));
#201353=CARTESIAN_POINT('Ctrl Pts',(9.44473897999995,11.6,4.66532372299999));
#201354=CARTESIAN_POINT('Ctrl Pts',(9.44621818699994,15.2,4.66645576299998));
#201355=CARTESIAN_POINT('Ctrl Pts',(9.44621818699994,11.6,4.66645576299998));
#201356=CARTESIAN_POINT('Ctrl Pts',(9.44770216299995,15.2,4.66759360699999));
#201357=CARTESIAN_POINT('Ctrl Pts',(9.44770216299995,11.6,4.66759360699999));
#201358=CARTESIAN_POINT('Ctrl Pts',(9.44919088599995,15.2,4.66873725399999));
#201359=CARTESIAN_POINT('Ctrl Pts',(9.44919088599995,11.6,4.66873725399999));
#201360=CARTESIAN_POINT('Ctrl Pts',(9.45068433699995,15.2,4.66988670299998));
#201361=CARTESIAN_POINT('Ctrl Pts',(9.45068433699995,11.6,4.66988670299998));
#201362=CARTESIAN_POINT('Ctrl Pts',(9.45218249399994,15.2,4.67104195499999));
#201363=CARTESIAN_POINT('Ctrl Pts',(9.45218249399994,11.6,4.67104195499999));
#201364=CARTESIAN_POINT('Ctrl Pts',(9.45368533799994,15.2,4.67220300799998));
#201365=CARTESIAN_POINT('Ctrl Pts',(9.45368533799994,11.6,4.67220300799998));
#201366=CARTESIAN_POINT('Ctrl Pts',(9.45519284899994,15.2,4.67336986399999));
#201367=CARTESIAN_POINT('Ctrl Pts',(9.45519284899994,11.6,4.67336986399999));
#201368=CARTESIAN_POINT('Ctrl Pts',(9.45670500599994,15.2,4.67454251999998));
#201369=CARTESIAN_POINT('Ctrl Pts',(9.45670500599994,11.6,4.67454251999998));
#201370=CARTESIAN_POINT('Ctrl Pts',(9.45822179099994,15.2,4.67572097799999));
#201371=CARTESIAN_POINT('Ctrl Pts',(9.45822179099994,11.6,4.67572097799999));
#201372=CARTESIAN_POINT('Ctrl Pts',(9.45974318299994,15.2,4.67690523599998));
#201373=CARTESIAN_POINT('Ctrl Pts',(9.45974318299994,11.6,4.67690523599998));
#201374=CARTESIAN_POINT('Ctrl Pts',(9.46126916199994,15.2,4.67809529399998));
#201375=CARTESIAN_POINT('Ctrl Pts',(9.46126916199994,11.6,4.67809529399998));
#201376=CARTESIAN_POINT('Ctrl Pts',(9.46279970999995,15.2,4.67929115199999));
#201377=CARTESIAN_POINT('Ctrl Pts',(9.46279970999995,11.6,4.67929115199999));
#201378=CARTESIAN_POINT('Ctrl Pts',(9.46433480399994,15.2,4.68049280999999));
#201379=CARTESIAN_POINT('Ctrl Pts',(9.46433480399994,11.6,4.68049280999998));
#201380=CARTESIAN_POINT('Ctrl Pts',(9.46587442699995,15.2,4.68170026699998));
#201381=CARTESIAN_POINT('Ctrl Pts',(9.46587442699995,11.6,4.68170026699998));
#201382=CARTESIAN_POINT('Ctrl Pts',(9.46741855999995,15.2,4.68291352199999));
#201383=CARTESIAN_POINT('Ctrl Pts',(9.46741855999995,11.6,4.68291352199999));
#201384=CARTESIAN_POINT('Ctrl Pts',(9.46896718199995,15.2,4.68413257599998));
#201385=CARTESIAN_POINT('Ctrl Pts',(9.46896718199995,11.6,4.68413257599998));
#201386=CARTESIAN_POINT('Ctrl Pts',(9.47052027399995,15.2,4.68535742699999));
#201387=CARTESIAN_POINT('Ctrl Pts',(9.47052027399995,11.6,4.68535742699998));
#201388=CARTESIAN_POINT('Ctrl Pts',(9.47207781699994,15.2,4.68658807499998));
#201389=CARTESIAN_POINT('Ctrl Pts',(9.47207781699994,11.6,4.68658807499998));
#201390=CARTESIAN_POINT('Ctrl Pts',(9.47363979099995,15.2,4.68782451999999));
#201391=CARTESIAN_POINT('Ctrl Pts',(9.47363979099995,11.6,4.68782451999999));
#201392=CARTESIAN_POINT('Ctrl Pts',(9.47520617799994,15.2,4.68906676099999));
#201393=CARTESIAN_POINT('Ctrl Pts',(9.47520617799994,11.6,4.68906676099999));
#201394=CARTESIAN_POINT('Ctrl Pts',(9.47677695899995,15.2,4.69031479799998));
#201395=CARTESIAN_POINT('Ctrl Pts',(9.47677695899995,11.6,4.69031479799998));
#201396=CARTESIAN_POINT('Ctrl Pts',(9.47835211299994,15.2,4.69156863099998));
#201397=CARTESIAN_POINT('Ctrl Pts',(9.47835211299994,11.6,4.69156863099998));
#201398=CARTESIAN_POINT('Ctrl Pts',(9.47993162399994,15.2,4.69282825799999));
#201399=CARTESIAN_POINT('Ctrl Pts',(9.47993162399994,11.6,4.69282825799999));
#201400=CARTESIAN_POINT('Ctrl Pts',(9.48151547099994,15.2,4.69409367999998));
#201401=CARTESIAN_POINT('Ctrl Pts',(9.48151547099994,11.6,4.69409367999998));
#201402=CARTESIAN_POINT('Ctrl Pts',(9.48310363399995,15.2,4.69536489599999));
#201403=CARTESIAN_POINT('Ctrl Pts',(9.48310363399995,11.6,4.69536489599999));
#201404=CARTESIAN_POINT('Ctrl Pts',(9.48469609699995,15.2,4.69664190399998));
#201405=CARTESIAN_POINT('Ctrl Pts',(9.48469609699995,11.6,4.69664190399998));
#201406=CARTESIAN_POINT('Ctrl Pts',(9.48629283999994,15.2,4.69792470599998));
#201407=CARTESIAN_POINT('Ctrl Pts',(9.48629283999994,11.6,4.69792470599998));
#201408=CARTESIAN_POINT('Ctrl Pts',(9.48789384499995,15.2,4.69921329999998));
#201409=CARTESIAN_POINT('Ctrl Pts',(9.48789384499995,11.6,4.69921329999998));
#201410=CARTESIAN_POINT('Ctrl Pts',(9.48949909199994,15.2,4.70050768499998));
#201411=CARTESIAN_POINT('Ctrl Pts',(9.48949909199994,11.6,4.70050768499998));
#201412=CARTESIAN_POINT('Ctrl Pts',(9.49110856299994,15.2,4.70180786099998));
#201413=CARTESIAN_POINT('Ctrl Pts',(9.49110856299994,11.6,4.70180786099998));
#201414=CARTESIAN_POINT('Ctrl Pts',(9.49272223999994,15.2,4.70311382799999));
#201415=CARTESIAN_POINT('Ctrl Pts',(9.49272223999994,11.6,4.70311382799998));
#201416=CARTESIAN_POINT('Ctrl Pts',(9.49434010399995,15.2,4.70442558399998));
#201417=CARTESIAN_POINT('Ctrl Pts',(9.49434010399995,11.6,4.70442558399998));
#201418=CARTESIAN_POINT('Ctrl Pts',(9.49596213899994,15.2,4.70574312999998));
#201419=CARTESIAN_POINT('Ctrl Pts',(9.49596213899994,11.6,4.70574312999998));
#201420=CARTESIAN_POINT('Ctrl Pts',(9.49758832299995,15.2,4.70706646399999));
#201421=CARTESIAN_POINT('Ctrl Pts',(9.49758832299995,11.6,4.70706646399999));
#201422=CARTESIAN_POINT('Ctrl Pts',(9.49921863899995,15.2,4.70839558599998));
#201423=CARTESIAN_POINT('Ctrl Pts',(9.49921863899995,11.6,4.70839558599998));
#201424=CARTESIAN_POINT('Ctrl Pts',(9.50085307099994,15.2,4.70973049499998));
#201425=CARTESIAN_POINT('Ctrl Pts',(9.50085307099994,11.6,4.70973049499998));
#201426=CARTESIAN_POINT('Ctrl Pts',(9.50249159799995,15.2,4.71107119199999));
#201427=CARTESIAN_POINT('Ctrl Pts',(9.50249159799995,11.6,4.71107119199999));
#201428=CARTESIAN_POINT('Ctrl Pts',(9.50413420299995,15.2,4.71241767399999));
#201429=CARTESIAN_POINT('Ctrl Pts',(9.50413420299995,11.6,4.71241767399999));
#201430=CARTESIAN_POINT('Ctrl Pts',(9.50578086799995,15.2,4.71376994199999));
#201431=CARTESIAN_POINT('Ctrl Pts',(9.50578086799995,11.6,4.71376994199998));
#201432=CARTESIAN_POINT('Ctrl Pts',(9.50743157599995,15.2,4.71512799399999));
#201433=CARTESIAN_POINT('Ctrl Pts',(9.50743157599995,11.6,4.71512799399999));
#201434=CARTESIAN_POINT('Ctrl Pts',(9.50908630799994,15.2,4.71649182999998));
#201435=CARTESIAN_POINT('Ctrl Pts',(9.50908630799994,11.6,4.71649182999998));
#201436=CARTESIAN_POINT('Ctrl Pts',(9.51074504599994,15.2,4.71786144999999));
#201437=CARTESIAN_POINT('Ctrl Pts',(9.51074504599994,11.6,4.71786144999999));
#201438=CARTESIAN_POINT('Ctrl Pts',(9.51240777299994,15.2,4.71923685199998));
#201439=CARTESIAN_POINT('Ctrl Pts',(9.51240777299994,11.6,4.71923685199998));
#201440=CARTESIAN_POINT('Ctrl Pts',(9.51407447099994,15.2,4.72061803599999));
#201441=CARTESIAN_POINT('Ctrl Pts',(9.51407447099994,11.6,4.72061803599999));
#201442=CARTESIAN_POINT('Ctrl Pts',(9.51574512199995,15.2,4.72200500099999));
#201443=CARTESIAN_POINT('Ctrl Pts',(9.51574512199995,11.6,4.72200500099999));
#201444=CARTESIAN_POINT('Ctrl Pts',(9.51741970899995,15.2,4.72339774699999));
#201445=CARTESIAN_POINT('Ctrl Pts',(9.51741970899995,11.6,4.72339774699999));
#201446=CARTESIAN_POINT('Ctrl Pts',(9.51909821399994,15.2,4.72479627299998));
#201447=CARTESIAN_POINT('Ctrl Pts',(9.51909821399994,11.6,4.72479627299998));
#201448=CARTESIAN_POINT('Ctrl Pts',(9.52078061899994,15.2,4.72620057699999));
#201449=CARTESIAN_POINT('Ctrl Pts',(9.52078061899994,11.6,4.72620057699999));
#201450=CARTESIAN_POINT('Ctrl Pts',(9.52246690899995,15.2,4.72761065899999));
#201451=CARTESIAN_POINT('Ctrl Pts',(9.52246690899995,11.6,4.72761065899998));
#201452=CARTESIAN_POINT('Ctrl Pts',(9.52415706299995,15.2,4.72902651899999));
#201453=CARTESIAN_POINT('Ctrl Pts',(9.52415706299995,11.6,4.72902651899999));
#201454=CARTESIAN_POINT('Ctrl Pts',(9.52585106599994,15.2,4.73044815499998));
#201455=CARTESIAN_POINT('Ctrl Pts',(9.52585106599994,11.6,4.73044815499998));
#201456=CARTESIAN_POINT('Ctrl Pts',(9.52754889999994,15.2,4.73187556799999));
#201457=CARTESIAN_POINT('Ctrl Pts',(9.52754889999994,11.6,4.73187556799999));
#201458=CARTESIAN_POINT('Ctrl Pts',(9.52925054799995,15.2,4.73330875599999));
#201459=CARTESIAN_POINT('Ctrl Pts',(9.52925054799995,11.6,4.73330875599998));
#201460=CARTESIAN_POINT('Ctrl Pts',(9.53095599299994,15.2,4.73474771699999));
#201461=CARTESIAN_POINT('Ctrl Pts',(9.53095599299994,11.6,4.73474771699998));
#201462=CARTESIAN_POINT('Ctrl Pts',(9.53266521799994,15.2,4.73619245199998));
#201463=CARTESIAN_POINT('Ctrl Pts',(9.53266521799994,11.6,4.73619245199998));
#201464=CARTESIAN_POINT('Ctrl Pts',(9.53437820499994,15.2,4.73764295999998));
#201465=CARTESIAN_POINT('Ctrl Pts',(9.53437820499994,11.6,4.73764295999998));
#201466=CARTESIAN_POINT('Ctrl Pts',(9.53609493699994,15.2,4.73909923999998));
#201467=CARTESIAN_POINT('Ctrl Pts',(9.53609493699994,11.6,4.73909923999998));
#201468=CARTESIAN_POINT('Ctrl Pts',(9.53781539899994,15.2,4.74056128999998));
#201469=CARTESIAN_POINT('Ctrl Pts',(9.53781539899994,11.6,4.74056128999998));
#201470=CARTESIAN_POINT('Ctrl Pts',(9.53953957299994,15.2,4.74202910999999));
#201471=CARTESIAN_POINT('Ctrl Pts',(9.53953957299994,11.6,4.74202910999998));
#201472=CARTESIAN_POINT('Ctrl Pts',(9.54126743999995,15.2,4.74350269999999));
#201473=CARTESIAN_POINT('Ctrl Pts',(9.54126743999995,11.6,4.74350269999999));
#201474=CARTESIAN_POINT('Ctrl Pts',(9.54299898599994,15.2,4.74498205899998));
#201475=CARTESIAN_POINT('Ctrl Pts',(9.54299898599994,11.6,4.74498205899998));
#201476=CARTESIAN_POINT('Ctrl Pts',(9.54473419399994,15.2,4.74646718399999));
#201477=CARTESIAN_POINT('Ctrl Pts',(9.54473419399994,11.6,4.74646718399998));
#201478=CARTESIAN_POINT('Ctrl Pts',(9.54647304499994,15.2,4.74795807599998));
#201479=CARTESIAN_POINT('Ctrl Pts',(9.54647304499994,11.6,4.74795807599998));
#201480=CARTESIAN_POINT('Ctrl Pts',(9.54821552499994,15.2,4.74945473499999));
#201481=CARTESIAN_POINT('Ctrl Pts',(9.54821552499994,11.6,4.74945473499999));
#201482=CARTESIAN_POINT('Ctrl Pts',(9.54996161699994,15.2,4.75095715699998));
#201483=CARTESIAN_POINT('Ctrl Pts',(9.54996161699994,11.6,4.75095715699998));
#201484=CARTESIAN_POINT('Ctrl Pts',(9.55171130299994,15.2,4.75246534399999));
#201485=CARTESIAN_POINT('Ctrl Pts',(9.55171130299994,11.6,4.75246534399999));
#201486=CARTESIAN_POINT('Ctrl Pts',(9.55346456699995,15.2,4.75397929399998));
#201487=CARTESIAN_POINT('Ctrl Pts',(9.55346456699995,11.6,4.75397929399998));
#201488=CARTESIAN_POINT('Ctrl Pts',(9.55522139299994,15.2,4.75549900599999));
#201489=CARTESIAN_POINT('Ctrl Pts',(9.55522139299994,11.6,4.75549900599999));
#201490=CARTESIAN_POINT('Ctrl Pts',(9.55698176499994,15.2,4.75702447899998));
#201491=CARTESIAN_POINT('Ctrl Pts',(9.55698176499994,11.6,4.75702447899998));
#201492=CARTESIAN_POINT('Ctrl Pts',(9.55874566599995,15.2,4.75855571199999));
#201493=CARTESIAN_POINT('Ctrl Pts',(9.55874566599995,11.6,4.75855571199998));
#201494=CARTESIAN_POINT('Ctrl Pts',(9.56051307899994,15.2,4.76009270399998));
#201495=CARTESIAN_POINT('Ctrl Pts',(9.56051307899994,11.6,4.76009270399998));
#201496=CARTESIAN_POINT('Ctrl Pts',(9.56228398899994,15.2,4.76163545499999));
#201497=CARTESIAN_POINT('Ctrl Pts',(9.56228398899994,11.6,4.76163545499999));
#201498=CARTESIAN_POINT('Ctrl Pts',(9.56405837899995,15.2,4.76318396199999));
#201499=CARTESIAN_POINT('Ctrl Pts',(9.56405837899995,11.6,4.76318396199999));
#201500=CARTESIAN_POINT('Ctrl Pts',(9.56583623399995,15.2,4.76473822599999));
#201501=CARTESIAN_POINT('Ctrl Pts',(9.56583623399995,11.6,4.76473822599999));
#201502=CARTESIAN_POINT('Ctrl Pts',(9.56761753699995,15.2,4.76629824599998));
#201503=CARTESIAN_POINT('Ctrl Pts',(9.56761753699995,11.6,4.76629824599998));
#201504=CARTESIAN_POINT('Ctrl Pts',(9.56940227099994,15.2,4.76786401999998));
#201505=CARTESIAN_POINT('Ctrl Pts',(9.56940227099994,11.6,4.76786401999998));
#201506=CARTESIAN_POINT('Ctrl Pts',(9.57119042099994,15.2,4.76943554699999));
#201507=CARTESIAN_POINT('Ctrl Pts',(9.57119042099994,11.6,4.76943554699999));
#201508=CARTESIAN_POINT('Ctrl Pts',(9.57298197099995,15.2,4.77101282699999));
#201509=CARTESIAN_POINT('Ctrl Pts',(9.57298197099995,11.6,4.77101282699999));
#201510=CARTESIAN_POINT('Ctrl Pts',(9.57477690499994,15.2,4.77259585799998));
#201511=CARTESIAN_POINT('Ctrl Pts',(9.57477690499994,11.6,4.77259585799998));
#201512=CARTESIAN_POINT('Ctrl Pts',(9.57657520799994,15.2,4.77418463899999));
#201513=CARTESIAN_POINT('Ctrl Pts',(9.57657520799994,11.6,4.77418463899998));
#201514=CARTESIAN_POINT('Ctrl Pts',(9.57837686399994,15.2,4.77577916999999));
#201515=CARTESIAN_POINT('Ctrl Pts',(9.57837686399994,11.6,4.77577916999999));
#201516=CARTESIAN_POINT('Ctrl Pts',(9.58018185399995,15.2,4.77737944799999));
#201517=CARTESIAN_POINT('Ctrl Pts',(9.58018185399995,11.6,4.77737944799998));
#201518=CARTESIAN_POINT('Ctrl Pts',(9.58199016599995,15.2,4.77898547499999));
#201519=CARTESIAN_POINT('Ctrl Pts',(9.58199016599995,11.6,4.77898547499999));
#201520=CARTESIAN_POINT('Ctrl Pts',(9.58380178399995,15.2,4.78059724599999));
#201521=CARTESIAN_POINT('Ctrl Pts',(9.58380178399995,11.6,4.78059724599999));
#201522=CARTESIAN_POINT('Ctrl Pts',(9.58561669099995,15.2,4.78221476299999));
#201523=CARTESIAN_POINT('Ctrl Pts',(9.58561669099995,11.6,4.78221476299998));
#201524=CARTESIAN_POINT('Ctrl Pts',(9.58743487199994,15.2,4.78383802399998));
#201525=CARTESIAN_POINT('Ctrl Pts',(9.58743487199994,11.6,4.78383802399998));
#201526=CARTESIAN_POINT('Ctrl Pts',(9.58925631099994,15.2,4.78546702899998));
#201527=CARTESIAN_POINT('Ctrl Pts',(9.58925631099994,11.6,4.78546702899998));
#201528=CARTESIAN_POINT('Ctrl Pts',(9.59108099299995,15.2,4.78710177399999));
#201529=CARTESIAN_POINT('Ctrl Pts',(9.59108099299995,11.6,4.78710177399999));
#201530=CARTESIAN_POINT('Ctrl Pts',(9.59290890099994,15.2,4.78874226099999));
#201531=CARTESIAN_POINT('Ctrl Pts',(9.59290890099994,11.6,4.78874226099998));
#201532=CARTESIAN_POINT('Ctrl Pts',(9.59474002199994,15.2,4.79038848699999));
#201533=CARTESIAN_POINT('Ctrl Pts',(9.59474002199994,11.6,4.79038848699999));
#201534=CARTESIAN_POINT('Ctrl Pts',(9.59657433999995,15.2,4.79204045099999));
#201535=CARTESIAN_POINT('Ctrl Pts',(9.59657433999995,11.6,4.79204045099998));
#201536=CARTESIAN_POINT('Ctrl Pts',(9.59841183799995,15.2,4.79369815299999));
#201537=CARTESIAN_POINT('Ctrl Pts',(9.59841183799995,11.6,4.79369815299999));
#201538=CARTESIAN_POINT('Ctrl Pts',(9.60025250199994,15.2,4.79536159099998));
#201539=CARTESIAN_POINT('Ctrl Pts',(9.60025250199994,11.6,4.79536159099998));
#201540=CARTESIAN_POINT('Ctrl Pts',(9.60209631699995,15.2,4.79703076499998));
#201541=CARTESIAN_POINT('Ctrl Pts',(9.60209631699995,11.6,4.79703076499998));
#201542=CARTESIAN_POINT('Ctrl Pts',(9.60394326799995,15.2,4.79870567199999));
#201543=CARTESIAN_POINT('Ctrl Pts',(9.60394326799995,11.6,4.79870567199998));
#201544=CARTESIAN_POINT('Ctrl Pts',(9.60579333899994,15.2,4.80038631299998));
#201545=CARTESIAN_POINT('Ctrl Pts',(9.60579333899994,11.6,4.80038631299998));
#201546=CARTESIAN_POINT('Ctrl Pts',(9.60764651399994,15.2,4.80207268499999));
#201547=CARTESIAN_POINT('Ctrl Pts',(9.60764651399994,11.6,4.80207268499999));
#201548=CARTESIAN_POINT('Ctrl Pts',(9.60950277999994,15.2,4.80376478599998));
#201549=CARTESIAN_POINT('Ctrl Pts',(9.60950277999994,11.6,4.80376478599998));
#201550=CARTESIAN_POINT('Ctrl Pts',(9.61136212099994,15.2,4.80546261799999));
#201551=CARTESIAN_POINT('Ctrl Pts',(9.61136212099994,11.6,4.80546261799999));
#201552=CARTESIAN_POINT('Ctrl Pts',(9.61322452199994,15.2,4.80716617799998));
#201553=CARTESIAN_POINT('Ctrl Pts',(9.61322452199994,11.6,4.80716617799998));
#201554=CARTESIAN_POINT('Ctrl Pts',(9.61508996699994,15.2,4.80887546399998));
#201555=CARTESIAN_POINT('Ctrl Pts',(9.61508996699994,11.6,4.80887546399998));
#201556=CARTESIAN_POINT('Ctrl Pts',(9.61695844299994,15.2,4.81059047699999));
#201557=CARTESIAN_POINT('Ctrl Pts',(9.61695844299994,11.6,4.81059047699999));
#201558=CARTESIAN_POINT('Ctrl Pts',(9.61882993399995,15.2,4.81231121399999));
#201559=CARTESIAN_POINT('Ctrl Pts',(9.61882993399995,11.6,4.81231121399999));
#201560=CARTESIAN_POINT('Ctrl Pts',(9.62070442599994,15.2,4.81403767499998));
#201561=CARTESIAN_POINT('Ctrl Pts',(9.62070442599994,11.6,4.81403767499998));
#201562=CARTESIAN_POINT('Ctrl Pts',(9.62258190299995,15.2,4.81576985699999));
#201563=CARTESIAN_POINT('Ctrl Pts',(9.62258190299995,11.6,4.81576985699998));
#201564=CARTESIAN_POINT('Ctrl Pts',(9.62446235099994,15.2,4.81750776099998));
#201565=CARTESIAN_POINT('Ctrl Pts',(9.62446235099994,11.6,4.81750776099998));
#201566=CARTESIAN_POINT('Ctrl Pts',(9.62634575599994,15.2,4.81925138399999));
#201567=CARTESIAN_POINT('Ctrl Pts',(9.62634575599994,11.6,4.81925138399998));
#201568=CARTESIAN_POINT('Ctrl Pts',(9.62823210099994,15.2,4.82100072599999));
#201569=CARTESIAN_POINT('Ctrl Pts',(9.62823210099994,11.6,4.82100072599999));
#201570=CARTESIAN_POINT('Ctrl Pts',(9.63012137399994,15.2,4.82275578399998));
#201571=CARTESIAN_POINT('Ctrl Pts',(9.63012137399994,11.6,4.82275578399998));
#201572=CARTESIAN_POINT('Ctrl Pts',(9.63201355899994,15.2,4.82451655899998));
#201573=CARTESIAN_POINT('Ctrl Pts',(9.63201355899994,11.6,4.82451655899998));
#201574=CARTESIAN_POINT('Ctrl Pts',(9.63390864199994,15.2,4.82628304899999));
#201575=CARTESIAN_POINT('Ctrl Pts',(9.63390864199994,11.6,4.82628304899999));
#201576=CARTESIAN_POINT('Ctrl Pts',(9.63580660699994,15.2,4.82805525099998));
#201577=CARTESIAN_POINT('Ctrl Pts',(9.63580660699994,11.6,4.82805525099998));
#201578=CARTESIAN_POINT('Ctrl Pts',(9.63770744199994,15.2,4.82983316599999));
#201579=CARTESIAN_POINT('Ctrl Pts',(9.63770744199994,11.6,4.82983316599999));
#201580=CARTESIAN_POINT('Ctrl Pts',(9.63961113099994,15.2,4.83161679299998));
#201581=CARTESIAN_POINT('Ctrl Pts',(9.63961113099994,11.6,4.83161679299998));
#201582=CARTESIAN_POINT('Ctrl Pts',(9.64151765999994,15.2,4.83340612899998));
#201583=CARTESIAN_POINT('Ctrl Pts',(9.64151765999994,11.6,4.83340612899998));
#201584=CARTESIAN_POINT('Ctrl Pts',(9.64342701399995,15.2,4.83520117199999));
#201585=CARTESIAN_POINT('Ctrl Pts',(9.64342701399995,11.6,4.83520117199998));
#201586=CARTESIAN_POINT('Ctrl Pts',(9.64533917899994,15.2,4.83700192299998));
#201587=CARTESIAN_POINT('Ctrl Pts',(9.64533917899994,11.6,4.83700192299998));
#201588=CARTESIAN_POINT('Ctrl Pts',(9.64725414199994,15.2,4.83880837999998));
#201589=CARTESIAN_POINT('Ctrl Pts',(9.64725414199994,11.6,4.83880837999998));
#201590=CARTESIAN_POINT('Ctrl Pts',(9.64917188799994,15.2,4.84062053999998));
#201591=CARTESIAN_POINT('Ctrl Pts',(9.64917188799994,11.6,4.84062053999998));
#201592=CARTESIAN_POINT('Ctrl Pts',(9.65109240199994,15.2,4.84243840399999));
#201593=CARTESIAN_POINT('Ctrl Pts',(9.65109240199994,11.6,4.84243840399999));
#201594=CARTESIAN_POINT('Ctrl Pts',(9.65301566999995,15.2,4.84426196999999));
#201595=CARTESIAN_POINT('Ctrl Pts',(9.65301566999995,11.6,4.84426196999998));
#201596=CARTESIAN_POINT('Ctrl Pts',(9.65494167899994,15.2,4.84609123599999));
#201597=CARTESIAN_POINT('Ctrl Pts',(9.65494167899994,11.6,4.84609123599998));
#201598=CARTESIAN_POINT('Ctrl Pts',(9.65687041399995,15.2,4.84792620099999));
#201599=CARTESIAN_POINT('Ctrl Pts',(9.65687041399995,11.6,4.84792620099998));
#201600=CARTESIAN_POINT('Ctrl Pts',(9.65880185999995,15.2,4.84976686399998));
#201601=CARTESIAN_POINT('Ctrl Pts',(9.65880185999995,11.6,4.84976686399998));
#201602=CARTESIAN_POINT('Ctrl Pts',(9.66073600599995,15.2,4.85161322299999));
#201603=CARTESIAN_POINT('Ctrl Pts',(9.66073600599995,11.6,4.85161322299999));
#201604=CARTESIAN_POINT('Ctrl Pts',(9.66267283399995,15.2,4.85346527699999));
#201605=CARTESIAN_POINT('Ctrl Pts',(9.66267283399995,11.6,4.85346527699999));
#201606=CARTESIAN_POINT('Ctrl Pts',(9.66461233399994,15.2,4.85532302499998));
#201607=CARTESIAN_POINT('Ctrl Pts',(9.66461233399994,11.6,4.85532302499998));
#201608=CARTESIAN_POINT('Ctrl Pts',(9.66655448999994,15.2,4.85718646399998));
#201609=CARTESIAN_POINT('Ctrl Pts',(9.66655448999994,11.6,4.85718646399998));
#201610=CARTESIAN_POINT('Ctrl Pts',(9.66849928799994,15.2,4.85905559599999));
#201611=CARTESIAN_POINT('Ctrl Pts',(9.66849928799994,11.6,4.85905559599999));
#201612=CARTESIAN_POINT('Ctrl Pts',(9.67044671499995,15.2,4.86093041599998));
#201613=CARTESIAN_POINT('Ctrl Pts',(9.67044671499995,11.6,4.86093041599998));
#201614=CARTESIAN_POINT('Ctrl Pts',(9.67239675599994,15.2,4.86281092499999));
#201615=CARTESIAN_POINT('Ctrl Pts',(9.67239675599994,11.6,4.86281092499999));
#201616=CARTESIAN_POINT('Ctrl Pts',(9.67434939899994,15.2,4.86469711899999));
#201617=CARTESIAN_POINT('Ctrl Pts',(9.67434939899994,11.6,4.86469711899998));
#201618=CARTESIAN_POINT('Ctrl Pts',(9.67630462799994,15.2,4.86658899999998));
#201619=CARTESIAN_POINT('Ctrl Pts',(9.67630462799994,11.6,4.86658899999998));
#201620=CARTESIAN_POINT('Ctrl Pts',(9.67826243199994,15.2,4.86848656399999));
#201621=CARTESIAN_POINT('Ctrl Pts',(9.67826243199994,11.6,4.86848656399999));
#201622=CARTESIAN_POINT('Ctrl Pts',(9.68022279599994,15.2,4.87038981099998));
#201623=CARTESIAN_POINT('Ctrl Pts',(9.68022279599994,11.6,4.87038981099998));
#201624=CARTESIAN_POINT('Ctrl Pts',(9.68218570499995,15.2,4.87229873799999));
#201625=CARTESIAN_POINT('Ctrl Pts',(9.68218570499995,11.6,4.87229873799999));
#201626=CARTESIAN_POINT('Ctrl Pts',(9.68415114899994,15.2,4.87421334499999));
#201627=CARTESIAN_POINT('Ctrl Pts',(9.68415114899994,11.6,4.87421334499999));
#201628=CARTESIAN_POINT('Ctrl Pts',(9.68611910999994,15.2,4.87613362999999));
#201629=CARTESIAN_POINT('Ctrl Pts',(9.68611910999994,11.6,4.87613362999998));
#201630=CARTESIAN_POINT('Ctrl Pts',(9.68808957799994,15.2,4.87805959199999));
#201631=CARTESIAN_POINT('Ctrl Pts',(9.68808957799994,11.6,4.87805959199999));
#201632=CARTESIAN_POINT('Ctrl Pts',(9.69006253799994,15.2,4.87999122899998));
#201633=CARTESIAN_POINT('Ctrl Pts',(9.69006253799994,11.6,4.87999122899998));
#201634=CARTESIAN_POINT('Ctrl Pts',(9.69203797799995,15.2,4.88192853999998));
#201635=CARTESIAN_POINT('Ctrl Pts',(9.69203797799995,11.6,4.88192853999998));
#201636=CARTESIAN_POINT('Ctrl Pts',(9.69401588199995,15.2,4.88387152299998));
#201637=CARTESIAN_POINT('Ctrl Pts',(9.69401588199995,11.6,4.88387152299998));
#201638=CARTESIAN_POINT('Ctrl Pts',(9.69599623899994,15.2,4.88582017699999));
#201639=CARTESIAN_POINT('Ctrl Pts',(9.69599623899994,11.6,4.88582017699999));
#201640=CARTESIAN_POINT('Ctrl Pts',(9.69797903399994,15.2,4.88777450099998));
#201641=CARTESIAN_POINT('Ctrl Pts',(9.69797903399994,11.6,4.88777450099998));
#201642=CARTESIAN_POINT('Ctrl Pts',(9.69996425399994,15.2,4.88973449099999));
#201643=CARTESIAN_POINT('Ctrl Pts',(9.69996425399994,11.6,4.88973449099999));
#201644=CARTESIAN_POINT('Ctrl Pts',(9.70195188699994,15.2,4.89170014899998));
#201645=CARTESIAN_POINT('Ctrl Pts',(9.70195188699994,11.6,4.89170014899998));
#201646=CARTESIAN_POINT('Ctrl Pts',(9.70394191899994,15.2,4.89367147199999));
#201647=CARTESIAN_POINT('Ctrl Pts',(9.70394191899994,11.6,4.89367147199999));
#201648=CARTESIAN_POINT('Ctrl Pts',(9.70593433699995,15.2,4.89564845699999));
#201649=CARTESIAN_POINT('Ctrl Pts',(9.70593433699995,11.6,4.89564845699998));
#201650=CARTESIAN_POINT('Ctrl Pts',(9.70792912699994,15.2,4.89763110499998));
#201651=CARTESIAN_POINT('Ctrl Pts',(9.70792912699994,11.6,4.89763110499998));
#201652=CARTESIAN_POINT('Ctrl Pts',(9.70992627599994,15.2,4.89961941299998));
#201653=CARTESIAN_POINT('Ctrl Pts',(9.70992627599994,11.6,4.89961941299998));
#201654=CARTESIAN_POINT('Ctrl Pts',(9.71192577199995,15.2,4.90161337999999));
#201655=CARTESIAN_POINT('Ctrl Pts',(9.71192577199995,11.6,4.90161337999999));
#201656=CARTESIAN_POINT('Ctrl Pts',(9.71392760099994,15.2,4.90361300399999));
#201657=CARTESIAN_POINT('Ctrl Pts',(9.71392760099994,11.6,4.90361300399999));
#201658=CARTESIAN_POINT('Ctrl Pts',(9.71593175099994,15.2,4.90561828399999));
#201659=CARTESIAN_POINT('Ctrl Pts',(9.71593175099994,11.6,4.90561828399999));
#201660=CARTESIAN_POINT('Ctrl Pts',(9.71793820699995,15.2,4.90762921799998));
#201661=CARTESIAN_POINT('Ctrl Pts',(9.71793820699995,11.6,4.90762921799998));
#201662=CARTESIAN_POINT('Ctrl Pts',(9.71994695799994,15.2,4.90964580499998));
#201663=CARTESIAN_POINT('Ctrl Pts',(9.71994695799994,11.6,4.90964580499998));
#201664=CARTESIAN_POINT('Ctrl Pts',(9.72195798999994,15.2,4.91166804299999));
#201665=CARTESIAN_POINT('Ctrl Pts',(9.72195798999994,11.6,4.91166804299999));
#201666=CARTESIAN_POINT('Ctrl Pts',(9.72397129099994,15.2,4.91369592999998));
#201667=CARTESIAN_POINT('Ctrl Pts',(9.72397129099994,11.6,4.91369592999998));
#201668=CARTESIAN_POINT('Ctrl Pts',(9.72598684699994,15.2,4.91572946599998));
#201669=CARTESIAN_POINT('Ctrl Pts',(9.72598684699994,11.6,4.91572946599998));
#201670=CARTESIAN_POINT('Ctrl Pts',(9.72800464599995,15.2,4.91776864699998));
#201671=CARTESIAN_POINT('Ctrl Pts',(9.72800464599995,11.6,4.91776864699998));
#201672=CARTESIAN_POINT('Ctrl Pts',(9.73002467399994,15.2,4.91981347399999));
#201673=CARTESIAN_POINT('Ctrl Pts',(9.73002467399994,11.6,4.91981347399999));
#201674=CARTESIAN_POINT('Ctrl Pts',(9.73204691999995,15.2,4.92186394399998));
#201675=CARTESIAN_POINT('Ctrl Pts',(9.73204691999995,11.6,4.92186394399998));
#201676=CARTESIAN_POINT('Ctrl Pts',(9.73407136999995,15.2,4.92392005599999));
#201677=CARTESIAN_POINT('Ctrl Pts',(9.73407136999995,11.6,4.92392005599999));
#201678=CARTESIAN_POINT('Ctrl Pts',(9.73609801199995,15.2,4.92598180799998));
#201679=CARTESIAN_POINT('Ctrl Pts',(9.73609801199995,11.6,4.92598180799998));
#201680=CARTESIAN_POINT('Ctrl Pts',(9.73812683299995,15.2,4.92804919799998));
#201681=CARTESIAN_POINT('Ctrl Pts',(9.73812683299995,11.6,4.92804919799998));
#201682=CARTESIAN_POINT('Ctrl Pts',(9.74015781999995,15.2,4.93012222599998));
#201683=CARTESIAN_POINT('Ctrl Pts',(9.74015781999995,11.6,4.93012222599998));
#201684=CARTESIAN_POINT('Ctrl Pts',(9.74219095999995,15.2,4.93220088799998));
#201685=CARTESIAN_POINT('Ctrl Pts',(9.74219095999995,11.6,4.93220088799998));
#201686=CARTESIAN_POINT('Ctrl Pts',(9.74422624199994,15.2,4.93428518399998));
#201687=CARTESIAN_POINT('Ctrl Pts',(9.74422624199994,11.6,4.93428518399998));
#201688=CARTESIAN_POINT('Ctrl Pts',(9.74626365199994,15.2,4.93637511299998));
#201689=CARTESIAN_POINT('Ctrl Pts',(9.74626365199994,11.6,4.93637511299998));
#201690=CARTESIAN_POINT('Ctrl Pts',(9.74830317899994,15.2,4.93847067099999));
#201691=CARTESIAN_POINT('Ctrl Pts',(9.74830317899994,11.6,4.93847067099999));
#201692=CARTESIAN_POINT('Ctrl Pts',(9.75034480799994,15.2,4.94057185899998));
#201693=CARTESIAN_POINT('Ctrl Pts',(9.75034480799994,11.6,4.94057185899998));
#201694=CARTESIAN_POINT('Ctrl Pts',(9.75238852899994,15.2,4.94267867299998));
#201695=CARTESIAN_POINT('Ctrl Pts',(9.75238852899994,11.6,4.94267867299998));
#201696=CARTESIAN_POINT('Ctrl Pts',(9.75443432899995,15.2,4.94479111299999));
#201697=CARTESIAN_POINT('Ctrl Pts',(9.75443432899995,11.6,4.94479111299999));
#201698=CARTESIAN_POINT('Ctrl Pts',(9.75648219399995,15.2,4.94690917699998));
#201699=CARTESIAN_POINT('Ctrl Pts',(9.75648219399995,11.6,4.94690917699998));
#201700=CARTESIAN_POINT('Ctrl Pts',(9.75853211299994,15.2,4.94903286299999));
#201701=CARTESIAN_POINT('Ctrl Pts',(9.75853211299994,11.6,4.94903286299999));
#201702=CARTESIAN_POINT('Ctrl Pts',(9.76058407399995,15.2,4.95116216999998));
#201703=CARTESIAN_POINT('Ctrl Pts',(9.76058407399995,11.6,4.95116216999998));
#201704=CARTESIAN_POINT('Ctrl Pts',(9.76263806299994,15.2,4.95329709499998));
#201705=CARTESIAN_POINT('Ctrl Pts',(9.76263806299994,11.6,4.95329709499998));
#201706=CARTESIAN_POINT('Ctrl Pts',(9.76469407099994,15.2,4.95543763899998));
#201707=CARTESIAN_POINT('Ctrl Pts',(9.76469407099994,11.6,4.95543763899998));
#201708=CARTESIAN_POINT('Ctrl Pts',(9.76675208199994,15.2,4.95758379699998));
#201709=CARTESIAN_POINT('Ctrl Pts',(9.76675208199994,11.6,4.95758379699998));
#201710=CARTESIAN_POINT('Ctrl Pts',(9.76881208499995,15.2,4.95973556899998));
#201711=CARTESIAN_POINT('Ctrl Pts',(9.76881208499995,11.6,4.95973556899998));
#201712=CARTESIAN_POINT('Ctrl Pts',(9.77087406899994,15.2,4.96189295299998));
#201713=CARTESIAN_POINT('Ctrl Pts',(9.77087406899994,11.6,4.96189295299998));
#201714=CARTESIAN_POINT('Ctrl Pts',(9.77293801999994,15.2,4.96405594799998));
#201715=CARTESIAN_POINT('Ctrl Pts',(9.77293801999994,11.6,4.96405594799998));
#201716=CARTESIAN_POINT('Ctrl Pts',(9.77500392799995,15.2,4.96622455099998));
#201717=CARTESIAN_POINT('Ctrl Pts',(9.77500392799995,11.6,4.96622455099998));
#201718=CARTESIAN_POINT('Ctrl Pts',(9.77707177899994,15.2,4.96839876199999));
#201719=CARTESIAN_POINT('Ctrl Pts',(9.77707177899994,11.6,4.96839876199999));
#201720=CARTESIAN_POINT('Ctrl Pts',(9.77914156199994,15.2,4.97057857799999));
#201721=CARTESIAN_POINT('Ctrl Pts',(9.77914156199994,11.6,4.97057857799999));
#201722=CARTESIAN_POINT('Ctrl Pts',(9.78121326399994,15.2,4.97276399699999));
#201723=CARTESIAN_POINT('Ctrl Pts',(9.78121326399994,11.6,4.97276399699999));
#201724=CARTESIAN_POINT('Ctrl Pts',(9.78328687399994,15.2,4.97495501899999));
#201725=CARTESIAN_POINT('Ctrl Pts',(9.78328687399994,11.6,4.97495501899999));
#201726=CARTESIAN_POINT('Ctrl Pts',(9.78536237899995,15.2,4.97715163999998));
#201727=CARTESIAN_POINT('Ctrl Pts',(9.78536237899995,11.6,4.97715163999998));
#201728=CARTESIAN_POINT('Ctrl Pts',(9.78743976799995,15.2,4.97935385999998));
#201729=CARTESIAN_POINT('Ctrl Pts',(9.78743976799995,11.6,4.97935385999998));
#201730=CARTESIAN_POINT('Ctrl Pts',(9.78951902799994,15.2,4.98156167799999));
#201731=CARTESIAN_POINT('Ctrl Pts',(9.78951902799994,11.6,4.98156167799999));
#201732=CARTESIAN_POINT('Ctrl Pts',(9.79160014799995,15.2,4.98377508899999));
#201733=CARTESIAN_POINT('Ctrl Pts',(9.79160014799995,11.6,4.98377508899999));
#201734=CARTESIAN_POINT('Ctrl Pts',(9.79368311599995,15.2,4.98599409399999));
#201735=CARTESIAN_POINT('Ctrl Pts',(9.79368311599995,11.6,4.98599409399999));
#201736=CARTESIAN_POINT('Ctrl Pts',(9.79576791999994,15.2,4.98821869099999));
#201737=CARTESIAN_POINT('Ctrl Pts',(9.79576791999994,11.6,4.98821869099999));
#201738=CARTESIAN_POINT('Ctrl Pts',(9.79785454699994,15.2,4.99044887699998));
#201739=CARTESIAN_POINT('Ctrl Pts',(9.79785454699994,11.6,4.99044887699998));
#201740=CARTESIAN_POINT('Ctrl Pts',(9.79994298799994,15.2,4.99268464999999));
#201741=CARTESIAN_POINT('Ctrl Pts',(9.79994298799994,11.6,4.99268464999999));
#201742=CARTESIAN_POINT('Ctrl Pts',(9.80203322899994,15.2,4.99492601099998));
#201743=CARTESIAN_POINT('Ctrl Pts',(9.80203322899994,11.6,4.99492601099998));
#201744=CARTESIAN_POINT('Ctrl Pts',(9.80412525799995,15.2,4.99717295599999));
#201745=CARTESIAN_POINT('Ctrl Pts',(9.80412525799995,11.6,4.99717295599999));
#201746=CARTESIAN_POINT('Ctrl Pts',(9.80621906499995,15.2,4.99942548299998));
#201747=CARTESIAN_POINT('Ctrl Pts',(9.80621906499995,11.6,4.99942548299998));
#201748=CARTESIAN_POINT('Ctrl Pts',(9.80831463599995,15.2,5.00168359099998));
#201749=CARTESIAN_POINT('Ctrl Pts',(9.80831463599995,11.6,5.00168359099998));
#201750=CARTESIAN_POINT('Ctrl Pts',(9.81041196099994,15.2,5.00394727899998));
#201751=CARTESIAN_POINT('Ctrl Pts',(9.81041196099994,11.6,5.00394727899998));
#201752=CARTESIAN_POINT('Ctrl Pts',(9.81251102899994,15.2,5.00621654299999));
#201753=CARTESIAN_POINT('Ctrl Pts',(9.81251102899994,11.6,5.00621654299999));
#201754=CARTESIAN_POINT('Ctrl Pts',(9.81461182699995,15.2,5.00849138199998));
#201755=CARTESIAN_POINT('Ctrl Pts',(9.81461182699995,11.6,5.00849138199998));
#201756=CARTESIAN_POINT('Ctrl Pts',(9.81671434399994,15.2,5.01077179599999));
#201757=CARTESIAN_POINT('Ctrl Pts',(9.81671434399994,11.6,5.01077179599999));
#201758=CARTESIAN_POINT('Ctrl Pts',(9.81881856699994,15.2,5.01305778199999));
#201759=CARTESIAN_POINT('Ctrl Pts',(9.81881856699994,11.6,5.01305778199999));
#201760=CARTESIAN_POINT('Ctrl Pts',(9.82092448599994,15.2,5.01534933699999));
#201761=CARTESIAN_POINT('Ctrl Pts',(9.82092448599994,11.6,5.01534933699999));
#201762=CARTESIAN_POINT('Ctrl Pts',(9.82303208999994,15.2,5.01764645999998));
#201763=CARTESIAN_POINT('Ctrl Pts',(9.82303208999994,11.6,5.01764645999998));
#201764=CARTESIAN_POINT('Ctrl Pts',(9.82514136599995,15.2,5.01994915099999));
#201765=CARTESIAN_POINT('Ctrl Pts',(9.82514136599995,11.6,5.01994915099999));
#201766=CARTESIAN_POINT('Ctrl Pts',(9.82725230399994,15.2,5.02225740599999));
#201767=CARTESIAN_POINT('Ctrl Pts',(9.82725230399994,11.6,5.02225740599999));
#201768=CARTESIAN_POINT('Ctrl Pts',(9.82936489099995,15.2,5.02457122199999));
#201769=CARTESIAN_POINT('Ctrl Pts',(9.82936489099995,11.6,5.02457122199999));
#201770=CARTESIAN_POINT('Ctrl Pts',(9.83147911699995,15.2,5.02689060099998));
#201771=CARTESIAN_POINT('Ctrl Pts',(9.83147911699995,11.6,5.02689060099998));
#201772=CARTESIAN_POINT('Ctrl Pts',(9.83359496999994,15.2,5.02921553799998));
#201773=CARTESIAN_POINT('Ctrl Pts',(9.83359496999994,11.6,5.02921553799998));
#201774=CARTESIAN_POINT('Ctrl Pts',(9.83571243799994,15.2,5.03154603299999));
#201775=CARTESIAN_POINT('Ctrl Pts',(9.83571243799994,11.6,5.03154603299999));
#201776=CARTESIAN_POINT('Ctrl Pts',(9.83783150999994,15.2,5.03388208199999));
#201777=CARTESIAN_POINT('Ctrl Pts',(9.83783150999994,11.6,5.03388208199999));
#201778=CARTESIAN_POINT('Ctrl Pts',(9.83995217599994,15.2,5.03622368599999));
#201779=CARTESIAN_POINT('Ctrl Pts',(9.83995217599994,11.6,5.03622368599999));
#201780=CARTESIAN_POINT('Ctrl Pts',(9.84207442399994,15.2,5.03857083999999));
#201781=CARTESIAN_POINT('Ctrl Pts',(9.84207442399994,11.6,5.03857083999999));
#201782=CARTESIAN_POINT('Ctrl Pts',(9.84419824199994,15.2,5.04092354499999));
#201783=CARTESIAN_POINT('Ctrl Pts',(9.84419824199994,11.6,5.04092354499999));
#201784=CARTESIAN_POINT('Ctrl Pts',(9.84632361899994,15.2,5.04328179799998));
#201785=CARTESIAN_POINT('Ctrl Pts',(9.84632361899994,11.6,5.04328179799998));
#201786=CARTESIAN_POINT('Ctrl Pts',(9.84845054499995,15.2,5.04564559599999));
#201787=CARTESIAN_POINT('Ctrl Pts',(9.84845054499995,11.6,5.04564559599999));
#201788=CARTESIAN_POINT('Ctrl Pts',(9.85057900699994,15.2,5.04801493799999));
#201789=CARTESIAN_POINT('Ctrl Pts',(9.85057900699994,11.6,5.04801493799999));
#201790=CARTESIAN_POINT('Ctrl Pts',(9.85270899399995,15.2,5.05038982299999));
#201791=CARTESIAN_POINT('Ctrl Pts',(9.85270899399995,11.6,5.05038982299999));
#201792=CARTESIAN_POINT('Ctrl Pts',(9.85484049599994,15.2,5.05277024799998));
#201793=CARTESIAN_POINT('Ctrl Pts',(9.85484049599994,11.6,5.05277024799998));
#201794=CARTESIAN_POINT('Ctrl Pts',(9.85697350299995,15.2,5.05515621099998));
#201795=CARTESIAN_POINT('Ctrl Pts',(9.85697350299995,11.6,5.05515621099998));
#201796=CARTESIAN_POINT('Ctrl Pts',(9.85910800099994,15.2,5.05754771199998));
#201797=CARTESIAN_POINT('Ctrl Pts',(9.85910800099994,11.6,5.05754771199998));
#201798=CARTESIAN_POINT('Ctrl Pts',(9.86124398099994,15.2,5.05994474699998));
#201799=CARTESIAN_POINT('Ctrl Pts',(9.86124398099994,11.6,5.05994474699998));
#201800=CARTESIAN_POINT('Ctrl Pts',(9.86338143099994,15.2,5.06234731299998));
#201801=CARTESIAN_POINT('Ctrl Pts',(9.86338143099994,11.6,5.06234731299998));
#201802=CARTESIAN_POINT('Ctrl Pts',(9.86552033999994,15.2,5.06475541199999));
#201803=CARTESIAN_POINT('Ctrl Pts',(9.86552033999994,11.6,5.06475541199999));
#201804=CARTESIAN_POINT('Ctrl Pts',(9.86766069799994,15.2,5.06716903899999));
#201805=CARTESIAN_POINT('Ctrl Pts',(9.86766069799994,11.6,5.06716903899999));
#201806=CARTESIAN_POINT('Ctrl Pts',(9.86980249199994,15.2,5.06958819299999));
#201807=CARTESIAN_POINT('Ctrl Pts',(9.86980249199994,11.6,5.06958819299999));
#201808=CARTESIAN_POINT('Ctrl Pts',(9.87194571399994,15.2,5.07201287199998));
#201809=CARTESIAN_POINT('Ctrl Pts',(9.87194571399994,11.6,5.07201287199998));
#201810=CARTESIAN_POINT('Ctrl Pts',(9.87409035199994,15.2,5.07444307399999));
#201811=CARTESIAN_POINT('Ctrl Pts',(9.87409035199994,11.6,5.07444307399999));
#201812=CARTESIAN_POINT('Ctrl Pts',(9.87623639299994,15.2,5.07687879699999));
#201813=CARTESIAN_POINT('Ctrl Pts',(9.87623639299994,11.6,5.07687879699999));
#201814=CARTESIAN_POINT('Ctrl Pts',(9.87838382799995,15.2,5.07932003999999));
#201815=CARTESIAN_POINT('Ctrl Pts',(9.87838382799995,11.6,5.07932003999999));
#201816=CARTESIAN_POINT('Ctrl Pts',(9.88053264699994,15.2,5.08176679899999));
#201817=CARTESIAN_POINT('Ctrl Pts',(9.88053264699994,11.6,5.08176679899999));
#201818=CARTESIAN_POINT('Ctrl Pts',(9.88268283699995,15.2,5.08421907399998));
#201819=CARTESIAN_POINT('Ctrl Pts',(9.88268283699995,11.6,5.08421907399998));
#201820=CARTESIAN_POINT('Ctrl Pts',(9.88483438899994,15.2,5.08667686299999));
#201821=CARTESIAN_POINT('Ctrl Pts',(9.88483438899994,11.6,5.08667686299999));
#201822=CARTESIAN_POINT('Ctrl Pts',(9.88698729099994,15.2,5.08914016199999));
#201823=CARTESIAN_POINT('Ctrl Pts',(9.88698729099994,11.6,5.08914016199999));
#201824=CARTESIAN_POINT('Ctrl Pts',(9.88914153299995,15.2,5.09160897099999));
#201825=CARTESIAN_POINT('Ctrl Pts',(9.88914153299995,11.6,5.09160897099999));
#201826=CARTESIAN_POINT('Ctrl Pts',(9.89129710499994,15.2,5.09408328799999));
#201827=CARTESIAN_POINT('Ctrl Pts',(9.89129710499994,11.6,5.09408328799999));
#201828=CARTESIAN_POINT('Ctrl Pts',(9.89345399399994,15.2,5.09656310999999));
#201829=CARTESIAN_POINT('Ctrl Pts',(9.89345399399994,11.6,5.09656310999999));
#201830=CARTESIAN_POINT('Ctrl Pts',(9.89561219199994,15.2,5.09904843499999));
#201831=CARTESIAN_POINT('Ctrl Pts',(9.89561219199994,11.6,5.09904843499999));
#201832=CARTESIAN_POINT('Ctrl Pts',(9.89777168699994,15.2,5.10153926199998));
#201833=CARTESIAN_POINT('Ctrl Pts',(9.89777168699994,11.6,5.10153926199998));
#201834=CARTESIAN_POINT('Ctrl Pts',(9.89993246699994,15.2,5.10403558799998));
#201835=CARTESIAN_POINT('Ctrl Pts',(9.89993246699994,11.6,5.10403558799998));
#201836=CARTESIAN_POINT('Ctrl Pts',(9.90209452399995,15.2,5.10653741199998));
#201837=CARTESIAN_POINT('Ctrl Pts',(9.90209452399995,11.6,5.10653741199998));
#201838=CARTESIAN_POINT('Ctrl Pts',(9.90425784599994,15.2,5.10904473199999));
#201839=CARTESIAN_POINT('Ctrl Pts',(9.90425784599994,11.6,5.10904473199999));
#201840=CARTESIAN_POINT('Ctrl Pts',(9.90642242299995,15.2,5.11155754499999));
#201841=CARTESIAN_POINT('Ctrl Pts',(9.90642242299995,11.6,5.11155754499999));
#201842=CARTESIAN_POINT('Ctrl Pts',(9.90858824399995,15.2,5.11407584799999));
#201843=CARTESIAN_POINT('Ctrl Pts',(9.90858824399995,11.6,5.11407584799999));
#201844=CARTESIAN_POINT('Ctrl Pts',(9.91075529899994,15.2,5.11659964199998));
#201845=CARTESIAN_POINT('Ctrl Pts',(9.91075529899994,11.6,5.11659964199998));
#201846=CARTESIAN_POINT('Ctrl Pts',(9.91292357699994,15.2,5.11912892399998));
#201847=CARTESIAN_POINT('Ctrl Pts',(9.91292357699994,11.6,5.11912892399998));
#201848=CARTESIAN_POINT('Ctrl Pts',(9.91509306699994,15.2,5.12166369099998));
#201849=CARTESIAN_POINT('Ctrl Pts',(9.91509306699994,11.6,5.12166369099998));
#201850=CARTESIAN_POINT('Ctrl Pts',(9.91726375999994,15.2,5.12420394099999));
#201851=CARTESIAN_POINT('Ctrl Pts',(9.91726375999994,11.6,5.12420394099999));
#201852=CARTESIAN_POINT('Ctrl Pts',(9.91943564399994,15.2,5.12674967299999));
#201853=CARTESIAN_POINT('Ctrl Pts',(9.91943564399994,11.6,5.12674967299999));
#201854=CARTESIAN_POINT('Ctrl Pts',(9.92160870899994,15.2,5.12930088399998));
#201855=CARTESIAN_POINT('Ctrl Pts',(9.92160870899994,11.6,5.12930088399998));
#201856=CARTESIAN_POINT('Ctrl Pts',(9.92378294699994,15.2,5.13185757199999));
#201857=CARTESIAN_POINT('Ctrl Pts',(9.92378294699994,11.6,5.13185757199999));
#201858=CARTESIAN_POINT('Ctrl Pts',(9.92595834399994,15.2,5.13441973499998));
#201859=CARTESIAN_POINT('Ctrl Pts',(9.92595834399994,11.6,5.13441973499998));
#201860=CARTESIAN_POINT('Ctrl Pts',(9.92813489199994,15.2,5.13698737299999));
#201861=CARTESIAN_POINT('Ctrl Pts',(9.92813489199994,11.6,5.13698737299999));
#201862=CARTESIAN_POINT('Ctrl Pts',(9.93031257999995,15.2,5.13956047999999));
#201863=CARTESIAN_POINT('Ctrl Pts',(9.93031257999995,11.6,5.13956047999999));
#201864=CARTESIAN_POINT('Ctrl Pts',(9.93249139799994,15.2,5.14213905799998));
#201865=CARTESIAN_POINT('Ctrl Pts',(9.93249139799994,11.6,5.14213905799998));
#201866=CARTESIAN_POINT('Ctrl Pts',(9.93467133499994,15.2,5.14472310099999));
#201867=CARTESIAN_POINT('Ctrl Pts',(9.93467133499994,11.6,5.14472310099999));
#201868=CARTESIAN_POINT('Ctrl Pts',(9.93685238099994,15.2,5.14731261099998));
#201869=CARTESIAN_POINT('Ctrl Pts',(9.93685238099994,11.6,5.14731261099998));
#201870=CARTESIAN_POINT('Ctrl Pts',(9.93903452599995,15.2,5.14990758299999));
#201871=CARTESIAN_POINT('Ctrl Pts',(9.93903452599995,11.6,5.14990758299999));
#201872=CARTESIAN_POINT('Ctrl Pts',(9.94121775999995,15.2,5.15250801599999));
#201873=CARTESIAN_POINT('Ctrl Pts',(9.94121775999995,11.6,5.15250801599999));
#201874=CARTESIAN_POINT('Ctrl Pts',(9.94340207299994,15.2,5.15511390799999));
#201875=CARTESIAN_POINT('Ctrl Pts',(9.94340207299994,11.6,5.15511390799999));
#201876=CARTESIAN_POINT('Ctrl Pts',(9.94558745299994,15.2,5.15772525699998));
#201877=CARTESIAN_POINT('Ctrl Pts',(9.94558745299994,11.6,5.15772525699998));
#201878=CARTESIAN_POINT('Ctrl Pts',(9.94777389299994,15.2,5.16034205899999));
#201879=CARTESIAN_POINT('Ctrl Pts',(9.94777389299994,11.6,5.16034205899999));
#201880=CARTESIAN_POINT('Ctrl Pts',(9.94996137999994,15.2,5.16296431599999));
#201881=CARTESIAN_POINT('Ctrl Pts',(9.94996137999994,11.6,5.16296431599999));
#201882=CARTESIAN_POINT('Ctrl Pts',(9.95214990599995,15.2,5.16559202199999));
#201883=CARTESIAN_POINT('Ctrl Pts',(9.95214990599995,11.6,5.16559202199999));
#201884=CARTESIAN_POINT('Ctrl Pts',(9.95433945899994,15.2,5.16822517599999));
#201885=CARTESIAN_POINT('Ctrl Pts',(9.95433945899994,11.6,5.16822517599999));
#201886=CARTESIAN_POINT('Ctrl Pts',(9.95653002999994,15.2,5.17086377699999));
#201887=CARTESIAN_POINT('Ctrl Pts',(9.95653002999994,11.6,5.17086377699999));
#201888=CARTESIAN_POINT('Ctrl Pts',(9.95872160899994,15.2,5.17350782199999));
#201889=CARTESIAN_POINT('Ctrl Pts',(9.95872160899994,11.6,5.17350782199999));
#201890=CARTESIAN_POINT('Ctrl Pts',(9.96091418499994,15.2,5.17615730899998));
#201891=CARTESIAN_POINT('Ctrl Pts',(9.96091418499994,11.6,5.17615730899998));
#201892=CARTESIAN_POINT('Ctrl Pts',(9.96310774999994,15.2,5.17881223599999));
#201893=CARTESIAN_POINT('Ctrl Pts',(9.96310774999994,11.6,5.17881223599999));
#201894=CARTESIAN_POINT('Ctrl Pts',(9.96530229299994,15.2,5.18147260099998));
#201895=CARTESIAN_POINT('Ctrl Pts',(9.96530229299994,11.6,5.18147260099998));
#201896=CARTESIAN_POINT('Ctrl Pts',(9.96749780299995,15.2,5.18413840099999));
#201897=CARTESIAN_POINT('Ctrl Pts',(9.96749780299995,11.6,5.18413840099999));
#201898=CARTESIAN_POINT('Ctrl Pts',(9.96969427099994,15.2,5.18680963599999));
#201899=CARTESIAN_POINT('Ctrl Pts',(9.96969427099994,11.6,5.18680963599999));
#201900=CARTESIAN_POINT('Ctrl Pts',(9.97189168699995,15.2,5.18948630099998));
#201901=CARTESIAN_POINT('Ctrl Pts',(9.97189168699995,11.6,5.18948630099998));
#201902=CARTESIAN_POINT('Ctrl Pts',(9.97409004199995,15.2,5.19216839499999));
#201903=CARTESIAN_POINT('Ctrl Pts',(9.97409004199995,11.6,5.19216839499999));
#201904=CARTESIAN_POINT('Ctrl Pts',(9.97628932499994,15.2,5.19485591699999));
#201905=CARTESIAN_POINT('Ctrl Pts',(9.97628932499994,11.6,5.19485591699999));
#201906=CARTESIAN_POINT('Ctrl Pts',(9.97848952599995,15.2,5.19754886499998));
#201907=CARTESIAN_POINT('Ctrl Pts',(9.97848952599995,11.6,5.19754886499998));
#201908=CARTESIAN_POINT('Ctrl Pts',(9.98069063599995,15.2,5.20024723399998));
#201909=CARTESIAN_POINT('Ctrl Pts',(9.98069063599995,11.6,5.20024723399998));
#201910=CARTESIAN_POINT('Ctrl Pts',(9.98289264399994,15.2,5.20295102499999));
#201911=CARTESIAN_POINT('Ctrl Pts',(9.98289264399994,11.6,5.20295102499999));
#201912=CARTESIAN_POINT('Ctrl Pts',(9.98509554099994,15.2,5.20566023299998));
#201913=CARTESIAN_POINT('Ctrl Pts',(9.98509554099994,11.6,5.20566023299998));
#201914=CARTESIAN_POINT('Ctrl Pts',(9.98729931799994,15.2,5.20837485899998));
#201915=CARTESIAN_POINT('Ctrl Pts',(9.98729931799994,11.6,5.20837485899998));
#201916=CARTESIAN_POINT('Ctrl Pts',(9.98950396399995,15.2,5.21109489899998));
#201917=CARTESIAN_POINT('Ctrl Pts',(9.98950396399995,11.6,5.21109489899998));
#201918=CARTESIAN_POINT('Ctrl Pts',(9.99170946999994,15.2,5.21382035199998));
#201919=CARTESIAN_POINT('Ctrl Pts',(9.99170946999994,11.6,5.21382035199998));
#201920=CARTESIAN_POINT('Ctrl Pts',(9.99391582599995,15.2,5.21655121299998));
#201921=CARTESIAN_POINT('Ctrl Pts',(9.99391582599995,11.6,5.21655121299998));
#201922=CARTESIAN_POINT('Ctrl Pts',(9.99612302199995,15.2,5.21928748299998));
#201923=CARTESIAN_POINT('Ctrl Pts',(9.99612302199995,11.6,5.21928748299998));
#201924=CARTESIAN_POINT('Ctrl Pts',(9.99833104799994,15.2,5.22202915799999));
#201925=CARTESIAN_POINT('Ctrl Pts',(9.99833104799994,11.6,5.22202915799999));
#201926=CARTESIAN_POINT('Ctrl Pts',(10.0005398949999,15.2,5.22477623699999));
#201927=CARTESIAN_POINT('Ctrl Pts',(10.0005398949999,11.6,5.22477623699999));
#201928=CARTESIAN_POINT('Ctrl Pts',(10.0027495549999,15.2,5.22752871599998));
#201929=CARTESIAN_POINT('Ctrl Pts',(10.0027495549999,11.6,5.22752871599998));
#201930=CARTESIAN_POINT('Ctrl Pts',(10.0049600139999,15.2,5.23028659599999));
#201931=CARTESIAN_POINT('Ctrl Pts',(10.0049600139999,11.6,5.23028659599999));
#201932=CARTESIAN_POINT('Ctrl Pts',(10.0071712669999,15.2,5.23304987199998));
#201933=CARTESIAN_POINT('Ctrl Pts',(10.0071712669999,11.6,5.23304987199998));
#201934=CARTESIAN_POINT('Ctrl Pts',(10.0093833019999,15.2,5.23581854099999));
#201935=CARTESIAN_POINT('Ctrl Pts',(10.0093833019999,11.6,5.23581854099999));
#201936=CARTESIAN_POINT('Ctrl Pts',(10.0115961109999,15.2,5.23859260499999));
#201937=CARTESIAN_POINT('Ctrl Pts',(10.0115961109999,11.6,5.23859260499999));
#201938=CARTESIAN_POINT('Ctrl Pts',(10.0138096819999,15.2,5.24137205699999));
#201939=CARTESIAN_POINT('Ctrl Pts',(10.0138096819999,11.6,5.24137205699999));
#201940=CARTESIAN_POINT('Ctrl Pts',(10.0160240069999,15.2,5.24415689899998));
#201941=CARTESIAN_POINT('Ctrl Pts',(10.0160240069999,11.6,5.24415689899998));
#201942=CARTESIAN_POINT('Ctrl Pts',(10.0182390769999,15.2,5.24694712599998));
#201943=CARTESIAN_POINT('Ctrl Pts',(10.0182390769999,11.6,5.24694712599998));
#201944=CARTESIAN_POINT('Ctrl Pts',(10.0204548809999,15.2,5.24974273599998));
#201945=CARTESIAN_POINT('Ctrl Pts',(10.0204548809999,11.6,5.24974273599998));
#201946=CARTESIAN_POINT('Ctrl Pts',(10.0226714119999,15.2,5.25254372899998));
#201947=CARTESIAN_POINT('Ctrl Pts',(10.0226714119999,11.6,5.25254372899998));
#201948=CARTESIAN_POINT('Ctrl Pts',(10.0248886579999,15.2,5.25535009899999));
#201949=CARTESIAN_POINT('Ctrl Pts',(10.0248886579999,11.6,5.25535009899999));
#201950=CARTESIAN_POINT('Ctrl Pts',(10.0271066099999,15.2,5.25816184799999));
#201951=CARTESIAN_POINT('Ctrl Pts',(10.0271066099999,11.6,5.25816184799999));
#201952=CARTESIAN_POINT('Ctrl Pts',(10.0293252589999,15.2,5.26097896999998));
#201953=CARTESIAN_POINT('Ctrl Pts',(10.0293252589999,11.6,5.26097896999998));
#201954=CARTESIAN_POINT('Ctrl Pts',(10.0315445959999,15.2,5.26380146499999));
#201955=CARTESIAN_POINT('Ctrl Pts',(10.0315445959999,11.6,5.26380146499999));
#201956=CARTESIAN_POINT('Ctrl Pts',(10.0337646119999,15.2,5.26662933099999));
#201957=CARTESIAN_POINT('Ctrl Pts',(10.0337646119999,11.6,5.26662933099999));
#201958=CARTESIAN_POINT('Ctrl Pts',(10.0359852959999,15.2,5.26946256499999));
#201959=CARTESIAN_POINT('Ctrl Pts',(10.0359852959999,11.6,5.26946256499999));
#201960=CARTESIAN_POINT('Ctrl Pts',(10.0382066409999,15.2,5.27230116399998));
#201961=CARTESIAN_POINT('Ctrl Pts',(10.0382066409999,11.6,5.27230116399998));
#201962=CARTESIAN_POINT('Ctrl Pts',(10.0404286359999,15.2,5.27514512699998));
#201963=CARTESIAN_POINT('Ctrl Pts',(10.0404286359999,11.6,5.27514512699998));
#201964=CARTESIAN_POINT('Ctrl Pts',(10.0426512719999,15.2,5.27799445199998));
#201965=CARTESIAN_POINT('Ctrl Pts',(10.0426512719999,11.6,5.27799445199998));
#201966=CARTESIAN_POINT('Ctrl Pts',(10.0448745389999,15.2,5.28084913399999));
#201967=CARTESIAN_POINT('Ctrl Pts',(10.0448745389999,11.6,5.28084913399999));
#201968=CARTESIAN_POINT('Ctrl Pts',(10.0470984289999,15.2,5.28370917499998));
#201969=CARTESIAN_POINT('Ctrl Pts',(10.0470984289999,11.6,5.28370917499998));
#201970=CARTESIAN_POINT('Ctrl Pts',(10.0493229319999,15.2,5.28657456899998));
#201971=CARTESIAN_POINT('Ctrl Pts',(10.0493229319999,11.6,5.28657456899998));
#201972=CARTESIAN_POINT('Ctrl Pts',(10.0515480399999,15.2,5.28944531599999));
#201973=CARTESIAN_POINT('Ctrl Pts',(10.0515480399999,11.6,5.28944531599999));
#201974=CARTESIAN_POINT('Ctrl Pts',(10.0537737409999,15.2,5.29232141299998));
#201975=CARTESIAN_POINT('Ctrl Pts',(10.0537737409999,11.6,5.29232141299998));
#201976=CARTESIAN_POINT('Ctrl Pts',(10.0560000299999,15.2,5.29520285799999));
#201977=CARTESIAN_POINT('Ctrl Pts',(10.0560000299999,11.6,5.29520285799999));
#201978=CARTESIAN_POINT('Ctrl Pts',(10.0582268939999,15.2,5.29808964699999));
#201979=CARTESIAN_POINT('Ctrl Pts',(10.0582268939999,11.6,5.29808964699999));
#201980=CARTESIAN_POINT('Ctrl Pts',(10.0604543249999,15.2,5.30098177999999));
#201981=CARTESIAN_POINT('Ctrl Pts',(10.0604543249999,11.6,5.30098177999999));
#201982=CARTESIAN_POINT('Ctrl Pts',(10.0626823149999,15.2,5.30387925299999));
#201983=CARTESIAN_POINT('Ctrl Pts',(10.0626823149999,11.6,5.30387925299999));
#201984=CARTESIAN_POINT('Ctrl Pts',(10.0649108539999,15.2,5.30678206699999));
#201985=CARTESIAN_POINT('Ctrl Pts',(10.0649108539999,11.6,5.30678206699999));
#201986=CARTESIAN_POINT('Ctrl Pts',(10.0671399319999,15.2,5.30969021499998));
#201987=CARTESIAN_POINT('Ctrl Pts',(10.0671399319999,11.6,5.30969021499998));
#201988=CARTESIAN_POINT('Ctrl Pts',(10.0693695419999,15.2,5.31260369799998));
#201989=CARTESIAN_POINT('Ctrl Pts',(10.0693695419999,11.6,5.31260369799998));
#201990=CARTESIAN_POINT('Ctrl Pts',(10.0715996729999,15.2,5.31552251199999));
#201991=CARTESIAN_POINT('Ctrl Pts',(10.0715996729999,11.6,5.31552251199999));
#201992=CARTESIAN_POINT('Ctrl Pts',(10.0738303179999,15.2,5.31844665599999));
#201993=CARTESIAN_POINT('Ctrl Pts',(10.0738303179999,11.6,5.31844665599999));
#201994=CARTESIAN_POINT('Ctrl Pts',(10.0760614659999,15.2,5.32137612699999));
#201995=CARTESIAN_POINT('Ctrl Pts',(10.0760614659999,11.6,5.32137612699999));
#201996=CARTESIAN_POINT('Ctrl Pts',(10.0782931079999,15.2,5.32431092299999));
#201997=CARTESIAN_POINT('Ctrl Pts',(10.0782931079999,11.6,5.32431092299999));
#201998=CARTESIAN_POINT('Ctrl Pts',(10.0805252349999,15.2,5.32725104099999));
#201999=CARTESIAN_POINT('Ctrl Pts',(10.0805252349999,11.6,5.32725104099999));
#202000=CARTESIAN_POINT('Ctrl Pts',(10.0827578399999,15.2,5.33019647899999));
#202001=CARTESIAN_POINT('Ctrl Pts',(10.0827578399999,11.6,5.33019647899999));
#202002=CARTESIAN_POINT('Ctrl Pts',(10.0849909119999,15.2,5.33314723499998));
#202003=CARTESIAN_POINT('Ctrl Pts',(10.0849909119999,11.6,5.33314723499998));
#202004=CARTESIAN_POINT('Ctrl Pts',(10.0872244429999,15.2,5.33610330699998));
#202005=CARTESIAN_POINT('Ctrl Pts',(10.0872244429999,11.6,5.33610330699998));
#202006=CARTESIAN_POINT('Ctrl Pts',(10.0894584239999,15.2,5.33906469199999));
#202007=CARTESIAN_POINT('Ctrl Pts',(10.0894584239999,11.6,5.33906469199999));
#202008=CARTESIAN_POINT('Ctrl Pts',(10.0916928469999,15.2,5.34203138799998));
#202009=CARTESIAN_POINT('Ctrl Pts',(10.0916928469999,11.6,5.34203138799998));
#202010=CARTESIAN_POINT('Ctrl Pts',(10.0939277019999,15.2,5.34500339199998));
#202011=CARTESIAN_POINT('Ctrl Pts',(10.0939277019999,11.6,5.34500339199998));
#202012=CARTESIAN_POINT('Ctrl Pts',(10.0961629809999,15.2,5.34798070299999));
#202013=CARTESIAN_POINT('Ctrl Pts',(10.0961629809999,11.6,5.34798070299999));
#202014=CARTESIAN_POINT('Ctrl Pts',(10.0983986739999,15.2,5.35096331799998));
#202015=CARTESIAN_POINT('Ctrl Pts',(10.0983986739999,11.6,5.35096331799998));
#202016=CARTESIAN_POINT('Ctrl Pts',(10.1006347719999,15.2,5.35395123399999));
#202017=CARTESIAN_POINT('Ctrl Pts',(10.1006347719999,11.6,5.35395123399999));
#202018=CARTESIAN_POINT('Ctrl Pts',(10.1028712649999,15.2,5.35694444899999));
#202019=CARTESIAN_POINT('Ctrl Pts',(10.1028712649999,11.6,5.35694444899999));
#202020=CARTESIAN_POINT('Ctrl Pts',(10.1051081459999,15.2,5.35994296199998));
#202021=CARTESIAN_POINT('Ctrl Pts',(10.1051081459999,11.6,5.35994296199998));
#202022=CARTESIAN_POINT('Ctrl Pts',(10.1073454039999,15.2,5.36294676699999));
#202023=CARTESIAN_POINT('Ctrl Pts',(10.1073454039999,11.6,5.36294676699999));
#202024=CARTESIAN_POINT('Ctrl Pts',(10.1095830319999,15.2,5.36595586499999));
#202025=CARTESIAN_POINT('Ctrl Pts',(10.1095830319999,11.6,5.36595586499999));
#202026=CARTESIAN_POINT('Ctrl Pts',(10.1118210219999,15.2,5.36897025299999));
#202027=CARTESIAN_POINT('Ctrl Pts',(10.1118210219999,11.6,5.36897025299999));
#202028=CARTESIAN_POINT('Ctrl Pts',(10.1140593669999,15.2,5.37198992899998));
#202029=CARTESIAN_POINT('Ctrl Pts',(10.1140593669999,11.6,5.37198992899998));
#202030=CARTESIAN_POINT('Ctrl Pts',(10.1162980569999,15.2,5.37501488899998));
#202031=CARTESIAN_POINT('Ctrl Pts',(10.1162980569999,11.6,5.37501488899998));
#202032=CARTESIAN_POINT('Ctrl Pts',(10.1185370849999,15.2,5.37804513399998));
#202033=CARTESIAN_POINT('Ctrl Pts',(10.1185370849999,11.6,5.37804513399998));
#202034=CARTESIAN_POINT('Ctrl Pts',(10.1207764439999,15.2,5.38108065899999));
#202035=CARTESIAN_POINT('Ctrl Pts',(10.1207764439999,11.6,5.38108065899999));
#202036=CARTESIAN_POINT('Ctrl Pts',(10.1230161179999,15.2,5.38412146299999));
#202037=CARTESIAN_POINT('Ctrl Pts',(10.1230161179999,11.6,5.38412146299999));
#202038=CARTESIAN_POINT('Ctrl Pts',(10.1252561029999,15.2,5.38716754199999));
#202039=CARTESIAN_POINT('Ctrl Pts',(10.1252561029999,11.6,5.38716754199999));
#202040=CARTESIAN_POINT('Ctrl Pts',(10.1274963839999,15.2,5.39021889299999));
#202041=CARTESIAN_POINT('Ctrl Pts',(10.1274963839999,11.6,5.39021889299999));
#202042=CARTESIAN_POINT('Ctrl Pts',(10.1297369509999,15.2,5.39327551299999));
#202043=CARTESIAN_POINT('Ctrl Pts',(10.1297369509999,11.6,5.39327551299999));
#202044=CARTESIAN_POINT('Ctrl Pts',(10.1319777959999,15.2,5.39633739999999));
#202045=CARTESIAN_POINT('Ctrl Pts',(10.1319777959999,11.6,5.39633739999999));
#202046=CARTESIAN_POINT('Ctrl Pts',(10.1342189099999,15.2,5.39940455199999));
#202047=CARTESIAN_POINT('Ctrl Pts',(10.1342189099999,11.6,5.39940455199999));
#202048=CARTESIAN_POINT('Ctrl Pts',(10.1364602879999,15.2,5.40247696699999));
#202049=CARTESIAN_POINT('Ctrl Pts',(10.1364602879999,11.6,5.40247696699999));
#202050=CARTESIAN_POINT('Ctrl Pts',(10.1387019259999,15.2,5.40555464399999));
#202051=CARTESIAN_POINT('Ctrl Pts',(10.1387019259999,11.6,5.40555464399999));
#202052=CARTESIAN_POINT('Ctrl Pts',(10.1409438219999,15.2,5.40863758099999));
#202053=CARTESIAN_POINT('Ctrl Pts',(10.1409438219999,11.6,5.40863758099999));
#202054=CARTESIAN_POINT('Ctrl Pts',(10.1427375439999,15.2,5.41110813999998));
#202055=CARTESIAN_POINT('Ctrl Pts',(10.1427375439999,11.6,5.41110813999998));
#202056=CARTESIAN_POINT('Ctrl Pts',(10.1440829499999,15.2,5.41296342599999));
#202057=CARTESIAN_POINT('Ctrl Pts',(10.1440829499999,11.6,5.41296342599999));
#202058=CARTESIAN_POINT('Ctrl Pts',(10.1449799389999,15.2,5.41420133599999));
#202059=CARTESIAN_POINT('Ctrl Pts',(10.1449799389999,11.6,5.41420133599999));
#202060=CARTESIAN_POINT('Ctrl Pts',(10.1454284469999,15.2,5.41482055299999));
#202061=CARTESIAN_POINT('Ctrl Pts',(10.1454284469999,11.6,5.41482055299999));
#202062=CARTESIAN_POINT('Ctrl Pts',(9.31239140099994,15.2,4.57383771099998));
#202063=CARTESIAN_POINT('Ctrl Pts',(9.31392144680189,15.2,4.57476026769956));
#202064=CARTESIAN_POINT('Ctrl Pts',(9.31549767341897,15.2,4.57571692949402));
#202065=CARTESIAN_POINT('Ctrl Pts',(9.31711891381397,15.2,4.57670776739141));
#202066=CARTESIAN_POINT('Ctrl Pts',(9.31874797264965,15.2,4.57770338360999));
#202067=CARTESIAN_POINT('Ctrl Pts',(9.32042248385082,15.2,4.57873349868146));
#202068=CARTESIAN_POINT('Ctrl Pts',(9.32214129986625,15.2,4.57979816304467));
#202069=CARTESIAN_POINT('Ctrl Pts',(9.3241465849834,15.2,4.58104027132335));
#202070=CARTESIAN_POINT('Ctrl Pts',(9.32621217660936,15.2,4.58232940557774));
#202071=CARTESIAN_POINT('Ctrl Pts',(9.32833631004309,15.2,4.58366563461676));
#202072=CARTESIAN_POINT('Ctrl Pts',(9.33015699605605,15.2,4.58481097392682));
#202073=CARTESIAN_POINT('Ctrl Pts',(9.33202069553284,15.2,4.58599091516364));
#202074=CARTESIAN_POINT('Ctrl Pts',(9.33392633190099,15.2,4.58720549637584));
#202075=CARTESIAN_POINT('Ctrl Pts',(9.33614957407085,15.2,4.58862250762459));
#202076=CARTESIAN_POINT('Ctrl Pts',(9.33842989701372,15.2,4.59008667009452));
#202077=CARTESIAN_POINT('Ctrl Pts',(9.34076564432333,15.2,4.59159803785873));
#202078=CARTESIAN_POINT('Ctrl Pts',(9.34276771367966,15.2,4.59289349609363));
#202079=CARTESIAN_POINT('Ctrl Pts',(9.34481050330659,15.2,4.59422363630412));
#202080=CARTESIAN_POINT('Ctrl Pts',(9.3468930019431,15.2,4.59558849061538));
#202081=CARTESIAN_POINT('Ctrl Pts',(9.34932258340195,15.2,4.59718082045921));
#202082=CARTESIAN_POINT('Ctrl Pts',(9.35180621226842,15.2,4.59882039919461));
#202083=CARTESIAN_POINT('Ctrl Pts',(9.35434232328794,15.2,4.600507268809));
#202084=CARTESIAN_POINT('Ctrl Pts',(9.35651613298711,15.2,4.60195315721876));
#202085=CARTESIAN_POINT('Ctrl Pts',(9.35872850338876,15.2,4.6034337928863));
#202086=CARTESIAN_POINT('Ctrl Pts',(9.3609784792093,15.2,4.60494919521327));
#202087=CARTESIAN_POINT('Ctrl Pts',(9.36360345069336,15.2,4.60671716438827));
#202088=CARTESIAN_POINT('Ctrl Pts',(9.36627960436232,15.2,4.60853245688356));
#202089=CARTESIAN_POINT('Ctrl Pts',(9.36900546349522,15.2,4.61039510533424));
#202090=CARTESIAN_POINT('Ctrl Pts',(9.37134191445341,15.2,4.61199166133557));
#202091=CARTESIAN_POINT('Ctrl Pts',(9.37371488616263,15.2,4.61362300806846));
#202092=CARTESIAN_POINT('Ctrl Pts',(9.37612347224964,15.2,4.61528916141119));
#202093=CARTESIAN_POINT('Ctrl Pts',(9.37853205811786,15.2,4.61695531460258));
#202094=CARTESIAN_POINT('Ctrl Pts',(9.38097625855661,15.2,4.61865627504632));
#202095=CARTESIAN_POINT('Ctrl Pts',(9.38345519046654,15.2,4.62039205498325));
#202096=CARTESIAN_POINT('Ctrl Pts',(9.38593412237647,15.2,4.62212783492018));
#202097=CARTESIAN_POINT('Ctrl Pts',(9.38844778575411,15.2,4.62389843460277));
#202098=CARTESIAN_POINT('Ctrl Pts',(9.39099531978686,15.2,4.62570386362536));
#202099=CARTESIAN_POINT('Ctrl Pts',(9.39354285405101,15.2,4.62750929281193));
#202100=CARTESIAN_POINT('Ctrl Pts',(9.39612425591511,15.2,4.62934954974141));
#202101=CARTESIAN_POINT('Ctrl Pts',(9.39873868897653,15.2,4.63122464292932));
#202102=CARTESIAN_POINT('Ctrl Pts',(9.40135312180048,15.2,4.63309973594691));
#202103=CARTESIAN_POINT('Ctrl Pts',(9.40400058107225,15.2,4.63500966558724));
#202104=CARTESIAN_POINT('Ctrl Pts',(9.40668024822489,15.2,4.63695443351659));
#202105=CARTESIAN_POINT('Ctrl Pts',(9.4098065267319,15.2,4.63922332955191));
#202106=CARTESIAN_POINT('Ctrl Pts',(9.41297664099816,15.2,4.6415396452332));
#202107=CARTESIAN_POINT('Ctrl Pts',(9.41618931726636,15.2,4.64390338215434));
#202108=CARTESIAN_POINT('Ctrl Pts',(9.41894303963903,15.2,4.6459294422673));
#202109=CARTESIAN_POINT('Ctrl Pts',(9.42172803225219,15.2,4.6479903423594));
#202110=CARTESIAN_POINT('Ctrl Pts',(9.42454351448322,15.2,4.65008607928325));
#202111=CARTESIAN_POINT('Ctrl Pts',(9.42735899671425,15.2,4.65218181620711));
#202112=CARTESIAN_POINT('Ctrl Pts',(9.43020496568432,15.2,4.65431239024637));
#202113=CARTESIAN_POINT('Ctrl Pts',(9.43308065822178,15.2,4.65647779627387));
#202114=CARTESIAN_POINT('Ctrl Pts',(9.43595635102045,15.2,4.65864320249805));
#202115=CARTESIAN_POINT('Ctrl Pts',(9.43886176683284,15.2,4.6608434404277));
#202116=CARTESIAN_POINT('Ctrl Pts',(9.44179615657809,15.2,4.66307850346856));
#202117=CARTESIAN_POINT('Ctrl Pts',(9.44473054605679,15.2,4.6653135663064));
#202118=CARTESIAN_POINT('Ctrl Pts',(9.44769390903798,15.2,4.66758345288251));
#202119=CARTESIAN_POINT('Ctrl Pts',(9.45068551352626,15.2,4.66988815372597));
#202120=CARTESIAN_POINT('Ctrl Pts',(9.45367711801453,15.2,4.67219285456944));
#202121=CARTESIAN_POINT('Ctrl Pts',(9.45669696187919,15.2,4.67453236995845));
#202122=CARTESIAN_POINT('Ctrl Pts',(9.4597443296006,15.2,4.67690668587067));
#202123=CARTESIAN_POINT('Ctrl Pts',(9.46279169759881,15.2,4.67928100199854));
#202124=CARTESIAN_POINT('Ctrl Pts',(9.46586658883378,15.2,4.68169012056408));
#202125=CARTESIAN_POINT('Ctrl Pts',(9.46896829983799,15.2,4.68413402553298));
#202126=CARTESIAN_POINT('Ctrl Pts',(9.47207001056045,15.2,4.68657793027989));
#202127=CARTESIAN_POINT('Ctrl Pts',(9.47519854057708,15.2,4.68905661983519));
#202128=CARTESIAN_POINT('Ctrl Pts',(9.47835320238027,15.2,4.69157007966205));
#202129=CARTESIAN_POINT('Ctrl Pts',(9.48098208731177,15.2,4.69366462959387));
#202130=CARTESIAN_POINT('Ctrl Pts',(9.48362911829559,15.2,4.69578332435561));
#202131=CARTESIAN_POINT('Ctrl Pts',(9.48629390565762,15.2,4.69792615414854));
#202132=CARTESIAN_POINT('Ctrl Pts',(9.48895869301966,15.2,4.70006898394147));
#202133=CARTESIAN_POINT('Ctrl Pts',(9.49164123368286,15.2,4.70223594668768));
#202134=CARTESIAN_POINT('Ctrl Pts',(9.49434114701338,15.2,4.70442703172936));
#202135=CARTESIAN_POINT('Ctrl Pts',(9.49758104289229,15.2,4.70705633368384));
#202136=CARTESIAN_POINT('Ctrl Pts',(9.50084595104441,15.2,4.70972037065632));
#202137=CARTESIAN_POINT('Ctrl Pts',(9.50413521800823,15.2,4.71241912047492));
#202138=CARTESIAN_POINT('Ctrl Pts',(9.506876273911,15.2,4.7146680787388));
#202139=CARTESIAN_POINT('Ctrl Pts',(9.50963424740545,15.2,4.71694114255181));
#202140=CARTESIAN_POINT('Ctrl Pts',(9.51240876575141,15.2,4.71923829749285));
#202141=CARTESIAN_POINT('Ctrl Pts',(9.51518328409738,15.2,4.72153545243388));
#202142=CARTESIAN_POINT('Ctrl Pts',(9.51797434704942,15.2,4.72385669998554));
#202143=CARTESIAN_POINT('Ctrl Pts',(9.52078159038359,15.2,4.72620202165345));
#202144=CARTESIAN_POINT('Ctrl Pts',(9.52358883371776,15.2,4.72854734332137));
#202145=CARTESIAN_POINT('Ctrl Pts',(9.5264122556293,15.2,4.73091674199979));
#202146=CARTESIAN_POINT('Ctrl Pts',(9.52925149743569,15.2,4.73331019943161));
#202147=CARTESIAN_POINT('Ctrl Pts',(9.5320907392421,15.2,4.73570365686343));
#202148=CARTESIAN_POINT('Ctrl Pts',(9.53494579974981,15.2,4.73812117432644));
#202149=CARTESIAN_POINT('Ctrl Pts',(9.53781632732485,15.2,4.74056273278344));
#202150=CARTESIAN_POINT('Ctrl Pts',(9.5406868548999,15.2,4.74300429124043));
#202151=CARTESIAN_POINT('Ctrl Pts',(9.54357284558923,15.2,4.74546989248472));
#202152=CARTESIAN_POINT('Ctrl Pts',(9.54647395260438,15.2,4.74795951804224));
#202153=CARTESIAN_POINT('Ctrl Pts',(9.54937505961951,15.2,4.75044914359977));
#202154=CARTESIAN_POINT('Ctrl Pts',(9.55229128383209,15.2,4.75296279255213));
#202155=CARTESIAN_POINT('Ctrl Pts',(9.55522227987495,15.2,4.75550044658186));
#202156=CARTESIAN_POINT('Ctrl Pts',(9.55815327559833,15.2,4.75803810033498));
#202157=CARTESIAN_POINT('Ctrl Pts',(9.56109904322545,15.2,4.76059975867886));
#202158=CARTESIAN_POINT('Ctrl Pts',(9.56405924484605,15.2,4.76318540089507));
#202159=CARTESIAN_POINT('Ctrl Pts',(9.56701944678933,15.2,4.76577104339312));
#202160=CARTESIAN_POINT('Ctrl Pts',(9.56999408210459,15.2,4.76838067212409));
#202161=CARTESIAN_POINT('Ctrl Pts',(9.57298281661732,15.2,4.77101426441379));
#202162=CARTESIAN_POINT('Ctrl Pts',(9.57597155113005,15.2,4.77364785670349));
#202163=CARTESIAN_POINT('Ctrl Pts',(9.57897438605647,15.2,4.77630541258449));
#202164=CARTESIAN_POINT('Ctrl Pts',(9.58199099209701,15.2,4.77898691070753));
#202165=CARTESIAN_POINT('Ctrl Pts',(9.58500759813753,15.2,4.78166840883055));
#202166=CARTESIAN_POINT('Ctrl Pts',(9.58803797611216,15.2,4.78437384907626));
#202167=CARTESIAN_POINT('Ctrl Pts',(9.59108179917995,15.2,4.78710320914151));
#202168=CARTESIAN_POINT('Ctrl Pts',(9.59412562224773,15.2,4.78983256920675));
#202169=CARTESIAN_POINT('Ctrl Pts',(9.59718289246654,15.2,4.79258584833636));
#202170=CARTESIAN_POINT('Ctrl Pts',(9.60025328954919,15.2,4.79536302479344));
#202171=CARTESIAN_POINT('Ctrl Pts',(9.60332368663183,15.2,4.79814020125053));
#202172=CARTESIAN_POINT('Ctrl Pts',(9.60640721154263,15.2,4.8009412744277));
#202173=CARTESIAN_POINT('Ctrl Pts',(9.60950354855582,15.2,4.80376621852365));
#202174=CARTESIAN_POINT('Ctrl Pts',(9.61198061830137,15.2,4.80602617392358));
#202175=CARTESIAN_POINT('Ctrl Pts',(9.61446588720061,15.2,4.80830140828345));
#202176=CARTESIAN_POINT('Ctrl Pts',(9.61695919712842,15.2,4.81059190835738));
#202177=CARTESIAN_POINT('Ctrl Pts',(9.62007583436833,15.2,4.81345503329373));
#202178=CARTESIAN_POINT('Ctrl Pts',(9.62320503513204,15.2,4.81634201014538));
#202179=CARTESIAN_POINT('Ctrl Pts',(9.62634649145248,15.2,4.81925281410566));
#202180=CARTESIAN_POINT('Ctrl Pts',(9.62885965630339,15.2,4.82158145708352));
#202181=CARTESIAN_POINT('Ctrl Pts',(9.6313806654227,15.2,4.82392534914551));
#202182=CARTESIAN_POINT('Ctrl Pts',(9.6339093623266,15.2,4.82628447684054));
#202183=CARTESIAN_POINT('Ctrl Pts',(9.63707023371486,15.2,4.82923338670041));
#202184=CARTESIAN_POINT('Ctrl Pts',(9.64024311945042,15.2,4.8322061040292));
#202185=CARTESIAN_POINT('Ctrl Pts',(9.64342771675651,15.2,4.83520259897329));
#202186=CARTESIAN_POINT('Ctrl Pts',(9.64597539474023,15.2,4.83759979505921));
#202187=CARTESIAN_POINT('Ctrl Pts',(9.64853057095349,15.2,4.84001220998522));
#202188=CARTESIAN_POINT('Ctrl Pts',(9.65109309092722,15.2,4.84243982989685));
#202189=CARTESIAN_POINT('Ctrl Pts',(9.65429624071982,15.2,4.845474354621));
#202190=CARTESIAN_POINT('Ctrl Pts',(9.65751086726542,15.2,4.8485326364567));
#202191=CARTESIAN_POINT('Ctrl Pts',(9.66073667698853,15.2,4.85161464715307));
#202192=CARTESIAN_POINT('Ctrl Pts',(9.66396248636002,15.2,4.85469665751349));
#202193=CARTESIAN_POINT('Ctrl Pts',(9.66719948033001,15.2,4.85780239751699));
#202194=CARTESIAN_POINT('Ctrl Pts',(9.6704473681001,15.2,4.86093183779893));
#202195=CARTESIAN_POINT('Ctrl Pts',(9.67304567874099,15.2,4.86343539043382));
#202196=CARTESIAN_POINT('Ctrl Pts',(9.6756509615242,15.2,4.86595411075348));
#202197=CARTESIAN_POINT('Ctrl Pts',(9.67826307199992,15.2,4.86848798472493));
#202198=CARTESIAN_POINT('Ctrl Pts',(9.68087518247563,15.2,4.87102185869638));
#202199=CARTESIAN_POINT('Ctrl Pts',(9.68349411904933,15.2,4.87357088501956));
#202200=CARTESIAN_POINT('Ctrl Pts',(9.68611973713754,15.2,4.87613504966084));
#202201=CARTESIAN_POINT('Ctrl Pts',(9.68874535486801,15.2,4.87869921395275));
#202202=CARTESIAN_POINT('Ctrl Pts',(9.69137765619632,15.2,4.88127851639296));
#202203=CARTESIAN_POINT('Ctrl Pts',(9.69401649521479,15.2,4.88387294074816));
#202204=CARTESIAN_POINT('Ctrl Pts',(9.69665533459279,15.2,4.88646736545686));
#202205=CARTESIAN_POINT('Ctrl Pts',(9.69930071187999,15.2,4.88907691186781));
#202206=CARTESIAN_POINT('Ctrl Pts',(9.70195248719182,15.2,4.89170156567906));
#202207=CARTESIAN_POINT('Ctrl Pts',(9.70460426214236,15.2,4.89432621913271));
#202208=CARTESIAN_POINT('Ctrl Pts',(9.70726243417816,15.2,4.89696597790938));
#202209=CARTESIAN_POINT('Ctrl Pts',(9.70992686251549,15.2,4.8996208275247));
#202210=CARTESIAN_POINT('Ctrl Pts',(9.71325739820943,15.2,4.90293938981514));
#202211=CARTESIAN_POINT('Ctrl Pts',(9.71659771088846,15.2,4.90628153051064));
#202212=CARTESIAN_POINT('Ctrl Pts',(9.71994752826477,15.2,4.9096472177481));
#202213=CARTESIAN_POINT('Ctrl Pts',(9.72262738231187,15.2,4.91233976768481));
#202214=CARTESIAN_POINT('Ctrl Pts',(9.72531332028995,15.2,4.91504738687294));
#202215=CARTESIAN_POINT('Ctrl Pts',(9.72800520371505,15.2,4.91777005891176));
#202216=CARTESIAN_POINT('Ctrl Pts',(9.73137005781304,15.2,4.92117339877481));
#202217=CARTESIAN_POINT('Ctrl Pts',(9.73474420341393,15.2,4.92460025986044));
#202218=CARTESIAN_POINT('Ctrl Pts',(9.73812737494245,15.2,4.92805060791791));
#202219=CARTESIAN_POINT('Ctrl Pts',(9.74218718062915,15.2,4.93219102543644));
#202220=CARTESIAN_POINT('Ctrl Pts',(9.74625998326219,15.2,4.93636526424749));
#202221=CARTESIAN_POINT('Ctrl Pts',(9.75034533119763,15.2,4.94057326576273));
#202222=CARTESIAN_POINT('Ctrl Pts',(9.75306889636423,15.2,4.94337859997882));
#202223=CARTESIAN_POINT('Ctrl Pts',(9.75579803803804,15.2,4.94619893955857));
#202224=CARTESIAN_POINT('Ctrl Pts',(9.75853262303615,15.2,4.94903426776969));
#202225=CARTESIAN_POINT('Ctrl Pts',(9.76126720840685,15.2,4.95186959636712));
#202226=CARTESIAN_POINT('Ctrl Pts',(9.76400723839524,15.2,4.95471991376043));
#202227=CARTESIAN_POINT('Ctrl Pts',(9.76675258000179,15.2,4.95758520048521));
#202228=CARTESIAN_POINT('Ctrl Pts',(9.77018425682296,15.2,4.961166808696));
#202229=CARTESIAN_POINT('Ctrl Pts',(9.77362423554171,15.2,4.96477180800835));
#202230=CARTESIAN_POINT('Ctrl Pts',(9.7770722622088,15.2,4.96840016349569));
#202231=CARTESIAN_POINT('Ctrl Pts',(9.78120989405898,15.2,4.9727541899223));
#202232=CARTESIAN_POINT('Ctrl Pts',(9.7853591148332,15.2,4.97714184755452));
#202233=CARTESIAN_POINT('Ctrl Pts',(9.7895194927649,15.2,4.98156307605911));
#202234=CARTESIAN_POINT('Ctrl Pts',(9.79229307830464,15.2,4.98451056199657));
#202235=CARTESIAN_POINT('Ctrl Pts',(9.79507162314495,15.2,4.98747296791077));
#202236=CARTESIAN_POINT('Ctrl Pts',(9.79785500068584,15.2,4.99045027401846));
#202237=CARTESIAN_POINT('Ctrl Pts',(9.80063837784751,15.2,4.99342757972049));
#202238=CARTESIAN_POINT('Ctrl Pts',(9.80342658838388,15.2,4.99641978802167));
#202239=CARTESIAN_POINT('Ctrl Pts',(9.80621950562802,15.2,4.99942687781366));
#202240=CARTESIAN_POINT('Ctrl Pts',(9.80901242325269,15.2,5.00243396801537));
#202241=CARTESIAN_POINT('Ctrl Pts',(9.81181004814268,15.2,5.00545594064017));
#202242=CARTESIAN_POINT('Ctrl Pts',(9.81461225696239,15.2,5.00849277597333));
#202243=CARTESIAN_POINT('Ctrl Pts',(9.81811501779612,15.2,5.0122888199329));
#202244=CARTESIAN_POINT('Ctrl Pts',(9.82162493830183,15.2,5.0161080877446));
#202245=CARTESIAN_POINT('Ctrl Pts',(9.82514178170497,15.2,5.0199505422597));
#202246=CARTESIAN_POINT('Ctrl Pts',(9.82795525619748,15.2,5.02302450562049));
#202247=CARTESIAN_POINT('Ctrl Pts',(9.83077316071664,15.2,5.02611330600517));
#202248=CARTESIAN_POINT('Ctrl Pts',(9.83359537334877,15.2,5.02921692701632));
#202249=CARTESIAN_POINT('Ctrl Pts',(9.83641758636542,15.2,5.03232054845034));
#202250=CARTESIAN_POINT('Ctrl Pts',(9.83924410719627,15.2,5.03543898857892));
#202251=CARTESIAN_POINT('Ctrl Pts',(9.84207481673971,15.2,5.03857222797288));
#202252=CARTESIAN_POINT('Ctrl Pts',(9.8463208806692,15.2,5.04327208663693));
#202253=CARTESIAN_POINT('Ctrl Pts',(9.85057636513958,15.2,5.04800524459828));
#202254=CARTESIAN_POINT('Ctrl Pts',(9.85484087198422,15.2,5.05277163225696));
#202255=CARTESIAN_POINT('Ctrl Pts',(9.8583946278172,15.2,5.05674362211684));
#202256=CARTESIAN_POINT('Ctrl Pts',(9.86195464797069,15.2,5.06073868942956));
#202257=CARTESIAN_POINT('Ctrl Pts',(9.86552070222298,15.2,5.06475679403107));
#202258=CARTESIAN_POINT('Ctrl Pts',(9.86837354578029,15.2,5.06797127788747));
#202259=CARTESIAN_POINT('Ctrl Pts',(9.87123025165023,15.2,5.07120050477702));
#202260=CARTESIAN_POINT('Ctrl Pts',(9.87409070325095,15.2,5.07444445478866));
#202261=CARTESIAN_POINT('Ctrl Pts',(9.87695115446193,15.2,5.07768840435831));
#202262=CARTESIAN_POINT('Ctrl Pts',(9.87981535064186,15.2,5.08094707681769));
#202263=CARTESIAN_POINT('Ctrl Pts',(9.88268317724052,15.2,5.0842204522158));
#202264=CARTESIAN_POINT('Ctrl Pts',(9.88555100422991,15.2,5.08749382805992));
#202265=CARTESIAN_POINT('Ctrl Pts',(9.88842246157484,15.2,5.09078190533578));
#202266=CARTESIAN_POINT('Ctrl Pts',(9.8912974347088,15.2,5.0940846647376));
#202267=CARTESIAN_POINT('Ctrl Pts',(9.89417240745102,15.2,5.09738742368943));
#202268=CARTESIAN_POINT('Ctrl Pts',(9.89705089599465,15.2,5.10070486265938));
#202269=CARTESIAN_POINT('Ctrl Pts',(9.89993278598103,15.2,5.10403696221933));
#202270=CARTESIAN_POINT('Ctrl Pts',(9.90425562154958,15.2,5.10903511224024));
#202271=CARTESIAN_POINT('Ctrl Pts',(9.90858611391919,15.2,5.11406624694868));
#202272=CARTESIAN_POINT('Ctrl Pts',(9.91292388048942,15.2,5.11913029581025));
#202273=CARTESIAN_POINT('Ctrl Pts',(9.91509276357754,15.2,5.12166232001104));
#202274=CARTESIAN_POINT('Ctrl Pts',(9.91726346590713,15.2,5.12420257192406));
#202275=CARTESIAN_POINT('Ctrl Pts',(9.91943593968694,15.2,5.12675104325142));
#202276=CARTESIAN_POINT('Ctrl Pts',(9.92160841346676,15.2,5.12929951457876));
#202277=CARTESIAN_POINT('Ctrl Pts',(9.92378266033273,15.2,5.13185620382213));
#202278=CARTESIAN_POINT('Ctrl Pts',(9.92595863196215,15.2,5.13442110397965));
#202279=CARTESIAN_POINT('Ctrl Pts',(9.92813460359157,15.2,5.13698600413717));
#202280=CARTESIAN_POINT('Ctrl Pts',(9.93031230121245,15.2,5.13955911407704));
#202281=CARTESIAN_POINT('Ctrl Pts',(9.93249167775827,15.2,5.14214042431659));
#202282=CARTESIAN_POINT('Ctrl Pts',(9.93467105430408,15.2,5.14472173455614));
#202283=CARTESIAN_POINT('Ctrl Pts',(9.93685210942485,15.2,5.1473112456787));
#202284=CARTESIAN_POINT('Ctrl Pts',(9.93903479801204,15.2,5.14990894795858));
#202285=CARTESIAN_POINT('Ctrl Pts',(9.94121748659924,15.2,5.15250665023845));
#202286=CARTESIAN_POINT('Ctrl Pts',(9.94340180833077,15.2,5.15511254434293));
#202287=CARTESIAN_POINT('Ctrl Pts',(9.94558771752703,15.2,5.15772661979425));
#202288=CARTESIAN_POINT('Ctrl Pts',(9.94777362672328,15.2,5.16034069524556));
#202289=CARTESIAN_POINT('Ctrl Pts',(9.94996112375248,15.2,5.16296295360654));
#202290=CARTESIAN_POINT('Ctrl Pts',(9.95215016229772,15.2,5.1655933834265));
#202291=CARTESIAN_POINT('Ctrl Pts',(9.95433920124064,15.2,5.16822381372433));
#202292=CARTESIAN_POINT('Ctrl Pts',(9.9565297817257,15.2,5.17086241685783));
#202293=CARTESIAN_POINT('Ctrl Pts',(9.95872185875282,15.2,5.17350918307693));
#202294=CARTESIAN_POINT('Ctrl Pts',(9.96237531993369,15.2,5.17792045946768));
#202295=CARTESIAN_POINT('Ctrl Pts',(9.96603293980633,15.2,5.18235441119767));
#202296=CARTESIAN_POINT('Ctrl Pts',(9.9696945084872,15.2,5.18681099411619));
#202297=CARTESIAN_POINT('Ctrl Pts',(9.97189144961591,15.2,5.18948494377015));
#202298=CARTESIAN_POINT('Ctrl Pts',(9.97408981369542,15.2,5.19216703924958));
#202299=CARTESIAN_POINT('Ctrl Pts',(9.97628955493388,15.2,5.1948572739955));
#202300=CARTESIAN_POINT('Ctrl Pts',(9.97848929617234,15.2,5.19754750874142));
#202301=CARTESIAN_POINT('Ctrl Pts',(9.98069041481994,15.2,5.20024588035938));
#202302=CARTESIAN_POINT('Ctrl Pts',(9.98289286649003,15.2,5.20295237959508));
#202303=CARTESIAN_POINT('Ctrl Pts',(9.98509531816012,15.2,5.20565887883078));
#202304=CARTESIAN_POINT('Ctrl Pts',(9.98729910386338,15.2,5.20837350606551));
#202305=CARTESIAN_POINT('Ctrl Pts',(9.98950417899161,15.2,5.21109625221659));
#202306=CARTESIAN_POINT('Ctrl Pts',(9.99170925411983,15.2,5.21381899836768));
#202307=CARTESIAN_POINT('Ctrl Pts',(9.99391561913965,15.2,5.21654986178508));
#202308=CARTESIAN_POINT('Ctrl Pts',(9.99612322926766,15.2,5.21928883397652));
#202309=CARTESIAN_POINT('Ctrl Pts',(9.99833083939567,15.2,5.22202780616795));
#202310=CARTESIAN_POINT('Ctrl Pts',(10.0005396956591,15.2,5.22477488629702));
#202311=CARTESIAN_POINT('Ctrl Pts',(10.0027497543974,15.2,5.22753006566695));
#202312=CARTESIAN_POINT('Ctrl Pts',(10.0049598131356,15.2,5.23028524503687));
#202313=CARTESIAN_POINT('Ctrl Pts',(10.0071710738982,15.2,5.2330485228809));
#202314=CARTESIAN_POINT('Ctrl Pts',(10.0093834949843,15.2,5.23581988907078));
#202315=CARTESIAN_POINT('Ctrl Pts',(10.0115959164723,15.2,5.23859125576412));
#202316=CARTESIAN_POINT('Ctrl Pts',(10.0138094967274,15.2,5.24137071126807));
#202317=CARTESIAN_POINT('Ctrl Pts',(10.0160241937161,15.2,5.24415824588262));
#202318=CARTESIAN_POINT('Ctrl Pts',(10.0182388903024,15.2,5.24694577999077));
#202319=CARTESIAN_POINT('Ctrl Pts',(10.0204547034721,15.2,5.24974139239017));
#202320=CARTESIAN_POINT('Ctrl Pts',(10.0226715910166,15.2,5.25254507362233));
#202321=CARTESIAN_POINT('Ctrl Pts',(10.0256274409417,15.2,5.25628331509543));
#202322=CARTESIAN_POINT('Ctrl Pts',(10.0285851979359,15.2,5.26003590037957));
#202323=CARTESIAN_POINT('Ctrl Pts',(10.0315447652494,15.2,5.26380280712571));
#202324=CARTESIAN_POINT('Ctrl Pts',(10.0337644412385,15.2,5.26662798782687));
#202325=CARTESIAN_POINT('Ctrl Pts',(10.0359851345113,15.2,5.26946122432197));
#202326=CARTESIAN_POINT('Ctrl Pts',(10.0382068040009,15.2,5.272302505611));
#202327=CARTESIAN_POINT('Ctrl Pts',(10.040428473087,15.2,5.27514378638386));
#202328=CARTESIAN_POINT('Ctrl Pts',(10.0426511173831,15.2,5.27799311286298));
#202329=CARTESIAN_POINT('Ctrl Pts',(10.0448746951635,15.2,5.28085047423617));
#202330=CARTESIAN_POINT('Ctrl Pts',(10.0470982729439,15.2,5.28370783560936));
#202331=CARTESIAN_POINT('Ctrl Pts',(10.04932278484,15.2,5.28657323213364));
#202332=CARTESIAN_POINT('Ctrl Pts',(10.0515481885509,15.2,5.2894466538216));
#202333=CARTESIAN_POINT('Ctrl Pts',(10.0537735922617,15.2,5.29232007550957));
#202334=CARTESIAN_POINT('Ctrl Pts',(10.0559998889975,15.2,5.29520152223825));
#202335=CARTESIAN_POINT('Ctrl Pts',(10.0582270357499,15.2,5.2980909829666));
#202336=CARTESIAN_POINT('Ctrl Pts',(10.0604541825023,15.2,5.30098044369494));
#202337=CARTESIAN_POINT('Ctrl Pts',(10.0626821808214,15.2,5.30387791960631));
#202338=CARTESIAN_POINT('Ctrl Pts',(10.064910988532,15.2,5.30678340025003));
#202339=CARTESIAN_POINT('Ctrl Pts',(10.0678827324161,15.2,5.31065737479357));
#202340=CARTESIAN_POINT('Ctrl Pts',(10.0708559163318,15.2,5.31454557819352));
#202341=CARTESIAN_POINT('Ctrl Pts',(10.0738304441982,15.2,5.31844798832461));
#202342=CARTESIAN_POINT('Ctrl Pts',(10.0760613398954,15.2,5.32137479565708));
#202343=CARTESIAN_POINT('Ctrl Pts',(10.078292989541,15.2,5.32430959359372));
#202344=CARTESIAN_POINT('Ctrl Pts',(10.08052535471,15.2,5.32725237132083));
#202345=CARTESIAN_POINT('Ctrl Pts',(10.0827577198789,15.2,5.33019514904794));
#202346=CARTESIAN_POINT('Ctrl Pts',(10.0849908002978,15.2,5.33314590707409));
#202347=CARTESIAN_POINT('Ctrl Pts',(10.0872245555083,15.2,5.33610463525826));
#202348=CARTESIAN_POINT('Ctrl Pts',(10.0894583107188,15.2,5.33906336344242));
#202349=CARTESIAN_POINT('Ctrl Pts',(10.0916927415709,15.2,5.34203006118459));
#202350=CARTESIAN_POINT('Ctrl Pts',(10.0939278077397,15.2,5.34500471840916));
#202351=CARTESIAN_POINT('Ctrl Pts',(10.0961628739084,15.2,5.34797937563372));
#202352=CARTESIAN_POINT('Ctrl Pts',(10.0983985755202,15.2,5.35096199276492));
#202353=CARTESIAN_POINT('Ctrl Pts',(10.1006348703423,15.2,5.35395255817974));
#202354=CARTESIAN_POINT('Ctrl Pts',(10.1036165970425,15.2,5.35793997909502));
#202355=CARTESIAN_POINT('Ctrl Pts',(10.1065993780895,15.2,5.36194153056136));
#202356=CARTESIAN_POINT('Ctrl Pts',(10.1095831227522,15.2,5.36595718783667));
#202357=CARTESIAN_POINT('Ctrl Pts',(10.1118209310459,15.2,5.36896893051959));
#202358=CARTESIAN_POINT('Ctrl Pts',(10.1140592831646,15.2,5.3719886079766));
#202359=CARTESIAN_POINT('Ctrl Pts',(10.1162981414999,15.2,5.37501621019993));
#202360=CARTESIAN_POINT('Ctrl Pts',(10.1185369998353,15.2,5.37804381242326));
#202361=CARTESIAN_POINT('Ctrl Pts',(10.1207763667872,15.2,5.3810793403296));
#202362=CARTESIAN_POINT('Ctrl Pts',(10.1230161954141,15.2,5.38412278142666));
#202363=CARTESIAN_POINT('Ctrl Pts',(10.1252560240411,15.2,5.38716622252373));
#202364=CARTESIAN_POINT('Ctrl Pts',(10.127496314736,15.2,5.39021757578404));
#202365=CARTESIAN_POINT('Ctrl Pts',(10.1297370200581,15.2,5.39327682915811));
#202366=CARTESIAN_POINT('Ctrl Pts',(10.1319777253802,15.2,5.39633608253219));
#202367=CARTESIAN_POINT('Ctrl Pts',(10.1342188448594,15.2,5.39940323605904));
#202368=CARTESIAN_POINT('Ctrl Pts',(10.136460352528,15.2,5.40247828182125));
#202369=CARTESIAN_POINT('Ctrl Pts',(10.1394490296908,15.2,5.40657834320993));
#202370=CARTESIAN_POINT('Ctrl Pts',(10.1424383928518,15.2,5.41069243854174));
#202371=CARTESIAN_POINT('Ctrl Pts',(10.1454284469999,15.2,5.41482055299999));
#202372=CARTESIAN_POINT('Ctrl Pts',(9.31239140099994,12.2,4.57383771099998));
#202373=CARTESIAN_POINT('Ctrl Pts',(9.31392144680189,12.2,4.57476026769956));
#202374=CARTESIAN_POINT('Ctrl Pts',(9.31549767341897,12.2,4.57571692949402));
#202375=CARTESIAN_POINT('Ctrl Pts',(9.31711891381397,12.2,4.57670776739141));
#202376=CARTESIAN_POINT('Ctrl Pts',(9.31874797264965,12.2,4.57770338360999));
#202377=CARTESIAN_POINT('Ctrl Pts',(9.32042248385082,12.2,4.57873349868146));
#202378=CARTESIAN_POINT('Ctrl Pts',(9.32214129986625,12.2,4.57979816304467));
#202379=CARTESIAN_POINT('Ctrl Pts',(9.3241465849834,12.2,4.58104027132335));
#202380=CARTESIAN_POINT('Ctrl Pts',(9.32621217660936,12.2,4.58232940557774));
#202381=CARTESIAN_POINT('Ctrl Pts',(9.32833631004309,12.2,4.58366563461676));
#202382=CARTESIAN_POINT('Ctrl Pts',(9.33015699605605,12.2,4.58481097392682));
#202383=CARTESIAN_POINT('Ctrl Pts',(9.33202069553284,12.2,4.58599091516364));
#202384=CARTESIAN_POINT('Ctrl Pts',(9.33392633190098,12.2,4.58720549637584));
#202385=CARTESIAN_POINT('Ctrl Pts',(9.33614957407084,12.2,4.58862250762459));
#202386=CARTESIAN_POINT('Ctrl Pts',(9.33842989701372,12.2,4.59008667009452));
#202387=CARTESIAN_POINT('Ctrl Pts',(9.34076564432333,12.2,4.59159803785873));
#202388=CARTESIAN_POINT('Ctrl Pts',(9.34276771367966,12.2,4.59289349609363));
#202389=CARTESIAN_POINT('Ctrl Pts',(9.34481050330659,12.2,4.59422363630412));
#202390=CARTESIAN_POINT('Ctrl Pts',(9.3468930019431,12.2,4.59558849061538));
#202391=CARTESIAN_POINT('Ctrl Pts',(9.34932258340195,12.2,4.59718082045921));
#202392=CARTESIAN_POINT('Ctrl Pts',(9.35180621226842,12.2,4.59882039919461));
#202393=CARTESIAN_POINT('Ctrl Pts',(9.35434232328794,12.2,4.600507268809));
#202394=CARTESIAN_POINT('Ctrl Pts',(9.35651613298711,12.2,4.60195315721876));
#202395=CARTESIAN_POINT('Ctrl Pts',(9.35872850338876,12.2,4.6034337928863));
#202396=CARTESIAN_POINT('Ctrl Pts',(9.36097847920929,12.2,4.60494919521327));
#202397=CARTESIAN_POINT('Ctrl Pts',(9.36322845482546,12.2,4.6064645974026));
#202398=CARTESIAN_POINT('Ctrl Pts',(9.36551603434266,12.2,4.60801476769917));
#202399=CARTESIAN_POINT('Ctrl Pts',(9.36784028600821,12.2,4.60959972672492));
#202400=CARTESIAN_POINT('Ctrl Pts',(9.37016453767377,12.2,4.61118468575067));
#202401=CARTESIAN_POINT('Ctrl Pts',(9.37252546320421,12.2,4.61280443283609));
#202402=CARTESIAN_POINT('Ctrl Pts',(9.37492215123479,12.2,4.61445898485662));
#202403=CARTESIAN_POINT('Ctrl Pts',(9.37731883948308,12.2,4.61611353702745));
#202404=CARTESIAN_POINT('Ctrl Pts',(9.37975129316532,12.2,4.61780289367487));
#202405=CARTESIAN_POINT('Ctrl Pts',(9.38221862330217,12.2,4.61952706693787));
#202406=CARTESIAN_POINT('Ctrl Pts',(9.38468595321489,12.2,4.62125124004426));
#202407=CARTESIAN_POINT('Ctrl Pts',(9.38718815954827,12.2,4.62301023159936));
#202408=CARTESIAN_POINT('Ctrl Pts',(9.38972437946771,12.2,4.62480405145907));
#202409=CARTESIAN_POINT('Ctrl Pts',(9.39226059938715,12.2,4.62659787131879));
#202410=CARTESIAN_POINT('Ctrl Pts',(9.3948308306375,12.2,4.62842651815939));
#202411=CARTESIAN_POINT('Ctrl Pts',(9.39743422887481,12.2,4.63028999917351));
#202412=CARTESIAN_POINT('Ctrl Pts',(9.4000376273486,12.2,4.63215348035689));
#202413=CARTESIAN_POINT('Ctrl Pts',(9.40267419441815,12.2,4.63405179783625));
#202414=CARTESIAN_POINT('Ctrl Pts',(9.40534310281581,12.2,4.63598495294398));
#202415=CARTESIAN_POINT('Ctrl Pts',(9.40801201097104,12.2,4.63791810787611));
#202416=CARTESIAN_POINT('Ctrl Pts',(9.41071326184628,12.2,4.63988610110609));
#202417=CARTESIAN_POINT('Ctrl Pts',(9.41344604800947,12.2,4.64188893495917));
#202418=CARTESIAN_POINT('Ctrl Pts',(9.41617883417266,12.2,4.64389176881224));
#202419=CARTESIAN_POINT('Ctrl Pts',(9.41894315591726,12.2,4.64592944248062));
#202420=CARTESIAN_POINT('Ctrl Pts',(9.42173822431436,12.2,4.64800195440379));
#202421=CARTESIAN_POINT('Ctrl Pts',(9.42453329296533,12.2,4.65007446651521));
#202422=CARTESIAN_POINT('Ctrl Pts',(9.42735910974518,12.2,4.65218181759766));
#202423=CARTESIAN_POINT('Ctrl Pts',(9.43021490231951,12.2,4.65432400171676));
#202424=CARTESIAN_POINT('Ctrl Pts',(9.43307069463444,12.2,4.65646618564129));
#202425=CARTESIAN_POINT('Ctrl Pts',(9.43595646228017,12.2,4.65864320443279));
#202426=CARTESIAN_POINT('Ctrl Pts',(9.43887145267555,12.2,4.66085504935395));
#202427=CARTESIAN_POINT('Ctrl Pts',(9.44178644307091,12.2,4.6630668942751));
#202428=CARTESIAN_POINT('Ctrl Pts',(9.4447306541389,12.2,4.66531356687679));
#202429=CARTESIAN_POINT('Ctrl Pts',(9.447703349613,12.2,4.66759505762573));
#202430=CARTESIAN_POINT('Ctrl Pts',(9.45067604508711,12.2,4.66987654837468));
#202431=CARTESIAN_POINT('Ctrl Pts',(9.45367722400671,12.2,4.67219285629814));
#202432=CARTESIAN_POINT('Ctrl Pts',(9.45670616264474,12.2,4.67454397021032));
#202433=CARTESIAN_POINT('Ctrl Pts',(9.45973510155791,12.2,4.67689508433607));
#202434=CARTESIAN_POINT('Ctrl Pts',(9.46279180181548,12.2,4.67928100451521));
#202435=CARTESIAN_POINT('Ctrl Pts',(9.46587555465141,12.2,4.68170171664866));
#202436=CARTESIAN_POINT('Ctrl Pts',(9.46895930720722,12.2,4.68412242856224));
#202437=CARTESIAN_POINT('Ctrl Pts',(9.47207011191492,12.2,4.68657793207805));
#202438=CARTESIAN_POINT('Ctrl Pts',(9.47520727648181,12.2,4.6890682099988));
#202439=CARTESIAN_POINT('Ctrl Pts',(9.47782158038254,12.2,4.69114344167482));
#202440=CARTESIAN_POINT('Ctrl Pts',(9.48045418979989,12.2,4.69324282403325));
#202441=CARTESIAN_POINT('Ctrl Pts',(9.48310470896656,12.2,4.69536634403325));
#202442=CARTESIAN_POINT('Ctrl Pts',(9.48575522813323,12.2,4.69748986403325));
#202443=CARTESIAN_POINT('Ctrl Pts',(9.48842366038359,12.2,4.69963752303009));
#202444=CARTESIAN_POINT('Ctrl Pts',(9.49110961449303,12.2,4.70180930873444));
#202445=CARTESIAN_POINT('Ctrl Pts',(9.49379556860247,12.2,4.7039810944388));
#202446=CARTESIAN_POINT('Ctrl Pts',(9.49649904737149,12.2,4.70617700707734));
#202447=CARTESIAN_POINT('Ctrl Pts',(9.49921966813626,12.2,4.70839703291192));
#202448=CARTESIAN_POINT('Ctrl Pts',(9.50194028890104,12.2,4.7106170587465));
#202449=CARTESIAN_POINT('Ctrl Pts',(9.50467805142371,12.2,4.71286120014716));
#202450=CARTESIAN_POINT('Ctrl Pts',(9.50743258218848,12.2,4.71512944014841));
#202451=CARTESIAN_POINT('Ctrl Pts',(9.51018711295324,12.2,4.71739768014967));
#202452=CARTESIAN_POINT('Ctrl Pts',(9.51295841027204,12.2,4.7196900206293));
#202453=CARTESIAN_POINT('Ctrl Pts',(9.51574610631524,12.2,4.72200644651058));
#202454=CARTESIAN_POINT('Ctrl Pts',(9.51853380235842,12.2,4.72432287239186));
#202455=CARTESIAN_POINT('Ctrl Pts',(9.52133789705082,12.2,4.72666338340171));
#202456=CARTESIAN_POINT('Ctrl Pts',(9.52415802559378,12.2,4.72902796333422));
#202457=CARTESIAN_POINT('Ctrl Pts',(9.52697815413675,12.2,4.73139254326673));
#202458=CARTESIAN_POINT('Ctrl Pts',(9.52981431797721,12.2,4.73378119320244));
#202459=CARTESIAN_POINT('Ctrl Pts',(9.53266615888126,12.2,4.73619389556551));
#202460=CARTESIAN_POINT('Ctrl Pts',(9.53551799947446,12.2,4.73860659766559));
#202461=CARTESIAN_POINT('Ctrl Pts',(9.53838551764944,12.2,4.74104335162605));
#202462=CARTESIAN_POINT('Ctrl Pts',(9.54126835934783,12.2,4.74350414191139));
#202463=CARTESIAN_POINT('Ctrl Pts',(9.54415120136044,12.2,4.74596493246496));
#202464=CARTESIAN_POINT('Ctrl Pts',(9.54704936916453,12.2,4.74844975705706));
#202465=CARTESIAN_POINT('Ctrl Pts',(9.54996251513554,12.2,4.75095859788845));
#202466=CARTESIAN_POINT('Ctrl Pts',(9.55287566110655,12.2,4.75346743871982));
#202467=CARTESIAN_POINT('Ctrl Pts',(9.55580378408458,12.2,4.75600029723823));
#202468=CARTESIAN_POINT('Ctrl Pts',(9.55874654367502,12.2,4.75855715146153));
#202469=CARTESIAN_POINT('Ctrl Pts',(9.56168930326545,12.2,4.76111400568482));
#202470=CARTESIAN_POINT('Ctrl Pts',(9.56464669929527,12.2,4.76369485621429));
#202471=CARTESIAN_POINT('Ctrl Pts',(9.56761839457232,12.2,4.76629968433805));
#202472=CARTESIAN_POINT('Ctrl Pts',(9.57059008984936,12.2,4.76890451246181));
#202473=CARTESIAN_POINT('Ctrl Pts',(9.57357608262674,12.2,4.77153331651116));
#202474=CARTESIAN_POINT('Ctrl Pts',(9.5765760460288,12.2,4.77418607630158));
#202475=CARTESIAN_POINT('Ctrl Pts',(9.57957600943086,12.2,4.77683883609201));
#202476=CARTESIAN_POINT('Ctrl Pts',(9.58258993811383,12.2,4.77951555064693));
#202477=CARTESIAN_POINT('Ctrl Pts',(9.58561750929366,12.2,4.78221619884011));
#202478=CARTESIAN_POINT('Ctrl Pts',(9.58864508047348,12.2,4.78491684703329));
#202479=CARTESIAN_POINT('Ctrl Pts',(9.59168629101776,12.2,4.78764142989713));
#202480=CARTESIAN_POINT('Ctrl Pts',(9.59474082123992,12.2,4.79038992150677));
#202481=CARTESIAN_POINT('Ctrl Pts',(9.59779535146208,12.2,4.7931384131164));
#202482=CARTESIAN_POINT('Ctrl Pts',(9.60086319855546,12.2,4.79591081560547));
#202483=CARTESIAN_POINT('Ctrl Pts',(9.60394404799991,12.2,4.79870710546659));
#202484=CARTESIAN_POINT('Ctrl Pts',(9.6064087276898,12.2,4.8009441374774));
#202485=CARTESIAN_POINT('Ctrl Pts',(9.6088817266501,12.2,4.803196455865));
#202486=CARTESIAN_POINT('Ctrl Pts',(9.61136288639726,12.2,4.80546405037902));
#202487=CARTESIAN_POINT('Ctrl Pts',(9.61384404580635,12.2,4.80773164458409));
#202488=CARTESIAN_POINT('Ctrl Pts',(9.61633336409106,12.2,4.81001451331751));
#202489=CARTESIAN_POINT('Ctrl Pts',(9.61883068423155,12.2,4.81231264497336));
#202490=CARTESIAN_POINT('Ctrl Pts',(9.62132800471231,12.2,4.81461077694233));
#202491=CARTESIAN_POINT('Ctrl Pts',(9.62383332625916,12.2,4.81692417081053));
#202492=CARTESIAN_POINT('Ctrl Pts',(9.62634649145248,12.2,4.81925281410566));
#202493=CARTESIAN_POINT('Ctrl Pts',(9.62885965630339,12.2,4.82158145708352));
#202494=CARTESIAN_POINT('Ctrl Pts',(9.63138066542271,12.2,4.82392534914551));
#202495=CARTESIAN_POINT('Ctrl Pts',(9.6339093623266,12.2,4.82628447684054));
#202496=CARTESIAN_POINT('Ctrl Pts',(9.63643805957503,12.2,4.82864360485701));
#202497=CARTESIAN_POINT('Ctrl Pts',(9.63897444597214,12.2,4.83101796992636));
#202498=CARTESIAN_POINT('Ctrl Pts',(9.64151836662743,12.2,4.83340755612175));
#202499=CARTESIAN_POINT('Ctrl Pts',(9.64406228693611,12.2,4.83579714199156));
#202500=CARTESIAN_POINT('Ctrl Pts',(9.6466137416199,12.2,4.83820195003162));
#202501=CARTESIAN_POINT('Ctrl Pts',(9.64917257979913,12.2,4.84062196577723));
#202502=CARTESIAN_POINT('Ctrl Pts',(9.65173141832699,12.2,4.84304198185257));
#202503=CARTESIAN_POINT('Ctrl Pts',(9.6542976392974,12.2,4.8454772070575));
#202504=CARTESIAN_POINT('Ctrl Pts',(9.65687109199369,12.2,4.84792762569205));
#202505=CARTESIAN_POINT('Ctrl Pts',(9.65944454433934,12.2,4.85037804399273));
#202506=CARTESIAN_POINT('Ctrl Pts',(9.66202522872402,12.2,4.85284365623412));
#202507=CARTESIAN_POINT('Ctrl Pts',(9.66461299764112,12.2,4.85532444743169));
#202508=CARTESIAN_POINT('Ctrl Pts',(9.66720076691081,12.2,4.85780523896728));
#202509=CARTESIAN_POINT('Ctrl Pts',(9.66979561875931,12.2,4.86030121114528));
#202510=CARTESIAN_POINT('Ctrl Pts',(9.67239740667934,12.2,4.86281234650535));
#202511=CARTESIAN_POINT('Ctrl Pts',(9.67499919424488,12.2,4.86532348152328));
#202512=CARTESIAN_POINT('Ctrl Pts',(9.67760791813403,12.2,4.86784978165206));
#202513=CARTESIAN_POINT('Ctrl Pts',(9.68022343186395,12.2,4.87039123060941));
#202514=CARTESIAN_POINT('Ctrl Pts',(9.68283894595024,12.2,4.87293267991302));
#202515=CARTESIAN_POINT('Ctrl Pts',(9.68546125037149,12.2,4.87548927810815));
#202516=CARTESIAN_POINT('Ctrl Pts',(9.68809020102671,12.2,4.87806101076002));
#202517=CARTESIAN_POINT('Ctrl Pts',(9.69071915132374,12.2,4.88063274306148));
#202518=CARTESIAN_POINT('Ctrl Pts',(9.69335474852347,12.2,4.8832196092082));
#202519=CARTESIAN_POINT('Ctrl Pts',(9.69599684808461,12.2,4.88582159404951));
#202520=CARTESIAN_POINT('Ctrl Pts',(9.69863894800573,12.2,4.88842357924534));
#202521=CARTESIAN_POINT('Ctrl Pts',(9.70128755018022,12.2,4.89104068216757));
#202522=CARTESIAN_POINT('Ctrl Pts',(9.70394251549158,12.2,4.89367288753326));
#202523=CARTESIAN_POINT('Ctrl Pts',(9.70659748080295,12.2,4.89630509289894));
#202524=CARTESIAN_POINT('Ctrl Pts',(9.70925880700115,12.2,4.89895240071358));
#202525=CARTESIAN_POINT('Ctrl Pts',(9.71192635570274,12.2,4.90161479469357));
#202526=CARTESIAN_POINT('Ctrl Pts',(9.71459390404087,12.2,4.90427718831081));
#202527=CARTESIAN_POINT('Ctrl Pts',(9.7172676745828,12.2,4.90695466817825));
#202528=CARTESIAN_POINT('Ctrl Pts',(9.71994752826477,12.2,4.9096472177481));
#202529=CARTESIAN_POINT('Ctrl Pts',(9.72262738231187,12.2,4.91233976768481));
#202530=CARTESIAN_POINT('Ctrl Pts',(9.72531332028995,12.2,4.91504738687293));
#202531=CARTESIAN_POINT('Ctrl Pts',(9.72800520371505,12.2,4.91777005891176));
#202532=CARTESIAN_POINT('Ctrl Pts',(9.73069708677338,12.2,4.92049273057962));
#202533=CARTESIAN_POINT('Ctrl Pts',(9.7333949161948,12.2,4.9232304562955));
#202534=CARTESIAN_POINT('Ctrl Pts',(9.73609855652896,12.2,4.9259832172917));
#202535=CARTESIAN_POINT('Ctrl Pts',(9.73880219723148,12.2,4.92873597866296));
#202536=CARTESIAN_POINT('Ctrl Pts',(9.7415116475237,12.2,4.93150377594792));
#202537=CARTESIAN_POINT('Ctrl Pts',(9.74422677441894,12.2,4.93428659262881));
#202538=CARTESIAN_POINT('Ctrl Pts',(9.74694190094423,12.2,4.93706940893054));
#202539=CARTESIAN_POINT('Ctrl Pts',(9.74966270290867,12.2,4.93986724359549));
#202540=CARTESIAN_POINT('Ctrl Pts',(9.75238904851876,12.2,4.94268007925345));
#202541=CARTESIAN_POINT('Ctrl Pts',(9.75511539450032,12.2,4.94549291529466));
#202542=CARTESIAN_POINT('Ctrl Pts',(9.75784728239366,12.2,4.94832075338767));
#202543=CARTESIAN_POINT('Ctrl Pts',(9.76058458126542,12.2,4.9511635747658));
#202544=CARTESIAN_POINT('Ctrl Pts',(9.76332187976422,12.2,4.9540063957566));
#202545=CARTESIAN_POINT('Ctrl Pts',(9.76606458996958,12.2,4.95686420118412));
#202546=CARTESIAN_POINT('Ctrl Pts',(9.7688125798262,12.2,4.95973697159148));
#202547=CARTESIAN_POINT('Ctrl Pts',(9.77156057005723,12.2,4.96260974239025));
#202548=CARTESIAN_POINT('Ctrl Pts',(9.7743138407248,12.2,4.96549747894763));
#202549=CARTESIAN_POINT('Ctrl Pts',(9.77707226220881,12.2,4.9684001634957));
#202550=CARTESIAN_POINT('Ctrl Pts',(9.77983068331699,12.2,4.97130284764828));
#202551=CARTESIAN_POINT('Ctrl Pts',(9.7825942550908,12.2,4.97422047889231));
#202552=CARTESIAN_POINT('Ctrl Pts',(9.78536284953059,12.2,4.97715303926212));
#202553=CARTESIAN_POINT('Ctrl Pts',(9.78813144434761,12.2,4.9800856000315));
#202554=CARTESIAN_POINT('Ctrl Pts',(9.79090506156238,12.2,4.98303309077458));
#202555=CARTESIAN_POINT('Ctrl Pts',(9.79368357499159,12.2,4.98599549199159));
#202556=CARTESIAN_POINT('Ctrl Pts',(9.79646208842081,12.2,4.98895789320861));
#202557=CARTESIAN_POINT('Ctrl Pts',(9.79924549754225,12.2,4.99193520367457));
#202558=CARTESIAN_POINT('Ctrl Pts',(9.80203367647246,12.2,4.99492740750583));
#202559=CARTESIAN_POINT('Ctrl Pts',(9.80482185502279,12.2,4.9979196109294));
#202560=CARTESIAN_POINT('Ctrl Pts',(9.80761480294737,12.2,5.00092670553401));
#202561=CARTESIAN_POINT('Ctrl Pts',(9.81041239673136,12.2,5.00394867302287));
#202562=CARTESIAN_POINT('Ctrl Pts',(9.81320999089653,12.2,5.00697064092348));
#202563=CARTESIAN_POINT('Ctrl Pts',(9.81601223113041,12.2,5.01000748081996));
#202564=CARTESIAN_POINT('Ctrl Pts',(9.81881899145051,12.2,5.01305917476556));
#202565=CARTESIAN_POINT('Ctrl Pts',(9.82162575138817,12.2,5.01611086829536));
#202566=CARTESIAN_POINT('Ctrl Pts',(9.82443703421968,12.2,5.01917741568158));
#202567=CARTESIAN_POINT('Ctrl Pts',(9.82725271604479,12.2,5.02225879603983));
#202568=CARTESIAN_POINT('Ctrl Pts',(9.83006839825352,12.2,5.02534017681792));
#202569=CARTESIAN_POINT('Ctrl Pts',(9.83288848028938,12.2,5.02843639250017));
#202570=CARTESIAN_POINT('Ctrl Pts',(9.83571283941812,12.2,5.03154742199311));
#202571=CARTESIAN_POINT('Ctrl Pts',(9.83853719816205,12.2,5.03465845106218));
#202572=CARTESIAN_POINT('Ctrl Pts',(9.84136583625859,12.2,5.03778429366772));
#202573=CARTESIAN_POINT('Ctrl Pts',(9.84419863152672,12.2,5.04092493174332));
#202574=CARTESIAN_POINT('Ctrl Pts',(9.84703142718082,12.2,5.04406557024682));
#202575=CARTESIAN_POINT('Ctrl Pts',(9.84986838127157,12.2,5.04722100170495));
#202576=CARTESIAN_POINT('Ctrl Pts',(9.85270937298221,12.2,5.05039120826756));
#202577=CARTESIAN_POINT('Ctrl Pts',(9.85555036430577,12.2,5.05356141439823));
#202578=CARTESIAN_POINT('Ctrl Pts',(9.85839539613025,12.2,5.05674639548595));
#202579=CARTESIAN_POINT('Ctrl Pts',(9.86124434809488,12.2,5.05994612932737));
#202580=CARTESIAN_POINT('Ctrl Pts',(9.86480553834178,12.2,5.06394579695611));
#202581=CARTESIAN_POINT('Ctrl Pts',(9.86837285282768,12.2,5.06796851859778));
#202582=CARTESIAN_POINT('Ctrl Pts',(9.87194606775794,12.2,5.07201425248547));
#202583=CARTESIAN_POINT('Ctrl Pts',(9.87480463985795,12.2,5.07525083977203));
#202584=CARTESIAN_POINT('Ctrl Pts',(9.87766698508338,12.2,5.07850215551588));
#202585=CARTESIAN_POINT('Ctrl Pts',(9.88053299001759,12.2,5.0817681782504));
#202586=CARTESIAN_POINT('Ctrl Pts',(9.88339899456131,12.2,5.08503420053992));
#202587=CARTESIAN_POINT('Ctrl Pts',(9.88626865709412,12.2,5.08831493056397));
#202588=CARTESIAN_POINT('Ctrl Pts',(9.88914186505803,12.2,5.09161034751349));
#202589=CARTESIAN_POINT('Ctrl Pts',(9.89201507341341,12.2,5.09490576491201));
#202590=CARTESIAN_POINT('Ctrl Pts',(9.89489182613933,12.2,5.09821586841193));
#202591=CARTESIAN_POINT('Ctrl Pts',(9.89777200851875,12.2,5.10154063703853));
#202592=CARTESIAN_POINT('Ctrl Pts',(9.90065219050575,12.2,5.10486540521214));
#202593=CARTESIAN_POINT('Ctrl Pts',(9.90353580293927,12.2,5.10820484003835));
#202594=CARTESIAN_POINT('Ctrl Pts',(9.90642273353625,12.2,5.11155891698487));
#202595=CARTESIAN_POINT('Ctrl Pts',(9.90930966452657,12.2,5.11491299438837));
#202596=CARTESIAN_POINT('Ctrl Pts',(9.91219991338939,12.2,5.11828171706076));
#202597=CARTESIAN_POINT('Ctrl Pts',(9.9150933677269,12.2,5.12166506176056));
#202598=CARTESIAN_POINT('Ctrl Pts',(9.91726345828292,12.2,5.12420257005493));
#202599=CARTESIAN_POINT('Ctrl Pts',(9.91943535168372,12.2,5.1267483039955));
#202600=CARTESIAN_POINT('Ctrl Pts',(9.92160900219796,12.2,5.12930225324761));
#202601=CARTESIAN_POINT('Ctrl Pts',(9.92378265271218,12.2,5.13185620249971));
#202602=CARTESIAN_POINT('Ctrl Pts',(9.92595805972523,12.2,5.13441836779733));
#202603=CARTESIAN_POINT('Ctrl Pts',(9.92813517677099,12.2,5.13698874003657));
#202604=CARTESIAN_POINT('Ctrl Pts',(9.93031229381675,12.2,5.1395591122758));
#202605=CARTESIAN_POINT('Ctrl Pts',(9.93249112118739,12.2,5.14213769084781));
#202606=CARTESIAN_POINT('Ctrl Pts',(9.93467161177458,12.2,5.14472446712768));
#202607=CARTESIAN_POINT('Ctrl Pts',(9.93685210275791,12.2,5.14731124387749));
#202608=CARTESIAN_POINT('Ctrl Pts',(9.9390342573084,12.2,5.14990621860465));
#202609=CARTESIAN_POINT('Ctrl Pts',(9.94121803020934,12.2,5.15250938131743));
#202610=CARTESIAN_POINT('Ctrl Pts',(9.94340180271356,12.2,5.15511254355731));
#202611=CARTESIAN_POINT('Ctrl Pts',(9.94558719255975,12.2,5.15772389382017));
#202612=CARTESIAN_POINT('Ctrl Pts',(9.94777415521473,12.2,5.16034342319014));
#202613=CARTESIAN_POINT('Ctrl Pts',(9.94996111786971,12.2,5.16296295256011));
#202614=CARTESIAN_POINT('Ctrl Pts',(9.95214965260145,12.2,5.16559066078244));
#202615=CARTESIAN_POINT('Ctrl Pts',(9.95433971373034,12.2,5.16822653802071));
#202616=CARTESIAN_POINT('Ctrl Pts',(9.95725979510292,12.2,5.17174104084547));
#202617=CARTESIAN_POINT('Ctrl Pts',(9.96018259014993,12.2,5.17527006748119));
#202618=CARTESIAN_POINT('Ctrl Pts',(9.96310799402163,12.2,5.17881359491223));
#202619=CARTESIAN_POINT('Ctrl Pts',(9.96530204742362,12.2,5.18147124108902));
#202620=CARTESIAN_POINT('Ctrl Pts',(9.96749756695938,12.2,5.18413704397646));
#202621=CARTESIAN_POINT('Ctrl Pts',(9.9696945084872,12.2,5.18681099411619));
#202622=CARTESIAN_POINT('Ctrl Pts',(9.97189144961591,12.2,5.18948494377014));
#202623=CARTESIAN_POINT('Ctrl Pts',(9.97408981369543,12.2,5.19216703924959));
#202624=CARTESIAN_POINT('Ctrl Pts',(9.97628955493388,12.2,5.1948572739955));
#202625=CARTESIAN_POINT('Ctrl Pts',(9.97848929617234,12.2,5.19754750874143));
#202626=CARTESIAN_POINT('Ctrl Pts',(9.98069041481993,12.2,5.20024588035938));
#202627=CARTESIAN_POINT('Ctrl Pts',(9.98289286649003,12.2,5.20295237959508));
#202628=CARTESIAN_POINT('Ctrl Pts',(9.98509531816012,12.2,5.20565887883078));
#202629=CARTESIAN_POINT('Ctrl Pts',(9.98729910386338,12.2,5.20837350606551));
#202630=CARTESIAN_POINT('Ctrl Pts',(9.98950417899161,12.2,5.21109625221659));
#202631=CARTESIAN_POINT('Ctrl Pts',(9.99170925411983,12.2,5.21381899836768));
#202632=CARTESIAN_POINT('Ctrl Pts',(9.99391561913965,12.2,5.21654986178508));
#202633=CARTESIAN_POINT('Ctrl Pts',(9.99612322926766,12.2,5.21928883397652));
#202634=CARTESIAN_POINT('Ctrl Pts',(9.99833083939567,12.2,5.22202780616795));
#202635=CARTESIAN_POINT('Ctrl Pts',(10.0005396956591,12.2,5.22477488629703));
#202636=CARTESIAN_POINT('Ctrl Pts',(10.0027497543974,12.2,5.22753006566695));
#202637=CARTESIAN_POINT('Ctrl Pts',(10.0049598131356,12.2,5.23028524503687));
#202638=CARTESIAN_POINT('Ctrl Pts',(10.0071710738982,12.2,5.2330485228809));
#202639=CARTESIAN_POINT('Ctrl Pts',(10.0093834949843,12.2,5.23581988907078));
#202640=CARTESIAN_POINT('Ctrl Pts',(10.0115959164723,12.2,5.23859125576411));
#202641=CARTESIAN_POINT('Ctrl Pts',(10.0138094967274,12.2,5.24137071126807));
#202642=CARTESIAN_POINT('Ctrl Pts',(10.0160241937161,12.2,5.24415824588262));
#202643=CARTESIAN_POINT('Ctrl Pts',(10.0182388903024,12.2,5.24694577999077));
#202644=CARTESIAN_POINT('Ctrl Pts',(10.0204547034721,12.2,5.24974139239017));
#202645=CARTESIAN_POINT('Ctrl Pts',(10.0226715910166,12.2,5.25254507362233));
#202646=CARTESIAN_POINT('Ctrl Pts',(10.0248884785611,12.2,5.25534875485449));
#202647=CARTESIAN_POINT('Ctrl Pts',(10.0271064388306,12.2,5.25816050491905));
#202648=CARTESIAN_POINT('Ctrl Pts',(10.0293254309999,12.2,5.26098031323327));
#202649=CARTESIAN_POINT('Ctrl Pts',(10.0315444231693,12.2,5.26380012154749));
#202650=CARTESIAN_POINT('Ctrl Pts',(10.0337644473053,12.2,5.26662798972803));
#202651=CARTESIAN_POINT('Ctrl Pts',(10.0359854609745,12.2,5.26946390595762));
#202652=CARTESIAN_POINT('Ctrl Pts',(10.0382064746437,12.2,5.27229982218721));
#202653=CARTESIAN_POINT('Ctrl Pts',(10.0404284785563,12.2,5.27514378734362));
#202654=CARTESIAN_POINT('Ctrl Pts',(10.0426514293365,12.2,5.27799579075655));
#202655=CARTESIAN_POINT('Ctrl Pts',(10.0448743801167,12.2,5.28084779416948));
#202656=CARTESIAN_POINT('Ctrl Pts',(10.0470982781459,12.2,5.28370783632999));
#202657=CARTESIAN_POINT('Ctrl Pts',(10.0493230827316,12.2,5.2865759065997));
#202658=CARTESIAN_POINT('Ctrl Pts',(10.0515478877215,12.2,5.28944397739043));
#202659=CARTESIAN_POINT('Ctrl Pts',(10.0537735983283,12.2,5.29232007740844));
#202660=CARTESIAN_POINT('Ctrl Pts',(10.056000174277,12.2,5.29520419466202));
#202661=CARTESIAN_POINT('Ctrl Pts',(10.0582267498212,12.2,5.29808831139165));
#202662=CARTESIAN_POINT('Ctrl Pts',(10.060454188907,12.2,5.30098044535419));
#202663=CARTESIAN_POINT('Ctrl Pts',(10.0626824524928,12.2,5.30388058849952));
#202664=CARTESIAN_POINT('Ctrl Pts',(10.0649107160786,12.2,5.30678073164485));
#202665=CARTESIAN_POINT('Ctrl Pts',(10.0671398026062,12.2,5.30968888257857));
#202666=CARTESIAN_POINT('Ctrl Pts',(10.0693696722853,12.2,5.31260503077759));
#202667=CARTESIAN_POINT('Ctrl Pts',(10.0715995419644,12.2,5.3155211789766));
#202668=CARTESIAN_POINT('Ctrl Pts',(10.0738301953189,12.2,5.31844532504053));
#202669=CARTESIAN_POINT('Ctrl Pts',(10.0760615894979,12.2,5.32137745823894));
#202670=CARTESIAN_POINT('Ctrl Pts',(10.078292983677,12.2,5.32430959143735));
#202671=CARTESIAN_POINT('Ctrl Pts',(10.0805251189044,12.2,5.32724971145321));
#202672=CARTESIAN_POINT('Ctrl Pts',(10.0827579565316,12.2,5.33019780817872));
#202673=CARTESIAN_POINT('Ctrl Pts',(10.0849907941587,12.2,5.33314590490424));
#202674=CARTESIAN_POINT('Ctrl Pts',(10.0872243328275,12.2,5.33610197891256));
#202675=CARTESIAN_POINT('Ctrl Pts',(10.0894585339962,12.2,5.33906601909544));
#202676=CARTESIAN_POINT('Ctrl Pts',(10.0916927355708,12.2,5.3420300598168));
#202677=CARTESIAN_POINT('Ctrl Pts',(10.0939275994623,12.2,5.34500206646539));
#202678=CARTESIAN_POINT('Ctrl Pts',(10.0961630849956,12.2,5.34798202964957));
#202679=CARTESIAN_POINT('Ctrl Pts',(10.0983985701228,12.2,5.35096199229238));
#202680=CARTESIAN_POINT('Ctrl Pts',(10.1006346761188,12.2,5.35394991028789));
#202681=CARTESIAN_POINT('Ctrl Pts',(10.1028713623994,12.2,5.35694577403797));
#202682=CARTESIAN_POINT('Ctrl Pts',(10.1051080486799,12.2,5.35994163778804));
#202683=CARTESIAN_POINT('Ctrl Pts',(10.1073453144585,12.2,5.36294544515376));
#202684=CARTESIAN_POINT('Ctrl Pts',(10.1095831227522,12.2,5.36595718783667));
#202685=CARTESIAN_POINT('Ctrl Pts',(10.1118209310459,12.2,5.36896893051959));
#202686=CARTESIAN_POINT('Ctrl Pts',(10.1140592831646,12.2,5.3719886079766));
#202687=CARTESIAN_POINT('Ctrl Pts',(10.1162981414999,12.2,5.37501621019992));
#202688=CARTESIAN_POINT('Ctrl Pts',(10.1185369998353,12.2,5.37804381242326));
#202689=CARTESIAN_POINT('Ctrl Pts',(10.1207763667872,12.2,5.3810793403296));
#202690=CARTESIAN_POINT('Ctrl Pts',(10.1230161954141,12.2,5.38412278142666));
#202691=CARTESIAN_POINT('Ctrl Pts',(10.1252560240411,12.2,5.38716622252373));
#202692=CARTESIAN_POINT('Ctrl Pts',(10.127496314736,12.2,5.39021757578404));
#202693=CARTESIAN_POINT('Ctrl Pts',(10.1297370200581,12.2,5.39327682915812));
#202694=CARTESIAN_POINT('Ctrl Pts',(10.1319777253802,12.2,5.3963360825322));
#202695=CARTESIAN_POINT('Ctrl Pts',(10.1342188448594,12.2,5.39940323605904));
#202696=CARTESIAN_POINT('Ctrl Pts',(10.136460352528,12.2,5.40247828182125));
#202697=CARTESIAN_POINT('Ctrl Pts',(10.1394490296908,12.2,5.40657834320993));
#202698=CARTESIAN_POINT('Ctrl Pts',(10.1424383928518,12.2,5.41069243854174));
#202699=CARTESIAN_POINT('Ctrl Pts',(10.1454284469999,12.2,5.41482055299999));
#202700=CARTESIAN_POINT('Ctrl Pts',(9.95917514599994,15.2,5.75020264099999));
#202701=CARTESIAN_POINT('Ctrl Pts',(9.95917514599994,11.6,5.75020264099999));
#202702=CARTESIAN_POINT('Ctrl Pts',(9.95841243099994,15.2,5.75014920999998));
#202703=CARTESIAN_POINT('Ctrl Pts',(9.95841243099994,11.6,5.75014920999998));
#202704=CARTESIAN_POINT('Ctrl Pts',(9.95688745999994,15.2,5.75004209399999));
#202705=CARTESIAN_POINT('Ctrl Pts',(9.95688745999994,11.6,5.75004209399999));
#202706=CARTESIAN_POINT('Ctrl Pts',(9.95460138399994,15.2,5.74988064799999));
#202707=CARTESIAN_POINT('Ctrl Pts',(9.95460138399994,11.6,5.74988064799999));
#202708=CARTESIAN_POINT('Ctrl Pts',(9.95155604399995,15.2,5.74966384999998));
#202709=CARTESIAN_POINT('Ctrl Pts',(9.95155604399995,11.6,5.74966384999998));
#202710=CARTESIAN_POINT('Ctrl Pts',(9.94775396999995,15.2,5.74939028999999));
#202711=CARTESIAN_POINT('Ctrl Pts',(9.94775396999995,11.6,5.74939028999999));
#202712=CARTESIAN_POINT('Ctrl Pts',(9.94395649899995,15.2,5.74911416799999));
#202713=CARTESIAN_POINT('Ctrl Pts',(9.94395649899995,11.6,5.74911416799999));
#202714=CARTESIAN_POINT('Ctrl Pts',(9.94016363099995,15.2,5.74883548499999));
#202715=CARTESIAN_POINT('Ctrl Pts',(9.94016363099995,11.6,5.74883548499999));
#202716=CARTESIAN_POINT('Ctrl Pts',(9.93637536999995,15.2,5.74855424299999));
#202717=CARTESIAN_POINT('Ctrl Pts',(9.93637536999995,11.6,5.74855424299999));
#202718=CARTESIAN_POINT('Ctrl Pts',(9.93259172199994,15.2,5.74827044899998));
#202719=CARTESIAN_POINT('Ctrl Pts',(9.93259172199994,11.6,5.74827044899998));
#202720=CARTESIAN_POINT('Ctrl Pts',(9.92881268899995,15.2,5.74798410599998));
#202721=CARTESIAN_POINT('Ctrl Pts',(9.92881268899995,11.6,5.74798410599998));
#202722=CARTESIAN_POINT('Ctrl Pts',(9.92503828399995,15.2,5.74769521999999));
#202723=CARTESIAN_POINT('Ctrl Pts',(9.92503828399995,11.6,5.74769521999999));
#202724=CARTESIAN_POINT('Ctrl Pts',(9.92126850899995,15.2,5.74740379999999));
#202725=CARTESIAN_POINT('Ctrl Pts',(9.92126850899995,11.6,5.74740379999999));
#202726=CARTESIAN_POINT('Ctrl Pts',(9.91750337599995,15.2,5.74710985399999));
#202727=CARTESIAN_POINT('Ctrl Pts',(9.91750337599995,11.6,5.74710985399999));
#202728=CARTESIAN_POINT('Ctrl Pts',(9.91374289199995,15.2,5.74681338699998));
#202729=CARTESIAN_POINT('Ctrl Pts',(9.91374289199995,11.6,5.74681338699998));
#202730=CARTESIAN_POINT('Ctrl Pts',(9.90998706399994,15.2,5.74651440899999));
#202731=CARTESIAN_POINT('Ctrl Pts',(9.90998706399994,11.6,5.74651440899999));
#202732=CARTESIAN_POINT('Ctrl Pts',(9.90623589999995,15.2,5.74621292499998));
#202733=CARTESIAN_POINT('Ctrl Pts',(9.90623589999995,11.6,5.74621292499998));
#202734=CARTESIAN_POINT('Ctrl Pts',(9.90248940499994,15.2,5.74590894099998));
#202735=CARTESIAN_POINT('Ctrl Pts',(9.90248940499994,11.6,5.74590894099998));
#202736=CARTESIAN_POINT('Ctrl Pts',(9.89874758699995,15.2,5.74560246199999));
#202737=CARTESIAN_POINT('Ctrl Pts',(9.89874758699995,11.6,5.74560246199999));
#202738=CARTESIAN_POINT('Ctrl Pts',(9.89501044999994,15.2,5.74529349399998));
#202739=CARTESIAN_POINT('Ctrl Pts',(9.89501044999994,11.6,5.74529349399998));
#202740=CARTESIAN_POINT('Ctrl Pts',(9.89127800099994,15.2,5.74498204399998));
#202741=CARTESIAN_POINT('Ctrl Pts',(9.89127800099994,11.6,5.74498204399998));
#202742=CARTESIAN_POINT('Ctrl Pts',(9.88755024699995,15.2,5.74466811599999));
#202743=CARTESIAN_POINT('Ctrl Pts',(9.88755024699995,11.6,5.74466811599999));
#202744=CARTESIAN_POINT('Ctrl Pts',(9.88382719199994,15.2,5.74435171599998));
#202745=CARTESIAN_POINT('Ctrl Pts',(9.88382719199994,11.6,5.74435171599998));
#202746=CARTESIAN_POINT('Ctrl Pts',(9.88010884599994,15.2,5.74403285099999));
#202747=CARTESIAN_POINT('Ctrl Pts',(9.88010884599994,11.6,5.74403285099999));
#202748=CARTESIAN_POINT('Ctrl Pts',(9.87639521399995,15.2,5.74371152899998));
#202749=CARTESIAN_POINT('Ctrl Pts',(9.87639521399995,11.6,5.74371152899998));
#202750=CARTESIAN_POINT('Ctrl Pts',(9.87268630299994,15.2,5.74338775499999));
#202751=CARTESIAN_POINT('Ctrl Pts',(9.87268630299994,11.6,5.74338775499999));
#202752=CARTESIAN_POINT('Ctrl Pts',(9.86898211999995,15.2,5.74306153399998));
#202753=CARTESIAN_POINT('Ctrl Pts',(9.86898211999995,11.6,5.74306153399998));
#202754=CARTESIAN_POINT('Ctrl Pts',(9.86528267199994,15.2,5.74273287599999));
#202755=CARTESIAN_POINT('Ctrl Pts',(9.86528267199994,11.6,5.74273287599999));
#202756=CARTESIAN_POINT('Ctrl Pts',(9.86158796599995,15.2,5.74240178399998));
#202757=CARTESIAN_POINT('Ctrl Pts',(9.86158796599995,11.6,5.74240178399998));
#202758=CARTESIAN_POINT('Ctrl Pts',(9.85789800899994,15.2,5.74206826699999));
#202759=CARTESIAN_POINT('Ctrl Pts',(9.85789800899994,11.6,5.74206826699999));
#202760=CARTESIAN_POINT('Ctrl Pts',(9.85421280599994,15.2,5.74173232999998));
#202761=CARTESIAN_POINT('Ctrl Pts',(9.85421280599994,11.6,5.74173232999998));
#202762=CARTESIAN_POINT('Ctrl Pts',(9.85053236499994,15.2,5.74139397699999));
#202763=CARTESIAN_POINT('Ctrl Pts',(9.85053236499994,11.6,5.74139397699999));
#202764=CARTESIAN_POINT('Ctrl Pts',(9.84685669199994,15.2,5.74105321899999));
#202765=CARTESIAN_POINT('Ctrl Pts',(9.84685669199994,11.6,5.74105321899999));
#202766=CARTESIAN_POINT('Ctrl Pts',(9.84318579299994,15.2,5.74071005899999));
#202767=CARTESIAN_POINT('Ctrl Pts',(9.84318579299994,11.6,5.74071005899999));
#202768=CARTESIAN_POINT('Ctrl Pts',(9.83951967699995,15.2,5.74036450399999));
#202769=CARTESIAN_POINT('Ctrl Pts',(9.83951967699995,11.6,5.74036450399999));
#202770=CARTESIAN_POINT('Ctrl Pts',(9.83585834799995,15.2,5.74001656099998));
#202771=CARTESIAN_POINT('Ctrl Pts',(9.83585834799995,11.6,5.74001656099998));
#202772=CARTESIAN_POINT('Ctrl Pts',(9.83220181499994,15.2,5.73966623599999));
#202773=CARTESIAN_POINT('Ctrl Pts',(9.83220181499994,11.6,5.73966623599999));
#202774=CARTESIAN_POINT('Ctrl Pts',(9.82855008299994,15.2,5.73931353499999));
#202775=CARTESIAN_POINT('Ctrl Pts',(9.82855008299994,11.6,5.73931353499999));
#202776=CARTESIAN_POINT('Ctrl Pts',(9.82490315999994,15.2,5.73895846699998));
#202777=CARTESIAN_POINT('Ctrl Pts',(9.82490315999994,11.6,5.73895846699998));
#202778=CARTESIAN_POINT('Ctrl Pts',(9.82126105299994,15.2,5.73860103599999));
#202779=CARTESIAN_POINT('Ctrl Pts',(9.82126105299994,11.6,5.73860103599999));
#202780=CARTESIAN_POINT('Ctrl Pts',(9.81762376699994,15.2,5.73824124899998));
#202781=CARTESIAN_POINT('Ctrl Pts',(9.81762376699994,11.6,5.73824124899998));
#202782=CARTESIAN_POINT('Ctrl Pts',(9.81399130999994,15.2,5.73787911299998));
#202783=CARTESIAN_POINT('Ctrl Pts',(9.81399130999994,11.6,5.73787911299998));
#202784=CARTESIAN_POINT('Ctrl Pts',(9.81036368999994,15.2,5.73751463399999));
#202785=CARTESIAN_POINT('Ctrl Pts',(9.81036368999994,11.6,5.73751463399999));
#202786=CARTESIAN_POINT('Ctrl Pts',(9.80674090999995,15.2,5.73714781899999));
#202787=CARTESIAN_POINT('Ctrl Pts',(9.80674090999995,11.6,5.73714781899999));
#202788=CARTESIAN_POINT('Ctrl Pts',(9.80312298099994,15.2,5.73677867599999));
#202789=CARTESIAN_POINT('Ctrl Pts',(9.80312298099994,11.6,5.73677867599999));
#202790=CARTESIAN_POINT('Ctrl Pts',(9.79950990699994,15.2,5.73640720799999));
#202791=CARTESIAN_POINT('Ctrl Pts',(9.79950990699994,11.6,5.73640720799999));
#202792=CARTESIAN_POINT('Ctrl Pts',(9.79590169599994,15.2,5.73603342499998));
#202793=CARTESIAN_POINT('Ctrl Pts',(9.79590169599994,11.6,5.73603342499998));
#202794=CARTESIAN_POINT('Ctrl Pts',(9.79229835399994,15.2,5.73565733199998));
#202795=CARTESIAN_POINT('Ctrl Pts',(9.79229835399994,11.6,5.73565733199998));
#202796=CARTESIAN_POINT('Ctrl Pts',(9.78869988999995,15.2,5.73527893499998));
#202797=CARTESIAN_POINT('Ctrl Pts',(9.78869988999995,11.6,5.73527893499998));
#202798=CARTESIAN_POINT('Ctrl Pts',(9.78510630799994,15.2,5.73489824299998));
#202799=CARTESIAN_POINT('Ctrl Pts',(9.78510630799994,11.6,5.73489824299998));
#202800=CARTESIAN_POINT('Ctrl Pts',(9.78151761599995,15.2,5.73451526099999));
#202801=CARTESIAN_POINT('Ctrl Pts',(9.78151761599995,11.6,5.73451526099999));
#202802=CARTESIAN_POINT('Ctrl Pts',(9.77793381999994,15.2,5.73412999599999));
#202803=CARTESIAN_POINT('Ctrl Pts',(9.77793381999994,11.6,5.73412999599999));
#202804=CARTESIAN_POINT('Ctrl Pts',(9.77435492799994,15.2,5.73374245399998));
#202805=CARTESIAN_POINT('Ctrl Pts',(9.77435492799994,11.6,5.73374245399998));
#202806=CARTESIAN_POINT('Ctrl Pts',(9.77078094799994,15.2,5.73335264399999));
#202807=CARTESIAN_POINT('Ctrl Pts',(9.77078094799994,11.6,5.73335264399999));
#202808=CARTESIAN_POINT('Ctrl Pts',(9.76721188399994,15.2,5.73296056999999));
#202809=CARTESIAN_POINT('Ctrl Pts',(9.76721188399994,11.6,5.73296056999999));
#202810=CARTESIAN_POINT('Ctrl Pts',(9.76364774399994,15.2,5.73256623999999));
#202811=CARTESIAN_POINT('Ctrl Pts',(9.76364774399994,11.6,5.73256623999999));
#202812=CARTESIAN_POINT('Ctrl Pts',(9.76008853499994,15.2,5.73216966199999));
#202813=CARTESIAN_POINT('Ctrl Pts',(9.76008853499994,11.6,5.73216966199999));
#202814=CARTESIAN_POINT('Ctrl Pts',(9.75653426499995,15.2,5.73177084099999));
#202815=CARTESIAN_POINT('Ctrl Pts',(9.75653426499995,11.6,5.73177084099999));
#202816=CARTESIAN_POINT('Ctrl Pts',(9.75298493899994,15.2,5.73136978499999));
#202817=CARTESIAN_POINT('Ctrl Pts',(9.75298493899994,11.6,5.73136978499999));
#202818=CARTESIAN_POINT('Ctrl Pts',(9.74944056499995,15.2,5.73096649999999));
#202819=CARTESIAN_POINT('Ctrl Pts',(9.74944056499995,11.6,5.73096649999999));
#202820=CARTESIAN_POINT('Ctrl Pts',(9.74590114799994,15.2,5.73056099299999));
#202821=CARTESIAN_POINT('Ctrl Pts',(9.74590114799994,11.6,5.73056099299999));
#202822=CARTESIAN_POINT('Ctrl Pts',(9.74236669799994,15.2,5.73015327099998));
#202823=CARTESIAN_POINT('Ctrl Pts',(9.74236669799994,11.6,5.73015327099998));
#202824=CARTESIAN_POINT('Ctrl Pts',(9.73883722099995,15.2,5.72974334099998));
#202825=CARTESIAN_POINT('Ctrl Pts',(9.73883722099995,11.6,5.72974334099998));
#202826=CARTESIAN_POINT('Ctrl Pts',(9.73531272199994,15.2,5.72933120999998));
#202827=CARTESIAN_POINT('Ctrl Pts',(9.73531272199994,11.6,5.72933120999998));
#202828=CARTESIAN_POINT('Ctrl Pts',(9.73179320799994,15.2,5.72891688399999));
#202829=CARTESIAN_POINT('Ctrl Pts',(9.73179320799994,11.6,5.72891688399999));
#202830=CARTESIAN_POINT('Ctrl Pts',(9.72827868999994,15.2,5.72850037199998));
#202831=CARTESIAN_POINT('Ctrl Pts',(9.72827868999994,11.6,5.72850037199998));
#202832=CARTESIAN_POINT('Ctrl Pts',(9.72476916999995,15.2,5.72808167999998));
#202833=CARTESIAN_POINT('Ctrl Pts',(9.72476916999995,11.6,5.72808167999998));
#202834=CARTESIAN_POINT('Ctrl Pts',(9.72126465599995,15.2,5.72766081399998));
#202835=CARTESIAN_POINT('Ctrl Pts',(9.72126465599995,11.6,5.72766081399998));
#202836=CARTESIAN_POINT('Ctrl Pts',(9.71776515699995,15.2,5.72723778199999));
#202837=CARTESIAN_POINT('Ctrl Pts',(9.71776515699995,11.6,5.72723778199999));
#202838=CARTESIAN_POINT('Ctrl Pts',(9.71427067999995,15.2,5.72681258999998));
#202839=CARTESIAN_POINT('Ctrl Pts',(9.71427067999995,11.6,5.72681258999998));
#202840=CARTESIAN_POINT('Ctrl Pts',(9.71078122899995,15.2,5.72638524699999));
#202841=CARTESIAN_POINT('Ctrl Pts',(9.71078122899995,11.6,5.72638524699999));
#202842=CARTESIAN_POINT('Ctrl Pts',(9.70729681399994,15.2,5.72595575799999));
#202843=CARTESIAN_POINT('Ctrl Pts',(9.70729681399994,11.6,5.72595575799999));
#202844=CARTESIAN_POINT('Ctrl Pts',(9.70381743999994,15.2,5.72552413199999));
#202845=CARTESIAN_POINT('Ctrl Pts',(9.70381743999994,11.6,5.72552413199999));
#202846=CARTESIAN_POINT('Ctrl Pts',(9.70034311499995,15.2,5.72509037399998));
#202847=CARTESIAN_POINT('Ctrl Pts',(9.70034311499995,11.6,5.72509037399998));
#202848=CARTESIAN_POINT('Ctrl Pts',(9.69687384599995,15.2,5.72465449299998));
#202849=CARTESIAN_POINT('Ctrl Pts',(9.69687384599995,11.6,5.72465449299998));
#202850=CARTESIAN_POINT('Ctrl Pts',(9.69340963899995,15.2,5.72421649499999));
#202851=CARTESIAN_POINT('Ctrl Pts',(9.69340963899995,11.6,5.72421649499999));
#202852=CARTESIAN_POINT('Ctrl Pts',(9.68995050199995,15.2,5.72377638799999));
#202853=CARTESIAN_POINT('Ctrl Pts',(9.68995050199995,11.6,5.72377638799999));
#202854=CARTESIAN_POINT('Ctrl Pts',(9.68649644099994,15.2,5.72333417799998));
#202855=CARTESIAN_POINT('Ctrl Pts',(9.68649644099994,11.6,5.72333417799998));
#202856=CARTESIAN_POINT('Ctrl Pts',(9.68304746299994,15.2,5.72288987399999));
#202857=CARTESIAN_POINT('Ctrl Pts',(9.68304746299994,11.6,5.72288987399999));
#202858=CARTESIAN_POINT('Ctrl Pts',(9.67960357799994,15.2,5.72244348099999));
#202859=CARTESIAN_POINT('Ctrl Pts',(9.67960357799994,11.6,5.72244348099999));
#202860=CARTESIAN_POINT('Ctrl Pts',(9.67616478999994,15.2,5.72199500699998));
#202861=CARTESIAN_POINT('Ctrl Pts',(9.67616478999994,11.6,5.72199500699998));
#202862=CARTESIAN_POINT('Ctrl Pts',(9.67273110599994,15.2,5.72154445999999));
#202863=CARTESIAN_POINT('Ctrl Pts',(9.67273110599994,11.6,5.72154445999999));
#202864=CARTESIAN_POINT('Ctrl Pts',(9.66930253399994,15.2,5.72109184799999));
#202865=CARTESIAN_POINT('Ctrl Pts',(9.66930253399994,11.6,5.72109184799999));
#202866=CARTESIAN_POINT('Ctrl Pts',(9.66587907999994,15.2,5.72063717499999));
#202867=CARTESIAN_POINT('Ctrl Pts',(9.66587907999994,11.6,5.72063717499999));
#202868=CARTESIAN_POINT('Ctrl Pts',(9.66246075399994,15.2,5.72018045199999));
#202869=CARTESIAN_POINT('Ctrl Pts',(9.66246075399994,11.6,5.72018045199999));
#202870=CARTESIAN_POINT('Ctrl Pts',(9.65904755999994,15.2,5.71972168499999));
#202871=CARTESIAN_POINT('Ctrl Pts',(9.65904755999994,11.6,5.71972168499999));
#202872=CARTESIAN_POINT('Ctrl Pts',(9.65563950499994,15.2,5.71926088099998));
#202873=CARTESIAN_POINT('Ctrl Pts',(9.65563950499994,11.6,5.71926088099998));
#202874=CARTESIAN_POINT('Ctrl Pts',(9.65223659799994,15.2,5.71879804699999));
#202875=CARTESIAN_POINT('Ctrl Pts',(9.65223659799994,11.6,5.71879804699999));
#202876=CARTESIAN_POINT('Ctrl Pts',(9.64883884499995,15.2,5.71833318999998));
#202877=CARTESIAN_POINT('Ctrl Pts',(9.64883884499995,11.6,5.71833318999998));
#202878=CARTESIAN_POINT('Ctrl Pts',(9.64544625399995,15.2,5.71786631999998));
#202879=CARTESIAN_POINT('Ctrl Pts',(9.64544625399995,11.6,5.71786631999998));
#202880=CARTESIAN_POINT('Ctrl Pts',(9.64205882999994,15.2,5.71739744199999));
#202881=CARTESIAN_POINT('Ctrl Pts',(9.64205882999994,11.6,5.71739744199999));
#202882=CARTESIAN_POINT('Ctrl Pts',(9.63867658199995,15.2,5.71692656499999));
#202883=CARTESIAN_POINT('Ctrl Pts',(9.63867658199995,11.6,5.71692656499999));
#202884=CARTESIAN_POINT('Ctrl Pts',(9.63529951699994,15.2,5.71645369399998));
#202885=CARTESIAN_POINT('Ctrl Pts',(9.63529951699994,11.6,5.71645369399998));
#202886=CARTESIAN_POINT('Ctrl Pts',(9.63192764199994,15.2,5.71597883899998));
#202887=CARTESIAN_POINT('Ctrl Pts',(9.63192764199994,11.6,5.71597883899998));
#202888=CARTESIAN_POINT('Ctrl Pts',(9.62856096299994,15.2,5.71550200699999));
#202889=CARTESIAN_POINT('Ctrl Pts',(9.62856096299994,11.6,5.71550200699999));
#202890=CARTESIAN_POINT('Ctrl Pts',(9.62519948899994,15.2,5.71502320599999));
#202891=CARTESIAN_POINT('Ctrl Pts',(9.62519948899994,11.6,5.71502320599999));
#202892=CARTESIAN_POINT('Ctrl Pts',(9.62184322499994,15.2,5.71454244099999));
#202893=CARTESIAN_POINT('Ctrl Pts',(9.62184322499994,11.6,5.71454244099999));
#202894=CARTESIAN_POINT('Ctrl Pts',(9.61849217999994,15.2,5.71405972199998));
#202895=CARTESIAN_POINT('Ctrl Pts',(9.61849217999994,11.6,5.71405972199998));
#202896=CARTESIAN_POINT('Ctrl Pts',(9.61514635999994,15.2,5.71357505599998));
#202897=CARTESIAN_POINT('Ctrl Pts',(9.61514635999994,11.6,5.71357505599998));
#202898=CARTESIAN_POINT('Ctrl Pts',(9.61180577299995,15.2,5.71308845099999));
#202899=CARTESIAN_POINT('Ctrl Pts',(9.61180577299995,11.6,5.71308845099999));
#202900=CARTESIAN_POINT('Ctrl Pts',(9.60847042599994,15.2,5.71259991399998));
#202901=CARTESIAN_POINT('Ctrl Pts',(9.60847042599994,11.6,5.71259991399998));
#202902=CARTESIAN_POINT('Ctrl Pts',(9.60514032499994,15.2,5.71210945199999));
#202903=CARTESIAN_POINT('Ctrl Pts',(9.60514032499994,11.6,5.71210945199999));
#202904=CARTESIAN_POINT('Ctrl Pts',(9.60181547999994,15.2,5.71161707499999));
#202905=CARTESIAN_POINT('Ctrl Pts',(9.60181547999994,11.6,5.71161707499999));
#202906=CARTESIAN_POINT('Ctrl Pts',(9.59849589499994,15.2,5.71112278799998));
#202907=CARTESIAN_POINT('Ctrl Pts',(9.59849589499994,11.6,5.71112278799998));
#202908=CARTESIAN_POINT('Ctrl Pts',(9.59518157899995,15.2,5.71062659899999));
#202909=CARTESIAN_POINT('Ctrl Pts',(9.59518157899995,11.6,5.71062659899999));
#202910=CARTESIAN_POINT('Ctrl Pts',(9.59187253899995,15.2,5.71012851899999));
#202911=CARTESIAN_POINT('Ctrl Pts',(9.59187253899995,11.6,5.71012851899999));
#202912=CARTESIAN_POINT('Ctrl Pts',(9.58856878199994,15.2,5.70962855199999));
#202913=CARTESIAN_POINT('Ctrl Pts',(9.58856878199994,11.6,5.70962855199999));
#202914=CARTESIAN_POINT('Ctrl Pts',(9.58527031499995,15.2,5.70912670699999));
#202915=CARTESIAN_POINT('Ctrl Pts',(9.58527031499995,11.6,5.70912670699999));
#202916=CARTESIAN_POINT('Ctrl Pts',(9.58197714599994,15.2,5.70862299299999));
#202917=CARTESIAN_POINT('Ctrl Pts',(9.58197714599994,11.6,5.70862299299999));
#202918=CARTESIAN_POINT('Ctrl Pts',(9.57868928099994,15.2,5.70811741599999));
#202919=CARTESIAN_POINT('Ctrl Pts',(9.57868928099994,11.6,5.70811741599999));
#202920=CARTESIAN_POINT('Ctrl Pts',(9.57540672899994,15.2,5.70760998399999));
#202921=CARTESIAN_POINT('Ctrl Pts',(9.57540672899994,11.6,5.70760998399999));
#202922=CARTESIAN_POINT('Ctrl Pts',(9.57212949599995,15.2,5.70710070699998));
#202923=CARTESIAN_POINT('Ctrl Pts',(9.57212949599995,11.6,5.70710070699998));
#202924=CARTESIAN_POINT('Ctrl Pts',(9.56885758899995,15.2,5.70658958999999));
#202925=CARTESIAN_POINT('Ctrl Pts',(9.56885758899995,11.6,5.70658958999999));
#202926=CARTESIAN_POINT('Ctrl Pts',(9.56559101699994,15.2,5.70607664299998));
#202927=CARTESIAN_POINT('Ctrl Pts',(9.56559101699994,11.6,5.70607664299998));
#202928=CARTESIAN_POINT('Ctrl Pts',(9.56232978499994,15.2,5.70556187299999));
#202929=CARTESIAN_POINT('Ctrl Pts',(9.56232978499994,11.6,5.70556187299999));
#202930=CARTESIAN_POINT('Ctrl Pts',(9.55907390099994,15.2,5.70504528899999));
#202931=CARTESIAN_POINT('Ctrl Pts',(9.55907390099994,11.6,5.70504528899999));
#202932=CARTESIAN_POINT('Ctrl Pts',(9.55582337399994,15.2,5.70452689699999));
#202933=CARTESIAN_POINT('Ctrl Pts',(9.55582337399994,11.6,5.70452689699999));
#202934=CARTESIAN_POINT('Ctrl Pts',(9.55257820899994,15.2,5.70400670599999));
#202935=CARTESIAN_POINT('Ctrl Pts',(9.55257820899994,11.6,5.70400670599999));
#202936=CARTESIAN_POINT('Ctrl Pts',(9.54933841599994,15.2,5.70348472499998));
#202937=CARTESIAN_POINT('Ctrl Pts',(9.54933841599994,11.6,5.70348472499998));
#202938=CARTESIAN_POINT('Ctrl Pts',(9.54610399999994,15.2,5.70296096099998));
#202939=CARTESIAN_POINT('Ctrl Pts',(9.54610399999994,11.6,5.70296096099998));
#202940=CARTESIAN_POINT('Ctrl Pts',(9.54287496799994,15.2,5.70243542199999));
#202941=CARTESIAN_POINT('Ctrl Pts',(9.54287496799994,11.6,5.70243542199999));
#202942=CARTESIAN_POINT('Ctrl Pts',(9.53965132899994,15.2,5.70190811599999));
#202943=CARTESIAN_POINT('Ctrl Pts',(9.53965132899994,11.6,5.70190811599999));
#202944=CARTESIAN_POINT('Ctrl Pts',(9.53643308999995,15.2,5.70137905199999));
#202945=CARTESIAN_POINT('Ctrl Pts',(9.53643308999995,11.6,5.70137905199999));
#202946=CARTESIAN_POINT('Ctrl Pts',(9.53322025799994,15.2,5.70084823799998));
#202947=CARTESIAN_POINT('Ctrl Pts',(9.53322025799994,11.6,5.70084823799998));
#202948=CARTESIAN_POINT('Ctrl Pts',(9.53001284099994,15.2,5.70031568099999));
#202949=CARTESIAN_POINT('Ctrl Pts',(9.53001284099994,11.6,5.70031568099999));
#202950=CARTESIAN_POINT('Ctrl Pts',(9.52681084499994,15.2,5.69978138999998));
#202951=CARTESIAN_POINT('Ctrl Pts',(9.52681084499994,11.6,5.69978138999998));
#202952=CARTESIAN_POINT('Ctrl Pts',(9.52361427899995,15.2,5.69924537299999));
#202953=CARTESIAN_POINT('Ctrl Pts',(9.52361427899995,11.6,5.69924537299999));
#202954=CARTESIAN_POINT('Ctrl Pts',(9.52042314999994,15.2,5.69870763799998));
#202955=CARTESIAN_POINT('Ctrl Pts',(9.52042314999994,11.6,5.69870763799998));
#202956=CARTESIAN_POINT('Ctrl Pts',(9.51723746399994,15.2,5.69816819399998));
#202957=CARTESIAN_POINT('Ctrl Pts',(9.51723746399994,11.6,5.69816819399998));
#202958=CARTESIAN_POINT('Ctrl Pts',(9.51405722999995,15.2,5.69762704899999));
#202959=CARTESIAN_POINT('Ctrl Pts',(9.51405722999995,11.6,5.69762704899999));
#202960=CARTESIAN_POINT('Ctrl Pts',(9.51088245499994,15.2,5.69708421099998));
#202961=CARTESIAN_POINT('Ctrl Pts',(9.51088245499994,11.6,5.69708421099998));
#202962=CARTESIAN_POINT('Ctrl Pts',(9.50771314699994,15.2,5.69653968799999));
#202963=CARTESIAN_POINT('Ctrl Pts',(9.50771314699994,11.6,5.69653968799999));
#202964=CARTESIAN_POINT('Ctrl Pts',(9.50454931099994,15.2,5.69599348799999));
#202965=CARTESIAN_POINT('Ctrl Pts',(9.50454931099994,11.6,5.69599348799999));
#202966=CARTESIAN_POINT('Ctrl Pts',(9.50139095799994,15.2,5.69544562099999));
#202967=CARTESIAN_POINT('Ctrl Pts',(9.50139095799994,11.6,5.69544562099999));
#202968=CARTESIAN_POINT('Ctrl Pts',(9.49823809299994,15.2,5.69489609399999));
#202969=CARTESIAN_POINT('Ctrl Pts',(9.49823809299994,11.6,5.69489609399999));
#202970=CARTESIAN_POINT('Ctrl Pts',(9.49509072499995,15.2,5.69434491599999));
#202971=CARTESIAN_POINT('Ctrl Pts',(9.49509072499995,11.6,5.69434491599999));
#202972=CARTESIAN_POINT('Ctrl Pts',(9.49194885999994,15.2,5.69379209499999));
#202973=CARTESIAN_POINT('Ctrl Pts',(9.49194885999994,11.6,5.69379209499999));
#202974=CARTESIAN_POINT('Ctrl Pts',(9.48881250599995,15.2,5.69323763999999));
#202975=CARTESIAN_POINT('Ctrl Pts',(9.48881250599995,11.6,5.69323763999999));
#202976=CARTESIAN_POINT('Ctrl Pts',(9.48568167099994,15.2,5.69268155999998));
#202977=CARTESIAN_POINT('Ctrl Pts',(9.48568167099994,11.6,5.69268155999998));
#202978=CARTESIAN_POINT('Ctrl Pts',(9.48255636299994,15.2,5.69212386099998));
#202979=CARTESIAN_POINT('Ctrl Pts',(9.48255636299994,11.6,5.69212386099998));
#202980=CARTESIAN_POINT('Ctrl Pts',(9.47943658699995,15.2,5.69156455499999));
#202981=CARTESIAN_POINT('Ctrl Pts',(9.47943658699995,11.6,5.69156455499999));
#202982=CARTESIAN_POINT('Ctrl Pts',(9.47632235299994,15.2,5.69100364699998));
#202983=CARTESIAN_POINT('Ctrl Pts',(9.47632235299994,11.6,5.69100364699998));
#202984=CARTESIAN_POINT('Ctrl Pts',(9.47321366799994,15.2,5.69044114799999));
#202985=CARTESIAN_POINT('Ctrl Pts',(9.47321366799994,11.6,5.69044114799999));
#202986=CARTESIAN_POINT('Ctrl Pts',(9.47011053899995,15.2,5.68987706599999));
#202987=CARTESIAN_POINT('Ctrl Pts',(9.47011053899995,11.6,5.68987706599999));
#202988=CARTESIAN_POINT('Ctrl Pts',(9.46701297399994,15.2,5.68931140899998));
#202989=CARTESIAN_POINT('Ctrl Pts',(9.46701297399994,11.6,5.68931140899998));
#202990=CARTESIAN_POINT('Ctrl Pts',(9.46392097999994,15.2,5.68874418599999));
#202991=CARTESIAN_POINT('Ctrl Pts',(9.46392097999994,11.6,5.68874418599999));
#202992=CARTESIAN_POINT('Ctrl Pts',(9.46083456599995,15.2,5.68817540699998));
#202993=CARTESIAN_POINT('Ctrl Pts',(9.46083456599995,11.6,5.68817540699998));
#202994=CARTESIAN_POINT('Ctrl Pts',(9.45775373799994,15.2,5.68760507899999));
#202995=CARTESIAN_POINT('Ctrl Pts',(9.45775373799994,11.6,5.68760507899999));
#202996=CARTESIAN_POINT('Ctrl Pts',(9.45467850399995,15.2,5.68703321099999));
#202997=CARTESIAN_POINT('Ctrl Pts',(9.45467850399995,11.6,5.68703321099999));
#202998=CARTESIAN_POINT('Ctrl Pts',(9.45160887199994,15.2,5.68645981199998));
#202999=CARTESIAN_POINT('Ctrl Pts',(9.45160887199994,11.6,5.68645981199998));
#203000=CARTESIAN_POINT('Ctrl Pts',(9.44854484899994,15.2,5.68588488999998));
#203001=CARTESIAN_POINT('Ctrl Pts',(9.44854484899994,11.6,5.68588488999998));
#203002=CARTESIAN_POINT('Ctrl Pts',(9.44548644299994,15.2,5.68530845399999));
#203003=CARTESIAN_POINT('Ctrl Pts',(9.44548644299994,11.6,5.68530845399999));
#203004=CARTESIAN_POINT('Ctrl Pts',(9.44243366199995,15.2,5.68473051499998));
#203005=CARTESIAN_POINT('Ctrl Pts',(9.44243366199995,11.6,5.68473051499998));
#203006=CARTESIAN_POINT('Ctrl Pts',(9.43938651299994,15.2,5.68415107899998));
#203007=CARTESIAN_POINT('Ctrl Pts',(9.43938651299994,11.6,5.68415107899998));
#203008=CARTESIAN_POINT('Ctrl Pts',(9.43634500399994,15.2,5.68357015699998));
#203009=CARTESIAN_POINT('Ctrl Pts',(9.43634500399994,11.6,5.68357015699998));
#203010=CARTESIAN_POINT('Ctrl Pts',(9.43330914299995,15.2,5.68298775599998));
#203011=CARTESIAN_POINT('Ctrl Pts',(9.43330914299995,11.6,5.68298775599998));
#203012=CARTESIAN_POINT('Ctrl Pts',(9.43027893599995,15.2,5.68240388599998));
#203013=CARTESIAN_POINT('Ctrl Pts',(9.43027893599995,11.6,5.68240388599998));
#203014=CARTESIAN_POINT('Ctrl Pts',(9.42725439399995,15.2,5.68181855599998));
#203015=CARTESIAN_POINT('Ctrl Pts',(9.42725439399995,11.6,5.68181855599998));
#203016=CARTESIAN_POINT('Ctrl Pts',(9.42423552099994,15.2,5.68123177399999));
#203017=CARTESIAN_POINT('Ctrl Pts',(9.42423552099994,11.6,5.68123177399999));
#203018=CARTESIAN_POINT('Ctrl Pts',(9.42122232599995,15.2,5.68064355099998));
#203019=CARTESIAN_POINT('Ctrl Pts',(9.42122232599995,11.6,5.68064355099998));
#203020=CARTESIAN_POINT('Ctrl Pts',(9.41821481799994,15.2,5.68005389299999));
#203021=CARTESIAN_POINT('Ctrl Pts',(9.41821481799994,11.6,5.68005389299999));
#203022=CARTESIAN_POINT('Ctrl Pts',(9.41521300399994,15.2,5.67946281199998));
#203023=CARTESIAN_POINT('Ctrl Pts',(9.41521300399994,11.6,5.67946281199998));
#203024=CARTESIAN_POINT('Ctrl Pts',(9.41221688999994,15.2,5.67887031499998));
#203025=CARTESIAN_POINT('Ctrl Pts',(9.41221688999994,11.6,5.67887031499998));
#203026=CARTESIAN_POINT('Ctrl Pts',(9.40922648699994,15.2,5.67827641199998));
#203027=CARTESIAN_POINT('Ctrl Pts',(9.40922648699994,11.6,5.67827641199998));
#203028=CARTESIAN_POINT('Ctrl Pts',(9.40624179999995,15.2,5.67768111199998));
#203029=CARTESIAN_POINT('Ctrl Pts',(9.40624179999995,11.6,5.67768111199998));
#203030=CARTESIAN_POINT('Ctrl Pts',(9.40326283699994,15.2,5.67708442399999));
#203031=CARTESIAN_POINT('Ctrl Pts',(9.40326283699994,11.6,5.67708442399999));
#203032=CARTESIAN_POINT('Ctrl Pts',(9.40028960699994,15.2,5.67648635799999));
#203033=CARTESIAN_POINT('Ctrl Pts',(9.40028960699994,11.6,5.67648635799999));
#203034=CARTESIAN_POINT('Ctrl Pts',(9.39732211799994,15.2,5.67588692199998));
#203035=CARTESIAN_POINT('Ctrl Pts',(9.39732211799994,11.6,5.67588692199998));
#203036=CARTESIAN_POINT('Ctrl Pts',(9.39436037699994,15.2,5.67528612499999));
#203037=CARTESIAN_POINT('Ctrl Pts',(9.39436037699994,11.6,5.67528612499999));
#203038=CARTESIAN_POINT('Ctrl Pts',(9.39140439099994,15.2,5.67468397899999));
#203039=CARTESIAN_POINT('Ctrl Pts',(9.39140439099994,11.6,5.67468397899999));
#203040=CARTESIAN_POINT('Ctrl Pts',(9.38845416799994,15.2,5.67408048999998));
#203041=CARTESIAN_POINT('Ctrl Pts',(9.38845416799994,11.6,5.67408048999998));
#203042=CARTESIAN_POINT('Ctrl Pts',(9.38550971799994,15.2,5.67347566799998));
#203043=CARTESIAN_POINT('Ctrl Pts',(9.38550971799994,11.6,5.67347566799998));
#203044=CARTESIAN_POINT('Ctrl Pts',(9.38257104799994,15.2,5.67286952399999));
#203045=CARTESIAN_POINT('Ctrl Pts',(9.38257104799994,11.6,5.67286952399999));
#203046=CARTESIAN_POINT('Ctrl Pts',(9.37963816299994,15.2,5.67226206499999));
#203047=CARTESIAN_POINT('Ctrl Pts',(9.37963816299994,11.6,5.67226206499999));
#203048=CARTESIAN_POINT('Ctrl Pts',(9.37671107399994,15.2,5.67165330199998));
#203049=CARTESIAN_POINT('Ctrl Pts',(9.37671107399994,11.6,5.67165330199998));
#203050=CARTESIAN_POINT('Ctrl Pts',(9.37378978799994,15.2,5.67104324499999));
#203051=CARTESIAN_POINT('Ctrl Pts',(9.37378978799994,11.6,5.67104324499999));
#203052=CARTESIAN_POINT('Ctrl Pts',(9.37087431199994,15.2,5.67043190199998));
#203053=CARTESIAN_POINT('Ctrl Pts',(9.37087431199994,11.6,5.67043190199998));
#203054=CARTESIAN_POINT('Ctrl Pts',(9.36796465499994,15.2,5.66981928199999));
#203055=CARTESIAN_POINT('Ctrl Pts',(9.36796465499994,11.6,5.66981928199999));
#203056=CARTESIAN_POINT('Ctrl Pts',(9.36506082499994,15.2,5.66920539599998));
#203057=CARTESIAN_POINT('Ctrl Pts',(9.36506082499994,11.6,5.66920539599998));
#203058=CARTESIAN_POINT('Ctrl Pts',(9.36216282899995,15.2,5.66859025299999));
#203059=CARTESIAN_POINT('Ctrl Pts',(9.36216282899995,11.6,5.66859025299999));
#203060=CARTESIAN_POINT('Ctrl Pts',(9.35927067599994,15.2,5.66797386399998));
#203061=CARTESIAN_POINT('Ctrl Pts',(9.35927067599994,11.6,5.66797386399998));
#203062=CARTESIAN_POINT('Ctrl Pts',(9.35638437199995,15.2,5.66735623499999));
#203063=CARTESIAN_POINT('Ctrl Pts',(9.35638437199995,11.6,5.66735623499999));
#203064=CARTESIAN_POINT('Ctrl Pts',(9.35350392699995,15.2,5.66673737799999));
#203065=CARTESIAN_POINT('Ctrl Pts',(9.35350392699995,11.6,5.66673737799999));
#203066=CARTESIAN_POINT('Ctrl Pts',(9.35062934799994,15.2,5.66611730299999));
#203067=CARTESIAN_POINT('Ctrl Pts',(9.35062934799994,11.6,5.66611730299999));
#203068=CARTESIAN_POINT('Ctrl Pts',(9.34776064299994,15.2,5.66549601799998));
#203069=CARTESIAN_POINT('Ctrl Pts',(9.34776064299994,11.6,5.66549601799998));
#203070=CARTESIAN_POINT('Ctrl Pts',(9.34489781999994,15.2,5.66487353499999));
#203071=CARTESIAN_POINT('Ctrl Pts',(9.34489781999994,11.6,5.66487353499999));
#203072=CARTESIAN_POINT('Ctrl Pts',(9.34204088699994,15.2,5.66424986199999));
#203073=CARTESIAN_POINT('Ctrl Pts',(9.34204088699994,11.6,5.66424986199999));
#203074=CARTESIAN_POINT('Ctrl Pts',(9.33918985299995,15.2,5.66362500899999));
#203075=CARTESIAN_POINT('Ctrl Pts',(9.33918985299995,11.6,5.66362500899999));
#203076=CARTESIAN_POINT('Ctrl Pts',(9.33634472399994,15.2,5.66299898499998));
#203077=CARTESIAN_POINT('Ctrl Pts',(9.33634472399994,11.6,5.66299898499998));
#203078=CARTESIAN_POINT('Ctrl Pts',(9.33350550899995,15.2,5.66237180199998));
#203079=CARTESIAN_POINT('Ctrl Pts',(9.33350550899995,11.6,5.66237180199998));
#203080=CARTESIAN_POINT('Ctrl Pts',(9.33067221599994,15.2,5.66174346799999));
#203081=CARTESIAN_POINT('Ctrl Pts',(9.33067221599994,11.6,5.66174346799999));
#203082=CARTESIAN_POINT('Ctrl Pts',(9.32784485399995,15.2,5.66111399399999));
#203083=CARTESIAN_POINT('Ctrl Pts',(9.32784485399995,11.6,5.66111399399999));
#203084=CARTESIAN_POINT('Ctrl Pts',(9.32502342999994,15.2,5.66048338899999));
#203085=CARTESIAN_POINT('Ctrl Pts',(9.32502342999994,11.6,5.66048338899999));
#203086=CARTESIAN_POINT('Ctrl Pts',(9.32220795199994,15.2,5.65985166299999));
#203087=CARTESIAN_POINT('Ctrl Pts',(9.32220795199994,11.6,5.65985166299999));
#203088=CARTESIAN_POINT('Ctrl Pts',(9.31939842799994,15.2,5.65921882599999));
#203089=CARTESIAN_POINT('Ctrl Pts',(9.31939842799994,11.6,5.65921882599999));
#203090=CARTESIAN_POINT('Ctrl Pts',(9.31659486699994,15.2,5.65858488899998));
#203091=CARTESIAN_POINT('Ctrl Pts',(9.31659486699994,11.6,5.65858488899998));
#203092=CARTESIAN_POINT('Ctrl Pts',(9.31379727599994,15.2,5.65794985999998));
#203093=CARTESIAN_POINT('Ctrl Pts',(9.31379727599994,11.6,5.65794985999998));
#203094=CARTESIAN_POINT('Ctrl Pts',(9.31100566399994,15.2,5.65731375099999));
#203095=CARTESIAN_POINT('Ctrl Pts',(9.31100566399994,11.6,5.65731375099999));
#203096=CARTESIAN_POINT('Ctrl Pts',(9.30822003899994,15.2,5.65667657099999));
#203097=CARTESIAN_POINT('Ctrl Pts',(9.30822003899994,11.6,5.65667657099999));
#203098=CARTESIAN_POINT('Ctrl Pts',(9.30544040899994,15.2,5.65603833099999));
#203099=CARTESIAN_POINT('Ctrl Pts',(9.30544040899994,11.6,5.65603833099999));
#203100=CARTESIAN_POINT('Ctrl Pts',(9.30266678099994,15.2,5.65539904099998));
#203101=CARTESIAN_POINT('Ctrl Pts',(9.30266678099994,11.6,5.65539904099998));
#203102=CARTESIAN_POINT('Ctrl Pts',(9.29989916399995,15.2,5.65475870899999));
#203103=CARTESIAN_POINT('Ctrl Pts',(9.29989916399995,11.6,5.65475870899999));
#203104=CARTESIAN_POINT('Ctrl Pts',(9.29713756699994,15.2,5.65411734799999));
#203105=CARTESIAN_POINT('Ctrl Pts',(9.29713756699994,11.6,5.65411734799999));
#203106=CARTESIAN_POINT('Ctrl Pts',(9.29438199799994,15.2,5.65347496699999));
#203107=CARTESIAN_POINT('Ctrl Pts',(9.29438199799994,11.6,5.65347496699999));
#203108=CARTESIAN_POINT('Ctrl Pts',(9.29163246399994,15.2,5.65283157699999));
#203109=CARTESIAN_POINT('Ctrl Pts',(9.29163246399994,11.6,5.65283157699999));
#203110=CARTESIAN_POINT('Ctrl Pts',(9.28888897399995,15.2,5.65218718699998));
#203111=CARTESIAN_POINT('Ctrl Pts',(9.28888897399995,11.6,5.65218718699998));
#203112=CARTESIAN_POINT('Ctrl Pts',(9.28615153699995,15.2,5.65154180799999));
#203113=CARTESIAN_POINT('Ctrl Pts',(9.28615153699995,11.6,5.65154180799999));
#203114=CARTESIAN_POINT('Ctrl Pts',(9.28342015899995,15.2,5.65089544999999));
#203115=CARTESIAN_POINT('Ctrl Pts',(9.28342015899995,11.6,5.65089544999999));
#203116=CARTESIAN_POINT('Ctrl Pts',(9.28069484999994,15.2,5.65024812499999));
#203117=CARTESIAN_POINT('Ctrl Pts',(9.28069484999994,11.6,5.65024812499999));
#203118=CARTESIAN_POINT('Ctrl Pts',(9.27797561899995,15.2,5.64959983999999));
#203119=CARTESIAN_POINT('Ctrl Pts',(9.27797561899995,11.6,5.64959983999999));
#203120=CARTESIAN_POINT('Ctrl Pts',(9.27526247199994,15.2,5.64895060899998));
#203121=CARTESIAN_POINT('Ctrl Pts',(9.27526247199994,11.6,5.64895060899998));
#203122=CARTESIAN_POINT('Ctrl Pts',(9.27255541799994,15.2,5.64830044099998));
#203123=CARTESIAN_POINT('Ctrl Pts',(9.27255541799994,11.6,5.64830044099998));
#203124=CARTESIAN_POINT('Ctrl Pts',(9.26985446699994,15.2,5.64764934699999));
#203125=CARTESIAN_POINT('Ctrl Pts',(9.26985446699994,11.6,5.64764934699999));
#203126=CARTESIAN_POINT('Ctrl Pts',(9.26715962499994,15.2,5.64699733499998));
#203127=CARTESIAN_POINT('Ctrl Pts',(9.26715962499994,11.6,5.64699733499998));
#203128=CARTESIAN_POINT('Ctrl Pts',(9.26447090199994,15.2,5.64634441999999));
#203129=CARTESIAN_POINT('Ctrl Pts',(9.26447090199994,11.6,5.64634441999999));
#203130=CARTESIAN_POINT('Ctrl Pts',(9.26178830499994,15.2,5.64569060999998));
#203131=CARTESIAN_POINT('Ctrl Pts',(9.26178830499994,11.6,5.64569060999998));
#203132=CARTESIAN_POINT('Ctrl Pts',(9.25911184299995,15.2,5.64503591499999));
#203133=CARTESIAN_POINT('Ctrl Pts',(9.25911184299995,11.6,5.64503591499999));
#203134=CARTESIAN_POINT('Ctrl Pts',(9.25644152499994,15.2,5.64438034699998));
#203135=CARTESIAN_POINT('Ctrl Pts',(9.25644152499994,11.6,5.64438034699998));
#203136=CARTESIAN_POINT('Ctrl Pts',(9.25377735799995,15.2,5.64372391599999));
#203137=CARTESIAN_POINT('Ctrl Pts',(9.25377735799995,11.6,5.64372391599999));
#203138=CARTESIAN_POINT('Ctrl Pts',(9.25111935099994,15.2,5.64306663299998));
#203139=CARTESIAN_POINT('Ctrl Pts',(9.25111935099994,11.6,5.64306663299998));
#203140=CARTESIAN_POINT('Ctrl Pts',(9.24846751299994,15.2,5.64240850999998));
#203141=CARTESIAN_POINT('Ctrl Pts',(9.24846751299994,11.6,5.64240850999998));
#203142=CARTESIAN_POINT('Ctrl Pts',(9.24582185199995,15.2,5.64174955399999));
#203143=CARTESIAN_POINT('Ctrl Pts',(9.24582185199995,11.6,5.64174955399999));
#203144=CARTESIAN_POINT('Ctrl Pts',(9.24318237599994,15.2,5.64108978099998));
#203145=CARTESIAN_POINT('Ctrl Pts',(9.24318237599994,11.6,5.64108978099998));
#203146=CARTESIAN_POINT('Ctrl Pts',(9.24054909399995,15.2,5.64042919699999));
#203147=CARTESIAN_POINT('Ctrl Pts',(9.24054909399995,11.6,5.64042919699999));
#203148=CARTESIAN_POINT('Ctrl Pts',(9.23792201399994,15.2,5.63976781699999));
#203149=CARTESIAN_POINT('Ctrl Pts',(9.23792201399994,11.6,5.63976781699999));
#203150=CARTESIAN_POINT('Ctrl Pts',(9.23530114399994,15.2,5.63910564999999));
#203151=CARTESIAN_POINT('Ctrl Pts',(9.23530114399994,11.6,5.63910564999999));
#203152=CARTESIAN_POINT('Ctrl Pts',(9.23268649399994,15.2,5.63844270699998));
#203153=CARTESIAN_POINT('Ctrl Pts',(9.23268649399994,11.6,5.63844270699998));
#203154=CARTESIAN_POINT('Ctrl Pts',(9.23007807099994,15.2,5.63777899799998));
#203155=CARTESIAN_POINT('Ctrl Pts',(9.23007807099994,11.6,5.63777899799998));
#203156=CARTESIAN_POINT('Ctrl Pts',(9.22747588499995,15.2,5.63711453599999));
#203157=CARTESIAN_POINT('Ctrl Pts',(9.22747588499995,11.6,5.63711453599999));
#203158=CARTESIAN_POINT('Ctrl Pts',(9.22487994299994,15.2,5.63644933199999));
#203159=CARTESIAN_POINT('Ctrl Pts',(9.22487994299994,11.6,5.63644933199999));
#203160=CARTESIAN_POINT('Ctrl Pts',(9.22229025399995,15.2,5.63578339499998));
#203161=CARTESIAN_POINT('Ctrl Pts',(9.22229025399995,11.6,5.63578339499998));
#203162=CARTESIAN_POINT('Ctrl Pts',(9.21970682699994,15.2,5.63511673799999));
#203163=CARTESIAN_POINT('Ctrl Pts',(9.21970682699994,11.6,5.63511673799999));
#203164=CARTESIAN_POINT('Ctrl Pts',(9.21712967099995,15.2,5.63444937099998));
#203165=CARTESIAN_POINT('Ctrl Pts',(9.21712967099995,11.6,5.63444937099998));
#203166=CARTESIAN_POINT('Ctrl Pts',(9.21455879299995,15.2,5.63378130699999));
#203167=CARTESIAN_POINT('Ctrl Pts',(9.21455879299995,11.6,5.63378130699999));
#203168=CARTESIAN_POINT('Ctrl Pts',(9.21199420199994,15.2,5.63311255599999));
#203169=CARTESIAN_POINT('Ctrl Pts',(9.21199420199994,11.6,5.63311255599999));
#203170=CARTESIAN_POINT('Ctrl Pts',(9.20943590799994,15.2,5.63244312799998));
#203171=CARTESIAN_POINT('Ctrl Pts',(9.20943590799994,11.6,5.63244312799998));
#203172=CARTESIAN_POINT('Ctrl Pts',(9.20688391799995,15.2,5.63177303699998));
#203173=CARTESIAN_POINT('Ctrl Pts',(9.20688391799995,11.6,5.63177303699998));
#203174=CARTESIAN_POINT('Ctrl Pts',(9.20433824099994,15.2,5.63110229299999));
#203175=CARTESIAN_POINT('Ctrl Pts',(9.20433824099994,11.6,5.63110229299999));
#203176=CARTESIAN_POINT('Ctrl Pts',(9.20179888699994,15.2,5.63043090699999));
#203177=CARTESIAN_POINT('Ctrl Pts',(9.20179888699994,11.6,5.63043090699999));
#203178=CARTESIAN_POINT('Ctrl Pts',(9.19926586299994,15.2,5.62975889199999));
#203179=CARTESIAN_POINT('Ctrl Pts',(9.19926586299994,11.6,5.62975889199999));
#203180=CARTESIAN_POINT('Ctrl Pts',(9.19673917799994,15.2,5.62908625699999));
#203181=CARTESIAN_POINT('Ctrl Pts',(9.19673917799994,11.6,5.62908625699999));
#203182=CARTESIAN_POINT('Ctrl Pts',(9.19421883999994,15.2,5.62841301499999));
#203183=CARTESIAN_POINT('Ctrl Pts',(9.19421883999994,11.6,5.62841301499999));
#203184=CARTESIAN_POINT('Ctrl Pts',(9.19170485999994,15.2,5.62773917799999));
#203185=CARTESIAN_POINT('Ctrl Pts',(9.19170485999994,11.6,5.62773917799999));
#203186=CARTESIAN_POINT('Ctrl Pts',(9.18919724499995,15.2,5.62706475599998));
#203187=CARTESIAN_POINT('Ctrl Pts',(9.18919724499995,11.6,5.62706475599998));
#203188=CARTESIAN_POINT('Ctrl Pts',(9.18669600399994,15.2,5.62638976199998));
#203189=CARTESIAN_POINT('Ctrl Pts',(9.18669600399994,11.6,5.62638976199998));
#203190=CARTESIAN_POINT('Ctrl Pts',(9.18420114599994,15.2,5.62571420799999));
#203191=CARTESIAN_POINT('Ctrl Pts',(9.18420114599994,11.6,5.62571420799999));
#203192=CARTESIAN_POINT('Ctrl Pts',(9.18171267899995,15.2,5.62503810399999));
#203193=CARTESIAN_POINT('Ctrl Pts',(9.18171267899995,11.6,5.62503810399999));
#203194=CARTESIAN_POINT('Ctrl Pts',(9.17923061299994,15.2,5.62436146299999));
#203195=CARTESIAN_POINT('Ctrl Pts',(9.17923061299994,11.6,5.62436146299999));
#203196=CARTESIAN_POINT('Ctrl Pts',(9.17675495599994,15.2,5.62368429599999));
#203197=CARTESIAN_POINT('Ctrl Pts',(9.17675495599994,11.6,5.62368429599999));
#203198=CARTESIAN_POINT('Ctrl Pts',(9.17428571599994,15.2,5.62300661499999));
#203199=CARTESIAN_POINT('Ctrl Pts',(9.17428571599994,11.6,5.62300661499999));
#203200=CARTESIAN_POINT('Ctrl Pts',(9.17182290399994,15.2,5.62232843199999));
#203201=CARTESIAN_POINT('Ctrl Pts',(9.17182290399994,11.6,5.62232843199999));
#203202=CARTESIAN_POINT('Ctrl Pts',(9.16936652699994,15.2,5.62164975999998));
#203203=CARTESIAN_POINT('Ctrl Pts',(9.16936652699994,11.6,5.62164975999998));
#203204=CARTESIAN_POINT('Ctrl Pts',(9.16691659499994,15.2,5.62097060899998));
#203205=CARTESIAN_POINT('Ctrl Pts',(9.16691659499994,11.6,5.62097060899998));
#203206=CARTESIAN_POINT('Ctrl Pts',(9.16447311499994,15.2,5.62029099199999));
#203207=CARTESIAN_POINT('Ctrl Pts',(9.16447311499994,11.6,5.62029099199999));
#203208=CARTESIAN_POINT('Ctrl Pts',(9.16203609799994,15.2,5.61961092099998));
#203209=CARTESIAN_POINT('Ctrl Pts',(9.16203609799994,11.6,5.61961092099998));
#203210=CARTESIAN_POINT('Ctrl Pts',(9.15960555199994,15.2,5.61893040699999));
#203211=CARTESIAN_POINT('Ctrl Pts',(9.15960555199994,11.6,5.61893040699999));
#203212=CARTESIAN_POINT('Ctrl Pts',(9.15718148699994,15.2,5.61824946399998));
#203213=CARTESIAN_POINT('Ctrl Pts',(9.15718148699994,11.6,5.61824946399998));
#203214=CARTESIAN_POINT('Ctrl Pts',(9.15476390899994,15.2,5.61756810199999));
#203215=CARTESIAN_POINT('Ctrl Pts',(9.15476390899994,11.6,5.61756810199999));
#203216=CARTESIAN_POINT('Ctrl Pts',(9.15235282999994,15.2,5.61688633399999));
#203217=CARTESIAN_POINT('Ctrl Pts',(9.15235282999994,11.6,5.61688633399999));
#203218=CARTESIAN_POINT('Ctrl Pts',(9.14994825699995,15.2,5.61620417299999));
#203219=CARTESIAN_POINT('Ctrl Pts',(9.14994825699995,11.6,5.61620417299999));
#203220=CARTESIAN_POINT('Ctrl Pts',(9.14755020099994,15.2,5.61552162999998));
#203221=CARTESIAN_POINT('Ctrl Pts',(9.14755020099994,11.6,5.61552162999998));
#203222=CARTESIAN_POINT('Ctrl Pts',(9.14515866899994,15.2,5.61483871699998));
#203223=CARTESIAN_POINT('Ctrl Pts',(9.14515866899994,11.6,5.61483871699998));
#203224=CARTESIAN_POINT('Ctrl Pts',(9.14277367099994,15.2,5.61415544799999));
#203225=CARTESIAN_POINT('Ctrl Pts',(9.14277367099994,11.6,5.61415544799999));
#203226=CARTESIAN_POINT('Ctrl Pts',(9.14039521599994,15.2,5.61347183499999));
#203227=CARTESIAN_POINT('Ctrl Pts',(9.14039521599994,11.6,5.61347183499999));
#203228=CARTESIAN_POINT('Ctrl Pts',(9.13802331299994,15.2,5.61278788899998));
#203229=CARTESIAN_POINT('Ctrl Pts',(9.13802331299994,11.6,5.61278788899998));
#203230=CARTESIAN_POINT('Ctrl Pts',(9.13565796999994,15.2,5.61210362299998));
#203231=CARTESIAN_POINT('Ctrl Pts',(9.13565796999994,11.6,5.61210362299998));
#203232=CARTESIAN_POINT('Ctrl Pts',(9.13329919699994,15.2,5.61141905099999));
#203233=CARTESIAN_POINT('Ctrl Pts',(9.13329919699994,11.6,5.61141905099999));
#203234=CARTESIAN_POINT('Ctrl Pts',(9.13094700399995,15.2,5.61073418299999));
#203235=CARTESIAN_POINT('Ctrl Pts',(9.13094700399995,11.6,5.61073418299999));
#203236=CARTESIAN_POINT('Ctrl Pts',(9.12860139899994,15.2,5.61004903299998));
#203237=CARTESIAN_POINT('Ctrl Pts',(9.12860139899994,11.6,5.61004903299998));
#203238=CARTESIAN_POINT('Ctrl Pts',(9.12626239099994,15.2,5.60936361399998));
#203239=CARTESIAN_POINT('Ctrl Pts',(9.12626239099994,11.6,5.60936361399998));
#203240=CARTESIAN_POINT('Ctrl Pts',(9.12392998999995,15.2,5.60867793699998));
#203241=CARTESIAN_POINT('Ctrl Pts',(9.12392998999995,11.6,5.60867793699998));
#203242=CARTESIAN_POINT('Ctrl Pts',(9.12160420399994,15.2,5.60799201699999));
#203243=CARTESIAN_POINT('Ctrl Pts',(9.12160420399994,11.6,5.60799201699999));
#203244=CARTESIAN_POINT('Ctrl Pts',(9.11928504399994,15.2,5.60730586399998));
#203245=CARTESIAN_POINT('Ctrl Pts',(9.11928504399994,11.6,5.60730586399998));
#203246=CARTESIAN_POINT('Ctrl Pts',(9.11697251599995,15.2,5.60661949299998));
#203247=CARTESIAN_POINT('Ctrl Pts',(9.11697251599995,11.6,5.60661949299998));
#203248=CARTESIAN_POINT('Ctrl Pts',(9.11466663299995,15.2,5.60593291599999));
#203249=CARTESIAN_POINT('Ctrl Pts',(9.11466663299995,11.6,5.60593291599999));
#203250=CARTESIAN_POINT('Ctrl Pts',(9.11236740099995,15.2,5.60524614599998));
#203251=CARTESIAN_POINT('Ctrl Pts',(9.11236740099995,11.6,5.60524614599998));
#203252=CARTESIAN_POINT('Ctrl Pts',(9.11007483199995,15.2,5.60455919599999));
#203253=CARTESIAN_POINT('Ctrl Pts',(9.11007483199995,11.6,5.60455919599999));
#203254=CARTESIAN_POINT('Ctrl Pts',(9.10778893399995,15.2,5.60387207799998));
#203255=CARTESIAN_POINT('Ctrl Pts',(9.10778893399995,11.6,5.60387207799998));
#203256=CARTESIAN_POINT('Ctrl Pts',(9.10550971499994,15.2,5.60318480599998));
#203257=CARTESIAN_POINT('Ctrl Pts',(9.10550971499994,11.6,5.60318480599998));
#203258=CARTESIAN_POINT('Ctrl Pts',(9.10323718599994,15.2,5.60249739199998));
#203259=CARTESIAN_POINT('Ctrl Pts',(9.10323718599994,11.6,5.60249739199998));
#203260=CARTESIAN_POINT('Ctrl Pts',(9.10097135599995,15.2,5.60180985099999));
#203261=CARTESIAN_POINT('Ctrl Pts',(9.10097135599995,11.6,5.60180985099999));
#203262=CARTESIAN_POINT('Ctrl Pts',(9.09871223299995,15.2,5.60112219399999));
#203263=CARTESIAN_POINT('Ctrl Pts',(9.09871223299995,11.6,5.60112219399999));
#203264=CARTESIAN_POINT('Ctrl Pts',(9.09645982899994,15.2,5.60043443499998));
#203265=CARTESIAN_POINT('Ctrl Pts',(9.09645982899994,11.6,5.60043443499998));
#203266=CARTESIAN_POINT('Ctrl Pts',(9.09421415199994,15.2,5.59974658699999));
#203267=CARTESIAN_POINT('Ctrl Pts',(9.09421415199994,11.6,5.59974658699999));
#203268=CARTESIAN_POINT('Ctrl Pts',(9.09197521099994,15.2,5.59905866399999));
#203269=CARTESIAN_POINT('Ctrl Pts',(9.09197521099994,11.6,5.59905866399999));
#203270=CARTESIAN_POINT('Ctrl Pts',(9.08974301599994,15.2,5.59837067899998));
#203271=CARTESIAN_POINT('Ctrl Pts',(9.08974301599994,11.6,5.59837067899998));
#203272=CARTESIAN_POINT('Ctrl Pts',(9.08751757499994,15.2,5.59768264499999));
#203273=CARTESIAN_POINT('Ctrl Pts',(9.08751757499994,11.6,5.59768264499999));
#203274=CARTESIAN_POINT('Ctrl Pts',(9.08529889899994,15.2,5.59699457499998));
#203275=CARTESIAN_POINT('Ctrl Pts',(9.08529889899994,11.6,5.59699457499998));
#203276=CARTESIAN_POINT('Ctrl Pts',(9.08308699699995,15.2,5.59630648299999));
#203277=CARTESIAN_POINT('Ctrl Pts',(9.08308699699995,11.6,5.59630648299999));
#203278=CARTESIAN_POINT('Ctrl Pts',(9.08088187999994,15.2,5.59561838299998));
#203279=CARTESIAN_POINT('Ctrl Pts',(9.08088187999994,11.6,5.59561838299998));
#203280=CARTESIAN_POINT('Ctrl Pts',(9.07868355399994,15.2,5.59493028699999));
#203281=CARTESIAN_POINT('Ctrl Pts',(9.07868355399994,11.6,5.59493028699999));
#203282=CARTESIAN_POINT('Ctrl Pts',(9.07649203099994,15.2,5.59424220999999));
#203283=CARTESIAN_POINT('Ctrl Pts',(9.07649203099994,11.6,5.59424220999999));
#203284=CARTESIAN_POINT('Ctrl Pts',(9.07430732099994,15.2,5.59355416599999));
#203285=CARTESIAN_POINT('Ctrl Pts',(9.07430732099994,11.6,5.59355416599999));
#203286=CARTESIAN_POINT('Ctrl Pts',(9.07212943199994,15.2,5.59286616699998));
#203287=CARTESIAN_POINT('Ctrl Pts',(9.07212943199994,11.6,5.59286616699998));
#203288=CARTESIAN_POINT('Ctrl Pts',(9.06995837399995,15.2,5.59217822799998));
#203289=CARTESIAN_POINT('Ctrl Pts',(9.06995837399995,11.6,5.59217822799998));
#203290=CARTESIAN_POINT('Ctrl Pts',(9.06779415699994,15.2,5.59149036099999));
#203291=CARTESIAN_POINT('Ctrl Pts',(9.06779415699994,11.6,5.59149036099999));
#203292=CARTESIAN_POINT('Ctrl Pts',(9.06563679099994,15.2,5.59080258199998));
#203293=CARTESIAN_POINT('Ctrl Pts',(9.06563679099994,11.6,5.59080258199998));
#203294=CARTESIAN_POINT('Ctrl Pts',(9.06348628499994,15.2,5.59011490399998));
#203295=CARTESIAN_POINT('Ctrl Pts',(9.06348628499994,11.6,5.59011490399998));
#203296=CARTESIAN_POINT('Ctrl Pts',(9.06134264799995,15.2,5.58942733999999));
#203297=CARTESIAN_POINT('Ctrl Pts',(9.06134264799995,11.6,5.58942733999999));
#203298=CARTESIAN_POINT('Ctrl Pts',(9.05920589099994,15.2,5.58873990499999));
#203299=CARTESIAN_POINT('Ctrl Pts',(9.05920589099994,11.6,5.58873990499999));
#203300=CARTESIAN_POINT('Ctrl Pts',(9.05707602299995,15.2,5.58805261299998));
#203301=CARTESIAN_POINT('Ctrl Pts',(9.05707602299995,11.6,5.58805261299998));
#203302=CARTESIAN_POINT('Ctrl Pts',(9.05495305299995,15.2,5.58736547799998));
#203303=CARTESIAN_POINT('Ctrl Pts',(9.05495305299995,11.6,5.58736547799998));
#203304=CARTESIAN_POINT('Ctrl Pts',(9.05283699199994,15.2,5.58667851399999));
#203305=CARTESIAN_POINT('Ctrl Pts',(9.05283699199994,11.6,5.58667851399999));
#203306=CARTESIAN_POINT('Ctrl Pts',(9.05072784999994,15.2,5.58599173499999));
#203307=CARTESIAN_POINT('Ctrl Pts',(9.05072784999994,11.6,5.58599173499999));
#203308=CARTESIAN_POINT('Ctrl Pts',(9.04862563599995,15.2,5.58530515499999));
#203309=CARTESIAN_POINT('Ctrl Pts',(9.04862563599995,11.6,5.58530515499999));
#203310=CARTESIAN_POINT('Ctrl Pts',(9.04653035899995,15.2,5.58461878899998));
#203311=CARTESIAN_POINT('Ctrl Pts',(9.04653035899995,11.6,5.58461878899998));
#203312=CARTESIAN_POINT('Ctrl Pts',(9.04444203099994,15.2,5.58393264999999));
#203313=CARTESIAN_POINT('Ctrl Pts',(9.04444203099994,11.6,5.58393264999999));
#203314=CARTESIAN_POINT('Ctrl Pts',(9.04236065999994,15.2,5.58324675499998));
#203315=CARTESIAN_POINT('Ctrl Pts',(9.04236065999994,11.6,5.58324675499998));
#203316=CARTESIAN_POINT('Ctrl Pts',(9.04028625599994,15.2,5.58256111499999));
#203317=CARTESIAN_POINT('Ctrl Pts',(9.04028625599994,11.6,5.58256111499999));
#203318=CARTESIAN_POINT('Ctrl Pts',(9.03821882999994,15.2,5.58187574599998));
#203319=CARTESIAN_POINT('Ctrl Pts',(9.03821882999994,11.6,5.58187574599998));
#203320=CARTESIAN_POINT('Ctrl Pts',(9.03615839099994,15.2,5.58119066299999));
#203321=CARTESIAN_POINT('Ctrl Pts',(9.03615839099994,11.6,5.58119066299999));
#203322=CARTESIAN_POINT('Ctrl Pts',(9.03410494899994,15.2,5.58050587999999));
#203323=CARTESIAN_POINT('Ctrl Pts',(9.03410494899994,11.6,5.58050587999999));
#203324=CARTESIAN_POINT('Ctrl Pts',(9.03205851499994,15.2,5.57982141199999));
#203325=CARTESIAN_POINT('Ctrl Pts',(9.03205851499994,11.6,5.57982141199999));
#203326=CARTESIAN_POINT('Ctrl Pts',(9.03001909699995,15.2,5.57913727299999));
#203327=CARTESIAN_POINT('Ctrl Pts',(9.03001909699995,11.6,5.57913727299999));
#203328=CARTESIAN_POINT('Ctrl Pts',(9.02798670599994,15.2,5.57845347799999));
#203329=CARTESIAN_POINT('Ctrl Pts',(9.02798670599994,11.6,5.57845347799999));
#203330=CARTESIAN_POINT('Ctrl Pts',(9.02596135199994,15.2,5.57777004299999));
#203331=CARTESIAN_POINT('Ctrl Pts',(9.02596135199994,11.6,5.57777004299999));
#203332=CARTESIAN_POINT('Ctrl Pts',(9.02394304599994,15.2,5.57708698099999));
#203333=CARTESIAN_POINT('Ctrl Pts',(9.02394304599994,11.6,5.57708698099999));
#203334=CARTESIAN_POINT('Ctrl Pts',(9.02193179699994,15.2,5.57640430699998));
#203335=CARTESIAN_POINT('Ctrl Pts',(9.02193179699994,11.6,5.57640430699998));
#203336=CARTESIAN_POINT('Ctrl Pts',(9.01992761499995,15.2,5.57572203699999));
#203337=CARTESIAN_POINT('Ctrl Pts',(9.01992761499995,11.6,5.57572203699999));
#203338=CARTESIAN_POINT('Ctrl Pts',(9.01793051099994,15.2,5.57504018599998));
#203339=CARTESIAN_POINT('Ctrl Pts',(9.01793051099994,11.6,5.57504018599998));
#203340=CARTESIAN_POINT('Ctrl Pts',(9.01594049299994,15.2,5.57435876699999));
#203341=CARTESIAN_POINT('Ctrl Pts',(9.01594049299994,11.6,5.57435876699999));
#203342=CARTESIAN_POINT('Ctrl Pts',(9.01395757299994,15.2,5.57367779799999));
#203343=CARTESIAN_POINT('Ctrl Pts',(9.01395757299994,11.6,5.57367779799999));
#203344=CARTESIAN_POINT('Ctrl Pts',(9.01198176199994,15.2,5.57299729199999));
#203345=CARTESIAN_POINT('Ctrl Pts',(9.01198176199994,11.6,5.57299729199999));
#203346=CARTESIAN_POINT('Ctrl Pts',(9.01001306899994,15.2,5.57231726599999));
#203347=CARTESIAN_POINT('Ctrl Pts',(9.01001306899994,11.6,5.57231726599999));
#203348=CARTESIAN_POINT('Ctrl Pts',(9.00805150299994,15.2,5.57163773399999));
#203349=CARTESIAN_POINT('Ctrl Pts',(9.00805150299994,11.6,5.57163773399999));
#203350=CARTESIAN_POINT('Ctrl Pts',(9.00609707499994,15.2,5.57095871199999));
#203351=CARTESIAN_POINT('Ctrl Pts',(9.00609707499994,11.6,5.57095871199999));
#203352=CARTESIAN_POINT('Ctrl Pts',(9.00414979799995,15.2,5.57028021399999));
#203353=CARTESIAN_POINT('Ctrl Pts',(9.00414979799995,11.6,5.57028021399999));
#203354=CARTESIAN_POINT('Ctrl Pts',(9.00220967899994,15.2,5.56960225599998));
#203355=CARTESIAN_POINT('Ctrl Pts',(9.00220967899994,11.6,5.56960225599998));
#203356=CARTESIAN_POINT('Ctrl Pts',(9.00027672899994,15.2,5.56892485499999));
#203357=CARTESIAN_POINT('Ctrl Pts',(9.00027672899994,11.6,5.56892485499999));
#203358=CARTESIAN_POINT('Ctrl Pts',(8.99835095899994,15.2,5.56824802499998));
#203359=CARTESIAN_POINT('Ctrl Pts',(8.99835095899994,11.6,5.56824802499998));
#203360=CARTESIAN_POINT('Ctrl Pts',(8.99643237899994,15.2,5.56757178299998));
#203361=CARTESIAN_POINT('Ctrl Pts',(8.99643237899994,11.6,5.56757178299998));
#203362=CARTESIAN_POINT('Ctrl Pts',(8.99452099899994,15.2,5.56689614199998));
#203363=CARTESIAN_POINT('Ctrl Pts',(8.99452099899994,11.6,5.56689614199998));
#203364=CARTESIAN_POINT('Ctrl Pts',(8.99261682999994,15.2,5.56622111999998));
#203365=CARTESIAN_POINT('Ctrl Pts',(8.99261682999994,11.6,5.56622111999998));
#203366=CARTESIAN_POINT('Ctrl Pts',(8.99071988199994,15.2,5.56554673199999));
#203367=CARTESIAN_POINT('Ctrl Pts',(8.99071988199994,11.6,5.56554673199999));
#203368=CARTESIAN_POINT('Ctrl Pts',(8.98883016699994,15.2,5.56487299599999));
#203369=CARTESIAN_POINT('Ctrl Pts',(8.98883016699994,11.6,5.56487299599999));
#203370=CARTESIAN_POINT('Ctrl Pts',(8.98694769299994,15.2,5.56419992299999));
#203371=CARTESIAN_POINT('Ctrl Pts',(8.98694769299994,11.6,5.56419992299999));
#203372=CARTESIAN_POINT('Ctrl Pts',(8.98507247199994,15.2,5.56352753399998));
#203373=CARTESIAN_POINT('Ctrl Pts',(8.98507247199994,11.6,5.56352753399998));
#203374=CARTESIAN_POINT('Ctrl Pts',(8.98320451499995,15.2,5.56285584199999));
#203375=CARTESIAN_POINT('Ctrl Pts',(8.98320451499995,11.6,5.56285584199999));
#203376=CARTESIAN_POINT('Ctrl Pts',(8.98134383099995,15.2,5.56218486499999));
#203377=CARTESIAN_POINT('Ctrl Pts',(8.98134383099995,11.6,5.56218486499999));
#203378=CARTESIAN_POINT('Ctrl Pts',(8.97949043199995,15.2,5.56151461699999));
#203379=CARTESIAN_POINT('Ctrl Pts',(8.97949043199995,11.6,5.56151461699999));
#203380=CARTESIAN_POINT('Ctrl Pts',(8.97764432699995,15.2,5.56084511599998));
#203381=CARTESIAN_POINT('Ctrl Pts',(8.97764432699995,11.6,5.56084511599998));
#203382=CARTESIAN_POINT('Ctrl Pts',(8.97580552899995,15.2,5.56017637699998));
#203383=CARTESIAN_POINT('Ctrl Pts',(8.97580552899995,11.6,5.56017637699998));
#203384=CARTESIAN_POINT('Ctrl Pts',(8.97397404599995,15.2,5.55950841699998));
#203385=CARTESIAN_POINT('Ctrl Pts',(8.97397404599995,11.6,5.55950841699998));
#203386=CARTESIAN_POINT('Ctrl Pts',(8.97214989099994,15.2,5.55884125399999));
#203387=CARTESIAN_POINT('Ctrl Pts',(8.97214989099994,11.6,5.55884125399999));
#203388=CARTESIAN_POINT('Ctrl Pts',(8.97033307399994,15.2,5.55817490099999));
#203389=CARTESIAN_POINT('Ctrl Pts',(8.97033307399994,11.6,5.55817490099999));
#203390=CARTESIAN_POINT('Ctrl Pts',(8.96852360399994,15.2,5.55750937699998));
#203391=CARTESIAN_POINT('Ctrl Pts',(8.96852360399994,11.6,5.55750937699998));
#203392=CARTESIAN_POINT('Ctrl Pts',(8.96672149499994,15.2,5.55684469799999));
#203393=CARTESIAN_POINT('Ctrl Pts',(8.96672149499994,11.6,5.55684469799999));
#203394=CARTESIAN_POINT('Ctrl Pts',(8.96492675499994,15.2,5.55618087899998));
#203395=CARTESIAN_POINT('Ctrl Pts',(8.96492675499994,11.6,5.55618087899998));
#203396=CARTESIAN_POINT('Ctrl Pts',(8.96313939599995,15.2,5.55551794099999));
#203397=CARTESIAN_POINT('Ctrl Pts',(8.96313939599995,11.6,5.55551794099999));
#203398=CARTESIAN_POINT('Ctrl Pts',(8.96135942899994,15.2,5.55485589599999));
#203399=CARTESIAN_POINT('Ctrl Pts',(8.96135942899994,11.6,5.55485589599999));
#203400=CARTESIAN_POINT('Ctrl Pts',(8.95958686399995,15.2,5.55419476399998));
#203401=CARTESIAN_POINT('Ctrl Pts',(8.95958686399995,11.6,5.55419476399998));
#203402=CARTESIAN_POINT('Ctrl Pts',(8.95782171299994,15.2,5.55353455899999));
#203403=CARTESIAN_POINT('Ctrl Pts',(8.95782171299994,11.6,5.55353455899999));
#203404=CARTESIAN_POINT('Ctrl Pts',(8.95606398699995,15.2,5.55287530099999));
#203405=CARTESIAN_POINT('Ctrl Pts',(8.95606398699995,11.6,5.55287530099999));
#203406=CARTESIAN_POINT('Ctrl Pts',(8.95431369499994,15.2,5.55221700599999));
#203407=CARTESIAN_POINT('Ctrl Pts',(8.95431369499994,11.6,5.55221700599999));
#203408=CARTESIAN_POINT('Ctrl Pts',(8.95257084999994,15.2,5.55155968999999));
#203409=CARTESIAN_POINT('Ctrl Pts',(8.95257084999994,11.6,5.55155968999999));
#203410=CARTESIAN_POINT('Ctrl Pts',(8.95083546399994,15.2,5.55090337199999));
#203411=CARTESIAN_POINT('Ctrl Pts',(8.95083546399994,11.6,5.55090337199999));
#203412=CARTESIAN_POINT('Ctrl Pts',(8.94910754399995,15.2,5.55024806799998));
#203413=CARTESIAN_POINT('Ctrl Pts',(8.94910754399995,11.6,5.55024806799998));
#203414=CARTESIAN_POINT('Ctrl Pts',(8.94738710499994,15.2,5.54959379599998));
#203415=CARTESIAN_POINT('Ctrl Pts',(8.94738710499994,11.6,5.54959379599998));
#203416=CARTESIAN_POINT('Ctrl Pts',(8.94567415599994,15.2,5.54894057199999));
#203417=CARTESIAN_POINT('Ctrl Pts',(8.94567415599994,11.6,5.54894057199999));
#203418=CARTESIAN_POINT('Ctrl Pts',(8.94396870899994,15.2,5.54828841499998));
#203419=CARTESIAN_POINT('Ctrl Pts',(8.94396870899994,11.6,5.54828841499998));
#203420=CARTESIAN_POINT('Ctrl Pts',(8.94227077499994,15.2,5.54763734099998));
#203421=CARTESIAN_POINT('Ctrl Pts',(8.94227077499994,11.6,5.54763734099998));
#203422=CARTESIAN_POINT('Ctrl Pts',(8.94058036499995,15.2,5.54698736999998));
#203423=CARTESIAN_POINT('Ctrl Pts',(8.94058036499995,11.6,5.54698736999998));
#203424=CARTESIAN_POINT('Ctrl Pts',(8.93889749099994,15.2,5.54633851799998));
#203425=CARTESIAN_POINT('Ctrl Pts',(8.93889749099994,11.6,5.54633851799998));
#203426=CARTESIAN_POINT('Ctrl Pts',(8.93722216299994,15.2,5.54569080199999));
#203427=CARTESIAN_POINT('Ctrl Pts',(8.93722216299994,11.6,5.54569080199999));
#203428=CARTESIAN_POINT('Ctrl Pts',(8.93555439299995,15.2,5.54504424099999));
#203429=CARTESIAN_POINT('Ctrl Pts',(8.93555439299995,11.6,5.54504424099999));
#203430=CARTESIAN_POINT('Ctrl Pts',(8.93389419199995,15.2,5.54439885199999));
#203431=CARTESIAN_POINT('Ctrl Pts',(8.93389419199995,11.6,5.54439885199999));
#203432=CARTESIAN_POINT('Ctrl Pts',(8.93224157199995,15.2,5.54375465399998));
#203433=CARTESIAN_POINT('Ctrl Pts',(8.93224157199995,11.6,5.54375465399998));
#203434=CARTESIAN_POINT('Ctrl Pts',(8.93059654299994,15.2,5.54311166499998));
#203435=CARTESIAN_POINT('Ctrl Pts',(8.93059654299994,11.6,5.54311166499998));
#203436=CARTESIAN_POINT('Ctrl Pts',(8.92895911799994,15.2,5.54246990199999));
#203437=CARTESIAN_POINT('Ctrl Pts',(8.92895911799994,11.6,5.54246990199999));
#203438=CARTESIAN_POINT('Ctrl Pts',(8.92732930899994,15.2,5.54182938399999));
#203439=CARTESIAN_POINT('Ctrl Pts',(8.92732930899994,11.6,5.54182938399999));
#203440=CARTESIAN_POINT('Ctrl Pts',(8.92570712399994,15.2,5.54119012899999));
#203441=CARTESIAN_POINT('Ctrl Pts',(8.92570712399994,11.6,5.54119012899999));
#203442=CARTESIAN_POINT('Ctrl Pts',(8.92409257799994,15.2,5.54055215499999));
#203443=CARTESIAN_POINT('Ctrl Pts',(8.92409257799994,11.6,5.54055215499999));
#203444=CARTESIAN_POINT('Ctrl Pts',(8.92248568099994,15.2,5.53991548099999));
#203445=CARTESIAN_POINT('Ctrl Pts',(8.92248568099994,11.6,5.53991548099999));
#203446=CARTESIAN_POINT('Ctrl Pts',(8.92088644399994,15.2,5.53928012499998));
#203447=CARTESIAN_POINT('Ctrl Pts',(8.92088644399994,11.6,5.53928012499998));
#203448=CARTESIAN_POINT('Ctrl Pts',(8.91929488099995,15.2,5.53864610499998));
#203449=CARTESIAN_POINT('Ctrl Pts',(8.91929488099995,11.6,5.53864610499998));
#203450=CARTESIAN_POINT('Ctrl Pts',(8.91771100199995,15.2,5.53801344099998));
#203451=CARTESIAN_POINT('Ctrl Pts',(8.91771100199995,11.6,5.53801344099998));
#203452=CARTESIAN_POINT('Ctrl Pts',(8.91613481799994,15.2,5.53738214999999));
#203453=CARTESIAN_POINT('Ctrl Pts',(8.91613481799994,11.6,5.53738214999999));
#203454=CARTESIAN_POINT('Ctrl Pts',(8.91456634199994,15.2,5.53675225299998));
#203455=CARTESIAN_POINT('Ctrl Pts',(8.91456634199994,11.6,5.53675225299998));
#203456=CARTESIAN_POINT('Ctrl Pts',(8.91300558499994,15.2,5.53612376599999));
#203457=CARTESIAN_POINT('Ctrl Pts',(8.91300558499994,11.6,5.53612376599999));
#203458=CARTESIAN_POINT('Ctrl Pts',(8.91145255799995,15.2,5.53549671099999));
#203459=CARTESIAN_POINT('Ctrl Pts',(8.91145255799995,11.6,5.53549671099999));
#203460=CARTESIAN_POINT('Ctrl Pts',(8.90990727399994,15.2,5.53487110399999));
#203461=CARTESIAN_POINT('Ctrl Pts',(8.90990727399994,11.6,5.53487110399999));
#203462=CARTESIAN_POINT('Ctrl Pts',(8.90836974499994,15.2,5.53424696699999));
#203463=CARTESIAN_POINT('Ctrl Pts',(8.90836974499994,11.6,5.53424696699999));
#203464=CARTESIAN_POINT('Ctrl Pts',(8.90683998299994,15.2,5.53362431599999));
#203465=CARTESIAN_POINT('Ctrl Pts',(8.90683998299994,11.6,5.53362431599999));
#203466=CARTESIAN_POINT('Ctrl Pts',(8.90531799899994,15.2,5.53300317299998));
#203467=CARTESIAN_POINT('Ctrl Pts',(8.90531799899994,11.6,5.53300317299998));
#203468=CARTESIAN_POINT('Ctrl Pts',(8.90380380499994,15.2,5.53238355599999));
#203469=CARTESIAN_POINT('Ctrl Pts',(8.90380380499994,11.6,5.53238355599999));
#203470=CARTESIAN_POINT('Ctrl Pts',(8.90229741299994,15.2,5.53176548399998));
#203471=CARTESIAN_POINT('Ctrl Pts',(8.90229741299994,11.6,5.53176548399998));
#203472=CARTESIAN_POINT('Ctrl Pts',(8.90079883499994,15.2,5.53114897899999));
#203473=CARTESIAN_POINT('Ctrl Pts',(8.90079883499994,11.6,5.53114897899999));
#203474=CARTESIAN_POINT('Ctrl Pts',(8.89930808499994,15.2,5.53053405699998));
#203475=CARTESIAN_POINT('Ctrl Pts',(8.89930808499994,11.6,5.53053405699998));
#203476=CARTESIAN_POINT('Ctrl Pts',(8.89782517099994,15.2,5.52992073899999));
#203477=CARTESIAN_POINT('Ctrl Pts',(8.89782517099994,11.6,5.52992073899999));
#203478=CARTESIAN_POINT('Ctrl Pts',(8.89635010799994,15.2,5.52930904599998));
#203479=CARTESIAN_POINT('Ctrl Pts',(8.89635010799994,11.6,5.52930904599998));
#203480=CARTESIAN_POINT('Ctrl Pts',(8.89488290799994,15.2,5.52869899699999));
#203481=CARTESIAN_POINT('Ctrl Pts',(8.89488290799994,11.6,5.52869899699999));
#203482=CARTESIAN_POINT('Ctrl Pts',(8.89342358299994,15.2,5.52809061099998));
#203483=CARTESIAN_POINT('Ctrl Pts',(8.89342358299994,11.6,5.52809061099998));
#203484=CARTESIAN_POINT('Ctrl Pts',(8.89197214599994,15.2,5.52748390799999));
#203485=CARTESIAN_POINT('Ctrl Pts',(8.89197214599994,11.6,5.52748390799999));
#203486=CARTESIAN_POINT('Ctrl Pts',(8.89052860699995,15.2,5.52687890999999));
#203487=CARTESIAN_POINT('Ctrl Pts',(8.89052860699995,11.6,5.52687890999999));
#203488=CARTESIAN_POINT('Ctrl Pts',(8.88909297899995,15.2,5.52627563599999));
#203489=CARTESIAN_POINT('Ctrl Pts',(8.88909297899995,11.6,5.52627563599999));
#203490=CARTESIAN_POINT('Ctrl Pts',(8.88766527599994,15.2,5.52567410599998));
#203491=CARTESIAN_POINT('Ctrl Pts',(8.88766527599994,11.6,5.52567410599998));
#203492=CARTESIAN_POINT('Ctrl Pts',(8.88624550899995,15.2,5.52507433999998));
#203493=CARTESIAN_POINT('Ctrl Pts',(8.88624550899995,11.6,5.52507433999998));
#203494=CARTESIAN_POINT('Ctrl Pts',(8.88483369099994,15.2,5.52447635799999));
#203495=CARTESIAN_POINT('Ctrl Pts',(8.88483369099994,11.6,5.52447635799999));
#203496=CARTESIAN_POINT('Ctrl Pts',(8.88342983399994,15.2,5.52388018299999));
#203497=CARTESIAN_POINT('Ctrl Pts',(8.88342983399994,11.6,5.52388018299999));
#203498=CARTESIAN_POINT('Ctrl Pts',(8.88203394899995,15.2,5.52328583399999));
#203499=CARTESIAN_POINT('Ctrl Pts',(8.88203394899995,11.6,5.52328583399999));
#203500=CARTESIAN_POINT('Ctrl Pts',(8.88064605099995,15.2,5.52269333099999));
#203501=CARTESIAN_POINT('Ctrl Pts',(8.88064605099995,11.6,5.52269333099999));
#203502=CARTESIAN_POINT('Ctrl Pts',(8.87926615299994,15.2,5.52210269599998));
#203503=CARTESIAN_POINT('Ctrl Pts',(8.87926615299994,11.6,5.52210269599998));
#203504=CARTESIAN_POINT('Ctrl Pts',(8.87789426599995,15.2,5.52151394899998));
#203505=CARTESIAN_POINT('Ctrl Pts',(8.87789426599995,11.6,5.52151394899998));
#203506=CARTESIAN_POINT('Ctrl Pts',(8.87653040199995,15.2,5.52092711099998));
#203507=CARTESIAN_POINT('Ctrl Pts',(8.87653040199995,11.6,5.52092711099998));
#203508=CARTESIAN_POINT('Ctrl Pts',(8.87517457499994,15.2,5.52034220399998));
#203509=CARTESIAN_POINT('Ctrl Pts',(8.87517457499994,11.6,5.52034220399998));
#203510=CARTESIAN_POINT('Ctrl Pts',(8.87382679799994,15.2,5.51975924799999));
#203511=CARTESIAN_POINT('Ctrl Pts',(8.87382679799994,11.6,5.51975924799999));
#203512=CARTESIAN_POINT('Ctrl Pts',(8.87248708199994,15.2,5.51917826499999));
#203513=CARTESIAN_POINT('Ctrl Pts',(8.87248708199994,11.6,5.51917826499999));
#203514=CARTESIAN_POINT('Ctrl Pts',(8.87115544199995,15.2,5.51859927599998));
#203515=CARTESIAN_POINT('Ctrl Pts',(8.87115544199995,11.6,5.51859927599998));
#203516=CARTESIAN_POINT('Ctrl Pts',(8.86983188899995,15.2,5.51802230299998));
#203517=CARTESIAN_POINT('Ctrl Pts',(8.86983188899995,11.6,5.51802230299998));
#203518=CARTESIAN_POINT('Ctrl Pts',(8.86851643699995,15.2,5.51744736599999));
#203519=CARTESIAN_POINT('Ctrl Pts',(8.86851643699995,11.6,5.51744736599999));
#203520=CARTESIAN_POINT('Ctrl Pts',(8.86720909899994,15.2,5.51687448799999));
#203521=CARTESIAN_POINT('Ctrl Pts',(8.86720909899994,11.6,5.51687448799999));
#203522=CARTESIAN_POINT('Ctrl Pts',(8.86590988599994,15.2,5.51630369099998));
#203523=CARTESIAN_POINT('Ctrl Pts',(8.86590988599994,11.6,5.51630369099998));
#203524=CARTESIAN_POINT('Ctrl Pts',(8.86461881499994,15.2,5.51573499599999));
#203525=CARTESIAN_POINT('Ctrl Pts',(8.86461881499994,11.6,5.51573499599999));
#203526=CARTESIAN_POINT('Ctrl Pts',(8.86333589499994,15.2,5.51516842399998));
#203527=CARTESIAN_POINT('Ctrl Pts',(8.86333589499994,11.6,5.51516842399998));
#203528=CARTESIAN_POINT('Ctrl Pts',(8.86206114199994,15.2,5.51460399899998));
#203529=CARTESIAN_POINT('Ctrl Pts',(8.86206114199994,11.6,5.51460399899998));
#203530=CARTESIAN_POINT('Ctrl Pts',(8.86079456699994,15.2,5.51404174299999));
#203531=CARTESIAN_POINT('Ctrl Pts',(8.86079456699994,11.6,5.51404174299999));
#203532=CARTESIAN_POINT('Ctrl Pts',(8.85953618399994,15.2,5.51348167599999));
#203533=CARTESIAN_POINT('Ctrl Pts',(8.85953618399994,11.6,5.51348167599999));
#203534=CARTESIAN_POINT('Ctrl Pts',(8.85828600699995,15.2,5.51292382299999));
#203535=CARTESIAN_POINT('Ctrl Pts',(8.85828600699995,11.6,5.51292382299999));
#203536=CARTESIAN_POINT('Ctrl Pts',(8.85704404899995,15.2,5.51236820399998));
#203537=CARTESIAN_POINT('Ctrl Pts',(8.85704404899995,11.6,5.51236820399998));
#203538=CARTESIAN_POINT('Ctrl Pts',(8.85581032199994,15.2,5.51181484299998));
#203539=CARTESIAN_POINT('Ctrl Pts',(8.85581032199994,11.6,5.51181484299998));
#203540=CARTESIAN_POINT('Ctrl Pts',(8.85458484099994,15.2,5.51126376199999));
#203541=CARTESIAN_POINT('Ctrl Pts',(8.85458484099994,11.6,5.51126376199999));
#203542=CARTESIAN_POINT('Ctrl Pts',(8.85336761799994,15.2,5.51071498499999));
#203543=CARTESIAN_POINT('Ctrl Pts',(8.85336761799994,11.6,5.51071498499999));
#203544=CARTESIAN_POINT('Ctrl Pts',(8.85215866799994,15.2,5.51016853299998));
#203545=CARTESIAN_POINT('Ctrl Pts',(8.85215866799994,11.6,5.51016853299998));
#203546=CARTESIAN_POINT('Ctrl Pts',(8.85095800299995,15.2,5.50962442999998));
#203547=CARTESIAN_POINT('Ctrl Pts',(8.85095800299995,11.6,5.50962442999998));
#203548=CARTESIAN_POINT('Ctrl Pts',(8.84976563899994,15.2,5.50908269999999));
#203549=CARTESIAN_POINT('Ctrl Pts',(8.84976563899994,11.6,5.50908269999999));
#203550=CARTESIAN_POINT('Ctrl Pts',(8.84858158699994,15.2,5.50854336299999));
#203551=CARTESIAN_POINT('Ctrl Pts',(8.84858158699994,11.6,5.50854336299999));
#203552=CARTESIAN_POINT('Ctrl Pts',(8.84740586099995,15.2,5.50800644699999));
#203553=CARTESIAN_POINT('Ctrl Pts',(8.84740586099995,11.6,5.50800644699999));
#203554=CARTESIAN_POINT('Ctrl Pts',(8.84623847599994,15.2,5.50747196999998));
#203555=CARTESIAN_POINT('Ctrl Pts',(8.84623847599994,11.6,5.50747196999998));
#203556=CARTESIAN_POINT('Ctrl Pts',(8.84507944399994,15.2,5.50693995899999));
#203557=CARTESIAN_POINT('Ctrl Pts',(8.84507944399994,11.6,5.50693995899999));
#203558=CARTESIAN_POINT('Ctrl Pts',(8.84392878099994,15.2,5.50641043699999));
#203559=CARTESIAN_POINT('Ctrl Pts',(8.84392878099994,11.6,5.50641043699999));
#203560=CARTESIAN_POINT('Ctrl Pts',(8.84278649899995,15.2,5.50588342799998));
#203561=CARTESIAN_POINT('Ctrl Pts',(8.84278649899995,11.6,5.50588342799998));
#203562=CARTESIAN_POINT('Ctrl Pts',(8.84165261299995,15.2,5.50535895499999));
#203563=CARTESIAN_POINT('Ctrl Pts',(8.84165261299995,11.6,5.50535895499999));
#203564=CARTESIAN_POINT('Ctrl Pts',(8.84052713599995,15.2,5.50483704199999));
#203565=CARTESIAN_POINT('Ctrl Pts',(8.84052713599995,11.6,5.50483704199999));
#203566=CARTESIAN_POINT('Ctrl Pts',(8.83941008399994,15.2,5.50431771299999));
#203567=CARTESIAN_POINT('Ctrl Pts',(8.83941008399994,11.6,5.50431771299999));
#203568=CARTESIAN_POINT('Ctrl Pts',(8.83830146799994,15.2,5.50380099199998));
#203569=CARTESIAN_POINT('Ctrl Pts',(8.83830146799994,11.6,5.50380099199998));
#203570=CARTESIAN_POINT('Ctrl Pts',(8.83720130399994,15.2,5.50328690399999));
#203571=CARTESIAN_POINT('Ctrl Pts',(8.83720130399994,11.6,5.50328690399999));
#203572=CARTESIAN_POINT('Ctrl Pts',(8.83610960699994,15.2,5.50277547399999));
#203573=CARTESIAN_POINT('Ctrl Pts',(8.83610960699994,11.6,5.50277547399999));
#203574=CARTESIAN_POINT('Ctrl Pts',(8.83502638899994,15.2,5.50226672399998));
#203575=CARTESIAN_POINT('Ctrl Pts',(8.83502638899994,11.6,5.50226672399998));
#203576=CARTESIAN_POINT('Ctrl Pts',(8.83395166499995,15.2,5.50176068099999));
#203577=CARTESIAN_POINT('Ctrl Pts',(8.83395166499995,11.6,5.50176068099999));
#203578=CARTESIAN_POINT('Ctrl Pts',(8.83288545099994,15.2,5.50125736999998));
#203579=CARTESIAN_POINT('Ctrl Pts',(8.83288545099994,11.6,5.50125736999998));
#203580=CARTESIAN_POINT('Ctrl Pts',(8.83182775899994,15.2,5.50075681399999));
#203581=CARTESIAN_POINT('Ctrl Pts',(8.83182775899994,11.6,5.50075681399999));
#203582=CARTESIAN_POINT('Ctrl Pts',(8.83077860499995,15.2,5.50025903799998));
#203583=CARTESIAN_POINT('Ctrl Pts',(8.83077860499995,11.6,5.50025903799998));
#203584=CARTESIAN_POINT('Ctrl Pts',(8.82973800299995,15.2,5.49976406899999));
#203585=CARTESIAN_POINT('Ctrl Pts',(8.82973800299995,11.6,5.49976406899999));
#203586=CARTESIAN_POINT('Ctrl Pts',(8.82870596699994,15.2,5.49927192999998));
#203587=CARTESIAN_POINT('Ctrl Pts',(8.82870596699994,11.6,5.49927192999998));
#203588=CARTESIAN_POINT('Ctrl Pts',(8.82768251199994,15.2,5.49878264899998));
#203589=CARTESIAN_POINT('Ctrl Pts',(8.82768251199994,11.6,5.49878264899998));
#203590=CARTESIAN_POINT('Ctrl Pts',(8.82666765299994,15.2,5.49829624999998));
#203591=CARTESIAN_POINT('Ctrl Pts',(8.82666765299994,11.6,5.49829624999998));
#203592=CARTESIAN_POINT('Ctrl Pts',(8.82566140499994,15.2,5.49781275799998));
#203593=CARTESIAN_POINT('Ctrl Pts',(8.82566140499994,11.6,5.49781275799998));
#203594=CARTESIAN_POINT('Ctrl Pts',(8.82466378099994,15.2,5.49733219899998));
#203595=CARTESIAN_POINT('Ctrl Pts',(8.82466378099994,11.6,5.49733219899998));
#203596=CARTESIAN_POINT('Ctrl Pts',(8.82367479799994,15.2,5.49685459999999));
#203597=CARTESIAN_POINT('Ctrl Pts',(8.82367479799994,11.6,5.49685459999999));
#203598=CARTESIAN_POINT('Ctrl Pts',(8.82269446899994,15.2,5.49637998599999));
#203599=CARTESIAN_POINT('Ctrl Pts',(8.82269446899994,11.6,5.49637998599999));
#203600=CARTESIAN_POINT('Ctrl Pts',(8.82172280999994,15.2,5.49590838499999));
#203601=CARTESIAN_POINT('Ctrl Pts',(8.82172280999994,11.6,5.49590838499999));
#203602=CARTESIAN_POINT('Ctrl Pts',(8.82075983499995,15.2,5.49543981999999));
#203603=CARTESIAN_POINT('Ctrl Pts',(8.82075983499995,11.6,5.49543981999999));
#203604=CARTESIAN_POINT('Ctrl Pts',(8.81980556099995,15.2,5.49497431899999));
#203605=CARTESIAN_POINT('Ctrl Pts',(8.81980556099995,11.6,5.49497431899999));
#203606=CARTESIAN_POINT('Ctrl Pts',(8.81886000299994,15.2,5.49451190899998));
#203607=CARTESIAN_POINT('Ctrl Pts',(8.81886000299994,11.6,5.49451190899998));
#203608=CARTESIAN_POINT('Ctrl Pts',(8.81792317299994,15.2,5.49405261699999));
#203609=CARTESIAN_POINT('Ctrl Pts',(8.81792317299994,11.6,5.49405261699999));
#203610=CARTESIAN_POINT('Ctrl Pts',(8.81699508899995,15.2,5.49359646799999));
#203611=CARTESIAN_POINT('Ctrl Pts',(8.81699508899995,11.6,5.49359646799999));
#203612=CARTESIAN_POINT('Ctrl Pts',(8.81607576599994,15.2,5.49314348999999));
#203613=CARTESIAN_POINT('Ctrl Pts',(8.81607576599994,11.6,5.49314348999999));
#203614=CARTESIAN_POINT('Ctrl Pts',(8.81516521899994,15.2,5.49269370999999));
#203615=CARTESIAN_POINT('Ctrl Pts',(8.81516521899994,11.6,5.49269370999999));
#203616=CARTESIAN_POINT('Ctrl Pts',(8.81426346299994,15.2,5.49224715599999));
#203617=CARTESIAN_POINT('Ctrl Pts',(8.81426346299994,11.6,5.49224715599999));
#203618=CARTESIAN_POINT('Ctrl Pts',(8.81337051299995,15.2,5.49180385399998));
#203619=CARTESIAN_POINT('Ctrl Pts',(8.81337051299995,11.6,5.49180385399998));
#203620=CARTESIAN_POINT('Ctrl Pts',(8.81248638699994,15.2,5.49136383299999));
#203621=CARTESIAN_POINT('Ctrl Pts',(8.81248638699994,11.6,5.49136383299999));
#203622=CARTESIAN_POINT('Ctrl Pts',(8.81161109899994,15.2,5.49092711899998));
#203623=CARTESIAN_POINT('Ctrl Pts',(8.81161109899994,11.6,5.49092711899998));
#203624=CARTESIAN_POINT('Ctrl Pts',(8.81074466299994,15.2,5.49049374099998));
#203625=CARTESIAN_POINT('Ctrl Pts',(8.81074466299994,11.6,5.49049374099998));
#203626=CARTESIAN_POINT('Ctrl Pts',(8.80988709799994,15.2,5.49006372699999));
#203627=CARTESIAN_POINT('Ctrl Pts',(8.80988709799994,11.6,5.49006372699999));
#203628=CARTESIAN_POINT('Ctrl Pts',(8.80903841799995,15.2,5.48963710299999));
#203629=CARTESIAN_POINT('Ctrl Pts',(8.80903841799995,11.6,5.48963710299999));
#203630=CARTESIAN_POINT('Ctrl Pts',(8.80819863999994,15.2,5.48921389999999));
#203631=CARTESIAN_POINT('Ctrl Pts',(8.80819863999994,11.6,5.48921389999999));
#203632=CARTESIAN_POINT('Ctrl Pts',(8.80736777699994,15.2,5.48879414499999));
#203633=CARTESIAN_POINT('Ctrl Pts',(8.80736777699994,11.6,5.48879414499999));
#203634=CARTESIAN_POINT('Ctrl Pts',(8.80655058299994,15.2,5.48838026399999));
#203635=CARTESIAN_POINT('Ctrl Pts',(8.80655058299994,11.6,5.48838026399999));
#203636=CARTESIAN_POINT('Ctrl Pts',(8.80590482999994,15.2,5.48805240199999));
#203637=CARTESIAN_POINT('Ctrl Pts',(8.80590482999994,11.6,5.48805240199999));
#203638=CARTESIAN_POINT('Ctrl Pts',(8.80542564399994,15.2,5.48780866099998));
#203639=CARTESIAN_POINT('Ctrl Pts',(8.80542564399994,11.6,5.48780866099998));
#203640=CARTESIAN_POINT('Ctrl Pts',(8.80510947799995,15.2,5.48764764399999));
#203641=CARTESIAN_POINT('Ctrl Pts',(8.80510947799995,11.6,5.48764764399999));
#203642=CARTESIAN_POINT('Ctrl Pts',(8.80495412799995,15.2,5.48756847999999));
#203643=CARTESIAN_POINT('Ctrl Pts',(8.80495412799995,11.6,5.48756847999999));
#203644=CARTESIAN_POINT('',(8.80495412746567,12.2,5.48756847941583));
#203645=CARTESIAN_POINT('',(8.80495412746567,15.2,5.48756847941583));
#203646=CARTESIAN_POINT('',(8.80495412699995,12.2,5.48756847899998));
#203647=CARTESIAN_POINT('Ctrl Pts',(9.95917514599994,12.2,5.75020264099999));
#203648=CARTESIAN_POINT('Ctrl Pts',(9.95536157030715,12.2,5.74993548595142));
#203649=CARTESIAN_POINT('Ctrl Pts',(9.95155489341636,12.2,5.74966449046052));
#203650=CARTESIAN_POINT('Ctrl Pts',(9.94775512114579,12.2,5.74938964953395));
#203651=CARTESIAN_POINT('Ctrl Pts',(9.94395534887523,12.2,5.74911480860738));
#203652=CARTESIAN_POINT('Ctrl Pts',(9.94016247816818,12.2,5.74883612260804));
#203653=CARTESIAN_POINT('Ctrl Pts',(9.93637652394912,12.2,5.7485536050213));
#203654=CARTESIAN_POINT('Ctrl Pts',(9.93259056973007,12.2,5.74827108743457));
#203655=CARTESIAN_POINT('Ctrl Pts',(9.92881153168612,12.2,5.74798473883553));
#203656=CARTESIAN_POINT('Ctrl Pts',(9.92503944240555,12.2,5.74769458655493));
#203657=CARTESIAN_POINT('Ctrl Pts',(9.92126735243973,12.2,5.74740443422161));
#203658=CARTESIAN_POINT('Ctrl Pts',(9.9175022111092,12.2,5.74711048106222));
#203659=CARTESIAN_POINT('Ctrl Pts',(9.91374405518896,12.2,5.74681275914344));
#203660=CARTESIAN_POINT('Ctrl Pts',(9.90998589995145,12.2,5.74651503727874));
#203661=CARTESIAN_POINT('Ctrl Pts',(9.90623472967193,12.2,5.74621354825591));
#203662=CARTESIAN_POINT('Ctrl Pts',(9.90249057380857,12.2,5.74590831722501));
#203663=CARTESIAN_POINT('Ctrl Pts',(9.89874641794522,12.2,5.74560308619412));
#203664=CARTESIAN_POINT('Ctrl Pts',(9.89500927564456,12.2,5.7452941130898));
#203665=CARTESIAN_POINT('Ctrl Pts',(9.89127917472151,12.2,5.74498142451639));
#203666=CARTESIAN_POINT('Ctrl Pts',(9.88754907379846,12.2,5.74466873594298));
#203667=CARTESIAN_POINT('Ctrl Pts',(9.88382601290183,12.2,5.74435232967344));
#203668=CARTESIAN_POINT('Ctrl Pts',(9.88011002451994,12.2,5.7440322367253));
#203669=CARTESIAN_POINT('Ctrl Pts',(9.87639403613804,12.2,5.74371214377716));
#203670=CARTESIAN_POINT('Ctrl Pts',(9.8726851189363,12.2,5.74338836367343));
#203671=CARTESIAN_POINT('Ctrl Pts',(9.86898330415351,12.2,5.74306092472731));
#203672=CARTESIAN_POINT('Ctrl Pts',(9.86528148937072,12.2,5.74273348578119));
#203673=CARTESIAN_POINT('Ctrl Pts',(9.86158677765411,12.2,5.74240238867699));
#203674=CARTESIAN_POINT('Ctrl Pts',(9.85789919832879,12.2,5.74206766206465));
#203675=CARTESIAN_POINT('Ctrl Pts',(9.85421161833356,12.2,5.7417329353915));
#203676=CARTESIAN_POINT('Ctrl Pts',(9.850531170632,12.2,5.74139457709232));
#203677=CARTESIAN_POINT('Ctrl Pts',(9.84685788472413,12.2,5.7410526184588));
#203678=CARTESIAN_POINT('Ctrl Pts',(9.84196017129248,12.2,5.74059667371764));
#203679=CARTESIAN_POINT('Ctrl Pts',(9.83707519084653,12.2,5.74013432515579));
#203680=CARTESIAN_POINT('Ctrl Pts',(9.83220301527822,12.2,5.73966564202533));
#203681=CARTESIAN_POINT('Ctrl Pts',(9.82854888343602,12.2,5.73931412966153));
#203682=CARTESIAN_POINT('Ctrl Pts',(9.82490195449846,12.2,5.73895905544237));
#203683=CARTESIAN_POINT('Ctrl Pts',(9.82126225867174,12.2,5.73860044703904));
#203684=CARTESIAN_POINT('Ctrl Pts',(9.81762256284502,12.2,5.73824183863572));
#203685=CARTESIAN_POINT('Ctrl Pts',(9.8139901001428,12.2,5.73787969644929));
#203686=CARTESIAN_POINT('Ctrl Pts',(9.81036490085686,12.2,5.73751405008805));
#203687=CARTESIAN_POINT('Ctrl Pts',(9.80553130136988,12.2,5.73702652156212));
#203688=CARTESIAN_POINT('Ctrl Pts',(9.8007106147221,12.2,5.73653276425977));
#203689=CARTESIAN_POINT('Ctrl Pts',(9.79590291327162,12.2,5.736032847508));
#203690=CARTESIAN_POINT('Ctrl Pts',(9.79229713751129,12.2,5.73565790997824));
#203691=CARTESIAN_POINT('Ctrl Pts',(9.78869866678903,12.2,5.73527950700487));
#203692=CARTESIAN_POINT('Ctrl Pts',(9.78510753048649,12.2,5.73489767051702));
#203693=CARTESIAN_POINT('Ctrl Pts',(9.78151639418396,12.2,5.73451583402918));
#203694=CARTESIAN_POINT('Ctrl Pts',(9.77793259172721,12.2,5.73413056244457));
#203695=CARTESIAN_POINT('Ctrl Pts',(9.77435615635651,12.2,5.73374188700065));
#203696=CARTESIAN_POINT('Ctrl Pts',(9.76958757542909,12.2,5.73322365302836));
#203697=CARTESIAN_POINT('Ctrl Pts',(9.76483208820603,12.2,5.73269936653867));
#203698=CARTESIAN_POINT('Ctrl Pts',(9.76008976933733,12.2,5.7321691012316));
#203699=CARTESIAN_POINT('Ctrl Pts',(9.75653303050887,12.2,5.73177140228743));
#203700=CARTESIAN_POINT('Ctrl Pts',(9.75298369903787,12.2,5.73137033990198));
#203701=CARTESIAN_POINT('Ctrl Pts',(9.74944180429156,12.2,5.73096594450001));
#203702=CARTESIAN_POINT('Ctrl Pts',(9.74589990954524,12.2,5.73056154909804));
#203703=CARTESIAN_POINT('Ctrl Pts',(9.74236545327363,12.2,5.73015382072953));
#203704=CARTESIAN_POINT('Ctrl Pts',(9.73883846590113,12.2,5.72974279078642));
#203705=CARTESIAN_POINT('Ctrl Pts',(9.73531147852862,12.2,5.72933176084331));
#203706=CARTESIAN_POINT('Ctrl Pts',(9.7317919588615,12.2,5.72891742858608));
#203707=CARTESIAN_POINT('Ctrl Pts',(9.72827994022945,12.2,5.72849982708077));
#203708=CARTESIAN_POINT('Ctrl Pts',(9.7247679215974,12.2,5.72808222557546));
#203709=CARTESIAN_POINT('Ctrl Pts',(9.72126340065288,12.2,5.72766135347661));
#203710=CARTESIAN_POINT('Ctrl Pts',(9.71776641323724,12.2,5.72723724211746));
#203711=CARTESIAN_POINT('Ctrl Pts',(9.71426942518632,12.2,5.72681313068126));
#203712=CARTESIAN_POINT('Ctrl Pts',(9.71077996797918,12.2,5.72638578060249));
#203713=CARTESIAN_POINT('Ctrl Pts',(9.70729807351585,12.2,5.72595522362281));
#203714=CARTESIAN_POINT('Ctrl Pts',(9.70381617968505,12.2,5.72552466672135));
#203715=CARTESIAN_POINT('Ctrl Pts',(9.70034184842886,12.2,5.72509090262006));
#203716=CARTESIAN_POINT('Ctrl Pts',(9.69687511113881,12.2,5.72465396371899));
#203717=CARTESIAN_POINT('Ctrl Pts',(9.69225279496202,12.2,5.72407137854403));
#203718=CARTESIAN_POINT('Ctrl Pts',(9.68764397794407,12.2,5.72348314911955));
#203719=CARTESIAN_POINT('Ctrl Pts',(9.68304873686676,12.2,5.72288935186114));
#203720=CARTESIAN_POINT('Ctrl Pts',(9.67960230590225,12.2,5.7224440038971));
#203721=CARTESIAN_POINT('Ctrl Pts',(9.67616351202427,12.2,5.72199552279828));
#203722=CARTESIAN_POINT('Ctrl Pts',(9.67273238473122,12.2,5.72154394381512));
#203723=CARTESIAN_POINT('Ctrl Pts',(9.66930125681485,12.2,5.72109236474991));
#203724=CARTESIAN_POINT('Ctrl Pts',(9.66587779631731,12.2,5.72063768543383));
#203725=CARTESIAN_POINT('Ctrl Pts',(9.66246203628026,12.2,5.72017994090855));
#203726=CARTESIAN_POINT('Ctrl Pts',(9.65904627686376,12.2,5.71972219646643));
#203727=CARTESIAN_POINT('Ctrl Pts',(9.65563821543851,12.2,5.71926138599948));
#203728=CARTESIAN_POINT('Ctrl Pts',(9.65223788614605,12.2,5.7187975412244));
#203729=CARTESIAN_POINT('Ctrl Pts',(9.6488375568536,12.2,5.71833369644932));
#203730=CARTESIAN_POINT('Ctrl Pts',(9.64544495920584,12.2,5.71786681911798));
#203731=CARTESIAN_POINT('Ctrl Pts',(9.64206012398015,12.2,5.71739694221625));
#203732=CARTESIAN_POINT('Ctrl Pts',(9.63867528875446,12.2,5.71692706531451));
#203733=CARTESIAN_POINT('Ctrl Pts',(9.63529821729588,12.2,5.71645418761863));
#203734=CARTESIAN_POINT('Ctrl Pts',(9.63192894102795,12.2,5.71597834475877));
#203735=CARTESIAN_POINT('Ctrl Pts',(9.62855966476003,12.2,5.71550250189891));
#203736=CARTESIAN_POINT('Ctrl Pts',(9.6251981838444,12.2,5.71502369380138));
#203737=CARTESIAN_POINT('Ctrl Pts',(9.62184453009057,12.2,5.71454195252747));
#203738=CARTESIAN_POINT('Ctrl Pts',(9.61849087633673,12.2,5.71406021125356));
#203739=CARTESIAN_POINT('Ctrl Pts',(9.61514505005736,12.2,5.71357553850485));
#203740=CARTESIAN_POINT('Ctrl Pts',(9.61180708371924,12.2,5.71308796810629));
#203741=CARTESIAN_POINT('Ctrl Pts',(9.60735646153079,12.2,5.7124378741825));
#203742=CARTESIAN_POINT('Ctrl Pts',(9.60291981226906,12.2,5.71178262884134));
#203743=CARTESIAN_POINT('Ctrl Pts',(9.59849721223022,12.2,5.71112231252456));
#203744=CARTESIAN_POINT('Ctrl Pts',(9.59518026250237,12.2,5.71062707533195));
#203745=CARTESIAN_POINT('Ctrl Pts',(9.59187121578131,12.2,5.71012898773453));
#203746=CARTESIAN_POINT('Ctrl Pts',(9.58857010451123,12.2,5.70962808250046));
#203747=CARTESIAN_POINT('Ctrl Pts',(9.58416862241797,12.2,5.70896020879438));
#203748=CARTESIAN_POINT('Ctrl Pts',(9.57978124755788,12.2,5.70828732780163));
#203749=CARTESIAN_POINT('Ctrl Pts',(9.57540805804321,12.2,5.70760952259752));
#203750=CARTESIAN_POINT('Ctrl Pts',(9.57103486912439,12.2,5.70693171748576));
#203751=CARTESIAN_POINT('Ctrl Pts',(9.56667586506485,12.2,5.70624898797464));
#203752=CARTESIAN_POINT('Ctrl Pts',(9.56233112236354,12.2,5.70556141953117));
#203753=CARTESIAN_POINT('Ctrl Pts',(9.55798637907026,12.2,5.70487385099401));
#203754=CARTESIAN_POINT('Ctrl Pts',(9.55365589875662,12.2,5.70418144173039));
#203755=CARTESIAN_POINT('Ctrl Pts',(9.54933975964033,12.2,5.70348427915715));
#203756=CARTESIAN_POINT('Ctrl Pts',(9.54502362111214,12.2,5.70278711667889));
#203757=CARTESIAN_POINT('Ctrl Pts',(9.54072182159263,12.2,5.70208519899132));
#203758=CARTESIAN_POINT('Ctrl Pts',(9.53643444210885,12.2,5.70137861454939));
#203759=CARTESIAN_POINT('Ctrl Pts',(9.53107521731601,12.2,5.70049538392476));
#203760=CARTESIAN_POINT('Ctrl Pts',(9.52573852258208,12.2,5.69960485878607));
#203761=CARTESIAN_POINT('Ctrl Pts',(9.52042451112256,12.2,5.69870721080033));
#203762=CARTESIAN_POINT('Ctrl Pts',(9.51617330172327,12.2,5.69798909237261));
#203763=CARTESIAN_POINT('Ctrl Pts',(9.51193660998819,12.2,5.69726641640414));
#203764=CARTESIAN_POINT('Ctrl Pts',(9.50771451443732,12.2,5.69653926866113));
#203765=CARTESIAN_POINT('Ctrl Pts',(9.5034924194617,12.2,5.6958121210172));
#203766=CARTESIAN_POINT('Ctrl Pts',(9.49928492198987,12.2,5.6950805036469));
#203767=CARTESIAN_POINT('Ctrl Pts',(9.49509210110946,12.2,5.69434450531846));
#203768=CARTESIAN_POINT('Ctrl Pts',(9.49089927965777,12.2,5.69360850688974));
#203769=CARTESIAN_POINT('Ctrl Pts',(9.48672113442726,12.2,5.69286812822716));
#203770=CARTESIAN_POINT('Ctrl Pts',(9.48255774570133,12.2,5.69212345913075));
#203771=CARTESIAN_POINT('Ctrl Pts',(9.47839435754265,12.2,5.69137879013579));
#203772=CARTESIAN_POINT('Ctrl Pts',(9.47424572562801,12.2,5.69062983073218));
#203773=CARTESIAN_POINT('Ctrl Pts',(9.47011193059148,12.2,5.6898766723676));
#203774=CARTESIAN_POINT('Ctrl Pts',(9.46597813499171,12.2,5.6891235139004));
#203775=CARTESIAN_POINT('Ctrl Pts',(9.46185917683167,12.2,5.68836615697948));
#203776=CARTESIAN_POINT('Ctrl Pts',(9.45775513616452,12.2,5.68760469393771));
#203777=CARTESIAN_POINT('Ctrl Pts',(9.45365109605656,12.2,5.6868432309997));
#203778=CARTESIAN_POINT('Ctrl Pts',(9.44956197340949,12.2,5.68607766065973));
#203779=CARTESIAN_POINT('Ctrl Pts',(9.44548784990768,12.2,5.68530807833416));
#203780=CARTESIAN_POINT('Ctrl Pts',(9.44141372585077,12.2,5.68453849590374));
#203781=CARTESIAN_POINT('Ctrl Pts',(9.4373546011664,12.2,5.6837649017315));
#203782=CARTESIAN_POINT('Ctrl Pts',(9.4333105565388,12.2,5.68298738874114));
#203783=CARTESIAN_POINT('Ctrl Pts',(9.4282555010298,12.2,5.68201549755615));
#203784=CARTESIAN_POINT('Ctrl Pts',(9.4232240085935,12.2,5.68103748499148));
#203785=CARTESIAN_POINT('Ctrl Pts',(9.41821624116419,12.2,5.68005353714395));
#203786=CARTESIAN_POINT('Ctrl Pts',(9.41421002754824,12.2,5.67926637893027));
#203787=CARTESIAN_POINT('Ctrl Pts',(9.41021899705703,12.2,5.67847542268402));
#203788=CARTESIAN_POINT('Ctrl Pts',(9.40624323165826,12.2,5.67768076513826));
#203789=CARTESIAN_POINT('Ctrl Pts',(9.4022674657178,12.2,5.67688610748422));
#203790=CARTESIAN_POINT('Ctrl Pts',(9.39830696647322,12.2,5.6760877487437));
#203791=CARTESIAN_POINT('Ctrl Pts',(9.39436181575821,12.2,5.6752857877));
#203792=CARTESIAN_POINT('Ctrl Pts',(9.3904166650432,12.2,5.6744838266563));
#203793=CARTESIAN_POINT('Ctrl Pts',(9.38648686298276,12.2,5.67367826286216));
#203794=CARTESIAN_POINT('Ctrl Pts',(9.38257249365989,12.2,5.67286919515105));
#203795=CARTESIAN_POINT('Ctrl Pts',(9.37572234814487,12.2,5.67145332682194));
#203796=CARTESIAN_POINT('Ctrl Pts',(9.36891946199662,12.2,5.6700267271161));
#203797=CARTESIAN_POINT('Ctrl Pts',(9.36216429004059,12.2,5.66858994152542));
#203798=CARTESIAN_POINT('Ctrl Pts',(9.3583041913292,12.2,5.667768921092));
#203799=CARTESIAN_POINT('Ctrl Pts',(9.35445967150579,12.2,5.66694457273319));
#203800=CARTESIAN_POINT('Ctrl Pts',(9.35063081618702,12.2,5.66611700046565));
#203801=CARTESIAN_POINT('Ctrl Pts',(9.34680196138996,12.2,5.66528942831087));
#203802=CARTESIAN_POINT('Ctrl Pts',(9.34298877087331,12.2,5.66445863320254));
#203803=CARTESIAN_POINT('Ctrl Pts',(9.339191329826,12.2,5.66362471639599));
#203804=CARTESIAN_POINT('Ctrl Pts',(9.3353938882613,12.2,5.66279079947581));
#203805=CARTESIAN_POINT('Ctrl Pts',(9.33161219490472,12.2,5.66195376284672));
#203806=CARTESIAN_POINT('Ctrl Pts',(9.32784633820051,12.2,5.66111371118963));
#203807=CARTESIAN_POINT('Ctrl Pts',(9.32408048200939,12.2,5.660273659647));
#203808=CARTESIAN_POINT('Ctrl Pts',(9.32033046026789,12.2,5.65943059232441));
#203809=CARTESIAN_POINT('Ctrl Pts',(9.31659636012708,12.2,5.65858461617164));
#203810=CARTESIAN_POINT('Ctrl Pts',(9.3128622594775,12.2,5.65773863990361));
#203811=CARTESIAN_POINT('Ctrl Pts',(9.30914408084367,12.2,5.65688975419971));
#203812=CARTESIAN_POINT('Ctrl Pts',(9.30544190951403,12.2,5.65603806848275));
#203813=CARTESIAN_POINT('Ctrl Pts',(9.30173973868881,12.2,5.65518638288183));
#203814=CARTESIAN_POINT('Ctrl Pts',(9.298053574846,12.2,5.65433189435868));
#203815=CARTESIAN_POINT('Ctrl Pts',(9.29438350736661,12.2,5.65347471487348));
#203816=CARTESIAN_POINT('Ctrl Pts',(9.29071343938716,12.2,5.65261753527149));
#203817=CARTESIAN_POINT('Ctrl Pts',(9.28705946671757,12.2,5.65175766253311));
#203818=CARTESIAN_POINT('Ctrl Pts',(9.28342167624154,12.2,5.65089520820833));
#203819=CARTESIAN_POINT('Ctrl Pts',(9.27978388576551,12.2,5.65003275388355));
#203820=CARTESIAN_POINT('Ctrl Pts',(9.27616227909968,12.2,5.64916771632514));
#203821=CARTESIAN_POINT('Ctrl Pts',(9.27255694312709,12.2,5.64830020933315));
#203822=CARTESIAN_POINT('Ctrl Pts',(9.26895160764571,12.2,5.64743270245938));
#203823=CARTESIAN_POINT('Ctrl Pts',(9.26536254347652,12.2,5.64656272414433));
#203824=CARTESIAN_POINT('Ctrl Pts',(9.26178983875232,12.2,5.64569038876726));
#203825=CARTESIAN_POINT('Ctrl Pts',(9.25821713354134,12.2,5.64481805327132));
#203826=CARTESIAN_POINT('Ctrl Pts',(9.25466078857625,12.2,5.64394335914075));
#203827=CARTESIAN_POINT('Ctrl Pts',(9.25112089266278,12.2,5.64306642281494));
#203828=CARTESIAN_POINT('Ctrl Pts',(9.24758099723162,12.2,5.64218948660863));
#203829=CARTESIAN_POINT('Ctrl Pts',(9.24405755161222,12.2,5.64131030594984));
#203830=CARTESIAN_POINT('Ctrl Pts',(9.24055064478673,12.2,5.64042899802202));
#203831=CARTESIAN_POINT('Ctrl Pts',(9.23704373748341,12.2,5.63954768997413));
#203832=CARTESIAN_POINT('Ctrl Pts',(9.2335533684712,12.2,5.63866425569749));
#203833=CARTESIAN_POINT('Ctrl Pts',(9.2300796297209,12.2,5.63777880960483));
#203834=CARTESIAN_POINT('Ctrl Pts',(9.22660589144391,12.2,5.63689336363281));
#203835=CARTESIAN_POINT('Ctrl Pts',(9.22314878251223,12.2,5.63600590858041));
#203836=CARTESIAN_POINT('Ctrl Pts',(9.21970839501462,12.2,5.63511656059768));
#203837=CARTESIAN_POINT('Ctrl Pts',(9.21626800704825,12.2,5.63422721249378));
#203838=CARTESIAN_POINT('Ctrl Pts',(9.21284433903388,12.2,5.63333597352575));
#203839=CARTESIAN_POINT('Ctrl Pts',(9.2094374837382,12.2,5.63244296214364));
#203840=CARTESIAN_POINT('Ctrl Pts',(9.20603062890669,12.2,5.6315499508832));
#203841=CARTESIAN_POINT('Ctrl Pts',(9.20264058651422,12.2,5.63065516924586));
#203842=CARTESIAN_POINT('Ctrl Pts',(9.1992674482311,12.2,5.6297587371634));
#203843=CARTESIAN_POINT('Ctrl Pts',(9.19589430948839,12.2,5.62886230495879));
#203844=CARTESIAN_POINT('Ctrl Pts',(9.19253807474126,12.2,5.627964222245));
#203845=CARTESIAN_POINT('Ctrl Pts',(9.18919883822704,12.2,5.6270646129181));
#203846=CARTESIAN_POINT('Ctrl Pts',(9.1858596021678,12.2,5.62616500371376));
#203847=CARTESIAN_POINT('Ctrl Pts',(9.18253736329961,12.2,5.62526386897085));
#203848=CARTESIAN_POINT('Ctrl Pts',(9.17923221579028,12.2,5.62436133165589));
#203849=CARTESIAN_POINT('Ctrl Pts',(9.17592706783062,12.2,5.62345879421795));
#203850=CARTESIAN_POINT('Ctrl Pts',(9.17263901013793,12.2,5.62255485438337));
#203851=CARTESIAN_POINT('Ctrl Pts',(9.16936813822266,12.2,5.62164964027437));
#203852=CARTESIAN_POINT('Ctrl Pts',(9.16609726675304,12.2,5.62074442628871));
#203853=CARTESIAN_POINT('Ctrl Pts',(9.16284357892735,12.2,5.6198379364574));
#203854=CARTESIAN_POINT('Ctrl Pts',(9.15960717274571,12.2,5.61893029986506));
#203855=CARTESIAN_POINT('Ctrl Pts',(9.15637076612311,12.2,5.61802266314904));
#203856=CARTESIAN_POINT('Ctrl Pts',(9.15315163805771,12.2,5.6171138789468));
#203857=CARTESIAN_POINT('Ctrl Pts',(9.14994988621654,12.2,5.61620407750832));
#203858=CARTESIAN_POINT('Ctrl Pts',(9.14594769663319,12.2,5.61506682577221));
#203859=CARTESIAN_POINT('Ctrl Pts',(9.14197265678225,12.2,5.61392798380454));
#203860=CARTESIAN_POINT('Ctrl Pts',(9.1380249530144,12.2,5.6127878090077));
#203861=CARTESIAN_POINT('Ctrl Pts',(9.13407724924654,12.2,5.61164763421084));
#203862=CARTESIAN_POINT('Ctrl Pts',(9.13015688206068,12.2,5.61050612765309));
#203863=CARTESIAN_POINT('Ctrl Pts',(9.12626404247878,12.2,5.60936354945859));
#203864=CARTESIAN_POINT('Ctrl Pts',(9.1223712028969,12.2,5.60822097126409));
#203865=CARTESIAN_POINT('Ctrl Pts',(9.11850589013095,12.2,5.60707732170295));
#203866=CARTESIAN_POINT('Ctrl Pts',(9.11466829554906,12.2,5.60593286767514));
#203867=CARTESIAN_POINT('Ctrl Pts',(9.11083070096718,12.2,5.60478841364731));
#203868=CARTESIAN_POINT('Ctrl Pts',(9.10702082514568,12.2,5.60364315416952));
#203869=CARTESIAN_POINT('Ctrl Pts',(9.10323886049437,12.2,5.60249736014171));
#203870=CARTESIAN_POINT('Ctrl Pts',(9.09945689584305,12.2,5.60135156611392));
#203871=CARTESIAN_POINT('Ctrl Pts',(9.09570284265165,12.2,5.60020523661863));
#203872=CARTESIAN_POINT('Ctrl Pts',(9.09197689705078,12.2,5.59905864836688));
#203873=CARTESIAN_POINT('Ctrl Pts',(9.08825095144993,12.2,5.59791206011514));
#203874=CARTESIAN_POINT('Ctrl Pts',(9.08455311190092,12.2,5.59676521199998));
#203875=CARTESIAN_POINT('Ctrl Pts',(9.08088357731991,12.2,5.59561838387498));
#203876=CARTESIAN_POINT('Ctrl Pts',(9.07721404273889,12.2,5.59447155574998));
#203877=CARTESIAN_POINT('Ctrl Pts',(9.07357281155278,12.2,5.59332474893888));
#203878=CARTESIAN_POINT('Ctrl Pts',(9.06996008377734,12.2,5.59217824588336));
#203879=CARTESIAN_POINT('Ctrl Pts',(9.06634735639569,12.2,5.5910317429528));
#203880=CARTESIAN_POINT('Ctrl Pts',(9.06276313291307,12.2,5.5898855446639));
#203881=CARTESIAN_POINT('Ctrl Pts',(9.05920761371494,12.2,5.58873994089983));
#203882=CARTESIAN_POINT('Ctrl Pts',(9.05565209412926,12.2,5.58759433701089));
#203883=CARTESIAN_POINT('Ctrl Pts',(9.05212527844311,12.2,5.58644932835526));
#203884=CARTESIAN_POINT('Ctrl Pts',(9.04862737073241,12.2,5.58530520863297));
#203885=CARTESIAN_POINT('Ctrl Pts',(9.04512946302171,12.2,5.58416108891067));
#203886=CARTESIAN_POINT('Ctrl Pts',(9.04166046351206,12.2,5.5830178590008));
#203887=CARTESIAN_POINT('Ctrl Pts',(9.03822057715763,12.2,5.58187581762423));
#203888=CARTESIAN_POINT('Ctrl Pts',(9.03478069080321,12.2,5.58073377624764));
#203889=CARTESIAN_POINT('Ctrl Pts',(9.03136991818942,12.2,5.57959292436904));
#203890=CARTESIAN_POINT('Ctrl Pts',(9.02798846547953,12.2,5.57845356804951));
#203891=CARTESIAN_POINT('Ctrl Pts',(9.02460701276966,12.2,5.57731421172998));
#203892=CARTESIAN_POINT('Ctrl Pts',(9.02125488303,12.2,5.5761763502966));
#203893=CARTESIAN_POINT('Ctrl Pts',(9.01793228275068,12.2,5.57504029411596));
#203894=CARTESIAN_POINT('Ctrl Pts',(9.01460968247136,12.2,5.57390423793531));
#203895=CARTESIAN_POINT('Ctrl Pts',(9.01131661419989,12.2,5.57276998773909));
#203896=CARTESIAN_POINT('Ctrl Pts',(9.00805328751832,12.2,5.57163786148393));
#203897=CARTESIAN_POINT('Ctrl Pts',(9.00478996083673,12.2,5.57050573522879));
#203898=CARTESIAN_POINT('Ctrl Pts',(9.00155638011096,12.2,5.56937572988331));
#203899=CARTESIAN_POINT('Ctrl Pts',(8.99835275649986,12.2,5.56824817196664));
#203900=CARTESIAN_POINT('Ctrl Pts',(8.99514913288876,12.2,5.56712061404998));
#203901=CARTESIAN_POINT('Ctrl Pts',(8.99197546674013,12.2,5.56599550044891));
#203902=CARTESIAN_POINT('Ctrl Pts',(8.98883197728149,12.2,5.5648731618327));
#203903=CARTESIAN_POINT('Ctrl Pts',(8.98505979006818,12.2,5.56352635554219));
#203904=CARTESIAN_POINT('Ctrl Pts',(8.98133105502724,12.2,5.5621835438745));
#203905=CARTESIAN_POINT('Ctrl Pts',(8.97764615390921,12.2,5.5608453065896));
#203906=CARTESIAN_POINT('Ctrl Pts',(8.97396125245647,12.2,5.55950706918311));
#203907=CARTESIAN_POINT('Ctrl Pts',(8.97032018441751,12.2,5.55817340797722));
#203908=CARTESIAN_POINT('Ctrl Pts',(8.96672333689116,12.2,5.55684491290517));
#203909=CARTESIAN_POINT('Ctrl Pts',(8.96312648969154,12.2,5.5555164179538));
#203910=CARTESIAN_POINT('Ctrl Pts',(8.95957386137946,12.2,5.55419309196341));
#203911=CARTESIAN_POINT('Ctrl Pts',(8.9560658453422,12.2,5.5528755416782));
#203912=CARTESIAN_POINT('Ctrl Pts',(8.95255782930494,12.2,5.55155799139299));
#203913=CARTESIAN_POINT('Ctrl Pts',(8.94909442563911,12.2,5.55024621683233));
#203914=CARTESIAN_POINT('Ctrl Pts',(8.94567603167802,12.2,5.54894083879614));
#203915=CARTESIAN_POINT('Ctrl Pts',(8.94225763771692,12.2,5.54763546075995));
#203916=CARTESIAN_POINT('Ctrl Pts',(8.93888425458646,12.2,5.546336481111));
#203917=CARTESIAN_POINT('Ctrl Pts',(8.93555628562096,12.2,5.54504453415747));
#203918=CARTESIAN_POINT('Ctrl Pts',(8.93222831635318,12.2,5.54375258708658));
#203919=CARTESIAN_POINT('Ctrl Pts',(8.92894576262307,12.2,5.54246767517467));
#203920=CARTESIAN_POINT('Ctrl Pts',(8.92570903353199,12.2,5.54119044918873));
#203921=CARTESIAN_POINT('Ctrl Pts',(8.92247230473491,12.2,5.5399132233188));
#203922=CARTESIAN_POINT('Ctrl Pts',(8.91928140288474,12.2,5.53864368333546));
#203923=CARTESIAN_POINT('Ctrl Pts',(8.91613674498463,12.2,5.53738249845888));
#203924=CARTESIAN_POINT('Ctrl Pts',(8.91299208708452,12.2,5.53612131358229));
#203925=CARTESIAN_POINT('Ctrl Pts',(8.9098936718165,12.2,5.53486848372431));
#203926=CARTESIAN_POINT('Ctrl Pts',(8.90684192784084,12.2,5.53362469310221));
#203927=CARTESIAN_POINT('Ctrl Pts',(8.90379018358799,12.2,5.53238090236713));
#203928=CARTESIAN_POINT('Ctrl Pts',(8.90078510847299,12.2,5.53114615289958));
#203929=CARTESIAN_POINT('Ctrl Pts',(8.89782713356385,12.2,5.52992114516658));
#203930=CARTESIAN_POINT('Ctrl Pts',(8.89486915892338,12.2,5.52869613754485));
#203931=CARTESIAN_POINT('Ctrl Pts',(8.89195828905192,12.2,5.5274808726289));
#203932=CARTESIAN_POINT('Ctrl Pts',(8.88909496022617,12.2,5.52627607200052));
#203933=CARTESIAN_POINT('Ctrl Pts',(8.88623163140042,12.2,5.52507127137212));
#203934=CARTESIAN_POINT('Ctrl Pts',(8.8834158451876,12.2,5.52387693257005));
#203935=CARTESIAN_POINT('Ctrl Pts',(8.8806480512849,12.2,5.52269379811226));
#203936=CARTESIAN_POINT('Ctrl Pts',(8.87788025713077,12.2,5.52151066354701));
#203937=CARTESIAN_POINT('Ctrl Pts',(8.8751604548178,12.2,5.52033873193327));
#203938=CARTESIAN_POINT('Ctrl Pts',(8.87248910070822,12.2,5.51917876339611));
#203939=CARTESIAN_POINT('Ctrl Pts',(8.8698177468413,12.2,5.51801879496433));
#203940=CARTESIAN_POINT('Ctrl Pts',(8.86719484163134,12.2,5.51687078998372));
#203941=CARTESIAN_POINT('Ctrl Pts',(8.86462085280818,12.2,5.51573552677496));
#203942=CARTESIAN_POINT('Ctrl Pts',(8.86204686398504,12.2,5.51460026356621));
#203943=CARTESIAN_POINT('Ctrl Pts',(8.85952178980104,12.2,5.51347774477317));
#203944=CARTESIAN_POINT('Ctrl Pts',(8.85704610701447,12.2,5.51236876859061));
#203945=CARTESIAN_POINT('Ctrl Pts',(8.85457042400302,12.2,5.51125979230731));
#203946=CARTESIAN_POINT('Ctrl Pts',(8.85214413080862,12.2,5.51016436125673));
#203947=CARTESIAN_POINT('Ctrl Pts',(8.84976771676584,12.2,5.5090832981988));
#203948=CARTESIAN_POINT('Ctrl Pts',(8.84699523403973,12.2,5.50782205811184));
#203949=CARTESIAN_POINT('Ctrl Pts',(8.84429063614501,12.2,5.5065803740872));
#203950=CARTESIAN_POINT('Ctrl Pts',(8.84165471549355,12.2,5.50535959510122));
#203951=CARTESIAN_POINT('Ctrl Pts',(8.8393953546713,12.2,5.50431321299104));
#203952=CARTESIAN_POINT('Ctrl Pts',(8.83718645180378,12.2,5.50328218934354));
#203953=CARTESIAN_POINT('Ctrl Pts',(8.83502851227299,12.2,5.50226740062268));
#203954=CARTESIAN_POINT('Ctrl Pts',(8.83251091644776,12.2,5.50108348058661));
#203955=CARTESIAN_POINT('Ctrl Pts',(8.83006269125468,12.2,5.49992165815931));
#203956=CARTESIAN_POINT('Ctrl Pts',(8.82768466119716,12.2,5.49878336960271));
#203957=CARTESIAN_POINT('Ctrl Pts',(8.82564634948126,12.2,5.49780769358313));
#203958=CARTESIAN_POINT('Ctrl Pts',(8.82365961233255,12.2,5.49684930573914));
#203959=CARTESIAN_POINT('Ctrl Pts',(8.82172498081399,12.2,5.49590914393915));
#203960=CARTESIAN_POINT('Ctrl Pts',(8.81946791097259,12.2,5.49481228863392));
#203961=CARTESIAN_POINT('Ctrl Pts',(8.81728176748612,12.2,5.49374023430846));
#203962=CARTESIAN_POINT('Ctrl Pts',(8.8151674169253,12.2,5.49269451657004));
#203963=CARTESIAN_POINT('Ctrl Pts',(8.81335511623294,12.2,5.49179818697529));
#203964=CARTESIAN_POINT('Ctrl Pts',(8.81159556159492,12.2,5.49092120774354));
#203965=CARTESIAN_POINT('Ctrl Pts',(8.80988931908888,12.2,5.49006457444825));
#203966=CARTESIAN_POINT('Ctrl Pts',(8.8081912654558,12.2,5.48921205244499));
#203967=CARTESIAN_POINT('Ctrl Pts',(8.80654600943141,12.2,5.48837967859438));
#203968=CARTESIAN_POINT('Ctrl Pts',(8.80495412799995,12.2,5.48756847999999));
#203969=CARTESIAN_POINT('Ctrl Pts',(8.80495412799995,15.2,5.48756847999999));
#203970=CARTESIAN_POINT('Ctrl Pts',(8.80654600943141,15.2,5.48837967859438));
#203971=CARTESIAN_POINT('Ctrl Pts',(8.8081912654558,15.2,5.48921205244499));
#203972=CARTESIAN_POINT('Ctrl Pts',(8.80988931908889,15.2,5.49006457444825));
#203973=CARTESIAN_POINT('Ctrl Pts',(8.81159556159492,15.2,5.49092120774355));
#203974=CARTESIAN_POINT('Ctrl Pts',(8.81335511623294,15.2,5.49179818697529));
#203975=CARTESIAN_POINT('Ctrl Pts',(8.8151674169253,15.2,5.49269451657004));
#203976=CARTESIAN_POINT('Ctrl Pts',(8.81697971745304,15.2,5.49359084608338));
#203977=CARTESIAN_POINT('Ctrl Pts',(8.81884476396952,15.2,5.4945065246089));
#203978=CARTESIAN_POINT('Ctrl Pts',(8.82076201023318,15.2,5.49544058599162));
#203979=CARTESIAN_POINT('Ctrl Pts',(8.82267925649684,15.2,5.49637464737434));
#203980=CARTESIAN_POINT('Ctrl Pts',(8.82464870084658,15.2,5.4973270899023));
#203981=CARTESIAN_POINT('Ctrl Pts',(8.8266698055378,15.2,5.49829697666451));
#203982=CARTESIAN_POINT('Ctrl Pts',(8.8286909104126,15.2,5.49926686351481));
#203983=CARTESIAN_POINT('Ctrl Pts',(8.8307636779788,15.2,5.5002541958202));
#203984=CARTESIAN_POINT('Ctrl Pts',(8.83288758176471,15.2,5.50125805887605));
#203985=CARTESIAN_POINT('Ctrl Pts',(8.83501148535769,15.2,5.5022619218407));
#203986=CARTESIAN_POINT('Ctrl Pts',(8.83718652736316,15.2,5.50328231912499));
#203987=CARTESIAN_POINT('Ctrl Pts',(8.83941219304253,15.2,5.50431836500876));
#203988=CARTESIAN_POINT('Ctrl Pts',(8.84200880313657,15.2,5.50552708526924));
#203989=CARTESIAN_POINT('Ctrl Pts',(8.84467431955873,15.2,5.50675710279612));
#203990=CARTESIAN_POINT('Ctrl Pts',(8.84740794648027,15.2,5.50800705694175));
#203991=CARTESIAN_POINT('Ctrl Pts',(8.84975105514856,15.2,5.50907844615382));
#203992=CARTESIAN_POINT('Ctrl Pts',(8.85214420385351,15.2,5.5101644837604));
#203993=CARTESIAN_POINT('Ctrl Pts',(8.85458690552597,15.2,5.51126433797546));
#203994=CARTESIAN_POINT('Ctrl Pts',(8.85702960719842,15.2,5.51236419219053));
#203995=CARTESIAN_POINT('Ctrl Pts',(8.85952186056438,15.2,5.51347786371345));
#203996=CARTESIAN_POINT('Ctrl Pts',(8.86206318638656,15.2,5.51460454117194));
#203997=CARTESIAN_POINT('Ctrl Pts',(8.86460451243961,15.2,5.51573121873278));
#203998=CARTESIAN_POINT('Ctrl Pts',(8.86719491163205,15.2,5.51687090567025));
#203999=CARTESIAN_POINT('Ctrl Pts',(8.86983391452919,15.2,5.51802281215052));
#204000=CARTESIAN_POINT('Ctrl Pts',(8.87247291718662,15.2,5.51917471852617));
#204001=CARTESIAN_POINT('Ctrl Pts',(8.8751605231798,15.2,5.52033884494797));
#204002=CARTESIAN_POINT('Ctrl Pts',(8.87789627191583,15.2,5.52151442632241));
#204003=CARTESIAN_POINT('Ctrl Pts',(8.88063202065186,15.2,5.52269000769687));
#204004=CARTESIAN_POINT('Ctrl Pts',(8.88341591327567,15.2,5.52387704158704));
#204005=CARTESIAN_POINT('Ctrl Pts',(8.88624749608741,15.2,5.52507478595973));
#204006=CARTESIAN_POINT('Ctrl Pts',(8.88907907889914,15.2,5.52627253033242));
#204007=CARTESIAN_POINT('Ctrl Pts',(8.8919583536321,15.2,5.52748098092045));
#204008=CARTESIAN_POINT('Ctrl Pts',(8.89488487643921,15.2,5.52869941262549));
#204009=CARTESIAN_POINT('Ctrl Pts',(8.89781139951215,15.2,5.52991784444121));
#204010=CARTESIAN_POINT('Ctrl Pts',(8.90078517149801,15.2,5.53114625669128));
#204011=CARTESIAN_POINT('Ctrl Pts',(8.90380575566468,15.2,5.53238394234246));
#204012=CARTESIAN_POINT('Ctrl Pts',(8.9073297703886,15.2,5.5338279088793));
#204013=CARTESIAN_POINT('Ctrl Pts',(8.91091750233601,15.2,5.53528449469138));
#204014=CARTESIAN_POINT('Ctrl Pts',(8.91456827209096,15.2,5.53675260568714));
#204015=CARTESIAN_POINT('Ctrl Pts',(8.91769750314708,15.2,5.53801098647532));
#204016=CARTESIAN_POINT('Ctrl Pts',(8.920873049299,15.2,5.53927783519046));
#204017=CARTESIAN_POINT('Ctrl Pts',(8.92409449043396,15.2,5.54055248006114));
#204018=CARTESIAN_POINT('Ctrl Pts',(8.92731593156891,15.2,5.54182712493184));
#204019=CARTESIAN_POINT('Ctrl Pts',(8.93058326800852,15.2,5.54310956580188));
#204020=CARTESIAN_POINT('Ctrl Pts',(8.93389608705284,15.2,5.54439914967139));
#204021=CARTESIAN_POINT('Ctrl Pts',(8.93720890609717,15.2,5.54568873354089));
#204022=CARTESIAN_POINT('Ctrl Pts',(8.94056720783897,15.2,5.54698545768905));
#204023=CARTESIAN_POINT('Ctrl Pts',(8.94397058687891,15.2,5.54828868564126));
#204024=CARTESIAN_POINT('Ctrl Pts',(8.94737396622797,15.2,5.54959191371184));
#204025=CARTESIAN_POINT('Ctrl Pts',(8.95082242182309,15.2,5.55090164269141));
#204026=CARTESIAN_POINT('Ctrl Pts',(8.9543155569321,15.2,5.5522172508467));
#204027=CARTESIAN_POINT('Ctrl Pts',(8.95839088074999,15.2,5.55375212684862));
#204028=CARTESIAN_POINT('Ctrl Pts',(8.96252701526716,15.2,5.5552950021688));
#204029=CARTESIAN_POINT('Ctrl Pts',(8.96672333689116,15.2,5.55684491290517));
#204030=CARTESIAN_POINT('Ctrl Pts',(8.97032018441752,15.2,5.55817340797722));
#204031=CARTESIAN_POINT('Ctrl Pts',(8.97396125245646,15.2,5.5595070691831));
#204032=CARTESIAN_POINT('Ctrl Pts',(8.97764615390921,15.2,5.5608453065896));
#204033=CARTESIAN_POINT('Ctrl Pts',(8.98133105502726,15.2,5.56218354387451));
#204034=CARTESIAN_POINT('Ctrl Pts',(8.98505979006818,15.2,5.56352635554219));
#204035=CARTESIAN_POINT('Ctrl Pts',(8.98883197728149,15.2,5.5648731618327));
#204036=CARTESIAN_POINT('Ctrl Pts',(8.99197546674013,15.2,5.56599550044891));
#204037=CARTESIAN_POINT('Ctrl Pts',(8.99514913288874,15.2,5.56712061404997));
#204038=CARTESIAN_POINT('Ctrl Pts',(8.99835275649986,15.2,5.56824817196664));
#204039=CARTESIAN_POINT('Ctrl Pts',(9.00155638011097,15.2,5.56937572988331));
#204040=CARTESIAN_POINT('Ctrl Pts',(9.00478996083675,15.2,5.57050573522879));
#204041=CARTESIAN_POINT('Ctrl Pts',(9.00805328751832,15.2,5.57163786148393));
#204042=CARTESIAN_POINT('Ctrl Pts',(9.01131661419988,15.2,5.57276998773908));
#204043=CARTESIAN_POINT('Ctrl Pts',(9.01460968247137,15.2,5.57390423793531));
#204044=CARTESIAN_POINT('Ctrl Pts',(9.01793228275068,15.2,5.57504029411595));
#204045=CARTESIAN_POINT('Ctrl Pts',(9.02125488302999,15.2,5.5761763502966));
#204046=CARTESIAN_POINT('Ctrl Pts',(9.02460701276966,15.2,5.57731421172998));
#204047=CARTESIAN_POINT('Ctrl Pts',(9.02798846547952,15.2,5.57845356804951));
#204048=CARTESIAN_POINT('Ctrl Pts',(9.0313699181894,15.2,5.57959292436903));
#204049=CARTESIAN_POINT('Ctrl Pts',(9.0347806908032,15.2,5.58073377624764));
#204050=CARTESIAN_POINT('Ctrl Pts',(9.03822057715763,15.2,5.58187581762423));
#204051=CARTESIAN_POINT('Ctrl Pts',(9.04166046351206,15.2,5.5830178590008));
#204052=CARTESIAN_POINT('Ctrl Pts',(9.04512946302171,15.2,5.58416108891067));
#204053=CARTESIAN_POINT('Ctrl Pts',(9.04862737073241,15.2,5.58530520863297));
#204054=CARTESIAN_POINT('Ctrl Pts',(9.05212527844311,15.2,5.58644932835527));
#204055=CARTESIAN_POINT('Ctrl Pts',(9.05565209412926,15.2,5.58759433701089));
#204056=CARTESIAN_POINT('Ctrl Pts',(9.05920761371494,15.2,5.58873994089983));
#204057=CARTESIAN_POINT('Ctrl Pts',(9.06347423706274,15.2,5.59011466551661));
#204058=CARTESIAN_POINT('Ctrl Pts',(9.06778219480995,15.2,5.59149024634994));
#204059=CARTESIAN_POINT('Ctrl Pts',(9.07213113998706,15.2,5.59286618204997));
#204060=CARTESIAN_POINT('Ctrl Pts',(9.07575526109965,15.2,5.59401279517499));
#204061=CARTESIAN_POINT('Ctrl Pts',(9.07940784546153,15.2,5.59515965619721));
#204062=CARTESIAN_POINT('Ctrl Pts',(9.08308869344911,15.2,5.59630648105832));
#204063=CARTESIAN_POINT('Ctrl Pts',(9.08676954143669,15.2,5.59745330591943));
#204064=CARTESIAN_POINT('Ctrl Pts',(9.09047865590627,15.2,5.59860009435916));
#204065=CARTESIAN_POINT('Ctrl Pts',(9.09421583644214,15.2,5.59974656837474));
#204066=CARTESIAN_POINT('Ctrl Pts',(9.09795301697802,15.2,5.60089304239033));
#204067=CARTESIAN_POINT('Ctrl Pts',(9.10171826603263,15.2,5.6020392008832));
#204068=CARTESIAN_POINT('Ctrl Pts',(9.10551138797936,15.2,5.60318477067482));
#204069=CARTESIAN_POINT('Ctrl Pts',(9.10930450992608,15.2,5.60433034046644));
#204070=CARTESIAN_POINT('Ctrl Pts',(9.11312550317881,15.2,5.60547532006082));
#204071=CARTESIAN_POINT('Ctrl Pts',(9.11697417769496,15.2,5.60661944165797));
#204072=CARTESIAN_POINT('Ctrl Pts',(9.12159258694654,15.2,5.60799238752467));
#204073=CARTESIAN_POINT('Ctrl Pts',(9.12625085457627,15.2,5.60936409678583));
#204074=CARTESIAN_POINT('Ctrl Pts',(9.13094865101035,15.2,5.61073411249228));
#204075=CARTESIAN_POINT('Ctrl Pts',(9.13486348151431,15.2,5.61187579228913));
#204076=CARTESIAN_POINT('Ctrl Pts',(9.13880576409157,15.2,5.61301629533011));
#204077=CARTESIAN_POINT('Ctrl Pts',(9.14277530700965,15.2,5.61415536206614));
#204078=CARTESIAN_POINT('Ctrl Pts',(9.14674484992774,15.2,5.61529442880218));
#204079=CARTESIAN_POINT('Ctrl Pts',(9.15074165445623,15.2,5.61643206071325));
#204080=CARTESIAN_POINT('Ctrl Pts',(9.15476553397154,15.2,5.61756800057427));
#204081=CARTESIAN_POINT('Ctrl Pts',(9.15798463732061,15.2,5.61847675238879));
#204082=CARTESIAN_POINT('Ctrl Pts',(9.16122106674667,15.2,5.61938442099994));
#204083=CARTESIAN_POINT('Ctrl Pts',(9.16447473025285,15.2,5.62029087836012));
#204084=CARTESIAN_POINT('Ctrl Pts',(9.16772839420232,15.2,5.6211973358438));
#204085=CARTESIAN_POINT('Ctrl Pts',(9.17099928938852,15.2,5.62210258158859));
#204086=CARTESIAN_POINT('Ctrl Pts',(9.1742873232355,15.2,5.62300648958221));
#204087=CARTESIAN_POINT('Ctrl Pts',(9.17757535663448,15.2,5.62391039745267));
#204088=CARTESIAN_POINT('Ctrl Pts',(9.18088052783003,15.2,5.62481296639561));
#204089=CARTESIAN_POINT('Ctrl Pts',(9.18420274322337,15.2,5.62571407037766));
#204090=CARTESIAN_POINT('Ctrl Pts',(9.18752495906935,15.2,5.62661517448248));
#204091=CARTESIAN_POINT('Ctrl Pts',(9.19086421827063,15.2,5.62751481473648));
#204092=CARTESIAN_POINT('Ctrl Pts',(9.19422042946883,15.2,5.62841286623394));
#204093=CARTESIAN_POINT('Ctrl Pts',(9.19757664020976,15.2,5.62931091760904));
#204094=CARTESIAN_POINT('Ctrl Pts',(9.20094980172726,15.2,5.63020738044334));
#204095=CARTESIAN_POINT('Ctrl Pts',(9.20433982117062,15.2,5.63110213237036));
#204096=CARTESIAN_POINT('Ctrl Pts',(9.20857734582124,15.2,5.63222057237058));
#204097=CARTESIAN_POINT('Ctrl Pts',(9.21284121273534,15.2,5.63333633900974));
#204098=CARTESIAN_POINT('Ctrl Pts',(9.21713123995542,15.2,5.63444919657943));
#204099=CARTESIAN_POINT('Ctrl Pts',(9.22056326191852,15.2,5.63533948268369));
#204100=CARTESIAN_POINT('Ctrl Pts',(9.22401202803647,15.2,5.63622790754271));
#204101=CARTESIAN_POINT('Ctrl Pts',(9.22747744601891,15.2,5.63711435048393));
#204102=CARTESIAN_POINT('Ctrl Pts',(9.23094286352918,15.2,5.63800079330437));
#204103=CARTESIAN_POINT('Ctrl Pts',(9.2344249338989,15.2,5.63888525663876));
#204104=CARTESIAN_POINT('Ctrl Pts',(9.23792356594453,15.2,5.63976762012239));
#204105=CARTESIAN_POINT('Ctrl Pts',(9.24229685635908,15.2,5.64087057456711));
#204106=CARTESIAN_POINT('Ctrl Pts',(9.24669602301209,15.2,5.64197025246743));
#204107=CARTESIAN_POINT('Ctrl Pts',(9.25112089266278,15.2,5.64306642281494));
#204108=CARTESIAN_POINT('Ctrl Pts',(9.25466078857626,15.2,5.64394335914075));
#204109=CARTESIAN_POINT('Ctrl Pts',(9.25821713354134,15.2,5.64481805327132));
#204110=CARTESIAN_POINT('Ctrl Pts',(9.26178983875232,15.2,5.64569038876726));
#204111=CARTESIAN_POINT('Ctrl Pts',(9.26536254347652,15.2,5.64656272414433));
#204112=CARTESIAN_POINT('Ctrl Pts',(9.2689516076457,15.2,5.64743270245938));
#204113=CARTESIAN_POINT('Ctrl Pts',(9.27255694312708,15.2,5.64830020933316));
#204114=CARTESIAN_POINT('Ctrl Pts',(9.27616227909968,15.2,5.64916771632514));
#204115=CARTESIAN_POINT('Ctrl Pts',(9.2797838857655,15.2,5.65003275388355));
#204116=CARTESIAN_POINT('Ctrl Pts',(9.28342167624154,15.2,5.65089520820833));
#204117=CARTESIAN_POINT('Ctrl Pts',(9.28705946671758,15.2,5.65175766253311));
#204118=CARTESIAN_POINT('Ctrl Pts',(9.29071343938716,15.2,5.65261753527149));
#204119=CARTESIAN_POINT('Ctrl Pts',(9.29438350736661,15.2,5.65347471487348));
#204120=CARTESIAN_POINT('Ctrl Pts',(9.29805357484601,15.2,5.65433189435868));
#204121=CARTESIAN_POINT('Ctrl Pts',(9.30173973868881,15.2,5.65518638288183));
#204122=CARTESIAN_POINT('Ctrl Pts',(9.30544190951403,15.2,5.65603806848275));
#204123=CARTESIAN_POINT('Ctrl Pts',(9.30914408084367,15.2,5.65688975419971));
#204124=CARTESIAN_POINT('Ctrl Pts',(9.3128622594775,15.2,5.65773863990362));
#204125=CARTESIAN_POINT('Ctrl Pts',(9.31659636012708,15.2,5.65858461617164));
#204126=CARTESIAN_POINT('Ctrl Pts',(9.32033046026789,15.2,5.65943059232441));
#204127=CARTESIAN_POINT('Ctrl Pts',(9.32408048200939,15.2,5.660273659647));
#204128=CARTESIAN_POINT('Ctrl Pts',(9.32784633820051,15.2,5.66111371118963));
#204129=CARTESIAN_POINT('Ctrl Pts',(9.33161219490472,15.2,5.66195376284672));
#204130=CARTESIAN_POINT('Ctrl Pts',(9.3353938882613,15.2,5.66279079947581));
#204131=CARTESIAN_POINT('Ctrl Pts',(9.339191329826,15.2,5.66362471639599));
#204132=CARTESIAN_POINT('Ctrl Pts',(9.3429887708733,15.2,5.66445863320254));
#204133=CARTESIAN_POINT('Ctrl Pts',(9.34680196138996,15.2,5.66528942831087));
#204134=CARTESIAN_POINT('Ctrl Pts',(9.35063081618702,15.2,5.66611700046565));
#204135=CARTESIAN_POINT('Ctrl Pts',(9.35445967150578,15.2,5.66694457273318));
#204136=CARTESIAN_POINT('Ctrl Pts',(9.3583041913292,15.2,5.667768921092));
#204137=CARTESIAN_POINT('Ctrl Pts',(9.36216429004059,15.2,5.66858994152542));
#204138=CARTESIAN_POINT('Ctrl Pts',(9.36602438822606,15.2,5.66941096184697));
#204139=CARTESIAN_POINT('Ctrl Pts',(9.36990006629928,15.2,5.67022865769353));
#204140=CARTESIAN_POINT('Ctrl Pts',(9.373791239952,15.2,5.67104292339016));
#204141=CARTESIAN_POINT('Ctrl Pts',(9.3776824141349,15.2,5.67185718919773));
#204142=CARTESIAN_POINT('Ctrl Pts',(9.3815890837559,15.2,5.6726680278222));
#204143=CARTESIAN_POINT('Ctrl Pts',(9.38551116330399,15.2,5.67347533753263));
#204144=CARTESIAN_POINT('Ctrl Pts',(9.38943324231771,15.2,5.67428264713306));
#204145=CARTESIAN_POINT('Ctrl Pts',(9.3933707354561,15.2,5.67508642754254));
#204146=CARTESIAN_POINT('Ctrl Pts',(9.3973235543536,15.2,5.67588658164417));
#204147=CARTESIAN_POINT('Ctrl Pts',(9.40127637378968,15.2,5.67668673585482));
#204148=CARTESIAN_POINT('Ctrl Pts',(9.40524452319667,15.2,5.67748326170679));
#204149=CARTESIAN_POINT('Ctrl Pts',(9.40922791602488,15.2,5.67827606275));
#204150=CARTESIAN_POINT('Ctrl Pts',(9.41420715678877,15.2,5.679267064));
#204151=CARTESIAN_POINT('Ctrl Pts',(9.4192102183964,15.2,5.68025224405166));
#204152=CARTESIAN_POINT('Ctrl Pts',(9.42423694050263,15.2,5.68123141370887));
#204153=CARTESIAN_POINT('Ctrl Pts',(9.42825831785886,15.2,5.68201474937059));
#204154=CARTESIAN_POINT('Ctrl Pts',(9.43229483643133,15.2,5.68279423948897));
#204155=CARTESIAN_POINT('Ctrl Pts',(9.43634641532079,15.2,5.68356978714819));
#204156=CARTESIAN_POINT('Ctrl Pts',(9.44141088934664,15.2,5.68453922180148));
#204157=CARTESIAN_POINT('Ctrl Pts',(9.44649889546656,15.2,5.68550249814654));
#204158=CARTESIAN_POINT('Ctrl Pts',(9.45161027358966,15.2,5.68645943113316));
#204159=CARTESIAN_POINT('Ctrl Pts',(9.45876620307341,15.2,5.6877991373353));
#204160=CARTESIAN_POINT('Ctrl Pts',(9.46596794198473,15.2,5.68912640927859));
#204161=CARTESIAN_POINT('Ctrl Pts',(9.4732150570054,15.2,5.69044075224949));
#204162=CARTESIAN_POINT('Ctrl Pts',(9.47942686955785,15.2,5.69156733188036));
#204163=CARTESIAN_POINT('Ctrl Pts',(9.48567201962926,15.2,5.69268441191886));
#204164=CARTESIAN_POINT('Ctrl Pts',(9.49195023706557,15.2,5.69379168637931));
#204165=CARTESIAN_POINT('Ctrl Pts',(9.49613571573661,15.2,5.69452986941999));
#204166=CARTESIAN_POINT('Ctrl Pts',(9.50033588967609,15.2,5.69526369412689));
#204167=CARTESIAN_POINT('Ctrl Pts',(9.50455068170276,15.2,5.6959930712255));
#204168=CARTESIAN_POINT('Ctrl Pts',(9.50981917144896,15.2,5.69690479254907));
#204169=CARTESIAN_POINT('Ctrl Pts',(9.51511049966305,15.2,5.6978095628146));
#204170=CARTESIAN_POINT('Ctrl Pts',(9.52042451112256,15.2,5.69870721080033));
#204171=CARTESIAN_POINT('Ctrl Pts',(9.52467571994265,15.2,5.69942532913022));
#204172=CARTESIAN_POINT('Ctrl Pts',(9.52894144616258,15.2,5.70013888909713));
#204173=CARTESIAN_POINT('Ctrl Pts',(9.53322161103342,15.2,5.70084780215076));
#204174=CARTESIAN_POINT('Ctrl Pts',(9.53750177648744,15.2,5.70155671530098));
#204175=CARTESIAN_POINT('Ctrl Pts',(9.54179638132058,15.2,5.70226098276476));
#204176=CARTESIAN_POINT('Ctrl Pts',(9.54610534601949,15.2,5.70296051725048));
#204177=CARTESIAN_POINT('Ctrl Pts',(9.5504143101313,15.2,5.70366005164089));
#204178=CARTESIAN_POINT('Ctrl Pts',(9.55473763330786,15.2,5.70435485380143));
#204179=CARTESIAN_POINT('Ctrl Pts',(9.55907523950737,15.2,5.70504483691219));
#204180=CARTESIAN_POINT('Ctrl Pts',(9.56449724769998,15.2,5.70590731587114));
#204181=CARTESIAN_POINT('Ctrl Pts',(9.56994157144779,15.2,5.70676226613856));
#204182=CARTESIAN_POINT('Ctrl Pts',(9.57540805804322,15.2,5.70760952259752));
#204183=CARTESIAN_POINT('Ctrl Pts',(9.58087454463863,15.2,5.70845677905648));
#204184=CARTESIAN_POINT('Ctrl Pts',(9.58636319564204,15.2,5.70929634222245));
#204185=CARTESIAN_POINT('Ctrl Pts',(9.59187385911026,15.2,5.7101280471951));
#204186=CARTESIAN_POINT('Ctrl Pts',(9.59628239012511,15.2,5.71079341120949));
#204187=CARTESIAN_POINT('Ctrl Pts',(9.60070500918112,15.2,5.71145374805982));
#204188=CARTESIAN_POINT('Ctrl Pts',(9.60514163931272,15.2,5.71210897326186));
#204189=CARTESIAN_POINT('Ctrl Pts',(9.60957826883983,15.2,5.71276419837462));
#204190=CARTESIAN_POINT('Ctrl Pts',(9.61402891001412,15.2,5.71341431270508));
#204191=CARTESIAN_POINT('Ctrl Pts',(9.61849348553661,15.2,5.71405923515289));
#204192=CARTESIAN_POINT('Ctrl Pts',(9.62407420539593,15.2,5.71486538827856));
#204193=CARTESIAN_POINT('Ctrl Pts',(9.6296766977954,15.2,5.71566342735715));
#204194=CARTESIAN_POINT('Ctrl Pts',(9.63530081383876,15.2,5.7164531978833));
#204195=CARTESIAN_POINT('Ctrl Pts',(9.63867528334217,15.2,5.71692706018177));
#204196=CARTESIAN_POINT('Ctrl Pts',(9.64205753825177,15.2,5.71739794453126));
#204197=CARTESIAN_POINT('Ctrl Pts',(9.64544754504421,15.2,5.71786581793134));
#204198=CARTESIAN_POINT('Ctrl Pts',(9.64883755245251,15.2,5.71833369141641));
#204199=CARTESIAN_POINT('Ctrl Pts',(9.65223531184631,15.2,5.71879855511732));
#204200=CARTESIAN_POINT('Ctrl Pts',(9.65564079271729,15.2,5.71926037360068));
#204201=CARTESIAN_POINT('Ctrl Pts',(9.66018143284749,15.2,5.71987613143868));
#204202=CARTESIAN_POINT('Ctrl Pts',(9.6647357970898,15.2,5.72048647697461));
#204203=CARTESIAN_POINT('Ctrl Pts',(9.66930381315992,15.2,5.72109133275884));
#204204=CARTESIAN_POINT('Ctrl Pts',(9.6727298253681,15.2,5.72154497461763));
#204205=CARTESIAN_POINT('Ctrl Pts',(9.67616351552148,15.2,5.72199552782362));
#204206=CARTESIAN_POINT('Ctrl Pts',(9.67960485160915,15.2,5.72244296066341));
#204207=CARTESIAN_POINT('Ctrl Pts',(9.68304618769682,15.2,5.7228903935032));
#204208=CARTESIAN_POINT('Ctrl Pts',(9.68649517192299,15.2,5.72333470431943));
#204209=CARTESIAN_POINT('Ctrl Pts',(9.68995177025469,15.2,5.72377586217883));
#204210=CARTESIAN_POINT('Ctrl Pts',(9.69340836921434,15.2,5.72421702011838));
#204211=CARTESIAN_POINT('Ctrl Pts',(9.69687258278448,15.2,5.72465502438204));
#204212=CARTESIAN_POINT('Ctrl Pts',(9.70034437974842,15.2,5.72508984331979));
#204213=CARTESIAN_POINT('Ctrl Pts',(9.70381617608165,15.2,5.72552466217856));
#204214=CARTESIAN_POINT('Ctrl Pts',(9.70729555608946,15.2,5.72595629517917));
#204215=CARTESIAN_POINT('Ctrl Pts',(9.71078248833843,15.2,5.72638471057998));
#204216=CARTESIAN_POINT('Ctrl Pts',(9.71426942058739,15.2,5.7268131259808));
#204217=CARTESIAN_POINT('Ctrl Pts',(9.71776390401438,15.2,5.72723832408048));
#204218=CARTESIAN_POINT('Ctrl Pts',(9.72126590973641,15.2,5.72766027248372));
#204219=CARTESIAN_POINT('Ctrl Pts',(9.72593525048706,15.2,5.72822287032915));
#204220=CARTESIAN_POINT('Ctrl Pts',(9.73061796023402,15.2,5.72877969072936));
#204221=CARTESIAN_POINT('Ctrl Pts',(9.73531396751543,15.2,5.72933066118492));
#204222=CARTESIAN_POINT('Ctrl Pts',(9.73883597377628,15.2,5.72974388912042));
#204223=CARTESIAN_POINT('Ctrl Pts',(9.74236545713923,15.2,5.73015382536334));
#204224=CARTESIAN_POINT('Ctrl Pts',(9.74590239048762,15.2,5.73056043933865));
#204225=CARTESIAN_POINT('Ctrl Pts',(9.74943932319346,15.2,5.73096705324009));
#204226=CARTESIAN_POINT('Ctrl Pts',(9.75298370408223,15.2,5.73137034437504));
#204227=CARTESIAN_POINT('Ctrl Pts',(9.75653550141217,15.2,5.73177028227688));
#204228=CARTESIAN_POINT('Ctrl Pts',(9.76127123097032,15.2,5.73230353278845));
#204229=CARTESIAN_POINT('Ctrl Pts',(9.7660201479786,15.2,5.73283082265678));
#204230=CARTESIAN_POINT('Ctrl Pts',(9.77078217625464,15.2,5.73335207794812));
#204231=CARTESIAN_POINT('Ctrl Pts',(9.77435369827269,15.2,5.7337430195054));
#204232=CARTESIAN_POINT('Ctrl Pts',(9.7779325968595,15.2,5.73413056731172));
#204233=CARTESIAN_POINT('Ctrl Pts',(9.78151884079837,15.2,5.73451469032541));
#204234=CARTESIAN_POINT('Ctrl Pts',(9.78510508408574,15.2,5.73489881326932));
#204235=CARTESIAN_POINT('Ctrl Pts',(9.78869867164675,15.2,5.73527951171823));
#204236=CARTESIAN_POINT('Ctrl Pts',(9.79229957415498,15.2,5.73565675609796));
#204237=CARTESIAN_POINT('Ctrl Pts',(9.79710077728126,15.2,5.73615974858144));
#204238=CARTESIAN_POINT('Ctrl Pts',(9.80191498419252,15.2,5.73665659890233));
#204239=CARTESIAN_POINT('Ctrl Pts',(9.80674212229706,15.2,5.73714723691818));
#204240=CARTESIAN_POINT('Ctrl Pts',(9.81036247603989,15.2,5.73751521544678));
#204241=CARTESIAN_POINT('Ctrl Pts',(9.81399010275721,15.2,5.73787970071729));
#204242=CARTESIAN_POINT('Ctrl Pts',(9.8176249734575,15.2,5.73824066166298));
#204243=CARTESIAN_POINT('Ctrl Pts',(9.82247146816477,15.2,5.73872194296763));
#204244=CARTESIAN_POINT('Ctrl Pts',(9.82733083904608,15.2,5.73919695883102));
#204245=CARTESIAN_POINT('Ctrl Pts',(9.83220301527822,15.2,5.73966564202533));
#204246=CARTESIAN_POINT('Ctrl Pts',(9.83585714712041,15.2,5.74001715438914));
#204247=CARTESIAN_POINT('Ctrl Pts',(9.83951848186322,15.2,5.74036510334397));
#204248=CARTESIAN_POINT('Ctrl Pts',(9.8431869887049,15.2,5.7407094602497));
#204249=CARTESIAN_POINT('Ctrl Pts',(9.84685549554658,15.2,5.74105381715544));
#204250=CARTESIAN_POINT('Ctrl Pts',(9.85053117479968,15.2,5.74139458165847));
#204251=CARTESIAN_POINT('Ctrl Pts',(9.85421399608192,15.2,5.74173172602154));
#204252=CARTESIAN_POINT('Ctrl Pts',(9.85789681736415,15.2,5.7420688703846));
#204253=CARTESIAN_POINT('Ctrl Pts',(9.86158678041257,15.2,5.74240239298959));
#204254=CARTESIAN_POINT('Ctrl Pts',(9.86528385669394,15.2,5.7427322674781));
#204255=CARTESIAN_POINT('Ctrl Pts',(9.87021329218351,15.2,5.7431721001694));
#204256=CARTESIAN_POINT('Ctrl Pts',(9.87515537289402,15.2,5.74360544608902));
#204257=CARTESIAN_POINT('Ctrl Pts',(9.88011002451994,15.2,5.7440322367253));
#204258=CARTESIAN_POINT('Ctrl Pts',(9.88382601290184,15.2,5.74435232967344));
#204259=CARTESIAN_POINT('Ctrl Pts',(9.88754907379846,15.2,5.74466873594298));
#204260=CARTESIAN_POINT('Ctrl Pts',(9.89127917472151,15.2,5.74498142451639));
#204261=CARTESIAN_POINT('Ctrl Pts',(9.89500927564456,15.2,5.7452941130898));
#204262=CARTESIAN_POINT('Ctrl Pts',(9.89874641794522,15.2,5.74560308619412));
#204263=CARTESIAN_POINT('Ctrl Pts',(9.90249057380857,15.2,5.74590831722501));
#204264=CARTESIAN_POINT('Ctrl Pts',(9.90623472967192,15.2,5.7462135482559));
#204265=CARTESIAN_POINT('Ctrl Pts',(9.90998589995145,15.2,5.74651503727874));
#204266=CARTESIAN_POINT('Ctrl Pts',(9.91374405518896,15.2,5.74681275914344));
#204267=CARTESIAN_POINT('Ctrl Pts',(9.91750221110919,15.2,5.74711048106222));
#204268=CARTESIAN_POINT('Ctrl Pts',(9.92126735243973,15.2,5.74740443422161));
#204269=CARTESIAN_POINT('Ctrl Pts',(9.92503944240555,15.2,5.74769458655493));
#204270=CARTESIAN_POINT('Ctrl Pts',(9.92881153168611,15.2,5.74798473883553));
#204271=CARTESIAN_POINT('Ctrl Pts',(9.93259056973007,15.2,5.74827108743457));
#204272=CARTESIAN_POINT('Ctrl Pts',(9.93637652394912,15.2,5.74855360502131));
#204273=CARTESIAN_POINT('Ctrl Pts',(9.94016247816818,15.2,5.74883612260804));
#204274=CARTESIAN_POINT('Ctrl Pts',(9.94395534887523,15.2,5.74911480860738));
#204275=CARTESIAN_POINT('Ctrl Pts',(9.94775512114579,15.2,5.74938964953395));
#204276=CARTESIAN_POINT('Ctrl Pts',(9.95155489341636,15.2,5.74966449046052));
#204277=CARTESIAN_POINT('Ctrl Pts',(9.95536157030715,15.2,5.74993548595142));
#204278=CARTESIAN_POINT('Ctrl Pts',(9.95917514599994,15.2,5.75020264099999));
#204279=CARTESIAN_POINT('Origin',(-5.66257110645729E-14,15.2,-1.77635683940025E-14));
#204280=CARTESIAN_POINT('',(8.56667970899995,15.2,5.85257411499998));
#204281=CARTESIAN_POINT('',(8.56667970899995,12.2,5.85257411499998));
#204282=CARTESIAN_POINT('',(8.56667970899995,15.2,5.85257411499998));
#204283=CARTESIAN_POINT('Origin',(-5.66257110645729E-14,12.2,-1.77635683940025E-14));
#204284=CARTESIAN_POINT('Origin',(-5.66257110645729E-14,15.2,-1.77635683940025E-14));
#204285=CARTESIAN_POINT('Origin',(-5.66257110645729E-14,15.2,-1.77635683940025E-14));
#204286=CARTESIAN_POINT('',(9.27155330199994,15.2,6.80355049699998));
#204287=CARTESIAN_POINT('',(9.03946594399994,15.2,7.10901226999999));
#204288=CARTESIAN_POINT('Origin',(-5.66257110645729E-14,15.2,-1.77635683940025E-14));
#204289=CARTESIAN_POINT('',(9.03946594399994,12.2,7.10901226999999));
#204290=CARTESIAN_POINT('',(9.03946594399994,15.2,7.10901226999999));
#204291=CARTESIAN_POINT('',(9.27155330199994,12.2,6.80355049699998));
#204292=CARTESIAN_POINT('Origin',(-5.66257110645729E-14,12.2,-1.77635683940025E-14));
#204293=CARTESIAN_POINT('',(9.27155330199994,15.2,6.80355049699998));
#204294=CARTESIAN_POINT('Ctrl Pts',(9.03946594399994,15.2,7.10901226999999));
#204295=CARTESIAN_POINT('Ctrl Pts',(9.03946594399994,11.6,7.10901226999999));
#204296=CARTESIAN_POINT('Ctrl Pts',(9.03871859599995,15.2,7.10885083699999));
#204297=CARTESIAN_POINT('Ctrl Pts',(9.03871859599995,11.6,7.10885083699999));
#204298=CARTESIAN_POINT('Ctrl Pts',(9.03722439199995,15.2,7.10852778399998));
#204299=CARTESIAN_POINT('Ctrl Pts',(9.03722439199995,11.6,7.10852778399998));
#204300=CARTESIAN_POINT('Ctrl Pts',(9.03498456099994,15.2,7.10804263999999));
#204301=CARTESIAN_POINT('Ctrl Pts',(9.03498456099994,11.6,7.10804263999999));
#204302=CARTESIAN_POINT('Ctrl Pts',(9.03200107099994,15.2,7.10739465099999));
#204303=CARTESIAN_POINT('Ctrl Pts',(9.03200107099994,11.6,7.10739465099999));
#204304=CARTESIAN_POINT('Ctrl Pts',(9.02827662899995,15.2,7.10658278399999));
#204305=CARTESIAN_POINT('Ctrl Pts',(9.02827662899995,11.6,7.10658278399999));
#204306=CARTESIAN_POINT('Ctrl Pts',(9.02455710699994,15.2,7.10576903499998));
#204307=CARTESIAN_POINT('Ctrl Pts',(9.02455710699994,11.6,7.10576903499998));
#204308=CARTESIAN_POINT('Ctrl Pts',(9.02084250599994,15.2,7.10495340799999));
#204309=CARTESIAN_POINT('Ctrl Pts',(9.02084250599994,11.6,7.10495340799999));
#204310=CARTESIAN_POINT('Ctrl Pts',(9.01713282899994,15.2,7.10413590399998));
#204311=CARTESIAN_POINT('Ctrl Pts',(9.01713282899994,11.6,7.10413590399998));
#204312=CARTESIAN_POINT('Ctrl Pts',(9.01342807999994,15.2,7.10331652899999));
#204313=CARTESIAN_POINT('Ctrl Pts',(9.01342807999994,11.6,7.10331652899999));
#204314=CARTESIAN_POINT('Ctrl Pts',(9.00972826499994,15.2,7.10249528799999));
#204315=CARTESIAN_POINT('Ctrl Pts',(9.00972826499994,11.6,7.10249528799999));
#204316=CARTESIAN_POINT('Ctrl Pts',(9.00603338799994,15.2,7.10167218799998));
#204317=CARTESIAN_POINT('Ctrl Pts',(9.00603338799994,11.6,7.10167218799998));
#204318=CARTESIAN_POINT('Ctrl Pts',(9.00234345899994,15.2,7.10084723999999));
#204319=CARTESIAN_POINT('Ctrl Pts',(9.00234345899994,11.6,7.10084723999999));
#204320=CARTESIAN_POINT('Ctrl Pts',(8.99865848199994,15.2,7.10002045099999));
#204321=CARTESIAN_POINT('Ctrl Pts',(8.99865848199994,11.6,7.10002045099999));
#204322=CARTESIAN_POINT('Ctrl Pts',(8.99497846499994,15.2,7.09919182899998));
#204323=CARTESIAN_POINT('Ctrl Pts',(8.99497846499994,11.6,7.09919182899998));
#204324=CARTESIAN_POINT('Ctrl Pts',(8.99130341599994,15.2,7.09836138399999));
#204325=CARTESIAN_POINT('Ctrl Pts',(8.99130341599994,11.6,7.09836138399999));
#204326=CARTESIAN_POINT('Ctrl Pts',(8.98763333799995,15.2,7.09752912199999));
#204327=CARTESIAN_POINT('Ctrl Pts',(8.98763333799995,11.6,7.09752912199999));
#204328=CARTESIAN_POINT('Ctrl Pts',(8.98396823899994,15.2,7.09669505099999));
#204329=CARTESIAN_POINT('Ctrl Pts',(8.98396823899994,11.6,7.09669505099999));
#204330=CARTESIAN_POINT('Ctrl Pts',(8.98030812399995,15.2,7.09585917499999));
#204331=CARTESIAN_POINT('Ctrl Pts',(8.98030812399995,11.6,7.09585917499999));
#204332=CARTESIAN_POINT('Ctrl Pts',(8.97665299699994,15.2,7.09502150199998));
#204333=CARTESIAN_POINT('Ctrl Pts',(8.97665299699994,11.6,7.09502150199998));
#204334=CARTESIAN_POINT('Ctrl Pts',(8.97300286299994,15.2,7.09418203899999));
#204335=CARTESIAN_POINT('Ctrl Pts',(8.97300286299994,11.6,7.09418203899999));
#204336=CARTESIAN_POINT('Ctrl Pts',(8.96935772799995,15.2,7.09334079099998));
#204337=CARTESIAN_POINT('Ctrl Pts',(8.96935772799995,11.6,7.09334079099998));
#204338=CARTESIAN_POINT('Ctrl Pts',(8.96571759699994,15.2,7.09249776699998));
#204339=CARTESIAN_POINT('Ctrl Pts',(8.96571759699994,11.6,7.09249776699998));
#204340=CARTESIAN_POINT('Ctrl Pts',(8.96208247799994,15.2,7.09165297199998));
#204341=CARTESIAN_POINT('Ctrl Pts',(8.96208247799994,11.6,7.09165297199998));
#204342=CARTESIAN_POINT('Ctrl Pts',(8.95845237299995,15.2,7.09080641399999));
#204343=CARTESIAN_POINT('Ctrl Pts',(8.95845237299995,11.6,7.09080641399999));
#204344=CARTESIAN_POINT('Ctrl Pts',(8.95482729199994,15.2,7.08995810299999));
#204345=CARTESIAN_POINT('Ctrl Pts',(8.95482729199994,11.6,7.08995810299999));
#204346=CARTESIAN_POINT('Ctrl Pts',(8.95120723799995,15.2,7.08910804299999));
#204347=CARTESIAN_POINT('Ctrl Pts',(8.95120723799995,11.6,7.08910804299999));
#204348=CARTESIAN_POINT('Ctrl Pts',(8.94759221899994,15.2,7.08825624399999));
#204349=CARTESIAN_POINT('Ctrl Pts',(8.94759221899994,11.6,7.08825624399999));
#204350=CARTESIAN_POINT('Ctrl Pts',(8.94398223899995,15.2,7.08740271099998));
#204351=CARTESIAN_POINT('Ctrl Pts',(8.94398223899995,11.6,7.08740271099998));
#204352=CARTESIAN_POINT('Ctrl Pts',(8.94037730399995,15.2,7.08654745199999));
#204353=CARTESIAN_POINT('Ctrl Pts',(8.94037730399995,11.6,7.08654745199999));
#204354=CARTESIAN_POINT('Ctrl Pts',(8.93677741999995,15.2,7.08569047499999));
#204355=CARTESIAN_POINT('Ctrl Pts',(8.93677741999995,11.6,7.08569047499999));
#204356=CARTESIAN_POINT('Ctrl Pts',(8.93318259299994,15.2,7.08483178599998));
#204357=CARTESIAN_POINT('Ctrl Pts',(8.93318259299994,11.6,7.08483178599998));
#204358=CARTESIAN_POINT('Ctrl Pts',(8.92959282899995,15.2,7.08397139299999));
#204359=CARTESIAN_POINT('Ctrl Pts',(8.92959282899995,11.6,7.08397139299999));
#204360=CARTESIAN_POINT('Ctrl Pts',(8.92600813099994,15.2,7.08310930299999));
#204361=CARTESIAN_POINT('Ctrl Pts',(8.92600813099994,11.6,7.08310930299999));
#204362=CARTESIAN_POINT('Ctrl Pts',(8.92242850799994,15.2,7.08224552199999));
#204363=CARTESIAN_POINT('Ctrl Pts',(8.92242850799994,11.6,7.08224552199999));
#204364=CARTESIAN_POINT('Ctrl Pts',(8.91885396299994,15.2,7.08138005899999));
#204365=CARTESIAN_POINT('Ctrl Pts',(8.91885396299994,11.6,7.08138005899999));
#204366=CARTESIAN_POINT('Ctrl Pts',(8.91528450599994,15.2,7.08051292099999));
#204367=CARTESIAN_POINT('Ctrl Pts',(8.91528450599994,11.6,7.08051292099999));
#204368=CARTESIAN_POINT('Ctrl Pts',(8.91172013699994,15.2,7.07964411399999));
#204369=CARTESIAN_POINT('Ctrl Pts',(8.91172013699994,11.6,7.07964411399999));
#204370=CARTESIAN_POINT('Ctrl Pts',(8.90816086699994,15.2,7.07877364899999));
#204371=CARTESIAN_POINT('Ctrl Pts',(8.90816086699994,11.6,7.07877364899999));
#204372=CARTESIAN_POINT('Ctrl Pts',(8.90460669799995,15.2,7.07790152999999));
#204373=CARTESIAN_POINT('Ctrl Pts',(8.90460669799995,11.6,7.07790152999999));
#204374=CARTESIAN_POINT('Ctrl Pts',(8.90105763799994,15.2,7.07702776599999));
#204375=CARTESIAN_POINT('Ctrl Pts',(8.90105763799994,11.6,7.07702776599999));
#204376=CARTESIAN_POINT('Ctrl Pts',(8.89751369099994,15.2,7.07615236299999));
#204377=CARTESIAN_POINT('Ctrl Pts',(8.89751369099994,11.6,7.07615236299999));
#204378=CARTESIAN_POINT('Ctrl Pts',(8.89397486399995,15.2,7.07527532999999));
#204379=CARTESIAN_POINT('Ctrl Pts',(8.89397486399995,11.6,7.07527532999999));
#204380=CARTESIAN_POINT('Ctrl Pts',(8.89044116399995,15.2,7.07439667399999));
#204381=CARTESIAN_POINT('Ctrl Pts',(8.89044116399995,11.6,7.07439667399999));
#204382=CARTESIAN_POINT('Ctrl Pts',(8.88691259399994,15.2,7.07351640199998));
#204383=CARTESIAN_POINT('Ctrl Pts',(8.88691259399994,11.6,7.07351640199998));
#204384=CARTESIAN_POINT('Ctrl Pts',(8.88338916199995,15.2,7.07263452199999));
#204385=CARTESIAN_POINT('Ctrl Pts',(8.88338916199995,11.6,7.07263452199999));
#204386=CARTESIAN_POINT('Ctrl Pts',(8.87987087299994,15.2,7.07175104099999));
#204387=CARTESIAN_POINT('Ctrl Pts',(8.87987087299994,11.6,7.07175104099999));
#204388=CARTESIAN_POINT('Ctrl Pts',(8.87635773099994,15.2,7.07086596699998));
#204389=CARTESIAN_POINT('Ctrl Pts',(8.87635773099994,11.6,7.07086596699998));
#204390=CARTESIAN_POINT('Ctrl Pts',(8.87284974399994,15.2,7.06997930699998));
#204391=CARTESIAN_POINT('Ctrl Pts',(8.87284974399994,11.6,7.06997930699998));
#204392=CARTESIAN_POINT('Ctrl Pts',(8.86934691799994,15.2,7.06909106899998));
#204393=CARTESIAN_POINT('Ctrl Pts',(8.86934691799994,11.6,7.06909106899998));
#204394=CARTESIAN_POINT('Ctrl Pts',(8.86584925799994,15.2,7.06820126099998));
#204395=CARTESIAN_POINT('Ctrl Pts',(8.86584925799994,11.6,7.06820126099998));
#204396=CARTESIAN_POINT('Ctrl Pts',(8.86235676999994,15.2,7.06730989099999));
#204397=CARTESIAN_POINT('Ctrl Pts',(8.86235676999994,11.6,7.06730989099999));
#204398=CARTESIAN_POINT('Ctrl Pts',(8.85886945899994,15.2,7.06641696499998));
#204399=CARTESIAN_POINT('Ctrl Pts',(8.85886945899994,11.6,7.06641696499998));
#204400=CARTESIAN_POINT('Ctrl Pts',(8.85538733199994,15.2,7.06552249099998));
#204401=CARTESIAN_POINT('Ctrl Pts',(8.85538733199994,11.6,7.06552249099998));
#204402=CARTESIAN_POINT('Ctrl Pts',(8.85191039299994,15.2,7.06462647799999));
#204403=CARTESIAN_POINT('Ctrl Pts',(8.85191039299994,11.6,7.06462647799999));
#204404=CARTESIAN_POINT('Ctrl Pts',(8.84843865099995,15.2,7.06372893099999));
#204405=CARTESIAN_POINT('Ctrl Pts',(8.84843865099995,11.6,7.06372893099999));
#204406=CARTESIAN_POINT('Ctrl Pts',(8.84497210899994,15.2,7.06282986199999));
#204407=CARTESIAN_POINT('Ctrl Pts',(8.84497210899994,11.6,7.06282986199999));
#204408=CARTESIAN_POINT('Ctrl Pts',(8.84151077299994,15.2,7.06192927399999));
#204409=CARTESIAN_POINT('Ctrl Pts',(8.84151077299994,11.6,7.06192927399999));
#204410=CARTESIAN_POINT('Ctrl Pts',(8.83805465099995,15.2,7.06102717799999));
#204411=CARTESIAN_POINT('Ctrl Pts',(8.83805465099995,11.6,7.06102717799999));
#204412=CARTESIAN_POINT('Ctrl Pts',(8.83460374599995,15.2,7.06012358099999));
#204413=CARTESIAN_POINT('Ctrl Pts',(8.83460374599995,11.6,7.06012358099999));
#204414=CARTESIAN_POINT('Ctrl Pts',(8.83115806599994,15.2,7.05921849099998));
#204415=CARTESIAN_POINT('Ctrl Pts',(8.83115806599994,11.6,7.05921849099998));
#204416=CARTESIAN_POINT('Ctrl Pts',(8.82771761599994,15.2,7.05831191399999));
#204417=CARTESIAN_POINT('Ctrl Pts',(8.82771761599994,11.6,7.05831191399999));
#204418=CARTESIAN_POINT('Ctrl Pts',(8.82428240299994,15.2,7.05740385899999));
#204419=CARTESIAN_POINT('Ctrl Pts',(8.82428240299994,11.6,7.05740385899999));
#204420=CARTESIAN_POINT('Ctrl Pts',(8.82085243099995,15.2,7.05649433499998));
#204421=CARTESIAN_POINT('Ctrl Pts',(8.82085243099995,11.6,7.05649433499998));
#204422=CARTESIAN_POINT('Ctrl Pts',(8.81742770599995,15.2,7.05558334799999));
#204423=CARTESIAN_POINT('Ctrl Pts',(8.81742770599995,11.6,7.05558334799999));
#204424=CARTESIAN_POINT('Ctrl Pts',(8.81400823499994,15.2,7.05467090699998));
#204425=CARTESIAN_POINT('Ctrl Pts',(8.81400823499994,11.6,7.05467090699998));
#204426=CARTESIAN_POINT('Ctrl Pts',(8.81059402299995,15.2,7.05375701899998));
#204427=CARTESIAN_POINT('Ctrl Pts',(8.81059402299995,11.6,7.05375701899998));
#204428=CARTESIAN_POINT('Ctrl Pts',(8.80718507599994,15.2,7.05284169299999));
#204429=CARTESIAN_POINT('Ctrl Pts',(8.80718507599994,11.6,7.05284169299999));
#204430=CARTESIAN_POINT('Ctrl Pts',(8.80378140199995,15.2,7.05192493599998));
#204431=CARTESIAN_POINT('Ctrl Pts',(8.80378140199995,11.6,7.05192493599998));
#204432=CARTESIAN_POINT('Ctrl Pts',(8.80038300299994,15.2,7.05100675699998));
#204433=CARTESIAN_POINT('Ctrl Pts',(8.80038300299994,11.6,7.05100675699998));
#204434=CARTESIAN_POINT('Ctrl Pts',(8.79698988899994,15.2,7.05008716199998));
#204435=CARTESIAN_POINT('Ctrl Pts',(8.79698988899994,11.6,7.05008716199998));
#204436=CARTESIAN_POINT('Ctrl Pts',(8.79360206099994,15.2,7.04916616199998));
#204437=CARTESIAN_POINT('Ctrl Pts',(8.79360206099994,11.6,7.04916616199998));
#204438=CARTESIAN_POINT('Ctrl Pts',(8.79021952999994,15.2,7.04824376099998));
#204439=CARTESIAN_POINT('Ctrl Pts',(8.79021952999994,11.6,7.04824376099998));
#204440=CARTESIAN_POINT('Ctrl Pts',(8.78684229799994,15.2,7.04731997099999));
#204441=CARTESIAN_POINT('Ctrl Pts',(8.78684229799994,11.6,7.04731997099999));
#204442=CARTESIAN_POINT('Ctrl Pts',(8.78347037299994,15.2,7.04639479699999));
#204443=CARTESIAN_POINT('Ctrl Pts',(8.78347037299994,11.6,7.04639479699999));
#204444=CARTESIAN_POINT('Ctrl Pts',(8.78010375999994,15.2,7.04546824999999));
#204445=CARTESIAN_POINT('Ctrl Pts',(8.78010375999994,11.6,7.04546824999999));
#204446=CARTESIAN_POINT('Ctrl Pts',(8.77674246599994,15.2,7.04454033599998));
#204447=CARTESIAN_POINT('Ctrl Pts',(8.77674246599994,11.6,7.04454033599998));
#204448=CARTESIAN_POINT('Ctrl Pts',(8.77338649599994,15.2,7.04361106299999));
#204449=CARTESIAN_POINT('Ctrl Pts',(8.77338649599994,11.6,7.04361106299999));
#204450=CARTESIAN_POINT('Ctrl Pts',(8.77003585599994,15.2,7.04268043999999));
#204451=CARTESIAN_POINT('Ctrl Pts',(8.77003585599994,11.6,7.04268043999999));
#204452=CARTESIAN_POINT('Ctrl Pts',(8.76669055199994,15.2,7.04174847499999));
#204453=CARTESIAN_POINT('Ctrl Pts',(8.76669055199994,11.6,7.04174847499999));
#204454=CARTESIAN_POINT('Ctrl Pts',(8.76335058999994,15.2,7.04081517599998));
#204455=CARTESIAN_POINT('Ctrl Pts',(8.76335058999994,11.6,7.04081517599998));
#204456=CARTESIAN_POINT('Ctrl Pts',(8.76001597499994,15.2,7.03988055099998));
#204457=CARTESIAN_POINT('Ctrl Pts',(8.76001597499994,11.6,7.03988055099998));
#204458=CARTESIAN_POINT('Ctrl Pts',(8.75668671499995,15.2,7.03894460699999));
#204459=CARTESIAN_POINT('Ctrl Pts',(8.75668671499995,11.6,7.03894460699999));
#204460=CARTESIAN_POINT('Ctrl Pts',(8.75336281399994,15.2,7.03800735499998));
#204461=CARTESIAN_POINT('Ctrl Pts',(8.75336281399994,11.6,7.03800735499998));
#204462=CARTESIAN_POINT('Ctrl Pts',(8.75004427899994,15.2,7.03706880299999));
#204463=CARTESIAN_POINT('Ctrl Pts',(8.75004427899994,11.6,7.03706880299999));
#204464=CARTESIAN_POINT('Ctrl Pts',(8.74673111599994,15.2,7.03612895699998));
#204465=CARTESIAN_POINT('Ctrl Pts',(8.74673111599994,11.6,7.03612895699998));
#204466=CARTESIAN_POINT('Ctrl Pts',(8.74342332999994,15.2,7.03518782599998));
#204467=CARTESIAN_POINT('Ctrl Pts',(8.74342332999994,11.6,7.03518782599998));
#204468=CARTESIAN_POINT('Ctrl Pts',(8.74012092799994,15.2,7.03424541899999));
#204469=CARTESIAN_POINT('Ctrl Pts',(8.74012092799994,11.6,7.03424541899999));
#204470=CARTESIAN_POINT('Ctrl Pts',(8.73682391499995,15.2,7.03330174299998));
#204471=CARTESIAN_POINT('Ctrl Pts',(8.73682391499995,11.6,7.03330174299998));
#204472=CARTESIAN_POINT('Ctrl Pts',(8.73353229799994,15.2,7.03235680799998));
#204473=CARTESIAN_POINT('Ctrl Pts',(8.73353229799994,11.6,7.03235680799998));
#204474=CARTESIAN_POINT('Ctrl Pts',(8.73024608099995,15.2,7.03141062299999));
#204475=CARTESIAN_POINT('Ctrl Pts',(8.73024608099995,11.6,7.03141062299999));
#204476=CARTESIAN_POINT('Ctrl Pts',(8.72696527299994,15.2,7.03046319399999));
#204477=CARTESIAN_POINT('Ctrl Pts',(8.72696527299994,11.6,7.03046319399999));
#204478=CARTESIAN_POINT('Ctrl Pts',(8.72368987799994,15.2,7.02951452999999));
#204479=CARTESIAN_POINT('Ctrl Pts',(8.72368987799994,11.6,7.02951452999999));
#204480=CARTESIAN_POINT('Ctrl Pts',(8.72041990199994,15.2,7.02856464099998));
#204481=CARTESIAN_POINT('Ctrl Pts',(8.72041990199994,11.6,7.02856464099998));
#204482=CARTESIAN_POINT('Ctrl Pts',(8.71715535199994,15.2,7.02761353499999));
#204483=CARTESIAN_POINT('Ctrl Pts',(8.71715535199994,11.6,7.02761353499999));
#204484=CARTESIAN_POINT('Ctrl Pts',(8.71389623199994,15.2,7.02666121899998));
#204485=CARTESIAN_POINT('Ctrl Pts',(8.71389623199994,11.6,7.02666121899998));
#204486=CARTESIAN_POINT('Ctrl Pts',(8.71064255099994,15.2,7.02570770199999));
#204487=CARTESIAN_POINT('Ctrl Pts',(8.71064255099994,11.6,7.02570770199999));
#204488=CARTESIAN_POINT('Ctrl Pts',(8.70739431399995,15.2,7.02475299199998));
#204489=CARTESIAN_POINT('Ctrl Pts',(8.70739431399995,11.6,7.02475299199998));
#204490=CARTESIAN_POINT('Ctrl Pts',(8.70415152399995,15.2,7.02379709899999));
#204491=CARTESIAN_POINT('Ctrl Pts',(8.70415152399995,11.6,7.02379709899999));
#204492=CARTESIAN_POINT('Ctrl Pts',(8.70091418999994,15.2,7.02284003199999));
#204493=CARTESIAN_POINT('Ctrl Pts',(8.70091418999994,11.6,7.02284003199999));
#204494=CARTESIAN_POINT('Ctrl Pts',(8.69768231899995,15.2,7.02188179799998));
#204495=CARTESIAN_POINT('Ctrl Pts',(8.69768231899995,11.6,7.02188179799998));
#204496=CARTESIAN_POINT('Ctrl Pts',(8.69445591399994,15.2,7.02092240599999));
#204497=CARTESIAN_POINT('Ctrl Pts',(8.69445591399994,11.6,7.02092240599999));
#204498=CARTESIAN_POINT('Ctrl Pts',(8.69123498299994,15.2,7.01996186499999));
#204499=CARTESIAN_POINT('Ctrl Pts',(8.69123498299994,11.6,7.01996186499999));
#204500=CARTESIAN_POINT('Ctrl Pts',(8.68801953099995,15.2,7.01900018299998));
#204501=CARTESIAN_POINT('Ctrl Pts',(8.68801953099995,11.6,7.01900018299998));
#204502=CARTESIAN_POINT('Ctrl Pts',(8.68480956499995,15.2,7.01803736999998));
#204503=CARTESIAN_POINT('Ctrl Pts',(8.68480956499995,11.6,7.01803736999998));
#204504=CARTESIAN_POINT('Ctrl Pts',(8.68160508999994,15.2,7.01707343299999));
#204505=CARTESIAN_POINT('Ctrl Pts',(8.68160508999994,11.6,7.01707343299999));
#204506=CARTESIAN_POINT('Ctrl Pts',(8.67840611299994,15.2,7.01610838099998));
#204507=CARTESIAN_POINT('Ctrl Pts',(8.67840611299994,11.6,7.01610838099998));
#204508=CARTESIAN_POINT('Ctrl Pts',(8.67521263999994,15.2,7.01514222399998));
#204509=CARTESIAN_POINT('Ctrl Pts',(8.67521263999994,11.6,7.01514222399998));
#204510=CARTESIAN_POINT('Ctrl Pts',(8.67202467599994,15.2,7.01417496899998));
#204511=CARTESIAN_POINT('Ctrl Pts',(8.67202467599994,11.6,7.01417496899998));
#204512=CARTESIAN_POINT('Ctrl Pts',(8.66884222899994,15.2,7.01320662699998));
#204513=CARTESIAN_POINT('Ctrl Pts',(8.66884222899994,11.6,7.01320662699998));
#204514=CARTESIAN_POINT('Ctrl Pts',(8.66566530299994,15.2,7.01223720499998));
#204515=CARTESIAN_POINT('Ctrl Pts',(8.66566530299994,11.6,7.01223720499998));
#204516=CARTESIAN_POINT('Ctrl Pts',(8.66249390499994,15.2,7.01126671199999));
#204517=CARTESIAN_POINT('Ctrl Pts',(8.66249390499994,11.6,7.01126671199999));
#204518=CARTESIAN_POINT('Ctrl Pts',(8.65932804199994,15.2,7.01029515699998));
#204519=CARTESIAN_POINT('Ctrl Pts',(8.65932804199994,11.6,7.01029515699998));
#204520=CARTESIAN_POINT('Ctrl Pts',(8.65616771699995,15.2,7.00932254899998));
#204521=CARTESIAN_POINT('Ctrl Pts',(8.65616771699995,11.6,7.00932254899998));
#204522=CARTESIAN_POINT('Ctrl Pts',(8.65301293899994,15.2,7.00834889699999));
#204523=CARTESIAN_POINT('Ctrl Pts',(8.65301293899994,11.6,7.00834889699999));
#204524=CARTESIAN_POINT('Ctrl Pts',(8.64986371499995,15.2,7.00737420999998));
#204525=CARTESIAN_POINT('Ctrl Pts',(8.64986371499995,11.6,7.00737420999998));
#204526=CARTESIAN_POINT('Ctrl Pts',(8.64672004799995,15.2,7.00639849699999));
#204527=CARTESIAN_POINT('Ctrl Pts',(8.64672004799995,11.6,7.00639849699999));
#204528=CARTESIAN_POINT('Ctrl Pts',(8.64358194499994,15.2,7.00542176599999));
#204529=CARTESIAN_POINT('Ctrl Pts',(8.64358194499994,11.6,7.00542176599999));
#204530=CARTESIAN_POINT('Ctrl Pts',(8.64044941299994,15.2,7.00444402599998));
#204531=CARTESIAN_POINT('Ctrl Pts',(8.64044941299994,11.6,7.00444402599998));
#204532=CARTESIAN_POINT('Ctrl Pts',(8.63732245799994,15.2,7.00346528799999));
#204533=CARTESIAN_POINT('Ctrl Pts',(8.63732245799994,11.6,7.00346528799999));
#204534=CARTESIAN_POINT('Ctrl Pts',(8.63420108499995,15.2,7.00248555899999));
#204535=CARTESIAN_POINT('Ctrl Pts',(8.63420108499995,11.6,7.00248555899999));
#204536=CARTESIAN_POINT('Ctrl Pts',(8.63108530199994,15.2,7.00150484999998));
#204537=CARTESIAN_POINT('Ctrl Pts',(8.63108530199994,11.6,7.00150484999998));
#204538=CARTESIAN_POINT('Ctrl Pts',(8.62797511399994,15.2,7.00052316799999));
#204539=CARTESIAN_POINT('Ctrl Pts',(8.62797511399994,11.6,7.00052316799999));
#204540=CARTESIAN_POINT('Ctrl Pts',(8.62487052699995,15.2,6.99954052199999));
#204541=CARTESIAN_POINT('Ctrl Pts',(8.62487052699995,11.6,6.99954052199999));
#204542=CARTESIAN_POINT('Ctrl Pts',(8.62177154699994,15.2,6.99855692299998));
#204543=CARTESIAN_POINT('Ctrl Pts',(8.62177154699994,11.6,6.99855692299998));
#204544=CARTESIAN_POINT('Ctrl Pts',(8.61867818099994,15.2,6.99757237799999));
#204545=CARTESIAN_POINT('Ctrl Pts',(8.61867818099994,11.6,6.99757237799999));
#204546=CARTESIAN_POINT('Ctrl Pts',(8.61559043399994,15.2,6.99658689899999));
#204547=CARTESIAN_POINT('Ctrl Pts',(8.61559043399994,11.6,6.99658689899999));
#204548=CARTESIAN_POINT('Ctrl Pts',(8.61250831399994,15.2,6.99560049199999));
#204549=CARTESIAN_POINT('Ctrl Pts',(8.61250831399994,11.6,6.99560049199999));
#204550=CARTESIAN_POINT('Ctrl Pts',(8.60943182399994,15.2,6.99461316899999));
#204551=CARTESIAN_POINT('Ctrl Pts',(8.60943182399994,11.6,6.99461316899999));
#204552=CARTESIAN_POINT('Ctrl Pts',(8.60636097399994,15.2,6.99362493599998));
#204553=CARTESIAN_POINT('Ctrl Pts',(8.60636097399994,11.6,6.99362493599998));
#204554=CARTESIAN_POINT('Ctrl Pts',(8.60329576799994,15.2,6.99263580599998));
#204555=CARTESIAN_POINT('Ctrl Pts',(8.60329576799994,11.6,6.99263580599998));
#204556=CARTESIAN_POINT('Ctrl Pts',(8.60023621199994,15.2,6.99164578599999));
#204557=CARTESIAN_POINT('Ctrl Pts',(8.60023621199994,11.6,6.99164578599999));
#204558=CARTESIAN_POINT('Ctrl Pts',(8.59718231199994,15.2,6.99065488499999));
#204559=CARTESIAN_POINT('Ctrl Pts',(8.59718231199994,11.6,6.99065488499999));
#204560=CARTESIAN_POINT('Ctrl Pts',(8.59413407599994,15.2,6.98966311399998));
#204561=CARTESIAN_POINT('Ctrl Pts',(8.59413407599994,11.6,6.98966311399998));
#204562=CARTESIAN_POINT('Ctrl Pts',(8.59109150899994,15.2,6.98867048199999));
#204563=CARTESIAN_POINT('Ctrl Pts',(8.59109150899994,11.6,6.98867048199999));
#204564=CARTESIAN_POINT('Ctrl Pts',(8.58805461599994,15.2,6.98767699699999));
#204565=CARTESIAN_POINT('Ctrl Pts',(8.58805461599994,11.6,6.98767699699999));
#204566=CARTESIAN_POINT('Ctrl Pts',(8.58502340499994,15.2,6.98668266799999));
#204567=CARTESIAN_POINT('Ctrl Pts',(8.58502340499994,11.6,6.98668266799999));
#204568=CARTESIAN_POINT('Ctrl Pts',(8.58199788199994,15.2,6.98568750799998));
#204569=CARTESIAN_POINT('Ctrl Pts',(8.58199788199994,11.6,6.98568750799998));
#204570=CARTESIAN_POINT('Ctrl Pts',(8.57897805299995,15.2,6.98469152199999));
#204571=CARTESIAN_POINT('Ctrl Pts',(8.57897805299995,11.6,6.98469152199999));
#204572=CARTESIAN_POINT('Ctrl Pts',(8.57596392399994,15.2,6.98369472299999));
#204573=CARTESIAN_POINT('Ctrl Pts',(8.57596392399994,11.6,6.98369472299999));
#204574=CARTESIAN_POINT('Ctrl Pts',(8.57295550099994,15.2,6.98269711899999));
#204575=CARTESIAN_POINT('Ctrl Pts',(8.57295550099994,11.6,6.98269711899999));
#204576=CARTESIAN_POINT('Ctrl Pts',(8.56995279099995,15.2,6.98169871899999));
#204577=CARTESIAN_POINT('Ctrl Pts',(8.56995279099995,11.6,6.98169871899999));
#204578=CARTESIAN_POINT('Ctrl Pts',(8.56695579999995,15.2,6.98069953299999));
#204579=CARTESIAN_POINT('Ctrl Pts',(8.56695579999995,11.6,6.98069953299999));
#204580=CARTESIAN_POINT('Ctrl Pts',(8.56396453399995,15.2,6.97969957099998));
#204581=CARTESIAN_POINT('Ctrl Pts',(8.56396453399995,11.6,6.97969957099998));
#204582=CARTESIAN_POINT('Ctrl Pts',(8.56097899899994,15.2,6.97869884199999));
#204583=CARTESIAN_POINT('Ctrl Pts',(8.56097899899994,11.6,6.97869884199999));
#204584=CARTESIAN_POINT('Ctrl Pts',(8.55799920199994,15.2,6.97769735699998));
#204585=CARTESIAN_POINT('Ctrl Pts',(8.55799920199994,11.6,6.97769735699998));
#204586=CARTESIAN_POINT('Ctrl Pts',(8.55502514699995,15.2,6.97669512399998));
#204587=CARTESIAN_POINT('Ctrl Pts',(8.55502514699995,11.6,6.97669512399998));
#204588=CARTESIAN_POINT('Ctrl Pts',(8.55205684399994,15.2,6.97569215299998));
#204589=CARTESIAN_POINT('Ctrl Pts',(8.55205684399994,11.6,6.97569215299998));
#204590=CARTESIAN_POINT('Ctrl Pts',(8.54909429799994,15.2,6.97468845499999));
#204591=CARTESIAN_POINT('Ctrl Pts',(8.54909429799994,11.6,6.97468845499999));
#204592=CARTESIAN_POINT('Ctrl Pts',(8.54613751299994,15.2,6.97368403699999));
#204593=CARTESIAN_POINT('Ctrl Pts',(8.54613751299994,11.6,6.97368403699999));
#204594=CARTESIAN_POINT('Ctrl Pts',(8.54318649699995,15.2,6.97267891199999));
#204595=CARTESIAN_POINT('Ctrl Pts',(8.54318649699995,11.6,6.97267891199999));
#204596=CARTESIAN_POINT('Ctrl Pts',(8.54024125699994,15.2,6.97167308799998));
#204597=CARTESIAN_POINT('Ctrl Pts',(8.54024125699994,11.6,6.97167308799998));
#204598=CARTESIAN_POINT('Ctrl Pts',(8.53730179799994,15.2,6.97066657499998));
#204599=CARTESIAN_POINT('Ctrl Pts',(8.53730179799994,11.6,6.97066657499998));
#204600=CARTESIAN_POINT('Ctrl Pts',(8.53436812699995,15.2,6.96965938299999));
#204601=CARTESIAN_POINT('Ctrl Pts',(8.53436812699995,11.6,6.96965938299999));
#204602=CARTESIAN_POINT('Ctrl Pts',(8.53144025099994,15.2,6.96865152099999));
#204603=CARTESIAN_POINT('Ctrl Pts',(8.53144025099994,11.6,6.96865152099999));
#204604=CARTESIAN_POINT('Ctrl Pts',(8.52851817399995,15.2,6.96764299999998));
#204605=CARTESIAN_POINT('Ctrl Pts',(8.52851817399995,11.6,6.96764299999998));
#204606=CARTESIAN_POINT('Ctrl Pts',(8.52560190399995,15.2,6.96663382999999));
#204607=CARTESIAN_POINT('Ctrl Pts',(8.52560190399995,11.6,6.96663382999999));
#204608=CARTESIAN_POINT('Ctrl Pts',(8.52269144699994,15.2,6.96562401999999));
#204609=CARTESIAN_POINT('Ctrl Pts',(8.52269144699994,11.6,6.96562401999999));
#204610=CARTESIAN_POINT('Ctrl Pts',(8.51978681099994,15.2,6.96461358099998));
#204611=CARTESIAN_POINT('Ctrl Pts',(8.51978681099994,11.6,6.96461358099998));
#204612=CARTESIAN_POINT('Ctrl Pts',(8.51688799999994,15.2,6.96360252199998));
#204613=CARTESIAN_POINT('Ctrl Pts',(8.51688799999994,11.6,6.96360252199998));
#204614=CARTESIAN_POINT('Ctrl Pts',(8.51399501999994,15.2,6.96259085299998));
#204615=CARTESIAN_POINT('Ctrl Pts',(8.51399501999994,11.6,6.96259085299998));
#204616=CARTESIAN_POINT('Ctrl Pts',(8.51110787899995,15.2,6.96157858499999));
#204617=CARTESIAN_POINT('Ctrl Pts',(8.51110787899995,11.6,6.96157858499999));
#204618=CARTESIAN_POINT('Ctrl Pts',(8.50822658299995,15.2,6.96056572799999));
#204619=CARTESIAN_POINT('Ctrl Pts',(8.50822658299995,11.6,6.96056572799999));
#204620=CARTESIAN_POINT('Ctrl Pts',(8.50535113799994,15.2,6.95955229099999));
#204621=CARTESIAN_POINT('Ctrl Pts',(8.50535113799994,11.6,6.95955229099999));
#204622=CARTESIAN_POINT('Ctrl Pts',(8.50248155099994,15.2,6.95853828499998));
#204623=CARTESIAN_POINT('Ctrl Pts',(8.50248155099994,11.6,6.95853828499998));
#204624=CARTESIAN_POINT('Ctrl Pts',(8.49961782799994,15.2,6.95752372099999));
#204625=CARTESIAN_POINT('Ctrl Pts',(8.49961782799994,11.6,6.95752372099999));
#204626=CARTESIAN_POINT('Ctrl Pts',(8.49675997499994,15.2,6.95650860699998));
#204627=CARTESIAN_POINT('Ctrl Pts',(8.49675997499994,11.6,6.95650860699998));
#204628=CARTESIAN_POINT('Ctrl Pts',(8.49390799999994,15.2,6.95549295399999));
#204629=CARTESIAN_POINT('Ctrl Pts',(8.49390799999994,11.6,6.95549295399999));
#204630=CARTESIAN_POINT('Ctrl Pts',(8.49106190599995,15.2,6.95447677399999));
#204631=CARTESIAN_POINT('Ctrl Pts',(8.49106190599995,11.6,6.95447677399999));
#204632=CARTESIAN_POINT('Ctrl Pts',(8.48822170299995,15.2,6.95346007399999));
#204633=CARTESIAN_POINT('Ctrl Pts',(8.48822170299995,11.6,6.95346007399999));
#204634=CARTESIAN_POINT('Ctrl Pts',(8.48538739499994,15.2,6.95244286799999));
#204635=CARTESIAN_POINT('Ctrl Pts',(8.48538739499994,11.6,6.95244286799999));
#204636=CARTESIAN_POINT('Ctrl Pts',(8.48255898999994,15.2,6.95142516299998));
#204637=CARTESIAN_POINT('Ctrl Pts',(8.48255898999994,11.6,6.95142516299998));
#204638=CARTESIAN_POINT('Ctrl Pts',(8.47973649299994,15.2,6.95040697199998));
#204639=CARTESIAN_POINT('Ctrl Pts',(8.47973649299994,11.6,6.95040697199998));
#204640=CARTESIAN_POINT('Ctrl Pts',(8.47691991299994,15.2,6.94938830399998));
#204641=CARTESIAN_POINT('Ctrl Pts',(8.47691991299994,11.6,6.94938830399998));
#204642=CARTESIAN_POINT('Ctrl Pts',(8.47410925299994,15.2,6.94836916899998));
#204643=CARTESIAN_POINT('Ctrl Pts',(8.47410925299994,11.6,6.94836916899998));
#204644=CARTESIAN_POINT('Ctrl Pts',(8.47130452199995,15.2,6.94734957899998));
#204645=CARTESIAN_POINT('Ctrl Pts',(8.47130452199995,11.6,6.94734957899998));
#204646=CARTESIAN_POINT('Ctrl Pts',(8.46850572399994,15.2,6.94632954299998));
#204647=CARTESIAN_POINT('Ctrl Pts',(8.46850572399994,11.6,6.94632954299998));
#204648=CARTESIAN_POINT('Ctrl Pts',(8.46571286899995,15.2,6.94530907199999));
#204649=CARTESIAN_POINT('Ctrl Pts',(8.46571286899995,11.6,6.94530907199999));
#204650=CARTESIAN_POINT('Ctrl Pts',(8.46292595999994,15.2,6.94428817699999));
#204651=CARTESIAN_POINT('Ctrl Pts',(8.46292595999994,11.6,6.94428817699999));
#204652=CARTESIAN_POINT('Ctrl Pts',(8.46014500499994,15.2,6.94326686699998));
#204653=CARTESIAN_POINT('Ctrl Pts',(8.46014500499994,11.6,6.94326686699998));
#204654=CARTESIAN_POINT('Ctrl Pts',(8.45737001099995,15.2,6.94224515399998));
#204655=CARTESIAN_POINT('Ctrl Pts',(8.45737001099995,11.6,6.94224515399998));
#204656=CARTESIAN_POINT('Ctrl Pts',(8.45460098399995,15.2,6.94122304799999));
#204657=CARTESIAN_POINT('Ctrl Pts',(8.45460098399995,11.6,6.94122304799999));
#204658=CARTESIAN_POINT('Ctrl Pts',(8.45183793099994,15.2,6.94020056099999));
#204659=CARTESIAN_POINT('Ctrl Pts',(8.45183793099994,11.6,6.94020056099999));
#204660=CARTESIAN_POINT('Ctrl Pts',(8.44908085599995,15.2,6.93917770199998));
#204661=CARTESIAN_POINT('Ctrl Pts',(8.44908085599995,11.6,6.93917770199998));
#204662=CARTESIAN_POINT('Ctrl Pts',(8.44632976799994,15.2,6.93815448199998));
#204663=CARTESIAN_POINT('Ctrl Pts',(8.44632976799994,11.6,6.93815448199998));
#204664=CARTESIAN_POINT('Ctrl Pts',(8.44358467399994,15.2,6.93713091199999));
#204665=CARTESIAN_POINT('Ctrl Pts',(8.44358467399994,11.6,6.93713091199999));
#204666=CARTESIAN_POINT('Ctrl Pts',(8.44084557799994,15.2,6.93610700299998));
#204667=CARTESIAN_POINT('Ctrl Pts',(8.44084557799994,11.6,6.93610700299998));
#204668=CARTESIAN_POINT('Ctrl Pts',(8.43811248799994,15.2,6.93508276499998));
#204669=CARTESIAN_POINT('Ctrl Pts',(8.43811248799994,11.6,6.93508276499998));
#204670=CARTESIAN_POINT('Ctrl Pts',(8.43538541199995,15.2,6.93405821099999));
#204671=CARTESIAN_POINT('Ctrl Pts',(8.43538541199995,11.6,6.93405821099999));
#204672=CARTESIAN_POINT('Ctrl Pts',(8.43266435299994,15.2,6.93303334799998));
#204673=CARTESIAN_POINT('Ctrl Pts',(8.43266435299994,11.6,6.93303334799998));
#204674=CARTESIAN_POINT('Ctrl Pts',(8.42994932099994,15.2,6.93200819099999));
#204675=CARTESIAN_POINT('Ctrl Pts',(8.42994932099994,11.6,6.93200819099999));
#204676=CARTESIAN_POINT('Ctrl Pts',(8.42724032099994,15.2,6.93098274799999));
#204677=CARTESIAN_POINT('Ctrl Pts',(8.42724032099994,11.6,6.93098274799999));
#204678=CARTESIAN_POINT('Ctrl Pts',(8.42453735899995,15.2,6.92995703099999));
#204679=CARTESIAN_POINT('Ctrl Pts',(8.42453735899995,11.6,6.92995703099999));
#204680=CARTESIAN_POINT('Ctrl Pts',(8.42184044199995,15.2,6.92893105099999));
#204681=CARTESIAN_POINT('Ctrl Pts',(8.42184044199995,11.6,6.92893105099999));
#204682=CARTESIAN_POINT('Ctrl Pts',(8.41914957699995,15.2,6.92790481899999));
#204683=CARTESIAN_POINT('Ctrl Pts',(8.41914957699995,11.6,6.92790481899999));
#204684=CARTESIAN_POINT('Ctrl Pts',(8.41646477099994,15.2,6.92687834499999));
#204685=CARTESIAN_POINT('Ctrl Pts',(8.41646477099994,11.6,6.92687834499999));
#204686=CARTESIAN_POINT('Ctrl Pts',(8.41378603099994,15.2,6.92585164199999));
#204687=CARTESIAN_POINT('Ctrl Pts',(8.41378603099994,11.6,6.92585164199999));
#204688=CARTESIAN_POINT('Ctrl Pts',(8.41111335999994,15.2,6.92482471999998));
#204689=CARTESIAN_POINT('Ctrl Pts',(8.41111335999994,11.6,6.92482471999998));
#204690=CARTESIAN_POINT('Ctrl Pts',(8.40844676899994,15.2,6.92379758999999));
#204691=CARTESIAN_POINT('Ctrl Pts',(8.40844676899994,11.6,6.92379758999999));
#204692=CARTESIAN_POINT('Ctrl Pts',(8.40578626199994,15.2,6.92277026299998));
#204693=CARTESIAN_POINT('Ctrl Pts',(8.40578626199994,11.6,6.92277026299998));
#204694=CARTESIAN_POINT('Ctrl Pts',(8.40313184599994,15.2,6.92174275099998));
#204695=CARTESIAN_POINT('Ctrl Pts',(8.40313184599994,11.6,6.92174275099998));
#204696=CARTESIAN_POINT('Ctrl Pts',(8.40048352899995,15.2,6.92071506499998));
#204697=CARTESIAN_POINT('Ctrl Pts',(8.40048352899995,11.6,6.92071506499998));
#204698=CARTESIAN_POINT('Ctrl Pts',(8.39784131599994,15.2,6.91968721599999));
#204699=CARTESIAN_POINT('Ctrl Pts',(8.39784131599994,11.6,6.91968721599999));
#204700=CARTESIAN_POINT('Ctrl Pts',(8.39520521499994,15.2,6.91865921399998));
#204701=CARTESIAN_POINT('Ctrl Pts',(8.39520521499994,11.6,6.91865921399998));
#204702=CARTESIAN_POINT('Ctrl Pts',(8.39257523199995,15.2,6.91763107399999));
#204703=CARTESIAN_POINT('Ctrl Pts',(8.39257523199995,11.6,6.91763107399999));
#204704=CARTESIAN_POINT('Ctrl Pts',(8.38995137299994,15.2,6.91660280399999));
#204705=CARTESIAN_POINT('Ctrl Pts',(8.38995137299994,11.6,6.91660280399999));
#204706=CARTESIAN_POINT('Ctrl Pts',(8.38733364499994,15.2,6.91557441599999));
#204707=CARTESIAN_POINT('Ctrl Pts',(8.38733364499994,11.6,6.91557441599999));
#204708=CARTESIAN_POINT('Ctrl Pts',(8.38472205599994,15.2,6.91454592099999));
#204709=CARTESIAN_POINT('Ctrl Pts',(8.38472205599994,11.6,6.91454592099999));
#204710=CARTESIAN_POINT('Ctrl Pts',(8.38211660999994,15.2,6.91351733199999));
#204711=CARTESIAN_POINT('Ctrl Pts',(8.38211660999994,11.6,6.91351733199999));
#204712=CARTESIAN_POINT('Ctrl Pts',(8.37951731699994,15.2,6.91248865999999));
#204713=CARTESIAN_POINT('Ctrl Pts',(8.37951731699994,11.6,6.91248865999999));
#204714=CARTESIAN_POINT('Ctrl Pts',(8.37692418099994,15.2,6.91145991599999));
#204715=CARTESIAN_POINT('Ctrl Pts',(8.37692418099994,11.6,6.91145991599999));
#204716=CARTESIAN_POINT('Ctrl Pts',(8.37433721099995,15.2,6.91043111099999));
#204717=CARTESIAN_POINT('Ctrl Pts',(8.37433721099995,11.6,6.91043111099999));
#204718=CARTESIAN_POINT('Ctrl Pts',(8.37175641099994,15.2,6.90940225799999));
#204719=CARTESIAN_POINT('Ctrl Pts',(8.37175641099994,11.6,6.90940225799999));
#204720=CARTESIAN_POINT('Ctrl Pts',(8.36918178899994,15.2,6.90837336799999));
#204721=CARTESIAN_POINT('Ctrl Pts',(8.36918178899994,11.6,6.90837336799999));
#204722=CARTESIAN_POINT('Ctrl Pts',(8.36661335299994,15.2,6.90734445299999));
#204723=CARTESIAN_POINT('Ctrl Pts',(8.36661335299994,11.6,6.90734445299999));
#204724=CARTESIAN_POINT('Ctrl Pts',(8.36405110799994,15.2,6.90631552499998));
#204725=CARTESIAN_POINT('Ctrl Pts',(8.36405110799994,11.6,6.90631552499998));
#204726=CARTESIAN_POINT('Ctrl Pts',(8.36149506199994,15.2,6.90528659299999));
#204727=CARTESIAN_POINT('Ctrl Pts',(8.36149506199994,11.6,6.90528659299999));
#204728=CARTESIAN_POINT('Ctrl Pts',(8.35894522099995,15.2,6.90425767199999));
#204729=CARTESIAN_POINT('Ctrl Pts',(8.35894522099995,11.6,6.90425767199999));
#204730=CARTESIAN_POINT('Ctrl Pts',(8.35640158999994,15.2,6.90322877199999));
#204731=CARTESIAN_POINT('Ctrl Pts',(8.35640158999994,11.6,6.90322877199999));
#204732=CARTESIAN_POINT('Ctrl Pts',(8.35386417999995,15.2,6.90219990599999));
#204733=CARTESIAN_POINT('Ctrl Pts',(8.35386417999995,11.6,6.90219990599999));
#204734=CARTESIAN_POINT('Ctrl Pts',(8.35133299399994,15.2,6.90117108499999));
#204735=CARTESIAN_POINT('Ctrl Pts',(8.35133299399994,11.6,6.90117108499999));
#204736=CARTESIAN_POINT('Ctrl Pts',(8.34880804099994,15.2,6.90014232099998));
#204737=CARTESIAN_POINT('Ctrl Pts',(8.34880804099994,11.6,6.90014232099998));
#204738=CARTESIAN_POINT('Ctrl Pts',(8.34628932799994,15.2,6.89911362499998));
#204739=CARTESIAN_POINT('Ctrl Pts',(8.34628932799994,11.6,6.89911362499998));
#204740=CARTESIAN_POINT('Ctrl Pts',(8.34377685899995,15.2,6.89808501099999));
#204741=CARTESIAN_POINT('Ctrl Pts',(8.34377685899995,11.6,6.89808501099999));
#204742=CARTESIAN_POINT('Ctrl Pts',(8.34127064199994,15.2,6.89705648999999));
#204743=CARTESIAN_POINT('Ctrl Pts',(8.34127064199994,11.6,6.89705648999999));
#204744=CARTESIAN_POINT('Ctrl Pts',(8.33877068699995,15.2,6.89602807399999));
#204745=CARTESIAN_POINT('Ctrl Pts',(8.33877068699995,11.6,6.89602807399999));
#204746=CARTESIAN_POINT('Ctrl Pts',(8.33627699599995,15.2,6.89499977499998));
#204747=CARTESIAN_POINT('Ctrl Pts',(8.33627699599995,11.6,6.89499977499998));
#204748=CARTESIAN_POINT('Ctrl Pts',(8.33378957899994,15.2,6.89397160599999));
#204749=CARTESIAN_POINT('Ctrl Pts',(8.33378957899994,11.6,6.89397160599999));
#204750=CARTESIAN_POINT('Ctrl Pts',(8.33130844099994,15.2,6.89294357699998));
#204751=CARTESIAN_POINT('Ctrl Pts',(8.33130844099994,11.6,6.89294357699998));
#204752=CARTESIAN_POINT('Ctrl Pts',(8.32883359199995,15.2,6.89191570199998));
#204753=CARTESIAN_POINT('Ctrl Pts',(8.32883359199995,11.6,6.89191570199998));
#204754=CARTESIAN_POINT('Ctrl Pts',(8.32636503499994,15.2,6.89088799199999));
#204755=CARTESIAN_POINT('Ctrl Pts',(8.32636503499994,11.6,6.89088799199999));
#204756=CARTESIAN_POINT('Ctrl Pts',(8.32390277799994,15.2,6.88986046099998));
#204757=CARTESIAN_POINT('Ctrl Pts',(8.32390277799994,11.6,6.88986046099998));
#204758=CARTESIAN_POINT('Ctrl Pts',(8.32144682899994,15.2,6.88883311999999));
#204759=CARTESIAN_POINT('Ctrl Pts',(8.32144682899994,11.6,6.88883311999999));
#204760=CARTESIAN_POINT('Ctrl Pts',(8.31899719499994,15.2,6.88780598099999));
#204761=CARTESIAN_POINT('Ctrl Pts',(8.31899719499994,11.6,6.88780598099999));
#204762=CARTESIAN_POINT('Ctrl Pts',(8.31655388099995,15.2,6.88677905699999));
#204763=CARTESIAN_POINT('Ctrl Pts',(8.31655388099995,11.6,6.88677905699999));
#204764=CARTESIAN_POINT('Ctrl Pts',(8.31411689599994,15.2,6.88575236099998));
#204765=CARTESIAN_POINT('Ctrl Pts',(8.31411689599994,11.6,6.88575236099998));
#204766=CARTESIAN_POINT('Ctrl Pts',(8.31168624599994,15.2,6.88472590299998));
#204767=CARTESIAN_POINT('Ctrl Pts',(8.31168624599994,11.6,6.88472590299998));
#204768=CARTESIAN_POINT('Ctrl Pts',(8.30926193799994,15.2,6.88369969999999));
#204769=CARTESIAN_POINT('Ctrl Pts',(8.30926193799994,11.6,6.88369969999999));
#204770=CARTESIAN_POINT('Ctrl Pts',(8.30684397799994,15.2,6.88267375999998));
#204771=CARTESIAN_POINT('Ctrl Pts',(8.30684397799994,11.6,6.88267375999998));
#204772=CARTESIAN_POINT('Ctrl Pts',(8.30443237399994,15.2,6.88164809699998));
#204773=CARTESIAN_POINT('Ctrl Pts',(8.30443237399994,11.6,6.88164809699998));
#204774=CARTESIAN_POINT('Ctrl Pts',(8.30202713399994,15.2,6.88062272299998));
#204775=CARTESIAN_POINT('Ctrl Pts',(8.30202713399994,11.6,6.88062272299998));
#204776=CARTESIAN_POINT('Ctrl Pts',(8.29962826099995,15.2,6.87959765299999));
#204777=CARTESIAN_POINT('Ctrl Pts',(8.29962826099995,11.6,6.87959765299999));
#204778=CARTESIAN_POINT('Ctrl Pts',(8.29723576699994,15.2,6.87857289799998));
#204779=CARTESIAN_POINT('Ctrl Pts',(8.29723576699994,11.6,6.87857289799998));
#204780=CARTESIAN_POINT('Ctrl Pts',(8.29484965599995,15.2,6.87754846999999));
#204781=CARTESIAN_POINT('Ctrl Pts',(8.29484965599995,11.6,6.87754846999999));
#204782=CARTESIAN_POINT('Ctrl Pts',(8.29246993599994,15.2,6.87652438299998));
#204783=CARTESIAN_POINT('Ctrl Pts',(8.29246993599994,11.6,6.87652438299998));
#204784=CARTESIAN_POINT('Ctrl Pts',(8.29009661399994,15.2,6.87550064899998));
#204785=CARTESIAN_POINT('Ctrl Pts',(8.29009661399994,11.6,6.87550064899998));
#204786=CARTESIAN_POINT('Ctrl Pts',(8.28772969499994,15.2,6.87447728199999));
#204787=CARTESIAN_POINT('Ctrl Pts',(8.28772969499994,11.6,6.87447728199999));
#204788=CARTESIAN_POINT('Ctrl Pts',(8.28536918899994,15.2,6.87345429299998));
#204789=CARTESIAN_POINT('Ctrl Pts',(8.28536918899994,11.6,6.87345429299998));
#204790=CARTESIAN_POINT('Ctrl Pts',(8.28301510099994,15.2,6.87243169599999));
#204791=CARTESIAN_POINT('Ctrl Pts',(8.28301510099994,11.6,6.87243169599999));
#204792=CARTESIAN_POINT('Ctrl Pts',(8.28066743899995,15.2,6.87140950299998));
#204793=CARTESIAN_POINT('Ctrl Pts',(8.28066743899995,11.6,6.87140950299998));
#204794=CARTESIAN_POINT('Ctrl Pts',(8.27832620999994,15.2,6.87038772899999));
#204795=CARTESIAN_POINT('Ctrl Pts',(8.27832620999994,11.6,6.87038772899999));
#204796=CARTESIAN_POINT('Ctrl Pts',(8.27599141999994,15.2,6.86936638599998));
#204797=CARTESIAN_POINT('Ctrl Pts',(8.27599141999994,11.6,6.86936638599998));
#204798=CARTESIAN_POINT('Ctrl Pts',(8.27366307799995,15.2,6.86834548599998));
#204799=CARTESIAN_POINT('Ctrl Pts',(8.27366307799995,11.6,6.86834548599998));
#204800=CARTESIAN_POINT('Ctrl Pts',(8.27134118899994,15.2,6.86732504299999));
#204801=CARTESIAN_POINT('Ctrl Pts',(8.27134118899994,11.6,6.86732504299999));
#204802=CARTESIAN_POINT('Ctrl Pts',(8.26902576199994,15.2,6.86630506999999));
#204803=CARTESIAN_POINT('Ctrl Pts',(8.26902576199994,11.6,6.86630506999999));
#204804=CARTESIAN_POINT('Ctrl Pts',(8.26671680299994,15.2,6.86528557999999));
#204805=CARTESIAN_POINT('Ctrl Pts',(8.26671680299994,11.6,6.86528557999999));
#204806=CARTESIAN_POINT('Ctrl Pts',(8.26441431799994,15.2,6.86426658699999));
#204807=CARTESIAN_POINT('Ctrl Pts',(8.26441431799994,11.6,6.86426658699999));
#204808=CARTESIAN_POINT('Ctrl Pts',(8.26211831599995,15.2,6.86324810299999));
#204809=CARTESIAN_POINT('Ctrl Pts',(8.26211831599995,11.6,6.86324810299999));
#204810=CARTESIAN_POINT('Ctrl Pts',(8.25982880499994,15.2,6.86223014299999));
#204811=CARTESIAN_POINT('Ctrl Pts',(8.25982880499994,11.6,6.86223014299999));
#204812=CARTESIAN_POINT('Ctrl Pts',(8.25754578899994,15.2,6.86121271799998));
#204813=CARTESIAN_POINT('Ctrl Pts',(8.25754578899994,11.6,6.86121271799998));
#204814=CARTESIAN_POINT('Ctrl Pts',(8.25526927699994,15.2,6.86019584399999));
#204815=CARTESIAN_POINT('Ctrl Pts',(8.25526927699994,11.6,6.86019584399999));
#204816=CARTESIAN_POINT('Ctrl Pts',(8.25299927599995,15.2,6.85917953199999));
#204817=CARTESIAN_POINT('Ctrl Pts',(8.25299927599995,11.6,6.85917953199999));
#204818=CARTESIAN_POINT('Ctrl Pts',(8.25073579299995,15.2,6.85816379699999));
#204819=CARTESIAN_POINT('Ctrl Pts',(8.25073579299995,11.6,6.85816379699999));
#204820=CARTESIAN_POINT('Ctrl Pts',(8.24847883499995,15.2,6.85714865199999));
#204821=CARTESIAN_POINT('Ctrl Pts',(8.24847883499995,11.6,6.85714865199999));
#204822=CARTESIAN_POINT('Ctrl Pts',(8.24622840999995,15.2,6.85613411099999));
#204823=CARTESIAN_POINT('Ctrl Pts',(8.24622840999995,11.6,6.85613411099999));
#204824=CARTESIAN_POINT('Ctrl Pts',(8.24398452499995,15.2,6.85512018699999));
#204825=CARTESIAN_POINT('Ctrl Pts',(8.24398452499995,11.6,6.85512018699999));
#204826=CARTESIAN_POINT('Ctrl Pts',(8.24174718699994,15.2,6.85410689399998));
#204827=CARTESIAN_POINT('Ctrl Pts',(8.24174718699994,11.6,6.85410689399998));
#204828=CARTESIAN_POINT('Ctrl Pts',(8.23951640199994,15.2,6.85309424599998));
#204829=CARTESIAN_POINT('Ctrl Pts',(8.23951640199994,11.6,6.85309424599998));
#204830=CARTESIAN_POINT('Ctrl Pts',(8.23729217799994,15.2,6.85208225499998));
#204831=CARTESIAN_POINT('Ctrl Pts',(8.23729217799994,11.6,6.85208225499998));
#204832=CARTESIAN_POINT('Ctrl Pts',(8.23507452399994,15.2,6.85107093599999));
#204833=CARTESIAN_POINT('Ctrl Pts',(8.23507452399994,11.6,6.85107093599999));
#204834=CARTESIAN_POINT('Ctrl Pts',(8.23286344499994,15.2,6.85006030399999));
#204835=CARTESIAN_POINT('Ctrl Pts',(8.23286344499994,11.6,6.85006030399999));
#204836=CARTESIAN_POINT('Ctrl Pts',(8.23065894899995,15.2,6.84905037099998));
#204837=CARTESIAN_POINT('Ctrl Pts',(8.23065894899995,11.6,6.84905037099998));
#204838=CARTESIAN_POINT('Ctrl Pts',(8.22846104299994,15.2,6.84804115099999));
#204839=CARTESIAN_POINT('Ctrl Pts',(8.22846104299994,11.6,6.84804115099999));
#204840=CARTESIAN_POINT('Ctrl Pts',(8.22626973499995,15.2,6.84703266099999));
#204841=CARTESIAN_POINT('Ctrl Pts',(8.22626973499995,11.6,6.84703266099999));
#204842=CARTESIAN_POINT('Ctrl Pts',(8.22408503299994,15.2,6.84602490999998));
#204843=CARTESIAN_POINT('Ctrl Pts',(8.22408503299994,11.6,6.84602490999998));
#204844=CARTESIAN_POINT('Ctrl Pts',(8.22190694099995,15.2,6.84501791499999));
#204845=CARTESIAN_POINT('Ctrl Pts',(8.22190694099995,11.6,6.84501791499999));
#204846=CARTESIAN_POINT('Ctrl Pts',(8.21973547099994,15.2,6.84401169099999));
#204847=CARTESIAN_POINT('Ctrl Pts',(8.21973547099994,11.6,6.84401169099999));
#204848=CARTESIAN_POINT('Ctrl Pts',(8.21757062599995,15.2,6.84300624899999));
#204849=CARTESIAN_POINT('Ctrl Pts',(8.21757062599995,11.6,6.84300624899999));
#204850=CARTESIAN_POINT('Ctrl Pts',(8.21541241599994,15.2,6.84200160599998));
#204851=CARTESIAN_POINT('Ctrl Pts',(8.21541241599994,11.6,6.84200160599998));
#204852=CARTESIAN_POINT('Ctrl Pts',(8.21326084699994,15.2,6.84099777499998));
#204853=CARTESIAN_POINT('Ctrl Pts',(8.21326084699994,11.6,6.84099777499998));
#204854=CARTESIAN_POINT('Ctrl Pts',(8.21111592699994,15.2,6.83999476999999));
#204855=CARTESIAN_POINT('Ctrl Pts',(8.21111592699994,11.6,6.83999476999999));
#204856=CARTESIAN_POINT('Ctrl Pts',(8.20897766399994,15.2,6.83899260599999));
#204857=CARTESIAN_POINT('Ctrl Pts',(8.20897766399994,11.6,6.83899260599999));
#204858=CARTESIAN_POINT('Ctrl Pts',(8.20684606299995,15.2,6.83799129599999));
#204859=CARTESIAN_POINT('Ctrl Pts',(8.20684606299995,11.6,6.83799129599999));
#204860=CARTESIAN_POINT('Ctrl Pts',(8.20472113499994,15.2,6.83699085699998));
#204861=CARTESIAN_POINT('Ctrl Pts',(8.20472113499994,11.6,6.83699085699998));
#204862=CARTESIAN_POINT('Ctrl Pts',(8.20260288499994,15.2,6.83599130199998));
#204863=CARTESIAN_POINT('Ctrl Pts',(8.20260288499994,11.6,6.83599130199998));
#204864=CARTESIAN_POINT('Ctrl Pts',(8.20049131999994,15.2,6.83499264399998));
#204865=CARTESIAN_POINT('Ctrl Pts',(8.20049131999994,11.6,6.83499264399998));
#204866=CARTESIAN_POINT('Ctrl Pts',(8.19838644899994,15.2,6.83399490099998));
#204867=CARTESIAN_POINT('Ctrl Pts',(8.19838644899994,11.6,6.83399490099998));
#204868=CARTESIAN_POINT('Ctrl Pts',(8.19628827799994,15.2,6.83299808399998));
#204869=CARTESIAN_POINT('Ctrl Pts',(8.19628827799994,11.6,6.83299808399998));
#204870=CARTESIAN_POINT('Ctrl Pts',(8.19419681699994,15.2,6.83200220999999));
#204871=CARTESIAN_POINT('Ctrl Pts',(8.19419681699994,11.6,6.83200220999999));
#204872=CARTESIAN_POINT('Ctrl Pts',(8.19211206999995,15.2,6.83100729199998));
#204873=CARTESIAN_POINT('Ctrl Pts',(8.19211206999995,11.6,6.83100729199998));
#204874=CARTESIAN_POINT('Ctrl Pts',(8.19003404699994,15.2,6.83001334599999));
#204875=CARTESIAN_POINT('Ctrl Pts',(8.19003404699994,11.6,6.83001334599999));
#204876=CARTESIAN_POINT('Ctrl Pts',(8.18796275399994,15.2,6.82902038599998));
#204877=CARTESIAN_POINT('Ctrl Pts',(8.18796275399994,11.6,6.82902038599998));
#204878=CARTESIAN_POINT('Ctrl Pts',(8.18589819999995,15.2,6.82802842899999));
#204879=CARTESIAN_POINT('Ctrl Pts',(8.18589819999995,11.6,6.82802842899999));
#204880=CARTESIAN_POINT('Ctrl Pts',(8.18384039099995,15.2,6.82703748699999));
#204881=CARTESIAN_POINT('Ctrl Pts',(8.18384039099995,11.6,6.82703748699999));
#204882=CARTESIAN_POINT('Ctrl Pts',(8.18178933599994,15.2,6.82604757499998));
#204883=CARTESIAN_POINT('Ctrl Pts',(8.18178933599994,11.6,6.82604757499998));
#204884=CARTESIAN_POINT('Ctrl Pts',(8.17974504099995,15.2,6.82505870999999));
#204885=CARTESIAN_POINT('Ctrl Pts',(8.17974504099995,11.6,6.82505870999999));
#204886=CARTESIAN_POINT('Ctrl Pts',(8.17770751499994,15.2,6.82407090699999));
#204887=CARTESIAN_POINT('Ctrl Pts',(8.17770751499994,11.6,6.82407090699999));
#204888=CARTESIAN_POINT('Ctrl Pts',(8.17567676399995,15.2,6.82308417899999));
#204889=CARTESIAN_POINT('Ctrl Pts',(8.17567676399995,11.6,6.82308417899999));
#204890=CARTESIAN_POINT('Ctrl Pts',(8.17365279699995,15.2,6.82209854299998));
#204891=CARTESIAN_POINT('Ctrl Pts',(8.17365279699995,11.6,6.82209854299998));
#204892=CARTESIAN_POINT('Ctrl Pts',(8.17163562099994,15.2,6.82111401199998));
#204893=CARTESIAN_POINT('Ctrl Pts',(8.17163562099994,11.6,6.82111401199998));
#204894=CARTESIAN_POINT('Ctrl Pts',(8.16962524399995,15.2,6.82013060399999));
#204895=CARTESIAN_POINT('Ctrl Pts',(8.16962524399995,11.6,6.82013060399999));
#204896=CARTESIAN_POINT('Ctrl Pts',(8.16762167299995,15.2,6.81914833299999));
#204897=CARTESIAN_POINT('Ctrl Pts',(8.16762167299995,11.6,6.81914833299999));
#204898=CARTESIAN_POINT('Ctrl Pts',(8.16562491599995,15.2,6.81816721399999));
#204899=CARTESIAN_POINT('Ctrl Pts',(8.16562491599995,11.6,6.81816721399999));
#204900=CARTESIAN_POINT('Ctrl Pts',(8.16363497999994,15.2,6.81718726399998));
#204901=CARTESIAN_POINT('Ctrl Pts',(8.16363497999994,11.6,6.81718726399998));
#204902=CARTESIAN_POINT('Ctrl Pts',(8.16165187399994,15.2,6.81620849599998));
#204903=CARTESIAN_POINT('Ctrl Pts',(8.16165187399994,11.6,6.81620849599998));
#204904=CARTESIAN_POINT('Ctrl Pts',(8.15967560399995,15.2,6.81523092699998));
#204905=CARTESIAN_POINT('Ctrl Pts',(8.15967560399995,11.6,6.81523092699998));
#204906=CARTESIAN_POINT('Ctrl Pts',(8.15770618099994,15.2,6.81425457199998));
#204907=CARTESIAN_POINT('Ctrl Pts',(8.15770618099994,11.6,6.81425457199998));
#204908=CARTESIAN_POINT('Ctrl Pts',(8.15574360699994,15.2,6.81327944699999));
#204909=CARTESIAN_POINT('Ctrl Pts',(8.15574360699994,11.6,6.81327944699999));
#204910=CARTESIAN_POINT('Ctrl Pts',(8.15378789499994,15.2,6.81230556799999));
#204911=CARTESIAN_POINT('Ctrl Pts',(8.15378789499994,11.6,6.81230556799999));
#204912=CARTESIAN_POINT('Ctrl Pts',(8.15183904999994,15.2,6.81133294999999));
#204913=CARTESIAN_POINT('Ctrl Pts',(8.15183904999994,11.6,6.81133294999999));
#204914=CARTESIAN_POINT('Ctrl Pts',(8.14989708099995,15.2,6.81036160899998));
#204915=CARTESIAN_POINT('Ctrl Pts',(8.14989708099995,11.6,6.81036160899998));
#204916=CARTESIAN_POINT('Ctrl Pts',(8.14796199499994,15.2,6.80939156099999));
#204917=CARTESIAN_POINT('Ctrl Pts',(8.14796199499994,11.6,6.80939156099999));
#204918=CARTESIAN_POINT('Ctrl Pts',(8.14603379999994,15.2,6.80842282199999));
#204919=CARTESIAN_POINT('Ctrl Pts',(8.14603379999994,11.6,6.80842282199999));
#204920=CARTESIAN_POINT('Ctrl Pts',(8.14411250399995,15.2,6.80745540699998));
#204921=CARTESIAN_POINT('Ctrl Pts',(8.14411250399995,11.6,6.80745540699998));
#204922=CARTESIAN_POINT('Ctrl Pts',(8.14219811399994,15.2,6.80648933399999));
#204923=CARTESIAN_POINT('Ctrl Pts',(8.14219811399994,11.6,6.80648933399999));
#204924=CARTESIAN_POINT('Ctrl Pts',(8.14029063899994,15.2,6.80552461599999));
#204925=CARTESIAN_POINT('Ctrl Pts',(8.14029063899994,11.6,6.80552461599999));
#204926=CARTESIAN_POINT('Ctrl Pts',(8.13839008599994,15.2,6.80456127199999));
#204927=CARTESIAN_POINT('Ctrl Pts',(8.13839008599994,11.6,6.80456127199999));
#204928=CARTESIAN_POINT('Ctrl Pts',(8.13649646199995,15.2,6.80359931699999));
#204929=CARTESIAN_POINT('Ctrl Pts',(8.13649646199995,11.6,6.80359931699999));
#204930=CARTESIAN_POINT('Ctrl Pts',(8.13460977799994,15.2,6.80263876599999));
#204931=CARTESIAN_POINT('Ctrl Pts',(8.13460977799994,11.6,6.80263876599999));
#204932=CARTESIAN_POINT('Ctrl Pts',(8.13273003799994,15.2,6.80167963699999));
#204933=CARTESIAN_POINT('Ctrl Pts',(8.13273003799994,11.6,6.80167963699999));
#204934=CARTESIAN_POINT('Ctrl Pts',(8.13085725199995,15.2,6.80072194599998));
#204935=CARTESIAN_POINT('Ctrl Pts',(8.13085725199995,11.6,6.80072194599998));
#204936=CARTESIAN_POINT('Ctrl Pts',(8.12899142799994,15.2,6.79976570899999));
#204937=CARTESIAN_POINT('Ctrl Pts',(8.12899142799994,11.6,6.79976570899999));
#204938=CARTESIAN_POINT('Ctrl Pts',(8.12713257399994,15.2,6.79881094299999));
#204939=CARTESIAN_POINT('Ctrl Pts',(8.12713257399994,11.6,6.79881094299999));
#204940=CARTESIAN_POINT('Ctrl Pts',(8.12528069599994,15.2,6.79785766399998));
#204941=CARTESIAN_POINT('Ctrl Pts',(8.12528069599994,11.6,6.79785766399998));
#204942=CARTESIAN_POINT('Ctrl Pts',(8.12343580399994,15.2,6.79690588799998));
#204943=CARTESIAN_POINT('Ctrl Pts',(8.12343580399994,11.6,6.79690588799998));
#204944=CARTESIAN_POINT('Ctrl Pts',(8.12159790499994,15.2,6.79595563299999));
#204945=CARTESIAN_POINT('Ctrl Pts',(8.12159790499994,11.6,6.79595563299999));
#204946=CARTESIAN_POINT('Ctrl Pts',(8.11976700799995,15.2,6.79500691499998));
#204947=CARTESIAN_POINT('Ctrl Pts',(8.11976700799995,11.6,6.79500691499998));
#204948=CARTESIAN_POINT('Ctrl Pts',(8.11794311899994,15.2,6.79405974999998));
#204949=CARTESIAN_POINT('Ctrl Pts',(8.11794311899994,11.6,6.79405974999998));
#204950=CARTESIAN_POINT('Ctrl Pts',(8.11612624899994,15.2,6.79311415699999));
#204951=CARTESIAN_POINT('Ctrl Pts',(8.11612624899994,11.6,6.79311415699999));
#204952=CARTESIAN_POINT('Ctrl Pts',(8.11431640299995,15.2,6.79217015099999));
#204953=CARTESIAN_POINT('Ctrl Pts',(8.11431640299995,11.6,6.79217015099999));
#204954=CARTESIAN_POINT('Ctrl Pts',(8.11251358999994,15.2,6.79122774899999));
#204955=CARTESIAN_POINT('Ctrl Pts',(8.11251358999994,11.6,6.79122774899999));
#204956=CARTESIAN_POINT('Ctrl Pts',(8.11071781999994,15.2,6.79028696799998));
#204957=CARTESIAN_POINT('Ctrl Pts',(8.11071781999994,11.6,6.79028696799998));
#204958=CARTESIAN_POINT('Ctrl Pts',(8.10892909899994,15.2,6.78934782499999));
#204959=CARTESIAN_POINT('Ctrl Pts',(8.10892909899994,11.6,6.78934782499999));
#204960=CARTESIAN_POINT('Ctrl Pts',(8.10714743499994,15.2,6.78841033799999));
#204961=CARTESIAN_POINT('Ctrl Pts',(8.10714743499994,11.6,6.78841033799999));
#204962=CARTESIAN_POINT('Ctrl Pts',(8.10537283599994,15.2,6.78747452299999));
#204963=CARTESIAN_POINT('Ctrl Pts',(8.10537283599994,11.6,6.78747452299999));
#204964=CARTESIAN_POINT('Ctrl Pts',(8.10360531199994,15.2,6.78654039899998));
#204965=CARTESIAN_POINT('Ctrl Pts',(8.10360531199994,11.6,6.78654039899998));
#204966=CARTESIAN_POINT('Ctrl Pts',(8.10184486799994,15.2,6.78560798099999));
#204967=CARTESIAN_POINT('Ctrl Pts',(8.10184486799994,11.6,6.78560798099999));
#204968=CARTESIAN_POINT('Ctrl Pts',(8.10009151599994,15.2,6.78467728899999));
#204969=CARTESIAN_POINT('Ctrl Pts',(8.10009151599994,11.6,6.78467728899999));
#204970=CARTESIAN_POINT('Ctrl Pts',(8.09834526099994,15.2,6.78374833799998));
#204971=CARTESIAN_POINT('Ctrl Pts',(8.09834526099994,11.6,6.78374833799998));
#204972=CARTESIAN_POINT('Ctrl Pts',(8.09660611299994,15.2,6.78282114599998));
#204973=CARTESIAN_POINT('Ctrl Pts',(8.09660611299994,11.6,6.78282114599998));
#204974=CARTESIAN_POINT('Ctrl Pts',(8.09487407999994,15.2,6.78189573099999));
#204975=CARTESIAN_POINT('Ctrl Pts',(8.09487407999994,11.6,6.78189573099999));
#204976=CARTESIAN_POINT('Ctrl Pts',(8.09314916899995,15.2,6.78097211099999));
#204977=CARTESIAN_POINT('Ctrl Pts',(8.09314916899995,11.6,6.78097211099999));
#204978=CARTESIAN_POINT('Ctrl Pts',(8.09143138899995,15.2,6.78005030299998));
#204979=CARTESIAN_POINT('Ctrl Pts',(8.09143138899995,11.6,6.78005030299998));
#204980=CARTESIAN_POINT('Ctrl Pts',(8.08972074799994,15.2,6.77913032599999));
#204981=CARTESIAN_POINT('Ctrl Pts',(8.08972074799994,11.6,6.77913032599999));
#204982=CARTESIAN_POINT('Ctrl Pts',(8.08801725499994,15.2,6.77821219599998));
#204983=CARTESIAN_POINT('Ctrl Pts',(8.08801725499994,11.6,6.77821219599998));
#204984=CARTESIAN_POINT('Ctrl Pts',(8.08632091699995,15.2,6.77729592999999));
#204985=CARTESIAN_POINT('Ctrl Pts',(8.08632091699995,11.6,6.77729592999999));
#204986=CARTESIAN_POINT('Ctrl Pts',(8.08463174399994,15.2,6.77638154999999));
#204987=CARTESIAN_POINT('Ctrl Pts',(8.08463174399994,11.6,6.77638154999999));
#204988=CARTESIAN_POINT('Ctrl Pts',(8.08294974399994,15.2,6.77546907099998));
#204989=CARTESIAN_POINT('Ctrl Pts',(8.08294974399994,11.6,6.77546907099998));
#204990=CARTESIAN_POINT('Ctrl Pts',(8.08127492299995,15.2,6.77455851099998));
#204991=CARTESIAN_POINT('Ctrl Pts',(8.08127492299995,11.6,6.77455851099998));
#204992=CARTESIAN_POINT('Ctrl Pts',(8.07960729299994,15.2,6.77364988999998));
#204993=CARTESIAN_POINT('Ctrl Pts',(8.07960729299994,11.6,6.77364988999998));
#204994=CARTESIAN_POINT('Ctrl Pts',(8.07794685899994,15.2,6.77274322499999));
#204995=CARTESIAN_POINT('Ctrl Pts',(8.07794685899994,11.6,6.77274322499999));
#204996=CARTESIAN_POINT('Ctrl Pts',(8.07629363199995,15.2,6.77183853299999));
#204997=CARTESIAN_POINT('Ctrl Pts',(8.07629363199995,11.6,6.77183853299999));
#204998=CARTESIAN_POINT('Ctrl Pts',(8.07464761799995,15.2,6.77093583499998));
#204999=CARTESIAN_POINT('Ctrl Pts',(8.07464761799995,11.6,6.77093583499998));
#205000=CARTESIAN_POINT('Ctrl Pts',(8.07300882799994,15.2,6.77003514799999));
#205001=CARTESIAN_POINT('Ctrl Pts',(8.07300882799994,11.6,6.77003514799999));
#205002=CARTESIAN_POINT('Ctrl Pts',(8.07137726799994,15.2,6.76913649099999));
#205003=CARTESIAN_POINT('Ctrl Pts',(8.07137726799994,11.6,6.76913649099999));
#205004=CARTESIAN_POINT('Ctrl Pts',(8.06975294899994,15.2,6.76823988099999));
#205005=CARTESIAN_POINT('Ctrl Pts',(8.06975294899994,11.6,6.76823988099999));
#205006=CARTESIAN_POINT('Ctrl Pts',(8.06813587699994,15.2,6.76734533899998));
#205007=CARTESIAN_POINT('Ctrl Pts',(8.06813587699994,11.6,6.76734533899998));
#205008=CARTESIAN_POINT('Ctrl Pts',(8.06652606199994,15.2,6.76645288099999));
#205009=CARTESIAN_POINT('Ctrl Pts',(8.06652606199994,11.6,6.76645288099999));
#205010=CARTESIAN_POINT('Ctrl Pts',(8.06492351199994,15.2,6.76556252899999));
#205011=CARTESIAN_POINT('Ctrl Pts',(8.06492351199994,11.6,6.76556252899999));
#205012=CARTESIAN_POINT('Ctrl Pts',(8.06332823499995,15.2,6.76467429899999));
#205013=CARTESIAN_POINT('Ctrl Pts',(8.06332823499995,11.6,6.76467429899999));
#205014=CARTESIAN_POINT('Ctrl Pts',(8.06174024099995,15.2,6.76378821199999));
#205015=CARTESIAN_POINT('Ctrl Pts',(8.06174024099995,11.6,6.76378821199999));
#205016=CARTESIAN_POINT('Ctrl Pts',(8.06015953799994,15.2,6.76290428499998));
#205017=CARTESIAN_POINT('Ctrl Pts',(8.06015953799994,11.6,6.76290428499998));
#205018=CARTESIAN_POINT('Ctrl Pts',(8.05858613399994,15.2,6.76202253899999));
#205019=CARTESIAN_POINT('Ctrl Pts',(8.05858613399994,11.6,6.76202253899999));
#205020=CARTESIAN_POINT('Ctrl Pts',(8.05702003799994,15.2,6.76114299299999));
#205021=CARTESIAN_POINT('Ctrl Pts',(8.05702003799994,11.6,6.76114299299999));
#205022=CARTESIAN_POINT('Ctrl Pts',(8.05546125799994,15.2,6.76026566499999));
#205023=CARTESIAN_POINT('Ctrl Pts',(8.05546125799994,11.6,6.76026566499999));
#205024=CARTESIAN_POINT('Ctrl Pts',(8.05390980499994,15.2,6.75939057399999));
#205025=CARTESIAN_POINT('Ctrl Pts',(8.05390980499994,11.6,6.75939057399999));
#205026=CARTESIAN_POINT('Ctrl Pts',(8.05236568499994,15.2,6.75851773999998));
#205027=CARTESIAN_POINT('Ctrl Pts',(8.05236568499994,11.6,6.75851773999998));
#205028=CARTESIAN_POINT('Ctrl Pts',(8.05082890799994,15.2,6.75764718399999));
#205029=CARTESIAN_POINT('Ctrl Pts',(8.05082890799994,11.6,6.75764718399999));
#205030=CARTESIAN_POINT('Ctrl Pts',(8.04929948099995,15.2,6.75677892399998));
#205031=CARTESIAN_POINT('Ctrl Pts',(8.04929948099995,11.6,6.75677892399998));
#205032=CARTESIAN_POINT('Ctrl Pts',(8.04777741499995,15.2,6.75591297799999));
#205033=CARTESIAN_POINT('Ctrl Pts',(8.04777741499995,11.6,6.75591297799999));
#205034=CARTESIAN_POINT('Ctrl Pts',(8.04626271799994,15.2,6.75504936999998));
#205035=CARTESIAN_POINT('Ctrl Pts',(8.04626271799994,11.6,6.75504936999998));
#205036=CARTESIAN_POINT('Ctrl Pts',(8.04475539899994,15.2,6.75418811499998));
#205037=CARTESIAN_POINT('Ctrl Pts',(8.04475539899994,11.6,6.75418811499998));
#205038=CARTESIAN_POINT('Ctrl Pts',(8.04325546599994,15.2,6.75332923599999));
#205039=CARTESIAN_POINT('Ctrl Pts',(8.04325546599994,11.6,6.75332923599999));
#205040=CARTESIAN_POINT('Ctrl Pts',(8.04176292899994,15.2,6.75247275199998));
#205041=CARTESIAN_POINT('Ctrl Pts',(8.04176292899994,11.6,6.75247275199998));
#205042=CARTESIAN_POINT('Ctrl Pts',(8.04027779499994,15.2,6.75161868299998));
#205043=CARTESIAN_POINT('Ctrl Pts',(8.04027779499994,11.6,6.75161868299998));
#205044=CARTESIAN_POINT('Ctrl Pts',(8.03880007499994,15.2,6.75076704899999));
#205045=CARTESIAN_POINT('Ctrl Pts',(8.03880007499994,11.6,6.75076704899999));
#205046=CARTESIAN_POINT('Ctrl Pts',(8.03732977699994,15.2,6.74991786899999));
#205047=CARTESIAN_POINT('Ctrl Pts',(8.03732977699994,11.6,6.74991786899999));
#205048=CARTESIAN_POINT('Ctrl Pts',(8.03586690899994,15.2,6.74907116499998));
#205049=CARTESIAN_POINT('Ctrl Pts',(8.03586690899994,11.6,6.74907116499998));
#205050=CARTESIAN_POINT('Ctrl Pts',(8.03441148099994,15.2,6.74822695799998));
#205051=CARTESIAN_POINT('Ctrl Pts',(8.03441148099994,11.6,6.74822695799998));
#205052=CARTESIAN_POINT('Ctrl Pts',(8.03296350099994,15.2,6.74738526499999));
#205053=CARTESIAN_POINT('Ctrl Pts',(8.03296350099994,11.6,6.74738526499999));
#205054=CARTESIAN_POINT('Ctrl Pts',(8.03152297999995,15.2,6.74654610999998));
#205055=CARTESIAN_POINT('Ctrl Pts',(8.03152297999995,11.6,6.74654610999998));
#205056=CARTESIAN_POINT('Ctrl Pts',(8.03008992399995,15.2,6.74570951199998));
#205057=CARTESIAN_POINT('Ctrl Pts',(8.03008992399995,11.6,6.74570951199998));
#205058=CARTESIAN_POINT('Ctrl Pts',(8.02866434499995,15.2,6.74487549099998));
#205059=CARTESIAN_POINT('Ctrl Pts',(8.02866434499995,11.6,6.74487549099998));
#205060=CARTESIAN_POINT('Ctrl Pts',(8.02724624999994,15.2,6.74404406999999));
#205061=CARTESIAN_POINT('Ctrl Pts',(8.02724624999994,11.6,6.74404406999999));
#205062=CARTESIAN_POINT('Ctrl Pts',(8.02583564899994,15.2,6.74321526699998));
#205063=CARTESIAN_POINT('Ctrl Pts',(8.02583564899994,11.6,6.74321526699998));
#205064=CARTESIAN_POINT('Ctrl Pts',(8.02443255099995,15.2,6.74238910499999));
#205065=CARTESIAN_POINT('Ctrl Pts',(8.02443255099995,11.6,6.74238910499999));
#205066=CARTESIAN_POINT('Ctrl Pts',(8.02303696499994,15.2,6.74156560299998));
#205067=CARTESIAN_POINT('Ctrl Pts',(8.02303696499994,11.6,6.74156560299998));
#205068=CARTESIAN_POINT('Ctrl Pts',(8.02164889999995,15.2,6.74074478499998));
#205069=CARTESIAN_POINT('Ctrl Pts',(8.02164889999995,11.6,6.74074478499998));
#205070=CARTESIAN_POINT('Ctrl Pts',(8.02026836499994,15.2,6.73992666999998));
#205071=CARTESIAN_POINT('Ctrl Pts',(8.02026836499994,11.6,6.73992666999998));
#205072=CARTESIAN_POINT('Ctrl Pts',(8.01889536899994,15.2,6.73911127899999));
#205073=CARTESIAN_POINT('Ctrl Pts',(8.01889536899994,11.6,6.73911127899999));
#205074=CARTESIAN_POINT('Ctrl Pts',(8.01752992299994,15.2,6.73829863499999));
#205075=CARTESIAN_POINT('Ctrl Pts',(8.01752992299994,11.6,6.73829863499999));
#205076=CARTESIAN_POINT('Ctrl Pts',(8.01617203399994,15.2,6.73748875799999));
#205077=CARTESIAN_POINT('Ctrl Pts',(8.01617203399994,11.6,6.73748875799999));
#205078=CARTESIAN_POINT('Ctrl Pts',(8.01482171199994,15.2,6.73668166999998));
#205079=CARTESIAN_POINT('Ctrl Pts',(8.01482171199994,11.6,6.73668166999998));
#205080=CARTESIAN_POINT('Ctrl Pts',(8.01347896699994,15.2,6.73587739199998));
#205081=CARTESIAN_POINT('Ctrl Pts',(8.01347896699994,11.6,6.73587739199998));
#205082=CARTESIAN_POINT('Ctrl Pts',(8.01214380699994,15.2,6.73507594799998));
#205083=CARTESIAN_POINT('Ctrl Pts',(8.01214380699994,11.6,6.73507594799998));
#205084=CARTESIAN_POINT('Ctrl Pts',(8.01081624199995,15.2,6.73427735699998));
#205085=CARTESIAN_POINT('Ctrl Pts',(8.01081624199995,11.6,6.73427735699998));
#205086=CARTESIAN_POINT('Ctrl Pts',(8.00949628099995,15.2,6.73348164099998));
#205087=CARTESIAN_POINT('Ctrl Pts',(8.00949628099995,11.6,6.73348164099998));
#205088=CARTESIAN_POINT('Ctrl Pts',(8.00818393499994,15.2,6.73268882499999));
#205089=CARTESIAN_POINT('Ctrl Pts',(8.00818393499994,11.6,6.73268882499999));
#205090=CARTESIAN_POINT('Ctrl Pts',(8.00687921199994,15.2,6.73189892799999));
#205091=CARTESIAN_POINT('Ctrl Pts',(8.00687921199994,11.6,6.73189892799999));
#205092=CARTESIAN_POINT('Ctrl Pts',(8.00558212099994,15.2,6.73111197299999));
#205093=CARTESIAN_POINT('Ctrl Pts',(8.00558212099994,11.6,6.73111197299999));
#205094=CARTESIAN_POINT('Ctrl Pts',(8.00429267199994,15.2,6.73032798199999));
#205095=CARTESIAN_POINT('Ctrl Pts',(8.00429267199994,11.6,6.73032798199999));
#205096=CARTESIAN_POINT('Ctrl Pts',(8.00301087399994,15.2,6.72954697899999));
#205097=CARTESIAN_POINT('Ctrl Pts',(8.00301087399994,11.6,6.72954697899999));
#205098=CARTESIAN_POINT('Ctrl Pts',(8.00173673799994,15.2,6.72876898499998));
#205099=CARTESIAN_POINT('Ctrl Pts',(8.00173673799994,11.6,6.72876898499998));
#205100=CARTESIAN_POINT('Ctrl Pts',(8.00047027299994,15.2,6.72799402299999));
#205101=CARTESIAN_POINT('Ctrl Pts',(8.00047027299994,11.6,6.72799402299999));
#205102=CARTESIAN_POINT('Ctrl Pts',(7.99921148699994,15.2,6.72722211399999));
#205103=CARTESIAN_POINT('Ctrl Pts',(7.99921148699994,11.6,6.72722211399999));
#205104=CARTESIAN_POINT('Ctrl Pts',(7.99796039099994,15.2,6.72645328399998));
#205105=CARTESIAN_POINT('Ctrl Pts',(7.99796039099994,11.6,6.72645328399998));
#205106=CARTESIAN_POINT('Ctrl Pts',(7.99671699399994,15.2,6.72568755299999));
#205107=CARTESIAN_POINT('Ctrl Pts',(7.99671699399994,11.6,6.72568755299999));
#205108=CARTESIAN_POINT('Ctrl Pts',(7.99548130699994,15.2,6.72492494499998));
#205109=CARTESIAN_POINT('Ctrl Pts',(7.99548130699994,11.6,6.72492494499998));
#205110=CARTESIAN_POINT('Ctrl Pts',(7.99425333799994,15.2,6.72416548299999));
#205111=CARTESIAN_POINT('Ctrl Pts',(7.99425333799994,11.6,6.72416548299999));
#205112=CARTESIAN_POINT('Ctrl Pts',(7.99303309699994,15.2,6.72340918999998));
#205113=CARTESIAN_POINT('Ctrl Pts',(7.99303309699994,11.6,6.72340918999998));
#205114=CARTESIAN_POINT('Ctrl Pts',(7.99182059499994,15.2,6.72265608999999));
#205115=CARTESIAN_POINT('Ctrl Pts',(7.99182059499994,11.6,6.72265608999999));
#205116=CARTESIAN_POINT('Ctrl Pts',(7.99061583999995,15.2,6.72190620499999));
#205117=CARTESIAN_POINT('Ctrl Pts',(7.99061583999995,11.6,6.72190620499999));
#205118=CARTESIAN_POINT('Ctrl Pts',(7.98941884299994,15.2,6.72115955999999));
#205119=CARTESIAN_POINT('Ctrl Pts',(7.98941884299994,11.6,6.72115955999999));
#205120=CARTESIAN_POINT('Ctrl Pts',(7.98822961399994,15.2,6.72041617699998));
#205121=CARTESIAN_POINT('Ctrl Pts',(7.98822961399994,11.6,6.72041617699998));
#205122=CARTESIAN_POINT('Ctrl Pts',(7.98704816099994,15.2,6.71967607999999));
#205123=CARTESIAN_POINT('Ctrl Pts',(7.98704816099994,11.6,6.71967607999999));
#205124=CARTESIAN_POINT('Ctrl Pts',(7.98587449499994,15.2,6.71893929399998));
#205125=CARTESIAN_POINT('Ctrl Pts',(7.98587449499994,11.6,6.71893929399998));
#205126=CARTESIAN_POINT('Ctrl Pts',(7.98470862699994,15.2,6.71820584199998));
#205127=CARTESIAN_POINT('Ctrl Pts',(7.98470862699994,11.6,6.71820584199998));
#205128=CARTESIAN_POINT('Ctrl Pts',(7.98355056499994,15.2,6.71747574699998));
#205129=CARTESIAN_POINT('Ctrl Pts',(7.98355056499994,11.6,6.71747574699998));
#205130=CARTESIAN_POINT('Ctrl Pts',(7.98240032199995,15.2,6.71674903499999));
#205131=CARTESIAN_POINT('Ctrl Pts',(7.98240032199995,11.6,6.71674903499999));
#205132=CARTESIAN_POINT('Ctrl Pts',(7.98125790399994,15.2,6.71602572899998));
#205133=CARTESIAN_POINT('Ctrl Pts',(7.98125790399994,11.6,6.71602572899998));
#205134=CARTESIAN_POINT('Ctrl Pts',(7.98012332299994,15.2,6.71530585399999));
#205135=CARTESIAN_POINT('Ctrl Pts',(7.98012332299994,11.6,6.71530585399999));
#205136=CARTESIAN_POINT('Ctrl Pts',(7.97899658999994,15.2,6.71458943299999));
#205137=CARTESIAN_POINT('Ctrl Pts',(7.97899658999994,11.6,6.71458943299999));
#205138=CARTESIAN_POINT('Ctrl Pts',(7.97787771299994,15.2,6.71387649199998));
#205139=CARTESIAN_POINT('Ctrl Pts',(7.97787771299994,11.6,6.71387649199998));
#205140=CARTESIAN_POINT('Ctrl Pts',(7.97676670299994,15.2,6.71316705499999));
#205141=CARTESIAN_POINT('Ctrl Pts',(7.97676670299994,11.6,6.71316705499999));
#205142=CARTESIAN_POINT('Ctrl Pts',(7.97566357099995,15.2,6.71246114699999));
#205143=CARTESIAN_POINT('Ctrl Pts',(7.97566357099995,11.6,6.71246114699999));
#205144=CARTESIAN_POINT('Ctrl Pts',(7.97456832699995,15.2,6.71175879199998));
#205145=CARTESIAN_POINT('Ctrl Pts',(7.97456832699995,11.6,6.71175879199998));
#205146=CARTESIAN_POINT('Ctrl Pts',(7.97348097899994,15.2,6.71106001599998));
#205147=CARTESIAN_POINT('Ctrl Pts',(7.97348097899994,11.6,6.71106001599998));
#205148=CARTESIAN_POINT('Ctrl Pts',(7.97240153999994,15.2,6.71036484399998));
#205149=CARTESIAN_POINT('Ctrl Pts',(7.97240153999994,11.6,6.71036484399998));
#205150=CARTESIAN_POINT('Ctrl Pts',(7.97133001899994,15.2,6.70967330099998));
#205151=CARTESIAN_POINT('Ctrl Pts',(7.97133001899994,11.6,6.70967330099998));
#205152=CARTESIAN_POINT('Ctrl Pts',(7.97026642699994,15.2,6.70898541299999));
#205153=CARTESIAN_POINT('Ctrl Pts',(7.97026642699994,11.6,6.70898541299999));
#205154=CARTESIAN_POINT('Ctrl Pts',(7.96921077299995,15.2,6.70830120399999));
#205155=CARTESIAN_POINT('Ctrl Pts',(7.96921077299995,11.6,6.70830120399999));
#205156=CARTESIAN_POINT('Ctrl Pts',(7.96816306799994,15.2,6.70762069999999));
#205157=CARTESIAN_POINT('Ctrl Pts',(7.96816306799994,11.6,6.70762069999999));
#205158=CARTESIAN_POINT('Ctrl Pts',(7.96712332399995,15.2,6.70694392699998));
#205159=CARTESIAN_POINT('Ctrl Pts',(7.96712332399995,11.6,6.70694392699998));
#205160=CARTESIAN_POINT('Ctrl Pts',(7.96609154999994,15.2,6.70627091099998));
#205161=CARTESIAN_POINT('Ctrl Pts',(7.96609154999994,11.6,6.70627091099998));
#205162=CARTESIAN_POINT('Ctrl Pts',(7.96506775499994,15.2,6.70560167799999));
#205163=CARTESIAN_POINT('Ctrl Pts',(7.96506775499994,11.6,6.70560167799999));
#205164=CARTESIAN_POINT('Ctrl Pts',(7.96405195199994,15.2,6.70493625299999));
#205165=CARTESIAN_POINT('Ctrl Pts',(7.96405195199994,11.6,6.70493625299999));
#205166=CARTESIAN_POINT('Ctrl Pts',(7.96304414999994,15.2,6.70427466299999));
#205167=CARTESIAN_POINT('Ctrl Pts',(7.96304414999994,11.6,6.70427466299999));
#205168=CARTESIAN_POINT('Ctrl Pts',(7.96204436099995,15.2,6.70361693399999));
#205169=CARTESIAN_POINT('Ctrl Pts',(7.96204436099995,11.6,6.70361693399999));
#205170=CARTESIAN_POINT('Ctrl Pts',(7.96105259399994,15.2,6.70296309299999));
#205171=CARTESIAN_POINT('Ctrl Pts',(7.96105259399994,11.6,6.70296309299999));
#205172=CARTESIAN_POINT('Ctrl Pts',(7.96006886099994,15.2,6.70231316599998));
#205173=CARTESIAN_POINT('Ctrl Pts',(7.96006886099994,11.6,6.70231316599998));
#205174=CARTESIAN_POINT('Ctrl Pts',(7.95909317099994,15.2,6.70166717899999));
#205175=CARTESIAN_POINT('Ctrl Pts',(7.95909317099994,11.6,6.70166717899999));
#205176=CARTESIAN_POINT('Ctrl Pts',(7.95812553699994,15.2,6.70102516099998));
#205177=CARTESIAN_POINT('Ctrl Pts',(7.95812553699994,11.6,6.70102516099998));
#205178=CARTESIAN_POINT('Ctrl Pts',(7.95716596799994,15.2,6.70038713599999));
#205179=CARTESIAN_POINT('Ctrl Pts',(7.95716596799994,11.6,6.70038713599999));
#205180=CARTESIAN_POINT('Ctrl Pts',(7.95621447399995,15.2,6.69975313299998));
#205181=CARTESIAN_POINT('Ctrl Pts',(7.95621447399995,11.6,6.69975313299998));
#205182=CARTESIAN_POINT('Ctrl Pts',(7.95527106899995,15.2,6.69912317999999));
#205183=CARTESIAN_POINT('Ctrl Pts',(7.95527106899995,11.6,6.69912317999999));
#205184=CARTESIAN_POINT('Ctrl Pts',(7.95433576199994,15.2,6.69849730199999));
#205185=CARTESIAN_POINT('Ctrl Pts',(7.95433576199994,11.6,6.69849730199999));
#205186=CARTESIAN_POINT('Ctrl Pts',(7.95340856399994,15.2,6.69787552699999));
#205187=CARTESIAN_POINT('Ctrl Pts',(7.95340856399994,11.6,6.69787552699999));
#205188=CARTESIAN_POINT('Ctrl Pts',(7.95248948499995,15.2,6.69725788299999));
#205189=CARTESIAN_POINT('Ctrl Pts',(7.95248948499995,11.6,6.69725788299999));
#205190=CARTESIAN_POINT('Ctrl Pts',(7.95157853699994,15.2,6.69664439899999));
#205191=CARTESIAN_POINT('Ctrl Pts',(7.95157853699994,11.6,6.69664439899999));
#205192=CARTESIAN_POINT('Ctrl Pts',(7.95067573199994,15.2,6.69603509999998));
#205193=CARTESIAN_POINT('Ctrl Pts',(7.95067573199994,11.6,6.69603509999998));
#205194=CARTESIAN_POINT('Ctrl Pts',(7.94978107899994,15.2,6.69543001699999));
#205195=CARTESIAN_POINT('Ctrl Pts',(7.94978107899994,11.6,6.69543001699999));
#205196=CARTESIAN_POINT('Ctrl Pts',(7.94889458999994,15.2,6.69482917499998));
#205197=CARTESIAN_POINT('Ctrl Pts',(7.94889458999994,11.6,6.69482917499998));
#205198=CARTESIAN_POINT('Ctrl Pts',(7.94801627599995,15.2,6.69423260599999));
#205199=CARTESIAN_POINT('Ctrl Pts',(7.94801627599995,11.6,6.69423260599999));
#205200=CARTESIAN_POINT('Ctrl Pts',(7.94714614999994,15.2,6.69364033599999));
#205201=CARTESIAN_POINT('Ctrl Pts',(7.94714614999994,11.6,6.69364033599999));
#205202=CARTESIAN_POINT('Ctrl Pts',(7.94628421999994,15.2,6.69305239299998));
#205203=CARTESIAN_POINT('Ctrl Pts',(7.94628421999994,11.6,6.69305239299998));
#205204=CARTESIAN_POINT('Ctrl Pts',(7.94543049999994,15.2,6.69246880699998));
#205205=CARTESIAN_POINT('Ctrl Pts',(7.94543049999994,11.6,6.69246880699998));
#205206=CARTESIAN_POINT('Ctrl Pts',(7.94458499899994,15.2,6.69188960699999));
#205207=CARTESIAN_POINT('Ctrl Pts',(7.94458499899994,11.6,6.69188960699999));
#205208=CARTESIAN_POINT('Ctrl Pts',(7.94374772999995,15.2,6.69131482099999));
#205209=CARTESIAN_POINT('Ctrl Pts',(7.94374772999995,11.6,6.69131482099999));
#205210=CARTESIAN_POINT('Ctrl Pts',(7.94291870399995,15.2,6.69074447799999));
#205211=CARTESIAN_POINT('Ctrl Pts',(7.94291870399995,11.6,6.69074447799999));
#205212=CARTESIAN_POINT('Ctrl Pts',(7.94209793199995,15.2,6.69017860899999));
#205213=CARTESIAN_POINT('Ctrl Pts',(7.94209793199995,11.6,6.69017860899999));
#205214=CARTESIAN_POINT('Ctrl Pts',(7.94128542699994,15.2,6.68961724199999));
#205215=CARTESIAN_POINT('Ctrl Pts',(7.94128542699994,11.6,6.68961724199999));
#205216=CARTESIAN_POINT('Ctrl Pts',(7.94048119799994,15.2,6.68906040599998));
#205217=CARTESIAN_POINT('Ctrl Pts',(7.94048119799994,11.6,6.68906040599998));
#205218=CARTESIAN_POINT('Ctrl Pts',(7.93968525799994,15.2,6.68850813299999));
#205219=CARTESIAN_POINT('Ctrl Pts',(7.93968525799994,11.6,6.68850813299999));
#205220=CARTESIAN_POINT('Ctrl Pts',(7.93889761899995,15.2,6.68796045099998));
#205221=CARTESIAN_POINT('Ctrl Pts',(7.93889761899995,11.6,6.68796045099998));
#205222=CARTESIAN_POINT('Ctrl Pts',(7.93811829199995,15.2,6.68741739099998));
#205223=CARTESIAN_POINT('Ctrl Pts',(7.93811829199995,11.6,6.68741739099998));
#205224=CARTESIAN_POINT('Ctrl Pts',(7.93734728899994,15.2,6.68687898099999));
#205225=CARTESIAN_POINT('Ctrl Pts',(7.93734728899994,11.6,6.68687898099999));
#205226=CARTESIAN_POINT('Ctrl Pts',(7.93658462199994,15.2,6.68634525499999));
#205227=CARTESIAN_POINT('Ctrl Pts',(7.93658462199994,11.6,6.68634525499999));
#205228=CARTESIAN_POINT('Ctrl Pts',(7.93583464599994,15.2,6.68581928799998));
#205229=CARTESIAN_POINT('Ctrl Pts',(7.93583464599994,11.6,6.68581928799998));
#205230=CARTESIAN_POINT('Ctrl Pts',(7.93524212599995,15.2,6.68540286399999));
#205231=CARTESIAN_POINT('Ctrl Pts',(7.93524212599995,11.6,6.68540286399999));
#205232=CARTESIAN_POINT('Ctrl Pts',(7.93480250499995,15.2,6.68509340799999));
#205233=CARTESIAN_POINT('Ctrl Pts',(7.93480250499995,11.6,6.68509340799999));
#205234=CARTESIAN_POINT('Ctrl Pts',(7.93451247199994,15.2,6.68488903399999));
#205235=CARTESIAN_POINT('Ctrl Pts',(7.93451247199994,11.6,6.68488903399999));
#205236=CARTESIAN_POINT('Ctrl Pts',(7.93436996999994,15.2,6.68478856799998));
#205237=CARTESIAN_POINT('Ctrl Pts',(7.93436996999994,11.6,6.68478856799998));
#205238=CARTESIAN_POINT('',(7.93436996899994,12.2,6.68478856799998));
#205239=CARTESIAN_POINT('',(7.93436996899994,15.2,6.68478856799998));
#205240=CARTESIAN_POINT('',(7.93436996899994,12.2,6.68478856799998));
#205241=CARTESIAN_POINT('Ctrl Pts',(9.03946594399994,12.2,7.10901226999999));
#205242=CARTESIAN_POINT('Ctrl Pts',(9.0357292033211,12.2,7.10820510485334));
#205243=CARTESIAN_POINT('Ctrl Pts',(9.03199984125262,12.2,7.10739512148574));
#205244=CARTESIAN_POINT('Ctrl Pts',(9.02827785941652,12.2,7.10658231363194));
#205245=CARTESIAN_POINT('Ctrl Pts',(9.02455587758041,12.2,7.10576950577814));
#205246=CARTESIAN_POINT('Ctrl Pts',(9.02084127436859,12.2,7.10495387545248));
#205247=CARTESIAN_POINT('Ctrl Pts',(9.01713406173388,12.2,7.10413543639999));
#205248=CARTESIAN_POINT('Ctrl Pts',(9.01342684909918,12.2,7.1033169973475));
#205249=CARTESIAN_POINT('Ctrl Pts',(9.00972702803836,12.2,7.10249574936599));
#205250=CARTESIAN_POINT('Ctrl Pts',(9.00603462575484,12.2,7.10167172614631));
#205251=CARTESIAN_POINT('Ctrl Pts',(9.00234222280054,12.2,7.10084770277693));
#205252=CARTESIAN_POINT('Ctrl Pts',(8.99865723923165,12.2,7.1000209059901));
#205253=CARTESIAN_POINT('Ctrl Pts',(8.99497970615653,12.2,7.09919137303583));
#205254=CARTESIAN_POINT('Ctrl Pts',(8.99007632983651,12.2,7.09808532934797));
#205255=CARTESIAN_POINT('Ctrl Pts',(8.98518619850922,12.2,7.09697442424131));
#205256=CARTESIAN_POINT('Ctrl Pts',(8.98030937140703,12.2,7.09585872583283));
#205257=CARTESIAN_POINT('Ctrl Pts',(8.97665175091428,12.2,7.09502195198847));
#205258=CARTESIAN_POINT('Ctrl Pts',(8.97300161223856,12.2,7.09418248255741));
#205259=CARTESIAN_POINT('Ctrl Pts',(8.96935897972972,12.2,7.09334034712958));
#205260=CARTESIAN_POINT('Ctrl Pts',(8.9657163472209,12.2,7.09249821170174));
#205261=CARTESIAN_POINT('Ctrl Pts',(8.96208122205994,12.2,7.09165340977026));
#205262=CARTESIAN_POINT('Ctrl Pts',(8.95845362973238,12.2,7.09080597588474));
#205263=CARTESIAN_POINT('Ctrl Pts',(8.9548260367458,12.2,7.08995854184528));
#205264=CARTESIAN_POINT('Ctrl Pts',(8.95120597758635,12.2,7.08910847592173));
#205265=CARTESIAN_POINT('Ctrl Pts',(8.94759347797903,12.2,7.08825581033912));
#205266=CARTESIAN_POINT('Ctrl Pts',(8.94398097902799,12.2,7.08740314491141));
#205267=CARTESIAN_POINT('Ctrl Pts',(8.94037603872654,12.2,7.08654787930885));
#205268=CARTESIAN_POINT('Ctrl Pts',(8.93677868385791,12.2,7.08569004692312));
#205269=CARTESIAN_POINT('Ctrl Pts',(8.93318132898928,12.2,7.0848322145374));
#205270=CARTESIAN_POINT('Ctrl Pts',(8.92959155958273,12.2,7.0839718151218));
#205271=CARTESIAN_POINT('Ctrl Pts',(8.92600939969664,12.2,7.08310888027422));
#205272=CARTESIAN_POINT('Ctrl Pts',(8.92242723981055,12.2,7.08224594542665));
#205273=CARTESIAN_POINT('Ctrl Pts',(8.91885269052311,12.2,7.08138047555652));
#205274=CARTESIAN_POINT('Ctrl Pts',(8.9152857780948,12.2,7.08051250379246));
#205275=CARTESIAN_POINT('Ctrl Pts',(8.91171886566649,12.2,7.07964453202839));
#205276=CARTESIAN_POINT('Ctrl Pts',(8.90815958947544,12.2,7.07877405966317));
#205277=CARTESIAN_POINT('Ctrl Pts',(8.90460797560381,12.2,7.07790111882011));
#205278=CARTESIAN_POINT('Ctrl Pts',(8.90105636173218,12.2,7.07702817797704));
#205279=CARTESIAN_POINT('Ctrl Pts',(8.89751240944337,12.2,7.07615276832581));
#205280=CARTESIAN_POINT('Ctrl Pts',(8.89397614648747,12.2,7.07527492444137));
#205281=CARTESIAN_POINT('Ctrl Pts',(8.89043988288915,12.2,7.07439708039746));
#205282=CARTESIAN_POINT('Ctrl Pts',(8.88691130760967,12.2,7.07351680156952));
#205283=CARTESIAN_POINT('Ctrl Pts',(8.88339044697402,12.2,7.07263412156591));
#205284=CARTESIAN_POINT('Ctrl Pts',(8.87986958697799,12.2,7.07175144172265));
#205285=CARTESIAN_POINT('Ctrl Pts',(8.87635643965195,12.2,7.07086636067398));
#205286=CARTESIAN_POINT('Ctrl Pts',(8.87285103356342,12.2,7.06997891232828));
#205287=CARTESIAN_POINT('Ctrl Pts',(8.86934562747489,12.2,7.06909146398258));
#205288=CARTESIAN_POINT('Ctrl Pts',(8.86584796275881,12.2,7.06820164930384));
#205289=CARTESIAN_POINT('Ctrl Pts',(8.86235806388629,12.2,7.06730950191939));
#205290=CARTESIAN_POINT('Ctrl Pts',(8.85886816501376,12.2,7.06641735453493));
#205291=CARTESIAN_POINT('Ctrl Pts',(8.85538603207365,12.2,7.06552287381742));
#205292=CARTESIAN_POINT('Ctrl Pts',(8.85191169219988,12.2,7.06462609455834));
#205293=CARTESIAN_POINT('Ctrl Pts',(8.84843735232612,12.2,7.06372931529925));
#205294=CARTESIAN_POINT('Ctrl Pts',(8.84497080525204,12.2,7.06283023828193));
#205295=CARTESIAN_POINT('Ctrl Pts',(8.84151207683536,12.2,7.06192889706488));
#205296=CARTESIAN_POINT('Ctrl Pts',(8.83805334841867,12.2,7.06102755584782));
#205297=CARTESIAN_POINT('Ctrl Pts',(8.83460243864312,12.2,7.06012395231425));
#205298=CARTESIAN_POINT('Ctrl Pts',(8.83115937426714,12.2,7.05921811947247));
#205299=CARTESIAN_POINT('Ctrl Pts',(8.82771630926568,12.2,7.05831228646613));
#205300=CARTESIAN_POINT('Ctrl Pts',(8.82428109046645,12.2,7.05740422408416));
#205301=CARTESIAN_POINT('Ctrl Pts',(8.82085374201108,12.2,7.05649396907657));
#205302=CARTESIAN_POINT('Ctrl Pts',(8.81742639417834,12.2,7.05558371423434));
#205303=CARTESIAN_POINT('Ctrl Pts',(8.81400691756881,12.2,7.0546712656524));
#205304=CARTESIAN_POINT('Ctrl Pts',(8.81059533860657,12.2,7.05375665930636));
#205305=CARTESIAN_POINT('Ctrl Pts',(8.80718375964434,12.2,7.05284205296031));
#205306=CARTESIAN_POINT('Ctrl Pts',(8.80378007972248,12.2,7.05192528919994));
#205307=CARTESIAN_POINT('Ctrl Pts',(8.80038432380488,12.2,7.05100640294147));
#205308=CARTESIAN_POINT('Ctrl Pts',(8.79698856788729,12.2,7.050087516683));
#205309=CARTESIAN_POINT('Ctrl Pts',(8.79360073576041,12.2,7.04916650844979));
#205310=CARTESIAN_POINT('Ctrl Pts',(8.79022085479989,12.2,7.04824341369167));
#205311=CARTESIAN_POINT('Ctrl Pts',(8.78684097383936,12.2,7.04732031893354));
#205312=CARTESIAN_POINT('Ctrl Pts',(8.7834690429785,12.2,7.0463951382505));
#205313=CARTESIAN_POINT('Ctrl Pts',(8.78010509010003,12.2,7.0454679083677));
#205314=CARTESIAN_POINT('Ctrl Pts',(8.77674113722156,12.2,7.04454067848491));
#205315=CARTESIAN_POINT('Ctrl Pts',(8.77338516219426,12.2,7.04361139802595));
#205316=CARTESIAN_POINT('Ctrl Pts',(8.77003719064772,12.2,7.04268010468016));
#205317=CARTESIAN_POINT('Ctrl Pts',(8.76668921910116,12.2,7.04174881133437));
#205318=CARTESIAN_POINT('Ctrl Pts',(8.76334925132296,12.2,7.04081550520297));
#205319=CARTESIAN_POINT('Ctrl Pts',(8.76001731444292,12.2,7.03988022148722));
#205320=CARTESIAN_POINT('Ctrl Pts',(8.75668537695758,12.2,7.03894493760156));
#205321=CARTESIAN_POINT('Ctrl Pts',(8.75336147029118,12.2,7.03800767783202));
#205322=CARTESIAN_POINT('Ctrl Pts',(8.75004562126871,12.2,7.03706847932025));
#205323=CARTESIAN_POINT('Ctrl Pts',(8.74672977284863,12.2,7.03612928097911));
#205324=CARTESIAN_POINT('Ctrl Pts',(8.74342198178642,12.2,7.03518814242974));
#205325=CARTESIAN_POINT('Ctrl Pts',(8.74012227490702,12.2,7.03424510167217));
#205326=CARTESIAN_POINT('Ctrl Pts',(8.73682256802762,12.2,7.0333020609146));
#205327=CARTESIAN_POINT('Ctrl Pts',(8.73353094505916,12.2,7.03235711836905));
#205328=CARTESIAN_POINT('Ctrl Pts',(8.73024743320524,12.2,7.03141031202414));
#205329=CARTESIAN_POINT('Ctrl Pts',(8.72696392135134,12.2,7.03046350567923));
#205330=CARTESIAN_POINT('Ctrl Pts',(8.72368852091569,12.2,7.0295148335873));
#205331=CARTESIAN_POINT('Ctrl Pts',(8.72042125847786,12.2,7.02856433674253));
#205332=CARTESIAN_POINT('Ctrl Pts',(8.71715399604003,12.2,7.02761383989776));
#205333=CARTESIAN_POINT('Ctrl Pts',(8.71389487088697,12.2,7.02666151658581));
#205334=CARTESIAN_POINT('Ctrl Pts',(8.71064391233771,12.2,7.02570740387063));
#205335=CARTESIAN_POINT('Ctrl Pts',(8.70739295378845,12.2,7.02475329115545));
#205336=CARTESIAN_POINT('Ctrl Pts',(8.70415015838862,12.2,7.02379739027373));
#205337=CARTESIAN_POINT('Ctrl Pts',(8.70091555642171,12.2,7.02283974047543));
#205338=CARTESIAN_POINT('Ctrl Pts',(8.6966027534074,12.2,7.02156287396171));
#205339=CARTESIAN_POINT('Ctrl Pts',(8.69230451406649,12.2,7.02028289602211));
#205340=CARTESIAN_POINT('Ctrl Pts',(8.68802090248032,12.2,7.01899990022412));
#205341=CARTESIAN_POINT('Ctrl Pts',(8.68480819408251,12.2,7.01803765346304));
#205342=CARTESIAN_POINT('Ctrl Pts',(8.68160371343455,12.2,7.01707370848684));
#205343=CARTESIAN_POINT('Ctrl Pts',(8.67840748899446,12.2,7.01610810472587));
#205344=CARTESIAN_POINT('Ctrl Pts',(8.67414585602057,12.2,7.01482063292764));
#205345=CARTESIAN_POINT('Ctrl Pts',(8.6698988997593,12.2,7.01353021277599));
#205346=CARTESIAN_POINT('Ctrl Pts',(8.66566668430793,12.2,7.01223693703855));
#205347=CARTESIAN_POINT('Ctrl Pts',(8.66143446943319,12.2,7.01094366147731));
#205348=CARTESIAN_POINT('Ctrl Pts',(8.65721699491211,12.2,7.00964752991645));
#205349=CARTESIAN_POINT('Ctrl Pts',(8.65301432781026,12.2,7.00834863835615));
#205350=CARTESIAN_POINT('Ctrl Pts',(8.6488116601358,12.2,7.00704974661887));
#205351=CARTESIAN_POINT('Ctrl Pts',(8.64462379779295,12.2,7.00574809408054));
#205352=CARTESIAN_POINT('Ctrl Pts',(8.64045080663611,12.2,7.00444377627738));
#205353=CARTESIAN_POINT('Ctrl Pts',(8.63627781604783,12.2,7.00313945865194));
#205354=CARTESIAN_POINT('Ctrl Pts',(8.63211969691766,12.2,7.00183247790536));
#205355=CARTESIAN_POINT('Ctrl Pts',(8.62797651458873,12.2,7.00052292712369));
#205356=CARTESIAN_POINT('Ctrl Pts',(8.62383333169529,12.2,6.99921337616361));
#205357=CARTESIAN_POINT('Ctrl Pts',(8.61970508465086,12.2,6.99790125668099));
#205358=CARTESIAN_POINT('Ctrl Pts',(8.6155918403721,12.2,6.99658666694251));
#205359=CARTESIAN_POINT('Ctrl Pts',(8.61147859665378,12.2,6.99527207738314));
#205360=CARTESIAN_POINT('Ctrl Pts',(8.60738035496395,12.2,6.99395501611039));
#205361=CARTESIAN_POINT('Ctrl Pts',(8.60329718109246,12.2,6.99263558370811));
#205362=CARTESIAN_POINT('Ctrl Pts',(8.59921400666464,12.2,6.99131615112604));
#205363=CARTESIAN_POINT('Ctrl Pts',(8.59514590002471,12.2,6.98999434577793));
#205364=CARTESIAN_POINT('Ctrl Pts',(8.5910929271937,12.2,6.98867026865006));
#205365=CARTESIAN_POINT('Ctrl Pts',(8.58703995491491,12.2,6.98734619170261));
#205366=CARTESIAN_POINT('Ctrl Pts',(8.58300211633029,12.2,6.98601984098337));
#205367=CARTESIAN_POINT('Ctrl Pts',(8.57897947865759,12.2,6.98469131892554));
#205368=CARTESIAN_POINT('Ctrl Pts',(8.57495684043681,12.2,6.9833627966867));
#205369=CARTESIAN_POINT('Ctrl Pts',(8.57094940214949,12.2,6.98203210334723));
#205370=CARTESIAN_POINT('Ctrl Pts',(8.56695723124717,12.2,6.98069933899075));
#205371=CARTESIAN_POINT('Ctrl Pts',(8.56296506088878,12.2,6.97936657481586));
#205372=CARTESIAN_POINT('Ctrl Pts',(8.5589881564503,12.2,6.9780317411174));
#205373=CARTESIAN_POINT('Ctrl Pts',(8.55502658560594,12.2,6.97669493972689));
#205374=CARTESIAN_POINT('Ctrl Pts',(8.55106501422181,12.2,6.97535813815425));
#205375=CARTESIAN_POINT('Ctrl Pts',(8.54711877786409,12.2,6.97401936900639));
#205376=CARTESIAN_POINT('Ctrl Pts',(8.54318794098321,12.2,6.97267873726666));
#205377=CARTESIAN_POINT('Ctrl Pts',(8.53925710410233,12.2,6.97133810552693));
#205378=CARTESIAN_POINT('Ctrl Pts',(8.53534166835655,12.2,6.96999561026198));
#205379=CARTESIAN_POINT('Ctrl Pts',(8.53144170014558,12.2,6.96865135602187));
#205380=CARTESIAN_POINT('Ctrl Pts',(8.5255917483605,12.2,6.96663497484487));
#205381=CARTESIAN_POINT('Ctrl Pts',(8.51977659904015,12.2,6.96461463830795));
#205382=CARTESIAN_POINT('Ctrl Pts',(8.51399647941834,12.2,6.96259070313133));
#205383=CARTESIAN_POINT('Ctrl Pts',(8.51014306651215,12.2,6.96124141307487));
#205384=CARTESIAN_POINT('Ctrl Pts',(8.50630522331396,12.2,6.95989052452984));
#205385=CARTESIAN_POINT('Ctrl Pts',(8.50248301762482,12.2,6.95853814569611));
#205386=CARTESIAN_POINT('Ctrl Pts',(8.4986608114149,12.2,6.95718576667811));
#205387=CARTESIAN_POINT('Ctrl Pts',(8.49485424279537,12.2,6.95583189629886));
#205388=CARTESIAN_POINT('Ctrl Pts',(8.49106337869988,12.2,6.95447664405833));
#205389=CARTESIAN_POINT('Ctrl Pts',(8.4872725146044,12.2,6.9531213918178));
#205390=CARTESIAN_POINT('Ctrl Pts',(8.4834973557885,12.2,6.95176475755489));
#205391=CARTESIAN_POINT('Ctrl Pts',(8.47973797158523,12.2,6.9504068525363));
#205392=CARTESIAN_POINT('Ctrl Pts',(8.47503874209946,12.2,6.9487094715406));
#205393=CARTESIAN_POINT('Ctrl Pts',(8.4703641582144,12.2,6.9470101029647));
#205394=CARTESIAN_POINT('Ctrl Pts',(8.46571435614975,12.2,6.94530896620584));
#205395=CARTESIAN_POINT('Ctrl Pts',(8.46199451388983,12.2,6.94394805657622));
#205396=CARTESIAN_POINT('Ctrl Pts',(8.4582905303981,12.2,6.94258601363261));
#205397=CARTESIAN_POINT('Ctrl Pts',(8.45460247747488,12.2,6.94122295272499));
#205398=CARTESIAN_POINT('Ctrl Pts',(8.45091442455165,12.2,6.93985989181737));
#205399=CARTESIAN_POINT('Ctrl Pts',(8.44724229913308,12.2,6.9384958119263));
#205400=CARTESIAN_POINT('Ctrl Pts',(8.44358617293545,12.2,6.93713082701848));
#205401=CARTESIAN_POINT('Ctrl Pts',(8.43993004723596,12.2,6.93576584229665));
#205402=CARTESIAN_POINT('Ctrl Pts',(8.43628991926427,12.2,6.93439995305929));
#205403=CARTESIAN_POINT('Ctrl Pts',(8.43266585971069,12.2,6.93303327444259));
#205404=CARTESIAN_POINT('Ctrl Pts',(8.42904179966332,12.2,6.93166659563967));
#205405=CARTESIAN_POINT('Ctrl Pts',(8.42543380849562,12.2,6.93029912800927));
#205406=CARTESIAN_POINT('Ctrl Pts',(8.42184195441262,12.2,6.92893098776797));
#205407=CARTESIAN_POINT('Ctrl Pts',(8.41825010081901,12.2,6.92756284771307));
#205408=CARTESIAN_POINT('Ctrl Pts',(8.41467438710943,12.2,6.92619403477772));
#205409=CARTESIAN_POINT('Ctrl Pts',(8.41111488023269,12.2,6.92482466811193));
#205410=CARTESIAN_POINT('Ctrl Pts',(8.40755537287097,12.2,6.92345530125956));
#205411=CARTESIAN_POINT('Ctrl Pts',(8.40401207415797,12.2,6.92208537968598));
#205412=CARTESIAN_POINT('Ctrl Pts',(8.40048505451318,12.2,6.9207150240428));
#205413=CARTESIAN_POINT('Ctrl Pts',(8.39695803534894,12.2,6.91934466858633));
#205414=CARTESIAN_POINT('Ctrl Pts',(8.39344729625945,12.2,6.91797387854719));
#205415=CARTESIAN_POINT('Ctrl Pts',(8.38995290604404,12.2,6.91660277460374));
#205416=CARTESIAN_POINT('Ctrl Pts',(8.38645851535251,12.2,6.91523167047348));
#205417=CARTESIAN_POINT('Ctrl Pts',(8.3829804748074,12.2,6.91386025140706));
#205418=CARTESIAN_POINT('Ctrl Pts',(8.37951885600872,12.2,6.91248864188786));
#205419=CARTESIAN_POINT('Ctrl Pts',(8.37605723768168,12.2,6.91111703255554));
#205420=CARTESIAN_POINT('Ctrl Pts',(8.37261204047605,12.2,6.9097452305721));
#205421=CARTESIAN_POINT('Ctrl Pts',(8.36918333597249,12.2,6.90837336194905));
#205422=CARTESIAN_POINT('Ctrl Pts',(8.36575463100178,12.2,6.90700149313908));
#205423=CARTESIAN_POINT('Ctrl Pts',(8.36234242056755,12.2,6.90562955662649));
#205424=CARTESIAN_POINT('Ctrl Pts',(8.35894677327244,12.2,6.90425767716284));
#205425=CARTESIAN_POINT('Ctrl Pts',(8.35555112643999,12.2,6.9028857978861));
#205426=CARTESIAN_POINT('Ctrl Pts',(8.35217204464038,12.2,6.90151397674825));
#205427=CARTESIAN_POINT('Ctrl Pts',(8.34880960152466,12.2,6.90014233824925));
#205428=CARTESIAN_POINT('Ctrl Pts',(8.34544715795081,12.2,6.89877069956336));
#205429=CARTESIAN_POINT('Ctrl Pts',(8.34210134992745,12.2,6.89739924528279));
#205430=CARTESIAN_POINT('Ctrl Pts',(8.33877225306428,12.2,6.89602810325738));
#205431=CARTESIAN_POINT('Ctrl Pts',(8.3354431566547,12.2,6.8946569614188));
#205432=CARTESIAN_POINT('Ctrl Pts',(8.33213076870157,12.2,6.89328613199817));
#205433=CARTESIAN_POINT('Ctrl Pts',(8.32883516558038,12.2,6.89191574349904));
#205434=CARTESIAN_POINT('Ctrl Pts',(8.32553956201018,12.2,6.8905453548132));
#205435=CARTESIAN_POINT('Ctrl Pts',(8.32226073976654,12.2,6.88917540871351));
#205436=CARTESIAN_POINT('Ctrl Pts',(8.31899877503321,12.2,6.88780603474999));
#205437=CARTESIAN_POINT('Ctrl Pts',(8.31573681029987,12.2,6.88643666078647));
#205438=CARTESIAN_POINT('Ctrl Pts',(8.31249170255185,12.2,6.88506785976191));
#205439=CARTESIAN_POINT('Ctrl Pts',(8.30926352448875,12.2,6.8836997655763));
#205440=CARTESIAN_POINT('Ctrl Pts',(8.30522830256963,12.2,6.8819896481239));
#205441=CARTESIAN_POINT('Ctrl Pts',(8.30121953287222,12.2,6.88028063049843));
#205442=CARTESIAN_POINT('Ctrl Pts',(8.2972373633041,12.2,6.87857297999002));
#205443=CARTESIAN_POINT('Ctrl Pts',(8.29405162712872,12.2,6.87720685935991));
#205444=CARTESIAN_POINT('Ctrl Pts',(8.2908829142133,12.2,6.87584161254377));
#205445=CARTESIAN_POINT('Ctrl Pts',(8.28773129820821,12.2,6.87447737652498));
#205446=CARTESIAN_POINT('Ctrl Pts',(8.28457968220312,12.2,6.87311314050619));
#205447=CARTESIAN_POINT('Ctrl Pts',(8.28144516460002,12.2,6.87174991326807));
#205448=CARTESIAN_POINT('Ctrl Pts',(8.27832781926519,12.2,6.87038783652728));
#205449=CARTESIAN_POINT('Ctrl Pts',(8.2752104743551,12.2,6.86902575997208));
#205450=CARTESIAN_POINT('Ctrl Pts',(8.27211030209734,12.2,6.86766483115426));
#205451=CARTESIAN_POINT('Ctrl Pts',(8.26902737900198,12.2,6.86630519075924));
#205452=CARTESIAN_POINT('Ctrl Pts',(8.26594445548657,12.2,6.86494555017896));
#205453=CARTESIAN_POINT('Ctrl Pts',(8.26287877906861,12.2,6.86358719847693));
#205454=CARTESIAN_POINT('Ctrl Pts',(8.25983042829315,12.2,6.86223027656979));
#205455=CARTESIAN_POINT('Ctrl Pts',(8.25601999003147,12.2,6.86053412427831));
#205456=CARTESIAN_POINT('Ctrl Pts',(8.25223661920634,12.2,6.8588402058952));
#205457=CARTESIAN_POINT('Ctrl Pts',(8.24848046775025,12.2,6.85714880277041));
#205458=CARTESIAN_POINT('Ctrl Pts',(8.24472431670358,12.2,6.85545739982999));
#205459=CARTESIAN_POINT('Ctrl Pts',(8.24099538457726,12.2,6.85376851262029));
#205460=CARTESIAN_POINT('Ctrl Pts',(8.23729382095071,12.2,6.85208242322052));
#205461=CARTESIAN_POINT('Ctrl Pts',(8.23359225692068,12.2,6.85039633363696));
#205462=CARTESIAN_POINT('Ctrl Pts',(8.22991806111245,12.2,6.84871304506445));
#205463=CARTESIAN_POINT('Ctrl Pts',(8.22627138694354,12.2,6.84703284603642));
#205464=CARTESIAN_POINT('Ctrl Pts',(8.22262471277462,12.2,6.84535264700839));
#205465=CARTESIAN_POINT('Ctrl Pts',(8.21900555826635,12.2,6.84367553568585));
#205466=CARTESIAN_POINT('Ctrl Pts',(8.21541407673632,12.2,6.84200180922724));
#205467=CARTESIAN_POINT('Ctrl Pts',(8.2111042986654,12.2,6.83999333736745));
#205468=CARTESIAN_POINT('Ctrl Pts',(8.20683436996365,12.2,6.83798973672343));
#205469=CARTESIAN_POINT('Ctrl Pts',(8.20260455585746,12.2,6.83599152609835));
#205470=CARTESIAN_POINT('Ctrl Pts',(8.19907971096108,12.2,6.83432635066819));
#205471=CARTESIAN_POINT('Ctrl Pts',(8.19558272439941,12.2,6.83266491934952));
#205472=CARTESIAN_POINT('Ctrl Pts',(8.19211375051281,12.2,6.83100753476652));
#205473=CARTESIAN_POINT('Ctrl Pts',(8.18864477662621,12.2,6.82935015018352));
#205474=CARTESIAN_POINT('Ctrl Pts',(8.1852038162012,12.2,6.82769681512838));
#205475=CARTESIAN_POINT('Ctrl Pts',(8.18179102557851,12.2,6.82604783651763));
#205476=CARTESIAN_POINT('Ctrl Pts',(8.17837823532779,12.2,6.82439885808662));
#205477=CARTESIAN_POINT('Ctrl Pts',(8.17499361394205,12.2,6.82275423969722));
#205478=CARTESIAN_POINT('Ctrl Pts',(8.17163732118055,12.2,6.82111429293114));
#205479=CARTESIAN_POINT('Ctrl Pts',(8.16828102805322,12.2,6.81947434598632));
#205480=CARTESIAN_POINT('Ctrl Pts',(8.1649530622949,12.2,6.81783907455807));
#205481=CARTESIAN_POINT('Ctrl Pts',(8.16165358347312,12.2,6.81620879594654));
#205482=CARTESIAN_POINT('Ctrl Pts',(8.15835410465134,12.2,6.81457851733502));
#205483=CARTESIAN_POINT('Ctrl Pts',(8.15508311341256,12.2,6.81295323313046));
#205484=CARTESIAN_POINT('Ctrl Pts',(8.1518407693597,12.2,6.81133326943805));
#205485=CARTESIAN_POINT('Ctrl Pts',(8.14859842530684,12.2,6.80971330574564));
#205486=CARTESIAN_POINT('Ctrl Pts',(8.14538472933206,12.2,6.8080986631833));
#205487=CARTESIAN_POINT('Ctrl Pts',(8.14219984294167,12.2,6.80648967290524));
#205488=CARTESIAN_POINT('Ctrl Pts',(8.13901495655129,12.2,6.80488068262717));
#205489=CARTESIAN_POINT('Ctrl Pts',(8.13585888043942,12.2,6.80327734438259));
#205490=CARTESIAN_POINT('Ctrl Pts',(8.13273177668789,12.2,6.80167999660448));
#205491=CARTESIAN_POINT('Ctrl Pts',(8.12960467293636,12.2,6.80008264882637));
#205492=CARTESIAN_POINT('Ctrl Pts',(8.12650654367112,12.2,6.7984912917136));
#205493=CARTESIAN_POINT('Ctrl Pts',(8.12343755226821,12.2,6.79690626823416));
#205494=CARTESIAN_POINT('Ctrl Pts',(8.1203685608653,12.2,6.79532124475473));
#205495=CARTESIAN_POINT('Ctrl Pts',(8.11732870910542,12.2,6.79374255630553));
#205496=CARTESIAN_POINT('Ctrl Pts',(8.1143181612582,12.2,6.79217055199997));
#205497=CARTESIAN_POINT('Ctrl Pts',(8.11130761341098,12.2,6.79059854769441));
#205498=CARTESIAN_POINT('Ctrl Pts',(8.10832637284494,12.2,6.78903322586174));
#205499=CARTESIAN_POINT('Ctrl Pts',(8.1053746047066,12.2,6.78747494571579));
#205500=CARTESIAN_POINT('Ctrl Pts',(8.10183248306929,12.2,6.78560500960859));
#205501=CARTESIAN_POINT('Ctrl Pts',(8.09833280324803,12.2,6.78374521185907));
#205502=CARTESIAN_POINT('Ctrl Pts',(8.09487586070512,12.2,6.78189617984245));
#205503=CARTESIAN_POINT('Ctrl Pts',(8.0914189178482,12.2,6.78004714765789));
#205504=CARTESIAN_POINT('Ctrl Pts',(8.08800470887987,12.2,6.77820888142463));
#205505=CARTESIAN_POINT('Ctrl Pts',(8.08463353686576,12.2,6.77638202507584));
#205506=CARTESIAN_POINT('Ctrl Pts',(8.08126236515784,12.2,6.77455516889299));
#205507=CARTESIAN_POINT('Ctrl Pts',(8.07793422624145,12.2,6.77273971960236));
#205508=CARTESIAN_POINT('Ctrl Pts',(8.07464942377936,12.2,6.7709363376684));
#205509=CARTESIAN_POINT('Ctrl Pts',(8.07136462131726,12.2,6.76913295573445));
#205510=CARTESIAN_POINT('Ctrl Pts',(8.06812315582669,12.2,6.76734163849119));
#205511=CARTESIAN_POINT('Ctrl Pts',(8.06492533044098,12.2,6.76556305963861));
#205512=CARTESIAN_POINT('Ctrl Pts',(8.06172750505528,12.2,6.76378448078601));
#205513=CARTESIAN_POINT('Ctrl Pts',(8.05857332152055,12.2,6.76201864013655));
#205514=CARTESIAN_POINT('Ctrl Pts',(8.05546309004723,12.2,6.76026622444931));
#205515=CARTESIAN_POINT('Ctrl Pts',(8.05235285829139,12.2,6.75851380860291));
#205516=CARTESIAN_POINT('Ctrl Pts',(8.04928657707312,12.2,6.7567748181494));
#205517=CARTESIAN_POINT('Ctrl Pts',(8.04626456232702,12.2,6.75504995822268));
#205518=CARTESIAN_POINT('Ctrl Pts',(8.0427388788683,12.2,6.75303762187651));
#205519=CARTESIAN_POINT('Ctrl Pts',(8.03927344600945,12.2,6.75104451508481));
#205520=CARTESIAN_POINT('Ctrl Pts',(8.0358687693013,12.2,6.74907178940094));
#205521=CARTESIAN_POINT('Ctrl Pts',(8.03295047463924,12.2,6.74738088147443));
#205522=CARTESIAN_POINT('Ctrl Pts',(8.03007681790642,12.2,6.74570494512434));
#205523=CARTESIAN_POINT('Ctrl Pts',(8.02724812333756,12.2,6.74404472445121));
#205524=CARTESIAN_POINT('Ctrl Pts',(8.02441942902563,12.2,6.74238450392889));
#205525=CARTESIAN_POINT('Ctrl Pts',(8.02163569701842,12.2,6.74073999717198));
#205526=CARTESIAN_POINT('Ctrl Pts',(8.01889725661596,12.2,6.73911196581375));
#205527=CARTESIAN_POINT('Ctrl Pts',(8.0161588162135,12.2,6.73748393445552));
#205528=CARTESIAN_POINT('Ctrl Pts',(8.0134656675454,12.2,6.73587237897535));
#205529=CARTESIAN_POINT('Ctrl Pts',(8.01081814330513,12.2,6.73427807594874));
#205530=CARTESIAN_POINT('Ctrl Pts',(8.00817061882438,12.2,6.73268377277733));
#205531=CARTESIAN_POINT('Ctrl Pts',(8.00556872181471,12.2,6.73110672459924));
#205532=CARTESIAN_POINT('Ctrl Pts',(8.00301278934409,12.2,6.72954773118173));
#205533=CARTESIAN_POINT('Ctrl Pts',(8.00003086847662,12.2,6.72772890574039));
#205534=CARTESIAN_POINT('Ctrl Pts',(7.99711151305915,12.2,6.72593465157874));
#205535=CARTESIAN_POINT('Ctrl Pts',(7.99425527027506,12.2,6.72416627542351));
#205536=CARTESIAN_POINT('Ctrl Pts',(7.99180706188851,12.2,6.7226505242563));
#205537=CARTESIAN_POINT('Ctrl Pts',(7.98940522491469,12.2,6.7211537867325));
#205538=CARTESIAN_POINT('Ctrl Pts',(7.98705010762171,12.2,6.71967690765288));
#205539=CARTESIAN_POINT('Ctrl Pts',(7.98469499054264,12.2,6.7182000287074));
#205540=CARTESIAN_POINT('Ctrl Pts',(7.9823865973208,12.2,6.71674300939667));
#205541=CARTESIAN_POINT('Ctrl Pts',(7.98012528497589,12.2,6.7153067175256));
#205542=CARTESIAN_POINT('Ctrl Pts',(7.97786397263098,12.2,6.71387042565454));
#205543=CARTESIAN_POINT('Ctrl Pts',(7.97564974154392,12.2,6.71245486093606));
#205544=CARTESIAN_POINT('Ctrl Pts',(7.97348295645272,12.2,6.71106091715189));
#205545=CARTESIAN_POINT('Ctrl Pts',(7.97131617116471,12.2,6.7096669732411));
#205546=CARTESIAN_POINT('Ctrl Pts',(7.96919683301319,12.2,6.70829465092577));
#205547=CARTESIAN_POINT('Ctrl Pts',(7.96712531629959,12.2,6.70694486611943));
#205548=CARTESIAN_POINT('Ctrl Pts',(7.96505379977415,12.2,6.70559508143567));
#205549=CARTESIAN_POINT('Ctrl Pts',(7.96303010065307,12.2,6.70426783511924));
#205550=CARTESIAN_POINT('Ctrl Pts',(7.96105460247486,12.2,6.70296407149994));
#205551=CARTESIAN_POINT('Ctrl Pts',(7.95907910429665,12.2,6.70166030788065));
#205552=CARTESIAN_POINT('Ctrl Pts',(7.95715180406014,12.2,6.70038002549835));
#205553=CARTESIAN_POINT('Ctrl Pts',(7.95527309369839,12.2,6.69912419889649));
#205554=CARTESIAN_POINT('Ctrl Pts',(7.953394383166,12.2,6.69786837218056));
#205555=CARTESIAN_POINT('Ctrl Pts',(7.95156425997445,12.2,6.69663699749083));
#205556=CARTESIAN_POINT('Ctrl Pts',(7.94978311979739,12.2,6.69543107717683));
#205557=CARTESIAN_POINT('Ctrl Pts',(7.94800197978211,12.2,6.69422515697239));
#205558=CARTESIAN_POINT('Ctrl Pts',(7.94626982492883,12.2,6.693044691721));
#205559=CARTESIAN_POINT('Ctrl Pts',(7.94458705698243,12.2,6.69189071050775));
#205560=CARTESIAN_POINT('Ctrl Pts',(7.94290428903604,12.2,6.6907367292945));
#205561=CARTESIAN_POINT('Ctrl Pts',(7.94127091035603,12.2,6.68960923087958));
#205562=CARTESIAN_POINT('Ctrl Pts',(7.93968733332804,12.2,6.688509280835));
#205563=CARTESIAN_POINT('Ctrl Pts',(7.93784742671344,12.2,6.68723128467378));
#205564=CARTESIAN_POINT('Ctrl Pts',(7.93607474793184,12.2,6.68599046144507));
#205565=CARTESIAN_POINT('Ctrl Pts',(7.93436996999994,12.2,6.68478856799998));
#205566=CARTESIAN_POINT('Ctrl Pts',(7.93436996999994,15.2,6.68478856799998));
#205567=CARTESIAN_POINT('Ctrl Pts',(7.93583020217336,15.2,6.68581805309871));
#205568=CARTESIAN_POINT('Ctrl Pts',(7.93734025309804,15.2,6.68687610405595));
#205569=CARTESIAN_POINT('Ctrl Pts',(7.9388996968374,15.2,6.68796160635605));
#205570=CARTESIAN_POINT('Ctrl Pts',(7.94046666100273,15.2,6.68905234349694));
#205571=CARTESIAN_POINT('Ctrl Pts',(7.94208349756759,15.2,6.69017080775629));
#205572=CARTESIAN_POINT('Ctrl Pts',(7.94374979091117,15.2,6.69131593187745));
#205573=CARTESIAN_POINT('Ctrl Pts',(7.9454160841034,15.2,6.69246105589459));
#205574=CARTESIAN_POINT('Ctrl Pts',(7.94713183283063,15.2,6.69363283707676));
#205575=CARTESIAN_POINT('Ctrl Pts',(7.94889663376652,15.2,6.69483024319994));
#205576=CARTESIAN_POINT('Ctrl Pts',(7.95066143470242,15.2,6.69602764932311));
#205577=CARTESIAN_POINT('Ctrl Pts',(7.95247528578891,15.2,6.6972506792804));
#205578=CARTESIAN_POINT('Ctrl Pts',(7.95433778906148,15.2,6.69849832762931));
#205579=CARTESIAN_POINT('Ctrl Pts',(7.9562002925032,15.2,6.69974597609154));
#205580=CARTESIAN_POINT('Ctrl Pts',(7.95811145072005,15.2,6.70101824167729));
#205581=CARTESIAN_POINT('Ctrl Pts',(7.96007087199678,15.2,6.7023141511662));
#205582=CARTESIAN_POINT('Ctrl Pts',(7.96203029309555,15.2,6.70361006053739));
#205583=CARTESIAN_POINT('Ctrl Pts',(7.96403797768271,15.2,6.70492961203486));
#205584=CARTESIAN_POINT('Ctrl Pts',(7.96609354478413,15.2,6.70627185674222));
#205585=CARTESIAN_POINT('Ctrl Pts',(7.96814911188555,15.2,6.70761410144959));
#205586=CARTESIAN_POINT('Ctrl Pts',(7.9702525611464,15.2,6.70897904048412));
#205587=CARTESIAN_POINT('Ctrl Pts',(7.9724035193995,15.2,6.71036575118279));
#205588=CARTESIAN_POINT('Ctrl Pts',(7.97455447784797,15.2,6.71175246200742));
#205589=CARTESIAN_POINT('Ctrl Pts',(7.97675294572737,15.2,6.71316094522642));
#205590=CARTESIAN_POINT('Ctrl Pts',(7.97899855426965,15.2,6.71459030313909));
#205591=CARTESIAN_POINT('Ctrl Pts',(7.98124416260797,15.2,6.71601966092194));
#205592=CARTESIAN_POINT('Ctrl Pts',(7.98353691226888,15.2,6.71746989346604));
#205593=CARTESIAN_POINT('Ctrl Pts',(7.98587644460257,15.2,6.71894012758016));
#205594=CARTESIAN_POINT('Ctrl Pts',(7.98821597693625,15.2,6.72041036169427));
#205595=CARTESIAN_POINT('Ctrl Pts',(7.99060229026621,15.2,6.72190059904011));
#205596=CARTESIAN_POINT('Ctrl Pts',(7.99303503159248,15.2,6.72340998815111));
#205597=CARTESIAN_POINT('Ctrl Pts',(7.99587322995379,15.2,6.72517094220533));
#205598=CARTESIAN_POINT('Ctrl Pts',(7.9987746229845,15.2,6.72695796531665));
#205599=CARTESIAN_POINT('Ctrl Pts',(8.00173865588018,15.2,6.728769743068));
#205600=CARTESIAN_POINT('Ctrl Pts',(8.00427925537319,15.2,6.73032269534568));
#205601=CARTESIAN_POINT('Ctrl Pts',(8.00686587926256,15.2,6.73189383758858));
#205602=CARTESIAN_POINT('Ctrl Pts',(8.0094981845816,15.2,6.73348236586345));
#205603=CARTESIAN_POINT('Ctrl Pts',(8.01213048990063,15.2,6.73507089413831));
#205604=CARTESIAN_POINT('Ctrl Pts',(8.01480847849673,15.2,6.73667680914985));
#205605=CARTESIAN_POINT('Ctrl Pts',(8.01753181197804,15.2,6.73829932658978));
#205606=CARTESIAN_POINT('Ctrl Pts',(8.02025514570673,15.2,6.73992184417708));
#205607=CARTESIAN_POINT('Ctrl Pts',(8.02302382724809,15.2,6.74156096571598));
#205608=CARTESIAN_POINT('Ctrl Pts',(8.0258375249034,15.2,6.74321592730689));
#205609=CARTESIAN_POINT('Ctrl Pts',(8.02865122230314,15.2,6.74487088874745));
#205610=CARTESIAN_POINT('Ctrl Pts',(8.0315099365576,15.2,6.74654168994505));
#205611=CARTESIAN_POINT('Ctrl Pts',(8.03441334286682,15.2,6.74822758646647));
#205612=CARTESIAN_POINT('Ctrl Pts',(8.03731674917604,15.2,6.74991348298789));
#205613=CARTESIAN_POINT('Ctrl Pts',(8.04026484617711,15.2,6.75161447488462));
#205614=CARTESIAN_POINT('Ctrl Pts',(8.0432573146487,15.2,6.75332983457132));
#205615=CARTESIAN_POINT('Ctrl Pts',(8.04674852804677,15.2,6.755331087643));
#205616=CARTESIAN_POINT('Ctrl Pts',(8.05030013778289,15.2,6.75735189628479));
#205617=CARTESIAN_POINT('Ctrl Pts',(8.05391163811468,15.2,6.75939113816309));
#205618=CARTESIAN_POINT('Ctrl Pts',(8.05700720966694,15.2,6.76113905968233));
#205619=CARTESIAN_POINT('Ctrl Pts',(8.06014678600487,15.2,6.76290052075525));
#205620=CARTESIAN_POINT('Ctrl Pts',(8.06333005538623,15.2,6.76467483452324));
#205621=CARTESIAN_POINT('Ctrl Pts',(8.06651332505673,15.2,6.76644914845239));
#205622=CARTESIAN_POINT('Ctrl Pts',(8.0697402869565,15.2,6.76823631448283));
#205623=CARTESIAN_POINT('Ctrl Pts',(8.07301063571995,15.2,6.77003565558141));
#205624=CARTESIAN_POINT('Ctrl Pts',(8.07628098418636,15.2,6.77183499651657));
#205625=CARTESIAN_POINT('Ctrl Pts',(8.07959471940516,15.2,6.77364651499044));
#205626=CARTESIAN_POINT('Ctrl Pts',(8.08295153879835,15.2,6.7754695507658));
#205627=CARTESIAN_POINT('Ctrl Pts',(8.08630835819154,15.2,6.77729258654116));
#205628=CARTESIAN_POINT('Ctrl Pts',(8.08970826191097,15.2,6.77912713888328));
#205629=CARTESIAN_POINT('Ctrl Pts',(8.0931509513663,15.2,6.78097256381548));
#205630=CARTESIAN_POINT('Ctrl Pts',(8.09659364113434,15.2,6.78281798891532));
#205631=CARTESIAN_POINT('Ctrl Pts',(8.10007911544526,15.2,6.78467428644332));
#205632=CARTESIAN_POINT('Ctrl Pts',(8.10360708239959,15.2,6.78654082572222));
#205633=CARTESIAN_POINT('Ctrl Pts',(8.1065470547013,15.2,6.78809627503655));
#205634=CARTESIAN_POINT('Ctrl Pts',(8.10951653305084,15.2,6.78965883764913));
#205635=CARTESIAN_POINT('Ctrl Pts',(8.11251535110879,15.2,6.79122815445524));
#205636=CARTESIAN_POINT('Ctrl Pts',(8.11611393264758,15.2,6.79311133455415));
#205637=CARTESIAN_POINT('Ctrl Pts',(8.11975476271853,15.2,6.79500424012795));
#205638=CARTESIAN_POINT('Ctrl Pts',(8.12343755226821,15.2,6.79690626823417));
#205639=CARTESIAN_POINT('Ctrl Pts',(8.1271203418179,15.2,6.79880829634039));
#205640=CARTESIAN_POINT('Ctrl Pts',(8.13084509115011,15.2,6.80071944428217));
#205641=CARTESIAN_POINT('Ctrl Pts',(8.13461151384478,15.2,6.80263912137872));
#205642=CARTESIAN_POINT('Ctrl Pts',(8.13900567388331,15.2,6.80487874477428));
#205643=CARTESIAN_POINT('Ctrl Pts',(8.14345655804975,15.2,6.80712997304422));
#205644=CARTESIAN_POINT('Ctrl Pts',(8.14796371775163,15.2,6.80939188824252));
#205645=CARTESIAN_POINT('Ctrl Pts',(8.15118311748855,15.2,6.81100754193043));
#205646=CARTESIAN_POINT('Ctrl Pts',(8.15443123042951,15.2,6.81262864849498));
#205647=CARTESIAN_POINT('Ctrl Pts',(8.15770789355601,15.2,6.81425487960636));
#205648=CARTESIAN_POINT('Ctrl Pts',(8.16098455668251,15.2,6.81588111071774));
#205649=CARTESIAN_POINT('Ctrl Pts',(8.16428977108326,15.2,6.81751246501231));
#205650=CARTESIAN_POINT('Ctrl Pts',(8.16762337670973,15.2,6.81914862112368));
#205651=CARTESIAN_POINT('Ctrl Pts',(8.17095698233621,15.2,6.82078477723504));
#205652=CARTESIAN_POINT('Ctrl Pts',(8.17431897920554,15.2,6.82242573547515));
#205653=CARTESIAN_POINT('Ctrl Pts',(8.17770920916852,15.2,6.82407117597433));
#205654=CARTESIAN_POINT('Ctrl Pts',(8.18177748497631,15.2,6.8260457045016));
#205655=CARTESIAN_POINT('Ctrl Pts',(8.18588641492562,15.2,6.82802668918051));
#205656=CARTESIAN_POINT('Ctrl Pts',(8.19003572952487,15.2,6.83001359252497));
#205657=CARTESIAN_POINT('Ctrl Pts',(8.19418504412412,15.2,6.83200049586945));
#205658=CARTESIAN_POINT('Ctrl Pts',(8.19837474213551,15.2,6.83399331565477));
#205659=CARTESIAN_POINT('Ctrl Pts',(8.20260455585746,15.2,6.83599152609835));
#205660=CARTESIAN_POINT('Ctrl Pts',(8.20612940075384,15.2,6.8376567015285));
#205661=CARTESIAN_POINT('Ctrl Pts',(8.20968210262846,15.2,6.8393256200797));
#205662=CARTESIAN_POINT('Ctrl Pts',(8.21326250901588,15.2,6.84099798139896));
#205663=CARTESIAN_POINT('Ctrl Pts',(8.21684291540332,15.2,6.84267034271821));
#205664=CARTESIAN_POINT('Ctrl Pts',(8.22045102477482,15.2,6.8443461460959));
#205665=CARTESIAN_POINT('Ctrl Pts',(8.22408668532894,15.2,6.84602509887353));
#205666=CARTESIAN_POINT('Ctrl Pts',(8.22917661018398,15.2,6.84837563279879));
#205667=CARTESIAN_POINT('Ctrl Pts',(8.23432053330838,15.2,6.85073233402004));
#205668=CARTESIAN_POINT('Ctrl Pts',(8.23951804226024,15.2,6.8530944102759));
#205669=CARTESIAN_POINT('Ctrl Pts',(8.24397304970202,15.2,6.85511904696153));
#205670=CARTESIAN_POINT('Ctrl Pts',(8.24846742258604,15.2,6.85714763152989));
#205671=CARTESIAN_POINT('Ctrl Pts',(8.25300090525296,15.2,6.85917967612258));
#205672=CARTESIAN_POINT('Ctrl Pts',(8.25677880761266,15.2,6.86087304667802));
#205673=CARTESIAN_POINT('Ctrl Pts',(8.26058386717306,15.2,6.86256881853906));
#205674=CARTESIAN_POINT('Ctrl Pts',(8.26441593849109,15.2,6.86426671416395));
#205675=CARTESIAN_POINT('Ctrl Pts',(8.2674815957126,15.2,6.86562503073789));
#205676=CARTESIAN_POINT('Ctrl Pts',(8.27056453818561,15.2,6.86698470646354));
#205677=CARTESIAN_POINT('Ctrl Pts',(8.27366469173316,15.2,6.86834560043913));
#205678=CARTESIAN_POINT('Ctrl Pts',(8.27676484485831,15.2,6.8697064942293));
#205679=CARTESIAN_POINT('Ctrl Pts',(8.27988220832615,15.2,6.87106860519172));
#205680=CARTESIAN_POINT('Ctrl Pts',(8.28301670723546,15.2,6.87243179691355));
#205681=CARTESIAN_POINT('Ctrl Pts',(8.28693483119239,15.2,6.87413578670513));
#205682=CARTESIAN_POINT('Ctrl Pts',(8.29087972869169,15.2,6.87584146109397));
#205683=CARTESIAN_POINT('Ctrl Pts',(8.29485125348197,15.2,6.87754855512168));
#205684=CARTESIAN_POINT('Ctrl Pts',(8.29802847348734,15.2,6.87891423041827));
#205685=CARTESIAN_POINT('Ctrl Pts',(8.30122273636515,15.2,6.8802808128305));
#205686=CARTESIAN_POINT('Ctrl Pts',(8.30443396542428,15.2,6.8816481694734));
#205687=CARTESIAN_POINT('Ctrl Pts',(8.30764519404587,15.2,6.88301552592999));
#205688=CARTESIAN_POINT('Ctrl Pts',(8.31087339048169,15.2,6.88438365272502));
#205689=CARTESIAN_POINT('Ctrl Pts',(8.31411847949309,15.2,6.88575242044642));
#205690=CARTESIAN_POINT('Ctrl Pts',(8.31736356894661,15.2,6.88712118835431));
#205691=CARTESIAN_POINT('Ctrl Pts',(8.32062555191328,15.2,6.88849059515674));
#205692=CARTESIAN_POINT('Ctrl Pts',(8.32390435525974,15.2,6.88986050862031));
#205693=CARTESIAN_POINT('Ctrl Pts',(8.32882255983269,15.2,6.89191537862903));
#205694=CARTESIAN_POINT('Ctrl Pts',(8.33377860822313,15.2,6.8939713904061));
#205695=CARTESIAN_POINT('Ctrl Pts',(8.33877225306428,15.2,6.89602810325738));
#205696=CARTESIAN_POINT('Ctrl Pts',(8.34293362391644,15.2,6.89774203069572));
#205697=CARTESIAN_POINT('Ctrl Pts',(8.34712110417766,15.2,6.89945644667221));
#205698=CARTESIAN_POINT('Ctrl Pts',(8.3513345522332,15.2,6.90117109924165));
#205699=CARTESIAN_POINT('Ctrl Pts',(8.35639068971615,15.2,6.90322868225023));
#205700=CARTESIAN_POINT('Ctrl Pts',(8.36148422029424,15.2,6.90528660824788));
#205701=CARTESIAN_POINT('Ctrl Pts',(8.36661490027864,15.2,6.90734444952591));
#205702=CARTESIAN_POINT('Ctrl Pts',(8.37003535391226,15.2,6.90871634383588));
#205703=CARTESIAN_POINT('Ctrl Pts',(8.37347231927362,15.2,6.91008820280404));
#205704=CARTESIAN_POINT('Ctrl Pts',(8.37692572274069,15.2,6.91145990087879));
#205705=CARTESIAN_POINT('Ctrl Pts',(8.38037912573722,15.2,6.91283159876665));
#205706=CARTESIAN_POINT('Ctrl Pts',(8.38384896876655,15.2,6.91420313515452));
#205707=CARTESIAN_POINT('Ctrl Pts',(8.38733517914656,15.2,6.91557438904245));
#205708=CARTESIAN_POINT('Ctrl Pts',(8.39082139000155,15.2,6.91694564311721));
#205709=CARTESIAN_POINT('Ctrl Pts',(8.39432396855558,15.2,6.91831661176722));
#205710=CARTESIAN_POINT('Ctrl Pts',(8.39784284398562,15.2,6.91968717779259));
#205711=CARTESIAN_POINT('Ctrl Pts',(8.4013617189362,15.2,6.92105774363121));
#205712=CARTESIAN_POINT('Ctrl Pts',(8.40489689168066,15.2,6.92242790392408));
#205713=CARTESIAN_POINT('Ctrl Pts',(8.40844828944424,15.2,6.92379754053439));
#205714=CARTESIAN_POINT('Ctrl Pts',(8.4128875370116,15.2,6.92550958643724));
#205715=CARTESIAN_POINT('Ctrl Pts',(8.41735213705356,15.2,6.92722081255954));
#205716=CARTESIAN_POINT('Ctrl Pts',(8.42184195441262,15.2,6.92893098776796));
#205717=CARTESIAN_POINT('Ctrl Pts',(8.42543380849563,15.2,6.93029912800927));
#205718=CARTESIAN_POINT('Ctrl Pts',(8.42904179966334,15.2,6.93166659563968));
#205719=CARTESIAN_POINT('Ctrl Pts',(8.43266585971069,15.2,6.93303327444259));
#205720=CARTESIAN_POINT('Ctrl Pts',(8.43628991926425,15.2,6.93439995305928));
#205721=CARTESIAN_POINT('Ctrl Pts',(8.43993004723596,15.2,6.93576584229665));
#205722=CARTESIAN_POINT('Ctrl Pts',(8.44358617293545,15.2,6.93713082701848));
#205723=CARTESIAN_POINT('Ctrl Pts',(8.44724229913307,15.2,6.9384958119263));
#205724=CARTESIAN_POINT('Ctrl Pts',(8.45091442455165,15.2,6.93985989181737));
#205725=CARTESIAN_POINT('Ctrl Pts',(8.45460247747488,15.2,6.94122295272499));
#205726=CARTESIAN_POINT('Ctrl Pts',(8.4582905303981,15.2,6.94258601363261));
#205727=CARTESIAN_POINT('Ctrl Pts',(8.46199451388984,15.2,6.94394805657623));
#205728=CARTESIAN_POINT('Ctrl Pts',(8.46571435614975,15.2,6.94530896620583));
#205729=CARTESIAN_POINT('Ctrl Pts',(8.46943419790283,15.2,6.94666987565001));
#205730=CARTESIAN_POINT('Ctrl Pts',(8.47316990067037,15.2,6.9480296532595));
#205731=CARTESIAN_POINT('Ctrl Pts',(8.47692139304733,15.2,6.94938818726573));
#205732=CARTESIAN_POINT('Ctrl Pts',(8.48067288593543,15.2,6.95074672145705));
#205733=CARTESIAN_POINT('Ctrl Pts',(8.4844401705273,15.2,6.95210401142293));
#205734=CARTESIAN_POINT('Ctrl Pts',(8.48822317740175,15.2,6.95345994766336));
#205735=CARTESIAN_POINT('Ctrl Pts',(8.49200618376075,15.2,6.95481588371903));
#205736=CARTESIAN_POINT('Ctrl Pts',(8.4958049122955,15.2,6.95617046591377));
#205737=CARTESIAN_POINT('Ctrl Pts',(8.49961929520487,15.2,6.95752358341436));
#205738=CARTESIAN_POINT('Ctrl Pts',(8.50343367863396,15.2,6.95887670109932));
#205739=CARTESIAN_POINT('Ctrl Pts',(8.5072637163538,15.2,6.96022835550076));
#205740=CARTESIAN_POINT('Ctrl Pts',(8.51110934056441,15.2,6.96157843785201));
#205741=CARTESIAN_POINT('Ctrl Pts',(8.51495496425105,15.2,6.96292852001931));
#205742=CARTESIAN_POINT('Ctrl Pts',(8.51881617377869,15.2,6.96427703102499));
#205743=CARTESIAN_POINT('Ctrl Pts',(8.5226929016541,15.2,6.96562386253788));
#205744=CARTESIAN_POINT('Ctrl Pts',(8.52656963005771,15.2,6.96697069423427));
#205745=CARTESIAN_POINT('Ctrl Pts',(8.53046187844162,15.2,6.96831584733116));
#205746=CARTESIAN_POINT('Ctrl Pts',(8.53436957604449,15.2,6.96965921562646));
#205747=CARTESIAN_POINT('Ctrl Pts',(8.53925419778185,15.2,6.97133842590408));
#205748=CARTESIAN_POINT('Ctrl Pts',(8.54416296360471,15.2,6.97301484654846));
#205749=CARTESIAN_POINT('Ctrl Pts',(8.54909573860597,15.2,6.97468827515942));
#205750=CARTESIAN_POINT('Ctrl Pts',(8.55304195828437,15.2,6.97602701793874));
#205751=CARTESIAN_POINT('Ctrl Pts',(8.55700354563677,15.2,6.97736384454578));
#205752=CARTESIAN_POINT('Ctrl Pts',(8.5609804328979,15.2,6.97869865278129));
#205753=CARTESIAN_POINT('Ctrl Pts',(8.5659515423807,15.2,6.98036716321209));
#205754=CARTESIAN_POINT('Ctrl Pts',(8.57094655775082,15.2,6.98203252032999));
#205755=CARTESIAN_POINT('Ctrl Pts',(8.57596535018013,15.2,6.98369452164961));
#205756=CARTESIAN_POINT('Ctrl Pts',(8.58098414260944,15.2,6.98535652296923));
#205757=CARTESIAN_POINT('Ctrl Pts',(8.58602671143105,15.2,6.98701517233044));
#205758=CARTESIAN_POINT('Ctrl Pts',(8.5910929271937,15.2,6.98867026865006));
#205759=CARTESIAN_POINT('Ctrl Pts',(8.59514590002471,15.2,6.98999434577792));
#205760=CARTESIAN_POINT('Ctrl Pts',(8.59921400666464,15.2,6.99131615112604));
#205761=CARTESIAN_POINT('Ctrl Pts',(8.60329718109246,15.2,6.99263558370811));
#205762=CARTESIAN_POINT('Ctrl Pts',(8.60738035496396,15.2,6.9939550161104));
#205763=CARTESIAN_POINT('Ctrl Pts',(8.61147859665379,15.2,6.99527207738314));
#205764=CARTESIAN_POINT('Ctrl Pts',(8.6155918403721,15.2,6.99658666694251));
#205765=CARTESIAN_POINT('Ctrl Pts',(8.62073339544031,15.2,6.99822990402604));
#205766=CARTESIAN_POINT('Ctrl Pts',(8.62589839201748,15.2,6.99986928193725));
#205767=CARTESIAN_POINT('Ctrl Pts',(8.63108670041905,15.2,7.00150460665969));
#205768=CARTESIAN_POINT('Ctrl Pts',(8.63523734736651,15.2,7.00281286650893));
#205769=CARTESIAN_POINT('Ctrl Pts',(8.63940291529916,15.2,7.00411853426429));
#205770=CARTESIAN_POINT('Ctrl Pts',(8.64358333834824,15.2,7.00542151395572));
#205771=CARTESIAN_POINT('Ctrl Pts',(8.64880886687479,15.2,7.00705023848124));
#205772=CARTESIAN_POINT('Ctrl Pts',(8.65405760473756,15.2,7.00867475937892));
#205773=CARTESIAN_POINT('Ctrl Pts',(8.65932942723945,15.2,7.01029489396191));
#205774=CARTESIAN_POINT('Ctrl Pts',(8.66460124974133,15.2,7.01191502854488));
#205775=CARTESIAN_POINT('Ctrl Pts',(8.66989615470471,15.2,7.01353077432778));
#205776=CARTESIAN_POINT('Ctrl Pts',(8.67521401797047,15.2,7.01514194974407));
#205777=CARTESIAN_POINT('Ctrl Pts',(8.678404735814,15.2,7.01610865495873));
#205778=CARTESIAN_POINT('Ctrl Pts',(8.68160371834249,15.2,7.01707371485678));
#205779=CARTESIAN_POINT('Ctrl Pts',(8.68481093838715,15.2,7.01803708920303));
#205780=CARTESIAN_POINT('Ctrl Pts',(8.69015630532246,15.2,7.01964271317181));
#205781=CARTESIAN_POINT('Ctrl Pts',(8.69552455294763,15.2,7.02124365742027));
#205782=CARTESIAN_POINT('Ctrl Pts',(8.7009155564217,15.2,7.02283974047543));
#205783=CARTESIAN_POINT('Ctrl Pts',(8.70522835884839,15.2,7.02411660681517));
#205784=CARTESIAN_POINT('Ctrl Pts',(8.70955572516209,15.2,7.02539036435254));
#205785=CARTESIAN_POINT('Ctrl Pts',(8.71389759136174,15.2,7.02666091863777));
#205786=CARTESIAN_POINT('Ctrl Pts',(8.71823945815298,15.2,7.02793147309611));
#205787=CARTESIAN_POINT('Ctrl Pts',(8.7225958249986,15.2,7.02919882436553));
#205788=CARTESIAN_POINT('Ctrl Pts',(8.72696662690087,15.2,7.03046288544174));
#205789=CARTESIAN_POINT('Ctrl Pts',(8.73133742820762,15.2,7.03172694634571));
#205790=CARTESIAN_POINT('Ctrl Pts',(8.73572266593428,15.2,7.03298771405252));
#205791=CARTESIAN_POINT('Ctrl Pts',(8.74012227490702,15.2,7.03424510167218));
#205792=CARTESIAN_POINT('Ctrl Pts',(8.74342198178643,15.2,7.03518814242974));
#205793=CARTESIAN_POINT('Ctrl Pts',(8.74672977284861,15.2,7.03612928097911));
#205794=CARTESIAN_POINT('Ctrl Pts',(8.7500456212687,15.2,7.03706847932025));
#205795=CARTESIAN_POINT('Ctrl Pts',(8.75336147029117,15.2,7.03800767783202));
#205796=CARTESIAN_POINT('Ctrl Pts',(8.75668537695759,15.2,7.03894493760156));
#205797=CARTESIAN_POINT('Ctrl Pts',(8.76001731444292,15.2,7.03988022148722));
#205798=CARTESIAN_POINT('Ctrl Pts',(8.76334925132296,15.2,7.04081550520297));
#205799=CARTESIAN_POINT('Ctrl Pts',(8.76668921910117,15.2,7.04174881133438));
#205800=CARTESIAN_POINT('Ctrl Pts',(8.77003719064772,15.2,7.04268010468016));
#205801=CARTESIAN_POINT('Ctrl Pts',(8.77338516219426,15.2,7.04361139802594));
#205802=CARTESIAN_POINT('Ctrl Pts',(8.77674113722156,15.2,7.04454067848491));
#205803=CARTESIAN_POINT('Ctrl Pts',(8.78010509010003,15.2,7.0454679083677));
#205804=CARTESIAN_POINT('Ctrl Pts',(8.78346904297849,15.2,7.0463951382505));
#205805=CARTESIAN_POINT('Ctrl Pts',(8.78684097383936,15.2,7.04732031893354));
#205806=CARTESIAN_POINT('Ctrl Pts',(8.79022085479988,15.2,7.04824341369167));
#205807=CARTESIAN_POINT('Ctrl Pts',(8.79360073576041,15.2,7.04916650844979));
#205808=CARTESIAN_POINT('Ctrl Pts',(8.79698856788729,15.2,7.050087516683));
#205809=CARTESIAN_POINT('Ctrl Pts',(8.80038432380488,15.2,7.05100640294147));
#205810=CARTESIAN_POINT('Ctrl Pts',(8.80378007972247,15.2,7.05192528919994));
#205811=CARTESIAN_POINT('Ctrl Pts',(8.80718375964434,15.2,7.05284205296031));
#205812=CARTESIAN_POINT('Ctrl Pts',(8.81059533860658,15.2,7.05375665930636));
#205813=CARTESIAN_POINT('Ctrl Pts',(8.81514411096941,15.2,7.05497613454518));
#205814=CARTESIAN_POINT('Ctrl Pts',(8.81970692394604,15.2,7.05619177325824));
#205815=CARTESIAN_POINT('Ctrl Pts',(8.82428371364084,15.2,7.05740349182402));
#205816=CARTESIAN_POINT('Ctrl Pts',(8.82771630560014,15.2,7.05831228066581));
#205817=CARTESIAN_POINT('Ctrl Pts',(8.83115676039184,15.2,7.05921886484952));
#205818=CARTESIAN_POINT('Ctrl Pts',(8.83460505222489,15.2,7.06012320773334));
#205819=CARTESIAN_POINT('Ctrl Pts',(8.84035220548878,15.2,7.06163044592778));
#205820=CARTESIAN_POINT('Ctrl Pts',(8.84612112553322,15.2,7.06313146240556));
#205821=CARTESIAN_POINT('Ctrl Pts',(8.85191169219989,15.2,7.06462609455834));
#205822=CARTESIAN_POINT('Ctrl Pts',(8.85538603207365,15.2,7.06552287381742));
#205823=CARTESIAN_POINT('Ctrl Pts',(8.85886816501377,15.2,7.06641735453493));
#205824=CARTESIAN_POINT('Ctrl Pts',(8.86235806388629,15.2,7.06730950191939));
#205825=CARTESIAN_POINT('Ctrl Pts',(8.8658479627588,15.2,7.06820164930383));
#205826=CARTESIAN_POINT('Ctrl Pts',(8.86934562747489,15.2,7.06909146398258));
#205827=CARTESIAN_POINT('Ctrl Pts',(8.87285103356343,15.2,7.06997891232828));
#205828=CARTESIAN_POINT('Ctrl Pts',(8.87635643965195,15.2,7.07086636067398));
#205829=CARTESIAN_POINT('Ctrl Pts',(8.87986958697799,15.2,7.07175144172265));
#205830=CARTESIAN_POINT('Ctrl Pts',(8.88339044697402,15.2,7.07263412156592));
#205831=CARTESIAN_POINT('Ctrl Pts',(8.88691130760967,15.2,7.07351680156952));
#205832=CARTESIAN_POINT('Ctrl Pts',(8.89043988288915,15.2,7.07439708039745));
#205833=CARTESIAN_POINT('Ctrl Pts',(8.89397614648747,15.2,7.07527492444137));
#205834=CARTESIAN_POINT('Ctrl Pts',(8.89751240944337,15.2,7.07615276832581));
#205835=CARTESIAN_POINT('Ctrl Pts',(8.90105636173219,15.2,7.07702817797705));
#205836=CARTESIAN_POINT('Ctrl Pts',(8.90460797560381,15.2,7.07790111882011));
#205837=CARTESIAN_POINT('Ctrl Pts',(8.90815958947543,15.2,7.07877405966317));
#205838=CARTESIAN_POINT('Ctrl Pts',(8.9117188656665,15.2,7.07964453202839));
#205839=CARTESIAN_POINT('Ctrl Pts',(8.9152857780948,15.2,7.08051250379246));
#205840=CARTESIAN_POINT('Ctrl Pts',(8.92004166111654,15.2,7.08166979942532));
#205841=CARTESIAN_POINT('Ctrl Pts',(8.92481112116026,15.2,7.08282264736955));
#205842=CARTESIAN_POINT('Ctrl Pts',(8.92959409476788,15.2,7.08397096855392));
#205843=CARTESIAN_POINT('Ctrl Pts',(8.93318132578819,15.2,7.08483220963776));
#205844=CARTESIAN_POINT('Ctrl Pts',(8.93677615801064,15.2,7.08569090512924));
#205845=CARTESIAN_POINT('Ctrl Pts',(8.94037856753523,15.2,7.08654702266997));
#205846=CARTESIAN_POINT('Ctrl Pts',(8.94518177914394,15.2,7.08768851246506));
#205847=CARTESIAN_POINT('Ctrl Pts',(8.94999845940367,15.2,7.0888254192441));
#205848=CARTESIAN_POINT('Ctrl Pts',(8.95482854839683,15.2,7.0899576657074));
#205849=CARTESIAN_POINT('Ctrl Pts',(8.96086616013184,15.2,7.09137297390223));
#205850=CARTESIAN_POINT('Ctrl Pts',(8.96692472264126,15.2,7.09278100124842));
#205851=CARTESIAN_POINT('Ctrl Pts',(8.97300411273825,15.2,7.09418159278257));
#205852=CARTESIAN_POINT('Ctrl Pts',(8.97665174666391,15.2,7.09502194767254));
#205853=CARTESIAN_POINT('Ctrl Pts',(8.98030687810118,15.2,7.09585962672239));
#205854=CARTESIAN_POINT('Ctrl Pts',(8.98396948459246,15.2,7.09669459969228));
#205855=CARTESIAN_POINT('Ctrl Pts',(8.98763209108373,15.2,7.09752957266218));
#205856=CARTESIAN_POINT('Ctrl Pts',(8.99130217374949,15.2,7.09836184023226));
#205857=CARTESIAN_POINT('Ctrl Pts',(8.99497970615653,15.2,7.09919137303583));
#205858=CARTESIAN_POINT('Ctrl Pts',(8.99865723923164,15.2,7.1000209059901));
#205859=CARTESIAN_POINT('Ctrl Pts',(9.00234222280053,15.2,7.10084770277693));
#205860=CARTESIAN_POINT('Ctrl Pts',(9.00603462575484,15.2,7.10167172614631));
#205861=CARTESIAN_POINT('Ctrl Pts',(9.01218862911353,15.2,7.10304509807931));
#205862=CARTESIAN_POINT('Ctrl Pts',(9.01836323491096,15.2,7.10441075245865));
#205863=CARTESIAN_POINT('Ctrl Pts',(9.02455833645625,15.2,7.1057685652974));
#205864=CARTESIAN_POINT('Ctrl Pts',(9.0295144185028,15.2,7.106854815746));
#205865=CARTESIAN_POINT('Ctrl Pts',(9.03448362264226,15.2,7.1079360497067));
#205866=CARTESIAN_POINT('Ctrl Pts',(9.03946594399994,15.2,7.10901226999999));
#205867=CARTESIAN_POINT('Ctrl Pts',(8.56667970899995,15.2,5.85257411499998));
#205868=CARTESIAN_POINT('Ctrl Pts',(8.56667970899995,11.6,5.85257411499998));
#205869=CARTESIAN_POINT('Ctrl Pts',(8.56681469199994,15.2,5.85268447899999));
#205870=CARTESIAN_POINT('Ctrl Pts',(8.56681469199994,11.6,5.85268447899999));
#205871=CARTESIAN_POINT('Ctrl Pts',(8.56708931799994,15.2,5.85290912899998));
#205872=CARTESIAN_POINT('Ctrl Pts',(8.56708931799994,11.6,5.85290912899998));
#205873=CARTESIAN_POINT('Ctrl Pts',(8.56750527399995,15.2,5.85324973199998));
#205874=CARTESIAN_POINT('Ctrl Pts',(8.56750527399995,11.6,5.85324973199998));
#205875=CARTESIAN_POINT('Ctrl Pts',(8.56806526099994,15.2,5.85370897499998));
#205876=CARTESIAN_POINT('Ctrl Pts',(8.56806526099994,11.6,5.85370897499998));
#205877=CARTESIAN_POINT('Ctrl Pts',(8.56877298299995,15.2,5.85429055399998));
#205878=CARTESIAN_POINT('Ctrl Pts',(8.56877298299995,11.6,5.85429055399998));
#205879=CARTESIAN_POINT('Ctrl Pts',(8.56949158199994,15.2,5.85488228199999));
#205880=CARTESIAN_POINT('Ctrl Pts',(8.56949158199994,11.6,5.85488228199999));
#205881=CARTESIAN_POINT('Ctrl Pts',(8.57021692599995,15.2,5.85548078499999));
#205882=CARTESIAN_POINT('Ctrl Pts',(8.57021692599995,11.6,5.85548078499999));
#205883=CARTESIAN_POINT('Ctrl Pts',(8.57094898299994,15.2,5.85608606099999));
#205884=CARTESIAN_POINT('Ctrl Pts',(8.57094898299994,11.6,5.85608606099999));
#205885=CARTESIAN_POINT('Ctrl Pts',(8.57168771799994,15.2,5.85669810599998));
#205886=CARTESIAN_POINT('Ctrl Pts',(8.57168771799994,11.6,5.85669810599998));
#205887=CARTESIAN_POINT('Ctrl Pts',(8.57243310299994,15.2,5.85731691899999));
#205888=CARTESIAN_POINT('Ctrl Pts',(8.57243310299994,11.6,5.85731691899999));
#205889=CARTESIAN_POINT('Ctrl Pts',(8.57318510299995,15.2,5.85794249299998));
#205890=CARTESIAN_POINT('Ctrl Pts',(8.57318510299995,11.6,5.85794249299998));
#205891=CARTESIAN_POINT('Ctrl Pts',(8.57394368799994,15.2,5.85857482799998));
#205892=CARTESIAN_POINT('Ctrl Pts',(8.57394368799994,11.6,5.85857482799998));
#205893=CARTESIAN_POINT('Ctrl Pts',(8.57470882599995,15.2,5.85921391999998));
#205894=CARTESIAN_POINT('Ctrl Pts',(8.57470882599995,11.6,5.85921391999998));
#205895=CARTESIAN_POINT('Ctrl Pts',(8.57548048599994,15.2,5.85985976499998));
#205896=CARTESIAN_POINT('Ctrl Pts',(8.57548048599994,11.6,5.85985976499998));
#205897=CARTESIAN_POINT('Ctrl Pts',(8.57625863499995,15.2,5.86051236099999));
#205898=CARTESIAN_POINT('Ctrl Pts',(8.57625863499995,11.6,5.86051236099999));
#205899=CARTESIAN_POINT('Ctrl Pts',(8.57704324399995,15.2,5.86117170499998));
#205900=CARTESIAN_POINT('Ctrl Pts',(8.57704324399995,11.6,5.86117170499998));
#205901=CARTESIAN_POINT('Ctrl Pts',(8.57783427999994,15.2,5.86183779199998));
#205902=CARTESIAN_POINT('Ctrl Pts',(8.57783427999994,11.6,5.86183779199998));
#205903=CARTESIAN_POINT('Ctrl Pts',(8.57863171399995,15.2,5.86251061999998));
#205904=CARTESIAN_POINT('Ctrl Pts',(8.57863171399995,11.6,5.86251061999998));
#205905=CARTESIAN_POINT('Ctrl Pts',(8.57943551499995,15.2,5.86319018599998));
#205906=CARTESIAN_POINT('Ctrl Pts',(8.57943551499995,11.6,5.86319018599998));
#205907=CARTESIAN_POINT('Ctrl Pts',(8.58024565199995,15.2,5.86387648699999));
#205908=CARTESIAN_POINT('Ctrl Pts',(8.58024565199995,11.6,5.86387648699999));
#205909=CARTESIAN_POINT('Ctrl Pts',(8.58106209399994,15.2,5.86456951899999));
#205910=CARTESIAN_POINT('Ctrl Pts',(8.58106209399994,11.6,5.86456951899999));
#205911=CARTESIAN_POINT('Ctrl Pts',(8.58188481199995,15.2,5.86526927999999));
#205912=CARTESIAN_POINT('Ctrl Pts',(8.58188481199995,11.6,5.86526927999999));
#205913=CARTESIAN_POINT('Ctrl Pts',(8.58271377499995,15.2,5.86597576499998));
#205914=CARTESIAN_POINT('Ctrl Pts',(8.58271377499995,11.6,5.86597576499998));
#205915=CARTESIAN_POINT('Ctrl Pts',(8.58354895399994,15.2,5.86668897399999));
#205916=CARTESIAN_POINT('Ctrl Pts',(8.58354895399994,11.6,5.86668897399999));
#205917=CARTESIAN_POINT('Ctrl Pts',(8.58439031899995,15.2,5.86740889999999));
#205918=CARTESIAN_POINT('Ctrl Pts',(8.58439031899995,11.6,5.86740889999999));
#205919=CARTESIAN_POINT('Ctrl Pts',(8.58523783999994,15.2,5.86813554199999));
#205920=CARTESIAN_POINT('Ctrl Pts',(8.58523783999994,11.6,5.86813554199999));
#205921=CARTESIAN_POINT('Ctrl Pts',(8.58609148699994,15.2,5.86886889799998));
#205922=CARTESIAN_POINT('Ctrl Pts',(8.58609148699994,11.6,5.86886889799998));
#205923=CARTESIAN_POINT('Ctrl Pts',(8.58695123199994,15.2,5.86960896199999));
#205924=CARTESIAN_POINT('Ctrl Pts',(8.58695123199994,11.6,5.86960896199999));
#205925=CARTESIAN_POINT('Ctrl Pts',(8.58781704399994,15.2,5.87035573299998));
#205926=CARTESIAN_POINT('Ctrl Pts',(8.58781704399994,11.6,5.87035573299998));
#205927=CARTESIAN_POINT('Ctrl Pts',(8.58868889599994,15.2,5.87110920699998));
#205928=CARTESIAN_POINT('Ctrl Pts',(8.58868889599994,11.6,5.87110920699998));
#205929=CARTESIAN_POINT('Ctrl Pts',(8.58956675699994,15.2,5.87186937999999));
#205930=CARTESIAN_POINT('Ctrl Pts',(8.58956675699994,11.6,5.87186937999999));
#205931=CARTESIAN_POINT('Ctrl Pts',(8.59045059999995,15.2,5.87263625099999));
#205932=CARTESIAN_POINT('Ctrl Pts',(8.59045059999995,11.6,5.87263625099999));
#205933=CARTESIAN_POINT('Ctrl Pts',(8.59134039399994,15.2,5.87340981499998));
#205934=CARTESIAN_POINT('Ctrl Pts',(8.59134039399994,11.6,5.87340981499998));
#205935=CARTESIAN_POINT('Ctrl Pts',(8.59223611299995,15.2,5.87419006999998));
#205936=CARTESIAN_POINT('Ctrl Pts',(8.59223611299995,11.6,5.87419006999998));
#205937=CARTESIAN_POINT('Ctrl Pts',(8.59313772599995,15.2,5.87497701299998));
#205938=CARTESIAN_POINT('Ctrl Pts',(8.59313772599995,11.6,5.87497701299998));
#205939=CARTESIAN_POINT('Ctrl Pts',(8.59404520799994,15.2,5.87577063899998));
#205940=CARTESIAN_POINT('Ctrl Pts',(8.59404520799994,11.6,5.87577063899998));
#205941=CARTESIAN_POINT('Ctrl Pts',(8.59495852899994,15.2,5.87657094699999));
#205942=CARTESIAN_POINT('Ctrl Pts',(8.59495852899994,11.6,5.87657094699999));
#205943=CARTESIAN_POINT('Ctrl Pts',(8.59587765999994,15.2,5.87737793199998));
#205944=CARTESIAN_POINT('Ctrl Pts',(8.59587765999994,11.6,5.87737793199998));
#205945=CARTESIAN_POINT('Ctrl Pts',(8.59680257499994,15.2,5.87819159299999));
#205946=CARTESIAN_POINT('Ctrl Pts',(8.59680257499994,11.6,5.87819159299999));
#205947=CARTESIAN_POINT('Ctrl Pts',(8.59773324399994,15.2,5.87901192399999));
#205948=CARTESIAN_POINT('Ctrl Pts',(8.59773324399994,11.6,5.87901192399999));
#205949=CARTESIAN_POINT('Ctrl Pts',(8.59866964199994,15.2,5.87983892599999));
#205950=CARTESIAN_POINT('Ctrl Pts',(8.59866964199994,11.6,5.87983892599999));
#205951=CARTESIAN_POINT('Ctrl Pts',(8.59961173899995,15.2,5.88067259099999));
#205952=CARTESIAN_POINT('Ctrl Pts',(8.59961173899995,11.6,5.88067259099999));
#205953=CARTESIAN_POINT('Ctrl Pts',(8.60055950899994,15.2,5.88151291899998));
#205954=CARTESIAN_POINT('Ctrl Pts',(8.60055950899994,11.6,5.88151291899998));
#205955=CARTESIAN_POINT('Ctrl Pts',(8.60151292399994,15.2,5.88235990599999));
#205956=CARTESIAN_POINT('Ctrl Pts',(8.60151292399994,11.6,5.88235990599999));
#205957=CARTESIAN_POINT('Ctrl Pts',(8.60247195899994,15.2,5.88321354999999));
#205958=CARTESIAN_POINT('Ctrl Pts',(8.60247195899994,11.6,5.88321354999999));
#205959=CARTESIAN_POINT('Ctrl Pts',(8.60343658399995,15.2,5.88407384599999));
#205960=CARTESIAN_POINT('Ctrl Pts',(8.60343658399995,11.6,5.88407384599999));
#205961=CARTESIAN_POINT('Ctrl Pts',(8.60440677399994,15.2,5.88494079199998));
#205962=CARTESIAN_POINT('Ctrl Pts',(8.60440677399994,11.6,5.88494079199998));
#205963=CARTESIAN_POINT('Ctrl Pts',(8.60538250099994,15.2,5.88581438399999));
#205964=CARTESIAN_POINT('Ctrl Pts',(8.60538250099994,11.6,5.88581438399999));
#205965=CARTESIAN_POINT('Ctrl Pts',(8.60636373899995,15.2,5.88669461999999));
#205966=CARTESIAN_POINT('Ctrl Pts',(8.60636373899995,11.6,5.88669461999999));
#205967=CARTESIAN_POINT('Ctrl Pts',(8.60735046099995,15.2,5.88758149599999));
#205968=CARTESIAN_POINT('Ctrl Pts',(8.60735046099995,11.6,5.88758149599999));
#205969=CARTESIAN_POINT('Ctrl Pts',(8.60834264199994,15.2,5.88847500899998));
#205970=CARTESIAN_POINT('Ctrl Pts',(8.60834264199994,11.6,5.88847500899998));
#205971=CARTESIAN_POINT('Ctrl Pts',(8.60934025399994,15.2,5.88937515599999));
#205972=CARTESIAN_POINT('Ctrl Pts',(8.60934025399994,11.6,5.88937515599999));
#205973=CARTESIAN_POINT('Ctrl Pts',(8.61034327099994,15.2,5.89028193299999));
#205974=CARTESIAN_POINT('Ctrl Pts',(8.61034327099994,11.6,5.89028193299999));
#205975=CARTESIAN_POINT('Ctrl Pts',(8.61135166799994,15.2,5.89119533799998));
#205976=CARTESIAN_POINT('Ctrl Pts',(8.61135166799994,11.6,5.89119533799998));
#205977=CARTESIAN_POINT('Ctrl Pts',(8.61236541699994,15.2,5.89211536899998));
#205978=CARTESIAN_POINT('Ctrl Pts',(8.61236541699994,11.6,5.89211536899998));
#205979=CARTESIAN_POINT('Ctrl Pts',(8.61338449399994,15.2,5.89304202099999));
#205980=CARTESIAN_POINT('Ctrl Pts',(8.61338449399994,11.6,5.89304202099999));
#205981=CARTESIAN_POINT('Ctrl Pts',(8.61440887299995,15.2,5.89397528999999));
#205982=CARTESIAN_POINT('Ctrl Pts',(8.61440887299995,11.6,5.89397528999999));
#205983=CARTESIAN_POINT('Ctrl Pts',(8.61543852799995,15.2,5.89491517399999));
#205984=CARTESIAN_POINT('Ctrl Pts',(8.61543852799995,11.6,5.89491517399999));
#205985=CARTESIAN_POINT('Ctrl Pts',(8.61647343299994,15.2,5.89586167199998));
#205986=CARTESIAN_POINT('Ctrl Pts',(8.61647343299994,11.6,5.89586167199998));
#205987=CARTESIAN_POINT('Ctrl Pts',(8.61751356299994,15.2,5.89681477699998));
#205988=CARTESIAN_POINT('Ctrl Pts',(8.61751356299994,11.6,5.89681477699998));
#205989=CARTESIAN_POINT('Ctrl Pts',(8.61855889399994,15.2,5.89777448799998));
#205990=CARTESIAN_POINT('Ctrl Pts',(8.61855889399994,11.6,5.89777448799998));
#205991=CARTESIAN_POINT('Ctrl Pts',(8.61960939799994,15.2,5.89874080299998));
#205992=CARTESIAN_POINT('Ctrl Pts',(8.61960939799994,11.6,5.89874080299998));
#205993=CARTESIAN_POINT('Ctrl Pts',(8.62066505299994,15.2,5.89971371599999));
#205994=CARTESIAN_POINT('Ctrl Pts',(8.62066505299994,11.6,5.89971371599999));
#205995=CARTESIAN_POINT('Ctrl Pts',(8.62172582999994,15.2,5.90069322599999));
#205996=CARTESIAN_POINT('Ctrl Pts',(8.62172582999994,11.6,5.90069322599999));
#205997=CARTESIAN_POINT('Ctrl Pts',(8.62279170899994,15.2,5.90167932799999));
#205998=CARTESIAN_POINT('Ctrl Pts',(8.62279170899994,11.6,5.90167932799999));
#205999=CARTESIAN_POINT('Ctrl Pts',(8.62386266099995,15.2,5.90267202099999));
#206000=CARTESIAN_POINT('Ctrl Pts',(8.62386266099995,11.6,5.90267202099999));
#206001=CARTESIAN_POINT('Ctrl Pts',(8.62493866399995,15.2,5.90367129999999));
#206002=CARTESIAN_POINT('Ctrl Pts',(8.62493866399995,11.6,5.90367129999999));
#206003=CARTESIAN_POINT('Ctrl Pts',(8.62601969299994,15.2,5.90467716399999));
#206004=CARTESIAN_POINT('Ctrl Pts',(8.62601969299994,11.6,5.90467716399999));
#206005=CARTESIAN_POINT('Ctrl Pts',(8.62710572199994,15.2,5.90568960799998));
#206006=CARTESIAN_POINT('Ctrl Pts',(8.62710572199994,11.6,5.90568960799998));
#206007=CARTESIAN_POINT('Ctrl Pts',(8.62819672799995,15.2,5.90670862899999));
#206008=CARTESIAN_POINT('Ctrl Pts',(8.62819672799995,11.6,5.90670862899999));
#206009=CARTESIAN_POINT('Ctrl Pts',(8.62929268599994,15.2,5.90773422499999));
#206010=CARTESIAN_POINT('Ctrl Pts',(8.62929268599994,11.6,5.90773422499999));
#206011=CARTESIAN_POINT('Ctrl Pts',(8.63039357199994,15.2,5.90876639099999));
#206012=CARTESIAN_POINT('Ctrl Pts',(8.63039357199994,11.6,5.90876639099999));
#206013=CARTESIAN_POINT('Ctrl Pts',(8.63149936299994,15.2,5.90980512599998));
#206014=CARTESIAN_POINT('Ctrl Pts',(8.63149936299994,11.6,5.90980512599998));
#206015=CARTESIAN_POINT('Ctrl Pts',(8.63261003299994,15.2,5.91085042599998));
#206016=CARTESIAN_POINT('Ctrl Pts',(8.63261003299994,11.6,5.91085042599998));
#206017=CARTESIAN_POINT('Ctrl Pts',(8.63372555899995,15.2,5.91190228799999));
#206018=CARTESIAN_POINT('Ctrl Pts',(8.63372555899995,11.6,5.91190228799999));
#206019=CARTESIAN_POINT('Ctrl Pts',(8.63484591899994,15.2,5.91296070799999));
#206020=CARTESIAN_POINT('Ctrl Pts',(8.63484591899994,11.6,5.91296070799999));
#206021=CARTESIAN_POINT('Ctrl Pts',(8.63597108699994,15.2,5.91402568299999));
#206022=CARTESIAN_POINT('Ctrl Pts',(8.63597108699994,11.6,5.91402568299999));
#206023=CARTESIAN_POINT('Ctrl Pts',(8.63710103999994,15.2,5.91509721099998));
#206024=CARTESIAN_POINT('Ctrl Pts',(8.63710103999994,11.6,5.91509721099998));
#206025=CARTESIAN_POINT('Ctrl Pts',(8.63823575599995,15.2,5.91617528699998));
#206026=CARTESIAN_POINT('Ctrl Pts',(8.63823575599995,11.6,5.91617528699998));
#206027=CARTESIAN_POINT('Ctrl Pts',(8.63937520799994,15.2,5.91725990999999));
#206028=CARTESIAN_POINT('Ctrl Pts',(8.63937520799994,11.6,5.91725990999999));
#206029=CARTESIAN_POINT('Ctrl Pts',(8.64051937599994,15.2,5.91835107599999));
#206030=CARTESIAN_POINT('Ctrl Pts',(8.64051937599994,11.6,5.91835107599999));
#206031=CARTESIAN_POINT('Ctrl Pts',(8.64166823699994,15.2,5.91944878099999));
#206032=CARTESIAN_POINT('Ctrl Pts',(8.64166823699994,11.6,5.91944878099999));
#206033=CARTESIAN_POINT('Ctrl Pts',(8.64282176499995,15.2,5.92055302299999));
#206034=CARTESIAN_POINT('Ctrl Pts',(8.64282176499995,11.6,5.92055302299999));
#206035=CARTESIAN_POINT('Ctrl Pts',(8.64397993899994,15.2,5.92166379699999));
#206036=CARTESIAN_POINT('Ctrl Pts',(8.64397993899994,11.6,5.92166379699999));
#206037=CARTESIAN_POINT('Ctrl Pts',(8.64514273599994,15.2,5.92278110299999));
#206038=CARTESIAN_POINT('Ctrl Pts',(8.64514273599994,11.6,5.92278110299999));
#206039=CARTESIAN_POINT('Ctrl Pts',(8.64631013299994,15.2,5.92390493599999));
#206040=CARTESIAN_POINT('Ctrl Pts',(8.64631013299994,11.6,5.92390493599999));
#206041=CARTESIAN_POINT('Ctrl Pts',(8.64748210699995,15.2,5.92503529199998));
#206042=CARTESIAN_POINT('Ctrl Pts',(8.64748210699995,11.6,5.92503529199998));
#206043=CARTESIAN_POINT('Ctrl Pts',(8.64865863499995,15.2,5.92617216999999));
#206044=CARTESIAN_POINT('Ctrl Pts',(8.64865863499995,11.6,5.92617216999999));
#206045=CARTESIAN_POINT('Ctrl Pts',(8.64983969599994,15.2,5.92731556399999));
#206046=CARTESIAN_POINT('Ctrl Pts',(8.64983969599994,11.6,5.92731556399999));
#206047=CARTESIAN_POINT('Ctrl Pts',(8.65102526499994,15.2,5.92846547399999));
#206048=CARTESIAN_POINT('Ctrl Pts',(8.65102526499994,11.6,5.92846547399999));
#206049=CARTESIAN_POINT('Ctrl Pts',(8.65221532199994,15.2,5.92962189399999));
#206050=CARTESIAN_POINT('Ctrl Pts',(8.65221532199994,11.6,5.92962189399999));
#206051=CARTESIAN_POINT('Ctrl Pts',(8.65340984299995,15.2,5.93078482399999));
#206052=CARTESIAN_POINT('Ctrl Pts',(8.65340984299995,11.6,5.93078482399999));
#206053=CARTESIAN_POINT('Ctrl Pts',(8.65460880699995,15.2,5.93195425699999));
#206054=CARTESIAN_POINT('Ctrl Pts',(8.65460880699995,11.6,5.93195425699999));
#206055=CARTESIAN_POINT('Ctrl Pts',(8.65581219099994,15.2,5.93313019299998));
#206056=CARTESIAN_POINT('Ctrl Pts',(8.65581219099994,11.6,5.93313019299998));
#206057=CARTESIAN_POINT('Ctrl Pts',(8.65701997299994,15.2,5.93431262699998));
#206058=CARTESIAN_POINT('Ctrl Pts',(8.65701997299994,11.6,5.93431262699998));
#206059=CARTESIAN_POINT('Ctrl Pts',(8.65823213199995,15.2,5.93550155699998));
#206060=CARTESIAN_POINT('Ctrl Pts',(8.65823213199995,11.6,5.93550155699998));
#206061=CARTESIAN_POINT('Ctrl Pts',(8.65944864499994,15.2,5.93669697899998));
#206062=CARTESIAN_POINT('Ctrl Pts',(8.65944864499994,11.6,5.93669697899998));
#206063=CARTESIAN_POINT('Ctrl Pts',(8.66066948999995,15.2,5.93789889099998));
#206064=CARTESIAN_POINT('Ctrl Pts',(8.66066948999995,11.6,5.93789889099998));
#206065=CARTESIAN_POINT('Ctrl Pts',(8.66189464699995,15.2,5.93910728899999));
#206066=CARTESIAN_POINT('Ctrl Pts',(8.66189464699995,11.6,5.93910728899999));
#206067=CARTESIAN_POINT('Ctrl Pts',(8.66312409299994,15.2,5.94032216899999));
#206068=CARTESIAN_POINT('Ctrl Pts',(8.66312409299994,11.6,5.94032216899999));
#206069=CARTESIAN_POINT('Ctrl Pts',(8.66435780599994,15.2,5.94154352899999));
#206070=CARTESIAN_POINT('Ctrl Pts',(8.66435780599994,11.6,5.94154352899999));
#206071=CARTESIAN_POINT('Ctrl Pts',(8.66559576699995,15.2,5.94277136599998));
#206072=CARTESIAN_POINT('Ctrl Pts',(8.66559576699995,11.6,5.94277136599998));
#206073=CARTESIAN_POINT('Ctrl Pts',(8.66683795199994,15.2,5.94400567599998));
#206074=CARTESIAN_POINT('Ctrl Pts',(8.66683795199994,11.6,5.94400567599998));
#206075=CARTESIAN_POINT('Ctrl Pts',(8.66808433999994,15.2,5.94524645699998));
#206076=CARTESIAN_POINT('Ctrl Pts',(8.66808433999994,11.6,5.94524645699998));
#206077=CARTESIAN_POINT('Ctrl Pts',(8.66933491099994,15.2,5.94649370499998));
#206078=CARTESIAN_POINT('Ctrl Pts',(8.66933491099994,11.6,5.94649370499998));
#206079=CARTESIAN_POINT('Ctrl Pts',(8.67058964199994,15.2,5.94774741499998));
#206080=CARTESIAN_POINT('Ctrl Pts',(8.67058964199994,11.6,5.94774741499998));
#206081=CARTESIAN_POINT('Ctrl Pts',(8.67184851399994,15.2,5.94900758799999));
#206082=CARTESIAN_POINT('Ctrl Pts',(8.67184851399994,11.6,5.94900758799999));
#206083=CARTESIAN_POINT('Ctrl Pts',(8.67311150499994,15.2,5.95027421799998));
#206084=CARTESIAN_POINT('Ctrl Pts',(8.67311150499994,11.6,5.95027421799998));
#206085=CARTESIAN_POINT('Ctrl Pts',(8.67437859499994,15.2,5.95154730199998));
#206086=CARTESIAN_POINT('Ctrl Pts',(8.67437859499994,11.6,5.95154730199998));
#206087=CARTESIAN_POINT('Ctrl Pts',(8.67564976199995,15.2,5.95282683799999));
#206088=CARTESIAN_POINT('Ctrl Pts',(8.67564976199995,11.6,5.95282683799999));
#206089=CARTESIAN_POINT('Ctrl Pts',(8.67692498499994,15.2,5.95411282099998));
#206090=CARTESIAN_POINT('Ctrl Pts',(8.67692498499994,11.6,5.95411282099998));
#206091=CARTESIAN_POINT('Ctrl Pts',(8.67820424499994,15.2,5.95540524999999));
#206092=CARTESIAN_POINT('Ctrl Pts',(8.67820424499994,11.6,5.95540524999999));
#206093=CARTESIAN_POINT('Ctrl Pts',(8.67948751899995,15.2,5.95670411999999));
#206094=CARTESIAN_POINT('Ctrl Pts',(8.67948751899995,11.6,5.95670411999999));
#206095=CARTESIAN_POINT('Ctrl Pts',(8.68077478899994,15.2,5.95800942899999));
#206096=CARTESIAN_POINT('Ctrl Pts',(8.68077478899994,11.6,5.95800942899999));
#206097=CARTESIAN_POINT('Ctrl Pts',(8.68206603399994,15.2,5.95932117299999));
#206098=CARTESIAN_POINT('Ctrl Pts',(8.68206603399994,11.6,5.95932117299999));
#206099=CARTESIAN_POINT('Ctrl Pts',(8.68336123199994,15.2,5.96063934899998));
#206100=CARTESIAN_POINT('Ctrl Pts',(8.68336123199994,11.6,5.96063934899998));
#206101=CARTESIAN_POINT('Ctrl Pts',(8.68466036399994,15.2,5.96196395499998));
#206102=CARTESIAN_POINT('Ctrl Pts',(8.68466036399994,11.6,5.96196395499998));
#206103=CARTESIAN_POINT('Ctrl Pts',(8.68596340899994,15.2,5.96329498599999));
#206104=CARTESIAN_POINT('Ctrl Pts',(8.68596340899994,11.6,5.96329498599999));
#206105=CARTESIAN_POINT('Ctrl Pts',(8.68727034799995,15.2,5.96463243999998));
#206106=CARTESIAN_POINT('Ctrl Pts',(8.68727034799995,11.6,5.96463243999998));
#206107=CARTESIAN_POINT('Ctrl Pts',(8.68858115999994,15.2,5.96597631299999));
#206108=CARTESIAN_POINT('Ctrl Pts',(8.68858115999994,11.6,5.96597631299999));
#206109=CARTESIAN_POINT('Ctrl Pts',(8.68989582599994,15.2,5.96732660299998));
#206110=CARTESIAN_POINT('Ctrl Pts',(8.68989582599994,11.6,5.96732660299998));
#206111=CARTESIAN_POINT('Ctrl Pts',(8.69121432399995,15.2,5.96868330599998));
#206112=CARTESIAN_POINT('Ctrl Pts',(8.69121432399995,11.6,5.96868330599998));
#206113=CARTESIAN_POINT('Ctrl Pts',(8.69253663599994,15.2,5.97004641899999));
#206114=CARTESIAN_POINT('Ctrl Pts',(8.69253663599994,11.6,5.97004641899999));
#206115=CARTESIAN_POINT('Ctrl Pts',(8.69386274199995,15.2,5.97141593799999));
#206116=CARTESIAN_POINT('Ctrl Pts',(8.69386274199995,11.6,5.97141593799999));
#206117=CARTESIAN_POINT('Ctrl Pts',(8.69519262199994,15.2,5.97279186099998));
#206118=CARTESIAN_POINT('Ctrl Pts',(8.69519262199994,11.6,5.97279186099998));
#206119=CARTESIAN_POINT('Ctrl Pts',(8.69652625699995,15.2,5.97417418499998));
#206120=CARTESIAN_POINT('Ctrl Pts',(8.69652625699995,11.6,5.97417418499998));
#206121=CARTESIAN_POINT('Ctrl Pts',(8.69786362599994,15.2,5.97556290499998));
#206122=CARTESIAN_POINT('Ctrl Pts',(8.69786362599994,11.6,5.97556290499998));
#206123=CARTESIAN_POINT('Ctrl Pts',(8.69920470899994,15.2,5.97695802099998));
#206124=CARTESIAN_POINT('Ctrl Pts',(8.69920470899994,11.6,5.97695802099998));
#206125=CARTESIAN_POINT('Ctrl Pts',(8.70054948899995,15.2,5.97835952599999));
#206126=CARTESIAN_POINT('Ctrl Pts',(8.70054948899995,11.6,5.97835952599999));
#206127=CARTESIAN_POINT('Ctrl Pts',(8.70189794499994,15.2,5.97976741899998));
#206128=CARTESIAN_POINT('Ctrl Pts',(8.70189794499994,11.6,5.97976741899998));
#206129=CARTESIAN_POINT('Ctrl Pts',(8.70325005799994,15.2,5.98118169699998));
#206130=CARTESIAN_POINT('Ctrl Pts',(8.70325005799994,11.6,5.98118169699998));
#206131=CARTESIAN_POINT('Ctrl Pts',(8.70460580899995,15.2,5.98260235599999));
#206132=CARTESIAN_POINT('Ctrl Pts',(8.70460580899995,11.6,5.98260235599999));
#206133=CARTESIAN_POINT('Ctrl Pts',(8.70596517899994,15.2,5.98402939299999));
#206134=CARTESIAN_POINT('Ctrl Pts',(8.70596517899994,11.6,5.98402939299999));
#206135=CARTESIAN_POINT('Ctrl Pts',(8.70732814799995,15.2,5.98546280499999));
#206136=CARTESIAN_POINT('Ctrl Pts',(8.70732814799995,11.6,5.98546280499999));
#206137=CARTESIAN_POINT('Ctrl Pts',(8.70869469799995,15.2,5.98690258799999));
#206138=CARTESIAN_POINT('Ctrl Pts',(8.70869469799995,11.6,5.98690258799999));
#206139=CARTESIAN_POINT('Ctrl Pts',(8.71006480999995,15.2,5.98834873999999));
#206140=CARTESIAN_POINT('Ctrl Pts',(8.71006480999995,11.6,5.98834873999999));
#206141=CARTESIAN_POINT('Ctrl Pts',(8.71143846399994,15.2,5.98980125699998));
#206142=CARTESIAN_POINT('Ctrl Pts',(8.71143846399994,11.6,5.98980125699998));
#206143=CARTESIAN_POINT('Ctrl Pts',(8.71281564199995,15.2,5.99126013699999));
#206144=CARTESIAN_POINT('Ctrl Pts',(8.71281564199995,11.6,5.99126013699999));
#206145=CARTESIAN_POINT('Ctrl Pts',(8.71419632499994,15.2,5.99272537499999));
#206146=CARTESIAN_POINT('Ctrl Pts',(8.71419632499994,11.6,5.99272537499999));
#206147=CARTESIAN_POINT('Ctrl Pts',(8.71558049399994,15.2,5.99419696999998));
#206148=CARTESIAN_POINT('Ctrl Pts',(8.71558049399994,11.6,5.99419696999998));
#206149=CARTESIAN_POINT('Ctrl Pts',(8.71696813099994,15.2,5.99567491599998));
#206150=CARTESIAN_POINT('Ctrl Pts',(8.71696813099994,11.6,5.99567491599998));
#206151=CARTESIAN_POINT('Ctrl Pts',(8.71835921699994,15.2,5.99715921099998));
#206152=CARTESIAN_POINT('Ctrl Pts',(8.71835921699994,11.6,5.99715921099998));
#206153=CARTESIAN_POINT('Ctrl Pts',(8.71975373299994,15.2,5.99864985399999));
#206154=CARTESIAN_POINT('Ctrl Pts',(8.71975373299994,11.6,5.99864985399999));
#206155=CARTESIAN_POINT('Ctrl Pts',(8.72115166199994,15.2,6.00014683799999));
#206156=CARTESIAN_POINT('Ctrl Pts',(8.72115166199994,11.6,6.00014683799999));
#206157=CARTESIAN_POINT('Ctrl Pts',(8.72255298499995,15.2,6.00165016199998));
#206158=CARTESIAN_POINT('Ctrl Pts',(8.72255298499995,11.6,6.00165016199998));
#206159=CARTESIAN_POINT('Ctrl Pts',(8.72395768199994,15.2,6.00315982299998));
#206160=CARTESIAN_POINT('Ctrl Pts',(8.72395768199994,11.6,6.00315982299998));
#206161=CARTESIAN_POINT('Ctrl Pts',(8.72536573799995,15.2,6.00467581699998));
#206162=CARTESIAN_POINT('Ctrl Pts',(8.72536573799995,11.6,6.00467581699998));
#206163=CARTESIAN_POINT('Ctrl Pts',(8.72677713199994,15.2,6.00619814099999));
#206164=CARTESIAN_POINT('Ctrl Pts',(8.72677713199994,11.6,6.00619814099999));
#206165=CARTESIAN_POINT('Ctrl Pts',(8.72819184599994,15.2,6.00772679099999));
#206166=CARTESIAN_POINT('Ctrl Pts',(8.72819184599994,11.6,6.00772679099999));
#206167=CARTESIAN_POINT('Ctrl Pts',(8.72960986399994,15.2,6.00926176599998));
#206168=CARTESIAN_POINT('Ctrl Pts',(8.72960986399994,11.6,6.00926176599998));
#206169=CARTESIAN_POINT('Ctrl Pts',(8.73103116499994,15.2,6.01080305999999));
#206170=CARTESIAN_POINT('Ctrl Pts',(8.73103116499994,11.6,6.01080305999999));
#206171=CARTESIAN_POINT('Ctrl Pts',(8.73245573399995,15.2,6.01235067199998));
#206172=CARTESIAN_POINT('Ctrl Pts',(8.73245573399995,11.6,6.01235067199998));
#206173=CARTESIAN_POINT('Ctrl Pts',(8.73388355099994,15.2,6.01390459899999));
#206174=CARTESIAN_POINT('Ctrl Pts',(8.73388355099994,11.6,6.01390459899999));
#206175=CARTESIAN_POINT('Ctrl Pts',(8.73531459999995,15.2,6.01546483499998));
#206176=CARTESIAN_POINT('Ctrl Pts',(8.73531459999995,11.6,6.01546483499998));
#206177=CARTESIAN_POINT('Ctrl Pts',(8.73674886199994,15.2,6.01703137999999));
#206178=CARTESIAN_POINT('Ctrl Pts',(8.73674886199994,11.6,6.01703137999999));
#206179=CARTESIAN_POINT('Ctrl Pts',(8.73818631899994,15.2,6.01860422699998));
#206180=CARTESIAN_POINT('Ctrl Pts',(8.73818631899994,11.6,6.01860422699998));
#206181=CARTESIAN_POINT('Ctrl Pts',(8.73962695399995,15.2,6.02018337699998));
#206182=CARTESIAN_POINT('Ctrl Pts',(8.73962695399995,11.6,6.02018337699998));
#206183=CARTESIAN_POINT('Ctrl Pts',(8.74107074799995,15.2,6.02176882399998));
#206184=CARTESIAN_POINT('Ctrl Pts',(8.74107074799995,11.6,6.02176882399998));
#206185=CARTESIAN_POINT('Ctrl Pts',(8.74251768599994,15.2,6.02336056599999));
#206186=CARTESIAN_POINT('Ctrl Pts',(8.74251768599994,11.6,6.02336056599999));
#206187=CARTESIAN_POINT('Ctrl Pts',(8.74396774799994,15.2,6.02495859899999));
#206188=CARTESIAN_POINT('Ctrl Pts',(8.74396774799994,11.6,6.02495859899999));
#206189=CARTESIAN_POINT('Ctrl Pts',(8.74542091899994,15.2,6.02656292099999));
#206190=CARTESIAN_POINT('Ctrl Pts',(8.74542091899994,11.6,6.02656292099999));
#206191=CARTESIAN_POINT('Ctrl Pts',(8.74687717899995,15.2,6.02817352699999));
#206192=CARTESIAN_POINT('Ctrl Pts',(8.74687717899995,11.6,6.02817352699999));
#206193=CARTESIAN_POINT('Ctrl Pts',(8.74833651199994,15.2,6.02979041499999));
#206194=CARTESIAN_POINT('Ctrl Pts',(8.74833651199994,11.6,6.02979041499999));
#206195=CARTESIAN_POINT('Ctrl Pts',(8.74979890299995,15.2,6.03141358199998));
#206196=CARTESIAN_POINT('Ctrl Pts',(8.74979890299995,11.6,6.03141358199998));
#206197=CARTESIAN_POINT('Ctrl Pts',(8.75126432999994,15.2,6.03304302299998));
#206198=CARTESIAN_POINT('Ctrl Pts',(8.75126432999994,11.6,6.03304302299998));
#206199=CARTESIAN_POINT('Ctrl Pts',(8.75273277899994,15.2,6.03467873699999));
#206200=CARTESIAN_POINT('Ctrl Pts',(8.75273277899994,11.6,6.03467873699999));
#206201=CARTESIAN_POINT('Ctrl Pts',(8.75420423299994,15.2,6.03632071999999));
#206202=CARTESIAN_POINT('Ctrl Pts',(8.75420423299994,11.6,6.03632071999999));
#206203=CARTESIAN_POINT('Ctrl Pts',(8.75567867299995,15.2,6.03796896799999));
#206204=CARTESIAN_POINT('Ctrl Pts',(8.75567867299995,11.6,6.03796896799999));
#206205=CARTESIAN_POINT('Ctrl Pts',(8.75715608399994,15.2,6.03962347899999));
#206206=CARTESIAN_POINT('Ctrl Pts',(8.75715608399994,11.6,6.03962347899999));
#206207=CARTESIAN_POINT('Ctrl Pts',(8.75863644699994,15.2,6.04128424799999));
#206208=CARTESIAN_POINT('Ctrl Pts',(8.75863644699994,11.6,6.04128424799999));
#206209=CARTESIAN_POINT('Ctrl Pts',(8.76011974799994,15.2,6.04295127299999));
#206210=CARTESIAN_POINT('Ctrl Pts',(8.76011974799994,11.6,6.04295127299999));
#206211=CARTESIAN_POINT('Ctrl Pts',(8.76160596799994,15.2,6.04462455099998));
#206212=CARTESIAN_POINT('Ctrl Pts',(8.76160596799994,11.6,6.04462455099998));
#206213=CARTESIAN_POINT('Ctrl Pts',(8.76309508999995,15.2,6.04630407799998));
#206214=CARTESIAN_POINT('Ctrl Pts',(8.76309508999995,11.6,6.04630407799998));
#206215=CARTESIAN_POINT('Ctrl Pts',(8.76458709899994,15.2,6.04798985099999));
#206216=CARTESIAN_POINT('Ctrl Pts',(8.76458709899994,11.6,6.04798985099999));
#206217=CARTESIAN_POINT('Ctrl Pts',(8.76608197799994,15.2,6.04968186699999));
#206218=CARTESIAN_POINT('Ctrl Pts',(8.76608197799994,11.6,6.04968186699999));
#206219=CARTESIAN_POINT('Ctrl Pts',(8.76757970799994,15.2,6.05138012299999));
#206220=CARTESIAN_POINT('Ctrl Pts',(8.76757970799994,11.6,6.05138012299999));
#206221=CARTESIAN_POINT('Ctrl Pts',(8.76908027599994,15.2,6.05308461599999));
#206222=CARTESIAN_POINT('Ctrl Pts',(8.76908027599994,11.6,6.05308461599999));
#206223=CARTESIAN_POINT('Ctrl Pts',(8.77058366299994,15.2,6.05479533999999));
#206224=CARTESIAN_POINT('Ctrl Pts',(8.77058366299994,11.6,6.05479533999999));
#206225=CARTESIAN_POINT('Ctrl Pts',(8.77208985199994,15.2,6.05651229599999));
#206226=CARTESIAN_POINT('Ctrl Pts',(8.77208985199994,11.6,6.05651229599999));
#206227=CARTESIAN_POINT('Ctrl Pts',(8.77359882999994,15.2,6.05823547699998));
#206228=CARTESIAN_POINT('Ctrl Pts',(8.77359882999994,11.6,6.05823547699998));
#206229=CARTESIAN_POINT('Ctrl Pts',(8.77511057699994,15.2,6.05996488199998));
#206230=CARTESIAN_POINT('Ctrl Pts',(8.77511057699994,11.6,6.05996488199998));
#206231=CARTESIAN_POINT('Ctrl Pts',(8.77662507799995,15.2,6.06170050699999));
#206232=CARTESIAN_POINT('Ctrl Pts',(8.77662507799995,11.6,6.06170050699999));
#206233=CARTESIAN_POINT('Ctrl Pts',(8.77814231699995,15.2,6.06344234899999));
#206234=CARTESIAN_POINT('Ctrl Pts',(8.77814231699995,11.6,6.06344234899999));
#206235=CARTESIAN_POINT('Ctrl Pts',(8.77966227899995,15.2,6.06519040399998));
#206236=CARTESIAN_POINT('Ctrl Pts',(8.77966227899995,11.6,6.06519040399998));
#206237=CARTESIAN_POINT('Ctrl Pts',(8.78118494499994,15.2,6.06694466999999));
#206238=CARTESIAN_POINT('Ctrl Pts',(8.78118494499994,11.6,6.06694466999999));
#206239=CARTESIAN_POINT('Ctrl Pts',(8.78271030099994,15.2,6.06870514299998));
#206240=CARTESIAN_POINT('Ctrl Pts',(8.78271030099994,11.6,6.06870514299998));
#206241=CARTESIAN_POINT('Ctrl Pts',(8.78423832999994,15.2,6.07047181899999));
#206242=CARTESIAN_POINT('Ctrl Pts',(8.78423832999994,11.6,6.07047181899999));
#206243=CARTESIAN_POINT('Ctrl Pts',(8.78576901699994,15.2,6.07224469699998));
#206244=CARTESIAN_POINT('Ctrl Pts',(8.78576901699994,11.6,6.07224469699998));
#206245=CARTESIAN_POINT('Ctrl Pts',(8.78730234599994,15.2,6.07402377099999));
#206246=CARTESIAN_POINT('Ctrl Pts',(8.78730234599994,11.6,6.07402377099999));
#206247=CARTESIAN_POINT('Ctrl Pts',(8.78883829999995,15.2,6.07580903899999));
#206248=CARTESIAN_POINT('Ctrl Pts',(8.78883829999995,11.6,6.07580903899999));
#206249=CARTESIAN_POINT('Ctrl Pts',(8.79037686299995,15.2,6.07760049799998));
#206250=CARTESIAN_POINT('Ctrl Pts',(8.79037686299995,11.6,6.07760049799998));
#206251=CARTESIAN_POINT('Ctrl Pts',(8.79191802099994,15.2,6.07939814499999));
#206252=CARTESIAN_POINT('Ctrl Pts',(8.79191802099994,11.6,6.07939814499999));
#206253=CARTESIAN_POINT('Ctrl Pts',(8.79346175599995,15.2,6.08120197499999));
#206254=CARTESIAN_POINT('Ctrl Pts',(8.79346175599995,11.6,6.08120197499999));
#206255=CARTESIAN_POINT('Ctrl Pts',(8.79500805399994,15.2,6.08301198699999));
#206256=CARTESIAN_POINT('Ctrl Pts',(8.79500805399994,11.6,6.08301198699999));
#206257=CARTESIAN_POINT('Ctrl Pts',(8.79655689899994,15.2,6.08482817699999));
#206258=CARTESIAN_POINT('Ctrl Pts',(8.79655689899994,11.6,6.08482817699999));
#206259=CARTESIAN_POINT('Ctrl Pts',(8.79810827499995,15.2,6.08665054099998));
#206260=CARTESIAN_POINT('Ctrl Pts',(8.79810827499995,11.6,6.08665054099998));
#206261=CARTESIAN_POINT('Ctrl Pts',(8.79966216599994,15.2,6.08847907499998));
#206262=CARTESIAN_POINT('Ctrl Pts',(8.79966216599994,11.6,6.08847907499998));
#206263=CARTESIAN_POINT('Ctrl Pts',(8.80121855799995,15.2,6.09031377899999));
#206264=CARTESIAN_POINT('Ctrl Pts',(8.80121855799995,11.6,6.09031377899999));
#206265=CARTESIAN_POINT('Ctrl Pts',(8.80277743299994,15.2,6.09215464499999));
#206266=CARTESIAN_POINT('Ctrl Pts',(8.80277743299994,11.6,6.09215464499999));
#206267=CARTESIAN_POINT('Ctrl Pts',(8.80433877799994,15.2,6.09400167399999));
#206268=CARTESIAN_POINT('Ctrl Pts',(8.80433877799994,11.6,6.09400167399999));
#206269=CARTESIAN_POINT('Ctrl Pts',(8.80590257699994,15.2,6.09585486099999));
#206270=CARTESIAN_POINT('Ctrl Pts',(8.80590257699994,11.6,6.09585486099999));
#206271=CARTESIAN_POINT('Ctrl Pts',(8.80746881299994,15.2,6.09771420199999));
#206272=CARTESIAN_POINT('Ctrl Pts',(8.80746881299994,11.6,6.09771420199999));
#206273=CARTESIAN_POINT('Ctrl Pts',(8.80903747399995,15.2,6.09957969499998));
#206274=CARTESIAN_POINT('Ctrl Pts',(8.80903747399995,11.6,6.09957969499998));
#206275=CARTESIAN_POINT('Ctrl Pts',(8.81060854099994,15.2,6.10145133499999));
#206276=CARTESIAN_POINT('Ctrl Pts',(8.81060854099994,11.6,6.10145133499999));
#206277=CARTESIAN_POINT('Ctrl Pts',(8.81218200199994,15.2,6.10332912099998));
#206278=CARTESIAN_POINT('Ctrl Pts',(8.81218200199994,11.6,6.10332912099998));
#206279=CARTESIAN_POINT('Ctrl Pts',(8.81375783899994,15.2,6.10521304799998));
#206280=CARTESIAN_POINT('Ctrl Pts',(8.81375783899994,11.6,6.10521304799998));
#206281=CARTESIAN_POINT('Ctrl Pts',(8.81533603999994,15.2,6.10710311399998));
#206282=CARTESIAN_POINT('Ctrl Pts',(8.81533603999994,11.6,6.10710311399998));
#206283=CARTESIAN_POINT('Ctrl Pts',(8.81691658799994,15.2,6.10899931499999));
#206284=CARTESIAN_POINT('Ctrl Pts',(8.81691658799994,11.6,6.10899931499999));
#206285=CARTESIAN_POINT('Ctrl Pts',(8.81849946799995,15.2,6.11090164599998));
#206286=CARTESIAN_POINT('Ctrl Pts',(8.81849946799995,11.6,6.11090164599998));
#206287=CARTESIAN_POINT('Ctrl Pts',(8.82008466499994,15.2,6.11281010699999));
#206288=CARTESIAN_POINT('Ctrl Pts',(8.82008466499994,11.6,6.11281010699999));
#206289=CARTESIAN_POINT('Ctrl Pts',(8.82167216399995,15.2,6.11472469299999));
#206290=CARTESIAN_POINT('Ctrl Pts',(8.82167216399995,11.6,6.11472469299999));
#206291=CARTESIAN_POINT('Ctrl Pts',(8.82326195199994,15.2,6.11664540099999));
#206292=CARTESIAN_POINT('Ctrl Pts',(8.82326195199994,11.6,6.11664540099999));
#206293=CARTESIAN_POINT('Ctrl Pts',(8.82485401099995,15.2,6.11857222699999));
#206294=CARTESIAN_POINT('Ctrl Pts',(8.82485401099995,11.6,6.11857222699999));
#206295=CARTESIAN_POINT('Ctrl Pts',(8.82644832899994,15.2,6.12050516799999));
#206296=CARTESIAN_POINT('Ctrl Pts',(8.82644832899994,11.6,6.12050516799999));
#206297=CARTESIAN_POINT('Ctrl Pts',(8.82804488899994,15.2,6.12244422099998));
#206298=CARTESIAN_POINT('Ctrl Pts',(8.82804488899994,11.6,6.12244422099998));
#206299=CARTESIAN_POINT('Ctrl Pts',(8.82964367799994,15.2,6.12438938399999));
#206300=CARTESIAN_POINT('Ctrl Pts',(8.82964367799994,11.6,6.12438938399999));
#206301=CARTESIAN_POINT('Ctrl Pts',(8.83124467999994,15.2,6.12634065099999));
#206302=CARTESIAN_POINT('Ctrl Pts',(8.83124467999994,11.6,6.12634065099999));
#206303=CARTESIAN_POINT('Ctrl Pts',(8.83284788199994,15.2,6.12829801999998));
#206304=CARTESIAN_POINT('Ctrl Pts',(8.83284788199994,11.6,6.12829801999998));
#206305=CARTESIAN_POINT('Ctrl Pts',(8.83445326699994,15.2,6.13026148799998));
#206306=CARTESIAN_POINT('Ctrl Pts',(8.83445326699994,11.6,6.13026148799998));
#206307=CARTESIAN_POINT('Ctrl Pts',(8.83606082299995,15.2,6.13223105099999));
#206308=CARTESIAN_POINT('Ctrl Pts',(8.83606082299995,11.6,6.13223105099999));
#206309=CARTESIAN_POINT('Ctrl Pts',(8.83767053399995,15.2,6.13420670699998));
#206310=CARTESIAN_POINT('Ctrl Pts',(8.83767053399995,11.6,6.13420670699998));
#206311=CARTESIAN_POINT('Ctrl Pts',(8.83928238599994,15.2,6.13618845099998));
#206312=CARTESIAN_POINT('Ctrl Pts',(8.83928238599994,11.6,6.13618845099998));
#206313=CARTESIAN_POINT('Ctrl Pts',(8.84089636399995,15.2,6.13817628099999));
#206314=CARTESIAN_POINT('Ctrl Pts',(8.84089636399995,11.6,6.13817628099999));
#206315=CARTESIAN_POINT('Ctrl Pts',(8.84251245399994,15.2,6.14017019299999));
#206316=CARTESIAN_POINT('Ctrl Pts',(8.84251245399994,11.6,6.14017019299999));
#206317=CARTESIAN_POINT('Ctrl Pts',(8.84413064299994,15.2,6.14217018399999));
#206318=CARTESIAN_POINT('Ctrl Pts',(8.84413064299994,11.6,6.14217018399999));
#206319=CARTESIAN_POINT('Ctrl Pts',(8.84575091399994,15.2,6.14417624999999));
#206320=CARTESIAN_POINT('Ctrl Pts',(8.84575091399994,11.6,6.14417624999999));
#206321=CARTESIAN_POINT('Ctrl Pts',(8.84737325499995,15.2,6.14618838899998));
#206322=CARTESIAN_POINT('Ctrl Pts',(8.84737325499995,11.6,6.14618838899998));
#206323=CARTESIAN_POINT('Ctrl Pts',(8.84899765099994,15.2,6.14820659599999));
#206324=CARTESIAN_POINT('Ctrl Pts',(8.84899765099994,11.6,6.14820659599999));
#206325=CARTESIAN_POINT('Ctrl Pts',(8.85062408799994,15.2,6.15023086999999));
#206326=CARTESIAN_POINT('Ctrl Pts',(8.85062408799994,11.6,6.15023086999999));
#206327=CARTESIAN_POINT('Ctrl Pts',(8.85225254999994,15.2,6.15226120499998));
#206328=CARTESIAN_POINT('Ctrl Pts',(8.85225254999994,11.6,6.15226120499998));
#206329=CARTESIAN_POINT('Ctrl Pts',(8.85388302599995,15.2,6.15429759899998));
#206330=CARTESIAN_POINT('Ctrl Pts',(8.85388302599995,11.6,6.15429759899998));
#206331=CARTESIAN_POINT('Ctrl Pts',(8.85551549999994,15.2,6.15634004899999));
#206332=CARTESIAN_POINT('Ctrl Pts',(8.85551549999994,11.6,6.15634004899999));
#206333=CARTESIAN_POINT('Ctrl Pts',(8.85714995899994,15.2,6.15838855199998));
#206334=CARTESIAN_POINT('Ctrl Pts',(8.85714995899994,11.6,6.15838855199998));
#206335=CARTESIAN_POINT('Ctrl Pts',(8.85878638799995,15.2,6.16044310299999));
#206336=CARTESIAN_POINT('Ctrl Pts',(8.85878638799995,11.6,6.16044310299999));
#206337=CARTESIAN_POINT('Ctrl Pts',(8.86042477299995,15.2,6.16250369999998));
#206338=CARTESIAN_POINT('Ctrl Pts',(8.86042477299995,11.6,6.16250369999998));
#206339=CARTESIAN_POINT('Ctrl Pts',(8.86206510099995,15.2,6.16457033999998));
#206340=CARTESIAN_POINT('Ctrl Pts',(8.86206510099995,11.6,6.16457033999998));
#206341=CARTESIAN_POINT('Ctrl Pts',(8.86370735799994,15.2,6.16664301699998));
#206342=CARTESIAN_POINT('Ctrl Pts',(8.86370735799994,11.6,6.16664301699998));
#206343=CARTESIAN_POINT('Ctrl Pts',(8.86535153099994,15.2,6.16872173199998));
#206344=CARTESIAN_POINT('Ctrl Pts',(8.86535153099994,11.6,6.16872173199998));
#206345=CARTESIAN_POINT('Ctrl Pts',(8.86699760299994,15.2,6.17080647799998));
#206346=CARTESIAN_POINT('Ctrl Pts',(8.86699760299994,11.6,6.17080647799998));
#206347=CARTESIAN_POINT('Ctrl Pts',(8.86864556399994,15.2,6.17289725399999));
#206348=CARTESIAN_POINT('Ctrl Pts',(8.86864556399994,11.6,6.17289725399999));
#206349=CARTESIAN_POINT('Ctrl Pts',(8.87029539799994,15.2,6.17499405499998));
#206350=CARTESIAN_POINT('Ctrl Pts',(8.87029539799994,11.6,6.17499405499998));
#206351=CARTESIAN_POINT('Ctrl Pts',(8.87194709099994,15.2,6.17709687799999));
#206352=CARTESIAN_POINT('Ctrl Pts',(8.87194709099994,11.6,6.17709687799999));
#206353=CARTESIAN_POINT('Ctrl Pts',(8.87360063099995,15.2,6.17920572099998));
#206354=CARTESIAN_POINT('Ctrl Pts',(8.87360063099995,11.6,6.17920572099998));
#206355=CARTESIAN_POINT('Ctrl Pts',(8.87525600399995,15.2,6.18132057799999));
#206356=CARTESIAN_POINT('Ctrl Pts',(8.87525600399995,11.6,6.18132057799999));
#206357=CARTESIAN_POINT('Ctrl Pts',(8.87691319699995,15.2,6.18344144999998));
#206358=CARTESIAN_POINT('Ctrl Pts',(8.87691319699995,11.6,6.18344144999998));
#206359=CARTESIAN_POINT('Ctrl Pts',(8.87857219499995,15.2,6.18556832899999));
#206360=CARTESIAN_POINT('Ctrl Pts',(8.87857219499995,11.6,6.18556832899999));
#206361=CARTESIAN_POINT('Ctrl Pts',(8.88023298399995,15.2,6.18770121299999));
#206362=CARTESIAN_POINT('Ctrl Pts',(8.88023298399995,11.6,6.18770121299999));
#206363=CARTESIAN_POINT('Ctrl Pts',(8.88189555299994,15.2,6.18984010099998));
#206364=CARTESIAN_POINT('Ctrl Pts',(8.88189555299994,11.6,6.18984010099998));
#206365=CARTESIAN_POINT('Ctrl Pts',(8.88355988699994,15.2,6.19198498699999));
#206366=CARTESIAN_POINT('Ctrl Pts',(8.88355988699994,11.6,6.19198498699999));
#206367=CARTESIAN_POINT('Ctrl Pts',(8.88522597299995,15.2,6.19413586899999));
#206368=CARTESIAN_POINT('Ctrl Pts',(8.88522597299995,11.6,6.19413586899999));
#206369=CARTESIAN_POINT('Ctrl Pts',(8.88689379699995,15.2,6.19629274299999));
#206370=CARTESIAN_POINT('Ctrl Pts',(8.88689379699995,11.6,6.19629274299999));
#206371=CARTESIAN_POINT('Ctrl Pts',(8.88856334799994,15.2,6.19845560599998));
#206372=CARTESIAN_POINT('Ctrl Pts',(8.88856334799994,11.6,6.19845560599998));
#206373=CARTESIAN_POINT('Ctrl Pts',(8.89023460899995,15.2,6.20062445499999));
#206374=CARTESIAN_POINT('Ctrl Pts',(8.89023460899995,11.6,6.20062445499999));
#206375=CARTESIAN_POINT('Ctrl Pts',(8.89190756899995,15.2,6.20279928499999));
#206376=CARTESIAN_POINT('Ctrl Pts',(8.89190756899995,11.6,6.20279928499999));
#206377=CARTESIAN_POINT('Ctrl Pts',(8.89358221599995,15.2,6.20498009499999));
#206378=CARTESIAN_POINT('Ctrl Pts',(8.89358221599995,11.6,6.20498009499999));
#206379=CARTESIAN_POINT('Ctrl Pts',(8.89525853299994,15.2,6.20716688099999));
#206380=CARTESIAN_POINT('Ctrl Pts',(8.89525853299994,11.6,6.20716688099999));
#206381=CARTESIAN_POINT('Ctrl Pts',(8.89693651199994,15.2,6.20935963799998));
#206382=CARTESIAN_POINT('Ctrl Pts',(8.89693651199994,11.6,6.20935963799998));
#206383=CARTESIAN_POINT('Ctrl Pts',(8.89861613499994,15.2,6.21155836399998));
#206384=CARTESIAN_POINT('Ctrl Pts',(8.89861613499994,11.6,6.21155836399998));
#206385=CARTESIAN_POINT('Ctrl Pts',(8.90029739199995,15.2,6.21376305599998));
#206386=CARTESIAN_POINT('Ctrl Pts',(8.90029739199995,11.6,6.21376305599998));
#206387=CARTESIAN_POINT('Ctrl Pts',(8.90198026899995,15.2,6.21597370999999));
#206388=CARTESIAN_POINT('Ctrl Pts',(8.90198026899995,11.6,6.21597370999999));
#206389=CARTESIAN_POINT('Ctrl Pts',(8.90366475299994,15.2,6.21819032099998));
#206390=CARTESIAN_POINT('Ctrl Pts',(8.90366475299994,11.6,6.21819032099998));
#206391=CARTESIAN_POINT('Ctrl Pts',(8.90535083099994,15.2,6.22041288899998));
#206392=CARTESIAN_POINT('Ctrl Pts',(8.90535083099994,11.6,6.22041288899998));
#206393=CARTESIAN_POINT('Ctrl Pts',(8.90703848999994,15.2,6.22264140899999));
#206394=CARTESIAN_POINT('Ctrl Pts',(8.90703848999994,11.6,6.22264140899999));
#206395=CARTESIAN_POINT('Ctrl Pts',(8.90872771799994,15.2,6.22487587699998));
#206396=CARTESIAN_POINT('Ctrl Pts',(8.90872771799994,11.6,6.22487587699998));
#206397=CARTESIAN_POINT('Ctrl Pts',(8.91041850099995,15.2,6.22711629099998));
#206398=CARTESIAN_POINT('Ctrl Pts',(8.91041850099995,11.6,6.22711629099998));
#206399=CARTESIAN_POINT('Ctrl Pts',(8.91211082699994,15.2,6.22936264599999));
#206400=CARTESIAN_POINT('Ctrl Pts',(8.91211082699994,11.6,6.22936264599999));
#206401=CARTESIAN_POINT('Ctrl Pts',(8.91380468299995,15.2,6.23161493999999));
#206402=CARTESIAN_POINT('Ctrl Pts',(8.91380468299995,11.6,6.23161493999999));
#206403=CARTESIAN_POINT('Ctrl Pts',(8.91550005599994,15.2,6.23387316899999));
#206404=CARTESIAN_POINT('Ctrl Pts',(8.91550005599994,11.6,6.23387316899999));
#206405=CARTESIAN_POINT('Ctrl Pts',(8.91719693299994,15.2,6.23613732899998));
#206406=CARTESIAN_POINT('Ctrl Pts',(8.91719693299994,11.6,6.23613732899998));
#206407=CARTESIAN_POINT('Ctrl Pts',(8.91889530199995,15.2,6.23840741899999));
#206408=CARTESIAN_POINT('Ctrl Pts',(8.91889530199995,11.6,6.23840741899999));
#206409=CARTESIAN_POINT('Ctrl Pts',(8.92059514999995,15.2,6.24068343399999));
#206410=CARTESIAN_POINT('Ctrl Pts',(8.92059514999995,11.6,6.24068343399999));
#206411=CARTESIAN_POINT('Ctrl Pts',(8.92229646399995,15.2,6.24296536899998));
#206412=CARTESIAN_POINT('Ctrl Pts',(8.92229646399995,11.6,6.24296536899998));
#206413=CARTESIAN_POINT('Ctrl Pts',(8.92399923199994,15.2,6.24525322299998));
#206414=CARTESIAN_POINT('Ctrl Pts',(8.92399923199994,11.6,6.24525322299998));
#206415=CARTESIAN_POINT('Ctrl Pts',(8.92570344199994,15.2,6.24754699299999));
#206416=CARTESIAN_POINT('Ctrl Pts',(8.92570344199994,11.6,6.24754699299999));
#206417=CARTESIAN_POINT('Ctrl Pts',(8.92740908099995,15.2,6.24984667299999));
#206418=CARTESIAN_POINT('Ctrl Pts',(8.92740908099995,11.6,6.24984667299999));
#206419=CARTESIAN_POINT('Ctrl Pts',(8.92911613499994,15.2,6.25215226099999));
#206420=CARTESIAN_POINT('Ctrl Pts',(8.92911613499994,11.6,6.25215226099999));
#206421=CARTESIAN_POINT('Ctrl Pts',(8.93082459399994,15.2,6.25446375399999));
#206422=CARTESIAN_POINT('Ctrl Pts',(8.93082459399994,11.6,6.25446375399999));
#206423=CARTESIAN_POINT('Ctrl Pts',(8.93253444299994,15.2,6.25678114999998));
#206424=CARTESIAN_POINT('Ctrl Pts',(8.93253444299994,11.6,6.25678114999998));
#206425=CARTESIAN_POINT('Ctrl Pts',(8.93424567199995,15.2,6.25910444199998));
#206426=CARTESIAN_POINT('Ctrl Pts',(8.93424567199995,11.6,6.25910444199998));
#206427=CARTESIAN_POINT('Ctrl Pts',(8.93595826799995,15.2,6.26143362999999));
#206428=CARTESIAN_POINT('Ctrl Pts',(8.93595826799995,11.6,6.26143362999999));
#206429=CARTESIAN_POINT('Ctrl Pts',(8.93767221799994,15.2,6.26376870799999));
#206430=CARTESIAN_POINT('Ctrl Pts',(8.93767221799994,11.6,6.26376870799999));
#206431=CARTESIAN_POINT('Ctrl Pts',(8.93938750999994,15.2,6.26610967499998));
#206432=CARTESIAN_POINT('Ctrl Pts',(8.93938750999994,11.6,6.26610967499998));
#206433=CARTESIAN_POINT('Ctrl Pts',(8.94110413199994,15.2,6.26845652599999));
#206434=CARTESIAN_POINT('Ctrl Pts',(8.94110413199994,11.6,6.26845652599999));
#206435=CARTESIAN_POINT('Ctrl Pts',(8.94282207099995,15.2,6.27080925799999));
#206436=CARTESIAN_POINT('Ctrl Pts',(8.94282207099995,11.6,6.27080925799999));
#206437=CARTESIAN_POINT('Ctrl Pts',(8.94454131499994,15.2,6.27316786599999));
#206438=CARTESIAN_POINT('Ctrl Pts',(8.94454131499994,11.6,6.27316786599999));
#206439=CARTESIAN_POINT('Ctrl Pts',(8.94626185299994,15.2,6.27553235099998));
#206440=CARTESIAN_POINT('Ctrl Pts',(8.94626185299994,11.6,6.27553235099998));
#206441=CARTESIAN_POINT('Ctrl Pts',(8.94798367199994,15.2,6.27790270599998));
#206442=CARTESIAN_POINT('Ctrl Pts',(8.94798367199994,11.6,6.27790270599998));
#206443=CARTESIAN_POINT('Ctrl Pts',(8.94970675999994,15.2,6.28027892699999));
#206444=CARTESIAN_POINT('Ctrl Pts',(8.94970675999994,11.6,6.28027892699999));
#206445=CARTESIAN_POINT('Ctrl Pts',(8.95143110399994,15.2,6.28266101399999));
#206446=CARTESIAN_POINT('Ctrl Pts',(8.95143110399994,11.6,6.28266101399999));
#206447=CARTESIAN_POINT('Ctrl Pts',(8.95315669399994,15.2,6.28504895999999));
#206448=CARTESIAN_POINT('Ctrl Pts',(8.95315669399994,11.6,6.28504895999999));
#206449=CARTESIAN_POINT('Ctrl Pts',(8.95488351599995,15.2,6.28744276399999));
#206450=CARTESIAN_POINT('Ctrl Pts',(8.95488351599995,11.6,6.28744276399999));
#206451=CARTESIAN_POINT('Ctrl Pts',(8.95661155799995,15.2,6.28984242199999));
#206452=CARTESIAN_POINT('Ctrl Pts',(8.95661155799995,11.6,6.28984242199999));
#206453=CARTESIAN_POINT('Ctrl Pts',(8.95834080899995,15.2,6.29224792999998));
#206454=CARTESIAN_POINT('Ctrl Pts',(8.95834080899995,11.6,6.29224792999998));
#206455=CARTESIAN_POINT('Ctrl Pts',(8.96007125799994,15.2,6.29465928599998));
#206456=CARTESIAN_POINT('Ctrl Pts',(8.96007125799994,11.6,6.29465928599998));
#206457=CARTESIAN_POINT('Ctrl Pts',(8.96180289099994,15.2,6.29707648499998));
#206458=CARTESIAN_POINT('Ctrl Pts',(8.96180289099994,11.6,6.29707648499998));
#206459=CARTESIAN_POINT('Ctrl Pts',(8.96353569799994,15.2,6.29949952399999));
#206460=CARTESIAN_POINT('Ctrl Pts',(8.96353569799994,11.6,6.29949952399999));
#206461=CARTESIAN_POINT('Ctrl Pts',(8.96526966599994,15.2,6.30192839999999));
#206462=CARTESIAN_POINT('Ctrl Pts',(8.96526966599994,11.6,6.30192839999999));
#206463=CARTESIAN_POINT('Ctrl Pts',(8.96700478399995,15.2,6.30436310899999));
#206464=CARTESIAN_POINT('Ctrl Pts',(8.96700478399995,11.6,6.30436310899999));
#206465=CARTESIAN_POINT('Ctrl Pts',(8.96874103899994,15.2,6.30680364899998));
#206466=CARTESIAN_POINT('Ctrl Pts',(8.96874103899994,11.6,6.30680364899998));
#206467=CARTESIAN_POINT('Ctrl Pts',(8.97047841899994,15.2,6.30925001499998));
#206468=CARTESIAN_POINT('Ctrl Pts',(8.97047841899994,11.6,6.30925001499998));
#206469=CARTESIAN_POINT('Ctrl Pts',(8.97221691399994,15.2,6.31170220499998));
#206470=CARTESIAN_POINT('Ctrl Pts',(8.97221691399994,11.6,6.31170220499998));
#206471=CARTESIAN_POINT('Ctrl Pts',(8.97395651199994,15.2,6.31416021399998));
#206472=CARTESIAN_POINT('Ctrl Pts',(8.97395651199994,11.6,6.31416021399998));
#206473=CARTESIAN_POINT('Ctrl Pts',(8.97569719999994,15.2,6.31662403999999));
#206474=CARTESIAN_POINT('Ctrl Pts',(8.97569719999994,11.6,6.31662403999999));
#206475=CARTESIAN_POINT('Ctrl Pts',(8.97743896899994,15.2,6.31909367799998));
#206476=CARTESIAN_POINT('Ctrl Pts',(8.97743896899994,11.6,6.31909367799998));
#206477=CARTESIAN_POINT('Ctrl Pts',(8.97918180399994,15.2,6.32156912499998));
#206478=CARTESIAN_POINT('Ctrl Pts',(8.97918180399994,11.6,6.32156912499998));
#206479=CARTESIAN_POINT('Ctrl Pts',(8.98092569499994,15.2,6.32405037899999));
#206480=CARTESIAN_POINT('Ctrl Pts',(8.98092569499994,11.6,6.32405037899999));
#206481=CARTESIAN_POINT('Ctrl Pts',(8.98267063099994,15.2,6.32653743699999));
#206482=CARTESIAN_POINT('Ctrl Pts',(8.98267063099994,11.6,6.32653743699999));
#206483=CARTESIAN_POINT('Ctrl Pts',(8.98441659999994,15.2,6.32903029299998));
#206484=CARTESIAN_POINT('Ctrl Pts',(8.98441659999994,11.6,6.32903029299998));
#206485=CARTESIAN_POINT('Ctrl Pts',(8.98616358999995,15.2,6.33152894399998));
#206486=CARTESIAN_POINT('Ctrl Pts',(8.98616358999995,11.6,6.33152894399998));
#206487=CARTESIAN_POINT('Ctrl Pts',(8.98791159099994,15.2,6.33403338899999));
#206488=CARTESIAN_POINT('Ctrl Pts',(8.98791159099994,11.6,6.33403338899999));
#206489=CARTESIAN_POINT('Ctrl Pts',(8.98966059099994,15.2,6.33654362099998));
#206490=CARTESIAN_POINT('Ctrl Pts',(8.98966059099994,11.6,6.33654362099998));
#206491=CARTESIAN_POINT('Ctrl Pts',(8.99141057699994,15.2,6.33905963999998));
#206492=CARTESIAN_POINT('Ctrl Pts',(8.99141057699994,11.6,6.33905963999998));
#206493=CARTESIAN_POINT('Ctrl Pts',(8.99316153799995,15.2,6.34158143999999));
#206494=CARTESIAN_POINT('Ctrl Pts',(8.99316153799995,11.6,6.34158143999999));
#206495=CARTESIAN_POINT('Ctrl Pts',(8.99491346499994,15.2,6.34410901999999));
#206496=CARTESIAN_POINT('Ctrl Pts',(8.99491346499994,11.6,6.34410901999999));
#206497=CARTESIAN_POINT('Ctrl Pts',(8.99666634399994,15.2,6.34664237499998));
#206498=CARTESIAN_POINT('Ctrl Pts',(8.99666634399994,11.6,6.34664237499998));
#206499=CARTESIAN_POINT('Ctrl Pts',(8.99842016599995,15.2,6.34918150199999));
#206500=CARTESIAN_POINT('Ctrl Pts',(8.99842016599995,11.6,6.34918150199999));
#206501=CARTESIAN_POINT('Ctrl Pts',(9.00017491699994,15.2,6.35172639699999));
#206502=CARTESIAN_POINT('Ctrl Pts',(9.00017491699994,11.6,6.35172639699999));
#206503=CARTESIAN_POINT('Ctrl Pts',(9.00193058899994,15.2,6.35427705699998));
#206504=CARTESIAN_POINT('Ctrl Pts',(9.00193058899994,11.6,6.35427705699998));
#206505=CARTESIAN_POINT('Ctrl Pts',(9.00368716799994,15.2,6.35683347799999));
#206506=CARTESIAN_POINT('Ctrl Pts',(9.00368716799994,11.6,6.35683347799999));
#206507=CARTESIAN_POINT('Ctrl Pts',(9.00544464399994,15.2,6.35939565799998));
#206508=CARTESIAN_POINT('Ctrl Pts',(9.00544464399994,11.6,6.35939565799998));
#206509=CARTESIAN_POINT('Ctrl Pts',(9.00720300599994,15.2,6.36196359199998));
#206510=CARTESIAN_POINT('Ctrl Pts',(9.00720300599994,11.6,6.36196359199998));
#206511=CARTESIAN_POINT('Ctrl Pts',(9.00896224199995,15.2,6.36453727799999));
#206512=CARTESIAN_POINT('Ctrl Pts',(9.00896224199995,11.6,6.36453727799999));
#206513=CARTESIAN_POINT('Ctrl Pts',(9.01072234199994,15.2,6.36711671099999));
#206514=CARTESIAN_POINT('Ctrl Pts',(9.01072234199994,11.6,6.36711671099999));
#206515=CARTESIAN_POINT('Ctrl Pts',(9.01248329499994,15.2,6.36970188899999));
#206516=CARTESIAN_POINT('Ctrl Pts',(9.01248329499994,11.6,6.36970188899999));
#206517=CARTESIAN_POINT('Ctrl Pts',(9.01424508899994,15.2,6.37229280699999));
#206518=CARTESIAN_POINT('Ctrl Pts',(9.01424508899994,11.6,6.37229280699999));
#206519=CARTESIAN_POINT('Ctrl Pts',(9.01600771199995,15.2,6.37488946299998));
#206520=CARTESIAN_POINT('Ctrl Pts',(9.01600771199995,11.6,6.37488946299998));
#206521=CARTESIAN_POINT('Ctrl Pts',(9.01777115599995,15.2,6.37749185299998));
#206522=CARTESIAN_POINT('Ctrl Pts',(9.01777115599995,11.6,6.37749185299998));
#206523=CARTESIAN_POINT('Ctrl Pts',(9.01953540799994,15.2,6.38009997399998));
#206524=CARTESIAN_POINT('Ctrl Pts',(9.01953540799994,11.6,6.38009997399998));
#206525=CARTESIAN_POINT('Ctrl Pts',(9.02130045699994,15.2,6.38271382099998));
#206526=CARTESIAN_POINT('Ctrl Pts',(9.02130045699994,11.6,6.38271382099998));
#206527=CARTESIAN_POINT('Ctrl Pts',(9.02306629199994,15.2,6.38533339199999));
#206528=CARTESIAN_POINT('Ctrl Pts',(9.02306629199994,11.6,6.38533339199999));
#206529=CARTESIAN_POINT('Ctrl Pts',(9.02483290299994,15.2,6.38795868399999));
#206530=CARTESIAN_POINT('Ctrl Pts',(9.02483290299994,11.6,6.38795868399999));
#206531=CARTESIAN_POINT('Ctrl Pts',(9.02660027799995,15.2,6.39058969199999));
#206532=CARTESIAN_POINT('Ctrl Pts',(9.02660027799995,11.6,6.39058969199999));
#206533=CARTESIAN_POINT('Ctrl Pts',(9.02836840899995,15.2,6.39322641399998));
#206534=CARTESIAN_POINT('Ctrl Pts',(9.02836840899995,11.6,6.39322641399998));
#206535=CARTESIAN_POINT('Ctrl Pts',(9.03013728099994,15.2,6.39586884499998));
#206536=CARTESIAN_POINT('Ctrl Pts',(9.03013728099994,11.6,6.39586884499998));
#206537=CARTESIAN_POINT('Ctrl Pts',(9.03190688599994,15.2,6.39851698299999));
#206538=CARTESIAN_POINT('Ctrl Pts',(9.03190688599994,11.6,6.39851698299999));
#206539=CARTESIAN_POINT('Ctrl Pts',(9.03367721299994,15.2,6.40117082399998));
#206540=CARTESIAN_POINT('Ctrl Pts',(9.03367721299994,11.6,6.40117082399998));
#206541=CARTESIAN_POINT('Ctrl Pts',(9.03544824899994,15.2,6.40383036399999));
#206542=CARTESIAN_POINT('Ctrl Pts',(9.03544824899994,11.6,6.40383036399999));
#206543=CARTESIAN_POINT('Ctrl Pts',(9.03721998599995,15.2,6.40649559999999));
#206544=CARTESIAN_POINT('Ctrl Pts',(9.03721998599995,11.6,6.40649559999999));
#206545=CARTESIAN_POINT('Ctrl Pts',(9.03899241199994,15.2,6.40916652899998));
#206546=CARTESIAN_POINT('Ctrl Pts',(9.03899241199994,11.6,6.40916652899998));
#206547=CARTESIAN_POINT('Ctrl Pts',(9.04076551699994,15.2,6.41184314699998));
#206548=CARTESIAN_POINT('Ctrl Pts',(9.04076551699994,11.6,6.41184314699998));
#206549=CARTESIAN_POINT('Ctrl Pts',(9.04253928999994,15.2,6.41452544999999));
#206550=CARTESIAN_POINT('Ctrl Pts',(9.04253928999994,11.6,6.41452544999999));
#206551=CARTESIAN_POINT('Ctrl Pts',(9.04431372099994,15.2,6.41721343699999));
#206552=CARTESIAN_POINT('Ctrl Pts',(9.04431372099994,11.6,6.41721343699999));
#206553=CARTESIAN_POINT('Ctrl Pts',(9.04608879799994,15.2,6.41990710099999));
#206554=CARTESIAN_POINT('Ctrl Pts',(9.04608879799994,11.6,6.41990710099999));
#206555=CARTESIAN_POINT('Ctrl Pts',(9.04786451099995,15.2,6.42260643999998));
#206556=CARTESIAN_POINT('Ctrl Pts',(9.04786451099995,11.6,6.42260643999998));
#206557=CARTESIAN_POINT('Ctrl Pts',(9.04964084999994,15.2,6.42531145199998));
#206558=CARTESIAN_POINT('Ctrl Pts',(9.04964084999994,11.6,6.42531145199998));
#206559=CARTESIAN_POINT('Ctrl Pts',(9.05141780299994,15.2,6.42802213199998));
#206560=CARTESIAN_POINT('Ctrl Pts',(9.05141780299994,11.6,6.42802213199998));
#206561=CARTESIAN_POINT('Ctrl Pts',(9.05319536099995,15.2,6.43073847599998));
#206562=CARTESIAN_POINT('Ctrl Pts',(9.05319536099995,11.6,6.43073847599998));
#206563=CARTESIAN_POINT('Ctrl Pts',(9.05497351399994,15.2,6.43346048299998));
#206564=CARTESIAN_POINT('Ctrl Pts',(9.05497351399994,11.6,6.43346048299998));
#206565=CARTESIAN_POINT('Ctrl Pts',(9.05675225099994,15.2,6.43618814699998));
#206566=CARTESIAN_POINT('Ctrl Pts',(9.05675225099994,11.6,6.43618814699998));
#206567=CARTESIAN_POINT('Ctrl Pts',(9.05853155999995,15.2,6.43892146399998));
#206568=CARTESIAN_POINT('Ctrl Pts',(9.05853155999995,11.6,6.43892146399998));
#206569=CARTESIAN_POINT('Ctrl Pts',(9.06031143299994,15.2,6.44166043399999));
#206570=CARTESIAN_POINT('Ctrl Pts',(9.06031143299994,11.6,6.44166043399999));
#206571=CARTESIAN_POINT('Ctrl Pts',(9.06209185699994,15.2,6.44440504999999));
#206572=CARTESIAN_POINT('Ctrl Pts',(9.06209185699994,11.6,6.44440504999999));
#206573=CARTESIAN_POINT('Ctrl Pts',(9.06387282499994,15.2,6.44715531099998));
#206574=CARTESIAN_POINT('Ctrl Pts',(9.06387282499994,11.6,6.44715531099998));
#206575=CARTESIAN_POINT('Ctrl Pts',(9.06565432399994,15.2,6.44991121299999));
#206576=CARTESIAN_POINT('Ctrl Pts',(9.06565432399994,11.6,6.44991121299999));
#206577=CARTESIAN_POINT('Ctrl Pts',(9.06743634399995,15.2,6.45267275099998));
#206578=CARTESIAN_POINT('Ctrl Pts',(9.06743634399995,11.6,6.45267275099998));
#206579=CARTESIAN_POINT('Ctrl Pts',(9.06921887499994,15.2,6.45543992199999));
#206580=CARTESIAN_POINT('Ctrl Pts',(9.06921887499994,11.6,6.45543992199999));
#206581=CARTESIAN_POINT('Ctrl Pts',(9.07100190699994,15.2,6.45821272499998));
#206582=CARTESIAN_POINT('Ctrl Pts',(9.07100190699994,11.6,6.45821272499998));
#206583=CARTESIAN_POINT('Ctrl Pts',(9.07278542999994,15.2,6.46099115299998));
#206584=CARTESIAN_POINT('Ctrl Pts',(9.07278542999994,11.6,6.46099115299998));
#206585=CARTESIAN_POINT('Ctrl Pts',(9.07456943399995,15.2,6.46377520499998));
#206586=CARTESIAN_POINT('Ctrl Pts',(9.07456943399995,11.6,6.46377520499998));
#206587=CARTESIAN_POINT('Ctrl Pts',(9.07635390799994,15.2,6.46656487599999));
#206588=CARTESIAN_POINT('Ctrl Pts',(9.07635390799994,11.6,6.46656487599999));
#206589=CARTESIAN_POINT('Ctrl Pts',(9.07813884099994,15.2,6.46936016399999));
#206590=CARTESIAN_POINT('Ctrl Pts',(9.07813884099994,11.6,6.46936016399999));
#206591=CARTESIAN_POINT('Ctrl Pts',(9.07992422599994,15.2,6.47216106399998));
#206592=CARTESIAN_POINT('Ctrl Pts',(9.07992422599994,11.6,6.47216106399998));
#206593=CARTESIAN_POINT('Ctrl Pts',(9.08171004899994,15.2,6.47496757299999));
#206594=CARTESIAN_POINT('Ctrl Pts',(9.08171004899994,11.6,6.47496757299999));
#206595=CARTESIAN_POINT('Ctrl Pts',(9.08349630299995,15.2,6.47777968799998));
#206596=CARTESIAN_POINT('Ctrl Pts',(9.08349630299995,11.6,6.47777968799998));
#206597=CARTESIAN_POINT('Ctrl Pts',(9.08528297599995,15.2,6.48059740499999));
#206598=CARTESIAN_POINT('Ctrl Pts',(9.08528297599995,11.6,6.48059740499999));
#206599=CARTESIAN_POINT('Ctrl Pts',(9.08707005899995,15.2,6.48342072099998));
#206600=CARTESIAN_POINT('Ctrl Pts',(9.08707005899995,11.6,6.48342072099998));
#206601=CARTESIAN_POINT('Ctrl Pts',(9.08885754099994,15.2,6.48624963299999));
#206602=CARTESIAN_POINT('Ctrl Pts',(9.08885754099994,11.6,6.48624963299999));
#206603=CARTESIAN_POINT('Ctrl Pts',(9.09064541299994,15.2,6.48908413499999));
#206604=CARTESIAN_POINT('Ctrl Pts',(9.09064541299994,11.6,6.48908413499999));
#206605=CARTESIAN_POINT('Ctrl Pts',(9.09243366399994,15.2,6.49192422699999));
#206606=CARTESIAN_POINT('Ctrl Pts',(9.09243366399994,11.6,6.49192422699999));
#206607=CARTESIAN_POINT('Ctrl Pts',(9.09422228599994,15.2,6.49476990299998));
#206608=CARTESIAN_POINT('Ctrl Pts',(9.09422228599994,11.6,6.49476990299998));
#206609=CARTESIAN_POINT('Ctrl Pts',(9.09601126799994,15.2,6.49762115899998));
#206610=CARTESIAN_POINT('Ctrl Pts',(9.09601126799994,11.6,6.49762115899998));
#206611=CARTESIAN_POINT('Ctrl Pts',(9.09780059799994,15.2,6.50047799499998));
#206612=CARTESIAN_POINT('Ctrl Pts',(9.09780059799994,11.6,6.50047799499998));
#206613=CARTESIAN_POINT('Ctrl Pts',(9.09959026799994,15.2,6.50334040299998));
#206614=CARTESIAN_POINT('Ctrl Pts',(9.09959026799994,11.6,6.50334040299998));
#206615=CARTESIAN_POINT('Ctrl Pts',(9.10138026999994,15.2,6.50620838299999));
#206616=CARTESIAN_POINT('Ctrl Pts',(9.10138026999994,11.6,6.50620838299999));
#206617=CARTESIAN_POINT('Ctrl Pts',(9.10317058999994,15.2,6.50908192999999));
#206618=CARTESIAN_POINT('Ctrl Pts',(9.10317058999994,11.6,6.50908192999999));
#206619=CARTESIAN_POINT('Ctrl Pts',(9.10496121999994,15.2,6.51196104099999));
#206620=CARTESIAN_POINT('Ctrl Pts',(9.10496121999994,11.6,6.51196104099999));
#206621=CARTESIAN_POINT('Ctrl Pts',(9.10675215199995,15.2,6.51484571199998));
#206622=CARTESIAN_POINT('Ctrl Pts',(9.10675215199995,11.6,6.51484571199998));
#206623=CARTESIAN_POINT('Ctrl Pts',(9.10854337499994,15.2,6.51773593999999));
#206624=CARTESIAN_POINT('Ctrl Pts',(9.10854337499994,11.6,6.51773593999999));
#206625=CARTESIAN_POINT('Ctrl Pts',(9.11033487799994,15.2,6.52063171999998));
#206626=CARTESIAN_POINT('Ctrl Pts',(9.11033487799994,11.6,6.52063171999998));
#206627=CARTESIAN_POINT('Ctrl Pts',(9.11212665199994,15.2,6.52353305199998));
#206628=CARTESIAN_POINT('Ctrl Pts',(9.11212665199994,11.6,6.52353305199998));
#206629=CARTESIAN_POINT('Ctrl Pts',(9.11391868799994,15.2,6.52643992799998));
#206630=CARTESIAN_POINT('Ctrl Pts',(9.11391868799994,11.6,6.52643992799998));
#206631=CARTESIAN_POINT('Ctrl Pts',(9.11571097599994,15.2,6.52935234799998));
#206632=CARTESIAN_POINT('Ctrl Pts',(9.11571097599994,11.6,6.52935234799998));
#206633=CARTESIAN_POINT('Ctrl Pts',(9.11750350599995,15.2,6.53227030699998));
#206634=CARTESIAN_POINT('Ctrl Pts',(9.11750350599995,11.6,6.53227030699998));
#206635=CARTESIAN_POINT('Ctrl Pts',(9.11929626799994,15.2,6.53519380099999));
#206636=CARTESIAN_POINT('Ctrl Pts',(9.11929626799994,11.6,6.53519380099999));
#206637=CARTESIAN_POINT('Ctrl Pts',(9.12108925299994,15.2,6.53812282799999));
#206638=CARTESIAN_POINT('Ctrl Pts',(9.12108925299994,11.6,6.53812282799999));
#206639=CARTESIAN_POINT('Ctrl Pts',(9.12288245099995,15.2,6.54105738299998));
#206640=CARTESIAN_POINT('Ctrl Pts',(9.12288245099995,11.6,6.54105738299998));
#206641=CARTESIAN_POINT('Ctrl Pts',(9.12467585299994,15.2,6.54399746299998));
#206642=CARTESIAN_POINT('Ctrl Pts',(9.12467585299994,11.6,6.54399746299998));
#206643=CARTESIAN_POINT('Ctrl Pts',(9.12646944899994,15.2,6.54694306399998));
#206644=CARTESIAN_POINT('Ctrl Pts',(9.12646944899994,11.6,6.54694306399998));
#206645=CARTESIAN_POINT('Ctrl Pts',(9.12826322899994,15.2,6.54989418499999));
#206646=CARTESIAN_POINT('Ctrl Pts',(9.12826322899994,11.6,6.54989418499999));
#206647=CARTESIAN_POINT('Ctrl Pts',(9.13005718399994,15.2,6.55285081999998));
#206648=CARTESIAN_POINT('Ctrl Pts',(9.13005718399994,11.6,6.55285081999998));
#206649=CARTESIAN_POINT('Ctrl Pts',(9.13185130399994,15.2,6.55581296599999));
#206650=CARTESIAN_POINT('Ctrl Pts',(9.13185130399994,11.6,6.55581296599999));
#206651=CARTESIAN_POINT('Ctrl Pts',(9.13364558099994,15.2,6.55878061899998));
#206652=CARTESIAN_POINT('Ctrl Pts',(9.13364558099994,11.6,6.55878061899998));
#206653=CARTESIAN_POINT('Ctrl Pts',(9.13544000399994,15.2,6.56175377599999));
#206654=CARTESIAN_POINT('Ctrl Pts',(9.13544000399994,11.6,6.56175377599999));
#206655=CARTESIAN_POINT('Ctrl Pts',(9.13723456499994,15.2,6.56473243399999));
#206656=CARTESIAN_POINT('Ctrl Pts',(9.13723456499994,11.6,6.56473243399999));
#206657=CARTESIAN_POINT('Ctrl Pts',(9.13902925199995,15.2,6.56771658899999));
#206658=CARTESIAN_POINT('Ctrl Pts',(9.13902925199995,11.6,6.56771658899999));
#206659=CARTESIAN_POINT('Ctrl Pts',(9.14082405799994,15.2,6.57070623799999));
#206660=CARTESIAN_POINT('Ctrl Pts',(9.14082405799994,11.6,6.57070623799999));
#206661=CARTESIAN_POINT('Ctrl Pts',(9.14261897099994,15.2,6.57370137599998));
#206662=CARTESIAN_POINT('Ctrl Pts',(9.14261897099994,11.6,6.57370137599998));
#206663=CARTESIAN_POINT('Ctrl Pts',(9.14441398599994,15.2,6.57670200099999));
#206664=CARTESIAN_POINT('Ctrl Pts',(9.14441398599994,11.6,6.57670200099999));
#206665=CARTESIAN_POINT('Ctrl Pts',(9.14620908999994,15.2,6.57970810799998));
#206666=CARTESIAN_POINT('Ctrl Pts',(9.14620908999994,11.6,6.57970810799998));
#206667=CARTESIAN_POINT('Ctrl Pts',(9.14800427399994,15.2,6.58271969499998));
#206668=CARTESIAN_POINT('Ctrl Pts',(9.14800427399994,11.6,6.58271969499998));
#206669=CARTESIAN_POINT('Ctrl Pts',(9.14979952999994,15.2,6.58573675799998));
#206670=CARTESIAN_POINT('Ctrl Pts',(9.14979952999994,11.6,6.58573675799998));
#206671=CARTESIAN_POINT('Ctrl Pts',(9.15159484799995,15.2,6.58875929299998));
#206672=CARTESIAN_POINT('Ctrl Pts',(9.15159484799995,11.6,6.58875929299998));
#206673=CARTESIAN_POINT('Ctrl Pts',(9.15339021899995,15.2,6.59178729599999));
#206674=CARTESIAN_POINT('Ctrl Pts',(9.15339021899995,11.6,6.59178729599999));
#206675=CARTESIAN_POINT('Ctrl Pts',(9.15518563399995,15.2,6.59482076599998));
#206676=CARTESIAN_POINT('Ctrl Pts',(9.15518563399995,11.6,6.59482076599998));
#206677=CARTESIAN_POINT('Ctrl Pts',(9.15698108299994,15.2,6.59785969599999));
#206678=CARTESIAN_POINT('Ctrl Pts',(9.15698108299994,11.6,6.59785969599999));
#206679=CARTESIAN_POINT('Ctrl Pts',(9.15877655699994,15.2,6.60090408599999));
#206680=CARTESIAN_POINT('Ctrl Pts',(9.15877655699994,11.6,6.60090408599999));
#206681=CARTESIAN_POINT('Ctrl Pts',(9.16057204699994,15.2,6.60395392999998));
#206682=CARTESIAN_POINT('Ctrl Pts',(9.16057204699994,11.6,6.60395392999998));
#206683=CARTESIAN_POINT('Ctrl Pts',(9.16236754399994,15.2,6.60700922399998));
#206684=CARTESIAN_POINT('Ctrl Pts',(9.16236754399994,11.6,6.60700922399998));
#206685=CARTESIAN_POINT('Ctrl Pts',(9.16416303799994,15.2,6.61006996599999));
#206686=CARTESIAN_POINT('Ctrl Pts',(9.16416303799994,11.6,6.61006996599999));
#206687=CARTESIAN_POINT('Ctrl Pts',(9.16595852199995,15.2,6.61313615199998));
#206688=CARTESIAN_POINT('Ctrl Pts',(9.16595852199995,11.6,6.61313615199998));
#206689=CARTESIAN_POINT('Ctrl Pts',(9.16775398399994,15.2,6.61620777999998));
#206690=CARTESIAN_POINT('Ctrl Pts',(9.16775398399994,11.6,6.61620777999998));
#206691=CARTESIAN_POINT('Ctrl Pts',(9.16954941699995,15.2,6.61928484299998));
#206692=CARTESIAN_POINT('Ctrl Pts',(9.16954941699995,11.6,6.61928484299998));
#206693=CARTESIAN_POINT('Ctrl Pts',(9.17134480999995,15.2,6.62236733999999));
#206694=CARTESIAN_POINT('Ctrl Pts',(9.17134480999995,11.6,6.62236733999999));
#206695=CARTESIAN_POINT('Ctrl Pts',(9.17314015699995,15.2,6.62545526799998));
#206696=CARTESIAN_POINT('Ctrl Pts',(9.17314015699995,11.6,6.62545526799998));
#206697=CARTESIAN_POINT('Ctrl Pts',(9.17493544599994,15.2,6.62854862099999));
#206698=CARTESIAN_POINT('Ctrl Pts',(9.17493544599994,11.6,6.62854862099999));
#206699=CARTESIAN_POINT('Ctrl Pts',(9.17673066899994,15.2,6.63164739699998));
#206700=CARTESIAN_POINT('Ctrl Pts',(9.17673066899994,11.6,6.63164739699998));
#206701=CARTESIAN_POINT('Ctrl Pts',(9.17852581699995,15.2,6.63475159199999));
#206702=CARTESIAN_POINT('Ctrl Pts',(9.17852581699995,11.6,6.63475159199999));
#206703=CARTESIAN_POINT('Ctrl Pts',(9.18032088299995,15.2,6.63786120299999));
#206704=CARTESIAN_POINT('Ctrl Pts',(9.18032088299995,11.6,6.63786120299999));
#206705=CARTESIAN_POINT('Ctrl Pts',(9.18211585399994,15.2,6.64097622599999));
#206706=CARTESIAN_POINT('Ctrl Pts',(9.18211585399994,11.6,6.64097622599999));
#206707=CARTESIAN_POINT('Ctrl Pts',(9.18391072399994,15.2,6.64409665799998));
#206708=CARTESIAN_POINT('Ctrl Pts',(9.18391072399994,11.6,6.64409665799998));
#206709=CARTESIAN_POINT('Ctrl Pts',(9.18570548299994,15.2,6.64722249499999));
#206710=CARTESIAN_POINT('Ctrl Pts',(9.18570548299994,11.6,6.64722249499999));
#206711=CARTESIAN_POINT('Ctrl Pts',(9.18750012399994,15.2,6.65035373299999));
#206712=CARTESIAN_POINT('Ctrl Pts',(9.18750012399994,11.6,6.65035373299999));
#206713=CARTESIAN_POINT('Ctrl Pts',(9.18929463499994,15.2,6.65349036999999));
#206714=CARTESIAN_POINT('Ctrl Pts',(9.18929463499994,11.6,6.65349036999999));
#206715=CARTESIAN_POINT('Ctrl Pts',(9.19108900999994,15.2,6.65663239999999));
#206716=CARTESIAN_POINT('Ctrl Pts',(9.19108900999994,11.6,6.65663239999999));
#206717=CARTESIAN_POINT('Ctrl Pts',(9.19288323699995,15.2,6.65977982199998));
#206718=CARTESIAN_POINT('Ctrl Pts',(9.19288323699995,11.6,6.65977982199998));
#206719=CARTESIAN_POINT('Ctrl Pts',(9.19467730999994,15.2,6.66293263099998));
#206720=CARTESIAN_POINT('Ctrl Pts',(9.19467730999994,11.6,6.66293263099998));
#206721=CARTESIAN_POINT('Ctrl Pts',(9.19647121899994,15.2,6.66609082299999));
#206722=CARTESIAN_POINT('Ctrl Pts',(9.19647121899994,11.6,6.66609082299999));
#206723=CARTESIAN_POINT('Ctrl Pts',(9.19826495499994,15.2,6.66925439599999));
#206724=CARTESIAN_POINT('Ctrl Pts',(9.19826495499994,11.6,6.66925439599999));
#206725=CARTESIAN_POINT('Ctrl Pts',(9.20005851099994,15.2,6.67242334499999));
#206726=CARTESIAN_POINT('Ctrl Pts',(9.20005851099994,11.6,6.67242334499999));
#206727=CARTESIAN_POINT('Ctrl Pts',(9.20185187499994,15.2,6.67559766799998));
#206728=CARTESIAN_POINT('Ctrl Pts',(9.20185187499994,11.6,6.67559766799998));
#206729=CARTESIAN_POINT('Ctrl Pts',(9.20364504099994,15.2,6.67877735899999));
#206730=CARTESIAN_POINT('Ctrl Pts',(9.20364504099994,11.6,6.67877735899999));
#206731=CARTESIAN_POINT('Ctrl Pts',(9.20543799999994,15.2,6.68196241699999));
#206732=CARTESIAN_POINT('Ctrl Pts',(9.20543799999994,11.6,6.68196241699999));
#206733=CARTESIAN_POINT('Ctrl Pts',(9.20723074199995,15.2,6.68515283699998));
#206734=CARTESIAN_POINT('Ctrl Pts',(9.20723074199995,11.6,6.68515283699998));
#206735=CARTESIAN_POINT('Ctrl Pts',(9.20902325999995,15.2,6.68834861599999));
#206736=CARTESIAN_POINT('Ctrl Pts',(9.20902325999995,11.6,6.68834861599999));
#206737=CARTESIAN_POINT('Ctrl Pts',(9.21081554299995,15.2,6.69154974999999));
#206738=CARTESIAN_POINT('Ctrl Pts',(9.21081554299995,11.6,6.69154974999999));
#206739=CARTESIAN_POINT('Ctrl Pts',(9.21260758499994,15.2,6.69475623599999));
#206740=CARTESIAN_POINT('Ctrl Pts',(9.21260758499994,11.6,6.69475623599999));
#206741=CARTESIAN_POINT('Ctrl Pts',(9.21439937499994,15.2,6.69796807099999));
#206742=CARTESIAN_POINT('Ctrl Pts',(9.21439937499994,11.6,6.69796807099999));
#206743=CARTESIAN_POINT('Ctrl Pts',(9.21619090599994,15.2,6.70118524899999));
#206744=CARTESIAN_POINT('Ctrl Pts',(9.21619090599994,11.6,6.70118524899999));
#206745=CARTESIAN_POINT('Ctrl Pts',(9.21798216799995,15.2,6.70440776899999));
#206746=CARTESIAN_POINT('Ctrl Pts',(9.21798216799995,11.6,6.70440776899999));
#206747=CARTESIAN_POINT('Ctrl Pts',(9.21977315299995,15.2,6.70763562499998));
#206748=CARTESIAN_POINT('Ctrl Pts',(9.21977315299995,11.6,6.70763562499998));
#206749=CARTESIAN_POINT('Ctrl Pts',(9.22156385299994,15.2,6.71086881599999));
#206750=CARTESIAN_POINT('Ctrl Pts',(9.22156385299994,11.6,6.71086881599999));
#206751=CARTESIAN_POINT('Ctrl Pts',(9.22335425899995,15.2,6.71410733599998));
#206752=CARTESIAN_POINT('Ctrl Pts',(9.22335425899995,11.6,6.71410733599998));
#206753=CARTESIAN_POINT('Ctrl Pts',(9.22514436299995,15.2,6.71735118499999));
#206754=CARTESIAN_POINT('Ctrl Pts',(9.22514436299995,11.6,6.71735118499999));
#206755=CARTESIAN_POINT('Ctrl Pts',(9.22693415699994,15.2,6.72060035599999));
#206756=CARTESIAN_POINT('Ctrl Pts',(9.22693415699994,11.6,6.72060035599999));
#206757=CARTESIAN_POINT('Ctrl Pts',(9.22872363199994,15.2,6.72385484699999));
#206758=CARTESIAN_POINT('Ctrl Pts',(9.22872363199994,11.6,6.72385484699999));
#206759=CARTESIAN_POINT('Ctrl Pts',(9.23051277899994,15.2,6.72711465399999));
#206760=CARTESIAN_POINT('Ctrl Pts',(9.23051277899994,11.6,6.72711465399999));
#206761=CARTESIAN_POINT('Ctrl Pts',(9.23230158999995,15.2,6.73037977299998));
#206762=CARTESIAN_POINT('Ctrl Pts',(9.23230158999995,11.6,6.73037977299998));
#206763=CARTESIAN_POINT('Ctrl Pts',(9.23409005699994,15.2,6.73365020099999));
#206764=CARTESIAN_POINT('Ctrl Pts',(9.23409005699994,11.6,6.73365020099999));
#206765=CARTESIAN_POINT('Ctrl Pts',(9.23587816899994,15.2,6.73692593499998));
#206766=CARTESIAN_POINT('Ctrl Pts',(9.23587816899994,11.6,6.73692593499998));
#206767=CARTESIAN_POINT('Ctrl Pts',(9.23766591999994,15.2,6.74020696899999));
#206768=CARTESIAN_POINT('Ctrl Pts',(9.23766591999994,11.6,6.74020696899999));
#206769=CARTESIAN_POINT('Ctrl Pts',(9.23945329899994,15.2,6.74349330199998));
#206770=CARTESIAN_POINT('Ctrl Pts',(9.23945329899994,11.6,6.74349330199998));
#206771=CARTESIAN_POINT('Ctrl Pts',(9.24124029999994,15.2,6.74678492799998));
#206772=CARTESIAN_POINT('Ctrl Pts',(9.24124029999994,11.6,6.74678492799998));
#206773=CARTESIAN_POINT('Ctrl Pts',(9.24302691299994,15.2,6.75008184599999));
#206774=CARTESIAN_POINT('Ctrl Pts',(9.24302691299994,11.6,6.75008184599999));
#206775=CARTESIAN_POINT('Ctrl Pts',(9.24481313099994,15.2,6.75338405099998));
#206776=CARTESIAN_POINT('Ctrl Pts',(9.24481313099994,11.6,6.75338405099998));
#206777=CARTESIAN_POINT('Ctrl Pts',(9.24659894799994,15.2,6.75669153999999));
#206778=CARTESIAN_POINT('Ctrl Pts',(9.24659894799994,11.6,6.75669153999999));
#206779=CARTESIAN_POINT('Ctrl Pts',(9.24838435499994,15.2,6.76000431099999));
#206780=CARTESIAN_POINT('Ctrl Pts',(9.24838435499994,11.6,6.76000431099999));
#206781=CARTESIAN_POINT('Ctrl Pts',(9.25016934499994,15.2,6.76332235799999));
#206782=CARTESIAN_POINT('Ctrl Pts',(9.25016934499994,11.6,6.76332235799999));
#206783=CARTESIAN_POINT('Ctrl Pts',(9.25195390799994,15.2,6.76664567999998));
#206784=CARTESIAN_POINT('Ctrl Pts',(9.25195390799994,11.6,6.76664567999998));
#206785=CARTESIAN_POINT('Ctrl Pts',(9.25373803599994,15.2,6.76997427199999));
#206786=CARTESIAN_POINT('Ctrl Pts',(9.25373803599994,11.6,6.76997427199999));
#206787=CARTESIAN_POINT('Ctrl Pts',(9.25552171699995,15.2,6.77330812899999));
#206788=CARTESIAN_POINT('Ctrl Pts',(9.25552171699995,11.6,6.77330812899999));
#206789=CARTESIAN_POINT('Ctrl Pts',(9.25730494299994,15.2,6.77664724599998));
#206790=CARTESIAN_POINT('Ctrl Pts',(9.25730494299994,11.6,6.77664724599998));
#206791=CARTESIAN_POINT('Ctrl Pts',(9.25908770199994,15.2,6.77999162099999));
#206792=CARTESIAN_POINT('Ctrl Pts',(9.25908770199994,11.6,6.77999162099999));
#206793=CARTESIAN_POINT('Ctrl Pts',(9.26086998599994,15.2,6.78334124699998));
#206794=CARTESIAN_POINT('Ctrl Pts',(9.26086998599994,11.6,6.78334124699998));
#206795=CARTESIAN_POINT('Ctrl Pts',(9.26265178899994,15.2,6.78669612499998));
#206796=CARTESIAN_POINT('Ctrl Pts',(9.26265178899994,11.6,6.78669612499998));
#206797=CARTESIAN_POINT('Ctrl Pts',(9.26443310199994,15.2,6.79005624799998));
#206798=CARTESIAN_POINT('Ctrl Pts',(9.26443310199994,11.6,6.79005624799998));
#206799=CARTESIAN_POINT('Ctrl Pts',(9.26621392399994,15.2,6.79342161599998));
#206800=CARTESIAN_POINT('Ctrl Pts',(9.26621392399994,11.6,6.79342161599998));
#206801=CARTESIAN_POINT('Ctrl Pts',(9.26799425299994,15.2,6.79679222999999));
#206802=CARTESIAN_POINT('Ctrl Pts',(9.26799425299994,11.6,6.79679222999999));
#206803=CARTESIAN_POINT('Ctrl Pts',(9.26941811999994,15.2,6.79949291499998));
#206804=CARTESIAN_POINT('Ctrl Pts',(9.26941811999994,11.6,6.79949291499998));
#206805=CARTESIAN_POINT('Ctrl Pts',(9.27048579799994,15.2,6.80152078799999));
#206806=CARTESIAN_POINT('Ctrl Pts',(9.27048579799994,11.6,6.80152078799999));
#206807=CARTESIAN_POINT('Ctrl Pts',(9.27119748299994,15.2,6.80287375299999));
#206808=CARTESIAN_POINT('Ctrl Pts',(9.27119748299994,11.6,6.80287375299999));
#206809=CARTESIAN_POINT('Ctrl Pts',(9.27155330199994,15.2,6.80355049599999));
#206810=CARTESIAN_POINT('Ctrl Pts',(9.27155330199994,11.6,6.80355049599999));
#206811=CARTESIAN_POINT('Ctrl Pts',(8.56667970899995,15.2,5.85257411499998));
#206812=CARTESIAN_POINT('Ctrl Pts',(8.5680628930964,15.2,5.85370502577855));
#206813=CARTESIAN_POINT('Ctrl Pts',(8.5694869244067,15.2,5.85487627485597));
#206814=CARTESIAN_POINT('Ctrl Pts',(8.5709506523979,15.2,5.85608775314224));
#206815=CARTESIAN_POINT('Ctrl Pts',(8.57242143922536,15.2,5.85730507378917));
#206816=CARTESIAN_POINT('Ctrl Pts',(8.57393230443574,15.2,5.85856301214596));
#206817=CARTESIAN_POINT('Ctrl Pts',(8.57548210843323,15.2,5.85986145286728));
#206818=CARTESIAN_POINT('Ctrl Pts',(8.57703191228994,15.2,5.86115989347067));
#206819=CARTESIAN_POINT('Ctrl Pts',(8.57862065432565,15.2,5.8624988373167));
#206820=CARTESIAN_POINT('Ctrl Pts',(8.58024722826654,15.2,5.86387816976658));
#206821=CARTESIAN_POINT('Ctrl Pts',(8.58187380220742,15.2,5.86525750221645));
#206822=CARTESIAN_POINT('Ctrl Pts',(8.58353820816439,15.2,5.86667722297458));
#206823=CARTESIAN_POINT('Ctrl Pts',(8.58523937135207,15.2,5.86813722032544));
#206824=CARTESIAN_POINT('Ctrl Pts',(8.58694053469429,15.2,5.86959721780893));
#206825=CARTESIAN_POINT('Ctrl Pts',(8.58867845563581,15.2,5.87109748993948));
#206826=CARTESIAN_POINT('Ctrl Pts',(8.59045208798488,15.2,5.87263792444283));
#206827=CARTESIAN_POINT('Ctrl Pts',(8.59252132548382,15.2,5.87443509782017));
#206828=CARTESIAN_POINT('Ctrl Pts',(8.59463917073834,15.2,5.87628693691257));
#206829=CARTESIAN_POINT('Ctrl Pts',(8.59680401336214,15.2,5.87819326040028));
#206830=CARTESIAN_POINT('Ctrl Pts',(8.59865959297066,15.2,5.87982725215201));
#206831=CARTESIAN_POINT('Ctrl Pts',(8.60054970122744,15.2,5.88150127369895));
#206832=CARTESIAN_POINT('Ctrl Pts',(8.60247335675124,15.2,5.88321521321174));
#206833=CARTESIAN_POINT('Ctrl Pts',(8.6043970121003,15.2,5.88492915256886));
#206834=CARTESIAN_POINT('Ctrl Pts',(8.60635421133064,15.2,5.88668300813266));
#206835=CARTESIAN_POINT('Ctrl Pts',(8.60834399976746,15.2,5.8884766674924));
#206836=CARTESIAN_POINT('Ctrl Pts',(8.61033378820427,15.2,5.89027032685213));
#206837=CARTESIAN_POINT('Ctrl Pts',(8.61235616229743,15.2,5.89210379097614));
#206838=CARTESIAN_POINT('Ctrl Pts',(8.61441019188808,15.2,5.89397694365633));
#206839=CARTESIAN_POINT('Ctrl Pts',(8.6164642216653,15.2,5.89585009650669));
#206840=CARTESIAN_POINT('Ctrl Pts',(8.61854990577146,15.2,5.89776294282028));
#206841=CARTESIAN_POINT('Ctrl Pts',(8.62066633380559,15.2,5.89971536542941));
#206842=CARTESIAN_POINT('Ctrl Pts',(8.62278276164747,15.2,5.90166778786119));
#206843=CARTESIAN_POINT('Ctrl Pts',(8.62492993542981,15.2,5.9036597878579));
#206844=CARTESIAN_POINT('Ctrl Pts',(8.627106966352,15.2,5.90569125236913));
#206845=CARTESIAN_POINT('Ctrl Pts',(8.62928399727419,15.2,5.90772271688036));
#206846=CARTESIAN_POINT('Ctrl Pts',(8.63149088542733,15.2,5.90979364605512));
#206847=CARTESIAN_POINT('Ctrl Pts',(8.63372676734483,15.2,5.91190392739341));
#206848=CARTESIAN_POINT('Ctrl Pts',(8.63596264926232,15.2,5.91401420873169));
#206849=CARTESIAN_POINT('Ctrl Pts',(8.63822752414354,15.2,5.91616384011022));
#206850=CARTESIAN_POINT('Ctrl Pts',(8.64052054897496,15.2,5.91835271052801));
#206851=CARTESIAN_POINT('Ctrl Pts',(8.64281357401467,15.2,5.92054158114462));
#206852=CARTESIAN_POINT('Ctrl Pts',(8.64513474718215,15.2,5.92276968904004));
#206853=CARTESIAN_POINT('Ctrl Pts',(8.64748324564467,15.2,5.92503692258198));
#206854=CARTESIAN_POINT('Ctrl Pts',(8.64983174389386,15.2,5.92730415591797));
#206855=CARTESIAN_POINT('Ctrl Pts',(8.65220756771585,15.2,5.92961051408417));
#206856=CARTESIAN_POINT('Ctrl Pts',(8.65460991187742,15.2,5.9319558825806));
#206857=CARTESIAN_POINT('Ctrl Pts',(8.65701225603899,15.2,5.93430125107702));
#206858=CARTESIAN_POINT('Ctrl Pts',(8.65944111983161,15.2,5.93668563184312));
#206859=CARTESIAN_POINT('Ctrl Pts',(8.66189571899069,15.2,5.93910890925246));
#206860=CARTESIAN_POINT('Ctrl Pts',(8.66435031837273,15.2,5.9415321868819));
#206861=CARTESIAN_POINT('Ctrl Pts',(8.66683065253225,15.2,5.94399436288172));
#206862=CARTESIAN_POINT('Ctrl Pts',(8.66933595116988,15.2,5.94649532068638));
#206863=CARTESIAN_POINT('Ctrl Pts',(8.67225879923911,15.2,5.94941310445107));
#206864=CARTESIAN_POINT('Ctrl Pts',(8.67521562943652,15.2,5.95238367869775));
#206865=CARTESIAN_POINT('Ctrl Pts',(8.67820524826226,15.2,5.95540685999247));
#206866=CARTESIAN_POINT('Ctrl Pts',(8.68076777898359,15.2,5.95799815854772));
#206867=CARTESIAN_POINT('Ctrl Pts',(8.68335440181564,15.2,5.96062810723174));
#206868=CARTESIAN_POINT('Ctrl Pts',(8.68596438262558,15.2,5.96329659187885));
#206869=CARTESIAN_POINT('Ctrl Pts',(8.68857436319844,15.2,5.96596507628358));
#206870=CARTESIAN_POINT('Ctrl Pts',(8.69120770284151,15.2,5.96867209749437));
#206871=CARTESIAN_POINT('Ctrl Pts',(8.69386368550703,15.2,5.97141753899034));
#206872=CARTESIAN_POINT('Ctrl Pts',(8.69651966817254,15.2,5.9741629804863));
#206873=CARTESIAN_POINT('Ctrl Pts',(8.69919829322183,15.2,5.97694684462246));
#206874=CARTESIAN_POINT('Ctrl Pts',(8.70189885895555,15.2,5.97976901493398));
#206875=CARTESIAN_POINT('Ctrl Pts',(8.70459942493457,15.2,5.98259118550184));
#206876=CARTESIAN_POINT('Ctrl Pts',(8.70732193266089,15.2,5.9854516627421));
#206877=CARTESIAN_POINT('Ctrl Pts',(8.71006569578205,15.2,5.98835033154708));
#206878=CARTESIAN_POINT('Ctrl Pts',(8.71235216492506,15.2,5.99076588875292));
#206879=CARTESIAN_POINT('Ctrl Pts',(8.71465339369052,15.2,5.99320796962066));
#206880=CARTESIAN_POINT('Ctrl Pts',(8.7169689935528,15.2,5.99567650358114));
#206881=CARTESIAN_POINT('Ctrl Pts',(8.71928459341506,15.2,5.99814503754163));
#206882=CARTESIAN_POINT('Ctrl Pts',(8.72161456367202,15.2,6.00064002790532));
#206883=CARTESIAN_POINT('Ctrl Pts',(8.7239585220065,15.2,6.00316140658806));
#206884=CARTESIAN_POINT('Ctrl Pts',(8.72677127190571,15.2,6.00618706089739));
#206885=CARTESIAN_POINT('Ctrl Pts',(8.72960416329157,15.2,6.00925071275516));
#206886=CARTESIAN_POINT('Ctrl Pts',(8.73245654618878,15.2,6.01235225089412));
#206887=CARTESIAN_POINT('Ctrl Pts',(8.73483353202283,15.2,6.01493686610382));
#206888=CARTESIAN_POINT('Ctrl Pts',(8.7372240554676,15.2,6.01754778784338));
#206889=CARTESIAN_POINT('Ctrl Pts',(8.73962774394052,15.2,6.02018495145588));
#206890=CARTESIAN_POINT('Ctrl Pts',(8.74203143241346,15.2,6.02282211506838));
#206891=CARTESIAN_POINT('Ctrl Pts',(8.74444828873749,15.2,6.02548551968159));
#206892=CARTESIAN_POINT('Ctrl Pts',(8.74687794754034,15.2,6.02817509780391));
#206893=CARTESIAN_POINT('Ctrl Pts',(8.74930760634317,15.2,6.03086467592622));
#206894=CARTESIAN_POINT('Ctrl Pts',(8.75175007054779,15.2,6.03358042787311));
#206895=CARTESIAN_POINT('Ctrl Pts',(8.75420497985435,15.2,6.03632228662523));
#206896=CARTESIAN_POINT('Ctrl Pts',(8.75665988916092,15.2,6.03906414537735));
#206897=CARTESIAN_POINT('Ctrl Pts',(8.75912724439545,15.2,6.04183210994103));
#206898=CARTESIAN_POINT('Ctrl Pts',(8.7616066938409,15.2,6.04462611362372));
#206899=CARTESIAN_POINT('Ctrl Pts',(8.76408614301609,15.2,6.04742011700186));
#206900=CARTESIAN_POINT('Ctrl Pts',(8.76657768737967,15.2,6.05024015992893));
#206901=CARTESIAN_POINT('Ctrl Pts',(8.76908098043915,15.2,6.05308617343601));
#206902=CARTESIAN_POINT('Ctrl Pts',(8.77208493260169,15.2,6.05650139020287));
#206903=CARTESIAN_POINT('Ctrl Pts',(8.77510579954927,15.2,6.05995400576511));
#206904=CARTESIAN_POINT('Ctrl Pts',(8.77814299788217,15.2,6.06344390245694));
#206905=CARTESIAN_POINT('Ctrl Pts',(8.78067399635499,15.2,6.06635214954162));
#206906=CARTESIAN_POINT('Ctrl Pts',(8.7832163332847,15.2,6.06928628678283));
#206907=CARTESIAN_POINT('Ctrl Pts',(8.78576967778803,15.2,6.07224624637696));
#206908=CARTESIAN_POINT('Ctrl Pts',(8.7888336910807,15.2,6.07579819776084));
#206909=CARTESIAN_POINT('Ctrl Pts',(8.79191355052904,15.2,6.07938733029834));
#206910=CARTESIAN_POINT('Ctrl Pts',(8.79500869074992,15.2,6.08301353149992));
#206911=CARTESIAN_POINT('Ctrl Pts',(8.79758797436103,15.2,6.08603536594437));
#206912=CARTESIAN_POINT('Ctrl Pts',(8.80017786915547,15.2,6.08908294014436));
#206913=CARTESIAN_POINT('Ctrl Pts',(8.80277805047492,15.2,6.09215618569992));
#206914=CARTESIAN_POINT('Ctrl Pts',(8.80589826794488,15.2,6.09584408023259));
#206915=CARTESIAN_POINT('Ctrl Pts',(8.80903330020322,15.2,6.09956894344534));
#206916=CARTESIAN_POINT('Ctrl Pts',(8.8121825957453,15.2,6.10333065591111));
#206917=CARTESIAN_POINT('Ctrl Pts',(8.81480700879237,15.2,6.10646541641316));
#206918=CARTESIAN_POINT('Ctrl Pts',(8.81744132895533,15.2,6.10962576611528));
#206919=CARTESIAN_POINT('Ctrl Pts',(8.82008524034373,15.2,6.11281163805839));
#206920=CARTESIAN_POINT('Ctrl Pts',(8.82272915173212,15.2,6.11599751000151));
#206921=CARTESIAN_POINT('Ctrl Pts',(8.82538265723187,15.2,6.11920890214527));
#206922=CARTESIAN_POINT('Ctrl Pts',(8.82804544605083,15.2,6.12244574825506));
#206923=CARTESIAN_POINT('Ctrl Pts',(8.83017567722211,15.2,6.12503522528401));
#206924=CARTESIAN_POINT('Ctrl Pts',(8.83231185069209,15.2,6.12764099153853));
#206925=CARTESIAN_POINT('Ctrl Pts',(8.83445381002743,15.2,6.13026301214715));
#206926=CARTESIAN_POINT('Ctrl Pts',(8.83659576907094,15.2,6.13288503239852));
#206927=CARTESIAN_POINT('Ctrl Pts',(8.83874351484201,15.2,6.13552330723169));
#206928=CARTESIAN_POINT('Ctrl Pts',(8.84089689183227,15.2,6.1381778012914));
#206929=CARTESIAN_POINT('Ctrl Pts',(8.84358861329014,15.2,6.14149591913729));
#206930=CARTESIAN_POINT('Ctrl Pts',(8.8462891356399,15.2,6.14483937880884));
#206931=CARTESIAN_POINT('Ctrl Pts',(8.84899816105614,15.2,6.1482081124881));
#206932=CARTESIAN_POINT('Ctrl Pts',(8.85116538150725,15.2,6.15090309957838));
#206933=CARTESIAN_POINT('Ctrl Pts',(8.8533380425436,15.2,6.15361426078727));
#206934=CARTESIAN_POINT('Ctrl Pts',(8.85551599654933,15.2,6.15634156262911));
#206935=CARTESIAN_POINT('Ctrl Pts',(8.85769395025832,15.2,6.15906886409935));
#206936=CARTESIAN_POINT('Ctrl Pts',(8.85987719475863,15.2,6.16181230492056));
#206937=CARTESIAN_POINT('Ctrl Pts',(8.86206558307941,15.2,6.16457184908281));
#206938=CARTESIAN_POINT('Ctrl Pts',(8.86425397169834,15.2,6.16733139362106));
#206939=CARTESIAN_POINT('Ctrl Pts',(8.8664475039929,15.2,6.17010704278621));
#206940=CARTESIAN_POINT('Ctrl Pts',(8.86864603244637,15.2,6.17289876049496));
#206941=CARTESIAN_POINT('Ctrl Pts',(8.87084456060029,15.2,6.17569047782334));
#206942=CARTESIAN_POINT('Ctrl Pts',(8.87304808295569,15.2,6.17849826241198));
#206943=CARTESIAN_POINT('Ctrl Pts',(8.87525645866284,15.2,6.18132208126526));
#206944=CARTESIAN_POINT('Ctrl Pts',(8.87746483467088,15.2,6.18414590050328));
#206945=CARTESIAN_POINT('Ctrl Pts',(8.879678060549,15.2,6.1869857517213));
#206946=CARTESIAN_POINT('Ctrl Pts',(8.88189599444795,15.2,6.18984160076687));
#206947=CARTESIAN_POINT('Ctrl Pts',(8.88411392804472,15.2,6.19269744942335));
#206948=CARTESIAN_POINT('Ctrl Pts',(8.88633656892387,15.2,6.19556929469327));
#206949=CARTESIAN_POINT('Ctrl Pts',(8.88856377518578,15.2,6.1984571020111));
#206950=CARTESIAN_POINT('Ctrl Pts',(8.89079098175113,15.2,6.20134490972241));
#206951=CARTESIAN_POINT('Ctrl Pts',(8.89302275239719,15.2,6.20424867866005));
#206952=CARTESIAN_POINT('Ctrl Pts',(8.89525894841812,15.2,6.20716837377692));
#206953=CARTESIAN_POINT('Ctrl Pts',(8.89749514413435,15.2,6.21008806849597));
#206954=CARTESIAN_POINT('Ctrl Pts',(8.89973576467797,15.2,6.21302368932974));
#206955=CARTESIAN_POINT('Ctrl Pts',(8.90198067038289,15.2,6.21597519880903));
#206956=CARTESIAN_POINT('Ctrl Pts',(8.90422557639367,15.2,6.21892670869046));
#206957=CARTESIAN_POINT('Ctrl Pts',(8.90647476742156,15.2,6.22189410903455));
#206958=CARTESIAN_POINT('Ctrl Pts',(8.9087281067666,15.2,6.22487736347492));
#206959=CARTESIAN_POINT('Ctrl Pts',(8.91098144611163,15.2,6.22786061791528));
#206960=CARTESIAN_POINT('Ctrl Pts',(8.91323893364324,15.2,6.23085972637972));
#206961=CARTESIAN_POINT('Ctrl Pts',(8.91550043237802,15.2,6.23387465226788));
#206962=CARTESIAN_POINT('Ctrl Pts',(8.91945805470169,15.2,6.23915077195598));
#206963=CARTESIAN_POINT('Ctrl Pts',(8.92342796201238,15.2,6.24447533789665));
#206964=CARTESIAN_POINT('Ctrl Pts',(8.92740943459731,15.2,6.24984814974075));
#206965=CARTESIAN_POINT('Ctrl Pts',(8.92968456205439,15.2,6.25291832829594));
#206966=CARTESIAN_POINT('Ctrl Pts',(8.93196346525637,15.2,6.25600426303358));
#206967=CARTESIAN_POINT('Ctrl Pts',(8.93424601393656,15.2,6.25910591620363));
#206968=CARTESIAN_POINT('Ctrl Pts',(8.93652856230575,15.2,6.26220756895108));
#206969=CARTESIAN_POINT('Ctrl Pts',(8.93881475505471,15.2,6.26532494099083));
#206970=CARTESIAN_POINT('Ctrl Pts',(8.94110446092603,15.2,6.26845799577872));
#206971=CARTESIAN_POINT('Ctrl Pts',(8.94396659349916,15.2,6.27237431458373));
#206972=CARTESIAN_POINT('Ctrl Pts',(8.94683421543458,15.2,6.27631513700315));
#206973=CARTESIAN_POINT('Ctrl Pts',(8.94970707383708,15.2,6.28028039318241));
#206974=CARTESIAN_POINT('Ctrl Pts',(8.95200536068434,15.2,6.28345259829872));
#206975=CARTESIAN_POINT('Ctrl Pts',(8.95430699953477,15.2,6.28664044093633));
#206976=CARTESIAN_POINT('Ctrl Pts',(8.95661186043839,15.2,6.28984388477862));
#206977=CARTESIAN_POINT('Ctrl Pts',(8.95891672102797,15.2,6.29304732818445));
#206978=CARTESIAN_POINT('Ctrl Pts',(8.96122480600498,15.2,6.29626637326537));
#206979=CARTESIAN_POINT('Ctrl Pts',(8.96353598793125,15.2,6.29950098277232));
#206980=CARTESIAN_POINT('Ctrl Pts',(8.96584717017242,15.2,6.30273559271998));
#206981=CARTESIAN_POINT('Ctrl Pts',(8.96816144901848,15.2,6.30598576745194));
#206982=CARTESIAN_POINT('Ctrl Pts',(8.97047869792273,15.2,6.30925147124204));
#206983=CARTESIAN_POINT('Ctrl Pts',(8.97395457096337,15.2,6.31415002648222));
#206984=CARTESIAN_POINT('Ctrl Pts',(8.97743713109518,15.2,6.31908351863633));
#206985=CARTESIAN_POINT('Ctrl Pts',(8.98092595605148,15.2,6.3240518297043));
#206986=CARTESIAN_POINT('Ctrl Pts',(8.98383331028737,15.2,6.32819208907803));
#206987=CARTESIAN_POINT('Ctrl Pts',(8.98674501732613,15.2,6.33235652534406));
#206988=CARTESIAN_POINT('Ctrl Pts',(8.98966083732594,15.2,6.33654506742614));
#206989=CARTESIAN_POINT('Ctrl Pts',(8.9919934934529,15.2,6.33989590127442));
#206990=CARTESIAN_POINT('Ctrl Pts',(8.9943287804142,15.2,6.34326216385));
#206991=CARTESIAN_POINT('Ctrl Pts',(8.99666658004752,15.2,6.34664381848238));
#206992=CARTESIAN_POINT('Ctrl Pts',(8.99900437936231,15.2,6.35002547265401));
#206993=CARTESIAN_POINT('Ctrl Pts',(9.00134469007511,15.2,6.3534225174483));
#206994=CARTESIAN_POINT('Ctrl Pts',(9.00368739205011,15.2,6.35683491744611));
#206995=CARTESIAN_POINT('Ctrl Pts',(9.0072014454914,15.2,6.36195351814023));
#206996=CARTESIAN_POINT('Ctrl Pts',(9.01072088114167,15.2,6.36710666826365));
#206997=CARTESIAN_POINT('Ctrl Pts',(9.01424529666743,15.2,6.37229424204872));
#206998=CARTESIAN_POINT('Ctrl Pts',(9.0165949066978,15.2,6.37575262410089));
#206999=CARTESIAN_POINT('Ctrl Pts',(9.01894673218841,15.2,6.37922630720309));
#207000=CARTESIAN_POINT('Ctrl Pts',(9.02130065350667,15.2,6.38271525198922));
#207001=CARTESIAN_POINT('Ctrl Pts',(9.02365457514564,15.2,6.38620419725072));
#207002=CARTESIAN_POINT('Ctrl Pts',(9.02601059384287,15.2,6.38970840671256));
#207003=CARTESIAN_POINT('Ctrl Pts',(9.02836859469381,15.2,6.39322784185036));
#207004=CARTESIAN_POINT('Ctrl Pts',(9.03072659522346,15.2,6.39674727650864));
#207005=CARTESIAN_POINT('Ctrl Pts',(9.0330865766612,15.2,6.40028193766774));
#207006=CARTESIAN_POINT('Ctrl Pts',(9.03544842402354,15.2,6.40383178770987));
#207007=CARTESIAN_POINT('Ctrl Pts',(9.03840073346781,15.2,6.40826910062526));
#207008=CARTESIAN_POINT('Ctrl Pts',(9.041355960696,15.2,6.41273014772717));
#207009=CARTESIAN_POINT('Ctrl Pts',(9.04431388251499,15.2,6.41721485628915));
#207010=CARTESIAN_POINT('Ctrl Pts',(9.04668022009914,15.2,6.42080262333426));
#207011=CARTESIAN_POINT('Ctrl Pts',(9.04904828155528,15.2,6.42440553269552));
#207012=CARTESIAN_POINT('Ctrl Pts',(9.05141795462904,15.2,6.42802354861647));
#207013=CARTESIAN_POINT('Ctrl Pts',(9.05378762737993,15.2,6.43164156404447));
#207014=CARTESIAN_POINT('Ctrl Pts',(9.05615891412505,15.2,6.43527468624827));
#207015=CARTESIAN_POINT('Ctrl Pts',(9.05853170076431,15.2,6.4389228768935));
#207016=CARTESIAN_POINT('Ctrl Pts',(9.06090448772687,15.2,6.44257106803579));
#207017=CARTESIAN_POINT('Ctrl Pts',(9.06327877612417,15.2,6.446234329276));
#207018=CARTESIAN_POINT('Ctrl Pts',(9.06565445459468,15.2,6.44991262255042));
#207019=CARTESIAN_POINT('Ctrl Pts',(9.06803013274149,15.2,6.45359091532368));
#207020=CARTESIAN_POINT('Ctrl Pts',(9.07040720007505,15.2,6.45728423930107));
#207021=CARTESIAN_POINT('Ctrl Pts',(9.07278555004719,15.2,6.46099255866358));
#207022=CARTESIAN_POINT('Ctrl Pts',(9.07516390034338,15.2,6.46470087853134));
#207023=CARTESIAN_POINT('Ctrl Pts',(9.07754353145642,15.2,6.46842419401763));
#207024=CARTESIAN_POINT('Ctrl Pts',(9.07992433575292,15.2,6.47216246655567));
#207025=CARTESIAN_POINT('Ctrl Pts',(9.08230513972502,15.2,6.47590073858438));
#207026=CARTESIAN_POINT('Ctrl Pts',(9.08468711627447,15.2,6.47965396804934));
#207027=CARTESIAN_POINT('Ctrl Pts',(9.08707015842082,15.2,6.48342211942823));
#207028=CARTESIAN_POINT('Ctrl Pts',(9.08945320089187,15.2,6.48719027132053));
#207029=CARTESIAN_POINT('Ctrl Pts',(9.09183730800098,15.2,6.49097334369148));
#207030=CARTESIAN_POINT('Ctrl Pts',(9.0942223761866,15.2,6.49477129834389));
#207031=CARTESIAN_POINT('Ctrl Pts',(9.09660744404725,15.2,6.49856925247883));
#207032=CARTESIAN_POINT('Ctrl Pts',(9.09899346924379,15.2,6.50238209023299));
#207033=CARTESIAN_POINT('Ctrl Pts',(9.10138034915968,15.2,6.50620977414077));
#207034=CARTESIAN_POINT('Ctrl Pts',(9.10317050950312,15.2,6.50908053772351));
#207035=CARTESIAN_POINT('Ctrl Pts',(9.1049611482967,15.2,6.51195965227528));
#207036=CARTESIAN_POINT('Ctrl Pts',(9.1067522251404,15.2,6.51484710186274));
#207037=CARTESIAN_POINT('Ctrl Pts',(9.10914032705637,15.2,6.51869703377174));
#207038=CARTESIAN_POINT('Ctrl Pts',(9.11152920296059,15.2,6.52256178386632));
#207039=CARTESIAN_POINT('Ctrl Pts',(9.11391875099831,15.2,6.52644131395562));
#207040=CARTESIAN_POINT('Ctrl Pts',(9.115710912108,15.2,6.52935096165473));
#207041=CARTESIAN_POINT('Ctrl Pts',(9.11750345090304,15.2,6.53226892380484));
#207042=CARTESIAN_POINT('Ctrl Pts',(9.11929632354619,15.2,6.5351951839061));
#207043=CARTESIAN_POINT('Ctrl Pts',(9.12108919618934,15.2,6.53812144400736));
#207044=CARTESIAN_POINT('Ctrl Pts',(9.12288240300749,15.2,6.54105600244977));
#207045=CARTESIAN_POINT('Ctrl Pts',(9.12467590110896,15.2,6.54399884263339));
#207046=CARTESIAN_POINT('Ctrl Pts',(9.12766506472,15.2,6.54890357645096));
#207047=CARTESIAN_POINT('Ctrl Pts',(9.13065503501453,15.2,6.55383131959625));
#207048=CARTESIAN_POINT('Ctrl Pts',(9.13364561717778,15.2,6.55878199442531));
#207049=CARTESIAN_POINT('Ctrl Pts',(9.13543996641054,15.2,6.56175239921482));
#207050=CARTESIAN_POINT('Ctrl Pts',(9.13723453567392,15.2,6.5647310602751));
#207051=CARTESIAN_POINT('Ctrl Pts',(9.13902928131702,15.2,6.56771796183212));
#207052=CARTESIAN_POINT('Ctrl Pts',(9.14142227572519,15.2,6.57170049760323));
#207053=CARTESIAN_POINT('Ctrl Pts',(9.14381558548893,15.2,6.57569768209795));
#207054=CARTESIAN_POINT('Ctrl Pts',(9.14620911000829,15.2,6.57970947798327));
#207055=CARTESIAN_POINT('Ctrl Pts',(9.14800425323474,15.2,6.58271832462396));
#207056=CARTESIAN_POINT('Ctrl Pts',(9.14979951736951,15.2,6.5857353910143));
#207057=CARTESIAN_POINT('Ctrl Pts',(9.15159486105425,15.2,6.58876065969531));
#207058=CARTESIAN_POINT('Ctrl Pts',(9.15398865285136,15.2,6.59279435163639));
#207059=CARTESIAN_POINT('Ctrl Pts',(9.15638258609726,15.2,6.59684262756945));
#207060=CARTESIAN_POINT('Ctrl Pts',(9.15877656134733,15.2,6.60090545010622));
#207061=CARTESIAN_POINT('Ctrl Pts',(9.16057204262179,15.2,6.60395256673202));
#207062=CARTESIAN_POINT('Ctrl Pts',(9.16236754751089,15.2,6.60700786371125));
#207063=CARTESIAN_POINT('Ctrl Pts',(9.16416303565399,15.2,6.61007132735065));
#207064=CARTESIAN_POINT('Ctrl Pts',(9.16595852379709,15.2,6.61313479099006));
#207065=CARTESIAN_POINT('Ctrl Pts',(9.16775399481517,15.2,6.6162064217618));
#207066=CARTESIAN_POINT('Ctrl Pts',(9.16954940704161,15.2,6.61928620148326));
#207067=CARTESIAN_POINT('Ctrl Pts',(9.17134481926806,15.2,6.62236598120472));
#207068=CARTESIAN_POINT('Ctrl Pts',(9.17314017406947,15.2,6.62545391225912));
#207069=CARTESIAN_POINT('Ctrl Pts',(9.17493542929593,15.2,6.62854997639593));
#207070=CARTESIAN_POINT('Ctrl Pts',(9.17732910314862,15.2,6.63267806228663));
#207071=CARTESIAN_POINT('Ctrl Pts',(9.17972260233739,15.2,6.63682060874297));
#207072=CARTESIAN_POINT('Ctrl Pts',(9.18211582891226,15.2,6.64097757858157));
#207073=CARTESIAN_POINT('Ctrl Pts',(9.18391074868036,15.2,6.64409530567733));
#207074=CARTESIAN_POINT('Ctrl Pts',(9.18570551635863,15.2,6.64722114565239));
#207075=CARTESIAN_POINT('Ctrl Pts',(9.18750009155158,15.2,6.65035508271944));
#207076=CARTESIAN_POINT('Ctrl Pts',(9.18929466674451,15.2,6.65348901978649));
#207077=CARTESIAN_POINT('Ctrl Pts',(9.19108904918869,15.2,6.65663105373059));
#207078=CARTESIAN_POINT('Ctrl Pts',(9.19288319846499,15.2,6.65978116875541));
#207079=CARTESIAN_POINT('Ctrl Pts',(9.19467734774129,15.2,6.66293128378023));
#207080=CARTESIAN_POINT('Ctrl Pts',(9.19647126461958,15.2,6.66608947908735));
#207081=CARTESIAN_POINT('Ctrl Pts',(9.19826490976277,15.2,6.66925573967994));
#207082=CARTESIAN_POINT('Ctrl Pts',(9.20065643683758,15.2,6.67347742085352));
#207083=CARTESIAN_POINT('Ctrl Pts',(9.20304747945122,15.2,6.67771343940939));
#207084=CARTESIAN_POINT('Ctrl Pts',(9.20543794597036,15.2,6.6819637578642));
#207085=CARTESIAN_POINT('Ctrl Pts',(9.2078284121638,15.2,6.6862140757399));
#207086=CARTESIAN_POINT('Ctrl Pts',(9.21021830142914,15.2,6.6904786925747));
#207087=CARTESIAN_POINT('Ctrl Pts',(9.21260752168658,15.2,6.69475757260411));
#207088=CARTESIAN_POINT('Ctrl Pts',(9.21559404725254,15.2,6.70010617307812));
#207089=CARTESIAN_POINT('Ctrl Pts',(9.21857952549361,15.2,6.70547705586522));
#207090=CARTESIAN_POINT('Ctrl Pts',(9.2215637793131,15.2,6.71087014794735));
#207091=CARTESIAN_POINT('Ctrl Pts',(9.22335433153973,15.2,6.71410600307905));
#207092=CARTESIAN_POINT('Ctrl Pts',(9.22514444317476,15.2,6.71734985464361));
#207093=CARTESIAN_POINT('Ctrl Pts',(9.22693407685981,15.2,6.72060168527437));
#207094=CARTESIAN_POINT('Ctrl Pts',(9.22872371086996,15.2,6.72385351649587));
#207095=CARTESIAN_POINT('Ctrl Pts',(9.23051286589665,15.2,6.7271133272363));
#207096=CARTESIAN_POINT('Ctrl Pts',(9.23230150436487,15.2,6.73038110096231));
#207097=CARTESIAN_POINT('Ctrl Pts',(9.23468635511427,15.2,6.73473813160759));
#207098=CARTESIAN_POINT('Ctrl Pts',(9.23707028553785,15.2,6.73910932001612));
#207099=CARTESIAN_POINT('Ctrl Pts',(9.239453204465,15.2,6.74349462528861));
#207100=CARTESIAN_POINT('Ctrl Pts',(9.24124039374151,15.2,6.74678360439236));
#207101=CARTESIAN_POINT('Ctrl Pts',(9.2430270137201,15.2,6.75008052497727));
#207102=CARTESIAN_POINT('Ctrl Pts',(9.24481303053026,15.2,6.75338537164817));
#207103=CARTESIAN_POINT('Ctrl Pts',(9.24778972532201,15.2,6.75889344963311));
#207104=CARTESIAN_POINT('Ctrl Pts',(9.25076475131095,15.2,6.76442354774921));
#207105=CARTESIAN_POINT('Ctrl Pts',(9.25373792408882,15.2,6.76997558788695));
#207106=CARTESIAN_POINT('Ctrl Pts',(9.2567110968667,15.2,6.77552762802469));
#207107=CARTESIAN_POINT('Ctrl Pts',(9.25968240391261,15.2,6.78110160259929));
#207108=CARTESIAN_POINT('Ctrl Pts',(9.262651666565,15.2,6.78669743630521));
#207109=CARTESIAN_POINT('Ctrl Pts',(9.26562092921739,15.2,6.79229327001113));
#207110=CARTESIAN_POINT('Ctrl Pts',(9.2685881416477,15.2,6.79791096716016));
#207111=CARTESIAN_POINT('Ctrl Pts',(9.27155330199994,15.2,6.80355049599999));
#207112=CARTESIAN_POINT('Ctrl Pts',(8.56667970899995,12.2,5.85257411499998));
#207113=CARTESIAN_POINT('Ctrl Pts',(8.5680628930964,12.2,5.85370502577855));
#207114=CARTESIAN_POINT('Ctrl Pts',(8.5694869244067,12.2,5.85487627485597));
#207115=CARTESIAN_POINT('Ctrl Pts',(8.5709506523979,12.2,5.85608775314224));
#207116=CARTESIAN_POINT('Ctrl Pts',(8.57242143922536,12.2,5.85730507378917));
#207117=CARTESIAN_POINT('Ctrl Pts',(8.57393230443574,12.2,5.85856301214596));
#207118=CARTESIAN_POINT('Ctrl Pts',(8.57548210843323,12.2,5.85986145286728));
#207119=CARTESIAN_POINT('Ctrl Pts',(8.57703191228994,12.2,5.86115989347067));
#207120=CARTESIAN_POINT('Ctrl Pts',(8.57862065432565,12.2,5.8624988373167));
#207121=CARTESIAN_POINT('Ctrl Pts',(8.58024722826654,12.2,5.86387816976658));
#207122=CARTESIAN_POINT('Ctrl Pts',(8.58187380220742,12.2,5.86525750221645));
#207123=CARTESIAN_POINT('Ctrl Pts',(8.58353820816439,12.2,5.86667722297458));
#207124=CARTESIAN_POINT('Ctrl Pts',(8.58523937135207,12.2,5.86813722032544));
#207125=CARTESIAN_POINT('Ctrl Pts',(8.58694053469429,12.2,5.86959721780893));
#207126=CARTESIAN_POINT('Ctrl Pts',(8.58867845563581,12.2,5.87109748993948));
#207127=CARTESIAN_POINT('Ctrl Pts',(8.59045208798488,12.2,5.87263792444283));
#207128=CARTESIAN_POINT('Ctrl Pts',(8.59252132548382,12.2,5.87443509782017));
#207129=CARTESIAN_POINT('Ctrl Pts',(8.59463917073834,12.2,5.87628693691257));
#207130=CARTESIAN_POINT('Ctrl Pts',(8.59680401336214,12.2,5.87819326040028));
#207131=CARTESIAN_POINT('Ctrl Pts',(8.59865959297066,12.2,5.87982725215201));
#207132=CARTESIAN_POINT('Ctrl Pts',(8.60054970122744,12.2,5.88150127369895));
#207133=CARTESIAN_POINT('Ctrl Pts',(8.60247335675124,12.2,5.88321521321174));
#207134=CARTESIAN_POINT('Ctrl Pts',(8.6043970121003,12.2,5.88492915256886));
#207135=CARTESIAN_POINT('Ctrl Pts',(8.60635421133066,12.2,5.88668300813268));
#207136=CARTESIAN_POINT('Ctrl Pts',(8.60834399976748,12.2,5.88847666749242));
#207137=CARTESIAN_POINT('Ctrl Pts',(8.61033378820429,12.2,5.89027032685214));
#207138=CARTESIAN_POINT('Ctrl Pts',(8.61235616229743,12.2,5.89210379097614));
#207139=CARTESIAN_POINT('Ctrl Pts',(8.61441019188808,12.2,5.89397694365633));
#207140=CARTESIAN_POINT('Ctrl Pts',(8.6164642216653,12.2,5.89585009650669));
#207141=CARTESIAN_POINT('Ctrl Pts',(8.61854990577146,12.2,5.89776294282028));
#207142=CARTESIAN_POINT('Ctrl Pts',(8.62066633380559,12.2,5.89971536542941));
#207143=CARTESIAN_POINT('Ctrl Pts',(8.62278276164747,12.2,5.90166778786119));
#207144=CARTESIAN_POINT('Ctrl Pts',(8.62492993542981,12.2,5.9036597878579));
#207145=CARTESIAN_POINT('Ctrl Pts',(8.627106966352,12.2,5.90569125236913));
#207146=CARTESIAN_POINT('Ctrl Pts',(8.62928399727419,12.2,5.90772271688036));
#207147=CARTESIAN_POINT('Ctrl Pts',(8.63149088542733,12.2,5.90979364605512));
#207148=CARTESIAN_POINT('Ctrl Pts',(8.63372676734483,12.2,5.91190392739341));
#207149=CARTESIAN_POINT('Ctrl Pts',(8.63596264926232,12.2,5.91401420873169));
#207150=CARTESIAN_POINT('Ctrl Pts',(8.63822752414355,12.2,5.91616384011022));
#207151=CARTESIAN_POINT('Ctrl Pts',(8.64052054897496,12.2,5.91835271052801));
#207152=CARTESIAN_POINT('Ctrl Pts',(8.64281357401468,12.2,5.92054158114462));
#207153=CARTESIAN_POINT('Ctrl Pts',(8.64513474718216,12.2,5.92276968904004));
#207154=CARTESIAN_POINT('Ctrl Pts',(8.64748324564467,12.2,5.92503692258198));
#207155=CARTESIAN_POINT('Ctrl Pts',(8.64983174389386,12.2,5.92730415591797));
#207156=CARTESIAN_POINT('Ctrl Pts',(8.65220756771584,12.2,5.92961051408416));
#207157=CARTESIAN_POINT('Ctrl Pts',(8.65460991187741,12.2,5.93195588258059));
#207158=CARTESIAN_POINT('Ctrl Pts',(8.65701225603898,12.2,5.93430125107701));
#207159=CARTESIAN_POINT('Ctrl Pts',(8.65944111983161,12.2,5.93668563184312));
#207160=CARTESIAN_POINT('Ctrl Pts',(8.66189571899069,12.2,5.93910890925246));
#207161=CARTESIAN_POINT('Ctrl Pts',(8.66435031837273,12.2,5.9415321868819));
#207162=CARTESIAN_POINT('Ctrl Pts',(8.66683065253225,12.2,5.94399436288172));
#207163=CARTESIAN_POINT('Ctrl Pts',(8.66933595116988,12.2,5.94649532068638));
#207164=CARTESIAN_POINT('Ctrl Pts',(8.67225879923911,12.2,5.94941310445107));
#207165=CARTESIAN_POINT('Ctrl Pts',(8.67521562943652,12.2,5.95238367869775));
#207166=CARTESIAN_POINT('Ctrl Pts',(8.67820524826226,12.2,5.95540685999247));
#207167=CARTESIAN_POINT('Ctrl Pts',(8.68076777898359,12.2,5.95799815854772));
#207168=CARTESIAN_POINT('Ctrl Pts',(8.68335440181564,12.2,5.96062810723174));
#207169=CARTESIAN_POINT('Ctrl Pts',(8.68596438262558,12.2,5.96329659187885));
#207170=CARTESIAN_POINT('Ctrl Pts',(8.68857436319844,12.2,5.96596507628358));
#207171=CARTESIAN_POINT('Ctrl Pts',(8.69120770284151,12.2,5.96867209749437));
#207172=CARTESIAN_POINT('Ctrl Pts',(8.69386368550703,12.2,5.97141753899034));
#207173=CARTESIAN_POINT('Ctrl Pts',(8.69651966817254,12.2,5.9741629804863));
#207174=CARTESIAN_POINT('Ctrl Pts',(8.69919829322183,12.2,5.97694684462246));
#207175=CARTESIAN_POINT('Ctrl Pts',(8.70189885895555,12.2,5.97976901493398));
#207176=CARTESIAN_POINT('Ctrl Pts',(8.70459942493458,12.2,5.98259118550184));
#207177=CARTESIAN_POINT('Ctrl Pts',(8.70732193266089,12.2,5.98545166274211));
#207178=CARTESIAN_POINT('Ctrl Pts',(8.71006569578205,12.2,5.98835033154709));
#207179=CARTESIAN_POINT('Ctrl Pts',(8.71235216492507,12.2,5.99076588875293));
#207180=CARTESIAN_POINT('Ctrl Pts',(8.71465339369052,12.2,5.99320796962066));
#207181=CARTESIAN_POINT('Ctrl Pts',(8.7169689935528,12.2,5.99567650358115));
#207182=CARTESIAN_POINT('Ctrl Pts',(8.71928459341506,12.2,5.99814503754163));
#207183=CARTESIAN_POINT('Ctrl Pts',(8.72161456367202,12.2,6.00064002790533));
#207184=CARTESIAN_POINT('Ctrl Pts',(8.72395852200651,12.2,6.00316140658807));
#207185=CARTESIAN_POINT('Ctrl Pts',(8.72677127190572,12.2,6.0061870608974));
#207186=CARTESIAN_POINT('Ctrl Pts',(8.72960416329157,12.2,6.00925071275516));
#207187=CARTESIAN_POINT('Ctrl Pts',(8.73245654618878,12.2,6.01235225089412));
#207188=CARTESIAN_POINT('Ctrl Pts',(8.73483353202283,12.2,6.01493686610382));
#207189=CARTESIAN_POINT('Ctrl Pts',(8.7372240554676,12.2,6.01754778784338));
#207190=CARTESIAN_POINT('Ctrl Pts',(8.73962774394052,12.2,6.02018495145588));
#207191=CARTESIAN_POINT('Ctrl Pts',(8.74203143241346,12.2,6.02282211506838));
#207192=CARTESIAN_POINT('Ctrl Pts',(8.74444828873749,12.2,6.02548551968159));
#207193=CARTESIAN_POINT('Ctrl Pts',(8.74687794754034,12.2,6.02817509780391));
#207194=CARTESIAN_POINT('Ctrl Pts',(8.74930760634317,12.2,6.03086467592622));
#207195=CARTESIAN_POINT('Ctrl Pts',(8.75175007054779,12.2,6.03358042787311));
#207196=CARTESIAN_POINT('Ctrl Pts',(8.75420497985435,12.2,6.03632228662523));
#207197=CARTESIAN_POINT('Ctrl Pts',(8.75665988916092,12.2,6.03906414537735));
#207198=CARTESIAN_POINT('Ctrl Pts',(8.75912724439545,12.2,6.04183210994103));
#207199=CARTESIAN_POINT('Ctrl Pts',(8.7616066938409,12.2,6.04462611362372));
#207200=CARTESIAN_POINT('Ctrl Pts',(8.76408614301609,12.2,6.04742011700186));
#207201=CARTESIAN_POINT('Ctrl Pts',(8.76657768737967,12.2,6.05024015992893));
#207202=CARTESIAN_POINT('Ctrl Pts',(8.76908098043915,12.2,6.05308617343601));
#207203=CARTESIAN_POINT('Ctrl Pts',(8.77158427377151,12.2,6.05593218725329));
#207204=CARTESIAN_POINT('Ctrl Pts',(8.7740993143315,12.2,6.05880417218411));
#207205=CARTESIAN_POINT('Ctrl Pts',(8.77662576217779,12.2,6.06170206086255));
#207206=CARTESIAN_POINT('Ctrl Pts',(8.77965749975856,12.2,6.06517952746619));
#207207=CARTESIAN_POINT('Ctrl Pts',(8.78270566421705,12.2,6.06869429467042));
#207208=CARTESIAN_POINT('Ctrl Pts',(8.78576967778803,12.2,6.07224624637696));
#207209=CARTESIAN_POINT('Ctrl Pts',(8.78832302229136,12.2,6.07520620597107));
#207210=CARTESIAN_POINT('Ctrl Pts',(8.79088737165252,12.2,6.07819198621395));
#207211=CARTESIAN_POINT('Ctrl Pts',(8.79346239707007,12.2,6.08120352086885));
#207212=CARTESIAN_POINT('Ctrl Pts',(8.79603742248763,12.2,6.08421505552374));
#207213=CARTESIAN_POINT('Ctrl Pts',(8.79862312544976,12.2,6.08725234545957));
#207214=CARTESIAN_POINT('Ctrl Pts',(8.80121917913115,12.2,6.09031531997557));
#207215=CARTESIAN_POINT('Ctrl Pts',(8.80381523281255,12.2,6.09337829449155));
#207216=CARTESIAN_POINT('Ctrl Pts',(8.80642163805244,12.2,6.09646695510517));
#207217=CARTESIAN_POINT('Ctrl Pts',(8.80903807590049,12.2,6.09958123219062));
#207218=CARTESIAN_POINT('Ctrl Pts',(8.81165451346335,12.2,6.1026955089366));
#207219=CARTESIAN_POINT('Ctrl Pts',(8.81428098302658,12.2,6.10583540448858));
#207220=CARTESIAN_POINT('Ctrl Pts',(8.81691717065511,12.2,6.10900084712756));
#207221=CARTESIAN_POINT('Ctrl Pts',(8.81955335857098,12.2,6.11216629011157));
#207222=CARTESIAN_POINT('Ctrl Pts',(8.82219926320895,12.2,6.11535728324798));
#207223=CARTESIAN_POINT('Ctrl Pts',(8.82485457536094,12.2,6.11857375532921));
#207224=CARTESIAN_POINT('Ctrl Pts',(8.8269788251983,12.2,6.12114693313444));
#207225=CARTESIAN_POINT('Ctrl Pts',(8.82910909550858,12.2,6.12373641928392));
#207226=CARTESIAN_POINT('Ctrl Pts',(8.83124522996804,12.2,6.12634217649336));
#207227=CARTESIAN_POINT('Ctrl Pts',(8.83338136413645,12.2,6.12894793334777));
#207228=CARTESIAN_POINT('Ctrl Pts',(8.83552336201105,12.2,6.13156996253314));
#207229=CARTESIAN_POINT('Ctrl Pts',(8.83767106889044,12.2,6.13420822859357));
#207230=CARTESIAN_POINT('Ctrl Pts',(8.83981877606245,12.2,6.13684649501346));
#207231=CARTESIAN_POINT('Ctrl Pts',(8.84197219170171,12.2,6.1395009982877));
#207232=CARTESIAN_POINT('Ctrl Pts',(8.84413116354159,12.2,6.14217170276659));
#207233=CARTESIAN_POINT('Ctrl Pts',(8.84629013538147,12.2,6.14484240724548));
#207234=CARTESIAN_POINT('Ctrl Pts',(8.84845466336088,12.2,6.14752931335402));
#207235=CARTESIAN_POINT('Ctrl Pts',(8.85062459464638,12.2,6.15023238572522));
#207236=CARTESIAN_POINT('Ctrl Pts',(8.85279452563623,12.2,6.15293545772814));
#207237=CARTESIAN_POINT('Ctrl Pts',(8.85496986128625,12.2,6.15565469528987));
#207238=CARTESIAN_POINT('Ctrl Pts',(8.85715045150677,12.2,6.15839006402306));
#207239=CARTESIAN_POINT('Ctrl Pts',(8.85933104202439,12.2,6.16112543312895));
#207240=CARTESIAN_POINT('Ctrl Pts',(8.86151688553822,12.2,6.16387693239996));
#207241=CARTESIAN_POINT('Ctrl Pts',(8.86370783732481,12.2,6.16664452688576));
#207242=CARTESIAN_POINT('Ctrl Pts',(8.86589878881288,12.2,6.16941212099449));
#207243=CARTESIAN_POINT('Ctrl Pts',(8.86809484621139,12.2,6.17219581145388));
#207244=CARTESIAN_POINT('Ctrl Pts',(8.87029586258671,12.2,6.17499556027953));
#207245=CARTESIAN_POINT('Ctrl Pts',(8.8724968792619,12.2,6.17779530948664));
#207246=CARTESIAN_POINT('Ctrl Pts',(8.87470285595884,12.2,6.18061111846928));
#207247=CARTESIAN_POINT('Ctrl Pts',(8.87691364857909,12.2,6.18344295221093));
#207248=CARTESIAN_POINT('Ctrl Pts',(8.87912444089812,12.2,6.18627478556674));
#207249=CARTESIAN_POINT('Ctrl Pts',(8.88134004649194,12.2,6.18912264098444));
#207250=CARTESIAN_POINT('Ctrl Pts',(8.88356032481013,12.2,6.19198648574929));
#207251=CARTESIAN_POINT('Ctrl Pts',(8.88578060343083,12.2,6.19485033090434));
#207252=CARTESIAN_POINT('Ctrl Pts',(8.88800555441322,12.2,6.19773016469463));
#207253=CARTESIAN_POINT('Ctrl Pts',(8.8902350339239,12.2,6.20062595052014));
#207254=CARTESIAN_POINT('Ctrl Pts',(8.89246451313081,12.2,6.2035217359511));
#207255=CARTESIAN_POINT('Ctrl Pts',(8.8946985230356,12.2,6.20643347485579));
#207256=CARTESIAN_POINT('Ctrl Pts',(8.89693692274181,12.2,6.20936112981685));
#207257=CARTESIAN_POINT('Ctrl Pts',(8.899175322753,12.2,6.2122887851768));
#207258=CARTESIAN_POINT('Ctrl Pts',(8.90141811167205,12.2,6.21523235789914));
#207259=CARTESIAN_POINT('Ctrl Pts',(8.90366515168366,12.2,6.21819181045034));
#207260=CARTESIAN_POINT('Ctrl Pts',(8.90591219138912,12.2,6.22115126259831));
#207261=CARTESIAN_POINT('Ctrl Pts',(8.90816348194653,12.2,6.22412659708759));
#207262=CARTESIAN_POINT('Ctrl Pts',(8.91041888637284,12.2,6.22711777578587));
#207263=CARTESIAN_POINT('Ctrl Pts',(8.91267429110643,12.2,6.23010895489169));
#207264=CARTESIAN_POINT('Ctrl Pts',(8.91493380991504,12.2,6.23311597829012));
#207265=CARTESIAN_POINT('Ctrl Pts',(8.91719730599314,12.2,6.23613881146865));
#207266=CARTESIAN_POINT('Ctrl Pts',(8.91946080176284,12.2,6.23916164423531));
#207267=CARTESIAN_POINT('Ctrl Pts',(8.92172827502853,12.2,6.24220028622684));
#207268=CARTESIAN_POINT('Ctrl Pts',(8.92399959212024,12.2,6.24525470147553));
#207269=CARTESIAN_POINT('Ctrl Pts',(8.92627090952141,12.2,6.2483091171404));
#207270=CARTESIAN_POINT('Ctrl Pts',(8.92854607080627,12.2,6.25137930404005));
#207271=CARTESIAN_POINT('Ctrl Pts',(8.9308249415416,12.2,6.25446522970826));
#207272=CARTESIAN_POINT('Ctrl Pts',(8.93310381227694,12.2,6.25755115537647));
#207273=CARTESIAN_POINT('Ctrl Pts',(8.93538639374878,12.2,6.26065281755481));
#207274=CARTESIAN_POINT('Ctrl Pts',(8.93767255387372,12.2,6.26377018072629));
#207275=CARTESIAN_POINT('Ctrl Pts',(8.94053025356266,12.2,6.26766688405352));
#207276=CARTESIAN_POINT('Ctrl Pts',(8.94339354409894,12.2,6.2715881192048));
#207277=CARTESIAN_POINT('Ctrl Pts',(8.94626217288305,12.2,6.27553381800883));
#207278=CARTESIAN_POINT('Ctrl Pts',(8.94855707628554,12.2,6.27869037756814));
#207279=CARTESIAN_POINT('Ctrl Pts',(8.95085539533558,12.2,6.2818625912456));
#207280=CARTESIAN_POINT('Ctrl Pts',(8.9531570020166,12.2,6.28505042447492));
#207281=CARTESIAN_POINT('Ctrl Pts',(8.95545860869761,12.2,6.28823825770425));
#207282=CARTESIAN_POINT('Ctrl Pts',(8.95776350095119,12.2,6.29144171089366));
#207283=CARTESIAN_POINT('Ctrl Pts',(8.96007155441063,12.2,6.29466074729291));
#207284=CARTESIAN_POINT('Ctrl Pts',(8.9623796075556,12.2,6.29787978325357));
#207285=CARTESIAN_POINT('Ctrl Pts',(8.9646908211576,12.2,6.3011144013626));
#207286=CARTESIAN_POINT('Ctrl Pts',(8.96700506825669,12.2,6.30436456672271));
#207287=CARTESIAN_POINT('Ctrl Pts',(8.9693193156711,12.2,6.30761473252566));
#207288=CARTESIAN_POINT('Ctrl Pts',(8.97163659534144,12.2,6.31088044563656));
#207289=CARTESIAN_POINT('Ctrl Pts',(8.97395678491262,12.2,6.31416166876141));
#207290=CARTESIAN_POINT('Ctrl Pts',(8.97627697416767,12.2,6.3174428914392));
#207291=CARTESIAN_POINT('Ctrl Pts',(8.97860007285292,12.2,6.32073962247608));
#207292=CARTESIAN_POINT('Ctrl Pts',(8.98092595605148,12.2,6.3240518297043));
#207293=CARTESIAN_POINT('Ctrl Pts',(8.98383331028737,12.2,6.32819208907803));
#207294=CARTESIAN_POINT('Ctrl Pts',(8.98674501732613,12.2,6.33235652534406));
#207295=CARTESIAN_POINT('Ctrl Pts',(8.98966083732594,12.2,6.33654506742614));
#207296=CARTESIAN_POINT('Ctrl Pts',(8.9919934934529,12.2,6.33989590127442));
#207297=CARTESIAN_POINT('Ctrl Pts',(8.9943287804142,12.2,6.34326216385));
#207298=CARTESIAN_POINT('Ctrl Pts',(8.99666658004752,12.2,6.34664381848238));
#207299=CARTESIAN_POINT('Ctrl Pts',(8.99900437936231,12.2,6.35002547265401));
#207300=CARTESIAN_POINT('Ctrl Pts',(9.00134469007511,12.2,6.3534225174483));
#207301=CARTESIAN_POINT('Ctrl Pts',(9.00368739205011,12.2,6.35683491744611));
#207302=CARTESIAN_POINT('Ctrl Pts',(9.00661576975825,12.2,6.36110041779207));
#207303=CARTESIAN_POINT('Ctrl Pts',(9.00954788422482,12.2,6.365389910897));
#207304=CARTESIAN_POINT('Ctrl Pts',(9.01248350505796,12.2,6.36970332374297));
#207305=CARTESIAN_POINT('Ctrl Pts',(9.01483200185247,12.2,6.37315405420781));
#207306=CARTESIAN_POINT('Ctrl Pts',(9.0171827412343,12.2,6.37662009405408));
#207307=CARTESIAN_POINT('Ctrl Pts',(9.01953560759136,12.2,6.38010140603017));
#207308=CARTESIAN_POINT('Ctrl Pts',(9.02188847362786,12.2,6.38358271753192));
#207309=CARTESIAN_POINT('Ctrl Pts',(9.02424346421952,12.2,6.38707930086493));
#207310=CARTESIAN_POINT('Ctrl Pts',(9.02660046674894,12.2,6.39059112018799));
#207311=CARTESIAN_POINT('Ctrl Pts',(9.02895746959952,12.2,6.39410293998952));
#207312=CARTESIAN_POINT('Ctrl Pts',(9.03131648285582,12.2,6.39762999524281));
#207313=CARTESIAN_POINT('Ctrl Pts',(9.03367739048463,12.2,6.40117224904799));
#207314=CARTESIAN_POINT('Ctrl Pts',(9.03603829779177,12.2,6.40471450237054));
#207315=CARTESIAN_POINT('Ctrl Pts',(9.03840109957382,12.2,6.40827195414927));
#207316=CARTESIAN_POINT('Ctrl Pts',(9.04076568366516,12.2,6.41184456775659));
#207317=CARTESIAN_POINT('Ctrl Pts',(9.04372141402097,12.2,6.41631033513083));
#207318=CARTESIAN_POINT('Ctrl Pts',(9.04667992812311,12.2,6.42079979267283));
#207319=CARTESIAN_POINT('Ctrl Pts',(9.0496410033313,12.2,6.42531286871324));
#207320=CARTESIAN_POINT('Ctrl Pts',(9.05200986362695,12.2,6.42892332974235));
#207321=CARTESIAN_POINT('Ctrl Pts',(9.05438036454227,12.2,6.43254890660384));
#207322=CARTESIAN_POINT('Ctrl Pts',(9.0567523942272,12.2,6.43618956058103));
#207323=CARTESIAN_POINT('Ctrl Pts',(9.05912442358895,12.2,6.43983021406218));
#207324=CARTESIAN_POINT('Ctrl Pts',(9.06149798078373,12.2,6.4434859459937));
#207325=CARTESIAN_POINT('Ctrl Pts',(9.06387295743032,12.2,6.44715672070901));
#207326=CARTESIAN_POINT('Ctrl Pts',(9.0662479344005,12.2,6.45082749592447));
#207327=CARTESIAN_POINT('Ctrl Pts',(9.06862432759243,12.2,6.45451331117771));
#207328=CARTESIAN_POINT('Ctrl Pts',(9.07100202994432,12.2,6.4582141316026));
#207329=CARTESIAN_POINT('Ctrl Pts',(9.0739741577222,12.2,6.46284015688159));
#207330=CARTESIAN_POINT('Ctrl Pts',(9.07694833054449,12.2,6.46748962613779));
#207331=CARTESIAN_POINT('Ctrl Pts',(9.07992433575292,12.2,6.47216246655567));
#207332=CARTESIAN_POINT('Ctrl Pts',(9.08230513972502,12.2,6.47590073858438));
#207333=CARTESIAN_POINT('Ctrl Pts',(9.08468711627447,12.2,6.47965396804934));
#207334=CARTESIAN_POINT('Ctrl Pts',(9.08707015842082,12.2,6.48342211942823));
#207335=CARTESIAN_POINT('Ctrl Pts',(9.08885744011176,12.2,6.48624823309075));
#207336=CARTESIAN_POINT('Ctrl Pts',(9.0906453206918,12.2,6.48908273891798));
#207337=CARTESIAN_POINT('Ctrl Pts',(9.09243375633506,12.2,6.49192562239685));
#207338=CARTESIAN_POINT('Ctrl Pts',(9.09422219230321,12.2,6.49476850639217));
#207339=CARTESIAN_POINT('Ctrl Pts',(9.09601118379659,12.2,6.49761976660661));
#207340=CARTESIAN_POINT('Ctrl Pts',(9.09780068339006,12.2,6.50047938869001));
#207341=CARTESIAN_POINT('Ctrl Pts',(9.09959018265844,12.2,6.50333901025391));
#207342=CARTESIAN_POINT('Ctrl Pts',(9.1013801934268,12.2,6.50620699270071));
#207343=CARTESIAN_POINT('Ctrl Pts',(9.10317066769511,12.2,6.50908332130526));
#207344=CARTESIAN_POINT('Ctrl Pts',(9.10555796661112,12.2,6.51291842593714));
#207345=CARTESIAN_POINT('Ctrl Pts',(9.10794609514599,12.2,6.51676836660781));
#207346=CARTESIAN_POINT('Ctrl Pts',(9.11033494540331,12.2,6.52063310737255));
#207347=CARTESIAN_POINT('Ctrl Pts',(9.11212658317767,12.2,6.52353166307774));
#207348=CARTESIAN_POINT('Ctrl Pts',(9.1139186280077,12.2,6.52643854310479));
#207349=CARTESIAN_POINT('Ctrl Pts',(9.11571103610919,12.2,6.52935373212275));
#207350=CARTESIAN_POINT('Ctrl Pts',(9.11750344453632,12.2,6.5322689216703));
#207351=CARTESIAN_POINT('Ctrl Pts',(9.11929621568019,12.2,6.53519241956185));
#207352=CARTESIAN_POINT('Ctrl Pts',(9.12108930664917,12.2,6.53812421065574));
#207353=CARTESIAN_POINT('Ctrl Pts',(9.12288239729241,12.2,6.54105600121702));
#207354=CARTESIAN_POINT('Ctrl Pts',(9.1246758080606,12.2,6.54399608367784));
#207355=CARTESIAN_POINT('Ctrl Pts',(9.12646949520379,12.2,6.54694444427977));
#207356=CARTESIAN_POINT('Ctrl Pts',(9.12826318234698,12.2,6.54989280488171));
#207357=CARTESIAN_POINT('Ctrl Pts',(9.13005714557528,12.2,6.55284944364684));
#207358=CARTESIAN_POINT('Ctrl Pts',(9.13185134322657,12.2,6.55581434276096));
#207359=CARTESIAN_POINT('Ctrl Pts',(9.13364554087788,12.2,6.55877924187508));
#207360=CARTESIAN_POINT('Ctrl Pts',(9.13543997338869,12.2,6.56175240214204));
#207361=CARTESIAN_POINT('Ctrl Pts',(9.13723459653998,12.2,6.56473380825556));
#207362=CARTESIAN_POINT('Ctrl Pts',(9.13902921969127,12.2,6.56771521436908));
#207363=CARTESIAN_POINT('Ctrl Pts',(9.14082403305286,12.2,6.5707048662996));
#207364=CARTESIAN_POINT('Ctrl Pts',(9.14261899623763,12.2,6.5737027473983));
#207365=CARTESIAN_POINT('Ctrl Pts',(9.14441395942239,12.2,6.57670062849698));
#207366=CARTESIAN_POINT('Ctrl Pts',(9.14620907240715,12.2,6.57970673878677));
#207367=CARTESIAN_POINT('Ctrl Pts',(9.14800429159192,12.2,6.5827210633428));
#207368=CARTESIAN_POINT('Ctrl Pts',(9.14979951110281,12.2,6.58573538844643));
#207369=CARTESIAN_POINT('Ctrl Pts',(9.15159483791374,12.2,6.58875792675239));
#207370=CARTESIAN_POINT('Ctrl Pts',(9.15339023038301,12.2,6.59178866336064));
#207371=CARTESIAN_POINT('Ctrl Pts',(9.15518562252611,12.2,6.5948193994183));
#207372=CARTESIAN_POINT('Ctrl Pts',(9.15698108007287,12.2,6.59785833348042));
#207373=CARTESIAN_POINT('Ctrl Pts',(9.15877656134733,12.2,6.60090545010622));
#207374=CARTESIAN_POINT('Ctrl Pts',(9.16057204262179,12.2,6.60395256673202));
#207375=CARTESIAN_POINT('Ctrl Pts',(9.16236754751089,12.2,6.60700786371125));
#207376=CARTESIAN_POINT('Ctrl Pts',(9.16416303565399,12.2,6.61007132735065));
#207377=CARTESIAN_POINT('Ctrl Pts',(9.16595852379709,12.2,6.61313479099006));
#207378=CARTESIAN_POINT('Ctrl Pts',(9.16775399481517,12.2,6.6162064217618));
#207379=CARTESIAN_POINT('Ctrl Pts',(9.16954940704161,12.2,6.61928620148326));
#207380=CARTESIAN_POINT('Ctrl Pts',(9.17134481926806,12.2,6.62236598120472));
#207381=CARTESIAN_POINT('Ctrl Pts',(9.17314017406947,12.2,6.62545391225912));
#207382=CARTESIAN_POINT('Ctrl Pts',(9.17493542929593,12.2,6.62854997639593));
#207383=CARTESIAN_POINT('Ctrl Pts',(9.17673068452238,12.2,6.63164604053273));
#207384=CARTESIAN_POINT('Ctrl Pts',(9.17852584127383,12.2,6.63475023873564));
#207385=CARTESIAN_POINT('Ctrl Pts',(9.18032085891697,12.2,6.63786255532979));
#207386=CARTESIAN_POINT('Ctrl Pts',(9.1821158768862,12.2,6.64097487248934));
#207387=CARTESIAN_POINT('Ctrl Pts',(9.18391075438039,12.2,6.64409530824285));
#207388=CARTESIAN_POINT('Ctrl Pts',(9.18570545384953,12.2,6.64722384594863));
#207389=CARTESIAN_POINT('Ctrl Pts',(9.18750015299263,12.2,6.65035238308606));
#207390=CARTESIAN_POINT('Ctrl Pts',(9.18929467312268,12.2,6.65348902278134));
#207391=CARTESIAN_POINT('Ctrl Pts',(9.1910889733971,12.2,6.6566337485751));
#207392=CARTESIAN_POINT('Ctrl Pts',(9.19348137365433,12.2,6.6608267161097));
#207393=CARTESIAN_POINT('Ctrl Pts',(9.1958733830138,12.2,6.66503405908155));
#207394=CARTESIAN_POINT('Ctrl Pts',(9.19826490976277,12.2,6.66925573967994));
#207395=CARTESIAN_POINT('Ctrl Pts',(9.20005855490596,12.2,6.67242200027252));
#207396=CARTESIAN_POINT('Ctrl Pts',(9.20185192720749,12.2,6.67559632588957));
#207397=CARTESIAN_POINT('Ctrl Pts',(9.20364498885073,12.2,6.67877870002285));
#207398=CARTESIAN_POINT('Ctrl Pts',(9.20603573792553,12.2,6.68302186591932));
#207399=CARTESIAN_POINT('Ctrl Pts',(9.20842593351326,12.2,6.68727934141724));
#207400=CARTESIAN_POINT('Ctrl Pts',(9.21081548270991,12.2,6.69155108800285));
#207401=CARTESIAN_POINT('Ctrl Pts',(9.21260764444461,12.2,6.69475489765105));
#207402=CARTESIAN_POINT('Ctrl Pts',(9.21439944307193,12.2,6.6979667358494));
#207403=CARTESIAN_POINT('Ctrl Pts',(9.21619083876499,12.2,6.70118658445535));
#207404=CARTESIAN_POINT('Ctrl Pts',(9.21798223445805,12.2,6.7044064330613));
#207405=CARTESIAN_POINT('Ctrl Pts',(9.21977322708646,12.2,6.70763429281564));
#207406=CARTESIAN_POINT('Ctrl Pts',(9.2215637793131,12.2,6.71087014794735));
#207407=CARTESIAN_POINT('Ctrl Pts',(9.22335433153973,12.2,6.71410600307905));
#207408=CARTESIAN_POINT('Ctrl Pts',(9.22514444317476,12.2,6.71734985464361));
#207409=CARTESIAN_POINT('Ctrl Pts',(9.22693407685981,12.2,6.72060168527437));
#207410=CARTESIAN_POINT('Ctrl Pts',(9.22872371086996,12.2,6.72385351649587));
#207411=CARTESIAN_POINT('Ctrl Pts',(9.23051286589665,12.2,6.7271133272363));
#207412=CARTESIAN_POINT('Ctrl Pts',(9.23230150436487,12.2,6.73038110096231));
#207413=CARTESIAN_POINT('Ctrl Pts',(9.23468635511427,12.2,6.73473813160759));
#207414=CARTESIAN_POINT('Ctrl Pts',(9.23707028553785,12.2,6.73910932001612));
#207415=CARTESIAN_POINT('Ctrl Pts',(9.239453204465,12.2,6.74349462528861));
#207416=CARTESIAN_POINT('Ctrl Pts',(9.24124039374151,12.2,6.74678360439236));
#207417=CARTESIAN_POINT('Ctrl Pts',(9.2430270137201,12.2,6.75008052497727));
#207418=CARTESIAN_POINT('Ctrl Pts',(9.24481303053026,12.2,6.75338537164817));
#207419=CARTESIAN_POINT('Ctrl Pts',(9.24659904734042,12.2,6.75669021831906));
#207420=CARTESIAN_POINT('Ctrl Pts',(9.24838446219229,12.2,6.76000299186442));
#207421=CARTESIAN_POINT('Ctrl Pts',(9.25016923787753,12.2,6.7633236759927));
#207422=CARTESIAN_POINT('Ctrl Pts',(9.25195401388701,12.2,6.76664436072422));
#207423=CARTESIAN_POINT('Ctrl Pts',(9.25373815067964,12.2,6.76997295755798));
#207424=CARTESIAN_POINT('Ctrl Pts',(9.25552160360541,12.2,6.77330944475229));
#207425=CARTESIAN_POINT('Ctrl Pts',(9.25789954029976,12.2,6.77775809333448));
#207426=CARTESIAN_POINT('Ctrl Pts',(9.26027625663727,12.2,6.78222076970644));
#207427=CARTESIAN_POINT('Ctrl Pts',(9.262651666565,12.2,6.78669743630522));
#207428=CARTESIAN_POINT('Ctrl Pts',(9.26562092921739,12.2,6.79229327001113));
#207429=CARTESIAN_POINT('Ctrl Pts',(9.2685881416477,12.2,6.79791096716016));
#207430=CARTESIAN_POINT('Ctrl Pts',(9.27155330199994,12.2,6.80355049599999));
#207431=CARTESIAN_POINT('Origin',(-5.66257110645729E-14,15.2,-1.77635683940025E-14));
#207432=CARTESIAN_POINT('',(7.6465751230011,15.2,7.01216898633437));
#207433=CARTESIAN_POINT('',(7.6465751230011,12.2,7.01216898633437));
#207434=CARTESIAN_POINT('',(7.64657512299994,15.2,7.01216898599998));
#207435=CARTESIAN_POINT('Origin',(-5.66257110645729E-14,12.2,-1.77635683940025E-14));
#207436=CARTESIAN_POINT('Origin',(-5.66257110645729E-14,15.2,-1.77635683940025E-14));
#207437=CARTESIAN_POINT('Origin',(-5.66257110645729E-14,15.2,-1.77635683940025E-14));
#207438=CARTESIAN_POINT('',(8.20893606999994,15.2,8.05377977099998));
#207439=CARTESIAN_POINT('',(7.93573928265107,15.2,8.32310290898369));
#207440=CARTESIAN_POINT('Origin',(-5.66257110645729E-14,15.2,-1.77635683940025E-14));
#207441=CARTESIAN_POINT('',(7.93573928265107,12.2,8.32310290898369));
#207442=CARTESIAN_POINT('',(7.93573928299995,15.2,8.32310290899999));
#207443=CARTESIAN_POINT('',(8.20893606999994,12.2,8.05377977099998));
#207444=CARTESIAN_POINT('Origin',(-5.66257110645729E-14,12.2,-1.77635683940025E-14));
#207445=CARTESIAN_POINT('',(8.20893606999994,15.2,8.05377977099998));
#207446=CARTESIAN_POINT('Ctrl Pts',(7.64657512299994,15.2,7.01216898699998));
#207447=CARTESIAN_POINT('Ctrl Pts',(7.64657512299994,11.6,7.01216898699998));
#207448=CARTESIAN_POINT('Ctrl Pts',(7.64669302599994,15.2,7.01229743699999));
#207449=CARTESIAN_POINT('Ctrl Pts',(7.64669302599994,11.6,7.01229743699999));
#207450=CARTESIAN_POINT('Ctrl Pts',(7.64693288599994,15.2,7.01255888399999));
#207451=CARTESIAN_POINT('Ctrl Pts',(7.64693288599994,11.6,7.01255888399999));
#207452=CARTESIAN_POINT('Ctrl Pts',(7.64729613399994,15.2,7.01295521799998));
#207453=CARTESIAN_POINT('Ctrl Pts',(7.64729613399994,11.6,7.01295521799998));
#207454=CARTESIAN_POINT('Ctrl Pts',(7.64778506499994,15.2,7.01348947999998));
#207455=CARTESIAN_POINT('Ctrl Pts',(7.64778506499994,11.6,7.01348947999998));
#207456=CARTESIAN_POINT('Ctrl Pts',(7.64840281599994,15.2,7.01416585899998));
#207457=CARTESIAN_POINT('Ctrl Pts',(7.64840281599994,11.6,7.01416585899998));
#207458=CARTESIAN_POINT('Ctrl Pts',(7.64902988999994,15.2,7.01485383099998));
#207459=CARTESIAN_POINT('Ctrl Pts',(7.64902988999994,11.6,7.01485383099998));
#207460=CARTESIAN_POINT('Ctrl Pts',(7.64966267399994,15.2,7.01554946999998));
#207461=CARTESIAN_POINT('Ctrl Pts',(7.64966267399994,11.6,7.01554946999998));
#207462=CARTESIAN_POINT('Ctrl Pts',(7.65030113899994,15.2,7.01625276699998));
#207463=CARTESIAN_POINT('Ctrl Pts',(7.65030113899994,11.6,7.01625276699998));
#207464=CARTESIAN_POINT('Ctrl Pts',(7.65094525299994,15.2,7.01696371599999));
#207465=CARTESIAN_POINT('Ctrl Pts',(7.65094525299994,11.6,7.01696371599999));
#207466=CARTESIAN_POINT('Ctrl Pts',(7.65159498499994,15.2,7.01768230799999));
#207467=CARTESIAN_POINT('Ctrl Pts',(7.65159498499994,11.6,7.01768230799999));
#207468=CARTESIAN_POINT('Ctrl Pts',(7.65225030199994,15.2,7.01840853699998));
#207469=CARTESIAN_POINT('Ctrl Pts',(7.65225030199994,11.6,7.01840853699998));
#207470=CARTESIAN_POINT('Ctrl Pts',(7.65291117499994,15.2,7.01914239299998));
#207471=CARTESIAN_POINT('Ctrl Pts',(7.65291117499994,11.6,7.01914239299998));
#207472=CARTESIAN_POINT('Ctrl Pts',(7.65357757199994,15.2,7.01988386999999));
#207473=CARTESIAN_POINT('Ctrl Pts',(7.65357757199994,11.6,7.01988386999999));
#207474=CARTESIAN_POINT('Ctrl Pts',(7.65424946499994,15.2,7.02063296099999));
#207475=CARTESIAN_POINT('Ctrl Pts',(7.65424946499994,11.6,7.02063296099999));
#207476=CARTESIAN_POINT('Ctrl Pts',(7.65492681899994,15.2,7.02138965599998));
#207477=CARTESIAN_POINT('Ctrl Pts',(7.65492681899994,11.6,7.02138965599998));
#207478=CARTESIAN_POINT('Ctrl Pts',(7.65560960699994,15.2,7.02215394999998));
#207479=CARTESIAN_POINT('Ctrl Pts',(7.65560960699994,11.6,7.02215394999998));
#207480=CARTESIAN_POINT('Ctrl Pts',(7.65629779899994,15.2,7.02292583299998));
#207481=CARTESIAN_POINT('Ctrl Pts',(7.65629779899994,11.6,7.02292583299998));
#207482=CARTESIAN_POINT('Ctrl Pts',(7.65699136199994,15.2,7.02370529999998));
#207483=CARTESIAN_POINT('Ctrl Pts',(7.65699136199994,11.6,7.02370529999998));
#207484=CARTESIAN_POINT('Ctrl Pts',(7.65769026799994,15.2,7.02449234199998));
#207485=CARTESIAN_POINT('Ctrl Pts',(7.65769026799994,11.6,7.02449234199998));
#207486=CARTESIAN_POINT('Ctrl Pts',(7.65839448899994,15.2,7.02528695099998));
#207487=CARTESIAN_POINT('Ctrl Pts',(7.65839448899994,11.6,7.02528695099998));
#207488=CARTESIAN_POINT('Ctrl Pts',(7.65910399199995,15.2,7.02608912199998));
#207489=CARTESIAN_POINT('Ctrl Pts',(7.65910399199995,11.6,7.02608912199998));
#207490=CARTESIAN_POINT('Ctrl Pts',(7.65981874999994,15.2,7.02689884499998));
#207491=CARTESIAN_POINT('Ctrl Pts',(7.65981874999994,11.6,7.02689884499998));
#207492=CARTESIAN_POINT('Ctrl Pts',(7.66053873199994,15.2,7.02771611299998));
#207493=CARTESIAN_POINT('Ctrl Pts',(7.66053873199994,11.6,7.02771611299998));
#207494=CARTESIAN_POINT('Ctrl Pts',(7.66126390999994,15.2,7.02854091999999));
#207495=CARTESIAN_POINT('Ctrl Pts',(7.66126390999994,11.6,7.02854091999999));
#207496=CARTESIAN_POINT('Ctrl Pts',(7.66199425499994,15.2,7.02937325699998));
#207497=CARTESIAN_POINT('Ctrl Pts',(7.66199425499994,11.6,7.02937325699998));
#207498=CARTESIAN_POINT('Ctrl Pts',(7.66272973699994,15.2,7.03021311899998));
#207499=CARTESIAN_POINT('Ctrl Pts',(7.66272973699994,11.6,7.03021311899998));
#207500=CARTESIAN_POINT('Ctrl Pts',(7.66347032799994,15.2,7.03106049599998));
#207501=CARTESIAN_POINT('Ctrl Pts',(7.66347032799994,11.6,7.03106049599998));
#207502=CARTESIAN_POINT('Ctrl Pts',(7.66421599899994,15.2,7.03191538099999));
#207503=CARTESIAN_POINT('Ctrl Pts',(7.66421599899994,11.6,7.03191538099999));
#207504=CARTESIAN_POINT('Ctrl Pts',(7.66496672199994,15.2,7.03277776899998));
#207505=CARTESIAN_POINT('Ctrl Pts',(7.66496672199994,11.6,7.03277776899998));
#207506=CARTESIAN_POINT('Ctrl Pts',(7.66572246899995,15.2,7.03364765099998));
#207507=CARTESIAN_POINT('Ctrl Pts',(7.66572246899995,11.6,7.03364765099998));
#207508=CARTESIAN_POINT('Ctrl Pts',(7.66648321099995,15.2,7.03452502099999));
#207509=CARTESIAN_POINT('Ctrl Pts',(7.66648321099995,11.6,7.03452502099999));
#207510=CARTESIAN_POINT('Ctrl Pts',(7.66724891999995,15.2,7.03540986999998));
#207511=CARTESIAN_POINT('Ctrl Pts',(7.66724891999995,11.6,7.03540986999998));
#207512=CARTESIAN_POINT('Ctrl Pts',(7.66801956799994,15.2,7.03630219099999));
#207513=CARTESIAN_POINT('Ctrl Pts',(7.66801956799994,11.6,7.03630219099999));
#207514=CARTESIAN_POINT('Ctrl Pts',(7.66879512799994,15.2,7.03720197899998));
#207515=CARTESIAN_POINT('Ctrl Pts',(7.66879512799994,11.6,7.03720197899998));
#207516=CARTESIAN_POINT('Ctrl Pts',(7.66957557199994,15.2,7.03810922399998));
#207517=CARTESIAN_POINT('Ctrl Pts',(7.66957557199994,11.6,7.03810922399998));
#207518=CARTESIAN_POINT('Ctrl Pts',(7.67036087199994,15.2,7.03902391999998));
#207519=CARTESIAN_POINT('Ctrl Pts',(7.67036087199994,11.6,7.03902391999998));
#207520=CARTESIAN_POINT('Ctrl Pts',(7.67115099999994,15.2,7.03994606099998));
#207521=CARTESIAN_POINT('Ctrl Pts',(7.67115099999994,11.6,7.03994606099998));
#207522=CARTESIAN_POINT('Ctrl Pts',(7.67194592999994,15.2,7.04087563799998));
#207523=CARTESIAN_POINT('Ctrl Pts',(7.67194592999994,11.6,7.04087563799998));
#207524=CARTESIAN_POINT('Ctrl Pts',(7.67274563399994,15.2,7.04181264599999));
#207525=CARTESIAN_POINT('Ctrl Pts',(7.67274563399994,11.6,7.04181264599999));
#207526=CARTESIAN_POINT('Ctrl Pts',(7.67355008499995,15.2,7.04275707599999));
#207527=CARTESIAN_POINT('Ctrl Pts',(7.67355008499995,11.6,7.04275707599999));
#207528=CARTESIAN_POINT('Ctrl Pts',(7.67435925699994,15.2,7.04370892199999));
#207529=CARTESIAN_POINT('Ctrl Pts',(7.67435925699994,11.6,7.04370892199999));
#207530=CARTESIAN_POINT('Ctrl Pts',(7.67517312199994,15.2,7.04466817699998));
#207531=CARTESIAN_POINT('Ctrl Pts',(7.67517312199994,11.6,7.04466817699998));
#207532=CARTESIAN_POINT('Ctrl Pts',(7.67599165499995,15.2,7.04563483399999));
#207533=CARTESIAN_POINT('Ctrl Pts',(7.67599165499995,11.6,7.04563483399999));
#207534=CARTESIAN_POINT('Ctrl Pts',(7.67681482699994,15.2,7.04660888499999));
#207535=CARTESIAN_POINT('Ctrl Pts',(7.67681482699994,11.6,7.04660888499999));
#207536=CARTESIAN_POINT('Ctrl Pts',(7.67764261399994,15.2,7.04759032499998));
#207537=CARTESIAN_POINT('Ctrl Pts',(7.67764261399994,11.6,7.04759032499998));
#207538=CARTESIAN_POINT('Ctrl Pts',(7.67847498699994,15.2,7.04857914399999));
#207539=CARTESIAN_POINT('Ctrl Pts',(7.67847498699994,11.6,7.04857914399999));
#207540=CARTESIAN_POINT('Ctrl Pts',(7.67931192299995,15.2,7.04957533799998));
#207541=CARTESIAN_POINT('Ctrl Pts',(7.67931192299995,11.6,7.04957533799998));
#207542=CARTESIAN_POINT('Ctrl Pts',(7.68015339199994,15.2,7.05057889899999));
#207543=CARTESIAN_POINT('Ctrl Pts',(7.68015339199994,11.6,7.05057889899999));
#207544=CARTESIAN_POINT('Ctrl Pts',(7.68099937299994,15.2,7.05158981999999));
#207545=CARTESIAN_POINT('Ctrl Pts',(7.68099937299994,11.6,7.05158981999999));
#207546=CARTESIAN_POINT('Ctrl Pts',(7.68184983599994,15.2,7.05260809399999));
#207547=CARTESIAN_POINT('Ctrl Pts',(7.68184983599994,11.6,7.05260809399999));
#207548=CARTESIAN_POINT('Ctrl Pts',(7.68270475699994,15.2,7.05363371399999));
#207549=CARTESIAN_POINT('Ctrl Pts',(7.68270475699994,11.6,7.05363371399999));
#207550=CARTESIAN_POINT('Ctrl Pts',(7.68356410999995,15.2,7.05466667399998));
#207551=CARTESIAN_POINT('Ctrl Pts',(7.68356410999995,11.6,7.05466667399998));
#207552=CARTESIAN_POINT('Ctrl Pts',(7.68442787099994,15.2,7.05570696599998));
#207553=CARTESIAN_POINT('Ctrl Pts',(7.68442787099994,11.6,7.05570696599998));
#207554=CARTESIAN_POINT('Ctrl Pts',(7.68529601099995,15.2,7.05675458499999));
#207555=CARTESIAN_POINT('Ctrl Pts',(7.68529601099995,11.6,7.05675458499999));
#207556=CARTESIAN_POINT('Ctrl Pts',(7.68616850899994,15.2,7.05780952199999));
#207557=CARTESIAN_POINT('Ctrl Pts',(7.68616850899994,11.6,7.05780952199999));
#207558=CARTESIAN_POINT('Ctrl Pts',(7.68704533799994,15.2,7.05887176999998));
#207559=CARTESIAN_POINT('Ctrl Pts',(7.68704533799994,11.6,7.05887176999998));
#207560=CARTESIAN_POINT('Ctrl Pts',(7.68792647099994,15.2,7.05994132599999));
#207561=CARTESIAN_POINT('Ctrl Pts',(7.68792647099994,11.6,7.05994132599999));
#207562=CARTESIAN_POINT('Ctrl Pts',(7.68881188699994,15.2,7.06101817899999));
#207563=CARTESIAN_POINT('Ctrl Pts',(7.68881188699994,11.6,7.06101817899999));
#207564=CARTESIAN_POINT('Ctrl Pts',(7.68970155799994,15.2,7.06210232399999));
#207565=CARTESIAN_POINT('Ctrl Pts',(7.68970155799994,11.6,7.06210232399999));
#207566=CARTESIAN_POINT('Ctrl Pts',(7.69059545999994,15.2,7.06319375399998));
#207567=CARTESIAN_POINT('Ctrl Pts',(7.69059545999994,11.6,7.06319375399998));
#207568=CARTESIAN_POINT('Ctrl Pts',(7.69149356799995,15.2,7.06429246399999));
#207569=CARTESIAN_POINT('Ctrl Pts',(7.69149356799995,11.6,7.06429246399999));
#207570=CARTESIAN_POINT('Ctrl Pts',(7.69239585999994,15.2,7.06539844399998));
#207571=CARTESIAN_POINT('Ctrl Pts',(7.69239585999994,11.6,7.06539844399998));
#207572=CARTESIAN_POINT('Ctrl Pts',(7.69330230899994,15.2,7.06651168999999));
#207573=CARTESIAN_POINT('Ctrl Pts',(7.69330230899994,11.6,7.06651168999999));
#207574=CARTESIAN_POINT('Ctrl Pts',(7.69421289099995,15.2,7.06763219399999));
#207575=CARTESIAN_POINT('Ctrl Pts',(7.69421289099995,11.6,7.06763219399999));
#207576=CARTESIAN_POINT('Ctrl Pts',(7.69512758299994,15.2,7.06875994999999));
#207577=CARTESIAN_POINT('Ctrl Pts',(7.69512758299994,11.6,7.06875994999999));
#207578=CARTESIAN_POINT('Ctrl Pts',(7.69604635999994,15.2,7.06989494999998));
#207579=CARTESIAN_POINT('Ctrl Pts',(7.69604635999994,11.6,7.06989494999998));
#207580=CARTESIAN_POINT('Ctrl Pts',(7.69696919799994,15.2,7.07103718999999));
#207581=CARTESIAN_POINT('Ctrl Pts',(7.69696919799994,11.6,7.07103718999999));
#207582=CARTESIAN_POINT('Ctrl Pts',(7.69789607399994,15.2,7.07218666199999));
#207583=CARTESIAN_POINT('Ctrl Pts',(7.69789607399994,11.6,7.07218666199999));
#207584=CARTESIAN_POINT('Ctrl Pts',(7.69882696299995,15.2,7.07334335899999));
#207585=CARTESIAN_POINT('Ctrl Pts',(7.69882696299995,11.6,7.07334335899999));
#207586=CARTESIAN_POINT('Ctrl Pts',(7.69976184199994,15.2,7.07450727399999));
#207587=CARTESIAN_POINT('Ctrl Pts',(7.69976184199994,11.6,7.07450727399999));
#207588=CARTESIAN_POINT('Ctrl Pts',(7.70070068699994,15.2,7.07567840199999));
#207589=CARTESIAN_POINT('Ctrl Pts',(7.70070068699994,11.6,7.07567840199999));
#207590=CARTESIAN_POINT('Ctrl Pts',(7.70164347599994,15.2,7.07685673499999));
#207591=CARTESIAN_POINT('Ctrl Pts',(7.70164347599994,11.6,7.07685673499999));
#207592=CARTESIAN_POINT('Ctrl Pts',(7.70259018299994,15.2,7.07804226699999));
#207593=CARTESIAN_POINT('Ctrl Pts',(7.70259018299994,11.6,7.07804226699999));
#207594=CARTESIAN_POINT('Ctrl Pts',(7.70354078799994,15.2,7.07923499199998));
#207595=CARTESIAN_POINT('Ctrl Pts',(7.70354078799994,11.6,7.07923499199998));
#207596=CARTESIAN_POINT('Ctrl Pts',(7.70449526399994,15.2,7.08043490399999));
#207597=CARTESIAN_POINT('Ctrl Pts',(7.70449526399994,11.6,7.08043490399999));
#207598=CARTESIAN_POINT('Ctrl Pts',(7.70545359099994,15.2,7.08164199399998));
#207599=CARTESIAN_POINT('Ctrl Pts',(7.70545359099994,11.6,7.08164199399998));
#207600=CARTESIAN_POINT('Ctrl Pts',(7.70641574499995,15.2,7.08285625699999));
#207601=CARTESIAN_POINT('Ctrl Pts',(7.70641574499995,11.6,7.08285625699999));
#207602=CARTESIAN_POINT('Ctrl Pts',(7.70738170299994,15.2,7.08407768799999));
#207603=CARTESIAN_POINT('Ctrl Pts',(7.70738170299994,11.6,7.08407768799999));
#207604=CARTESIAN_POINT('Ctrl Pts',(7.70835144199994,15.2,7.08530627799998));
#207605=CARTESIAN_POINT('Ctrl Pts',(7.70835144199994,11.6,7.08530627799998));
#207606=CARTESIAN_POINT('Ctrl Pts',(7.70932493799994,15.2,7.08654202199998));
#207607=CARTESIAN_POINT('Ctrl Pts',(7.70932493799994,11.6,7.08654202199998));
#207608=CARTESIAN_POINT('Ctrl Pts',(7.71030217199994,15.2,7.08778491299999));
#207609=CARTESIAN_POINT('Ctrl Pts',(7.71030217199994,11.6,7.08778491299999));
#207610=CARTESIAN_POINT('Ctrl Pts',(7.71128311799994,15.2,7.08903494499998));
#207611=CARTESIAN_POINT('Ctrl Pts',(7.71128311799994,11.6,7.08903494499998));
#207612=CARTESIAN_POINT('Ctrl Pts',(7.71226775599994,15.2,7.09029211199999));
#207613=CARTESIAN_POINT('Ctrl Pts',(7.71226775599994,11.6,7.09029211199999));
#207614=CARTESIAN_POINT('Ctrl Pts',(7.71325606199994,15.2,7.09155640599998));
#207615=CARTESIAN_POINT('Ctrl Pts',(7.71325606199994,11.6,7.09155640599998));
#207616=CARTESIAN_POINT('Ctrl Pts',(7.71424801399994,15.2,7.09282782199999));
#207617=CARTESIAN_POINT('Ctrl Pts',(7.71424801399994,11.6,7.09282782199999));
#207618=CARTESIAN_POINT('Ctrl Pts',(7.71524358999994,15.2,7.09410635399998));
#207619=CARTESIAN_POINT('Ctrl Pts',(7.71524358999994,11.6,7.09410635399998));
#207620=CARTESIAN_POINT('Ctrl Pts',(7.71624276799994,15.2,7.09539199399998));
#207621=CARTESIAN_POINT('Ctrl Pts',(7.71624276799994,11.6,7.09539199399998));
#207622=CARTESIAN_POINT('Ctrl Pts',(7.71724552699995,15.2,7.09668473599999));
#207623=CARTESIAN_POINT('Ctrl Pts',(7.71724552699995,11.6,7.09668473599999));
#207624=CARTESIAN_POINT('Ctrl Pts',(7.71825184399995,15.2,7.09798457599998));
#207625=CARTESIAN_POINT('Ctrl Pts',(7.71825184399995,11.6,7.09798457599998));
#207626=CARTESIAN_POINT('Ctrl Pts',(7.71926169599995,15.2,7.09929150499998));
#207627=CARTESIAN_POINT('Ctrl Pts',(7.71926169599995,11.6,7.09929150499998));
#207628=CARTESIAN_POINT('Ctrl Pts',(7.72027506399994,15.2,7.10060551799998));
#207629=CARTESIAN_POINT('Ctrl Pts',(7.72027506399994,11.6,7.10060551799998));
#207630=CARTESIAN_POINT('Ctrl Pts',(7.72129192499994,15.2,7.10192660699998));
#207631=CARTESIAN_POINT('Ctrl Pts',(7.72129192499994,11.6,7.10192660699998));
#207632=CARTESIAN_POINT('Ctrl Pts',(7.72231225799994,15.2,7.10325476899998));
#207633=CARTESIAN_POINT('Ctrl Pts',(7.72231225799994,11.6,7.10325476899998));
#207634=CARTESIAN_POINT('Ctrl Pts',(7.72333603899994,15.2,7.10458999399999));
#207635=CARTESIAN_POINT('Ctrl Pts',(7.72333603899994,11.6,7.10458999399999));
#207636=CARTESIAN_POINT('Ctrl Pts',(7.72436324999994,15.2,7.10593227899999));
#207637=CARTESIAN_POINT('Ctrl Pts',(7.72436324999994,11.6,7.10593227899999));
#207638=CARTESIAN_POINT('Ctrl Pts',(7.72539386899994,15.2,7.10728161499999));
#207639=CARTESIAN_POINT('Ctrl Pts',(7.72539386899994,11.6,7.10728161499999));
#207640=CARTESIAN_POINT('Ctrl Pts',(7.72642787299994,15.2,7.10863799699998));
#207641=CARTESIAN_POINT('Ctrl Pts',(7.72642787299994,11.6,7.10863799699998));
#207642=CARTESIAN_POINT('Ctrl Pts',(7.72746524199994,15.2,7.11000141999998));
#207643=CARTESIAN_POINT('Ctrl Pts',(7.72746524199994,11.6,7.11000141999998));
#207644=CARTESIAN_POINT('Ctrl Pts',(7.72850595599994,15.2,7.11137187599999));
#207645=CARTESIAN_POINT('Ctrl Pts',(7.72850595599994,11.6,7.11137187599999));
#207646=CARTESIAN_POINT('Ctrl Pts',(7.72954999199994,15.2,7.11274935899999));
#207647=CARTESIAN_POINT('Ctrl Pts',(7.72954999199994,11.6,7.11274935899999));
#207648=CARTESIAN_POINT('Ctrl Pts',(7.73059733099994,15.2,7.11413386299999));
#207649=CARTESIAN_POINT('Ctrl Pts',(7.73059733099994,11.6,7.11413386299999));
#207650=CARTESIAN_POINT('Ctrl Pts',(7.73164795099994,15.2,7.11552538199999));
#207651=CARTESIAN_POINT('Ctrl Pts',(7.73164795099994,11.6,7.11552538199999));
#207652=CARTESIAN_POINT('Ctrl Pts',(7.73270183099994,15.2,7.11692390999998));
#207653=CARTESIAN_POINT('Ctrl Pts',(7.73270183099994,11.6,7.11692390999998));
#207654=CARTESIAN_POINT('Ctrl Pts',(7.73375895099995,15.2,7.11832944099999));
#207655=CARTESIAN_POINT('Ctrl Pts',(7.73375895099995,11.6,7.11832944099999));
#207656=CARTESIAN_POINT('Ctrl Pts',(7.73481929099994,15.2,7.11974196899998));
#207657=CARTESIAN_POINT('Ctrl Pts',(7.73481929099994,11.6,7.11974196899998));
#207658=CARTESIAN_POINT('Ctrl Pts',(7.73588282999994,15.2,7.12116148599998));
#207659=CARTESIAN_POINT('Ctrl Pts',(7.73588282999994,11.6,7.12116148599998));
#207660=CARTESIAN_POINT('Ctrl Pts',(7.73694954799995,15.2,7.12258798699998));
#207661=CARTESIAN_POINT('Ctrl Pts',(7.73694954799995,11.6,7.12258798699998));
#207662=CARTESIAN_POINT('Ctrl Pts',(7.73801942299994,15.2,7.12402146799998));
#207663=CARTESIAN_POINT('Ctrl Pts',(7.73801942299994,11.6,7.12402146799998));
#207664=CARTESIAN_POINT('Ctrl Pts',(7.73909243699994,15.2,7.12546191899998));
#207665=CARTESIAN_POINT('Ctrl Pts',(7.73909243699994,11.6,7.12546191899998));
#207666=CARTESIAN_POINT('Ctrl Pts',(7.74016856799994,15.2,7.12690933699999));
#207667=CARTESIAN_POINT('Ctrl Pts',(7.74016856799994,11.6,7.12690933699999));
#207668=CARTESIAN_POINT('Ctrl Pts',(7.74124779699994,15.2,7.12836371399998));
#207669=CARTESIAN_POINT('Ctrl Pts',(7.74124779699994,11.6,7.12836371399998));
#207670=CARTESIAN_POINT('Ctrl Pts',(7.74233010399994,15.2,7.12982504499998));
#207671=CARTESIAN_POINT('Ctrl Pts',(7.74233010399994,11.6,7.12982504499998));
#207672=CARTESIAN_POINT('Ctrl Pts',(7.74341546799994,15.2,7.13129332399999));
#207673=CARTESIAN_POINT('Ctrl Pts',(7.74341546799994,11.6,7.13129332399999));
#207674=CARTESIAN_POINT('Ctrl Pts',(7.74450387099994,15.2,7.13276854399999));
#207675=CARTESIAN_POINT('Ctrl Pts',(7.74450387099994,11.6,7.13276854399999));
#207676=CARTESIAN_POINT('Ctrl Pts',(7.74559529099994,15.2,7.13425069899999));
#207677=CARTESIAN_POINT('Ctrl Pts',(7.74559529099994,11.6,7.13425069899999));
#207678=CARTESIAN_POINT('Ctrl Pts',(7.74668970999994,15.2,7.13573978499999));
#207679=CARTESIAN_POINT('Ctrl Pts',(7.74668970999994,11.6,7.13573978499999));
#207680=CARTESIAN_POINT('Ctrl Pts',(7.74778710799994,15.2,7.13723579299998));
#207681=CARTESIAN_POINT('Ctrl Pts',(7.74778710799994,11.6,7.13723579299998));
#207682=CARTESIAN_POINT('Ctrl Pts',(7.74888746499995,15.2,7.13873871999999));
#207683=CARTESIAN_POINT('Ctrl Pts',(7.74888746499995,11.6,7.13873871999999));
#207684=CARTESIAN_POINT('Ctrl Pts',(7.74999076099995,15.2,7.14024855699999));
#207685=CARTESIAN_POINT('Ctrl Pts',(7.74999076099995,11.6,7.14024855699999));
#207686=CARTESIAN_POINT('Ctrl Pts',(7.75109697799994,15.2,7.14176529899999));
#207687=CARTESIAN_POINT('Ctrl Pts',(7.75109697799994,11.6,7.14176529899999));
#207688=CARTESIAN_POINT('Ctrl Pts',(7.75220609499994,15.2,7.14328894099998));
#207689=CARTESIAN_POINT('Ctrl Pts',(7.75220609499994,11.6,7.14328894099998));
#207690=CARTESIAN_POINT('Ctrl Pts',(7.75331809499994,15.2,7.14481947699999));
#207691=CARTESIAN_POINT('Ctrl Pts',(7.75331809499994,11.6,7.14481947699999));
#207692=CARTESIAN_POINT('Ctrl Pts',(7.75443295699994,15.2,7.14635689999999));
#207693=CARTESIAN_POINT('Ctrl Pts',(7.75443295699994,11.6,7.14635689999999));
#207694=CARTESIAN_POINT('Ctrl Pts',(7.75555066199995,15.2,7.14790120399999));
#207695=CARTESIAN_POINT('Ctrl Pts',(7.75555066199995,11.6,7.14790120399999));
#207696=CARTESIAN_POINT('Ctrl Pts',(7.75667119099994,15.2,7.14945238399999));
#207697=CARTESIAN_POINT('Ctrl Pts',(7.75667119099994,11.6,7.14945238399999));
#207698=CARTESIAN_POINT('Ctrl Pts',(7.75779452599994,15.2,7.15101043399999));
#207699=CARTESIAN_POINT('Ctrl Pts',(7.75779452599994,11.6,7.15101043399999));
#207700=CARTESIAN_POINT('Ctrl Pts',(7.75892064599994,15.2,7.15257534699998));
#207701=CARTESIAN_POINT('Ctrl Pts',(7.75892064599994,11.6,7.15257534699998));
#207702=CARTESIAN_POINT('Ctrl Pts',(7.76004953399994,15.2,7.15414711799998));
#207703=CARTESIAN_POINT('Ctrl Pts',(7.76004953399994,11.6,7.15414711799998));
#207704=CARTESIAN_POINT('Ctrl Pts',(7.76118117099994,15.2,7.15572573999999));
#207705=CARTESIAN_POINT('Ctrl Pts',(7.76118117099994,11.6,7.15572573999999));
#207706=CARTESIAN_POINT('Ctrl Pts',(7.76231553799994,15.2,7.15731120699999));
#207707=CARTESIAN_POINT('Ctrl Pts',(7.76231553799994,11.6,7.15731120699999));
#207708=CARTESIAN_POINT('Ctrl Pts',(7.76345261599995,15.2,7.15890351599998));
#207709=CARTESIAN_POINT('Ctrl Pts',(7.76345261599995,11.6,7.15890351599998));
#207710=CARTESIAN_POINT('Ctrl Pts',(7.76459238699994,15.2,7.16050265899998));
#207711=CARTESIAN_POINT('Ctrl Pts',(7.76459238699994,11.6,7.16050265899998));
#207712=CARTESIAN_POINT('Ctrl Pts',(7.76573483199994,15.2,7.16210862899998));
#207713=CARTESIAN_POINT('Ctrl Pts',(7.76573483199994,11.6,7.16210862899998));
#207714=CARTESIAN_POINT('Ctrl Pts',(7.76687993199995,15.2,7.16372142099999));
#207715=CARTESIAN_POINT('Ctrl Pts',(7.76687993199995,11.6,7.16372142099999));
#207716=CARTESIAN_POINT('Ctrl Pts',(7.76802766899995,15.2,7.16534102999999));
#207717=CARTESIAN_POINT('Ctrl Pts',(7.76802766899995,11.6,7.16534102999999));
#207718=CARTESIAN_POINT('Ctrl Pts',(7.76917802599994,15.2,7.16696744899998));
#207719=CARTESIAN_POINT('Ctrl Pts',(7.76917802599994,11.6,7.16696744899998));
#207720=CARTESIAN_POINT('Ctrl Pts',(7.77033098399994,15.2,7.16860067399999));
#207721=CARTESIAN_POINT('Ctrl Pts',(7.77033098399994,11.6,7.16860067399999));
#207722=CARTESIAN_POINT('Ctrl Pts',(7.77148652399994,15.2,7.17024069699999));
#207723=CARTESIAN_POINT('Ctrl Pts',(7.77148652399994,11.6,7.17024069699999));
#207724=CARTESIAN_POINT('Ctrl Pts',(7.77264462799995,15.2,7.17188751199998));
#207725=CARTESIAN_POINT('Ctrl Pts',(7.77264462799995,11.6,7.17188751199998));
#207726=CARTESIAN_POINT('Ctrl Pts',(7.77380527899994,15.2,7.17354111599998));
#207727=CARTESIAN_POINT('Ctrl Pts',(7.77380527899994,11.6,7.17354111599998));
#207728=CARTESIAN_POINT('Ctrl Pts',(7.77496845899995,15.2,7.17520149999999));
#207729=CARTESIAN_POINT('Ctrl Pts',(7.77496845899995,11.6,7.17520149999999));
#207730=CARTESIAN_POINT('Ctrl Pts',(7.77613414799994,15.2,7.17686865999998));
#207731=CARTESIAN_POINT('Ctrl Pts',(7.77613414799994,11.6,7.17686865999998));
#207732=CARTESIAN_POINT('Ctrl Pts',(7.77730232999994,15.2,7.17854258899998));
#207733=CARTESIAN_POINT('Ctrl Pts',(7.77730232999994,11.6,7.17854258899998));
#207734=CARTESIAN_POINT('Ctrl Pts',(7.77847298599994,15.2,7.18022328399999));
#207735=CARTESIAN_POINT('Ctrl Pts',(7.77847298599994,11.6,7.18022328399999));
#207736=CARTESIAN_POINT('Ctrl Pts',(7.77964609999994,15.2,7.18191073499998));
#207737=CARTESIAN_POINT('Ctrl Pts',(7.77964609999994,11.6,7.18191073499998));
#207738=CARTESIAN_POINT('Ctrl Pts',(7.78082165299995,15.2,7.18360493899999));
#207739=CARTESIAN_POINT('Ctrl Pts',(7.78082165299995,11.6,7.18360493899999));
#207740=CARTESIAN_POINT('Ctrl Pts',(7.78199962799994,15.2,7.18530588799998));
#207741=CARTESIAN_POINT('Ctrl Pts',(7.78199962799994,11.6,7.18530588799998));
#207742=CARTESIAN_POINT('Ctrl Pts',(7.78318000599994,15.2,7.18701357999999));
#207743=CARTESIAN_POINT('Ctrl Pts',(7.78318000599994,11.6,7.18701357999999));
#207744=CARTESIAN_POINT('Ctrl Pts',(7.78436277199994,15.2,7.18872800599998));
#207745=CARTESIAN_POINT('Ctrl Pts',(7.78436277199994,11.6,7.18872800599998));
#207746=CARTESIAN_POINT('Ctrl Pts',(7.78554790599994,15.2,7.19044916099998));
#207747=CARTESIAN_POINT('Ctrl Pts',(7.78554790599994,11.6,7.19044916099998));
#207748=CARTESIAN_POINT('Ctrl Pts',(7.78673539199994,15.2,7.19217703999998));
#207749=CARTESIAN_POINT('Ctrl Pts',(7.78673539199994,11.6,7.19217703999998));
#207750=CARTESIAN_POINT('Ctrl Pts',(7.78792521299994,15.2,7.19391163699999));
#207751=CARTESIAN_POINT('Ctrl Pts',(7.78792521299994,11.6,7.19391163699999));
#207752=CARTESIAN_POINT('Ctrl Pts',(7.78911734999994,15.2,7.19565294599998));
#207753=CARTESIAN_POINT('Ctrl Pts',(7.78911734999994,11.6,7.19565294599998));
#207754=CARTESIAN_POINT('Ctrl Pts',(7.79031178799995,15.2,7.19740096099999));
#207755=CARTESIAN_POINT('Ctrl Pts',(7.79031178799995,11.6,7.19740096099999));
#207756=CARTESIAN_POINT('Ctrl Pts',(7.79150850799994,15.2,7.19915567599998));
#207757=CARTESIAN_POINT('Ctrl Pts',(7.79150850799994,11.6,7.19915567599998));
#207758=CARTESIAN_POINT('Ctrl Pts',(7.79270749399994,15.2,7.20091708699999));
#207759=CARTESIAN_POINT('Ctrl Pts',(7.79270749399994,11.6,7.20091708699999));
#207760=CARTESIAN_POINT('Ctrl Pts',(7.79390872899994,15.2,7.20268518699999));
#207761=CARTESIAN_POINT('Ctrl Pts',(7.79390872899994,11.6,7.20268518699999));
#207762=CARTESIAN_POINT('Ctrl Pts',(7.79511219599994,15.2,7.20445996999998));
#207763=CARTESIAN_POINT('Ctrl Pts',(7.79511219599994,11.6,7.20445996999998));
#207764=CARTESIAN_POINT('Ctrl Pts',(7.79631787699994,15.2,7.20624143099998));
#207765=CARTESIAN_POINT('Ctrl Pts',(7.79631787699994,11.6,7.20624143099998));
#207766=CARTESIAN_POINT('Ctrl Pts',(7.79752575599994,15.2,7.20802956399999));
#207767=CARTESIAN_POINT('Ctrl Pts',(7.79752575599994,11.6,7.20802956399999));
#207768=CARTESIAN_POINT('Ctrl Pts',(7.79873581599994,15.2,7.20982436299998));
#207769=CARTESIAN_POINT('Ctrl Pts',(7.79873581599994,11.6,7.20982436299998));
#207770=CARTESIAN_POINT('Ctrl Pts',(7.79994804099994,15.2,7.21162582399998));
#207771=CARTESIAN_POINT('Ctrl Pts',(7.79994804099994,11.6,7.21162582399998));
#207772=CARTESIAN_POINT('Ctrl Pts',(7.80116241299995,15.2,7.21343393899998));
#207773=CARTESIAN_POINT('Ctrl Pts',(7.80116241299995,11.6,7.21343393899998));
#207774=CARTESIAN_POINT('Ctrl Pts',(7.80237891699994,15.2,7.21524870399998));
#207775=CARTESIAN_POINT('Ctrl Pts',(7.80237891699994,11.6,7.21524870399998));
#207776=CARTESIAN_POINT('Ctrl Pts',(7.80359753599994,15.2,7.21707011199998));
#207777=CARTESIAN_POINT('Ctrl Pts',(7.80359753599994,11.6,7.21707011199998));
#207778=CARTESIAN_POINT('Ctrl Pts',(7.80481825099994,15.2,7.21889815899999));
#207779=CARTESIAN_POINT('Ctrl Pts',(7.80481825099994,11.6,7.21889815899999));
#207780=CARTESIAN_POINT('Ctrl Pts',(7.80604104899994,15.2,7.22073283799999));
#207781=CARTESIAN_POINT('Ctrl Pts',(7.80604104899994,11.6,7.22073283799999));
#207782=CARTESIAN_POINT('Ctrl Pts',(7.80726591199994,15.2,7.22257414399999));
#207783=CARTESIAN_POINT('Ctrl Pts',(7.80726591199994,11.6,7.22257414399999));
#207784=CARTESIAN_POINT('Ctrl Pts',(7.80849282299994,15.2,7.22442207199999));
#207785=CARTESIAN_POINT('Ctrl Pts',(7.80849282299994,11.6,7.22442207199999));
#207786=CARTESIAN_POINT('Ctrl Pts',(7.80972176699994,15.2,7.22627661499998));
#207787=CARTESIAN_POINT('Ctrl Pts',(7.80972176699994,11.6,7.22627661499998));
#207788=CARTESIAN_POINT('Ctrl Pts',(7.81095272699995,15.2,7.22813776799998));
#207789=CARTESIAN_POINT('Ctrl Pts',(7.81095272699995,11.6,7.22813776799998));
#207790=CARTESIAN_POINT('Ctrl Pts',(7.81218568699995,15.2,7.23000552499999));
#207791=CARTESIAN_POINT('Ctrl Pts',(7.81218568699995,11.6,7.23000552499999));
#207792=CARTESIAN_POINT('Ctrl Pts',(7.81342063099994,15.2,7.23187988099999));
#207793=CARTESIAN_POINT('Ctrl Pts',(7.81342063099994,11.6,7.23187988099999));
#207794=CARTESIAN_POINT('Ctrl Pts',(7.81465754299994,15.2,7.23376083099998));
#207795=CARTESIAN_POINT('Ctrl Pts',(7.81465754299994,11.6,7.23376083099998));
#207796=CARTESIAN_POINT('Ctrl Pts',(7.81589640599995,15.2,7.23564836699998));
#207797=CARTESIAN_POINT('Ctrl Pts',(7.81589640599995,11.6,7.23564836699998));
#207798=CARTESIAN_POINT('Ctrl Pts',(7.81713720499994,15.2,7.23754248699999));
#207799=CARTESIAN_POINT('Ctrl Pts',(7.81713720499994,11.6,7.23754248699999));
#207800=CARTESIAN_POINT('Ctrl Pts',(7.81837992399995,15.2,7.23944318299999));
#207801=CARTESIAN_POINT('Ctrl Pts',(7.81837992399995,11.6,7.23944318299999));
#207802=CARTESIAN_POINT('Ctrl Pts',(7.81962454699995,15.2,7.24135044899998));
#207803=CARTESIAN_POINT('Ctrl Pts',(7.81962454699995,11.6,7.24135044899998));
#207804=CARTESIAN_POINT('Ctrl Pts',(7.82087105799994,15.2,7.24326428099998));
#207805=CARTESIAN_POINT('Ctrl Pts',(7.82087105799994,11.6,7.24326428099998));
#207806=CARTESIAN_POINT('Ctrl Pts',(7.82211944199994,15.2,7.24518467399999));
#207807=CARTESIAN_POINT('Ctrl Pts',(7.82211944199994,11.6,7.24518467399999));
#207808=CARTESIAN_POINT('Ctrl Pts',(7.82336968099994,15.2,7.24711161999998));
#207809=CARTESIAN_POINT('Ctrl Pts',(7.82336968099994,11.6,7.24711161999998));
#207810=CARTESIAN_POINT('Ctrl Pts',(7.82462176299994,15.2,7.24904511499999));
#207811=CARTESIAN_POINT('Ctrl Pts',(7.82462176299994,11.6,7.24904511499999));
#207812=CARTESIAN_POINT('Ctrl Pts',(7.82587566799994,15.2,7.25098515199999));
#207813=CARTESIAN_POINT('Ctrl Pts',(7.82587566799994,11.6,7.25098515199999));
#207814=CARTESIAN_POINT('Ctrl Pts',(7.82713138399994,15.2,7.25293172799999));
#207815=CARTESIAN_POINT('Ctrl Pts',(7.82713138399994,11.6,7.25293172799999));
#207816=CARTESIAN_POINT('Ctrl Pts',(7.82838889399994,15.2,7.25488483599998));
#207817=CARTESIAN_POINT('Ctrl Pts',(7.82838889399994,11.6,7.25488483599998));
#207818=CARTESIAN_POINT('Ctrl Pts',(7.82964818299994,15.2,7.25684447099999));
#207819=CARTESIAN_POINT('Ctrl Pts',(7.82964818299994,11.6,7.25684447099999));
#207820=CARTESIAN_POINT('Ctrl Pts',(7.83090923499994,15.2,7.25881062599999));
#207821=CARTESIAN_POINT('Ctrl Pts',(7.83090923499994,11.6,7.25881062599999));
#207822=CARTESIAN_POINT('Ctrl Pts',(7.83217203599994,15.2,7.26078329699998));
#207823=CARTESIAN_POINT('Ctrl Pts',(7.83217203599994,11.6,7.26078329699998));
#207824=CARTESIAN_POINT('Ctrl Pts',(7.83343656799994,15.2,7.26276247899998));
#207825=CARTESIAN_POINT('Ctrl Pts',(7.83343656799994,11.6,7.26276247899998));
#207826=CARTESIAN_POINT('Ctrl Pts',(7.83470281799994,15.2,7.26474816499999));
#207827=CARTESIAN_POINT('Ctrl Pts',(7.83470281799994,11.6,7.26474816499999));
#207828=CARTESIAN_POINT('Ctrl Pts',(7.83597076999994,15.2,7.26674034999998));
#207829=CARTESIAN_POINT('Ctrl Pts',(7.83597076999994,11.6,7.26674034999998));
#207830=CARTESIAN_POINT('Ctrl Pts',(7.83724040899994,15.2,7.26873902899998));
#207831=CARTESIAN_POINT('Ctrl Pts',(7.83724040899994,11.6,7.26873902899998));
#207832=CARTESIAN_POINT('Ctrl Pts',(7.83851171999994,15.2,7.27074419599998));
#207833=CARTESIAN_POINT('Ctrl Pts',(7.83851171999994,11.6,7.27074419599998));
#207834=CARTESIAN_POINT('Ctrl Pts',(7.83978468599994,15.2,7.27275584499999));
#207835=CARTESIAN_POINT('Ctrl Pts',(7.83978468599994,11.6,7.27275584499999));
#207836=CARTESIAN_POINT('Ctrl Pts',(7.84105929599995,15.2,7.27477397199999));
#207837=CARTESIAN_POINT('Ctrl Pts',(7.84105929599995,11.6,7.27477397199999));
#207838=CARTESIAN_POINT('Ctrl Pts',(7.84233553099994,15.2,7.27679857099999));
#207839=CARTESIAN_POINT('Ctrl Pts',(7.84233553099994,11.6,7.27679857099999));
#207840=CARTESIAN_POINT('Ctrl Pts',(7.84361337799995,15.2,7.27882963499999));
#207841=CARTESIAN_POINT('Ctrl Pts',(7.84361337799995,11.6,7.27882963499999));
#207842=CARTESIAN_POINT('Ctrl Pts',(7.84489282199995,15.2,7.28086716099998));
#207843=CARTESIAN_POINT('Ctrl Pts',(7.84489282199995,11.6,7.28086716099998));
#207844=CARTESIAN_POINT('Ctrl Pts',(7.84617384799994,15.2,7.28291114199998));
#207845=CARTESIAN_POINT('Ctrl Pts',(7.84617384799994,11.6,7.28291114199998));
#207846=CARTESIAN_POINT('Ctrl Pts',(7.84745644099995,15.2,7.28496157299999));
#207847=CARTESIAN_POINT('Ctrl Pts',(7.84745644099995,11.6,7.28496157299999));
#207848=CARTESIAN_POINT('Ctrl Pts',(7.84874058699994,15.2,7.28701844899999));
#207849=CARTESIAN_POINT('Ctrl Pts',(7.84874058699994,11.6,7.28701844899999));
#207850=CARTESIAN_POINT('Ctrl Pts',(7.85002626999994,15.2,7.28908176299999));
#207851=CARTESIAN_POINT('Ctrl Pts',(7.85002626999994,11.6,7.28908176299999));
#207852=CARTESIAN_POINT('Ctrl Pts',(7.85131347599994,15.2,7.29115151199998));
#207853=CARTESIAN_POINT('Ctrl Pts',(7.85131347599994,11.6,7.29115151199998));
#207854=CARTESIAN_POINT('Ctrl Pts',(7.85260218999994,15.2,7.29322768799998));
#207855=CARTESIAN_POINT('Ctrl Pts',(7.85260218999994,11.6,7.29322768799998));
#207856=CARTESIAN_POINT('Ctrl Pts',(7.85389239799994,15.2,7.29531028699999));
#207857=CARTESIAN_POINT('Ctrl Pts',(7.85389239799994,11.6,7.29531028699999));
#207858=CARTESIAN_POINT('Ctrl Pts',(7.85518408499994,15.2,7.29739930399998));
#207859=CARTESIAN_POINT('Ctrl Pts',(7.85518408499994,11.6,7.29739930399998));
#207860=CARTESIAN_POINT('Ctrl Pts',(7.85647723799995,15.2,7.29949473199999));
#207861=CARTESIAN_POINT('Ctrl Pts',(7.85647723799995,11.6,7.29949473199999));
#207862=CARTESIAN_POINT('Ctrl Pts',(7.85777184099994,15.2,7.30159656799999));
#207863=CARTESIAN_POINT('Ctrl Pts',(7.85777184099994,11.6,7.30159656799999));
#207864=CARTESIAN_POINT('Ctrl Pts',(7.85906787899994,15.2,7.30370480499998));
#207865=CARTESIAN_POINT('Ctrl Pts',(7.85906787899994,11.6,7.30370480499998));
#207866=CARTESIAN_POINT('Ctrl Pts',(7.86036533899995,15.2,7.30581943799999));
#207867=CARTESIAN_POINT('Ctrl Pts',(7.86036533899995,11.6,7.30581943799999));
#207868=CARTESIAN_POINT('Ctrl Pts',(7.86166420599994,15.2,7.30794045999998));
#207869=CARTESIAN_POINT('Ctrl Pts',(7.86166420599994,11.6,7.30794045999998));
#207870=CARTESIAN_POINT('Ctrl Pts',(7.86296446599994,15.2,7.31006786799998));
#207871=CARTESIAN_POINT('Ctrl Pts',(7.86296446599994,11.6,7.31006786799998));
#207872=CARTESIAN_POINT('Ctrl Pts',(7.86426610499994,15.2,7.31220165499998));
#207873=CARTESIAN_POINT('Ctrl Pts',(7.86426610499994,11.6,7.31220165499998));
#207874=CARTESIAN_POINT('Ctrl Pts',(7.86556910799994,15.2,7.31434181699999));
#207875=CARTESIAN_POINT('Ctrl Pts',(7.86556910799994,11.6,7.31434181699999));
#207876=CARTESIAN_POINT('Ctrl Pts',(7.86687346199994,15.2,7.31648834799999));
#207877=CARTESIAN_POINT('Ctrl Pts',(7.86687346199994,11.6,7.31648834799999));
#207878=CARTESIAN_POINT('Ctrl Pts',(7.86817915099994,15.2,7.31864124199999));
#207879=CARTESIAN_POINT('Ctrl Pts',(7.86817915099994,11.6,7.31864124199999));
#207880=CARTESIAN_POINT('Ctrl Pts',(7.86948616399994,15.2,7.32080049499999));
#207881=CARTESIAN_POINT('Ctrl Pts',(7.86948616399994,11.6,7.32080049499999));
#207882=CARTESIAN_POINT('Ctrl Pts',(7.87079448499994,15.2,7.32296609999998));
#207883=CARTESIAN_POINT('Ctrl Pts',(7.87079448499994,11.6,7.32296609999998));
#207884=CARTESIAN_POINT('Ctrl Pts',(7.87210409899994,15.2,7.32513805299998));
#207885=CARTESIAN_POINT('Ctrl Pts',(7.87210409899994,11.6,7.32513805299998));
#207886=CARTESIAN_POINT('Ctrl Pts',(7.87341499399994,15.2,7.32731634799999));
#207887=CARTESIAN_POINT('Ctrl Pts',(7.87341499399994,11.6,7.32731634799999));
#207888=CARTESIAN_POINT('Ctrl Pts',(7.87472715499994,15.2,7.32950097999999));
#207889=CARTESIAN_POINT('Ctrl Pts',(7.87472715499994,11.6,7.32950097999999));
#207890=CARTESIAN_POINT('Ctrl Pts',(7.87604056899994,15.2,7.33169194399999));
#207891=CARTESIAN_POINT('Ctrl Pts',(7.87604056899994,11.6,7.33169194399999));
#207892=CARTESIAN_POINT('Ctrl Pts',(7.87735522199994,15.2,7.33388923399998));
#207893=CARTESIAN_POINT('Ctrl Pts',(7.87735522199994,11.6,7.33388923399998));
#207894=CARTESIAN_POINT('Ctrl Pts',(7.87867109999994,15.2,7.33609284399999));
#207895=CARTESIAN_POINT('Ctrl Pts',(7.87867109999994,11.6,7.33609284399999));
#207896=CARTESIAN_POINT('Ctrl Pts',(7.87998818899994,15.2,7.33830276999999));
#207897=CARTESIAN_POINT('Ctrl Pts',(7.87998818899994,11.6,7.33830276999999));
#207898=CARTESIAN_POINT('Ctrl Pts',(7.88130647599995,15.2,7.34051900599999));
#207899=CARTESIAN_POINT('Ctrl Pts',(7.88130647599995,11.6,7.34051900599999));
#207900=CARTESIAN_POINT('Ctrl Pts',(7.88262594599995,15.2,7.34274154699998));
#207901=CARTESIAN_POINT('Ctrl Pts',(7.88262594599995,11.6,7.34274154699998));
#207902=CARTESIAN_POINT('Ctrl Pts',(7.88394658699994,15.2,7.34497038799999));
#207903=CARTESIAN_POINT('Ctrl Pts',(7.88394658699994,11.6,7.34497038799999));
#207904=CARTESIAN_POINT('Ctrl Pts',(7.88526838499994,15.2,7.34720552299999));
#207905=CARTESIAN_POINT('Ctrl Pts',(7.88526838499994,11.6,7.34720552299999));
#207906=CARTESIAN_POINT('Ctrl Pts',(7.88659132599994,15.2,7.34944694699998));
#207907=CARTESIAN_POINT('Ctrl Pts',(7.88659132599994,11.6,7.34944694699998));
#207908=CARTESIAN_POINT('Ctrl Pts',(7.88791539499995,15.2,7.35169465499999));
#207909=CARTESIAN_POINT('Ctrl Pts',(7.88791539499995,11.6,7.35169465499999));
#207910=CARTESIAN_POINT('Ctrl Pts',(7.88924058199994,15.2,7.35394864099998));
#207911=CARTESIAN_POINT('Ctrl Pts',(7.88924058199994,11.6,7.35394864099998));
#207912=CARTESIAN_POINT('Ctrl Pts',(7.89056687199994,15.2,7.35620889999999));
#207913=CARTESIAN_POINT('Ctrl Pts',(7.89056687199994,11.6,7.35620889999999));
#207914=CARTESIAN_POINT('Ctrl Pts',(7.89189425199995,15.2,7.35847542799998));
#207915=CARTESIAN_POINT('Ctrl Pts',(7.89189425199995,11.6,7.35847542799998));
#207916=CARTESIAN_POINT('Ctrl Pts',(7.89322270799994,15.2,7.36074821699999));
#207917=CARTESIAN_POINT('Ctrl Pts',(7.89322270799994,11.6,7.36074821699999));
#207918=CARTESIAN_POINT('Ctrl Pts',(7.89455222599994,15.2,7.36302726399998));
#207919=CARTESIAN_POINT('Ctrl Pts',(7.89455222599994,11.6,7.36302726399998));
#207920=CARTESIAN_POINT('Ctrl Pts',(7.89588279399994,15.2,7.36531256299998));
#207921=CARTESIAN_POINT('Ctrl Pts',(7.89588279399994,11.6,7.36531256299998));
#207922=CARTESIAN_POINT('Ctrl Pts',(7.89721439899994,15.2,7.36760410899999));
#207923=CARTESIAN_POINT('Ctrl Pts',(7.89721439899994,11.6,7.36760410899999));
#207924=CARTESIAN_POINT('Ctrl Pts',(7.89854702699994,15.2,7.36990189599998));
#207925=CARTESIAN_POINT('Ctrl Pts',(7.89854702699994,11.6,7.36990189599998));
#207926=CARTESIAN_POINT('Ctrl Pts',(7.89988066499994,15.2,7.37220591999999));
#207927=CARTESIAN_POINT('Ctrl Pts',(7.89988066499994,11.6,7.37220591999999));
#207928=CARTESIAN_POINT('Ctrl Pts',(7.90121529899994,15.2,7.37451617399999));
#207929=CARTESIAN_POINT('Ctrl Pts',(7.90121529899994,11.6,7.37451617399999));
#207930=CARTESIAN_POINT('Ctrl Pts',(7.90255091899994,15.2,7.37683265399999));
#207931=CARTESIAN_POINT('Ctrl Pts',(7.90255091899994,11.6,7.37683265399999));
#207932=CARTESIAN_POINT('Ctrl Pts',(7.90388750899995,15.2,7.37915535499998));
#207933=CARTESIAN_POINT('Ctrl Pts',(7.90388750899995,11.6,7.37915535499998));
#207934=CARTESIAN_POINT('Ctrl Pts',(7.90522505699994,15.2,7.38148427099999));
#207935=CARTESIAN_POINT('Ctrl Pts',(7.90522505699994,11.6,7.38148427099999));
#207936=CARTESIAN_POINT('Ctrl Pts',(7.90656354999994,15.2,7.38381939599999));
#207937=CARTESIAN_POINT('Ctrl Pts',(7.90656354999994,11.6,7.38381939599999));
#207938=CARTESIAN_POINT('Ctrl Pts',(7.90790297499995,15.2,7.38616072699998));
#207939=CARTESIAN_POINT('Ctrl Pts',(7.90790297499995,11.6,7.38616072699998));
#207940=CARTESIAN_POINT('Ctrl Pts',(7.90924331999994,15.2,7.38850825899998));
#207941=CARTESIAN_POINT('Ctrl Pts',(7.90924331999994,11.6,7.38850825899998));
#207942=CARTESIAN_POINT('Ctrl Pts',(7.91058456999994,15.2,7.39086198299999));
#207943=CARTESIAN_POINT('Ctrl Pts',(7.91058456999994,11.6,7.39086198299999));
#207944=CARTESIAN_POINT('Ctrl Pts',(7.91192671499994,15.2,7.39322189699998));
#207945=CARTESIAN_POINT('Ctrl Pts',(7.91192671499994,11.6,7.39322189699998));
#207946=CARTESIAN_POINT('Ctrl Pts',(7.91326973899994,15.2,7.39558799399998));
#207947=CARTESIAN_POINT('Ctrl Pts',(7.91326973899994,11.6,7.39558799399998));
#207948=CARTESIAN_POINT('Ctrl Pts',(7.91461363199994,15.2,7.39796027099998));
#207949=CARTESIAN_POINT('Ctrl Pts',(7.91461363199994,11.6,7.39796027099998));
#207950=CARTESIAN_POINT('Ctrl Pts',(7.91595838099994,15.2,7.40033872099998));
#207951=CARTESIAN_POINT('Ctrl Pts',(7.91595838099994,11.6,7.40033872099998));
#207952=CARTESIAN_POINT('Ctrl Pts',(7.91730397199994,15.2,7.40272333899998));
#207953=CARTESIAN_POINT('Ctrl Pts',(7.91730397199994,11.6,7.40272333899998));
#207954=CARTESIAN_POINT('Ctrl Pts',(7.91865039399994,15.2,7.40511412099998));
#207955=CARTESIAN_POINT('Ctrl Pts',(7.91865039399994,11.6,7.40511412099998));
#207956=CARTESIAN_POINT('Ctrl Pts',(7.91999763299994,15.2,7.40751105999998));
#207957=CARTESIAN_POINT('Ctrl Pts',(7.91999763299994,11.6,7.40751105999998));
#207958=CARTESIAN_POINT('Ctrl Pts',(7.92134567599994,15.2,7.40991415199999));
#207959=CARTESIAN_POINT('Ctrl Pts',(7.92134567599994,11.6,7.40991415199999));
#207960=CARTESIAN_POINT('Ctrl Pts',(7.92269451299994,15.2,7.41232339099999));
#207961=CARTESIAN_POINT('Ctrl Pts',(7.92269451299994,11.6,7.41232339099999));
#207962=CARTESIAN_POINT('Ctrl Pts',(7.92404412999994,15.2,7.41473877199999));
#207963=CARTESIAN_POINT('Ctrl Pts',(7.92404412999994,11.6,7.41473877199999));
#207964=CARTESIAN_POINT('Ctrl Pts',(7.92539451299994,15.2,7.41716029099998));
#207965=CARTESIAN_POINT('Ctrl Pts',(7.92539451299994,11.6,7.41716029099998));
#207966=CARTESIAN_POINT('Ctrl Pts',(7.92674565299994,15.2,7.41958794199999));
#207967=CARTESIAN_POINT('Ctrl Pts',(7.92674565299994,11.6,7.41958794199999));
#207968=CARTESIAN_POINT('Ctrl Pts',(7.92809753399994,15.2,7.42202171999998));
#207969=CARTESIAN_POINT('Ctrl Pts',(7.92809753399994,11.6,7.42202171999998));
#207970=CARTESIAN_POINT('Ctrl Pts',(7.92945014599994,15.2,7.42446161799998));
#207971=CARTESIAN_POINT('Ctrl Pts',(7.92945014599994,11.6,7.42446161799998));
#207972=CARTESIAN_POINT('Ctrl Pts',(7.93080347599994,15.2,7.42690763399998));
#207973=CARTESIAN_POINT('Ctrl Pts',(7.93080347599994,11.6,7.42690763399998));
#207974=CARTESIAN_POINT('Ctrl Pts',(7.93215751199994,15.2,7.42935976099999));
#207975=CARTESIAN_POINT('Ctrl Pts',(7.93215751199994,11.6,7.42935976099999));
#207976=CARTESIAN_POINT('Ctrl Pts',(7.93351224099994,15.2,7.43181799299999));
#207977=CARTESIAN_POINT('Ctrl Pts',(7.93351224099994,11.6,7.43181799299999));
#207978=CARTESIAN_POINT('Ctrl Pts',(7.93486765099995,15.2,7.43428232699999));
#207979=CARTESIAN_POINT('Ctrl Pts',(7.93486765099995,11.6,7.43428232699999));
#207980=CARTESIAN_POINT('Ctrl Pts',(7.93622373099995,15.2,7.43675275699999));
#207981=CARTESIAN_POINT('Ctrl Pts',(7.93622373099995,11.6,7.43675275699999));
#207982=CARTESIAN_POINT('Ctrl Pts',(7.93758046899995,15.2,7.43922927699998));
#207983=CARTESIAN_POINT('Ctrl Pts',(7.93758046899995,11.6,7.43922927699998));
#207984=CARTESIAN_POINT('Ctrl Pts',(7.93893784999994,15.2,7.44171188299998));
#207985=CARTESIAN_POINT('Ctrl Pts',(7.93893784999994,11.6,7.44171188299998));
#207986=CARTESIAN_POINT('Ctrl Pts',(7.94029586499994,15.2,7.44420056899998));
#207987=CARTESIAN_POINT('Ctrl Pts',(7.94029586499994,11.6,7.44420056899998));
#207988=CARTESIAN_POINT('Ctrl Pts',(7.94165449999995,15.2,7.44669532999998));
#207989=CARTESIAN_POINT('Ctrl Pts',(7.94165449999995,11.6,7.44669532999998));
#207990=CARTESIAN_POINT('Ctrl Pts',(7.94301374399994,15.2,7.44919616099998));
#207991=CARTESIAN_POINT('Ctrl Pts',(7.94301374399994,11.6,7.44919616099998));
#207992=CARTESIAN_POINT('Ctrl Pts',(7.94437358499994,15.2,7.45170305799999));
#207993=CARTESIAN_POINT('Ctrl Pts',(7.94437358499994,11.6,7.45170305799999));
#207994=CARTESIAN_POINT('Ctrl Pts',(7.94573401199994,15.2,7.45421601399999));
#207995=CARTESIAN_POINT('Ctrl Pts',(7.94573401199994,11.6,7.45421601399999));
#207996=CARTESIAN_POINT('Ctrl Pts',(7.94709500999994,15.2,7.45673502499999));
#207997=CARTESIAN_POINT('Ctrl Pts',(7.94709500999994,11.6,7.45673502499999));
#207998=CARTESIAN_POINT('Ctrl Pts',(7.94845656999994,15.2,7.45926008499998));
#207999=CARTESIAN_POINT('Ctrl Pts',(7.94845656999994,11.6,7.45926008499998));
#208000=CARTESIAN_POINT('Ctrl Pts',(7.94981867799994,15.2,7.46179118999999));
#208001=CARTESIAN_POINT('Ctrl Pts',(7.94981867799994,11.6,7.46179118999999));
#208002=CARTESIAN_POINT('Ctrl Pts',(7.95118132499994,15.2,7.46432833399999));
#208003=CARTESIAN_POINT('Ctrl Pts',(7.95118132499994,11.6,7.46432833399999));
#208004=CARTESIAN_POINT('Ctrl Pts',(7.95254449699994,15.2,7.46687151199998));
#208005=CARTESIAN_POINT('Ctrl Pts',(7.95254449699994,11.6,7.46687151199998));
#208006=CARTESIAN_POINT('Ctrl Pts',(7.95390818299994,15.2,7.46942071899999));
#208007=CARTESIAN_POINT('Ctrl Pts',(7.95390818299994,11.6,7.46942071899999));
#208008=CARTESIAN_POINT('Ctrl Pts',(7.95527237099995,15.2,7.47197595099999));
#208009=CARTESIAN_POINT('Ctrl Pts',(7.95527237099995,11.6,7.47197595099999));
#208010=CARTESIAN_POINT('Ctrl Pts',(7.95663704999995,15.2,7.47453720099998));
#208011=CARTESIAN_POINT('Ctrl Pts',(7.95663704999995,11.6,7.47453720099998));
#208012=CARTESIAN_POINT('Ctrl Pts',(7.95800220699994,15.2,7.47710446499998));
#208013=CARTESIAN_POINT('Ctrl Pts',(7.95800220699994,11.6,7.47710446499998));
#208014=CARTESIAN_POINT('Ctrl Pts',(7.95936783099994,15.2,7.47967773799999));
#208015=CARTESIAN_POINT('Ctrl Pts',(7.95936783099994,11.6,7.47967773799999));
#208016=CARTESIAN_POINT('Ctrl Pts',(7.96073391099994,15.2,7.48225701399999));
#208017=CARTESIAN_POINT('Ctrl Pts',(7.96073391099994,11.6,7.48225701399999));
#208018=CARTESIAN_POINT('Ctrl Pts',(7.96210043599994,15.2,7.48484228899999));
#208019=CARTESIAN_POINT('Ctrl Pts',(7.96210043599994,11.6,7.48484228899999));
#208020=CARTESIAN_POINT('Ctrl Pts',(7.96346739099994,15.2,7.48743355699999));
#208021=CARTESIAN_POINT('Ctrl Pts',(7.96346739099994,11.6,7.48743355699999));
#208022=CARTESIAN_POINT('Ctrl Pts',(7.96483476899994,15.2,7.49003081299998));
#208023=CARTESIAN_POINT('Ctrl Pts',(7.96483476899994,11.6,7.49003081299998));
#208024=CARTESIAN_POINT('Ctrl Pts',(7.96620255699994,15.2,7.49263405299998));
#208025=CARTESIAN_POINT('Ctrl Pts',(7.96620255699994,11.6,7.49263405299998));
#208026=CARTESIAN_POINT('Ctrl Pts',(7.96757074099994,15.2,7.49524327099999));
#208027=CARTESIAN_POINT('Ctrl Pts',(7.96757074099994,11.6,7.49524327099999));
#208028=CARTESIAN_POINT('Ctrl Pts',(7.96893931299994,15.2,7.49785846199998));
#208029=CARTESIAN_POINT('Ctrl Pts',(7.96893931299994,11.6,7.49785846199998));
#208030=CARTESIAN_POINT('Ctrl Pts',(7.97030825999994,15.2,7.50047962099998));
#208031=CARTESIAN_POINT('Ctrl Pts',(7.97030825999994,11.6,7.50047962099998));
#208032=CARTESIAN_POINT('Ctrl Pts',(7.97167756999994,15.2,7.50310674299998));
#208033=CARTESIAN_POINT('Ctrl Pts',(7.97167756999994,11.6,7.50310674299998));
#208034=CARTESIAN_POINT('Ctrl Pts',(7.97304723399994,15.2,7.50573982299999));
#208035=CARTESIAN_POINT('Ctrl Pts',(7.97304723399994,11.6,7.50573982299999));
#208036=CARTESIAN_POINT('Ctrl Pts',(7.97441723799994,15.2,7.50837885499998));
#208037=CARTESIAN_POINT('Ctrl Pts',(7.97441723799994,11.6,7.50837885499998));
#208038=CARTESIAN_POINT('Ctrl Pts',(7.97578757299994,15.2,7.51102383499998));
#208039=CARTESIAN_POINT('Ctrl Pts',(7.97578757299994,11.6,7.51102383499998));
#208040=CARTESIAN_POINT('Ctrl Pts',(7.97715822599995,15.2,7.51367475799999));
#208041=CARTESIAN_POINT('Ctrl Pts',(7.97715822599995,11.6,7.51367475799999));
#208042=CARTESIAN_POINT('Ctrl Pts',(7.97852918799994,15.2,7.51633161899999));
#208043=CARTESIAN_POINT('Ctrl Pts',(7.97852918799994,11.6,7.51633161899999));
#208044=CARTESIAN_POINT('Ctrl Pts',(7.97990044399994,15.2,7.51899441299998));
#208045=CARTESIAN_POINT('Ctrl Pts',(7.97990044399994,11.6,7.51899441299998));
#208046=CARTESIAN_POINT('Ctrl Pts',(7.98127198699994,15.2,7.52166313299998));
#208047=CARTESIAN_POINT('Ctrl Pts',(7.98127198699994,11.6,7.52166313299998));
#208048=CARTESIAN_POINT('Ctrl Pts',(7.98264380399995,15.2,7.52433777599999));
#208049=CARTESIAN_POINT('Ctrl Pts',(7.98264380399995,11.6,7.52433777599999));
#208050=CARTESIAN_POINT('Ctrl Pts',(7.98401588399994,15.2,7.52701833699999));
#208051=CARTESIAN_POINT('Ctrl Pts',(7.98401588399994,11.6,7.52701833699999));
#208052=CARTESIAN_POINT('Ctrl Pts',(7.98538821699994,15.2,7.52970480999998));
#208053=CARTESIAN_POINT('Ctrl Pts',(7.98538821699994,11.6,7.52970480999998));
#208054=CARTESIAN_POINT('Ctrl Pts',(7.98676078999994,15.2,7.53239718999998));
#208055=CARTESIAN_POINT('Ctrl Pts',(7.98676078999994,11.6,7.53239718999998));
#208056=CARTESIAN_POINT('Ctrl Pts',(7.98813359199994,15.2,7.53509547299998));
#208057=CARTESIAN_POINT('Ctrl Pts',(7.98813359199994,11.6,7.53509547299998));
#208058=CARTESIAN_POINT('Ctrl Pts',(7.98950661399994,15.2,7.53779965299999));
#208059=CARTESIAN_POINT('Ctrl Pts',(7.98950661399994,11.6,7.53779965299999));
#208060=CARTESIAN_POINT('Ctrl Pts',(7.99087984399995,15.2,7.54050972499999));
#208061=CARTESIAN_POINT('Ctrl Pts',(7.99087984399995,11.6,7.54050972499999));
#208062=CARTESIAN_POINT('Ctrl Pts',(7.99225327199995,15.2,7.54322568499998));
#208063=CARTESIAN_POINT('Ctrl Pts',(7.99225327199995,11.6,7.54322568499998));
#208064=CARTESIAN_POINT('Ctrl Pts',(7.99362688499994,15.2,7.54594752699998));
#208065=CARTESIAN_POINT('Ctrl Pts',(7.99362688499994,11.6,7.54594752699998));
#208066=CARTESIAN_POINT('Ctrl Pts',(7.99500067299994,15.2,7.54867524499998));
#208067=CARTESIAN_POINT('Ctrl Pts',(7.99500067299994,11.6,7.54867524499998));
#208068=CARTESIAN_POINT('Ctrl Pts',(7.99637462599994,15.2,7.55140883699998));
#208069=CARTESIAN_POINT('Ctrl Pts',(7.99637462599994,11.6,7.55140883699998));
#208070=CARTESIAN_POINT('Ctrl Pts',(7.99774873399994,15.2,7.55414829599999));
#208071=CARTESIAN_POINT('Ctrl Pts',(7.99774873399994,11.6,7.55414829599999));
#208072=CARTESIAN_POINT('Ctrl Pts',(7.99912298399994,15.2,7.55689361599998));
#208073=CARTESIAN_POINT('Ctrl Pts',(7.99912298399994,11.6,7.55689361599998));
#208074=CARTESIAN_POINT('Ctrl Pts',(8.00049736599994,15.2,7.55964479299998));
#208075=CARTESIAN_POINT('Ctrl Pts',(8.00049736599994,11.6,7.55964479299998));
#208076=CARTESIAN_POINT('Ctrl Pts',(8.00187186999995,15.2,7.56240182299998));
#208077=CARTESIAN_POINT('Ctrl Pts',(8.00187186999995,11.6,7.56240182299998));
#208078=CARTESIAN_POINT('Ctrl Pts',(8.00324648399994,15.2,7.56516469899999));
#208079=CARTESIAN_POINT('Ctrl Pts',(8.00324648399994,11.6,7.56516469899999));
#208080=CARTESIAN_POINT('Ctrl Pts',(8.00462119899995,15.2,7.56793341899999));
#208081=CARTESIAN_POINT('Ctrl Pts',(8.00462119899995,11.6,7.56793341899999));
#208082=CARTESIAN_POINT('Ctrl Pts',(8.00599600299994,15.2,7.57070797499999));
#208083=CARTESIAN_POINT('Ctrl Pts',(8.00599600299994,11.6,7.57070797499999));
#208084=CARTESIAN_POINT('Ctrl Pts',(8.00737088599995,15.2,7.57348836199998));
#208085=CARTESIAN_POINT('Ctrl Pts',(8.00737088599995,11.6,7.57348836199998));
#208086=CARTESIAN_POINT('Ctrl Pts',(8.00874583699994,15.2,7.57627457799998));
#208087=CARTESIAN_POINT('Ctrl Pts',(8.00874583699994,11.6,7.57627457799998));
#208088=CARTESIAN_POINT('Ctrl Pts',(8.01012084599994,15.2,7.57906661499998));
#208089=CARTESIAN_POINT('Ctrl Pts',(8.01012084599994,11.6,7.57906661499998));
#208090=CARTESIAN_POINT('Ctrl Pts',(8.01149590299995,15.2,7.58186446999999));
#208091=CARTESIAN_POINT('Ctrl Pts',(8.01149590299995,11.6,7.58186446999999));
#208092=CARTESIAN_POINT('Ctrl Pts',(8.01287099699995,15.2,7.58466813699999));
#208093=CARTESIAN_POINT('Ctrl Pts',(8.01287099699995,11.6,7.58466813699999));
#208094=CARTESIAN_POINT('Ctrl Pts',(8.01424611599994,15.2,7.58747760999999));
#208095=CARTESIAN_POINT('Ctrl Pts',(8.01424611599994,11.6,7.58747760999999));
#208096=CARTESIAN_POINT('Ctrl Pts',(8.01562124999995,15.2,7.59029288699999));
#208097=CARTESIAN_POINT('Ctrl Pts',(8.01562124999995,11.6,7.59029288699999));
#208098=CARTESIAN_POINT('Ctrl Pts',(8.01699639099994,15.2,7.59311395999998));
#208099=CARTESIAN_POINT('Ctrl Pts',(8.01699639099994,11.6,7.59311395999998));
#208100=CARTESIAN_POINT('Ctrl Pts',(8.01837152699994,15.2,7.59594082499999));
#208101=CARTESIAN_POINT('Ctrl Pts',(8.01837152699994,11.6,7.59594082499999));
#208102=CARTESIAN_POINT('Ctrl Pts',(8.01974664599994,15.2,7.59877347799998));
#208103=CARTESIAN_POINT('Ctrl Pts',(8.01974664599994,11.6,7.59877347799998));
#208104=CARTESIAN_POINT('Ctrl Pts',(8.02112173999994,15.2,7.60161191299999));
#208105=CARTESIAN_POINT('Ctrl Pts',(8.02112173999994,11.6,7.60161191299999));
#208106=CARTESIAN_POINT('Ctrl Pts',(8.02249679899995,15.2,7.60445612599998));
#208107=CARTESIAN_POINT('Ctrl Pts',(8.02249679899995,11.6,7.60445612599998));
#208108=CARTESIAN_POINT('Ctrl Pts',(8.02387180999995,15.2,7.60730610999998));
#208109=CARTESIAN_POINT('Ctrl Pts',(8.02387180999995,11.6,7.60730610999998));
#208110=CARTESIAN_POINT('Ctrl Pts',(8.02524676499995,15.2,7.61016186299998));
#208111=CARTESIAN_POINT('Ctrl Pts',(8.02524676499995,11.6,7.61016186299998));
#208112=CARTESIAN_POINT('Ctrl Pts',(8.02662165299994,15.2,7.61302337699998));
#208113=CARTESIAN_POINT('Ctrl Pts',(8.02662165299994,11.6,7.61302337699998));
#208114=CARTESIAN_POINT('Ctrl Pts',(8.02799646399994,15.2,7.61589064899999));
#208115=CARTESIAN_POINT('Ctrl Pts',(8.02799646399994,11.6,7.61589064899999));
#208116=CARTESIAN_POINT('Ctrl Pts',(8.02937118699995,15.2,7.61876367399999));
#208117=CARTESIAN_POINT('Ctrl Pts',(8.02937118699995,11.6,7.61876367399999));
#208118=CARTESIAN_POINT('Ctrl Pts',(8.03074581299994,15.2,7.62164244599998));
#208119=CARTESIAN_POINT('Ctrl Pts',(8.03074581299994,11.6,7.62164244599998));
#208120=CARTESIAN_POINT('Ctrl Pts',(8.03212033199994,15.2,7.62452696099999));
#208121=CARTESIAN_POINT('Ctrl Pts',(8.03212033199994,11.6,7.62452696099999));
#208122=CARTESIAN_POINT('Ctrl Pts',(8.03349473299994,15.2,7.62741721399999));
#208123=CARTESIAN_POINT('Ctrl Pts',(8.03349473299994,11.6,7.62741721399999));
#208124=CARTESIAN_POINT('Ctrl Pts',(8.03486900499994,15.2,7.63031319899999));
#208125=CARTESIAN_POINT('Ctrl Pts',(8.03486900499994,11.6,7.63031319899999));
#208126=CARTESIAN_POINT('Ctrl Pts',(8.03624313899994,15.2,7.63321491099998));
#208127=CARTESIAN_POINT('Ctrl Pts',(8.03624313899994,11.6,7.63321491099998));
#208128=CARTESIAN_POINT('Ctrl Pts',(8.03761712599995,15.2,7.63612234699998));
#208129=CARTESIAN_POINT('Ctrl Pts',(8.03761712599995,11.6,7.63612234699998));
#208130=CARTESIAN_POINT('Ctrl Pts',(8.03899095499995,15.2,7.63903550099998));
#208131=CARTESIAN_POINT('Ctrl Pts',(8.03899095499995,11.6,7.63903550099998));
#208132=CARTESIAN_POINT('Ctrl Pts',(8.04036461599994,15.2,7.64195436799999));
#208133=CARTESIAN_POINT('Ctrl Pts',(8.04036461599994,11.6,7.64195436799999));
#208134=CARTESIAN_POINT('Ctrl Pts',(8.04173809999994,15.2,7.64487894199998));
#208135=CARTESIAN_POINT('Ctrl Pts',(8.04173809999994,11.6,7.64487894199998));
#208136=CARTESIAN_POINT('Ctrl Pts',(8.04311139399994,15.2,7.64780921999999));
#208137=CARTESIAN_POINT('Ctrl Pts',(8.04311139399994,11.6,7.64780921999999));
#208138=CARTESIAN_POINT('Ctrl Pts',(8.04448449099995,15.2,7.65074519599998));
#208139=CARTESIAN_POINT('Ctrl Pts',(8.04448449099995,11.6,7.65074519599998));
#208140=CARTESIAN_POINT('Ctrl Pts',(8.04585738099994,15.2,7.65368686499999));
#208141=CARTESIAN_POINT('Ctrl Pts',(8.04585738099994,11.6,7.65368686499999));
#208142=CARTESIAN_POINT('Ctrl Pts',(8.04723005199994,15.2,7.65663422199999));
#208143=CARTESIAN_POINT('Ctrl Pts',(8.04723005199994,11.6,7.65663422199999));
#208144=CARTESIAN_POINT('Ctrl Pts',(8.04860249599994,15.2,7.65958726299999));
#208145=CARTESIAN_POINT('Ctrl Pts',(8.04860249599994,11.6,7.65958726299999));
#208146=CARTESIAN_POINT('Ctrl Pts',(8.04997470299995,15.2,7.66254598199998));
#208147=CARTESIAN_POINT('Ctrl Pts',(8.04997470299995,11.6,7.66254598199998));
#208148=CARTESIAN_POINT('Ctrl Pts',(8.05134666299994,15.2,7.66551037499998));
#208149=CARTESIAN_POINT('Ctrl Pts',(8.05134666299994,11.6,7.66551037499998));
#208150=CARTESIAN_POINT('Ctrl Pts',(8.05271836599994,15.2,7.66848043599998));
#208151=CARTESIAN_POINT('Ctrl Pts',(8.05271836599994,11.6,7.66848043599998));
#208152=CARTESIAN_POINT('Ctrl Pts',(8.05408980299994,15.2,7.67145616099998));
#208153=CARTESIAN_POINT('Ctrl Pts',(8.05408980299994,11.6,7.67145616099998));
#208154=CARTESIAN_POINT('Ctrl Pts',(8.05546096299994,15.2,7.67443754599999));
#208155=CARTESIAN_POINT('Ctrl Pts',(8.05546096299994,11.6,7.67443754599999));
#208156=CARTESIAN_POINT('Ctrl Pts',(8.05683183699994,15.2,7.67742458299999));
#208157=CARTESIAN_POINT('Ctrl Pts',(8.05683183699994,11.6,7.67742458299999));
#208158=CARTESIAN_POINT('Ctrl Pts',(8.05820241499994,15.2,7.68041726999999));
#208159=CARTESIAN_POINT('Ctrl Pts',(8.05820241499994,11.6,7.68041726999999));
#208160=CARTESIAN_POINT('Ctrl Pts',(8.05957268699995,15.2,7.68341559999998));
#208161=CARTESIAN_POINT('Ctrl Pts',(8.05957268699995,11.6,7.68341559999998));
#208162=CARTESIAN_POINT('Ctrl Pts',(8.06094264599994,15.2,7.68641956999998));
#208163=CARTESIAN_POINT('Ctrl Pts',(8.06094264599994,11.6,7.68641956999998));
#208164=CARTESIAN_POINT('Ctrl Pts',(8.06231227799995,15.2,7.68942917499999));
#208165=CARTESIAN_POINT('Ctrl Pts',(8.06231227799995,11.6,7.68942917499999));
#208166=CARTESIAN_POINT('Ctrl Pts',(8.06368157799995,15.2,7.69244440799999));
#208167=CARTESIAN_POINT('Ctrl Pts',(8.06368157799995,11.6,7.69244440799999));
#208168=CARTESIAN_POINT('Ctrl Pts',(8.06505053199994,15.2,7.69546526699998));
#208169=CARTESIAN_POINT('Ctrl Pts',(8.06505053199994,11.6,7.69546526699998));
#208170=CARTESIAN_POINT('Ctrl Pts',(8.06641913399995,15.2,7.69849174399998));
#208171=CARTESIAN_POINT('Ctrl Pts',(8.06641913399995,11.6,7.69849174399998));
#208172=CARTESIAN_POINT('Ctrl Pts',(8.06778737299994,15.2,7.70152383699998));
#208173=CARTESIAN_POINT('Ctrl Pts',(8.06778737299994,11.6,7.70152383699998));
#208174=CARTESIAN_POINT('Ctrl Pts',(8.06915523899994,15.2,7.70456153799999));
#208175=CARTESIAN_POINT('Ctrl Pts',(8.06915523899994,11.6,7.70456153799999));
#208176=CARTESIAN_POINT('Ctrl Pts',(8.07052272299994,15.2,7.70760484499998));
#208177=CARTESIAN_POINT('Ctrl Pts',(8.07052272299994,11.6,7.70760484499998));
#208178=CARTESIAN_POINT('Ctrl Pts',(8.07188981699994,15.2,7.71065375199999));
#208179=CARTESIAN_POINT('Ctrl Pts',(8.07188981699994,11.6,7.71065375199999));
#208180=CARTESIAN_POINT('Ctrl Pts',(8.07325650899994,15.2,7.71370825499999));
#208181=CARTESIAN_POINT('Ctrl Pts',(8.07325650899994,11.6,7.71370825499999));
#208182=CARTESIAN_POINT('Ctrl Pts',(8.07462279199994,15.2,7.71676834699999));
#208183=CARTESIAN_POINT('Ctrl Pts',(8.07462279199994,11.6,7.71676834699999));
#208184=CARTESIAN_POINT('Ctrl Pts',(8.07598865399994,15.2,7.71983402599999));
#208185=CARTESIAN_POINT('Ctrl Pts',(8.07598865399994,11.6,7.71983402599999));
#208186=CARTESIAN_POINT('Ctrl Pts',(8.07735408799994,15.2,7.72290528399999));
#208187=CARTESIAN_POINT('Ctrl Pts',(8.07735408799994,11.6,7.72290528399999));
#208188=CARTESIAN_POINT('Ctrl Pts',(8.07871908299994,15.2,7.72598211799998));
#208189=CARTESIAN_POINT('Ctrl Pts',(8.07871908299994,11.6,7.72598211799998));
#208190=CARTESIAN_POINT('Ctrl Pts',(8.08008363099994,15.2,7.72906452199998));
#208191=CARTESIAN_POINT('Ctrl Pts',(8.08008363099994,11.6,7.72906452199998));
#208192=CARTESIAN_POINT('Ctrl Pts',(8.08144772299995,15.2,7.73215249199998));
#208193=CARTESIAN_POINT('Ctrl Pts',(8.08144772299995,11.6,7.73215249199998));
#208194=CARTESIAN_POINT('Ctrl Pts',(8.08281134699994,15.2,7.73524602399998));
#208195=CARTESIAN_POINT('Ctrl Pts',(8.08281134699994,11.6,7.73524602399998));
#208196=CARTESIAN_POINT('Ctrl Pts',(8.08417449699995,15.2,7.73834511199999));
#208197=CARTESIAN_POINT('Ctrl Pts',(8.08417449699995,11.6,7.73834511199999));
#208198=CARTESIAN_POINT('Ctrl Pts',(8.08553716199994,15.2,7.74144974999999));
#208199=CARTESIAN_POINT('Ctrl Pts',(8.08553716199994,11.6,7.74144974999999));
#208200=CARTESIAN_POINT('Ctrl Pts',(8.08689933199994,15.2,7.74455993599998));
#208201=CARTESIAN_POINT('Ctrl Pts',(8.08689933199994,11.6,7.74455993599998));
#208202=CARTESIAN_POINT('Ctrl Pts',(8.08826100099994,15.2,7.74767566199999));
#208203=CARTESIAN_POINT('Ctrl Pts',(8.08826100099994,11.6,7.74767566199999));
#208204=CARTESIAN_POINT('Ctrl Pts',(8.08962215599994,15.2,7.75079692599999));
#208205=CARTESIAN_POINT('Ctrl Pts',(8.08962215599994,11.6,7.75079692599999));
#208206=CARTESIAN_POINT('Ctrl Pts',(8.09098279099994,15.2,7.75392372099999));
#208207=CARTESIAN_POINT('Ctrl Pts',(8.09098279099994,11.6,7.75392372099999));
#208208=CARTESIAN_POINT('Ctrl Pts',(8.09234289399994,15.2,7.75705604499999));
#208209=CARTESIAN_POINT('Ctrl Pts',(8.09234289399994,11.6,7.75705604499999));
#208210=CARTESIAN_POINT('Ctrl Pts',(8.09370245799995,15.2,7.76019388899999));
#208211=CARTESIAN_POINT('Ctrl Pts',(8.09370245799995,11.6,7.76019388899999));
#208212=CARTESIAN_POINT('Ctrl Pts',(8.09506147399994,15.2,7.76333725099998));
#208213=CARTESIAN_POINT('Ctrl Pts',(8.09506147399994,11.6,7.76333725099998));
#208214=CARTESIAN_POINT('Ctrl Pts',(8.09641993199994,15.2,7.76648612399998));
#208215=CARTESIAN_POINT('Ctrl Pts',(8.09641993199994,11.6,7.76648612399998));
#208216=CARTESIAN_POINT('Ctrl Pts',(8.09777782299994,15.2,7.76964050699998));
#208217=CARTESIAN_POINT('Ctrl Pts',(8.09777782299994,11.6,7.76964050699998));
#208218=CARTESIAN_POINT('Ctrl Pts',(8.09913513899994,15.2,7.77280038999999));
#208219=CARTESIAN_POINT('Ctrl Pts',(8.09913513899994,11.6,7.77280038999999));
#208220=CARTESIAN_POINT('Ctrl Pts',(8.10049186899995,15.2,7.77596577299998));
#208221=CARTESIAN_POINT('Ctrl Pts',(8.10049186899995,11.6,7.77596577299998));
#208222=CARTESIAN_POINT('Ctrl Pts',(8.10184800599994,15.2,7.77913664799998));
#208223=CARTESIAN_POINT('Ctrl Pts',(8.10184800599994,11.6,7.77913664799998));
#208224=CARTESIAN_POINT('Ctrl Pts',(8.10320353999994,15.2,7.78231301199998));
#208225=CARTESIAN_POINT('Ctrl Pts',(8.10320353999994,11.6,7.78231301199998));
#208226=CARTESIAN_POINT('Ctrl Pts',(8.10455846199994,15.2,7.78549485899998));
#208227=CARTESIAN_POINT('Ctrl Pts',(8.10455846199994,11.6,7.78549485899998));
#208228=CARTESIAN_POINT('Ctrl Pts',(8.10591276399995,15.2,7.78868218399998));
#208229=CARTESIAN_POINT('Ctrl Pts',(8.10591276399995,11.6,7.78868218399998));
#208230=CARTESIAN_POINT('Ctrl Pts',(8.10726643599994,15.2,7.79187498299999));
#208231=CARTESIAN_POINT('Ctrl Pts',(8.10726643599994,11.6,7.79187498299999));
#208232=CARTESIAN_POINT('Ctrl Pts',(8.10861946999994,15.2,7.79507325099999));
#208233=CARTESIAN_POINT('Ctrl Pts',(8.10861946999994,11.6,7.79507325099999));
#208234=CARTESIAN_POINT('Ctrl Pts',(8.10997185699994,15.2,7.79827698299999));
#208235=CARTESIAN_POINT('Ctrl Pts',(8.10997185699994,11.6,7.79827698299999));
#208236=CARTESIAN_POINT('Ctrl Pts',(8.11132358699994,15.2,7.80148617399998));
#208237=CARTESIAN_POINT('Ctrl Pts',(8.11132358699994,11.6,7.80148617399998));
#208238=CARTESIAN_POINT('Ctrl Pts',(8.11267465299995,15.2,7.80470081999999));
#208239=CARTESIAN_POINT('Ctrl Pts',(8.11267465299995,11.6,7.80470081999999));
#208240=CARTESIAN_POINT('Ctrl Pts',(8.11402504499994,15.2,7.80792091499999));
#208241=CARTESIAN_POINT('Ctrl Pts',(8.11402504499994,11.6,7.80792091499999));
#208242=CARTESIAN_POINT('Ctrl Pts',(8.11537475499994,15.2,7.81114645499999));
#208243=CARTESIAN_POINT('Ctrl Pts',(8.11537475499994,11.6,7.81114645499999));
#208244=CARTESIAN_POINT('Ctrl Pts',(8.11672377399994,15.2,7.81437743399999));
#208245=CARTESIAN_POINT('Ctrl Pts',(8.11672377399994,11.6,7.81437743399999));
#208246=CARTESIAN_POINT('Ctrl Pts',(8.11807209199995,15.2,7.81761384899998));
#208247=CARTESIAN_POINT('Ctrl Pts',(8.11807209199995,11.6,7.81761384899998));
#208248=CARTESIAN_POINT('Ctrl Pts',(8.11941970299995,15.2,7.82085569399998));
#208249=CARTESIAN_POINT('Ctrl Pts',(8.11941970299995,11.6,7.82085569399998));
#208250=CARTESIAN_POINT('Ctrl Pts',(8.12076659499994,15.2,7.82410296499998));
#208251=CARTESIAN_POINT('Ctrl Pts',(8.12076659499994,11.6,7.82410296499998));
#208252=CARTESIAN_POINT('Ctrl Pts',(8.12211276199994,15.2,7.82735565499999));
#208253=CARTESIAN_POINT('Ctrl Pts',(8.12211276199994,11.6,7.82735565499999));
#208254=CARTESIAN_POINT('Ctrl Pts',(8.12345819499994,15.2,7.83061376199999));
#208255=CARTESIAN_POINT('Ctrl Pts',(8.12345819499994,11.6,7.83061376199999));
#208256=CARTESIAN_POINT('Ctrl Pts',(8.12480288299994,15.2,7.83387727999998));
#208257=CARTESIAN_POINT('Ctrl Pts',(8.12480288299994,11.6,7.83387727999998));
#208258=CARTESIAN_POINT('Ctrl Pts',(8.12614681999994,15.2,7.83714620399999));
#208259=CARTESIAN_POINT('Ctrl Pts',(8.12614681999994,11.6,7.83714620399999));
#208260=CARTESIAN_POINT('Ctrl Pts',(8.12748999699994,15.2,7.84042052999999));
#208261=CARTESIAN_POINT('Ctrl Pts',(8.12748999699994,11.6,7.84042052999999));
#208262=CARTESIAN_POINT('Ctrl Pts',(8.12883240399995,15.2,7.84370025199999));
#208263=CARTESIAN_POINT('Ctrl Pts',(8.12883240399995,11.6,7.84370025199999));
#208264=CARTESIAN_POINT('Ctrl Pts',(8.13017403399994,15.2,7.84698536599999));
#208265=CARTESIAN_POINT('Ctrl Pts',(8.13017403399994,11.6,7.84698536599999));
#208266=CARTESIAN_POINT('Ctrl Pts',(8.13151487799994,15.2,7.85027586699999));
#208267=CARTESIAN_POINT('Ctrl Pts',(8.13151487799994,11.6,7.85027586699999));
#208268=CARTESIAN_POINT('Ctrl Pts',(8.13285492699995,15.2,7.85357174999999));
#208269=CARTESIAN_POINT('Ctrl Pts',(8.13285492699995,11.6,7.85357174999999));
#208270=CARTESIAN_POINT('Ctrl Pts',(8.13419417199994,15.2,7.85687300999999));
#208271=CARTESIAN_POINT('Ctrl Pts',(8.13419417199994,11.6,7.85687300999999));
#208272=CARTESIAN_POINT('Ctrl Pts',(8.13553260699994,15.2,7.86017964299998));
#208273=CARTESIAN_POINT('Ctrl Pts',(8.13553260699994,11.6,7.86017964299998));
#208274=CARTESIAN_POINT('Ctrl Pts',(8.13687022199994,15.2,7.86349164399999));
#208275=CARTESIAN_POINT('Ctrl Pts',(8.13687022199994,11.6,7.86349164399999));
#208276=CARTESIAN_POINT('Ctrl Pts',(8.13820700799995,15.2,7.86680900799999));
#208277=CARTESIAN_POINT('Ctrl Pts',(8.13820700799995,11.6,7.86680900799999));
#208278=CARTESIAN_POINT('Ctrl Pts',(8.13954295599994,15.2,7.87013172999998));
#208279=CARTESIAN_POINT('Ctrl Pts',(8.13954295599994,11.6,7.87013172999998));
#208280=CARTESIAN_POINT('Ctrl Pts',(8.14087805899994,15.2,7.87345980499998));
#208281=CARTESIAN_POINT('Ctrl Pts',(8.14087805899994,11.6,7.87345980499998));
#208282=CARTESIAN_POINT('Ctrl Pts',(8.14221230899994,15.2,7.87679322899999));
#208283=CARTESIAN_POINT('Ctrl Pts',(8.14221230899994,11.6,7.87679322899999));
#208284=CARTESIAN_POINT('Ctrl Pts',(8.14354569599994,15.2,7.88013199699999));
#208285=CARTESIAN_POINT('Ctrl Pts',(8.14354569599994,11.6,7.88013199699999));
#208286=CARTESIAN_POINT('Ctrl Pts',(8.14487821399995,15.2,7.88347610399998));
#208287=CARTESIAN_POINT('Ctrl Pts',(8.14487821399995,11.6,7.88347610399998));
#208288=CARTESIAN_POINT('Ctrl Pts',(8.14620985199995,15.2,7.88682554499999));
#208289=CARTESIAN_POINT('Ctrl Pts',(8.14620985199995,11.6,7.88682554499999));
#208290=CARTESIAN_POINT('Ctrl Pts',(8.14754060299994,15.2,7.89018031599999));
#208291=CARTESIAN_POINT('Ctrl Pts',(8.14754060299994,11.6,7.89018031599999));
#208292=CARTESIAN_POINT('Ctrl Pts',(8.14887045999994,15.2,7.89354041099998));
#208293=CARTESIAN_POINT('Ctrl Pts',(8.14887045999994,11.6,7.89354041099998));
#208294=CARTESIAN_POINT('Ctrl Pts',(8.15019941199994,15.2,7.89690582699999));
#208295=CARTESIAN_POINT('Ctrl Pts',(8.15019941199994,11.6,7.89690582699999));
#208296=CARTESIAN_POINT('Ctrl Pts',(8.15152745299994,15.2,7.90027655699999));
#208297=CARTESIAN_POINT('Ctrl Pts',(8.15152745299994,11.6,7.90027655699999));
#208298=CARTESIAN_POINT('Ctrl Pts',(8.15285457299994,15.2,7.90365259799999));
#208299=CARTESIAN_POINT('Ctrl Pts',(8.15285457299994,11.6,7.90365259799999));
#208300=CARTESIAN_POINT('Ctrl Pts',(8.15418076399994,15.2,7.90703394499998));
#208301=CARTESIAN_POINT('Ctrl Pts',(8.15418076399994,11.6,7.90703394499998));
#208302=CARTESIAN_POINT('Ctrl Pts',(8.15550602099994,15.2,7.91042059199999));
#208303=CARTESIAN_POINT('Ctrl Pts',(8.15550602099994,11.6,7.91042059199999));
#208304=CARTESIAN_POINT('Ctrl Pts',(8.15683033099995,15.2,7.91381253499999));
#208305=CARTESIAN_POINT('Ctrl Pts',(8.15683033099995,11.6,7.91381253499999));
#208306=CARTESIAN_POINT('Ctrl Pts',(8.15815368899995,15.2,7.91720976999999));
#208307=CARTESIAN_POINT('Ctrl Pts',(8.15815368899995,11.6,7.91720976999999));
#208308=CARTESIAN_POINT('Ctrl Pts',(8.15947608599994,15.2,7.92061229099998));
#208309=CARTESIAN_POINT('Ctrl Pts',(8.15947608599994,11.6,7.92061229099998));
#208310=CARTESIAN_POINT('Ctrl Pts',(8.16079751299995,15.2,7.92402009399999));
#208311=CARTESIAN_POINT('Ctrl Pts',(8.16079751299995,11.6,7.92402009399999));
#208312=CARTESIAN_POINT('Ctrl Pts',(8.16211796399994,15.2,7.92743317399999));
#208313=CARTESIAN_POINT('Ctrl Pts',(8.16211796399994,11.6,7.92743317399999));
#208314=CARTESIAN_POINT('Ctrl Pts',(8.16343742899994,15.2,7.93085152599998));
#208315=CARTESIAN_POINT('Ctrl Pts',(8.16343742899994,11.6,7.93085152599998));
#208316=CARTESIAN_POINT('Ctrl Pts',(8.16475590099994,15.2,7.93427514699999));
#208317=CARTESIAN_POINT('Ctrl Pts',(8.16475590099994,11.6,7.93427514699999));
#208318=CARTESIAN_POINT('Ctrl Pts',(8.16607337199994,15.2,7.93770402899998));
#208319=CARTESIAN_POINT('Ctrl Pts',(8.16607337199994,11.6,7.93770402899998));
#208320=CARTESIAN_POINT('Ctrl Pts',(8.16738983299994,15.2,7.94113816999998));
#208321=CARTESIAN_POINT('Ctrl Pts',(8.16738983299994,11.6,7.94113816999998));
#208322=CARTESIAN_POINT('Ctrl Pts',(8.16870527599994,15.2,7.94457756299998));
#208323=CARTESIAN_POINT('Ctrl Pts',(8.16870527599994,11.6,7.94457756299998));
#208324=CARTESIAN_POINT('Ctrl Pts',(8.17001969299995,15.2,7.94802220599998));
#208325=CARTESIAN_POINT('Ctrl Pts',(8.17001969299995,11.6,7.94802220599998));
#208326=CARTESIAN_POINT('Ctrl Pts',(8.17133307699994,15.2,7.95147209099999));
#208327=CARTESIAN_POINT('Ctrl Pts',(8.17133307699994,11.6,7.95147209099999));
#208328=CARTESIAN_POINT('Ctrl Pts',(8.17264541999995,15.2,7.95492721699999));
#208329=CARTESIAN_POINT('Ctrl Pts',(8.17264541999995,11.6,7.95492721699999));
#208330=CARTESIAN_POINT('Ctrl Pts',(8.17395671199994,15.2,7.95838757499999));
#208331=CARTESIAN_POINT('Ctrl Pts',(8.17395671199994,11.6,7.95838757499999));
#208332=CARTESIAN_POINT('Ctrl Pts',(8.17526694799995,15.2,7.96185316399999));
#208333=CARTESIAN_POINT('Ctrl Pts',(8.17526694799995,11.6,7.96185316399999));
#208334=CARTESIAN_POINT('Ctrl Pts',(8.17657611899994,15.2,7.96532397699998));
#208335=CARTESIAN_POINT('Ctrl Pts',(8.17657611899994,11.6,7.96532397699998));
#208336=CARTESIAN_POINT('Ctrl Pts',(8.17788421699994,15.2,7.96880001099999));
#208337=CARTESIAN_POINT('Ctrl Pts',(8.17788421699994,11.6,7.96880001099999));
#208338=CARTESIAN_POINT('Ctrl Pts',(8.17919123399994,15.2,7.97228125999998));
#208339=CARTESIAN_POINT('Ctrl Pts',(8.17919123399994,11.6,7.97228125999998));
#208340=CARTESIAN_POINT('Ctrl Pts',(8.18049716299995,15.2,7.97576771899998));
#208341=CARTESIAN_POINT('Ctrl Pts',(8.18049716299995,11.6,7.97576771899998));
#208342=CARTESIAN_POINT('Ctrl Pts',(8.18180199499994,15.2,7.97925938399998));
#208343=CARTESIAN_POINT('Ctrl Pts',(8.18180199499994,11.6,7.97925938399998));
#208344=CARTESIAN_POINT('Ctrl Pts',(8.18310572199995,15.2,7.98275625099999));
#208345=CARTESIAN_POINT('Ctrl Pts',(8.18310572199995,11.6,7.98275625099999));
#208346=CARTESIAN_POINT('Ctrl Pts',(8.18440833599994,15.2,7.98625831199999));
#208347=CARTESIAN_POINT('Ctrl Pts',(8.18440833599994,11.6,7.98625831199999));
#208348=CARTESIAN_POINT('Ctrl Pts',(8.18570982799995,15.2,7.98976556499999));
#208349=CARTESIAN_POINT('Ctrl Pts',(8.18570982799995,11.6,7.98976556499999));
#208350=CARTESIAN_POINT('Ctrl Pts',(8.18701019199995,15.2,7.99327800499999));
#208351=CARTESIAN_POINT('Ctrl Pts',(8.18701019199995,11.6,7.99327800499999));
#208352=CARTESIAN_POINT('Ctrl Pts',(8.18830941999994,15.2,7.99679562499998));
#208353=CARTESIAN_POINT('Ctrl Pts',(8.18830941999994,11.6,7.99679562499998));
#208354=CARTESIAN_POINT('Ctrl Pts',(8.18960750499994,15.2,8.00031842399999));
#208355=CARTESIAN_POINT('Ctrl Pts',(8.18960750499994,11.6,8.00031842399999));
#208356=CARTESIAN_POINT('Ctrl Pts',(8.19090443899994,15.2,8.00384639699999));
#208357=CARTESIAN_POINT('Ctrl Pts',(8.19090443899994,11.6,8.00384639699999));
#208358=CARTESIAN_POINT('Ctrl Pts',(8.19220021699994,15.2,8.00737953699999));
#208359=CARTESIAN_POINT('Ctrl Pts',(8.19220021699994,11.6,8.00737953699999));
#208360=CARTESIAN_POINT('Ctrl Pts',(8.19349483099994,15.2,8.01091784299999));
#208361=CARTESIAN_POINT('Ctrl Pts',(8.19349483099994,11.6,8.01091784299999));
#208362=CARTESIAN_POINT('Ctrl Pts',(8.19478827199994,15.2,8.01446130799999));
#208363=CARTESIAN_POINT('Ctrl Pts',(8.19478827199994,11.6,8.01446130799999));
#208364=CARTESIAN_POINT('Ctrl Pts',(8.19608053199994,15.2,8.01800992699999));
#208365=CARTESIAN_POINT('Ctrl Pts',(8.19608053199994,11.6,8.01800992699999));
#208366=CARTESIAN_POINT('Ctrl Pts',(8.19737160099994,15.2,8.02156369499999));
#208367=CARTESIAN_POINT('Ctrl Pts',(8.19737160099994,11.6,8.02156369499999));
#208368=CARTESIAN_POINT('Ctrl Pts',(8.19866146999994,15.2,8.02512260499999));
#208369=CARTESIAN_POINT('Ctrl Pts',(8.19866146999994,11.6,8.02512260499999));
#208370=CARTESIAN_POINT('Ctrl Pts',(8.19995012899994,15.2,8.02868665099999));
#208371=CARTESIAN_POINT('Ctrl Pts',(8.19995012899994,11.6,8.02868665099999));
#208372=CARTESIAN_POINT('Ctrl Pts',(8.20123756999994,15.2,8.03225582899999));
#208373=CARTESIAN_POINT('Ctrl Pts',(8.20123756999994,11.6,8.03225582899999));
#208374=CARTESIAN_POINT('Ctrl Pts',(8.20252378699994,15.2,8.03583013499999));
#208375=CARTESIAN_POINT('Ctrl Pts',(8.20252378699994,11.6,8.03583013499999));
#208376=CARTESIAN_POINT('Ctrl Pts',(8.20380877399994,15.2,8.03940956399998));
#208377=CARTESIAN_POINT('Ctrl Pts',(8.20380877399994,11.6,8.03940956399998));
#208378=CARTESIAN_POINT('Ctrl Pts',(8.20509252799994,15.2,8.04299411599998));
#208379=CARTESIAN_POINT('Ctrl Pts',(8.20509252799994,11.6,8.04299411599998));
#208380=CARTESIAN_POINT('Ctrl Pts',(8.20637504799994,15.2,8.04658378899998));
#208381=CARTESIAN_POINT('Ctrl Pts',(8.20637504799994,11.6,8.04658378899998));
#208382=CARTESIAN_POINT('Ctrl Pts',(8.20740007499994,15.2,8.04945962199999));
#208383=CARTESIAN_POINT('Ctrl Pts',(8.20740007499994,11.6,8.04945962199999));
#208384=CARTESIAN_POINT('Ctrl Pts',(8.20816828899994,15.2,8.05161879999999));
#208385=CARTESIAN_POINT('Ctrl Pts',(8.20816828899994,11.6,8.05161879999999));
#208386=CARTESIAN_POINT('Ctrl Pts',(8.20868018299995,15.2,8.05305927699998));
#208387=CARTESIAN_POINT('Ctrl Pts',(8.20868018299995,11.6,8.05305927699998));
#208388=CARTESIAN_POINT('Ctrl Pts',(8.20893606999994,15.2,8.05377977099998));
#208389=CARTESIAN_POINT('Ctrl Pts',(8.20893606999994,11.6,8.05377977099998));
#208390=CARTESIAN_POINT('Ctrl Pts',(7.64657512299994,15.2,7.01216898699998));
#208391=CARTESIAN_POINT('Ctrl Pts',(7.64778328654791,15.2,7.01348522668636));
#208392=CARTESIAN_POINT('Ctrl Pts',(7.64902613283499,15.2,7.0148472224676));
#208393=CARTESIAN_POINT('Ctrl Pts',(7.65030255111842,15.2,7.01625467982076));
#208394=CARTESIAN_POINT('Ctrl Pts',(7.651585124936,15.2,7.01766892464472));
#208395=CARTESIAN_POINT('Ctrl Pts',(7.65290158847099,15.2,7.01912907727743));
#208396=CARTESIAN_POINT('Ctrl Pts',(7.65425083044716,15.2,7.02063486218735));
#208397=CARTESIAN_POINT('Ctrl Pts',(7.65560007230076,15.2,7.0221406469605));
#208398=CARTESIAN_POINT('Ctrl Pts',(7.65698209060125,15.2,7.02369206276625));
#208399=CARTESIAN_POINT('Ctrl Pts',(7.65839580954989,15.2,7.02528884145824));
#208400=CARTESIAN_POINT('Ctrl Pts',(7.65980952849853,15.2,7.02688562015022));
#208401=CARTESIAN_POINT('Ctrl Pts',(7.6612549458305,15.2,7.02852776000807));
#208402=CARTESIAN_POINT('Ctrl Pts',(7.66273101409884,15.2,7.0302149976118));
#208403=CARTESIAN_POINT('Ctrl Pts',(7.66420708250127,15.2,7.03190223536877));
#208404=CARTESIAN_POINT('Ctrl Pts',(7.66571380242329,15.2,7.03363456911039));
#208405=CARTESIAN_POINT('Ctrl Pts',(7.6672501549257,15.2,7.03541173821029));
#208406=CARTESIAN_POINT('Ctrl Pts',(7.66904256596918,15.2,7.03748510191804));
#208407=CARTESIAN_POINT('Ctrl Pts',(7.67087531161421,15.2,7.03961949183139));
#208408=CARTESIAN_POINT('Ctrl Pts',(7.67274682060312,15.2,7.04181450134301));
#208409=CARTESIAN_POINT('Ctrl Pts',(7.67435097135238,15.2,7.04369593828699));
#208410=CARTESIAN_POINT('Ctrl Pts',(7.67598360497184,15.2,7.04562191207094));
#208411=CARTESIAN_POINT('Ctrl Pts',(7.67764376073086,15.2,7.04759217001468));
#208412=CARTESIAN_POINT('Ctrl Pts',(7.67930391633907,15.2,7.04956242777943));
#208413=CARTESIAN_POINT('Ctrl Pts',(7.68099159523845,15.2,7.05157697021619));
#208414=CARTESIAN_POINT('Ctrl Pts',(7.68270586501735,15.2,7.05363554898419));
#208415=CARTESIAN_POINT('Ctrl Pts',(7.68442013479623,15.2,7.05569412775218));
#208416=CARTESIAN_POINT('Ctrl Pts',(7.68616099674403,15.2,7.05779674259635));
#208417=CARTESIAN_POINT('Ctrl Pts',(7.6879275415954,15.2,7.05994315018312));
#208418=CARTESIAN_POINT('Ctrl Pts',(7.68969408660722,15.2,7.06208955796485));
#208419=CARTESIAN_POINT('Ctrl Pts',(7.69148631527225,15.2,7.06427975580202));
#208420=CARTESIAN_POINT('Ctrl Pts',(7.69330334245629,15.2,7.06651350476006));
#208421=CARTESIAN_POINT('Ctrl Pts',(7.6951203694753,15.2,7.06874725351521));
#208422=CARTESIAN_POINT('Ctrl Pts',(7.69696219657678,15.2,7.07102455272568));
#208423=CARTESIAN_POINT('Ctrl Pts',(7.69882796059335,15.2,7.07334516364323));
#208424=CARTESIAN_POINT('Ctrl Pts',(7.70069372460993,15.2,7.07566577456079));
#208425=CARTESIAN_POINT('Ctrl Pts',(7.70258342734961,15.2,7.07802969765826));
#208426=CARTESIAN_POINT('Ctrl Pts',(7.70449622661242,15.2,7.08043669840224));
#208427=CARTESIAN_POINT('Ctrl Pts',(7.70640902587525,15.2,7.08284369914623));
#208428=CARTESIAN_POINT('Ctrl Pts',(7.70834492374246,15.2,7.08529377607167));
#208429=CARTESIAN_POINT('Ctrl Pts',(7.71030309983647,15.2,7.08778669797819));
#208430=CARTESIAN_POINT('Ctrl Pts',(7.71226127610836,15.2,7.09027962011115));
#208431=CARTESIAN_POINT('Ctrl Pts',(7.71424172989907,15.2,7.09281538834824));
#208432=CARTESIAN_POINT('Ctrl Pts',(7.71624366334244,15.2,7.09539376965728));
#208433=CARTESIAN_POINT('Ctrl Pts',(7.71824559660397,15.2,7.09797215073212));
#208434=CARTESIAN_POINT('Ctrl Pts',(7.72026900951376,15.2,7.10059314884522));
#208435=CARTESIAN_POINT('Ctrl Pts',(7.72231311993859,15.2,7.10325653466326));
#208436=CARTESIAN_POINT('Ctrl Pts',(7.7243572303634,15.2,7.10591992048131));
#208437=CARTESIAN_POINT('Ctrl Pts',(7.72642203988311,15.2,7.1086256945531));
#208438=CARTESIAN_POINT('Ctrl Pts',(7.72850678630601,15.2,7.1113736324504));
#208439=CARTESIAN_POINT('Ctrl Pts',(7.73059153291828,15.2,7.1141215705973));
#208440=CARTESIAN_POINT('Ctrl Pts',(7.73269621517416,15.2,7.1169116723566));
#208441=CARTESIAN_POINT('Ctrl Pts',(7.73482009087407,15.2,7.11974371642943));
#208442=CARTESIAN_POINT('Ctrl Pts',(7.73694396638108,15.2,7.12257576024503));
#208443=CARTESIAN_POINT('Ctrl Pts',(7.73908703397603,15.2,7.12544974549974));
#208444=CARTESIAN_POINT('Ctrl Pts',(7.7412485664906,15.2,7.12836545249026));
#208445=CARTESIAN_POINT('Ctrl Pts',(7.74341009900516,15.2,7.13128115948078));
#208446=CARTESIAN_POINT('Ctrl Pts',(7.74559009592475,15.2,7.13423858848483));
#208447=CARTESIAN_POINT('Ctrl Pts',(7.74778784751036,15.2,7.13723752237304));
#208448=CARTESIAN_POINT('Ctrl Pts',(7.7499855992956,15.2,7.14023645653366));
#208449=CARTESIAN_POINT('Ctrl Pts',(7.7522011038984,15.2,7.14327689414883));
#208450=CARTESIAN_POINT('Ctrl Pts',(7.75443366796593,15.2,7.14635862055647));
#208451=CARTESIAN_POINT('Ctrl Pts',(7.75666623183067,15.2,7.14944034668418));
#208452=CARTESIAN_POINT('Ctrl Pts',(7.7589158527489,15.2,7.15256336313987));
#208453=CARTESIAN_POINT('Ctrl Pts',(7.76118185349991,15.2,7.15572745127491));
#208454=CARTESIAN_POINT('Ctrl Pts',(7.76344785425091,15.2,7.15889153940994));
#208455=CARTESIAN_POINT('Ctrl Pts',(7.76573023273056,15.2,7.16209670508579));
#208456=CARTESIAN_POINT('Ctrl Pts',(7.76802832376098,15.2,7.16534273221101));
#208457=CARTESIAN_POINT('Ctrl Pts',(7.76994339968924,15.2,7.16804775491364));
#208458=CARTESIAN_POINT('Ctrl Pts',(7.77186938791277,15.2,7.17078115509872));
#208459=CARTESIAN_POINT('Ctrl Pts',(7.77380591110667,15.2,7.17354281086114));
#208460=CARTESIAN_POINT('Ctrl Pts',(7.77574243430056,15.2,7.17630446662355));
#208461=CARTESIAN_POINT('Ctrl Pts',(7.77768948963916,15.2,7.17909437795613));
#208462=CARTESIAN_POINT('Ctrl Pts',(7.77964670963864,15.2,7.18191242302411));
#208463=CARTESIAN_POINT('Ctrl Pts',(7.78160392963811,15.2,7.18473046809209));
#208464=CARTESIAN_POINT('Ctrl Pts',(7.78357131293987,15.2,7.18757664774091));
#208465=CARTESIAN_POINT('Ctrl Pts',(7.78554849399051,15.2,7.19045084199002));
#208466=CARTESIAN_POINT('Ctrl Pts',(7.78792111116508,15.2,7.19389987496365));
#208467=CARTESIAN_POINT('Ctrl Pts',(7.79030783790979,15.2,7.19738924908786));
#208468=CARTESIAN_POINT('Ctrl Pts',(7.7927080559883,15.2,7.20091875887354));
#208469=CARTESIAN_POINT('Ctrl Pts',(7.79470823779308,15.2,7.20386001713514));
#208470=CARTESIAN_POINT('Ctrl Pts',(7.79671778842654,15.2,7.20682914547103));
#208471=CARTESIAN_POINT('Ctrl Pts',(7.79873635699896,15.2,7.20982602811878));
#208472=CARTESIAN_POINT('Ctrl Pts',(7.80115863941788,15.2,7.21342228749208));
#208473=CARTESIAN_POINT('Ctrl Pts',(7.80359390730747,15.2,7.21705851078088));
#208474=CARTESIAN_POINT('Ctrl Pts',(7.80604156552505,15.2,7.22073449515061));
#208475=CARTESIAN_POINT('Ctrl Pts',(7.80808128059522,15.2,7.22379781529177));
#208476=CARTESIAN_POINT('Ctrl Pts',(7.81012959882382,15.2,7.22688874835002));
#208477=CARTESIAN_POINT('Ctrl Pts',(7.81218618326893,15.2,7.23000717515781));
#208478=CARTESIAN_POINT('Ctrl Pts',(7.81424276748988,15.2,7.23312560162571));
#208479=CARTESIAN_POINT('Ctrl Pts',(7.81630761717762,15.2,7.23627152447745));
#208480=CARTESIAN_POINT('Ctrl Pts',(7.81838039972881,15.2,7.23944482510153));
#208481=CARTESIAN_POINT('Ctrl Pts',(7.82045318250593,15.2,7.2426181260715));
#208482=CARTESIAN_POINT('Ctrl Pts',(7.82253389826626,15.2,7.24581880747434));
#208483=CARTESIAN_POINT('Ctrl Pts',(7.82462221854344,15.2,7.24904675011104));
#208484=CARTESIAN_POINT('Ctrl Pts',(7.82671053882061,15.2,7.25227469274774));
#208485=CARTESIAN_POINT('Ctrl Pts',(7.82880646325679,15.2,7.25552990007356));
#208486=CARTESIAN_POINT('Ctrl Pts',(7.83090967197247,15.2,7.25881225461065));
#208487=CARTESIAN_POINT('Ctrl Pts',(7.83301288068813,15.2,7.26209460914773));
#208488=CARTESIAN_POINT('Ctrl Pts',(7.83512337073404,15.2,7.26540411328326));
#208489=CARTESIAN_POINT('Ctrl Pts',(7.83724082684483,15.2,7.26874065078187));
#208490=CARTESIAN_POINT('Ctrl Pts',(7.83935828295559,15.2,7.2720771882805));
#208491=CARTESIAN_POINT('Ctrl Pts',(7.84148270336094,15.2,7.27544075927419));
#208492=CARTESIAN_POINT('Ctrl Pts',(7.8436137771106,15.2,7.27883125024501));
#208493=CARTESIAN_POINT('Ctrl Pts',(7.84617106574955,15.2,7.28289983963172));
#208494=CARTESIAN_POINT('Ctrl Pts',(7.8487379355647,15.2,7.28700719500659));
#208495=CARTESIAN_POINT('Ctrl Pts',(7.85131385328905,15.2,7.29115311923518));
#208496=CARTESIAN_POINT('Ctrl Pts',(7.8534604510417,15.2,7.29460805552745));
#208497=CARTESIAN_POINT('Ctrl Pts',(7.85561333416446,15.2,7.29808977485895));
#208498=CARTESIAN_POINT('Ctrl Pts',(7.85777219948422,15.2,7.3015981678077));
#208499=CARTESIAN_POINT('Ctrl Pts',(7.8599310650393,15.2,7.30510656113886));
#208500=CARTESIAN_POINT('Ctrl Pts',(7.86209591267761,15.2,7.30864162479734));
#208501=CARTESIAN_POINT('Ctrl Pts',(7.86426644573269,15.2,7.3122032482674));
#208502=CARTESIAN_POINT('Ctrl Pts',(7.8660028722714,15.2,7.31505254719872));
#208503=CARTESIAN_POINT('Ctrl Pts',(7.86774293662873,15.2,7.31791884480106));
#208504=CARTESIAN_POINT('Ctrl Pts',(7.86948649100946,15.2,7.32080208302689));
#208505=CARTESIAN_POINT('Ctrl Pts',(7.87210182234299,15.2,7.3251269399728));
#208506=CARTESIAN_POINT('Ctrl Pts',(7.87472499953583,15.2,7.32948991477177));
#208507=CARTESIAN_POINT('Ctrl Pts',(7.8773555281066,15.2,7.3338908137769));
#208508=CARTESIAN_POINT('Ctrl Pts',(7.87954763532857,15.2,7.33755822974776));
#208509=CARTESIAN_POINT('Ctrl Pts',(7.88174484555065,15.2,7.34125198203039));
#208510=CARTESIAN_POINT('Ctrl Pts',(7.88394687610595,15.2,7.34497196126512));
#208511=CARTESIAN_POINT('Ctrl Pts',(7.88570850064619,15.2,7.3479479448151));
#208512=CARTESIAN_POINT('Ctrl Pts',(7.88747320806044,15.2,7.35094071321255));
#208513=CARTESIAN_POINT('Ctrl Pts',(7.88924085802311,15.2,7.35395020969504));
#208514=CARTESIAN_POINT('Ctrl Pts',(7.89100850774494,15.2,7.35695970576748));
#208515=CARTESIAN_POINT('Ctrl Pts',(7.89277909921404,15.2,7.35998593028729));
#208516=CARTESIAN_POINT('Ctrl Pts',(7.89455248834665,15.2,7.36302882675965));
#208517=CARTESIAN_POINT('Ctrl Pts',(7.89632587772089,15.2,7.3660717236466));
#208518=CARTESIAN_POINT('Ctrl Pts',(7.89810206741491,15.2,7.36913129288557));
#208519=CARTESIAN_POINT('Ctrl Pts',(7.89988091417871,15.2,7.37220747777655));
#208520=CARTESIAN_POINT('Ctrl Pts',(7.90165976070015,15.2,7.37528366224841));
#208521=CARTESIAN_POINT('Ctrl Pts',(7.90344126715913,15.2,7.37837646275746));
#208522=CARTESIAN_POINT('Ctrl Pts',(7.90522529299107,15.2,7.38148582282382));
#208523=CARTESIAN_POINT('Ctrl Pts',(7.9074553254633,15.2,7.38537252322448));
#208524=CARTESIAN_POINT('Ctrl Pts',(7.90968929562603,15.2,7.38928510072164));
#208525=CARTESIAN_POINT('Ctrl Pts',(7.91192693465361,15.2,7.39322344252584));
#208526=CARTESIAN_POINT('Ctrl Pts',(7.91371704597325,15.2,7.39637411614091));
#208527=CARTESIAN_POINT('Ctrl Pts',(7.91550950582929,15.2,7.39954128067188));
#208528=CARTESIAN_POINT('Ctrl Pts',(7.91730417987167,15.2,7.40272488023533));
#208529=CARTESIAN_POINT('Ctrl Pts',(7.91909885366954,15.2,7.40590847936502));
#208530=CARTESIAN_POINT('Ctrl Pts',(7.9208957400185,15.2,7.40910851331197));
#208531=CARTESIAN_POINT('Ctrl Pts',(7.9226947077389,15.2,7.41232492604162));
#208532=CARTESIAN_POINT('Ctrl Pts',(7.92494341757323,15.2,7.41634544228235));
#208533=CARTESIAN_POINT('Ctrl Pts',(7.92719537543041,15.2,7.42039155281845));
#208534=CARTESIAN_POINT('Ctrl Pts',(7.92945032536082,15.2,7.42446314719213));
#208535=CARTESIAN_POINT('Ctrl Pts',(7.93125428540345,15.2,7.42772042286859));
#208536=CARTESIAN_POINT('Ctrl Pts',(7.93306015981854,15.2,7.43099400908866));
#208537=CARTESIAN_POINT('Ctrl Pts',(7.9348678186394,15.2,7.43428385126902));
#208538=CARTESIAN_POINT('Ctrl Pts',(7.93667547721397,15.2,7.43757369300114));
#208539=CARTESIAN_POINT('Ctrl Pts',(7.93848492120874,15.2,7.44087978993051));
#208540=CARTESIAN_POINT('Ctrl Pts',(7.94029601976215,15.2,7.44420208726793));
#208541=CARTESIAN_POINT('Ctrl Pts',(7.94210711856231,15.2,7.44752438505801));
#208542=CARTESIAN_POINT('Ctrl Pts',(7.94391987284929,15.2,7.45086288371266));
#208543=CARTESIAN_POINT('Ctrl Pts',(7.94573415494827,15.2,7.45421752800765));
#208544=CARTESIAN_POINT('Ctrl Pts',(7.94754843680006,15.2,7.45757217184558));
#208545=CARTESIAN_POINT('Ctrl Pts',(7.94936424484875,15.2,7.46094296144694));
#208546=CARTESIAN_POINT('Ctrl Pts',(7.95118145597783,15.2,7.46432984194618));
#208547=CARTESIAN_POINT('Ctrl Pts',(7.95299866735449,15.2,7.46771672290688));
#208548=CARTESIAN_POINT('Ctrl Pts',(7.95481728007706,15.2,7.47111969545868));
#208549=CARTESIAN_POINT('Ctrl Pts',(7.95663716951785,15.2,7.47453870449392));
#208550=CARTESIAN_POINT('Ctrl Pts',(7.95845705871067,15.2,7.47795771306332));
#208551=CARTESIAN_POINT('Ctrl Pts',(7.96027822463998,15.2,7.48139275892224));
#208552=CARTESIAN_POINT('Ctrl Pts',(7.96210054326866,15.2,7.48484378669402));
#208553=CARTESIAN_POINT('Ctrl Pts',(7.96437844174071,15.2,7.48915757176139));
#208554=CARTESIAN_POINT('Ctrl Pts',(7.96665814236277,15.2,7.49349632912564));
#208555=CARTESIAN_POINT('Ctrl Pts',(7.96893940645989,15.2,7.49785995342917));
#208556=CARTESIAN_POINT('Ctrl Pts',(7.97076441783703,15.2,7.50135085306225));
#208557=CARTESIAN_POINT('Ctrl Pts',(7.97259042916554,15.2,7.50485766761928));
#208558=CARTESIAN_POINT('Ctrl Pts',(7.97441732071785,15.2,7.508380341994));
#208559=CARTESIAN_POINT('Ctrl Pts',(7.97624421202125,15.2,7.51190301588875));
#208560=CARTESIAN_POINT('Ctrl Pts',(7.97807198399497,15.2,7.51544155213318));
#208561=CARTESIAN_POINT('Ctrl Pts',(7.97990051540098,15.2,7.51899589395213));
#208562=CARTESIAN_POINT('Ctrl Pts',(7.98218617984534,15.2,7.52343882158902));
#208563=CARTESIAN_POINT('Ctrl Pts',(7.98447303585634,15.2,7.52790644667549));
#208564=CARTESIAN_POINT('Ctrl Pts',(7.98676084696736,15.2,7.53239866514568));
#208565=CARTESIAN_POINT('Ctrl Pts',(7.98859109595593,15.2,7.53599244011769));
#208566=CARTESIAN_POINT('Ctrl Pts',(7.99042195878624,15.2,7.53960195463566));
#208567=CARTESIAN_POINT('Ctrl Pts',(7.99225331827494,15.2,7.54322715549992));
#208568=CARTESIAN_POINT('Ctrl Pts',(7.99454251751107,15.2,7.54775865633328));
#208569=CARTESIAN_POINT('Ctrl Pts',(7.99683249171299,15.2,7.55231466662041));
#208570=CARTESIAN_POINT('Ctrl Pts',(7.99912301700119,15.2,7.55689508025243));
#208571=CARTESIAN_POINT('Ctrl Pts',(8.00095543708196,15.2,7.56055941085848));
#208572=CARTESIAN_POINT('Ctrl Pts',(8.00278820967234,15.2,7.56423936111329));
#208573=CARTESIAN_POINT('Ctrl Pts',(8.00462122096691,15.2,7.56793487742072));
#208574=CARTESIAN_POINT('Ctrl Pts',(8.00645423251124,15.2,7.57163039423166));
#208575=CARTESIAN_POINT('Ctrl Pts',(8.00828748172504,15.2,7.57534147510519));
#208576=CARTESIAN_POINT('Ctrl Pts',(8.01012085799161,15.2,7.57906806947492));
#208577=CARTESIAN_POINT('Ctrl Pts',(8.01195423425818,15.2,7.58279466384465));
#208578=CARTESIAN_POINT('Ctrl Pts',(8.01378773636091,15.2,7.58653677044127));
#208579=CARTESIAN_POINT('Ctrl Pts',(8.01562125201639,15.2,7.59029433664763));
#208580=CARTESIAN_POINT('Ctrl Pts',(8.0183715252498,15.2,7.59593068544521));
#208581=CARTESIAN_POINT('Ctrl Pts',(8.02112183180807,15.2,7.60160181655014));
#208582=CARTESIAN_POINT('Ctrl Pts',(8.02387179612482,15.2,7.60730755251103));
#208583=CARTESIAN_POINT('Ctrl Pts',(8.0261634331387,15.2,7.6120623326512));
#208584=CARTESIAN_POINT('Ctrl Pts',(8.02845483368311,15.2,7.61684114351289));
#208585=CARTESIAN_POINT('Ctrl Pts',(8.03074578639144,15.2,7.62164388205583));
#208586=CARTESIAN_POINT('Ctrl Pts',(8.03303673909975,15.2,7.62644662059878));
#208587=CARTESIAN_POINT('Ctrl Pts',(8.03532724145141,15.2,7.63127328592465));
#208588=CARTESIAN_POINT('Ctrl Pts',(8.03761708677409,15.2,7.63612377707141));
#208589=CARTESIAN_POINT('Ctrl Pts',(8.03944896288249,15.2,7.64000416967159));
#208590=CARTESIAN_POINT('Ctrl Pts',(8.04128041833601,15.2,7.6438998091205));
#208591=CARTESIAN_POINT('Ctrl Pts',(8.04311134457526,15.2,7.64781064418869));
#208592=CARTESIAN_POINT('Ctrl Pts',(8.04494227106398,15.2,7.65172147978973));
#208593=CARTESIAN_POINT('Ctrl Pts',(8.04677267057764,15.2,7.65564750984538));
#208594=CARTESIAN_POINT('Ctrl Pts',(8.04860243689952,15.2,7.65958868283892));
#208595=CARTESIAN_POINT('Ctrl Pts',(8.05134708613306,15.2,7.66550044179226));
#208596=CARTESIAN_POINT('Ctrl Pts',(8.05409031275252,15.2,7.67144627239573));
#208597=CARTESIAN_POINT('Ctrl Pts',(8.0568317629987,15.2,7.67742599545555));
#208598=CARTESIAN_POINT('Ctrl Pts',(8.05865939666216,15.2,7.68141247785753));
#208599=CARTESIAN_POINT('Ctrl Pts',(8.06048624151297,15.2,7.68541402431124));
#208600=CARTESIAN_POINT('Ctrl Pts',(8.06231219522349,15.2,7.68943058269832));
#208601=CARTESIAN_POINT('Ctrl Pts',(8.06413814868524,15.2,7.69344714053815));
#208602=CARTESIAN_POINT('Ctrl Pts',(8.06596321081376,15.2,7.69747871027327));
#208603=CARTESIAN_POINT('Ctrl Pts',(8.06778727960916,15.2,7.70152523871927));
#208604=CARTESIAN_POINT('Ctrl Pts',(8.06915533126784,15.2,7.7045601351916));
#208605=CARTESIAN_POINT('Ctrl Pts',(8.07052282405012,15.2,7.70760344580231));
#208606=CARTESIAN_POINT('Ctrl Pts',(8.07188971627715,15.2,7.71065515038458));
#208607=CARTESIAN_POINT('Ctrl Pts',(8.07371223941205,15.2,7.7147240901972));
#208608=CARTESIAN_POINT('Ctrl Pts',(8.07553369338018,15.2,7.71880795058581));
#208609=CARTESIAN_POINT('Ctrl Pts',(8.07735397842375,15.2,7.72290667831014));
#208610=CARTESIAN_POINT('Ctrl Pts',(8.07871919208242,15.2,7.72598072382416));
#208611=CARTESIAN_POINT('Ctrl Pts',(8.08008374884951,15.2,7.72906313201222));
#208612=CARTESIAN_POINT('Ctrl Pts',(8.08144760604995,15.2,7.73215388248325));
#208613=CARTESIAN_POINT('Ctrl Pts',(8.0828114632504,15.2,7.73524463295429));
#208614=CARTESIAN_POINT('Ctrl Pts',(8.08417462135087,15.2,7.73834372514165));
#208615=CARTESIAN_POINT('Ctrl Pts',(8.08553703813477,15.2,7.74145113661136));
#208616=CARTESIAN_POINT('Ctrl Pts',(8.08735359401163,15.2,7.74559435228064));
#208617=CARTESIAN_POINT('Ctrl Pts',(8.08916883383769,15.2,7.74975235797114));
#208618=CARTESIAN_POINT('Ctrl Pts',(8.0909826583048,15.2,7.75392510379717));
#208619=CARTESIAN_POINT('Ctrl Pts',(8.09234302653157,15.2,7.75705466288243));
#208620=CARTESIAN_POINT('Ctrl Pts',(8.09370259849747,15.2,7.7601925120899));
#208621=CARTESIAN_POINT('Ctrl Pts',(8.09506133465637,15.2,7.76333862914299));
#208622=CARTESIAN_POINT('Ctrl Pts',(8.09642007081527,15.2,7.76648474619608));
#208623=CARTESIAN_POINT('Ctrl Pts',(8.09777797033258,15.2,7.76963913238148));
#208624=CARTESIAN_POINT('Ctrl Pts',(8.09913499253328,15.2,7.77280176493325));
#208625=CARTESIAN_POINT('Ctrl Pts',(8.10139669628329,15.2,7.77807281937772));
#208626=CARTESIAN_POINT('Ctrl Pts',(8.10365596275761,15.2,7.78336678309528));
#208627=CARTESIAN_POINT('Ctrl Pts',(8.10591260651785,15.2,7.78868355249449));
#208628=CARTESIAN_POINT('Ctrl Pts',(8.1072665927248,15.2,7.79187361401812));
#208629=CARTESIAN_POINT('Ctrl Pts',(8.10861963502502,15.2,7.79507188673231));
#208630=CARTESIAN_POINT('Ctrl Pts',(8.10997169277373,15.2,7.79827834775536));
#208631=CARTESIAN_POINT('Ctrl Pts',(8.11132375052243,15.2,7.80148480877841));
#208632=CARTESIAN_POINT('Ctrl Pts',(8.11267482410175,15.2,7.80469945891659));
#208633=CARTESIAN_POINT('Ctrl Pts',(8.11402487434444,15.2,7.80792227588211));
#208634=CARTESIAN_POINT('Ctrl Pts',(8.11537492458714,15.2,7.81114509284762));
#208635=CARTESIAN_POINT('Ctrl Pts',(8.11672395120493,15.2,7.81437607634594));
#208636=CARTESIAN_POINT('Ctrl Pts',(8.1180719149061,15.2,7.81761520581047));
#208637=CARTESIAN_POINT('Ctrl Pts',(8.11941987885214,15.2,7.82085433586344));
#208638=CARTESIAN_POINT('Ctrl Pts',(8.12076677941457,15.2,7.8241016112854));
#208639=CARTESIAN_POINT('Ctrl Pts',(8.12211257877667,15.2,7.82735700992628));
#208640=CARTESIAN_POINT('Ctrl Pts',(8.12345837789428,15.2,7.83061240797576));
#208641=CARTESIAN_POINT('Ctrl Pts',(8.12480307402504,15.2,7.83387593048748));
#208642=CARTESIAN_POINT('Ctrl Pts',(8.12614663025155,15.2,7.83714755511632));
#208643=CARTESIAN_POINT('Ctrl Pts',(8.12749018647806,15.2,7.84041917974517));
#208644=CARTESIAN_POINT('Ctrl Pts',(8.12883260144497,15.2,7.84369890614386));
#208645=CARTESIAN_POINT('Ctrl Pts',(8.13017383764613,15.2,7.84698671310843));
#208646=CARTESIAN_POINT('Ctrl Pts',(8.13151507384729,15.2,7.850274520073));
#208647=CARTESIAN_POINT('Ctrl Pts',(8.13285513018193,15.2,7.85357040723663));
#208648=CARTESIAN_POINT('Ctrl Pts',(8.13419396946662,15.2,7.8568743532416));
#208649=CARTESIAN_POINT('Ctrl Pts',(8.13597908867503,15.2,7.86127961498171));
#208650=CARTESIAN_POINT('Ctrl Pts',(8.13776204510261,15.2,7.86569920457345));
#208651=CARTESIAN_POINT('Ctrl Pts',(8.13954274503276,15.2,7.8701330689832));
#208652=CARTESIAN_POINT('Ctrl Pts',(8.14087826985906,15.2,7.87345846698845));
#208653=CARTESIAN_POINT('Ctrl Pts',(8.14221252711043,15.2,7.87679189515166));
#208654=CARTESIAN_POINT('Ctrl Pts',(8.14354547885356,15.2,7.8801333321143));
#208655=CARTESIAN_POINT('Ctrl Pts',(8.1448784305967,15.2,7.88347476907694));
#208656=CARTESIAN_POINT('Ctrl Pts',(8.14621007626013,15.2,7.88682421450968));
#208657=CARTESIAN_POINT('Ctrl Pts',(8.14754037946783,15.2,7.89018164702799));
#208658=CARTESIAN_POINT('Ctrl Pts',(8.14931411699755,15.2,7.89465822351574));
#208659=CARTESIAN_POINT('Ctrl Pts',(8.15108546735234,15.2,7.89914899940261));
#208660=CARTESIAN_POINT('Ctrl Pts',(8.15285434048574,15.2,7.90365392375505));
#208661=CARTESIAN_POINT('Ctrl Pts',(8.15418099563705,15.2,7.90703261778661));
#208662=CARTESIAN_POINT('Ctrl Pts',(8.15550625964635,15.2,7.91041926964552));
#208663=CARTESIAN_POINT('Ctrl Pts',(8.15683009325522,15.2,7.9138138587233));
#208664=CARTESIAN_POINT('Ctrl Pts',(8.1581539266236,15.2,7.91720844718438));
#208665=CARTESIAN_POINT('Ctrl Pts',(8.15947633082536,15.2,7.92061097266167));
#208666=CARTESIAN_POINT('Ctrl Pts',(8.16079726911058,15.2,7.92402141362181));
#208667=CARTESIAN_POINT('Ctrl Pts',(8.1621182073958,15.2,7.92743185458195));
#208668=CARTESIAN_POINT('Ctrl Pts',(8.16343767999306,15.2,7.9308502113286));
#208669=CARTESIAN_POINT('Ctrl Pts',(8.16475565074282,15.2,7.93427646230306));
#208670=CARTESIAN_POINT('Ctrl Pts',(8.16607362149259,15.2,7.93770271327752));
#208671=CARTESIAN_POINT('Ctrl Pts',(8.16739009017389,15.2,7.94113685797293));
#208672=CARTESIAN_POINT('Ctrl Pts',(8.16870501950709,15.2,7.94457887544681));
#208673=CARTESIAN_POINT('Ctrl Pts',(8.1700199488403,15.2,7.94802089292069));
#208674=CARTESIAN_POINT('Ctrl Pts',(8.17133334032114,15.2,7.95147078323282));
#208675=CARTESIAN_POINT('Ctrl Pts',(8.17264515714861,15.2,7.95492852468983));
#208676=CARTESIAN_POINT('Ctrl Pts',(8.17395697397607,15.2,7.95838626614683));
#208677=CARTESIAN_POINT('Ctrl Pts',(8.17526721667867,15.2,7.96185185847002));
#208678=CARTESIAN_POINT('Ctrl Pts',(8.17657585046467,15.2,7.96532528146773));
#208679=CARTESIAN_POINT('Ctrl Pts',(8.1778844844884,15.2,7.96879870509643));
#208680=CARTESIAN_POINT('Ctrl Pts',(8.17919150906171,15.2,7.97227995908574));
#208681=CARTESIAN_POINT('Ctrl Pts',(8.18049688904286,15.2,7.97576902126055));
#208682=CARTESIAN_POINT('Ctrl Pts',(8.18180226878687,15.2,7.97925808280151));
#208683=CARTESIAN_POINT('Ctrl Pts',(8.18310600338431,15.2,7.98275495389608));
#208684=CARTESIAN_POINT('Ctrl Pts',(8.18440805577685,15.2,7.98625961065307));
#208685=CARTESIAN_POINT('Ctrl Pts',(8.1857101081694,15.2,7.98976426741006));
#208686=CARTESIAN_POINT('Ctrl Pts',(8.18701047855548,15.2,7.99327671097764));
#208687=CARTESIAN_POINT('Ctrl Pts',(8.18830913438315,15.2,7.99679692010043));
#208688=CARTESIAN_POINT('Ctrl Pts',(8.18960779021083,15.2,8.00031712922324));
#208689=CARTESIAN_POINT('Ctrl Pts',(8.19090473074702,15.2,8.00384510591173));
#208690=CARTESIAN_POINT('Ctrl Pts',(8.19219992599163,15.2,8.00738082844994));
#208691=CARTESIAN_POINT('Ctrl Pts',(8.19349512123624,15.2,8.01091655098815));
#208692=CARTESIAN_POINT('Ctrl Pts',(8.1947885704559,15.2,8.01446002097602));
#208693=CARTESIAN_POINT('Ctrl Pts',(8.19608023411747,15.2,8.01801121384631));
#208694=CARTESIAN_POINT('Ctrl Pts',(8.19737189777903,15.2,8.02156240671661));
#208695=CARTESIAN_POINT('Ctrl Pts',(8.19866177483297,15.2,8.0251213215956));
#208696=CARTESIAN_POINT('Ctrl Pts',(8.1999498242674,15.2,8.02868793330996));
#208697=CARTESIAN_POINT('Ctrl Pts',(8.20123787370183,15.2,8.03225454502431));
#208698=CARTESIAN_POINT('Ctrl Pts',(8.20252409519971,15.2,8.03582885366694));
#208699=CARTESIAN_POINT('Ctrl Pts',(8.20380846548663,15.2,8.03941084395239));
#208700=CARTESIAN_POINT('Ctrl Pts',(8.20552095935807,15.2,8.04418683143348));
#208701=CARTESIAN_POINT('Ctrl Pts',(8.20723015620175,15.2,8.04897647635775));
#208702=CARTESIAN_POINT('Ctrl Pts',(8.20893606999994,15.2,8.05377977099998));
#208703=CARTESIAN_POINT('Ctrl Pts',(7.64657512299994,12.2,7.01216898699998));
#208704=CARTESIAN_POINT('Ctrl Pts',(7.64778328654791,12.2,7.01348522668636));
#208705=CARTESIAN_POINT('Ctrl Pts',(7.64902613283499,12.2,7.0148472224676));
#208706=CARTESIAN_POINT('Ctrl Pts',(7.65030255111842,12.2,7.01625467982076));
#208707=CARTESIAN_POINT('Ctrl Pts',(7.651585124936,12.2,7.01766892464472));
#208708=CARTESIAN_POINT('Ctrl Pts',(7.65290158847099,12.2,7.01912907727743));
#208709=CARTESIAN_POINT('Ctrl Pts',(7.65425083044716,12.2,7.02063486218735));
#208710=CARTESIAN_POINT('Ctrl Pts',(7.65560007230076,12.2,7.0221406469605));
#208711=CARTESIAN_POINT('Ctrl Pts',(7.65698209060125,12.2,7.02369206276625));
#208712=CARTESIAN_POINT('Ctrl Pts',(7.65839580954989,12.2,7.02528884145824));
#208713=CARTESIAN_POINT('Ctrl Pts',(7.65980952849853,12.2,7.02688562015022));
#208714=CARTESIAN_POINT('Ctrl Pts',(7.6612549458305,12.2,7.02852776000807));
#208715=CARTESIAN_POINT('Ctrl Pts',(7.66273101409884,12.2,7.0302149976118));
#208716=CARTESIAN_POINT('Ctrl Pts',(7.66420708250127,12.2,7.03190223536877));
#208717=CARTESIAN_POINT('Ctrl Pts',(7.66571380242329,12.2,7.03363456911039));
#208718=CARTESIAN_POINT('Ctrl Pts',(7.6672501549257,12.2,7.0354117382103));
#208719=CARTESIAN_POINT('Ctrl Pts',(7.66904256596918,12.2,7.03748510191804));
#208720=CARTESIAN_POINT('Ctrl Pts',(7.67087531161421,12.2,7.03961949183139));
#208721=CARTESIAN_POINT('Ctrl Pts',(7.67274682060312,12.2,7.04181450134301));
#208722=CARTESIAN_POINT('Ctrl Pts',(7.67435097135238,12.2,7.04369593828699));
#208723=CARTESIAN_POINT('Ctrl Pts',(7.67598360497184,12.2,7.04562191207094));
#208724=CARTESIAN_POINT('Ctrl Pts',(7.67764376073086,12.2,7.04759217001468));
#208725=CARTESIAN_POINT('Ctrl Pts',(7.67930391633907,12.2,7.04956242777943));
#208726=CARTESIAN_POINT('Ctrl Pts',(7.68099159523845,12.2,7.0515769702162));
#208727=CARTESIAN_POINT('Ctrl Pts',(7.68270586501735,12.2,7.05363554898419));
#208728=CARTESIAN_POINT('Ctrl Pts',(7.68442013479623,12.2,7.05569412775218));
#208729=CARTESIAN_POINT('Ctrl Pts',(7.68616099674403,12.2,7.05779674259634));
#208730=CARTESIAN_POINT('Ctrl Pts',(7.6879275415954,12.2,7.05994315018311));
#208731=CARTESIAN_POINT('Ctrl Pts',(7.68969408660721,12.2,7.06208955796484));
#208732=CARTESIAN_POINT('Ctrl Pts',(7.69148631527225,12.2,7.06427975580202));
#208733=CARTESIAN_POINT('Ctrl Pts',(7.69330334245629,12.2,7.06651350476006));
#208734=CARTESIAN_POINT('Ctrl Pts',(7.6951203694753,12.2,7.06874725351521));
#208735=CARTESIAN_POINT('Ctrl Pts',(7.69696219657678,12.2,7.07102455272568));
#208736=CARTESIAN_POINT('Ctrl Pts',(7.69882796059335,12.2,7.07334516364323));
#208737=CARTESIAN_POINT('Ctrl Pts',(7.70069372460993,12.2,7.07566577456079));
#208738=CARTESIAN_POINT('Ctrl Pts',(7.7025834273496,12.2,7.07802969765826));
#208739=CARTESIAN_POINT('Ctrl Pts',(7.70449622661242,12.2,7.08043669840224));
#208740=CARTESIAN_POINT('Ctrl Pts',(7.70640902587524,12.2,7.08284369914623));
#208741=CARTESIAN_POINT('Ctrl Pts',(7.70834492374246,12.2,7.08529377607167));
#208742=CARTESIAN_POINT('Ctrl Pts',(7.71030309983647,12.2,7.08778669797819));
#208743=CARTESIAN_POINT('Ctrl Pts',(7.71226127610836,12.2,7.09027962011115));
#208744=CARTESIAN_POINT('Ctrl Pts',(7.71424172989907,12.2,7.09281538834824));
#208745=CARTESIAN_POINT('Ctrl Pts',(7.71624366334244,12.2,7.09539376965728));
#208746=CARTESIAN_POINT('Ctrl Pts',(7.71824559660397,12.2,7.09797215073212));
#208747=CARTESIAN_POINT('Ctrl Pts',(7.72026900951376,12.2,7.10059314884521));
#208748=CARTESIAN_POINT('Ctrl Pts',(7.72231311993858,12.2,7.10325653466326));
#208749=CARTESIAN_POINT('Ctrl Pts',(7.72435723036339,12.2,7.1059199204813));
#208750=CARTESIAN_POINT('Ctrl Pts',(7.7264220398831,12.2,7.1086256945531));
#208751=CARTESIAN_POINT('Ctrl Pts',(7.72850678630601,12.2,7.1113736324504));
#208752=CARTESIAN_POINT('Ctrl Pts',(7.73059153291827,12.2,7.1141215705973));
#208753=CARTESIAN_POINT('Ctrl Pts',(7.73269621517416,12.2,7.1169116723566));
#208754=CARTESIAN_POINT('Ctrl Pts',(7.73482009087407,12.2,7.11974371642943));
#208755=CARTESIAN_POINT('Ctrl Pts',(7.73694396638108,12.2,7.12257576024503));
#208756=CARTESIAN_POINT('Ctrl Pts',(7.73908703397603,12.2,7.12544974549974));
#208757=CARTESIAN_POINT('Ctrl Pts',(7.7412485664906,12.2,7.12836545249026));
#208758=CARTESIAN_POINT('Ctrl Pts',(7.74341009900516,12.2,7.13128115948078));
#208759=CARTESIAN_POINT('Ctrl Pts',(7.74559009592475,12.2,7.13423858848483));
#208760=CARTESIAN_POINT('Ctrl Pts',(7.74778784751036,12.2,7.13723752237304));
#208761=CARTESIAN_POINT('Ctrl Pts',(7.7499855992956,12.2,7.14023645653366));
#208762=CARTESIAN_POINT('Ctrl Pts',(7.7522011038984,12.2,7.14327689414883));
#208763=CARTESIAN_POINT('Ctrl Pts',(7.75443366796593,12.2,7.14635862055647));
#208764=CARTESIAN_POINT('Ctrl Pts',(7.75666623183067,12.2,7.14944034668418));
#208765=CARTESIAN_POINT('Ctrl Pts',(7.75891585274889,12.2,7.15256336313986));
#208766=CARTESIAN_POINT('Ctrl Pts',(7.76118185349991,12.2,7.1557274512749));
#208767=CARTESIAN_POINT('Ctrl Pts',(7.76344785425091,12.2,7.15889153940993));
#208768=CARTESIAN_POINT('Ctrl Pts',(7.76573023273056,12.2,7.16209670508579));
#208769=CARTESIAN_POINT('Ctrl Pts',(7.76802832376098,12.2,7.16534273221101));
#208770=CARTESIAN_POINT('Ctrl Pts',(7.76994339968924,12.2,7.16804775491364));
#208771=CARTESIAN_POINT('Ctrl Pts',(7.77186938791277,12.2,7.17078115509872));
#208772=CARTESIAN_POINT('Ctrl Pts',(7.77380591110667,12.2,7.17354281086114));
#208773=CARTESIAN_POINT('Ctrl Pts',(7.77574243430056,12.2,7.17630446662355));
#208774=CARTESIAN_POINT('Ctrl Pts',(7.77768948963916,12.2,7.17909437795613));
#208775=CARTESIAN_POINT('Ctrl Pts',(7.77964670963864,12.2,7.18191242302411));
#208776=CARTESIAN_POINT('Ctrl Pts',(7.78160392963811,12.2,7.18473046809209));
#208777=CARTESIAN_POINT('Ctrl Pts',(7.78357131293986,12.2,7.1875766477409));
#208778=CARTESIAN_POINT('Ctrl Pts',(7.7855484939905,12.2,7.19045084199001));
#208779=CARTESIAN_POINT('Ctrl Pts',(7.78752567504114,12.2,7.19332503623913));
#208780=CARTESIAN_POINT('Ctrl Pts',(7.78951265511659,12.2,7.19622724573881));
#208781=CARTESIAN_POINT('Ctrl Pts',(7.79150907449159,12.2,7.19915734997492));
#208782=CARTESIAN_POINT('Ctrl Pts',(7.79350549386659,12.2,7.20208745421102));
#208783=CARTESIAN_POINT('Ctrl Pts',(7.79551135437518,12.2,7.20504545453235));
#208784=CARTESIAN_POINT('Ctrl Pts',(7.79752630125935,12.2,7.20803123051821));
#208785=CARTESIAN_POINT('Ctrl Pts',(7.79954124814353,12.2,7.21101700650407));
#208786=CARTESIAN_POINT('Ctrl Pts',(7.80156528407135,12.2,7.21403056018642));
#208787=CARTESIAN_POINT('Ctrl Pts',(7.80359806018291,12.2,7.21707177192397));
#208788=CARTESIAN_POINT('Ctrl Pts',(7.80563083629447,12.2,7.22011298366151));
#208789=CARTESIAN_POINT('Ctrl Pts',(7.8076723534336,12.2,7.22318185512338));
#208790=CARTESIAN_POINT('Ctrl Pts',(7.80972227114237,12.2,7.22627826769426));
#208791=CARTESIAN_POINT('Ctrl Pts',(7.81177218885114,12.2,7.22937468026514));
#208792=CARTESIAN_POINT('Ctrl Pts',(7.81383050728048,12.2,7.23249863385094));
#208793=CARTESIAN_POINT('Ctrl Pts',(7.8158968902315,12.2,7.23565001331584));
#208794=CARTESIAN_POINT('Ctrl Pts',(7.81796327318252,12.2,7.23880139278073));
#208795=CARTESIAN_POINT('Ctrl Pts',(7.82003772232163,12.2,7.24198019770035));
#208796=CARTESIAN_POINT('Ctrl Pts',(7.82211990607227,12.2,7.24518631270261));
#208797=CARTESIAN_POINT('Ctrl Pts',(7.82420208982293,12.2,7.24839242770487));
#208798=CARTESIAN_POINT('Ctrl Pts',(7.82629200866811,12.2,7.25162584982421));
#208799=CARTESIAN_POINT('Ctrl Pts',(7.82838933901592,12.2,7.25488646815974));
#208800=CARTESIAN_POINT('Ctrl Pts',(7.83048666913513,12.2,7.25814708613988));
#208801=CARTESIAN_POINT('Ctrl Pts',(7.83259141061558,12.2,7.26143489787432));
#208802=CARTESIAN_POINT('Ctrl Pts',(7.83470324323203,12.2,7.26474978931634));
#208803=CARTESIAN_POINT('Ctrl Pts',(7.83681507607868,12.2,7.26806468111968));
#208804=CARTESIAN_POINT('Ctrl Pts',(7.838934000078,12.2,7.27140665212259));
#208805=CARTESIAN_POINT('Ctrl Pts',(7.84105970202189,12.2,7.27477558955094));
#208806=CARTESIAN_POINT('Ctrl Pts',(7.84318540396578,12.2,7.2781445269793));
#208807=CARTESIAN_POINT('Ctrl Pts',(7.84531788187068,12.2,7.28154042878775));
#208808=CARTESIAN_POINT('Ctrl Pts',(7.84745682895349,12.2,7.28496318378556));
#208809=CARTESIAN_POINT('Ctrl Pts',(7.84959577603629,12.2,7.28838593878337));
#208810=CARTESIAN_POINT('Ctrl Pts',(7.85174119018754,12.2,7.29183554507461));
#208811=CARTESIAN_POINT('Ctrl Pts',(7.85389276751685,12.2,7.29531189107979));
#208812=CARTESIAN_POINT('Ctrl Pts',(7.85604434484615,12.2,7.29878823708496));
#208813=CARTESIAN_POINT('Ctrl Pts',(7.85820208679766,12.2,7.30229132324841));
#208814=CARTESIAN_POINT('Ctrl Pts',(7.8603656906168,12.2,7.30582103505257));
#208815=CARTESIAN_POINT('Ctrl Pts',(7.86252929443594,12.2,7.30935074685673));
#208816=CARTESIAN_POINT('Ctrl Pts',(7.86469876169133,12.2,7.31290708506158));
#208817=CARTESIAN_POINT('Ctrl Pts',(7.86687379564938,12.2,7.31648993853243));
#208818=CARTESIAN_POINT('Ctrl Pts',(7.86861382291065,12.2,7.31935622146531));
#208819=CARTESIAN_POINT('Ctrl Pts',(7.87035741479566,12.2,7.32223947390253));
#208820=CARTESIAN_POINT('Ctrl Pts',(7.87210441947845,12.2,7.32513963892918));
#208821=CARTESIAN_POINT('Ctrl Pts',(7.87385142392321,12.2,7.32803980356069));
#208822=CARTESIAN_POINT('Ctrl Pts',(7.8756018424724,12.2,7.33095688124006));
#208823=CARTESIAN_POINT('Ctrl Pts',(7.8773555281066,12.2,7.3338908137769));
#208824=CARTESIAN_POINT('Ctrl Pts',(7.87954763532857,12.2,7.33755822974776));
#208825=CARTESIAN_POINT('Ctrl Pts',(7.88174484555065,12.2,7.34125198203039));
#208826=CARTESIAN_POINT('Ctrl Pts',(7.88394687610595,12.2,7.34497196126512));
#208827=CARTESIAN_POINT('Ctrl Pts',(7.88570850064619,12.2,7.3479479448151));
#208828=CARTESIAN_POINT('Ctrl Pts',(7.88747320806044,12.2,7.35094071321255));
#208829=CARTESIAN_POINT('Ctrl Pts',(7.88924085802311,12.2,7.35395020969504));
#208830=CARTESIAN_POINT('Ctrl Pts',(7.89100850774494,12.2,7.35695970576748));
#208831=CARTESIAN_POINT('Ctrl Pts',(7.89277909921404,12.2,7.35998593028729));
#208832=CARTESIAN_POINT('Ctrl Pts',(7.89455248834665,12.2,7.36302882675965));
#208833=CARTESIAN_POINT('Ctrl Pts',(7.89632587772089,12.2,7.3660717236466));
#208834=CARTESIAN_POINT('Ctrl Pts',(7.89810206741491,12.2,7.36913129288557));
#208835=CARTESIAN_POINT('Ctrl Pts',(7.89988091417871,12.2,7.37220747777655));
#208836=CARTESIAN_POINT('Ctrl Pts',(7.90165976070015,12.2,7.37528366224841));
#208837=CARTESIAN_POINT('Ctrl Pts',(7.90344126715913,12.2,7.37837646275746));
#208838=CARTESIAN_POINT('Ctrl Pts',(7.90522529299107,12.2,7.38148582282382));
#208839=CARTESIAN_POINT('Ctrl Pts',(7.9074553254633,12.2,7.38537252322448));
#208840=CARTESIAN_POINT('Ctrl Pts',(7.90968929562603,12.2,7.38928510072164));
#208841=CARTESIAN_POINT('Ctrl Pts',(7.91192693465361,12.2,7.39322344252584));
#208842=CARTESIAN_POINT('Ctrl Pts',(7.91371704597325,12.2,7.39637411614091));
#208843=CARTESIAN_POINT('Ctrl Pts',(7.91550950582929,12.2,7.39954128067188));
#208844=CARTESIAN_POINT('Ctrl Pts',(7.91730417987167,12.2,7.40272488023534));
#208845=CARTESIAN_POINT('Ctrl Pts',(7.91909885366954,12.2,7.40590847936502));
#208846=CARTESIAN_POINT('Ctrl Pts',(7.9208957400185,12.2,7.40910851331197));
#208847=CARTESIAN_POINT('Ctrl Pts',(7.9226947077389,12.2,7.41232492604162));
#208848=CARTESIAN_POINT('Ctrl Pts',(7.92449367570441,12.2,7.4155413392095));
#208849=CARTESIAN_POINT('Ctrl Pts',(7.92629472271841,12.2,7.41877413329589));
#208850=CARTESIAN_POINT('Ctrl Pts',(7.92809771687235,12.2,7.42202325030735));
#208851=CARTESIAN_POINT('Ctrl Pts',(7.92990071078063,12.2,7.42527236687613));
#208852=CARTESIAN_POINT('Ctrl Pts',(7.93170565305519,12.2,7.42853780804164));
#208853=CARTESIAN_POINT('Ctrl Pts',(7.93351241096287,12.2,7.43181951793837));
#208854=CARTESIAN_POINT('Ctrl Pts',(7.9353191691167,12.2,7.43510122828223));
#208855=CARTESIAN_POINT('Ctrl Pts',(7.93712774563038,12.2,7.4383992087592));
#208856=CARTESIAN_POINT('Ctrl Pts',(7.93893800845951,12.2,7.44171340301052));
#208857=CARTESIAN_POINT('Ctrl Pts',(7.94074827104199,12.2,7.44502759681029));
#208858=CARTESIAN_POINT('Ctrl Pts',(7.94256022076295,12.2,7.44835800444743));
#208859=CARTESIAN_POINT('Ctrl Pts',(7.94437373117009,12.2,7.45170457222776));
#208860=CARTESIAN_POINT('Ctrl Pts',(7.94618724182433,12.2,7.45505114046406));
#208861=CARTESIAN_POINT('Ctrl Pts',(7.94800231055372,12.2,7.45841386751855));
#208862=CARTESIAN_POINT('Ctrl Pts',(7.94981881270827,12.2,7.46179269975825));
#208863=CARTESIAN_POINT('Ctrl Pts',(7.95163531486283,12.2,7.46517153199795));
#208864=CARTESIAN_POINT('Ctrl Pts',(7.95345325059811,12.2,7.46856646850622));
#208865=CARTESIAN_POINT('Ctrl Pts',(7.95527249403072,12.2,7.47197745608263));
#208866=CARTESIAN_POINT('Ctrl Pts',(7.95754654794967,12.2,7.47624118985601));
#208867=CARTESIAN_POINT('Ctrl Pts',(7.95982264504489,12.2,7.48053000209685));
#208868=CARTESIAN_POINT('Ctrl Pts',(7.96210054326866,12.2,7.48484378669403));
#208869=CARTESIAN_POINT('Ctrl Pts',(7.96392286214562,12.2,7.488294814936));
#208870=CARTESIAN_POINT('Ctrl Pts',(7.96574633502549,12.2,7.49176182528228));
#208871=CARTESIAN_POINT('Ctrl Pts',(7.96757083795827,12.2,7.49524476424992));
#208872=CARTESIAN_POINT('Ctrl Pts',(7.96939534089106,12.2,7.49872770321755));
#208873=CARTESIAN_POINT('Ctrl Pts',(7.97122087518504,12.2,7.5022265706203));
#208874=CARTESIAN_POINT('Ctrl Pts',(7.97304731934023,12.2,7.50574131159126));
#208875=CARTESIAN_POINT('Ctrl Pts',(7.97487376324658,12.2,7.50925605208334));
#208876=CARTESIAN_POINT('Ctrl Pts',(7.97670111759539,12.2,7.51278666650468));
#208877=CARTESIAN_POINT('Ctrl Pts',(7.97852926156537,12.2,7.51633310223085));
#208878=CARTESIAN_POINT('Ctrl Pts',(7.98035740578443,12.2,7.51987953844023));
#208879=CARTESIAN_POINT('Ctrl Pts',(7.98218634003541,12.2,7.5234417933411));
#208880=CARTESIAN_POINT('Ctrl Pts',(7.98401594752408,12.2,7.52701981559327));
#208881=CARTESIAN_POINT('Ctrl Pts',(7.98584555476348,12.2,7.53059783735794));
#208882=CARTESIAN_POINT('Ctrl Pts',(7.98767583257221,12.2,7.5341916251761));
#208883=CARTESIAN_POINT('Ctrl Pts',(7.98950666586694,12.2,7.53780112571333));
#208884=CARTESIAN_POINT('Ctrl Pts',(7.99133749941114,12.2,7.54141062674235));
#208885=CARTESIAN_POINT('Ctrl Pts',(7.99316888807762,12.2,7.54503584072326));
#208886=CARTESIAN_POINT('Ctrl Pts',(7.9950007143997,12.2,7.54867671375605));
#208887=CARTESIAN_POINT('Ctrl Pts',(7.9968325404722,12.2,7.55231758629278));
#208888=CARTESIAN_POINT('Ctrl Pts',(7.99866480683119,12.2,7.55597411842136));
#208889=CARTESIAN_POINT('Ctrl Pts',(8.00049739621736,12.2,7.55964625569216));
#208890=CARTESIAN_POINT('Ctrl Pts',(8.00232998585321,12.2,7.56331839346329));
#208891=CARTESIAN_POINT('Ctrl Pts',(8.00416289929155,12.2,7.56700613793053));
#208892=CARTESIAN_POINT('Ctrl Pts',(8.00599602289147,12.2,7.57070943307782));
#208893=CARTESIAN_POINT('Ctrl Pts',(8.00782914624163,12.2,7.57441272772054));
#208894=CARTESIAN_POINT('Ctrl Pts',(8.00966247936952,12.2,7.57813157536289));
#208895=CARTESIAN_POINT('Ctrl Pts',(8.01149591194184,12.2,7.58186592238936));
#208896=CARTESIAN_POINT('Ctrl Pts',(8.01332934476397,12.2,7.58560026992463));
#208897=CARTESIAN_POINT('Ctrl Pts',(8.01516287297628,12.2,7.58935011622459));
#208898=CARTESIAN_POINT('Ctrl Pts',(8.01699638975119,12.2,7.59311540800249));
#208899=CARTESIAN_POINT('Ctrl Pts',(8.01882990627629,12.2,7.59688069926738));
#208900=CARTESIAN_POINT('Ctrl Pts',(8.0206634080584,12.2,7.60066143764954));
#208901=CARTESIAN_POINT('Ctrl Pts',(8.02249678674186,12.2,7.60445756817093));
#208902=CARTESIAN_POINT('Ctrl Pts',(8.0243301656751,12.2,7.60825369920954));
#208903=CARTESIAN_POINT('Ctrl Pts',(8.02616342036114,12.2,7.61206522297743));
#208904=CARTESIAN_POINT('Ctrl Pts',(8.02799644201661,12.2,7.61589208724159));
#208905=CARTESIAN_POINT('Ctrl Pts',(8.02982946367209,12.2,7.61971895150575));
#208906=CARTESIAN_POINT('Ctrl Pts',(8.03166225341084,12.2,7.6235611560383));
#208907=CARTESIAN_POINT('Ctrl Pts',(8.03349470106622,12.2,7.62741864763897));
#208908=CARTESIAN_POINT('Ctrl Pts',(8.03532714847193,12.2,7.63127613871406));
#208909=CARTESIAN_POINT('Ctrl Pts',(8.03715925420401,12.2,7.63514891615031));
#208910=CARTESIAN_POINT('Ctrl Pts',(8.03899091300703,12.2,7.63903692923895));
#208911=CARTESIAN_POINT('Ctrl Pts',(8.04082257205961,12.2,7.64292494285733));
#208912=CARTESIAN_POINT('Ctrl Pts',(8.04265378265511,12.2,7.64682819023105));
#208913=CARTESIAN_POINT('Ctrl Pts',(8.04448443953259,12.2,7.6507466198906));
#208914=CARTESIAN_POINT('Ctrl Pts',(8.04631509616065,12.2,7.65466504901625));
#208915=CARTESIAN_POINT('Ctrl Pts',(8.04814519769434,12.2,7.65859865970659));
#208916=CARTESIAN_POINT('Ctrl Pts',(8.04997464110038,12.2,7.66254740016059));
#208917=CARTESIAN_POINT('Ctrl Pts',(8.05180408475569,12.2,7.6664961411526));
#208918=CARTESIAN_POINT('Ctrl Pts',(8.05363286995487,12.2,7.67046001176599));
#208919=CARTESIAN_POINT('Ctrl Pts',(8.05546089175687,12.2,7.67443895962738));
#208920=CARTESIAN_POINT('Ctrl Pts',(8.05728891330979,12.2,7.67841790694665));
#208921=CARTESIAN_POINT('Ctrl Pts',(8.05911617138044,12.2,7.68241192940106));
#208922=CARTESIAN_POINT('Ctrl Pts',(8.06094256417563,12.2,7.68642097840566));
#208923=CARTESIAN_POINT('Ctrl Pts',(8.06322555535625,12.2,7.69143229007108));
#208924=CARTESIAN_POINT('Ctrl Pts',(8.06550719342852,12.2,7.69646707774827));
#208925=CARTESIAN_POINT('Ctrl Pts',(8.06778727960916,12.2,7.70152523871927));
#208926=CARTESIAN_POINT('Ctrl Pts',(8.06915533126784,12.2,7.7045601351916));
#208927=CARTESIAN_POINT('Ctrl Pts',(8.07052282405012,12.2,7.70760344580231));
#208928=CARTESIAN_POINT('Ctrl Pts',(8.07188971627715,12.2,7.71065515038458));
#208929=CARTESIAN_POINT('Ctrl Pts',(8.07325660850417,12.2,7.71370685496685));
#208930=CARTESIAN_POINT('Ctrl Pts',(8.07462289946845,12.2,7.71676695219367));
#208931=CARTESIAN_POINT('Ctrl Pts',(8.07598854666891,12.2,7.71983542012268));
#208932=CARTESIAN_POINT('Ctrl Pts',(8.07735419411745,12.2,7.72290388860913));
#208933=CARTESIAN_POINT('Ctrl Pts',(8.07871919794917,12.2,7.72598072705629));
#208934=CARTESIAN_POINT('Ctrl Pts',(8.08008351727237,12.2,7.7290659141725));
#208935=CARTESIAN_POINT('Ctrl Pts',(8.08144783634771,12.2,7.73215110072822));
#208936=CARTESIAN_POINT('Ctrl Pts',(8.08281146933141,12.2,7.73524463731681));
#208937=CARTESIAN_POINT('Ctrl Pts',(8.08417437590682,12.2,7.7383464998715));
#208938=CARTESIAN_POINT('Ctrl Pts',(8.08553728248225,12.2,7.74144836242619));
#208939=CARTESIAN_POINT('Ctrl Pts',(8.08689946139447,12.2,7.74455855193521));
#208940=CARTESIAN_POINT('Ctrl Pts',(8.08826087255952,12.2,7.7476770464611));
#208941=CARTESIAN_POINT('Ctrl Pts',(8.08962228372457,12.2,7.750795540987));
#208942=CARTESIAN_POINT('Ctrl Pts',(8.09098292644194,12.2,7.75392234161348));
#208943=CARTESIAN_POINT('Ctrl Pts',(8.09234275923205,12.2,7.75705742505541));
#208944=CARTESIAN_POINT('Ctrl Pts',(8.09370259202214,12.2,7.76019250849735));
#208945=CARTESIAN_POINT('Ctrl Pts',(8.09506161636783,12.2,7.7633358736551));
#208946=CARTESIAN_POINT('Ctrl Pts',(8.09641979011023,12.2,7.76648750108154));
#208947=CARTESIAN_POINT('Ctrl Pts',(8.09777796385263,12.2,7.76963912850798));
#208948=CARTESIAN_POINT('Ctrl Pts',(8.09913528768675,12.2,7.77279901692553));
#208949=CARTESIAN_POINT('Ctrl Pts',(8.10049172042925,12.2,7.77596714535094));
#208950=CARTESIAN_POINT('Ctrl Pts',(8.10184815341816,12.2,7.7791352743519));
#208951=CARTESIAN_POINT('Ctrl Pts',(8.10320369583185,12.2,7.78231164311356));
#208952=CARTESIAN_POINT('Ctrl Pts',(8.10455830727859,12.2,7.78549622920251));
#208953=CARTESIAN_POINT('Ctrl Pts',(8.10591291847924,12.2,7.78868081471293));
#208954=CARTESIAN_POINT('Ctrl Pts',(8.10726659877667,12.2,7.79187361799144));
#208955=CARTESIAN_POINT('Ctrl Pts',(8.10861930850333,12.2,7.79507461761933));
#208956=CARTESIAN_POINT('Ctrl Pts',(8.10997201822998,12.2,7.79827561724721));
#208957=CARTESIAN_POINT('Ctrl Pts',(8.111323756463,12.2,7.80148481265029));
#208958=CARTESIAN_POINT('Ctrl Pts',(8.11267448466383,12.2,7.80470218261743));
#208959=CARTESIAN_POINT('Ctrl Pts',(8.11402521286466,12.2,7.80791955258457));
#208960=CARTESIAN_POINT('Ctrl Pts',(8.11537493099896,12.2,7.81114509646744));
#208961=CARTESIAN_POINT('Ctrl Pts',(8.11672359878329,12.2,7.81437879297494));
#208962=CARTESIAN_POINT('Ctrl Pts',(8.11807226656762,12.2,7.81761248948244));
#208963=CARTESIAN_POINT('Ctrl Pts',(8.11941988475199,12.2,7.82085433943129));
#208964=CARTESIAN_POINT('Ctrl Pts',(8.12076641357816,12.2,7.82410431943747));
#208965=CARTESIAN_POINT('Ctrl Pts',(8.12211294240431,12.2,7.82735429944365));
#208966=CARTESIAN_POINT('Ctrl Pts',(8.12345838307142,12.2,7.83061241020787));
#208967=CARTESIAN_POINT('Ctrl Pts',(8.12480269496485,12.2,7.83387863087641));
#208968=CARTESIAN_POINT('Ctrl Pts',(8.12614700685828,12.2,7.83714485154495));
#208969=CARTESIAN_POINT('Ctrl Pts',(8.127490191656,12.2,7.84041918177142));
#208970=CARTESIAN_POINT('Ctrl Pts',(8.12883220944072,12.2,7.84370159927603));
#208971=CARTESIAN_POINT('Ctrl Pts',(8.13017422746924,12.2,7.84698401737694));
#208972=CARTESIAN_POINT('Ctrl Pts',(8.13151507974747,12.2,7.85027452337188));
#208973=CARTESIAN_POINT('Ctrl Pts',(8.132854726317,12.2,7.85357309497736));
#208974=CARTESIAN_POINT('Ctrl Pts',(8.13419437264315,12.2,7.85687166598359));
#208975=CARTESIAN_POINT('Ctrl Pts',(8.13553281519438,12.2,7.86017830314777));
#208976=CARTESIAN_POINT('Ctrl Pts',(8.13687001489569,12.2,7.86349298511137));
#208977=CARTESIAN_POINT('Ctrl Pts',(8.13820721459699,12.2,7.86680766707496));
#208978=CARTESIAN_POINT('Ctrl Pts',(8.13954317003178,12.2,7.8701303932376));
#208979=CARTESIAN_POINT('Ctrl Pts',(8.14087784573329,12.2,7.87346114224159));
#208980=CARTESIAN_POINT('Ctrl Pts',(8.1422125214348,12.2,7.87679189124558));
#208981=CARTESIAN_POINT('Ctrl Pts',(8.14354591668635,12.2,7.8801306636409));
#208982=CARTESIAN_POINT('Ctrl Pts',(8.14487799388807,12.2,7.8834774371436));
#208983=CARTESIAN_POINT('Ctrl Pts',(8.14621007108978,12.2,7.88682421064629));
#208984=CARTESIAN_POINT('Ctrl Pts',(8.14754082972447,12.2,7.89017898543784));
#208985=CARTESIAN_POINT('Ctrl Pts',(8.1488702335344,12.2,7.89354174056606));
#208986=CARTESIAN_POINT('Ctrl Pts',(8.15019963734433,12.2,7.89690449569427));
#208987=CARTESIAN_POINT('Ctrl Pts',(8.15152768557544,12.2,7.90027523033727));
#208988=CARTESIAN_POINT('Ctrl Pts',(8.15285434048574,12.2,7.90365392375505));
#208989=CARTESIAN_POINT('Ctrl Pts',(8.15418099563705,12.2,7.90703261778662));
#208990=CARTESIAN_POINT('Ctrl Pts',(8.15550625964635,12.2,7.91041926964552));
#208991=CARTESIAN_POINT('Ctrl Pts',(8.15683009325522,12.2,7.9138138587233));
#208992=CARTESIAN_POINT('Ctrl Pts',(8.15859520433289,12.2,7.91833997646585));
#208993=CARTESIAN_POINT('Ctrl Pts',(8.1603577744692,12.2,7.92288020446209));
#208994=CARTESIAN_POINT('Ctrl Pts',(8.16211771738106,12.2,7.92743449164442));
#208995=CARTESIAN_POINT('Ctrl Pts',(8.1634376746249,12.2,7.9308502071863));
#208996=CARTESIAN_POINT('Ctrl Pts',(8.16475615394368,12.2,7.93427383187358));
#208997=CARTESIAN_POINT('Ctrl Pts',(8.16607311925348,12.2,7.93770534304443));
#208998=CARTESIAN_POINT('Ctrl Pts',(8.16739008456327,12.2,7.94113685421527));
#208999=CARTESIAN_POINT('Ctrl Pts',(8.16870553462772,12.2,7.9445762523081));
#209000=CARTESIAN_POINT('Ctrl Pts',(8.17001943445519,12.2,7.94802351580676));
#209001=CARTESIAN_POINT('Ctrl Pts',(8.17133333452135,12.2,7.95147077993168));
#209002=CARTESIAN_POINT('Ctrl Pts',(8.17264568464542,12.2,7.95492590978386));
#209003=CARTESIAN_POINT('Ctrl Pts',(8.17395644825237,12.2,7.95838888345486));
#209004=CARTESIAN_POINT('Ctrl Pts',(8.17526721162119,12.2,7.96185185649677));
#209005=CARTESIAN_POINT('Ctrl Pts',(8.17657639007345,12.2,7.96532267422163));
#209006=CARTESIAN_POINT('Ctrl Pts',(8.17788394690078,12.2,7.96880131513757));
#209007=CARTESIAN_POINT('Ctrl Pts',(8.17919150372813,12.2,7.9722799560535));
#209008=CARTESIAN_POINT('Ctrl Pts',(8.18049743995927,12.2,7.97576641908082));
#209009=CARTESIAN_POINT('Ctrl Pts',(8.18180171875114,12.2,7.97926068446977));
#209010=CARTESIAN_POINT('Ctrl Pts',(8.1835407570613,12.2,7.98391970477677));
#209011=CARTESIAN_POINT('Ctrl Pts',(8.18527684736629,12.2,7.98859259344596));
#209012=CARTESIAN_POINT('Ctrl Pts',(8.18700990772493,12.2,7.99327929928366));
#209013=CARTESIAN_POINT('Ctrl Pts',(8.18830970328908,12.2,7.99679432946014));
#209014=CARTESIAN_POINT('Ctrl Pts',(8.18960779461107,12.2,8.00031713288879));
#209015=CARTESIAN_POINT('Ctrl Pts',(8.19090415025756,12.2,8.0038476895696));
#209016=CARTESIAN_POINT('Ctrl Pts',(8.19220050566854,12.2,8.00737824560902));
#209017=CARTESIAN_POINT('Ctrl Pts',(8.19349512717131,12.2,8.01091655543141));
#209018=CARTESIAN_POINT('Ctrl Pts',(8.19478797687418,12.2,8.01446259688659));
#209019=CARTESIAN_POINT('Ctrl Pts',(8.19608082657705,12.2,8.01800863834176));
#209020=CARTESIAN_POINT('Ctrl Pts',(8.1973719043088,12.2,8.02156241154971));
#209021=CARTESIAN_POINT('Ctrl Pts',(8.19866116751779,12.2,8.02512388901984));
#209022=CARTESIAN_POINT('Ctrl Pts',(8.20038018505172,12.2,8.029872525431));
#209023=CARTESIAN_POINT('Ctrl Pts',(8.20209597184851,12.2,8.03463485712204));
#209024=CARTESIAN_POINT('Ctrl Pts',(8.20380846548663,12.2,8.0394108439524));
#209025=CARTESIAN_POINT('Ctrl Pts',(8.20552095935807,12.2,8.04418683143348));
#209026=CARTESIAN_POINT('Ctrl Pts',(8.20723015620175,12.2,8.04897647635775));
#209027=CARTESIAN_POINT('Ctrl Pts',(8.20893606999994,12.2,8.05377977099998));
#209028=CARTESIAN_POINT('Ctrl Pts',(7.93573928199995,15.2,8.32310290899999));
#209029=CARTESIAN_POINT('Ctrl Pts',(7.93573928199995,11.6,8.32310290899999));
#209030=CARTESIAN_POINT('Ctrl Pts',(7.93502251599994,15.2,8.32283676099999));
#209031=CARTESIAN_POINT('Ctrl Pts',(7.93502251599994,11.6,8.32283676099999));
#209032=CARTESIAN_POINT('Ctrl Pts',(7.93358949599994,15.2,8.32230434799998));
#209033=CARTESIAN_POINT('Ctrl Pts',(7.93358949599994,11.6,8.32230434799998));
#209034=CARTESIAN_POINT('Ctrl Pts',(7.93144150699994,15.2,8.32150538099998));
#209035=CARTESIAN_POINT('Ctrl Pts',(7.93144150699994,11.6,8.32150538099998));
#209036=CARTESIAN_POINT('Ctrl Pts',(7.92858060299995,15.2,8.32043939299999));
#209037=CARTESIAN_POINT('Ctrl Pts',(7.92858060299995,11.6,8.32043939299999));
#209038=CARTESIAN_POINT('Ctrl Pts',(7.92500961099995,15.2,8.31910574599998));
#209039=CARTESIAN_POINT('Ctrl Pts',(7.92500961099995,11.6,8.31910574599998));
#209040=CARTESIAN_POINT('Ctrl Pts',(7.92144375599995,15.2,8.31777093699999));
#209041=CARTESIAN_POINT('Ctrl Pts',(7.92144375599995,11.6,8.31777093699999));
#209042=CARTESIAN_POINT('Ctrl Pts',(7.91788303999994,15.2,8.31643496899999));
#209043=CARTESIAN_POINT('Ctrl Pts',(7.91788303999994,11.6,8.31643496899999));
#209044=CARTESIAN_POINT('Ctrl Pts',(7.91432746599994,15.2,8.31509784499998));
#209045=CARTESIAN_POINT('Ctrl Pts',(7.91432746599994,11.6,8.31509784499998));
#209046=CARTESIAN_POINT('Ctrl Pts',(7.91077703599995,15.2,8.31375956799998));
#209047=CARTESIAN_POINT('Ctrl Pts',(7.91077703599995,11.6,8.31375956799998));
#209048=CARTESIAN_POINT('Ctrl Pts',(7.90723175399994,15.2,8.31242014699999));
#209049=CARTESIAN_POINT('Ctrl Pts',(7.90723175399994,11.6,8.31242014699999));
#209050=CARTESIAN_POINT('Ctrl Pts',(7.90369162499994,15.2,8.31107958999999));
#209051=CARTESIAN_POINT('Ctrl Pts',(7.90369162499994,11.6,8.31107958999999));
#209052=CARTESIAN_POINT('Ctrl Pts',(7.90015665599994,15.2,8.30973790699998));
#209053=CARTESIAN_POINT('Ctrl Pts',(7.90015665599994,11.6,8.30973790699998));
#209054=CARTESIAN_POINT('Ctrl Pts',(7.89662685099994,15.2,8.30839510599999));
#209055=CARTESIAN_POINT('Ctrl Pts',(7.89662685099994,11.6,8.30839510599999));
#209056=CARTESIAN_POINT('Ctrl Pts',(7.89310221699994,15.2,8.30705119899999));
#209057=CARTESIAN_POINT('Ctrl Pts',(7.89310221699994,11.6,8.30705119899999));
#209058=CARTESIAN_POINT('Ctrl Pts',(7.88958275899994,15.2,8.30570619199998));
#209059=CARTESIAN_POINT('Ctrl Pts',(7.88958275899994,11.6,8.30570619199998));
#209060=CARTESIAN_POINT('Ctrl Pts',(7.88606848099994,15.2,8.30436009499999));
#209061=CARTESIAN_POINT('Ctrl Pts',(7.88606848099994,11.6,8.30436009499999));
#209062=CARTESIAN_POINT('Ctrl Pts',(7.88255938799994,15.2,8.30301291499998));
#209063=CARTESIAN_POINT('Ctrl Pts',(7.88255938799994,11.6,8.30301291499998));
#209064=CARTESIAN_POINT('Ctrl Pts',(7.87905548499995,15.2,8.30166465799999));
#209065=CARTESIAN_POINT('Ctrl Pts',(7.87905548499995,11.6,8.30166465799999));
#209066=CARTESIAN_POINT('Ctrl Pts',(7.87555677499994,15.2,8.30031533399998));
#209067=CARTESIAN_POINT('Ctrl Pts',(7.87555677499994,11.6,8.30031533399998));
#209068=CARTESIAN_POINT('Ctrl Pts',(7.87206326199994,15.2,8.29896494699998));
#209069=CARTESIAN_POINT('Ctrl Pts',(7.87206326199994,11.6,8.29896494699998));
#209070=CARTESIAN_POINT('Ctrl Pts',(7.86857495099994,15.2,8.29761350399998));
#209071=CARTESIAN_POINT('Ctrl Pts',(7.86857495099994,11.6,8.29761350399998));
#209072=CARTESIAN_POINT('Ctrl Pts',(7.86509184699994,15.2,8.29626101599998));
#209073=CARTESIAN_POINT('Ctrl Pts',(7.86509184699994,11.6,8.29626101599998));
#209074=CARTESIAN_POINT('Ctrl Pts',(7.86161395399994,15.2,8.29490748799999));
#209075=CARTESIAN_POINT('Ctrl Pts',(7.86161395399994,11.6,8.29490748799999));
#209076=CARTESIAN_POINT('Ctrl Pts',(7.85814127699994,15.2,8.29355293099999));
#209077=CARTESIAN_POINT('Ctrl Pts',(7.85814127699994,11.6,8.29355293099999));
#209078=CARTESIAN_POINT('Ctrl Pts',(7.85467382099994,15.2,8.29219735099999));
#209079=CARTESIAN_POINT('Ctrl Pts',(7.85467382099994,11.6,8.29219735099999));
#209080=CARTESIAN_POINT('Ctrl Pts',(7.85121158999995,15.2,8.29084075499999));
#209081=CARTESIAN_POINT('Ctrl Pts',(7.85121158999995,11.6,8.29084075499999));
#209082=CARTESIAN_POINT('Ctrl Pts',(7.84775458999994,15.2,8.28948315499999));
#209083=CARTESIAN_POINT('Ctrl Pts',(7.84775458999994,11.6,8.28948315499999));
#209084=CARTESIAN_POINT('Ctrl Pts',(7.84430282499994,15.2,8.28812455699998));
#209085=CARTESIAN_POINT('Ctrl Pts',(7.84430282499994,11.6,8.28812455699998));
#209086=CARTESIAN_POINT('Ctrl Pts',(7.84085629899994,15.2,8.28676496699998));
#209087=CARTESIAN_POINT('Ctrl Pts',(7.84085629899994,11.6,8.28676496699998));
#209088=CARTESIAN_POINT('Ctrl Pts',(7.83741501799994,15.2,8.28540439599998));
#209089=CARTESIAN_POINT('Ctrl Pts',(7.83741501799994,11.6,8.28540439599998));
#209090=CARTESIAN_POINT('Ctrl Pts',(7.83397898499994,15.2,8.28404284999999));
#209091=CARTESIAN_POINT('Ctrl Pts',(7.83397898499994,11.6,8.28404284999999));
#209092=CARTESIAN_POINT('Ctrl Pts',(7.83054820599994,15.2,8.28268033699998));
#209093=CARTESIAN_POINT('Ctrl Pts',(7.83054820599994,11.6,8.28268033699998));
#209094=CARTESIAN_POINT('Ctrl Pts',(7.82712268399994,15.2,8.28131686599999));
#209095=CARTESIAN_POINT('Ctrl Pts',(7.82712268399994,11.6,8.28131686599999));
#209096=CARTESIAN_POINT('Ctrl Pts',(7.82370242499994,15.2,8.27995244399998));
#209097=CARTESIAN_POINT('Ctrl Pts',(7.82370242499994,11.6,8.27995244399998));
#209098=CARTESIAN_POINT('Ctrl Pts',(7.82028743299994,15.2,8.27858707999999));
#209099=CARTESIAN_POINT('Ctrl Pts',(7.82028743299994,11.6,8.27858707999999));
#209100=CARTESIAN_POINT('Ctrl Pts',(7.81687771299994,15.2,8.27722078099999));
#209101=CARTESIAN_POINT('Ctrl Pts',(7.81687771299994,11.6,8.27722078099999));
#209102=CARTESIAN_POINT('Ctrl Pts',(7.81347326899994,15.2,8.27585355599999));
#209103=CARTESIAN_POINT('Ctrl Pts',(7.81347326899994,11.6,8.27585355599999));
#209104=CARTESIAN_POINT('Ctrl Pts',(7.81007410599995,15.2,8.27448541299999));
#209105=CARTESIAN_POINT('Ctrl Pts',(7.81007410599995,11.6,8.27448541299999));
#209106=CARTESIAN_POINT('Ctrl Pts',(7.80668022999994,15.2,8.27311635999998));
#209107=CARTESIAN_POINT('Ctrl Pts',(7.80668022999994,11.6,8.27311635999998));
#209108=CARTESIAN_POINT('Ctrl Pts',(7.80329164299994,15.2,8.27174640599999));
#209109=CARTESIAN_POINT('Ctrl Pts',(7.80329164299994,11.6,8.27174640599999));
#209110=CARTESIAN_POINT('Ctrl Pts',(7.79990835199994,15.2,8.27037555699999));
#209111=CARTESIAN_POINT('Ctrl Pts',(7.79990835199994,11.6,8.27037555699999));
#209112=CARTESIAN_POINT('Ctrl Pts',(7.79653035999995,15.2,8.26900382299998));
#209113=CARTESIAN_POINT('Ctrl Pts',(7.79653035999995,11.6,8.26900382299998));
#209114=CARTESIAN_POINT('Ctrl Pts',(7.79315767399994,15.2,8.26763121299999));
#209115=CARTESIAN_POINT('Ctrl Pts',(7.79315767399994,11.6,8.26763121299999));
#209116=CARTESIAN_POINT('Ctrl Pts',(7.78979029499994,15.2,8.26625773199999));
#209117=CARTESIAN_POINT('Ctrl Pts',(7.78979029499994,11.6,8.26625773199999));
#209118=CARTESIAN_POINT('Ctrl Pts',(7.78642823099994,15.2,8.26488339199998));
#209119=CARTESIAN_POINT('Ctrl Pts',(7.78642823099994,11.6,8.26488339199998));
#209120=CARTESIAN_POINT('Ctrl Pts',(7.78307148499994,15.2,8.26350819899999));
#209121=CARTESIAN_POINT('Ctrl Pts',(7.78307148499994,11.6,8.26350819899999));
#209122=CARTESIAN_POINT('Ctrl Pts',(7.77972006199994,15.2,8.26213216099998));
#209123=CARTESIAN_POINT('Ctrl Pts',(7.77972006199994,11.6,8.26213216099998));
#209124=CARTESIAN_POINT('Ctrl Pts',(7.77637396599994,15.2,8.26075528899998));
#209125=CARTESIAN_POINT('Ctrl Pts',(7.77637396599994,11.6,8.26075528899998));
#209126=CARTESIAN_POINT('Ctrl Pts',(7.77303320299994,15.2,8.25937758799999));
#209127=CARTESIAN_POINT('Ctrl Pts',(7.77303320299994,11.6,8.25937758799999));
#209128=CARTESIAN_POINT('Ctrl Pts',(7.76969777599994,15.2,8.25799906799999));
#209129=CARTESIAN_POINT('Ctrl Pts',(7.76969777599994,11.6,8.25799906799999));
#209130=CARTESIAN_POINT('Ctrl Pts',(7.76636769199994,15.2,8.25661973599999));
#209131=CARTESIAN_POINT('Ctrl Pts',(7.76636769199994,11.6,8.25661973599999));
#209132=CARTESIAN_POINT('Ctrl Pts',(7.76304295399994,15.2,8.25523960299999));
#209133=CARTESIAN_POINT('Ctrl Pts',(7.76304295399994,11.6,8.25523960299999));
#209134=CARTESIAN_POINT('Ctrl Pts',(7.75972356599994,15.2,8.25385867599999));
#209135=CARTESIAN_POINT('Ctrl Pts',(7.75972356599994,11.6,8.25385867599999));
#209136=CARTESIAN_POINT('Ctrl Pts',(7.75640953399995,15.2,8.25247696299999));
#209137=CARTESIAN_POINT('Ctrl Pts',(7.75640953399995,11.6,8.25247696299999));
#209138=CARTESIAN_POINT('Ctrl Pts',(7.75310086299994,15.2,8.25109447199999));
#209139=CARTESIAN_POINT('Ctrl Pts',(7.75310086299994,11.6,8.25109447199999));
#209140=CARTESIAN_POINT('Ctrl Pts',(7.74979755699994,15.2,8.24971121299999));
#209141=CARTESIAN_POINT('Ctrl Pts',(7.74979755699994,11.6,8.24971121299999));
#209142=CARTESIAN_POINT('Ctrl Pts',(7.74649961999994,15.2,8.24832719199998));
#209143=CARTESIAN_POINT('Ctrl Pts',(7.74649961999994,11.6,8.24832719199998));
#209144=CARTESIAN_POINT('Ctrl Pts',(7.74320705699994,15.2,8.24694242099999));
#209145=CARTESIAN_POINT('Ctrl Pts',(7.74320705699994,11.6,8.24694242099999));
#209146=CARTESIAN_POINT('Ctrl Pts',(7.73991987299994,15.2,8.24555690599999));
#209147=CARTESIAN_POINT('Ctrl Pts',(7.73991987299994,11.6,8.24555690599999));
#209148=CARTESIAN_POINT('Ctrl Pts',(7.73663807299994,15.2,8.24417065699999));
#209149=CARTESIAN_POINT('Ctrl Pts',(7.73663807299994,11.6,8.24417065699999));
#209150=CARTESIAN_POINT('Ctrl Pts',(7.73336166099994,15.2,8.24278367999998));
#209151=CARTESIAN_POINT('Ctrl Pts',(7.73336166099994,11.6,8.24278367999998));
#209152=CARTESIAN_POINT('Ctrl Pts',(7.73009064199995,15.2,8.24139598699999));
#209153=CARTESIAN_POINT('Ctrl Pts',(7.73009064199995,11.6,8.24139598699999));
#209154=CARTESIAN_POINT('Ctrl Pts',(7.72682502199994,15.2,8.24000758399999));
#209155=CARTESIAN_POINT('Ctrl Pts',(7.72682502199994,11.6,8.24000758399999));
#209156=CARTESIAN_POINT('Ctrl Pts',(7.72356480299995,15.2,8.23861848099998));
#209157=CARTESIAN_POINT('Ctrl Pts',(7.72356480299995,11.6,8.23861848099998));
#209158=CARTESIAN_POINT('Ctrl Pts',(7.72030999099995,15.2,8.23722868499999));
#209159=CARTESIAN_POINT('Ctrl Pts',(7.72030999099995,11.6,8.23722868499999));
#209160=CARTESIAN_POINT('Ctrl Pts',(7.71706059099994,15.2,8.23583820699999));
#209161=CARTESIAN_POINT('Ctrl Pts',(7.71706059099994,11.6,8.23583820699999));
#209162=CARTESIAN_POINT('Ctrl Pts',(7.71381660699994,15.2,8.23444705399999));
#209163=CARTESIAN_POINT('Ctrl Pts',(7.71381660699994,11.6,8.23444705399999));
#209164=CARTESIAN_POINT('Ctrl Pts',(7.71057804499995,15.2,8.23305523499998));
#209165=CARTESIAN_POINT('Ctrl Pts',(7.71057804499995,11.6,8.23305523499998));
#209166=CARTESIAN_POINT('Ctrl Pts',(7.70734490699994,15.2,8.23166275899998));
#209167=CARTESIAN_POINT('Ctrl Pts',(7.70734490699994,11.6,8.23166275899998));
#209168=CARTESIAN_POINT('Ctrl Pts',(7.70411720099994,15.2,8.23026963299998));
#209169=CARTESIAN_POINT('Ctrl Pts',(7.70411720099994,11.6,8.23026963299998));
#209170=CARTESIAN_POINT('Ctrl Pts',(7.70089492999994,15.2,8.22887586899999));
#209171=CARTESIAN_POINT('Ctrl Pts',(7.70089492999994,11.6,8.22887586899999));
#209172=CARTESIAN_POINT('Ctrl Pts',(7.69767809799994,15.2,8.22748147299999));
#209173=CARTESIAN_POINT('Ctrl Pts',(7.69767809799994,11.6,8.22748147299999));
#209174=CARTESIAN_POINT('Ctrl Pts',(7.69446671099994,15.2,8.22608645599999));
#209175=CARTESIAN_POINT('Ctrl Pts',(7.69446671099994,11.6,8.22608645599999));
#209176=CARTESIAN_POINT('Ctrl Pts',(7.69126077299994,15.2,8.22469082499998));
#209177=CARTESIAN_POINT('Ctrl Pts',(7.69126077299994,11.6,8.22469082499998));
#209178=CARTESIAN_POINT('Ctrl Pts',(7.68806028899994,15.2,8.22329458899999));
#209179=CARTESIAN_POINT('Ctrl Pts',(7.68806028899994,11.6,8.22329458899999));
#209180=CARTESIAN_POINT('Ctrl Pts',(7.68486526399994,15.2,8.22189775699999));
#209181=CARTESIAN_POINT('Ctrl Pts',(7.68486526399994,11.6,8.22189775699999));
#209182=CARTESIAN_POINT('Ctrl Pts',(7.68167570299994,15.2,8.22050033799999));
#209183=CARTESIAN_POINT('Ctrl Pts',(7.68167570299994,11.6,8.22050033799999));
#209184=CARTESIAN_POINT('Ctrl Pts',(7.67849160799994,15.2,8.21910234199999));
#209185=CARTESIAN_POINT('Ctrl Pts',(7.67849160799994,11.6,8.21910234199999));
#209186=CARTESIAN_POINT('Ctrl Pts',(7.67531298699994,15.2,8.21770377599999));
#209187=CARTESIAN_POINT('Ctrl Pts',(7.67531298699994,11.6,8.21770377599999));
#209188=CARTESIAN_POINT('Ctrl Pts',(7.67213984399994,15.2,8.21630465099998));
#209189=CARTESIAN_POINT('Ctrl Pts',(7.67213984399994,11.6,8.21630465099998));
#209190=CARTESIAN_POINT('Ctrl Pts',(7.66897218199994,15.2,8.21490497399999));
#209191=CARTESIAN_POINT('Ctrl Pts',(7.66897218199994,11.6,8.21490497399999));
#209192=CARTESIAN_POINT('Ctrl Pts',(7.66581000699994,15.2,8.21350475499998));
#209193=CARTESIAN_POINT('Ctrl Pts',(7.66581000699994,11.6,8.21350475499998));
#209194=CARTESIAN_POINT('Ctrl Pts',(7.66265332399994,15.2,8.21210400299999));
#209195=CARTESIAN_POINT('Ctrl Pts',(7.66265332399994,11.6,8.21210400299999));
#209196=CARTESIAN_POINT('Ctrl Pts',(7.65950213599995,15.2,8.21070272499998));
#209197=CARTESIAN_POINT('Ctrl Pts',(7.65950213599995,11.6,8.21070272499998));
#209198=CARTESIAN_POINT('Ctrl Pts',(7.65635644999994,15.2,8.20930093299998));
#209199=CARTESIAN_POINT('Ctrl Pts',(7.65635644999994,11.6,8.20930093299998));
#209200=CARTESIAN_POINT('Ctrl Pts',(7.65321626899994,15.2,8.20789863399998));
#209201=CARTESIAN_POINT('Ctrl Pts',(7.65321626899994,11.6,8.20789863399998));
#209202=CARTESIAN_POINT('Ctrl Pts',(7.65008159999994,15.2,8.20649583899998));
#209203=CARTESIAN_POINT('Ctrl Pts',(7.65008159999994,11.6,8.20649583899998));
#209204=CARTESIAN_POINT('Ctrl Pts',(7.64695244399995,15.2,8.20509255599998));
#209205=CARTESIAN_POINT('Ctrl Pts',(7.64695244399995,11.6,8.20509255599998));
#209206=CARTESIAN_POINT('Ctrl Pts',(7.64382880899994,15.2,8.20368879199999));
#209207=CARTESIAN_POINT('Ctrl Pts',(7.64382880899994,11.6,8.20368879199999));
#209208=CARTESIAN_POINT('Ctrl Pts',(7.64071069899994,15.2,8.20228455999998));
#209209=CARTESIAN_POINT('Ctrl Pts',(7.64071069899994,11.6,8.20228455999998));
#209210=CARTESIAN_POINT('Ctrl Pts',(7.63759811699994,15.2,8.20087986699999));
#209211=CARTESIAN_POINT('Ctrl Pts',(7.63759811699994,11.6,8.20087986699999));
#209212=CARTESIAN_POINT('Ctrl Pts',(7.63449106999994,15.2,8.19947472299998));
#209213=CARTESIAN_POINT('Ctrl Pts',(7.63449106999994,11.6,8.19947472299998));
#209214=CARTESIAN_POINT('Ctrl Pts',(7.63138956099994,15.2,8.19806913599999));
#209215=CARTESIAN_POINT('Ctrl Pts',(7.63138956099994,11.6,8.19806913599999));
#209216=CARTESIAN_POINT('Ctrl Pts',(7.62829359599994,15.2,8.19666311499999));
#209217=CARTESIAN_POINT('Ctrl Pts',(7.62829359599994,11.6,8.19666311499999));
#209218=CARTESIAN_POINT('Ctrl Pts',(7.62520317899994,15.2,8.19525667199999));
#209219=CARTESIAN_POINT('Ctrl Pts',(7.62520317899994,11.6,8.19525667199999));
#209220=CARTESIAN_POINT('Ctrl Pts',(7.62211831399994,15.2,8.19384981299999));
#209221=CARTESIAN_POINT('Ctrl Pts',(7.62211831399994,11.6,8.19384981299999));
#209222=CARTESIAN_POINT('Ctrl Pts',(7.61903900799994,15.2,8.19244254899999));
#209223=CARTESIAN_POINT('Ctrl Pts',(7.61903900799994,11.6,8.19244254899999));
#209224=CARTESIAN_POINT('Ctrl Pts',(7.61596526299994,15.2,8.19103488999998));
#209225=CARTESIAN_POINT('Ctrl Pts',(7.61596526299994,11.6,8.19103488999998));
#209226=CARTESIAN_POINT('Ctrl Pts',(7.61289708699994,15.2,8.18962684299999));
#209227=CARTESIAN_POINT('Ctrl Pts',(7.61289708699994,11.6,8.18962684299999));
#209228=CARTESIAN_POINT('Ctrl Pts',(7.60983448199994,15.2,8.18821841899998));
#209229=CARTESIAN_POINT('Ctrl Pts',(7.60983448199994,11.6,8.18821841899998));
#209230=CARTESIAN_POINT('Ctrl Pts',(7.60677745199994,15.2,8.18680962699998));
#209231=CARTESIAN_POINT('Ctrl Pts',(7.60677745199994,11.6,8.18680962699998));
#209232=CARTESIAN_POINT('Ctrl Pts',(7.60372600499994,15.2,8.18540047599999));
#209233=CARTESIAN_POINT('Ctrl Pts',(7.60372600499994,11.6,8.18540047599999));
#209234=CARTESIAN_POINT('Ctrl Pts',(7.60068014399994,15.2,8.18399097699999));
#209235=CARTESIAN_POINT('Ctrl Pts',(7.60068014399994,11.6,8.18399097699999));
#209236=CARTESIAN_POINT('Ctrl Pts',(7.59763987299994,15.2,8.18258113699999));
#209237=CARTESIAN_POINT('Ctrl Pts',(7.59763987299994,11.6,8.18258113699999));
#209238=CARTESIAN_POINT('Ctrl Pts',(7.59460519799994,15.2,8.18117096799998));
#209239=CARTESIAN_POINT('Ctrl Pts',(7.59460519799994,11.6,8.18117096799998));
#209240=CARTESIAN_POINT('Ctrl Pts',(7.59157612299994,15.2,8.17976047699998));
#209241=CARTESIAN_POINT('Ctrl Pts',(7.59157612299994,11.6,8.17976047699998));
#209242=CARTESIAN_POINT('Ctrl Pts',(7.58855265399994,15.2,8.17834967499999));
#209243=CARTESIAN_POINT('Ctrl Pts',(7.58855265399994,11.6,8.17834967499999));
#209244=CARTESIAN_POINT('Ctrl Pts',(7.58553479299994,15.2,8.17693857099999));
#209245=CARTESIAN_POINT('Ctrl Pts',(7.58553479299994,11.6,8.17693857099999));
#209246=CARTESIAN_POINT('Ctrl Pts',(7.58252254699994,15.2,8.17552717499998));
#209247=CARTESIAN_POINT('Ctrl Pts',(7.58252254699994,11.6,8.17552717499998));
#209248=CARTESIAN_POINT('Ctrl Pts',(7.57951592099994,15.2,8.17411549599999));
#209249=CARTESIAN_POINT('Ctrl Pts',(7.57951592099994,11.6,8.17411549599999));
#209250=CARTESIAN_POINT('Ctrl Pts',(7.57651491899995,15.2,8.17270354499998));
#209251=CARTESIAN_POINT('Ctrl Pts',(7.57651491899995,11.6,8.17270354499998));
#209252=CARTESIAN_POINT('Ctrl Pts',(7.57351954599994,15.2,8.17129132999998));
#209253=CARTESIAN_POINT('Ctrl Pts',(7.57351954599994,11.6,8.17129132999998));
#209254=CARTESIAN_POINT('Ctrl Pts',(7.57052980599994,15.2,8.16987885999998));
#209255=CARTESIAN_POINT('Ctrl Pts',(7.57052980599994,11.6,8.16987885999998));
#209256=CARTESIAN_POINT('Ctrl Pts',(7.56754570499995,15.2,8.16846614799999));
#209257=CARTESIAN_POINT('Ctrl Pts',(7.56754570499995,11.6,8.16846614799999));
#209258=CARTESIAN_POINT('Ctrl Pts',(7.56456724699994,15.2,8.16705319999999));
#209259=CARTESIAN_POINT('Ctrl Pts',(7.56456724699994,11.6,8.16705319999999));
#209260=CARTESIAN_POINT('Ctrl Pts',(7.56159443699994,15.2,8.16564002699998));
#209261=CARTESIAN_POINT('Ctrl Pts',(7.56159443699994,11.6,8.16564002699998));
#209262=CARTESIAN_POINT('Ctrl Pts',(7.55862727799994,15.2,8.16422663899999));
#209263=CARTESIAN_POINT('Ctrl Pts',(7.55862727799994,11.6,8.16422663899999));
#209264=CARTESIAN_POINT('Ctrl Pts',(7.55566577799994,15.2,8.16281304699999));
#209265=CARTESIAN_POINT('Ctrl Pts',(7.55566577799994,11.6,8.16281304699999));
#209266=CARTESIAN_POINT('Ctrl Pts',(7.55270993899994,15.2,8.16139925799998));
#209267=CARTESIAN_POINT('Ctrl Pts',(7.55270993899994,11.6,8.16139925799998));
#209268=CARTESIAN_POINT('Ctrl Pts',(7.54975976799994,15.2,8.15998528399999));
#209269=CARTESIAN_POINT('Ctrl Pts',(7.54975976799994,11.6,8.15998528399999));
#209270=CARTESIAN_POINT('Ctrl Pts',(7.54681526799994,15.2,8.15857113399998));
#209271=CARTESIAN_POINT('Ctrl Pts',(7.54681526799994,11.6,8.15857113399998));
#209272=CARTESIAN_POINT('Ctrl Pts',(7.54387644499994,15.2,8.15715681799999));
#209273=CARTESIAN_POINT('Ctrl Pts',(7.54387644499994,11.6,8.15715681799999));
#209274=CARTESIAN_POINT('Ctrl Pts',(7.54094330299995,15.2,8.15574234599998));
#209275=CARTESIAN_POINT('Ctrl Pts',(7.54094330299995,11.6,8.15574234599998));
#209276=CARTESIAN_POINT('Ctrl Pts',(7.53801584799994,15.2,8.15432772799999));
#209277=CARTESIAN_POINT('Ctrl Pts',(7.53801584799994,11.6,8.15432772799999));
#209278=CARTESIAN_POINT('Ctrl Pts',(7.53509408299994,15.2,8.15291297299999));
#209279=CARTESIAN_POINT('Ctrl Pts',(7.53509408299994,11.6,8.15291297299999));
#209280=CARTESIAN_POINT('Ctrl Pts',(7.53217801299995,15.2,8.15149809199998));
#209281=CARTESIAN_POINT('Ctrl Pts',(7.53217801299995,11.6,8.15149809199998));
#209282=CARTESIAN_POINT('Ctrl Pts',(7.52926764399994,15.2,8.15008309399998));
#209283=CARTESIAN_POINT('Ctrl Pts',(7.52926764399994,11.6,8.15008309399998));
#209284=CARTESIAN_POINT('Ctrl Pts',(7.52636298099994,15.2,8.14866798899999));
#209285=CARTESIAN_POINT('Ctrl Pts',(7.52636298099994,11.6,8.14866798899999));
#209286=CARTESIAN_POINT('Ctrl Pts',(7.52346402699994,15.2,8.14725278899999));
#209287=CARTESIAN_POINT('Ctrl Pts',(7.52346402699994,11.6,8.14725278899999));
#209288=CARTESIAN_POINT('Ctrl Pts',(7.52057078699995,15.2,8.14583750199999));
#209289=CARTESIAN_POINT('Ctrl Pts',(7.52057078699995,11.6,8.14583750199999));
#209290=CARTESIAN_POINT('Ctrl Pts',(7.51768326699994,15.2,8.14442213799998));
#209291=CARTESIAN_POINT('Ctrl Pts',(7.51768326699994,11.6,8.14442213799998));
#209292=CARTESIAN_POINT('Ctrl Pts',(7.51480147199994,15.2,8.14300670899998));
#209293=CARTESIAN_POINT('Ctrl Pts',(7.51480147199994,11.6,8.14300670899998));
#209294=CARTESIAN_POINT('Ctrl Pts',(7.51192540699994,15.2,8.14159122299999));
#209295=CARTESIAN_POINT('Ctrl Pts',(7.51192540699994,11.6,8.14159122299999));
#209296=CARTESIAN_POINT('Ctrl Pts',(7.50905507399994,15.2,8.14017569099999));
#209297=CARTESIAN_POINT('Ctrl Pts',(7.50905507399994,11.6,8.14017569099999));
#209298=CARTESIAN_POINT('Ctrl Pts',(7.50619048199994,15.2,8.13876012399999));
#209299=CARTESIAN_POINT('Ctrl Pts',(7.50619048199994,11.6,8.13876012399999));
#209300=CARTESIAN_POINT('Ctrl Pts',(7.50333163099994,15.2,8.13734453099999));
#209301=CARTESIAN_POINT('Ctrl Pts',(7.50333163099994,11.6,8.13734453099999));
#209302=CARTESIAN_POINT('Ctrl Pts',(7.50047852999994,15.2,8.13592892199999));
#209303=CARTESIAN_POINT('Ctrl Pts',(7.50047852999994,11.6,8.13592892199999));
#209304=CARTESIAN_POINT('Ctrl Pts',(7.49763118199994,15.2,8.13451330799998));
#209305=CARTESIAN_POINT('Ctrl Pts',(7.49763118199994,11.6,8.13451330799998));
#209306=CARTESIAN_POINT('Ctrl Pts',(7.49478959199994,15.2,8.13309769899998));
#209307=CARTESIAN_POINT('Ctrl Pts',(7.49478959199994,11.6,8.13309769899998));
#209308=CARTESIAN_POINT('Ctrl Pts',(7.49195376399994,15.2,8.13168210599999));
#209309=CARTESIAN_POINT('Ctrl Pts',(7.49195376399994,11.6,8.13168210599999));
#209310=CARTESIAN_POINT('Ctrl Pts',(7.48912370499994,15.2,8.13026653799999));
#209311=CARTESIAN_POINT('Ctrl Pts',(7.48912370499994,11.6,8.13026653799999));
#209312=CARTESIAN_POINT('Ctrl Pts',(7.48629941799994,15.2,8.12885100599999));
#209313=CARTESIAN_POINT('Ctrl Pts',(7.48629941799994,11.6,8.12885100599999));
#209314=CARTESIAN_POINT('Ctrl Pts',(7.48348090699994,15.2,8.12743552099998));
#209315=CARTESIAN_POINT('Ctrl Pts',(7.48348090699994,11.6,8.12743552099998));
#209316=CARTESIAN_POINT('Ctrl Pts',(7.48066817999994,15.2,8.12602009299999));
#209317=CARTESIAN_POINT('Ctrl Pts',(7.48066817999994,11.6,8.12602009299999));
#209318=CARTESIAN_POINT('Ctrl Pts',(7.47786123899994,15.2,8.12460473199998));
#209319=CARTESIAN_POINT('Ctrl Pts',(7.47786123899994,11.6,8.12460473199998));
#209320=CARTESIAN_POINT('Ctrl Pts',(7.47506008899994,15.2,8.12318944799999));
#209321=CARTESIAN_POINT('Ctrl Pts',(7.47506008899994,11.6,8.12318944799999));
#209322=CARTESIAN_POINT('Ctrl Pts',(7.47226473599994,15.2,8.12177425199998));
#209323=CARTESIAN_POINT('Ctrl Pts',(7.47226473599994,11.6,8.12177425199998));
#209324=CARTESIAN_POINT('Ctrl Pts',(7.46947518499994,15.2,8.12035915499998));
#209325=CARTESIAN_POINT('Ctrl Pts',(7.46947518499994,11.6,8.12035915499998));
#209326=CARTESIAN_POINT('Ctrl Pts',(7.46669143899994,15.2,8.11894416699998));
#209327=CARTESIAN_POINT('Ctrl Pts',(7.46669143899994,11.6,8.11894416699998));
#209328=CARTESIAN_POINT('Ctrl Pts',(7.46391350599994,15.2,8.11752929899999));
#209329=CARTESIAN_POINT('Ctrl Pts',(7.46391350599994,11.6,8.11752929899999));
#209330=CARTESIAN_POINT('Ctrl Pts',(7.46114138699994,15.2,8.11611456199999));
#209331=CARTESIAN_POINT('Ctrl Pts',(7.46114138699994,11.6,8.11611456199999));
#209332=CARTESIAN_POINT('Ctrl Pts',(7.45837508999994,15.2,8.11469996499999));
#209333=CARTESIAN_POINT('Ctrl Pts',(7.45837508999994,11.6,8.11469996499999));
#209334=CARTESIAN_POINT('Ctrl Pts',(7.45561461799994,15.2,8.11328551899998));
#209335=CARTESIAN_POINT('Ctrl Pts',(7.45561461799994,11.6,8.11328551899998));
#209336=CARTESIAN_POINT('Ctrl Pts',(7.45285997599994,15.2,8.11187123599998));
#209337=CARTESIAN_POINT('Ctrl Pts',(7.45285997599994,11.6,8.11187123599998));
#209338=CARTESIAN_POINT('Ctrl Pts',(7.45011116899994,15.2,8.11045712599999));
#209339=CARTESIAN_POINT('Ctrl Pts',(7.45011116899994,11.6,8.11045712599999));
#209340=CARTESIAN_POINT('Ctrl Pts',(7.44736820299994,15.2,8.10904319899999));
#209341=CARTESIAN_POINT('Ctrl Pts',(7.44736820299994,11.6,8.10904319899999));
#209342=CARTESIAN_POINT('Ctrl Pts',(7.44463108199994,15.2,8.10762946599999));
#209343=CARTESIAN_POINT('Ctrl Pts',(7.44463108199994,11.6,8.10762946599999));
#209344=CARTESIAN_POINT('Ctrl Pts',(7.44189980999994,15.2,8.10621593899998));
#209345=CARTESIAN_POINT('Ctrl Pts',(7.44189980999994,11.6,8.10621593899998));
#209346=CARTESIAN_POINT('Ctrl Pts',(7.43917439299994,15.2,8.10480262699999));
#209347=CARTESIAN_POINT('Ctrl Pts',(7.43917439299994,11.6,8.10480262699999));
#209348=CARTESIAN_POINT('Ctrl Pts',(7.43645483599994,15.2,8.10338954199998));
#209349=CARTESIAN_POINT('Ctrl Pts',(7.43645483599994,11.6,8.10338954199998));
#209350=CARTESIAN_POINT('Ctrl Pts',(7.43374114299994,15.2,8.10197669399999));
#209351=CARTESIAN_POINT('Ctrl Pts',(7.43374114299994,11.6,8.10197669399999));
#209352=CARTESIAN_POINT('Ctrl Pts',(7.43103331899994,15.2,8.10056409499998));
#209353=CARTESIAN_POINT('Ctrl Pts',(7.43103331899994,11.6,8.10056409499998));
#209354=CARTESIAN_POINT('Ctrl Pts',(7.42833136999994,15.2,8.09915175499999));
#209355=CARTESIAN_POINT('Ctrl Pts',(7.42833136999994,11.6,8.09915175499999));
#209356=CARTESIAN_POINT('Ctrl Pts',(7.42563529899994,15.2,8.09773968699999));
#209357=CARTESIAN_POINT('Ctrl Pts',(7.42563529899994,11.6,8.09773968699999));
#209358=CARTESIAN_POINT('Ctrl Pts',(7.42294511199994,15.2,8.09632789799998));
#209359=CARTESIAN_POINT('Ctrl Pts',(7.42294511199994,11.6,8.09632789799998));
#209360=CARTESIAN_POINT('Ctrl Pts',(7.42026081299994,15.2,8.09491640099999));
#209361=CARTESIAN_POINT('Ctrl Pts',(7.42026081299994,11.6,8.09491640099999));
#209362=CARTESIAN_POINT('Ctrl Pts',(7.41758240899994,15.2,8.09350520899999));
#209363=CARTESIAN_POINT('Ctrl Pts',(7.41758240899994,11.6,8.09350520899999));
#209364=CARTESIAN_POINT('Ctrl Pts',(7.41490990199994,15.2,8.09209432899999));
#209365=CARTESIAN_POINT('Ctrl Pts',(7.41490990199994,11.6,8.09209432899999));
#209366=CARTESIAN_POINT('Ctrl Pts',(7.41224329899994,15.2,8.09068377599999));
#209367=CARTESIAN_POINT('Ctrl Pts',(7.41224329899994,11.6,8.09068377599999));
#209368=CARTESIAN_POINT('Ctrl Pts',(7.40958260399994,15.2,8.08927355899998));
#209369=CARTESIAN_POINT('Ctrl Pts',(7.40958260399994,11.6,8.08927355899998));
#209370=CARTESIAN_POINT('Ctrl Pts',(7.40692782299995,15.2,8.08786368999998));
#209371=CARTESIAN_POINT('Ctrl Pts',(7.40692782299995,11.6,8.08786368999998));
#209372=CARTESIAN_POINT('Ctrl Pts',(7.40427895899994,15.2,8.08645417899999));
#209373=CARTESIAN_POINT('Ctrl Pts',(7.40427895899994,11.6,8.08645417899999));
#209374=CARTESIAN_POINT('Ctrl Pts',(7.40163601799994,15.2,8.08504503799998));
#209375=CARTESIAN_POINT('Ctrl Pts',(7.40163601799994,11.6,8.08504503799998));
#209376=CARTESIAN_POINT('Ctrl Pts',(7.39899900399994,15.2,8.08363627799999));
#209377=CARTESIAN_POINT('Ctrl Pts',(7.39899900399994,11.6,8.08363627799999));
#209378=CARTESIAN_POINT('Ctrl Pts',(7.39636792399994,15.2,8.08222790999999));
#209379=CARTESIAN_POINT('Ctrl Pts',(7.39636792399994,11.6,8.08222790999999));
#209380=CARTESIAN_POINT('Ctrl Pts',(7.39374278199994,15.2,8.08081994599998));
#209381=CARTESIAN_POINT('Ctrl Pts',(7.39374278199994,11.6,8.08081994599998));
#209382=CARTESIAN_POINT('Ctrl Pts',(7.39112357999994,15.2,8.07941239699998));
#209383=CARTESIAN_POINT('Ctrl Pts',(7.39112357999994,11.6,8.07941239699998));
#209384=CARTESIAN_POINT('Ctrl Pts',(7.38851032699994,15.2,8.07800527499998));
#209385=CARTESIAN_POINT('Ctrl Pts',(7.38851032699994,11.6,8.07800527499998));
#209386=CARTESIAN_POINT('Ctrl Pts',(7.38590302599994,15.2,8.07659858999998));
#209387=CARTESIAN_POINT('Ctrl Pts',(7.38590302599994,11.6,8.07659858999998));
#209388=CARTESIAN_POINT('Ctrl Pts',(7.38330168299994,15.2,8.07519235399998));
#209389=CARTESIAN_POINT('Ctrl Pts',(7.38330168299994,11.6,8.07519235399998));
#209390=CARTESIAN_POINT('Ctrl Pts',(7.38070630099994,15.2,8.07378657799998));
#209391=CARTESIAN_POINT('Ctrl Pts',(7.38070630099994,11.6,8.07378657799998));
#209392=CARTESIAN_POINT('Ctrl Pts',(7.37811688699994,15.2,8.07238127399999));
#209393=CARTESIAN_POINT('Ctrl Pts',(7.37811688699994,11.6,8.07238127399999));
#209394=CARTESIAN_POINT('Ctrl Pts',(7.37553344299994,15.2,8.07097645399999));
#209395=CARTESIAN_POINT('Ctrl Pts',(7.37553344299994,11.6,8.07097645399999));
#209396=CARTESIAN_POINT('Ctrl Pts',(7.37295597699994,15.2,8.06957212899999));
#209397=CARTESIAN_POINT('Ctrl Pts',(7.37295597699994,11.6,8.06957212899999));
#209398=CARTESIAN_POINT('Ctrl Pts',(7.37038449199994,15.2,8.06816830999999));
#209399=CARTESIAN_POINT('Ctrl Pts',(7.37038449199994,11.6,8.06816830999999));
#209400=CARTESIAN_POINT('Ctrl Pts',(7.36781899499994,15.2,8.06676500799998));
#209401=CARTESIAN_POINT('Ctrl Pts',(7.36781899499994,11.6,8.06676500799998));
#209402=CARTESIAN_POINT('Ctrl Pts',(7.36525948799994,15.2,8.06536223699998));
#209403=CARTESIAN_POINT('Ctrl Pts',(7.36525948799994,11.6,8.06536223699998));
#209404=CARTESIAN_POINT('Ctrl Pts',(7.36270597799995,15.2,8.06396000599998));
#209405=CARTESIAN_POINT('Ctrl Pts',(7.36270597799995,11.6,8.06396000599998));
#209406=CARTESIAN_POINT('Ctrl Pts',(7.36015846899994,15.2,8.06255832999998));
#209407=CARTESIAN_POINT('Ctrl Pts',(7.36015846899994,11.6,8.06255832999998));
#209408=CARTESIAN_POINT('Ctrl Pts',(7.35761696699995,15.2,8.06115721599999));
#209409=CARTESIAN_POINT('Ctrl Pts',(7.35761696699995,11.6,8.06115721599999));
#209410=CARTESIAN_POINT('Ctrl Pts',(7.35508147699995,15.2,8.05975668099999));
#209411=CARTESIAN_POINT('Ctrl Pts',(7.35508147699995,11.6,8.05975668099999));
#209412=CARTESIAN_POINT('Ctrl Pts',(7.35255200199994,15.2,8.05835673199999));
#209413=CARTESIAN_POINT('Ctrl Pts',(7.35255200199994,11.6,8.05835673199999));
#209414=CARTESIAN_POINT('Ctrl Pts',(7.35002854799994,15.2,8.05695738399999));
#209415=CARTESIAN_POINT('Ctrl Pts',(7.35002854799994,11.6,8.05695738399999));
#209416=CARTESIAN_POINT('Ctrl Pts',(7.34751111999994,15.2,8.05555864699999));
#209417=CARTESIAN_POINT('Ctrl Pts',(7.34751111999994,11.6,8.05555864699999));
#209418=CARTESIAN_POINT('Ctrl Pts',(7.34499972399994,15.2,8.05416053399998));
#209419=CARTESIAN_POINT('Ctrl Pts',(7.34499972399994,11.6,8.05416053399998));
#209420=CARTESIAN_POINT('Ctrl Pts',(7.34249436399995,15.2,8.05276305699999));
#209421=CARTESIAN_POINT('Ctrl Pts',(7.34249436399995,11.6,8.05276305699999));
#209422=CARTESIAN_POINT('Ctrl Pts',(7.33999504399995,15.2,8.05136622699998));
#209423=CARTESIAN_POINT('Ctrl Pts',(7.33999504399995,11.6,8.05136622699998));
#209424=CARTESIAN_POINT('Ctrl Pts',(7.33750177099994,15.2,8.04997005499999));
#209425=CARTESIAN_POINT('Ctrl Pts',(7.33750177099994,11.6,8.04997005499999));
#209426=CARTESIAN_POINT('Ctrl Pts',(7.33501454799995,15.2,8.04857455599999));
#209427=CARTESIAN_POINT('Ctrl Pts',(7.33501454799995,11.6,8.04857455599999));
#209428=CARTESIAN_POINT('Ctrl Pts',(7.33253337999995,15.2,8.04717973999999));
#209429=CARTESIAN_POINT('Ctrl Pts',(7.33253337999995,11.6,8.04717973999999));
#209430=CARTESIAN_POINT('Ctrl Pts',(7.33005827399994,15.2,8.04578561899999));
#209431=CARTESIAN_POINT('Ctrl Pts',(7.33005827399994,11.6,8.04578561899999));
#209432=CARTESIAN_POINT('Ctrl Pts',(7.32758923299994,15.2,8.04439220599999));
#209433=CARTESIAN_POINT('Ctrl Pts',(7.32758923299994,11.6,8.04439220599999));
#209434=CARTESIAN_POINT('Ctrl Pts',(7.32512626299994,15.2,8.04299951299999));
#209435=CARTESIAN_POINT('Ctrl Pts',(7.32512626299994,11.6,8.04299951299999));
#209436=CARTESIAN_POINT('Ctrl Pts',(7.32266936899994,15.2,8.04160755099998));
#209437=CARTESIAN_POINT('Ctrl Pts',(7.32266936899994,11.6,8.04160755099998));
#209438=CARTESIAN_POINT('Ctrl Pts',(7.32021855599994,15.2,8.04021633199999));
#209439=CARTESIAN_POINT('Ctrl Pts',(7.32021855599994,11.6,8.04021633199999));
#209440=CARTESIAN_POINT('Ctrl Pts',(7.31777382799994,15.2,8.03882586999999));
#209441=CARTESIAN_POINT('Ctrl Pts',(7.31777382799994,11.6,8.03882586999999));
#209442=CARTESIAN_POINT('Ctrl Pts',(7.31533518999994,15.2,8.03743617699999));
#209443=CARTESIAN_POINT('Ctrl Pts',(7.31533518999994,11.6,8.03743617699999));
#209444=CARTESIAN_POINT('Ctrl Pts',(7.31290264799994,15.2,8.03604726399998));
#209445=CARTESIAN_POINT('Ctrl Pts',(7.31290264799994,11.6,8.03604726399998));
#209446=CARTESIAN_POINT('Ctrl Pts',(7.31047620699995,15.2,8.03465914399998));
#209447=CARTESIAN_POINT('Ctrl Pts',(7.31047620699995,11.6,8.03465914399998));
#209448=CARTESIAN_POINT('Ctrl Pts',(7.30805587099994,15.2,8.03327182999999));
#209449=CARTESIAN_POINT('Ctrl Pts',(7.30805587099994,11.6,8.03327182999999));
#209450=CARTESIAN_POINT('Ctrl Pts',(7.30564164599994,15.2,8.03188533299998));
#209451=CARTESIAN_POINT('Ctrl Pts',(7.30564164599994,11.6,8.03188533299998));
#209452=CARTESIAN_POINT('Ctrl Pts',(7.30323353699994,15.2,8.03049966599998));
#209453=CARTESIAN_POINT('Ctrl Pts',(7.30323353699994,11.6,8.03049966599998));
#209454=CARTESIAN_POINT('Ctrl Pts',(7.30083154799994,15.2,8.02911484099998));
#209455=CARTESIAN_POINT('Ctrl Pts',(7.30083154799994,11.6,8.02911484099998));
#209456=CARTESIAN_POINT('Ctrl Pts',(7.29843568399994,15.2,8.02773087199999));
#209457=CARTESIAN_POINT('Ctrl Pts',(7.29843568399994,11.6,8.02773087199999));
#209458=CARTESIAN_POINT('Ctrl Pts',(7.29604595099994,15.2,8.02634777099998));
#209459=CARTESIAN_POINT('Ctrl Pts',(7.29604595099994,11.6,8.02634777099998));
#209460=CARTESIAN_POINT('Ctrl Pts',(7.29366235399994,15.2,8.02496554999999));
#209461=CARTESIAN_POINT('Ctrl Pts',(7.29366235399994,11.6,8.02496554999999));
#209462=CARTESIAN_POINT('Ctrl Pts',(7.29128489699994,15.2,8.02358422099999));
#209463=CARTESIAN_POINT('Ctrl Pts',(7.29128489699994,11.6,8.02358422099999));
#209464=CARTESIAN_POINT('Ctrl Pts',(7.28891358599994,15.2,8.02220379799999));
#209465=CARTESIAN_POINT('Ctrl Pts',(7.28891358599994,11.6,8.02220379799999));
#209466=CARTESIAN_POINT('Ctrl Pts',(7.28654842499994,15.2,8.02082429199999));
#209467=CARTESIAN_POINT('Ctrl Pts',(7.28654842499994,11.6,8.02082429199999));
#209468=CARTESIAN_POINT('Ctrl Pts',(7.28418941999994,15.2,8.01944571799999));
#209469=CARTESIAN_POINT('Ctrl Pts',(7.28418941999994,11.6,8.01944571799999));
#209470=CARTESIAN_POINT('Ctrl Pts',(7.28183657499994,15.2,8.01806808699999));
#209471=CARTESIAN_POINT('Ctrl Pts',(7.28183657499994,11.6,8.01806808699999));
#209472=CARTESIAN_POINT('Ctrl Pts',(7.27948989599994,15.2,8.01669141199999));
#209473=CARTESIAN_POINT('Ctrl Pts',(7.27948989599994,11.6,8.01669141199999));
#209474=CARTESIAN_POINT('Ctrl Pts',(7.27714938799994,15.2,8.01531570599998));
#209475=CARTESIAN_POINT('Ctrl Pts',(7.27714938799994,11.6,8.01531570599998));
#209476=CARTESIAN_POINT('Ctrl Pts',(7.27481505599994,15.2,8.01394098199999));
#209477=CARTESIAN_POINT('Ctrl Pts',(7.27481505599994,11.6,8.01394098199999));
#209478=CARTESIAN_POINT('Ctrl Pts',(7.27248690399994,15.2,8.01256725399998));
#209479=CARTESIAN_POINT('Ctrl Pts',(7.27248690399994,11.6,8.01256725399998));
#209480=CARTESIAN_POINT('Ctrl Pts',(7.27016493799994,15.2,8.01119453199998));
#209481=CARTESIAN_POINT('Ctrl Pts',(7.27016493799994,11.6,8.01119453199998));
#209482=CARTESIAN_POINT('Ctrl Pts',(7.26784916299994,15.2,8.00982283099999));
#209483=CARTESIAN_POINT('Ctrl Pts',(7.26784916299994,11.6,8.00982283099999));
#209484=CARTESIAN_POINT('Ctrl Pts',(7.26553958399994,15.2,8.00845216399999));
#209485=CARTESIAN_POINT('Ctrl Pts',(7.26553958399994,11.6,8.00845216399999));
#209486=CARTESIAN_POINT('Ctrl Pts',(7.26323620599994,15.2,8.00708254299998));
#209487=CARTESIAN_POINT('Ctrl Pts',(7.26323620599994,11.6,8.00708254299998));
#209488=CARTESIAN_POINT('Ctrl Pts',(7.26093903399994,15.2,8.00571398199999));
#209489=CARTESIAN_POINT('Ctrl Pts',(7.26093903399994,11.6,8.00571398199999));
#209490=CARTESIAN_POINT('Ctrl Pts',(7.25864807299994,15.2,8.00434649299999));
#209491=CARTESIAN_POINT('Ctrl Pts',(7.25864807299994,11.6,8.00434649299999));
#209492=CARTESIAN_POINT('Ctrl Pts',(7.25636332799994,15.2,8.00298009099999));
#209493=CARTESIAN_POINT('Ctrl Pts',(7.25636332799994,11.6,8.00298009099999));
#209494=CARTESIAN_POINT('Ctrl Pts',(7.25408480399994,15.2,8.00161478799998));
#209495=CARTESIAN_POINT('Ctrl Pts',(7.25408480399994,11.6,8.00161478799998));
#209496=CARTESIAN_POINT('Ctrl Pts',(7.25181250699994,15.2,8.00025059699998));
#209497=CARTESIAN_POINT('Ctrl Pts',(7.25181250699994,11.6,8.00025059699998));
#209498=CARTESIAN_POINT('Ctrl Pts',(7.24954643999994,15.2,7.99888753199999));
#209499=CARTESIAN_POINT('Ctrl Pts',(7.24954643999994,11.6,7.99888753199999));
#209500=CARTESIAN_POINT('Ctrl Pts',(7.24728661099994,15.2,7.99752560499999));
#209501=CARTESIAN_POINT('Ctrl Pts',(7.24728661099994,11.6,7.99752560499999));
#209502=CARTESIAN_POINT('Ctrl Pts',(7.24503302199994,15.2,7.99616483099998));
#209503=CARTESIAN_POINT('Ctrl Pts',(7.24503302199994,11.6,7.99616483099998));
#209504=CARTESIAN_POINT('Ctrl Pts',(7.24278568099994,15.2,7.99480522099999));
#209505=CARTESIAN_POINT('Ctrl Pts',(7.24278568099994,11.6,7.99480522099999));
#209506=CARTESIAN_POINT('Ctrl Pts',(7.24054459099994,15.2,7.99344679199999));
#209507=CARTESIAN_POINT('Ctrl Pts',(7.24054459099994,11.6,7.99344679199999));
#209508=CARTESIAN_POINT('Ctrl Pts',(7.23830975699994,15.2,7.99208955499999));
#209509=CARTESIAN_POINT('Ctrl Pts',(7.23830975699994,11.6,7.99208955499999));
#209510=CARTESIAN_POINT('Ctrl Pts',(7.23608118499994,15.2,7.99073352199999));
#209511=CARTESIAN_POINT('Ctrl Pts',(7.23608118499994,11.6,7.99073352199999));
#209512=CARTESIAN_POINT('Ctrl Pts',(7.23385888099994,15.2,7.98937870999998));
#209513=CARTESIAN_POINT('Ctrl Pts',(7.23385888099994,11.6,7.98937870999998));
#209514=CARTESIAN_POINT('Ctrl Pts',(7.23164284799994,15.2,7.98802513099999));
#209515=CARTESIAN_POINT('Ctrl Pts',(7.23164284799994,11.6,7.98802513099999));
#209516=CARTESIAN_POINT('Ctrl Pts',(7.22943309299994,15.2,7.98667279799999));
#209517=CARTESIAN_POINT('Ctrl Pts',(7.22943309299994,11.6,7.98667279799999));
#209518=CARTESIAN_POINT('Ctrl Pts',(7.22722961999994,15.2,7.98532172499999));
#209519=CARTESIAN_POINT('Ctrl Pts',(7.22722961999994,11.6,7.98532172499999));
#209520=CARTESIAN_POINT('Ctrl Pts',(7.22503243399994,15.2,7.98397192599998));
#209521=CARTESIAN_POINT('Ctrl Pts',(7.22503243399994,11.6,7.98397192599998));
#209522=CARTESIAN_POINT('Ctrl Pts',(7.22284154099994,15.2,7.98262341499999));
#209523=CARTESIAN_POINT('Ctrl Pts',(7.22284154099994,11.6,7.98262341499999));
#209524=CARTESIAN_POINT('Ctrl Pts',(7.22065694499994,15.2,7.98127620399999));
#209525=CARTESIAN_POINT('Ctrl Pts',(7.22065694499994,11.6,7.98127620399999));
#209526=CARTESIAN_POINT('Ctrl Pts',(7.21847865199994,15.2,7.97993030999999));
#209527=CARTESIAN_POINT('Ctrl Pts',(7.21847865199994,11.6,7.97993030999999));
#209528=CARTESIAN_POINT('Ctrl Pts',(7.21630666699994,15.2,7.97858574399999));
#209529=CARTESIAN_POINT('Ctrl Pts',(7.21630666699994,11.6,7.97858574399999));
#209530=CARTESIAN_POINT('Ctrl Pts',(7.21414099399994,15.2,7.97724252099999));
#209531=CARTESIAN_POINT('Ctrl Pts',(7.21414099399994,11.6,7.97724252099999));
#209532=CARTESIAN_POINT('Ctrl Pts',(7.21198163999994,15.2,7.97590065499998));
#209533=CARTESIAN_POINT('Ctrl Pts',(7.21198163999994,11.6,7.97590065499998));
#209534=CARTESIAN_POINT('Ctrl Pts',(7.20982860899994,15.2,7.97456015899999));
#209535=CARTESIAN_POINT('Ctrl Pts',(7.20982860899994,11.6,7.97456015899999));
#209536=CARTESIAN_POINT('Ctrl Pts',(7.20768190699994,15.2,7.97322104899998));
#209537=CARTESIAN_POINT('Ctrl Pts',(7.20768190699994,11.6,7.97322104899998));
#209538=CARTESIAN_POINT('Ctrl Pts',(7.20554153899994,15.2,7.97188333699999));
#209539=CARTESIAN_POINT('Ctrl Pts',(7.20554153899994,11.6,7.97188333699999));
#209540=CARTESIAN_POINT('Ctrl Pts',(7.20340750799994,15.2,7.97054703799999));
#209541=CARTESIAN_POINT('Ctrl Pts',(7.20340750799994,11.6,7.97054703799999));
#209542=CARTESIAN_POINT('Ctrl Pts',(7.20127982199994,15.2,7.96921216499998));
#209543=CARTESIAN_POINT('Ctrl Pts',(7.20127982199994,11.6,7.96921216499998));
#209544=CARTESIAN_POINT('Ctrl Pts',(7.19915848399994,15.2,7.96787873399998));
#209545=CARTESIAN_POINT('Ctrl Pts',(7.19915848399994,11.6,7.96787873399998));
#209546=CARTESIAN_POINT('Ctrl Pts',(7.19704350099994,15.2,7.96654675999999));
#209547=CARTESIAN_POINT('Ctrl Pts',(7.19704350099994,11.6,7.96654675999999));
#209548=CARTESIAN_POINT('Ctrl Pts',(7.19493487699994,15.2,7.96521625399999));
#209549=CARTESIAN_POINT('Ctrl Pts',(7.19493487699994,11.6,7.96521625399999));
#209550=CARTESIAN_POINT('Ctrl Pts',(7.19283261799994,15.2,7.96388723199998));
#209551=CARTESIAN_POINT('Ctrl Pts',(7.19283261799994,11.6,7.96388723199998));
#209552=CARTESIAN_POINT('Ctrl Pts',(7.19073672799994,15.2,7.96255970899999));
#209553=CARTESIAN_POINT('Ctrl Pts',(7.19073672799994,11.6,7.96255970899999));
#209554=CARTESIAN_POINT('Ctrl Pts',(7.18864721299994,15.2,7.96123369799999));
#209555=CARTESIAN_POINT('Ctrl Pts',(7.18864721299994,11.6,7.96123369799999));
#209556=CARTESIAN_POINT('Ctrl Pts',(7.18656407799994,15.2,7.95990921399999));
#209557=CARTESIAN_POINT('Ctrl Pts',(7.18656407799994,11.6,7.95990921399999));
#209558=CARTESIAN_POINT('Ctrl Pts',(7.18448732799994,15.2,7.95858627199999));
#209559=CARTESIAN_POINT('Ctrl Pts',(7.18448732799994,11.6,7.95858627199999));
#209560=CARTESIAN_POINT('Ctrl Pts',(7.18241696999994,15.2,7.95726488699999));
#209561=CARTESIAN_POINT('Ctrl Pts',(7.18241696999994,11.6,7.95726488699999));
#209562=CARTESIAN_POINT('Ctrl Pts',(7.18035300599994,15.2,7.95594507099998));
#209563=CARTESIAN_POINT('Ctrl Pts',(7.18035300599994,11.6,7.95594507099998));
#209564=CARTESIAN_POINT('Ctrl Pts',(7.17829544299994,15.2,7.95462684099999));
#209565=CARTESIAN_POINT('Ctrl Pts',(7.17829544299994,11.6,7.95462684099999));
#209566=CARTESIAN_POINT('Ctrl Pts',(7.17624428699994,15.2,7.95331021199999));
#209567=CARTESIAN_POINT('Ctrl Pts',(7.17624428699994,11.6,7.95331021199999));
#209568=CARTESIAN_POINT('Ctrl Pts',(7.17419954099995,15.2,7.95199519699998));
#209569=CARTESIAN_POINT('Ctrl Pts',(7.17419954099995,11.6,7.95199519699998));
#209570=CARTESIAN_POINT('Ctrl Pts',(7.17216121199994,15.2,7.95068181099998));
#209571=CARTESIAN_POINT('Ctrl Pts',(7.17216121199994,11.6,7.95068181099998));
#209572=CARTESIAN_POINT('Ctrl Pts',(7.17012930499994,15.2,7.94937006899998));
#209573=CARTESIAN_POINT('Ctrl Pts',(7.17012930499994,11.6,7.94937006899998));
#209574=CARTESIAN_POINT('Ctrl Pts',(7.16810382499995,15.2,7.94805998799998));
#209575=CARTESIAN_POINT('Ctrl Pts',(7.16810382499995,11.6,7.94805998799998));
#209576=CARTESIAN_POINT('Ctrl Pts',(7.16608477699994,15.2,7.94675157899999));
#209577=CARTESIAN_POINT('Ctrl Pts',(7.16608477699994,11.6,7.94675157899999));
#209578=CARTESIAN_POINT('Ctrl Pts',(7.16407216599994,15.2,7.94544485999998));
#209579=CARTESIAN_POINT('Ctrl Pts',(7.16407216599994,11.6,7.94544485999998));
#209580=CARTESIAN_POINT('Ctrl Pts',(7.16206599799994,15.2,7.94413984399998));
#209581=CARTESIAN_POINT('Ctrl Pts',(7.16206599799994,11.6,7.94413984399998));
#209582=CARTESIAN_POINT('Ctrl Pts',(7.16006627799994,15.2,7.94283654699999));
#209583=CARTESIAN_POINT('Ctrl Pts',(7.16006627799994,11.6,7.94283654699999));
#209584=CARTESIAN_POINT('Ctrl Pts',(7.15807301099994,15.2,7.94153498399999));
#209585=CARTESIAN_POINT('Ctrl Pts',(7.15807301099994,11.6,7.94153498399999));
#209586=CARTESIAN_POINT('Ctrl Pts',(7.15608620199994,15.2,7.94023516999999));
#209587=CARTESIAN_POINT('Ctrl Pts',(7.15608620199994,11.6,7.94023516999999));
#209588=CARTESIAN_POINT('Ctrl Pts',(7.15410585699994,15.2,7.93893712099998));
#209589=CARTESIAN_POINT('Ctrl Pts',(7.15410585699994,11.6,7.93893712099998));
#209590=CARTESIAN_POINT('Ctrl Pts',(7.15213198099995,15.2,7.93764085199999));
#209591=CARTESIAN_POINT('Ctrl Pts',(7.15213198099995,11.6,7.93764085199999));
#209592=CARTESIAN_POINT('Ctrl Pts',(7.15016457899995,15.2,7.93634637599999));
#209593=CARTESIAN_POINT('Ctrl Pts',(7.15016457899995,11.6,7.93634637599999));
#209594=CARTESIAN_POINT('Ctrl Pts',(7.14820365499994,15.2,7.93505370999998));
#209595=CARTESIAN_POINT('Ctrl Pts',(7.14820365499994,11.6,7.93505370999998));
#209596=CARTESIAN_POINT('Ctrl Pts',(7.14624921799994,15.2,7.93376286999998));
#209597=CARTESIAN_POINT('Ctrl Pts',(7.14624921799994,11.6,7.93376286999998));
#209598=CARTESIAN_POINT('Ctrl Pts',(7.14430126899994,15.2,7.93247387099999));
#209599=CARTESIAN_POINT('Ctrl Pts',(7.14430126899994,11.6,7.93247387099999));
#209600=CARTESIAN_POINT('Ctrl Pts',(7.14235981699994,15.2,7.93118672899999));
#209601=CARTESIAN_POINT('Ctrl Pts',(7.14235981699994,11.6,7.93118672899999));
#209602=CARTESIAN_POINT('Ctrl Pts',(7.14042486499994,15.2,7.92990145699999));
#209603=CARTESIAN_POINT('Ctrl Pts',(7.14042486499994,11.6,7.92990145699999));
#209604=CARTESIAN_POINT('Ctrl Pts',(7.13849641899994,15.2,7.92861807299998));
#209605=CARTESIAN_POINT('Ctrl Pts',(7.13849641899994,11.6,7.92861807299998));
#209606=CARTESIAN_POINT('Ctrl Pts',(7.13657448299994,15.2,7.92733659199998));
#209607=CARTESIAN_POINT('Ctrl Pts',(7.13657448299994,11.6,7.92733659199998));
#209608=CARTESIAN_POINT('Ctrl Pts',(7.13465906499994,15.2,7.92605702899999));
#209609=CARTESIAN_POINT('Ctrl Pts',(7.13465906499994,11.6,7.92605702899999));
#209610=CARTESIAN_POINT('Ctrl Pts',(7.13275016799994,15.2,7.92477940099998));
#209611=CARTESIAN_POINT('Ctrl Pts',(7.13275016799994,11.6,7.92477940099998));
#209612=CARTESIAN_POINT('Ctrl Pts',(7.13084779799994,15.2,7.92350372299998));
#209613=CARTESIAN_POINT('Ctrl Pts',(7.13084779799994,11.6,7.92350372299998));
#209614=CARTESIAN_POINT('Ctrl Pts',(7.12895196099994,15.2,7.92223000999999));
#209615=CARTESIAN_POINT('Ctrl Pts',(7.12895196099994,11.6,7.92223000999999));
#209616=CARTESIAN_POINT('Ctrl Pts',(7.12706265999994,15.2,7.92095827999999));
#209617=CARTESIAN_POINT('Ctrl Pts',(7.12706265999994,11.6,7.92095827999999));
#209618=CARTESIAN_POINT('Ctrl Pts',(7.12517990499994,15.2,7.91968854599999));
#209619=CARTESIAN_POINT('Ctrl Pts',(7.12517990499994,11.6,7.91968854599999));
#209620=CARTESIAN_POINT('Ctrl Pts',(7.12330369599994,15.2,7.91842082699999));
#209621=CARTESIAN_POINT('Ctrl Pts',(7.12330369599994,11.6,7.91842082699999));
#209622=CARTESIAN_POINT('Ctrl Pts',(7.12143404199994,15.2,7.91715513599998));
#209623=CARTESIAN_POINT('Ctrl Pts',(7.12143404199994,11.6,7.91715513599998));
#209624=CARTESIAN_POINT('Ctrl Pts',(7.11957094599994,15.2,7.91589149199999));
#209625=CARTESIAN_POINT('Ctrl Pts',(7.11957094599994,11.6,7.91589149199999));
#209626=CARTESIAN_POINT('Ctrl Pts',(7.11771441499994,15.2,7.91462990899999));
#209627=CARTESIAN_POINT('Ctrl Pts',(7.11771441499994,11.6,7.91462990899999));
#209628=CARTESIAN_POINT('Ctrl Pts',(7.11586445399995,15.2,7.91337040399998));
#209629=CARTESIAN_POINT('Ctrl Pts',(7.11586445399995,11.6,7.91337040399998));
#209630=CARTESIAN_POINT('Ctrl Pts',(7.11402106899994,15.2,7.91211299399999));
#209631=CARTESIAN_POINT('Ctrl Pts',(7.11402106899994,11.6,7.91211299399999));
#209632=CARTESIAN_POINT('Ctrl Pts',(7.11218426399994,15.2,7.91085769199999));
#209633=CARTESIAN_POINT('Ctrl Pts',(7.11218426399994,11.6,7.91085769199999));
#209634=CARTESIAN_POINT('Ctrl Pts',(7.11035404399994,15.2,7.90960451899998));
#209635=CARTESIAN_POINT('Ctrl Pts',(7.11035404399994,11.6,7.90960451899998));
#209636=CARTESIAN_POINT('Ctrl Pts',(7.10853041699994,15.2,7.90835348799998));
#209637=CARTESIAN_POINT('Ctrl Pts',(7.10853041699994,11.6,7.90835348799998));
#209638=CARTESIAN_POINT('Ctrl Pts',(7.10671338599994,15.2,7.90710461699998));
#209639=CARTESIAN_POINT('Ctrl Pts',(7.10671338599994,11.6,7.90710461699998));
#209640=CARTESIAN_POINT('Ctrl Pts',(7.10490295599994,15.2,7.90585792199998));
#209641=CARTESIAN_POINT('Ctrl Pts',(7.10490295599994,11.6,7.90585792199998));
#209642=CARTESIAN_POINT('Ctrl Pts',(7.10309913399994,15.2,7.90461341899999));
#209643=CARTESIAN_POINT('Ctrl Pts',(7.10309913399994,11.6,7.90461341899999));
#209644=CARTESIAN_POINT('Ctrl Pts',(7.10130192599994,15.2,7.90337112599998));
#209645=CARTESIAN_POINT('Ctrl Pts',(7.10130192599994,11.6,7.90337112599998));
#209646=CARTESIAN_POINT('Ctrl Pts',(7.09951133499994,15.2,7.90213105799998));
#209647=CARTESIAN_POINT('Ctrl Pts',(7.09951133499994,11.6,7.90213105799998));
#209648=CARTESIAN_POINT('Ctrl Pts',(7.09772736899994,15.2,7.90089323299998));
#209649=CARTESIAN_POINT('Ctrl Pts',(7.09772736899994,11.6,7.90089323299998));
#209650=CARTESIAN_POINT('Ctrl Pts',(7.09595003199994,15.2,7.89965766699999));
#209651=CARTESIAN_POINT('Ctrl Pts',(7.09595003199994,11.6,7.89965766699999));
#209652=CARTESIAN_POINT('Ctrl Pts',(7.09417932799994,15.2,7.89842437699999));
#209653=CARTESIAN_POINT('Ctrl Pts',(7.09417932799994,11.6,7.89842437699999));
#209654=CARTESIAN_POINT('Ctrl Pts',(7.09241526599994,15.2,7.89719338099999));
#209655=CARTESIAN_POINT('Ctrl Pts',(7.09241526599994,11.6,7.89719338099999));
#209656=CARTESIAN_POINT('Ctrl Pts',(7.09065784799995,15.2,7.89596469399999));
#209657=CARTESIAN_POINT('Ctrl Pts',(7.09065784799995,11.6,7.89596469399999));
#209658=CARTESIAN_POINT('Ctrl Pts',(7.08890708199994,15.2,7.89473833399998));
#209659=CARTESIAN_POINT('Ctrl Pts',(7.08890708199994,11.6,7.89473833399998));
#209660=CARTESIAN_POINT('Ctrl Pts',(7.08716297199994,15.2,7.89351431799999));
#209661=CARTESIAN_POINT('Ctrl Pts',(7.08716297199994,11.6,7.89351431799999));
#209662=CARTESIAN_POINT('Ctrl Pts',(7.08542552399994,15.2,7.89229266299999));
#209663=CARTESIAN_POINT('Ctrl Pts',(7.08542552399994,11.6,7.89229266299999));
#209664=CARTESIAN_POINT('Ctrl Pts',(7.08369474299994,15.2,7.89107338699999));
#209665=CARTESIAN_POINT('Ctrl Pts',(7.08369474299994,11.6,7.89107338699999));
#209666=CARTESIAN_POINT('Ctrl Pts',(7.08197063499994,15.2,7.88985650499999));
#209667=CARTESIAN_POINT('Ctrl Pts',(7.08197063499994,11.6,7.88985650499999));
#209668=CARTESIAN_POINT('Ctrl Pts',(7.08025320599995,15.2,7.88864203699998));
#209669=CARTESIAN_POINT('Ctrl Pts',(7.08025320599995,11.6,7.88864203699998));
#209670=CARTESIAN_POINT('Ctrl Pts',(7.07854245999994,15.2,7.88742999899998));
#209671=CARTESIAN_POINT('Ctrl Pts',(7.07854245999994,11.6,7.88742999899998));
#209672=CARTESIAN_POINT('Ctrl Pts',(7.07683840299994,15.2,7.88622040899998));
#209673=CARTESIAN_POINT('Ctrl Pts',(7.07683840299994,11.6,7.88622040899998));
#209674=CARTESIAN_POINT('Ctrl Pts',(7.07514103999995,15.2,7.88501328299999));
#209675=CARTESIAN_POINT('Ctrl Pts',(7.07514103999995,11.6,7.88501328299999));
#209676=CARTESIAN_POINT('Ctrl Pts',(7.07345037799994,15.2,7.88380863999999));
#209677=CARTESIAN_POINT('Ctrl Pts',(7.07345037799994,11.6,7.88380863999999));
#209678=CARTESIAN_POINT('Ctrl Pts',(7.07176642199994,15.2,7.88260649699998));
#209679=CARTESIAN_POINT('Ctrl Pts',(7.07176642199994,11.6,7.88260649699998));
#209680=CARTESIAN_POINT('Ctrl Pts',(7.07008917699994,15.2,7.88140687099999));
#209681=CARTESIAN_POINT('Ctrl Pts',(7.07008917699994,11.6,7.88140687099999));
#209682=CARTESIAN_POINT('Ctrl Pts',(7.06841864899994,15.2,7.88020978099999));
#209683=CARTESIAN_POINT('Ctrl Pts',(7.06841864899994,11.6,7.88020978099999));
#209684=CARTESIAN_POINT('Ctrl Pts',(7.06675484399995,15.2,7.87901524399999));
#209685=CARTESIAN_POINT('Ctrl Pts',(7.06675484399995,11.6,7.87901524399999));
#209686=CARTESIAN_POINT('Ctrl Pts',(7.06509776499994,15.2,7.87782327899999));
#209687=CARTESIAN_POINT('Ctrl Pts',(7.06509776499994,11.6,7.87782327899999));
#209688=CARTESIAN_POINT('Ctrl Pts',(7.06344742099994,15.2,7.87663390099999));
#209689=CARTESIAN_POINT('Ctrl Pts',(7.06344742099994,11.6,7.87663390099999));
#209690=CARTESIAN_POINT('Ctrl Pts',(7.06180381599994,15.2,7.87544713199999));
#209691=CARTESIAN_POINT('Ctrl Pts',(7.06180381599994,11.6,7.87544713199999));
#209692=CARTESIAN_POINT('Ctrl Pts',(7.06016695399994,15.2,7.87426298699998));
#209693=CARTESIAN_POINT('Ctrl Pts',(7.06016695399994,11.6,7.87426298699998));
#209694=CARTESIAN_POINT('Ctrl Pts',(7.05853684399994,15.2,7.87308148499999));
#209695=CARTESIAN_POINT('Ctrl Pts',(7.05853684399994,11.6,7.87308148499999));
#209696=CARTESIAN_POINT('Ctrl Pts',(7.05691348799995,15.2,7.87190264399998));
#209697=CARTESIAN_POINT('Ctrl Pts',(7.05691348799995,11.6,7.87190264399998));
#209698=CARTESIAN_POINT('Ctrl Pts',(7.05529689499994,15.2,7.87072648199998));
#209699=CARTESIAN_POINT('Ctrl Pts',(7.05529689499994,11.6,7.87072648199998));
#209700=CARTESIAN_POINT('Ctrl Pts',(7.05368706799994,15.2,7.86955301799999));
#209701=CARTESIAN_POINT('Ctrl Pts',(7.05368706799994,11.6,7.86955301799999));
#209702=CARTESIAN_POINT('Ctrl Pts',(7.05208401299994,15.2,7.86838227099998));
#209703=CARTESIAN_POINT('Ctrl Pts',(7.05208401299994,11.6,7.86838227099998));
#209704=CARTESIAN_POINT('Ctrl Pts',(7.05048773599994,15.2,7.86721425699999));
#209705=CARTESIAN_POINT('Ctrl Pts',(7.05048773599994,11.6,7.86721425699999));
#209706=CARTESIAN_POINT('Ctrl Pts',(7.04889824299994,15.2,7.86604899699999));
#209707=CARTESIAN_POINT('Ctrl Pts',(7.04889824299994,11.6,7.86604899699999));
#209708=CARTESIAN_POINT('Ctrl Pts',(7.04731553899994,15.2,7.86488650699999));
#209709=CARTESIAN_POINT('Ctrl Pts',(7.04731553899994,11.6,7.86488650699999));
#209710=CARTESIAN_POINT('Ctrl Pts',(7.04573962999994,15.2,7.86372680699999));
#209711=CARTESIAN_POINT('Ctrl Pts',(7.04573962999994,11.6,7.86372680699999));
#209712=CARTESIAN_POINT('Ctrl Pts',(7.04417052199994,15.2,7.86256991699998));
#209713=CARTESIAN_POINT('Ctrl Pts',(7.04417052199994,11.6,7.86256991699998));
#209714=CARTESIAN_POINT('Ctrl Pts',(7.04260821999994,15.2,7.86141585299998));
#209715=CARTESIAN_POINT('Ctrl Pts',(7.04260821999994,11.6,7.86141585299998));
#209716=CARTESIAN_POINT('Ctrl Pts',(7.04105272899994,15.2,7.86026463599999));
#209717=CARTESIAN_POINT('Ctrl Pts',(7.04105272899994,11.6,7.86026463599999));
#209718=CARTESIAN_POINT('Ctrl Pts',(7.03950405599994,15.2,7.85911628399998));
#209719=CARTESIAN_POINT('Ctrl Pts',(7.03950405599994,11.6,7.85911628399998));
#209720=CARTESIAN_POINT('Ctrl Pts',(7.03796220599994,15.2,7.85797081599998));
#209721=CARTESIAN_POINT('Ctrl Pts',(7.03796220599994,11.6,7.85797081599998));
#209722=CARTESIAN_POINT('Ctrl Pts',(7.03642718499994,15.2,7.85682825099999));
#209723=CARTESIAN_POINT('Ctrl Pts',(7.03642718499994,11.6,7.85682825099999));
#209724=CARTESIAN_POINT('Ctrl Pts',(7.03489899799994,15.2,7.85568860799999));
#209725=CARTESIAN_POINT('Ctrl Pts',(7.03489899799994,11.6,7.85568860799999));
#209726=CARTESIAN_POINT('Ctrl Pts',(7.03337765099994,15.2,7.85455190599999));
#209727=CARTESIAN_POINT('Ctrl Pts',(7.03337765099994,11.6,7.85455190599999));
#209728=CARTESIAN_POINT('Ctrl Pts',(7.03186315099994,15.2,7.85341816499999));
#209729=CARTESIAN_POINT('Ctrl Pts',(7.03186315099994,11.6,7.85341816499999));
#209730=CARTESIAN_POINT('Ctrl Pts',(7.03035550199994,15.2,7.85228740399998));
#209731=CARTESIAN_POINT('Ctrl Pts',(7.03035550199994,11.6,7.85228740399998));
#209732=CARTESIAN_POINT('Ctrl Pts',(7.02885470999994,15.2,7.85115964099998));
#209733=CARTESIAN_POINT('Ctrl Pts',(7.02885470999994,11.6,7.85115964099998));
#209734=CARTESIAN_POINT('Ctrl Pts',(7.02736078099995,15.2,7.85003489699999));
#209735=CARTESIAN_POINT('Ctrl Pts',(7.02736078099995,11.6,7.85003489699999));
#209736=CARTESIAN_POINT('Ctrl Pts',(7.02587372099994,15.2,7.84891319199998));
#209737=CARTESIAN_POINT('Ctrl Pts',(7.02587372099994,11.6,7.84891319199998));
#209738=CARTESIAN_POINT('Ctrl Pts',(7.02439353499994,15.2,7.84779454399998));
#209739=CARTESIAN_POINT('Ctrl Pts',(7.02439353499994,11.6,7.84779454399998));
#209740=CARTESIAN_POINT('Ctrl Pts',(7.02292022899995,15.2,7.84667897299999));
#209741=CARTESIAN_POINT('Ctrl Pts',(7.02292022899995,11.6,7.84667897299999));
#209742=CARTESIAN_POINT('Ctrl Pts',(7.02145380999994,15.2,7.84556649999999));
#209743=CARTESIAN_POINT('Ctrl Pts',(7.02145380999994,11.6,7.84556649999999));
#209744=CARTESIAN_POINT('Ctrl Pts',(7.01999428199994,15.2,7.84445714299999));
#209745=CARTESIAN_POINT('Ctrl Pts',(7.01999428199994,11.6,7.84445714299999));
#209746=CARTESIAN_POINT('Ctrl Pts',(7.01854165099994,15.2,7.84335092199999));
#209747=CARTESIAN_POINT('Ctrl Pts',(7.01854165099994,11.6,7.84335092199999));
#209748=CARTESIAN_POINT('Ctrl Pts',(7.01709592399994,15.2,7.84224785999999));
#209749=CARTESIAN_POINT('Ctrl Pts',(7.01709592399994,11.6,7.84224785999999));
#209750=CARTESIAN_POINT('Ctrl Pts',(7.01565710599994,15.2,7.84114797299999));
#209751=CARTESIAN_POINT('Ctrl Pts',(7.01565710599994,11.6,7.84114797299999));
#209752=CARTESIAN_POINT('Ctrl Pts',(7.01422520299994,15.2,7.84005128199999));
#209753=CARTESIAN_POINT('Ctrl Pts',(7.01422520299994,11.6,7.84005128199999));
#209754=CARTESIAN_POINT('Ctrl Pts',(7.01280021999994,15.2,7.83895780899999));
#209755=CARTESIAN_POINT('Ctrl Pts',(7.01280021999994,11.6,7.83895780899999));
#209756=CARTESIAN_POINT('Ctrl Pts',(7.01138216299994,15.2,7.83786757399999));
#209757=CARTESIAN_POINT('Ctrl Pts',(7.01138216299994,11.6,7.83786757399999));
#209758=CARTESIAN_POINT('Ctrl Pts',(7.00997103899994,15.2,7.83678059499999));
#209759=CARTESIAN_POINT('Ctrl Pts',(7.00997103899994,11.6,7.83678059499999));
#209760=CARTESIAN_POINT('Ctrl Pts',(7.00856685299994,15.2,7.83569689499998));
#209761=CARTESIAN_POINT('Ctrl Pts',(7.00856685299994,11.6,7.83569689499998));
#209762=CARTESIAN_POINT('Ctrl Pts',(7.00716961099995,15.2,7.83461649299999));
#209763=CARTESIAN_POINT('Ctrl Pts',(7.00716961099995,11.6,7.83461649299999));
#209764=CARTESIAN_POINT('Ctrl Pts',(7.00577931899995,15.2,7.83353940999999));
#209765=CARTESIAN_POINT('Ctrl Pts',(7.00577931899995,11.6,7.83353940999999));
#209766=CARTESIAN_POINT('Ctrl Pts',(7.00439598299995,15.2,7.83246566699999));
#209767=CARTESIAN_POINT('Ctrl Pts',(7.00439598299995,11.6,7.83246566699999));
#209768=CARTESIAN_POINT('Ctrl Pts',(7.00301960699995,15.2,7.83139528399998));
#209769=CARTESIAN_POINT('Ctrl Pts',(7.00301960699995,11.6,7.83139528399998));
#209770=CARTESIAN_POINT('Ctrl Pts',(7.00165019899995,15.2,7.83032828199998));
#209771=CARTESIAN_POINT('Ctrl Pts',(7.00165019899995,11.6,7.83032828199998));
#209772=CARTESIAN_POINT('Ctrl Pts',(7.00028776499994,15.2,7.82926468199998));
#209773=CARTESIAN_POINT('Ctrl Pts',(7.00028776499994,11.6,7.82926468199998));
#209774=CARTESIAN_POINT('Ctrl Pts',(6.99893230999994,15.2,7.82820450599999));
#209775=CARTESIAN_POINT('Ctrl Pts',(6.99893230999994,11.6,7.82820450599999));
#209776=CARTESIAN_POINT('Ctrl Pts',(6.99758383999994,15.2,7.82714777299999));
#209777=CARTESIAN_POINT('Ctrl Pts',(6.99758383999994,11.6,7.82714777299999));
#209778=CARTESIAN_POINT('Ctrl Pts',(6.99624235999995,15.2,7.82609450599999));
#209779=CARTESIAN_POINT('Ctrl Pts',(6.99624235999995,11.6,7.82609450599999));
#209780=CARTESIAN_POINT('Ctrl Pts',(6.99490787799994,15.2,7.82504472499999));
#209781=CARTESIAN_POINT('Ctrl Pts',(6.99490787799994,11.6,7.82504472499999));
#209782=CARTESIAN_POINT('Ctrl Pts',(6.99358039899994,15.2,7.82399845199999));
#209783=CARTESIAN_POINT('Ctrl Pts',(6.99358039899994,11.6,7.82399845199999));
#209784=CARTESIAN_POINT('Ctrl Pts',(6.99225992899994,15.2,7.82295570799998));
#209785=CARTESIAN_POINT('Ctrl Pts',(6.99225992899994,11.6,7.82295570799998));
#209786=CARTESIAN_POINT('Ctrl Pts',(6.99094647299995,15.2,7.82191651399998));
#209787=CARTESIAN_POINT('Ctrl Pts',(6.99094647299995,11.6,7.82191651399998));
#209788=CARTESIAN_POINT('Ctrl Pts',(6.98964003699994,15.2,7.82088089299998));
#209789=CARTESIAN_POINT('Ctrl Pts',(6.98964003699994,11.6,7.82088089299998));
#209790=CARTESIAN_POINT('Ctrl Pts',(6.98834062899994,15.2,7.81984886499998));
#209791=CARTESIAN_POINT('Ctrl Pts',(6.98834062899994,11.6,7.81984886499998));
#209792=CARTESIAN_POINT('Ctrl Pts',(6.98704825399994,15.2,7.81882045299999));
#209793=CARTESIAN_POINT('Ctrl Pts',(6.98704825399994,11.6,7.81882045299999));
#209794=CARTESIAN_POINT('Ctrl Pts',(6.98576291599994,15.2,7.81779567699999));
#209795=CARTESIAN_POINT('Ctrl Pts',(6.98576291599994,11.6,7.81779567699999));
#209796=CARTESIAN_POINT('Ctrl Pts',(6.98448462399995,15.2,7.81677456099998));
#209797=CARTESIAN_POINT('Ctrl Pts',(6.98448462399995,11.6,7.81677456099998));
#209798=CARTESIAN_POINT('Ctrl Pts',(6.98321338299994,15.2,7.81575712599999));
#209799=CARTESIAN_POINT('Ctrl Pts',(6.98321338299994,11.6,7.81575712599999));
#209800=CARTESIAN_POINT('Ctrl Pts',(6.98194919799994,15.2,7.81474339399999));
#209801=CARTESIAN_POINT('Ctrl Pts',(6.98194919799994,11.6,7.81474339399999));
#209802=CARTESIAN_POINT('Ctrl Pts',(6.98069207699994,15.2,7.81373338899999));
#209803=CARTESIAN_POINT('Ctrl Pts',(6.98069207699994,11.6,7.81373338899999));
#209804=CARTESIAN_POINT('Ctrl Pts',(6.97944202299994,15.2,7.81272712999999));
#209805=CARTESIAN_POINT('Ctrl Pts',(6.97944202299994,11.6,7.81272712999999));
#209806=CARTESIAN_POINT('Ctrl Pts',(6.97819904499994,15.2,7.81172464099999));
#209807=CARTESIAN_POINT('Ctrl Pts',(6.97819904499994,11.6,7.81172464099999));
#209808=CARTESIAN_POINT('Ctrl Pts',(6.97696314799994,15.2,7.81072594499998));
#209809=CARTESIAN_POINT('Ctrl Pts',(6.97696314799994,11.6,7.81072594499998));
#209810=CARTESIAN_POINT('Ctrl Pts',(6.97573433799994,15.2,7.80973106299999));
#209811=CARTESIAN_POINT('Ctrl Pts',(6.97573433799994,11.6,7.80973106299999));
#209812=CARTESIAN_POINT('Ctrl Pts',(6.97451262099994,15.2,7.80874001999998));
#209813=CARTESIAN_POINT('Ctrl Pts',(6.97451262099994,11.6,7.80874001999998));
#209814=CARTESIAN_POINT('Ctrl Pts',(6.97329800299994,15.2,7.80775283599999));
#209815=CARTESIAN_POINT('Ctrl Pts',(6.97329800299994,11.6,7.80775283599999));
#209816=CARTESIAN_POINT('Ctrl Pts',(6.97209049099994,15.2,7.80676953499999));
#209817=CARTESIAN_POINT('Ctrl Pts',(6.97209049099994,11.6,7.80676953499999));
#209818=CARTESIAN_POINT('Ctrl Pts',(6.97089008999995,15.2,7.80579014099998));
#209819=CARTESIAN_POINT('Ctrl Pts',(6.97089008999995,11.6,7.80579014099998));
#209820=CARTESIAN_POINT('Ctrl Pts',(6.96969680699994,15.2,7.80481467599999));
#209821=CARTESIAN_POINT('Ctrl Pts',(6.96969680699994,11.6,7.80481467599999));
#209822=CARTESIAN_POINT('Ctrl Pts',(6.96851064799994,15.2,7.80384316199999));
#209823=CARTESIAN_POINT('Ctrl Pts',(6.96851064799994,11.6,7.80384316199999));
#209824=CARTESIAN_POINT('Ctrl Pts',(6.96733161899994,15.2,7.80287562399998));
#209825=CARTESIAN_POINT('Ctrl Pts',(6.96733161899994,11.6,7.80287562399998));
#209826=CARTESIAN_POINT('Ctrl Pts',(6.96615972599994,15.2,7.80191208299998));
#209827=CARTESIAN_POINT('Ctrl Pts',(6.96615972599994,11.6,7.80191208299998));
#209828=CARTESIAN_POINT('Ctrl Pts',(6.96499497599994,15.2,7.80095256499998));
#209829=CARTESIAN_POINT('Ctrl Pts',(6.96499497599994,11.6,7.80095256499998));
#209830=CARTESIAN_POINT('Ctrl Pts',(6.96383737299994,15.2,7.79999709199998));
#209831=CARTESIAN_POINT('Ctrl Pts',(6.96383737299994,11.6,7.79999709199998));
#209832=CARTESIAN_POINT('Ctrl Pts',(6.96268692599994,15.2,7.79904568799999));
#209833=CARTESIAN_POINT('Ctrl Pts',(6.96268692599994,11.6,7.79904568799999));
#209834=CARTESIAN_POINT('Ctrl Pts',(6.96154363999994,15.2,7.79809837699998));
#209835=CARTESIAN_POINT('Ctrl Pts',(6.96154363999994,11.6,7.79809837699998));
#209836=CARTESIAN_POINT('Ctrl Pts',(6.96040752099995,15.2,7.79715518299999));
#209837=CARTESIAN_POINT('Ctrl Pts',(6.96040752099995,11.6,7.79715518299999));
#209838=CARTESIAN_POINT('Ctrl Pts',(6.95927857499994,15.2,7.79621612699999));
#209839=CARTESIAN_POINT('Ctrl Pts',(6.95927857499994,11.6,7.79621612699999));
#209840=CARTESIAN_POINT('Ctrl Pts',(6.95815680999995,15.2,7.79528123599999));
#209841=CARTESIAN_POINT('Ctrl Pts',(6.95815680999995,11.6,7.79528123599999));
#209842=CARTESIAN_POINT('Ctrl Pts',(6.95704222999994,15.2,7.79435053399999));
#209843=CARTESIAN_POINT('Ctrl Pts',(6.95704222999994,11.6,7.79435053399999));
#209844=CARTESIAN_POINT('Ctrl Pts',(6.95593484299994,15.2,7.79342404499998));
#209845=CARTESIAN_POINT('Ctrl Pts',(6.95593484299994,11.6,7.79342404499998));
#209846=CARTESIAN_POINT('Ctrl Pts',(6.95483465399994,15.2,7.79250179099999));
#209847=CARTESIAN_POINT('Ctrl Pts',(6.95483465399994,11.6,7.79250179099999));
#209848=CARTESIAN_POINT('Ctrl Pts',(6.95374166999994,15.2,7.79158379899999));
#209849=CARTESIAN_POINT('Ctrl Pts',(6.95374166999994,11.6,7.79158379899999));
#209850=CARTESIAN_POINT('Ctrl Pts',(6.95265589799994,15.2,7.79067009299999));
#209851=CARTESIAN_POINT('Ctrl Pts',(6.95265589799994,11.6,7.79067009299999));
#209852=CARTESIAN_POINT('Ctrl Pts',(6.95157734299994,15.2,7.78976069699999));
#209853=CARTESIAN_POINT('Ctrl Pts',(6.95157734299994,11.6,7.78976069699999));
#209854=CARTESIAN_POINT('Ctrl Pts',(6.95050601299994,15.2,7.78885563599999));
#209855=CARTESIAN_POINT('Ctrl Pts',(6.95050601299994,11.6,7.78885563599999));
#209856=CARTESIAN_POINT('Ctrl Pts',(6.94944191299994,15.2,7.78795493399999));
#209857=CARTESIAN_POINT('Ctrl Pts',(6.94944191299994,11.6,7.78795493399999));
#209858=CARTESIAN_POINT('Ctrl Pts',(6.94838504899994,15.2,7.78705861699999));
#209859=CARTESIAN_POINT('Ctrl Pts',(6.94838504899994,11.6,7.78705861699999));
#209860=CARTESIAN_POINT('Ctrl Pts',(6.94733542899994,15.2,7.78616670999998));
#209861=CARTESIAN_POINT('Ctrl Pts',(6.94733542899994,11.6,7.78616670999998));
#209862=CARTESIAN_POINT('Ctrl Pts',(6.94629305799995,15.2,7.78527923799999));
#209863=CARTESIAN_POINT('Ctrl Pts',(6.94629305799995,11.6,7.78527923799999));
#209864=CARTESIAN_POINT('Ctrl Pts',(6.94525794399994,15.2,7.78439622599999));
#209865=CARTESIAN_POINT('Ctrl Pts',(6.94525794399994,11.6,7.78439622599999));
#209866=CARTESIAN_POINT('Ctrl Pts',(6.94423009099994,15.2,7.78351769899999));
#209867=CARTESIAN_POINT('Ctrl Pts',(6.94423009099994,11.6,7.78351769899999));
#209868=CARTESIAN_POINT('Ctrl Pts',(6.94320950799994,15.2,7.78264368299999));
#209869=CARTESIAN_POINT('Ctrl Pts',(6.94320950799994,11.6,7.78264368299999));
#209870=CARTESIAN_POINT('Ctrl Pts',(6.94219619899994,15.2,7.78177420299999));
#209871=CARTESIAN_POINT('Ctrl Pts',(6.94219619899994,11.6,7.78177420299999));
#209872=CARTESIAN_POINT('Ctrl Pts',(6.94119017399994,15.2,7.78090928599998));
#209873=CARTESIAN_POINT('Ctrl Pts',(6.94119017399994,11.6,7.78090928599998));
#209874=CARTESIAN_POINT('Ctrl Pts',(6.94019143599995,15.2,7.78004895699999));
#209875=CARTESIAN_POINT('Ctrl Pts',(6.94019143599995,11.6,7.78004895699999));
#209876=CARTESIAN_POINT('Ctrl Pts',(6.93919999399994,15.2,7.77919324299998));
#209877=CARTESIAN_POINT('Ctrl Pts',(6.93919999399994,11.6,7.77919324299998));
#209878=CARTESIAN_POINT('Ctrl Pts',(6.93821585199994,15.2,7.77834216699999));
#209879=CARTESIAN_POINT('Ctrl Pts',(6.93821585199994,11.6,7.77834216699999));
#209880=CARTESIAN_POINT('Ctrl Pts',(6.93723901899994,15.2,7.77749575799999));
#209881=CARTESIAN_POINT('Ctrl Pts',(6.93723901899994,11.6,7.77749575799999));
#209882=CARTESIAN_POINT('Ctrl Pts',(6.93626949999994,15.2,7.77665404199999));
#209883=CARTESIAN_POINT('Ctrl Pts',(6.93626949999994,11.6,7.77665404199999));
#209884=CARTESIAN_POINT('Ctrl Pts',(6.93530730199994,15.2,7.77581704399999));
#209885=CARTESIAN_POINT('Ctrl Pts',(6.93530730199994,11.6,7.77581704399999));
#209886=CARTESIAN_POINT('Ctrl Pts',(6.93435243299994,15.2,7.77498479299998));
#209887=CARTESIAN_POINT('Ctrl Pts',(6.93435243299994,11.6,7.77498479299998));
#209888=CARTESIAN_POINT('Ctrl Pts',(6.93340489699994,15.2,7.77415731199999));
#209889=CARTESIAN_POINT('Ctrl Pts',(6.93340489699994,11.6,7.77415731199999));
#209890=CARTESIAN_POINT('Ctrl Pts',(6.93246470299994,15.2,7.77333463099998));
#209891=CARTESIAN_POINT('Ctrl Pts',(6.93246470299994,11.6,7.77333463099998));
#209892=CARTESIAN_POINT('Ctrl Pts',(6.93153185599994,15.2,7.77251677599998));
#209893=CARTESIAN_POINT('Ctrl Pts',(6.93153185599994,11.6,7.77251677599998));
#209894=CARTESIAN_POINT('Ctrl Pts',(6.93060636299994,15.2,7.77170377399998));
#209895=CARTESIAN_POINT('Ctrl Pts',(6.93060636299994,11.6,7.77170377399998));
#209896=CARTESIAN_POINT('Ctrl Pts',(6.92968823199994,15.2,7.77089565099998));
#209897=CARTESIAN_POINT('Ctrl Pts',(6.92968823199994,11.6,7.77089565099998));
#209898=CARTESIAN_POINT('Ctrl Pts',(6.92877746799994,15.2,7.77009243499998));
#209899=CARTESIAN_POINT('Ctrl Pts',(6.92877746799994,11.6,7.77009243499998));
#209900=CARTESIAN_POINT('Ctrl Pts',(6.92787407799995,15.2,7.76929415399999));
#209901=CARTESIAN_POINT('Ctrl Pts',(6.92787407799995,11.6,7.76929415399999));
#209902=CARTESIAN_POINT('Ctrl Pts',(6.92697806899995,15.2,7.76850083499999));
#209903=CARTESIAN_POINT('Ctrl Pts',(6.92697806899995,11.6,7.76850083499999));
#209904=CARTESIAN_POINT('Ctrl Pts',(6.92608944799994,15.2,7.76771250599998));
#209905=CARTESIAN_POINT('Ctrl Pts',(6.92608944799994,11.6,7.76771250599998));
#209906=CARTESIAN_POINT('Ctrl Pts',(6.92520822199994,15.2,7.76692919399999));
#209907=CARTESIAN_POINT('Ctrl Pts',(6.92520822199994,11.6,7.76692919399999));
#209908=CARTESIAN_POINT('Ctrl Pts',(6.92433439799994,15.2,7.76615092899998));
#209909=CARTESIAN_POINT('Ctrl Pts',(6.92433439799994,11.6,7.76615092899998));
#209910=CARTESIAN_POINT('Ctrl Pts',(6.92346798099994,15.2,7.76537773499999));
#209911=CARTESIAN_POINT('Ctrl Pts',(6.92346798099994,11.6,7.76537773499999));
#209912=CARTESIAN_POINT('Ctrl Pts',(6.92260897899994,15.2,7.76460964399998));
#209913=CARTESIAN_POINT('Ctrl Pts',(6.92260897899994,11.6,7.76460964399998));
#209914=CARTESIAN_POINT('Ctrl Pts',(6.92175739999994,15.2,7.76384668399999));
#209915=CARTESIAN_POINT('Ctrl Pts',(6.92175739999994,11.6,7.76384668399999));
#209916=CARTESIAN_POINT('Ctrl Pts',(6.92091324799994,15.2,7.76308888099998));
#209917=CARTESIAN_POINT('Ctrl Pts',(6.92091324799994,11.6,7.76308888099998));
#209918=CARTESIAN_POINT('Ctrl Pts',(6.92007653299994,15.2,7.76233626499998));
#209919=CARTESIAN_POINT('Ctrl Pts',(6.92007653299994,11.6,7.76233626499998));
#209920=CARTESIAN_POINT('Ctrl Pts',(6.91924725999994,15.2,7.76158886499999));
#209921=CARTESIAN_POINT('Ctrl Pts',(6.91924725999994,11.6,7.76158886499999));
#209922=CARTESIAN_POINT('Ctrl Pts',(6.91842543599994,15.2,7.76084670899999));
#209923=CARTESIAN_POINT('Ctrl Pts',(6.91842543599994,11.6,7.76084670899999));
#209924=CARTESIAN_POINT('Ctrl Pts',(6.91761106799994,15.2,7.76010982799999));
#209925=CARTESIAN_POINT('Ctrl Pts',(6.91761106799994,11.6,7.76010982799999));
#209926=CARTESIAN_POINT('Ctrl Pts',(6.91680416399994,15.2,7.75937824799998));
#209927=CARTESIAN_POINT('Ctrl Pts',(6.91680416399994,11.6,7.75937824799998));
#209928=CARTESIAN_POINT('Ctrl Pts',(6.91600472999994,15.2,7.75865200199998));
#209929=CARTESIAN_POINT('Ctrl Pts',(6.91600472999994,11.6,7.75865200199998));
#209930=CARTESIAN_POINT('Ctrl Pts',(6.91521277299994,15.2,7.75793111599998));
#209931=CARTESIAN_POINT('Ctrl Pts',(6.91521277299994,11.6,7.75793111599998));
#209932=CARTESIAN_POINT('Ctrl Pts',(6.91442829999994,15.2,7.75721562099999));
#209933=CARTESIAN_POINT('Ctrl Pts',(6.91442829999994,11.6,7.75721562099999));
#209934=CARTESIAN_POINT('Ctrl Pts',(6.91365131899994,15.2,7.75650554699999));
#209935=CARTESIAN_POINT('Ctrl Pts',(6.91365131899994,11.6,7.75650554699999));
#209936=CARTESIAN_POINT('Ctrl Pts',(6.91288183599994,15.2,7.75580092399998));
#209937=CARTESIAN_POINT('Ctrl Pts',(6.91288183599994,11.6,7.75580092399998));
#209938=CARTESIAN_POINT('Ctrl Pts',(6.91211985799994,15.2,7.75510178099999));
#209939=CARTESIAN_POINT('Ctrl Pts',(6.91211985799994,11.6,7.75510178099999));
#209940=CARTESIAN_POINT('Ctrl Pts',(6.91136539199994,15.2,7.75440814799998));
#209941=CARTESIAN_POINT('Ctrl Pts',(6.91136539199994,11.6,7.75440814799998));
#209942=CARTESIAN_POINT('Ctrl Pts',(6.91061844599994,15.2,7.75372005799999));
#209943=CARTESIAN_POINT('Ctrl Pts',(6.91061844599994,11.6,7.75372005799999));
#209944=CARTESIAN_POINT('Ctrl Pts',(6.90987902599994,15.2,7.75303753699998));
#209945=CARTESIAN_POINT('Ctrl Pts',(6.90987902599994,11.6,7.75303753699998));
#209946=CARTESIAN_POINT('Ctrl Pts',(6.90914713999994,15.2,7.75236061999999));
#209947=CARTESIAN_POINT('Ctrl Pts',(6.90914713999994,11.6,7.75236061999999));
#209948=CARTESIAN_POINT('Ctrl Pts',(6.90842279599994,15.2,7.75168933599998));
#209949=CARTESIAN_POINT('Ctrl Pts',(6.90842279599994,11.6,7.75168933599998));
#209950=CARTESIAN_POINT('Ctrl Pts',(6.90770599799994,15.2,7.75102371499998));
#209951=CARTESIAN_POINT('Ctrl Pts',(6.90770599799994,11.6,7.75102371499998));
#209952=CARTESIAN_POINT('Ctrl Pts',(6.90699675699994,15.2,7.75036378799999));
#209953=CARTESIAN_POINT('Ctrl Pts',(6.90699675699994,11.6,7.75036378799999));
#209954=CARTESIAN_POINT('Ctrl Pts',(6.90629507799994,15.2,7.74970958799998));
#209955=CARTESIAN_POINT('Ctrl Pts',(6.90629507799994,11.6,7.74970958799998));
#209956=CARTESIAN_POINT('Ctrl Pts',(6.90560096999994,15.2,7.74906114499998));
#209957=CARTESIAN_POINT('Ctrl Pts',(6.90560096999994,11.6,7.74906114499998));
#209958=CARTESIAN_POINT('Ctrl Pts',(6.90491443699995,15.2,7.74841849099998));
#209959=CARTESIAN_POINT('Ctrl Pts',(6.90491443699995,11.6,7.74841849099998));
#209960=CARTESIAN_POINT('Ctrl Pts',(6.90423548999994,15.2,7.74778165899999));
#209961=CARTESIAN_POINT('Ctrl Pts',(6.90423548999994,11.6,7.74778165899999));
#209962=CARTESIAN_POINT('Ctrl Pts',(6.90356800099994,15.2,7.74715431199999));
#209963=CARTESIAN_POINT('Ctrl Pts',(6.90356800099994,11.6,7.74715431199999));
#209964=CARTESIAN_POINT('Ctrl Pts',(6.90304077499994,15.2,7.74665780099999));
#209965=CARTESIAN_POINT('Ctrl Pts',(6.90304077499994,11.6,7.74665780099999));
#209966=CARTESIAN_POINT('Ctrl Pts',(6.90264966999995,15.2,7.74628893099998));
#209967=CARTESIAN_POINT('Ctrl Pts',(6.90264966999995,11.6,7.74628893099998));
#209968=CARTESIAN_POINT('Ctrl Pts',(6.90239167399994,15.2,7.74604536199998));
#209969=CARTESIAN_POINT('Ctrl Pts',(6.90239167399994,11.6,7.74604536199998));
#209970=CARTESIAN_POINT('Ctrl Pts',(6.90226491999994,15.2,7.74592563799998));
#209971=CARTESIAN_POINT('Ctrl Pts',(6.90226491999994,11.6,7.74592563799998));
#209972=CARTESIAN_POINT('',(6.90226491999994,12.2,7.74592563699999));
#209973=CARTESIAN_POINT('',(6.90226491999994,15.2,7.74592563699999));
#209974=CARTESIAN_POINT('',(6.90226491999994,12.2,7.74592563799998));
#209975=CARTESIAN_POINT('Ctrl Pts',(7.93573928199995,12.2,8.32310290899999));
#209976=CARTESIAN_POINT('Ctrl Pts',(7.93215544959198,12.2,8.32177216810586));
#209977=CARTESIAN_POINT('Ctrl Pts',(7.92857931898359,12.2,8.32043968349314));
#209978=CARTESIAN_POINT('Ctrl Pts',(7.92501089566235,12.2,8.31910545566979));
#209979=CARTESIAN_POINT('Ctrl Pts',(7.92144247234111,12.2,8.31777122784644));
#209980=CARTESIAN_POINT('Ctrl Pts',(7.91788175450335,12.2,8.31643525707682));
#209981=CARTESIAN_POINT('Ctrl Pts',(7.91432875270405,12.2,8.31509755705879));
#209982=CARTESIAN_POINT('Ctrl Pts',(7.91077575090475,12.2,8.31375985704076));
#209983=CARTESIAN_POINT('Ctrl Pts',(7.90723046416027,12.2,8.31242042797674));
#209984=CARTESIAN_POINT('Ctrl Pts',(7.90369291574608,12.2,8.3110793087757));
#209985=CARTESIAN_POINT('Ctrl Pts',(7.90015536668924,12.2,8.30973818933102));
#209986=CARTESIAN_POINT('Ctrl Pts',(7.89662555635958,12.2,8.3083953802692));
#209987=CARTESIAN_POINT('Ctrl Pts',(7.89310351022376,12.2,8.30705092374024));
#209988=CARTESIAN_POINT('Ctrl Pts',(7.88958146472777,12.2,8.30570646745552));
#209989=CARTESIAN_POINT('Ctrl Pts',(7.88606718263972,12.2,8.3043603634209));
#209990=CARTESIAN_POINT('Ctrl Pts',(7.88256068510114,12.2,8.3030126456364));
#209991=CARTESIAN_POINT('Ctrl Pts',(7.87905418756256,12.2,8.30166492785189));
#209992=CARTESIAN_POINT('Ctrl Pts',(7.87555547396904,12.2,8.30031559723916));
#209993=CARTESIAN_POINT('Ctrl Pts',(7.87206456249672,12.2,8.2989646830321));
#209994=CARTESIAN_POINT('Ctrl Pts',(7.8685736510244,12.2,8.29761376882504));
#209995=CARTESIAN_POINT('Ctrl Pts',(7.86509054247593,12.2,8.29626127245817));
#209996=CARTESIAN_POINT('Ctrl Pts',(7.86161525800305,12.2,8.29490723070956));
#209997=CARTESIAN_POINT('Ctrl Pts',(7.85813997353015,12.2,8.29355318896095));
#209998=CARTESIAN_POINT('Ctrl Pts',(7.85467251306878,12.2,8.29219760129846));
#209999=CARTESIAN_POINT('Ctrl Pts',(7.85121289811045,12.2,8.2908405040979));
#210000=CARTESIAN_POINT('Ctrl Pts',(7.84775328315213,12.2,8.28948340689733));
#210001=CARTESIAN_POINT('Ctrl Pts',(7.84430151397661,12.2,8.28812480174687));
#210002=CARTESIAN_POINT('Ctrl Pts',(7.84085761097567,12.2,8.28676472200483));
#210003=CARTESIAN_POINT('Ctrl Pts',(7.83741370734909,12.2,8.28540464201569));
#210004=CARTESIAN_POINT('Ctrl Pts',(7.83397767014971,12.2,8.28404308871781));
#210005=CARTESIAN_POINT('Ctrl Pts',(7.83054951952756,12.2,8.2826800971862));
#210006=CARTESIAN_POINT('Ctrl Pts',(7.82597865306934,12.2,8.28086277555672));
#210007=CARTESIAN_POINT('Ctrl Pts',(7.82142180716063,12.2,8.27904289774109));
#210008=CARTESIAN_POINT('Ctrl Pts',(7.81687903201132,12.2,8.2772205494929));
#210009=CARTESIAN_POINT('Ctrl Pts',(7.8134719504946,12.2,8.2758537882447));
#210010=CARTESIAN_POINT('Ctrl Pts',(7.81007278366381,12.2,8.27448563769937));
#210011=CARTESIAN_POINT('Ctrl Pts',(7.80668155266133,12.2,8.27311613487425));
#210012=CARTESIAN_POINT('Ctrl Pts',(7.80329032165885,12.2,8.27174663204912));
#210013=CARTESIAN_POINT('Ctrl Pts',(7.79990702573084,12.2,8.27037577563242));
#210014=CARTESIAN_POINT('Ctrl Pts',(7.79653168718572,12.2,8.2690036042658));
#210015=CARTESIAN_POINT('Ctrl Pts',(7.79203123538343,12.2,8.26717404227743));
#210016=CARTESIAN_POINT('Ctrl Pts',(7.78754492816917,12.2,8.26534214082649));
#210017=CARTESIAN_POINT('Ctrl Pts',(7.78307281573851,12.2,8.26350798777374));
#210018=CARTESIAN_POINT('Ctrl Pts',(7.77971873172017,12.2,8.26213237310913));
#210019=CARTESIAN_POINT('Ctrl Pts',(7.7763726315135,12.2,8.26075549297409));
#210020=CARTESIAN_POINT('Ctrl Pts',(7.77303453703626,12.2,8.25937738322624));
#210021=CARTESIAN_POINT('Ctrl Pts',(7.76969644255901,12.2,8.2579992734784));
#210022=CARTESIAN_POINT('Ctrl Pts',(7.76636635434213,12.2,8.25661993398352));
#210023=CARTESIAN_POINT('Ctrl Pts',(7.76304429187879,12.2,8.25523940465878));
#210024=CARTESIAN_POINT('Ctrl Pts',(7.75972222941546,12.2,8.25385887533405));
#210025=CARTESIAN_POINT('Ctrl Pts',(7.75640819301825,12.2,8.25247715455105));
#210026=CARTESIAN_POINT('Ctrl Pts',(7.7531022049706,12.2,8.25109428026813));
#210027=CARTESIAN_POINT('Ctrl Pts',(7.74979621632237,12.2,8.24971140573397));
#210028=CARTESIAN_POINT('Ctrl Pts',(7.74649827459306,12.2,8.24832737726616));
#210029=CARTESIAN_POINT('Ctrl Pts',(7.74320840103271,12.2,8.24694223473137));
#210030=CARTESIAN_POINT('Ctrl Pts',(7.73882190394833,12.2,8.24509537843771));
#210031=CARTESIAN_POINT('Ctrl Pts',(7.73444975060651,12.2,8.24324653931095));
#210032=CARTESIAN_POINT('Ctrl Pts',(7.73009199207294,12.2,8.2413958096846));
#210033=CARTESIAN_POINT('Ctrl Pts',(7.72682367302432,12.2,8.2400077624018));
#210034=CARTESIAN_POINT('Ctrl Pts',(7.72356345029108,12.2,8.23861865100442));
#210035=CARTESIAN_POINT('Ctrl Pts',(7.72031134462083,12.2,8.23722851473561));
#210036=CARTESIAN_POINT('Ctrl Pts',(7.71705923895058,12.2,8.23583837846679));
#210037=CARTESIAN_POINT('Ctrl Pts',(7.71381525122218,12.2,8.23444721781943));
#210038=CARTESIAN_POINT('Ctrl Pts',(7.71057940175531,12.2,8.23305507103681));
#210039=CARTESIAN_POINT('Ctrl Pts',(7.70734355170059,12.2,8.23166292400128));
#210040=CARTESIAN_POINT('Ctrl Pts',(7.70411584061482,12.2,8.23026979023215));
#210041=CARTESIAN_POINT('Ctrl Pts',(7.7008962890647,12.2,8.22887571073775));
#210042=CARTESIAN_POINT('Ctrl Pts',(7.69767673809946,12.2,8.22748163149661));
#210043=CARTESIAN_POINT('Ctrl Pts',(7.69446534661711,12.2,8.22608660629718));
#210044=CARTESIAN_POINT('Ctrl Pts',(7.69126213615087,12.2,8.22469067359782));
#210045=CARTESIAN_POINT('Ctrl Pts',(7.68805892568464,12.2,8.22329474089846));
#210046=CARTESIAN_POINT('Ctrl Pts',(7.68486389702898,12.2,8.22189790047096));
#210047=CARTESIAN_POINT('Ctrl Pts',(7.681677069547,12.2,8.22050019372372));
#210048=CARTESIAN_POINT('Ctrl Pts',(7.67849024206501,12.2,8.21910248697649));
#210049=CARTESIAN_POINT('Ctrl Pts',(7.67531161630202,12.2,8.21770391327344));
#210050=CARTESIAN_POINT('Ctrl Pts',(7.67214121427777,12.2,8.21630451302626));
#210051=CARTESIAN_POINT('Ctrl Pts',(7.66897081225352,12.2,8.21490511277908));
#210052=CARTESIAN_POINT('Ctrl Pts',(7.6658086330966,12.2,8.21350488585172));
#210053=CARTESIAN_POINT('Ctrl Pts',(7.66265469812714,12.2,8.21210387169435));
#210054=CARTESIAN_POINT('Ctrl Pts',(7.65950076315769,12.2,8.210702857537));
#210055=CARTESIAN_POINT('Ctrl Pts',(7.65635507218765,12.2,8.20930105643801));
#210056=CARTESIAN_POINT('Ctrl Pts',(7.65321764763385,12.2,8.20789851028074));
#210057=CARTESIAN_POINT('Ctrl Pts',(7.6500802225101,12.2,8.20649596386868));
#210058=CARTESIAN_POINT('Ctrl Pts',(7.64695106222198,12.2,8.20509267201473));
#210059=CARTESIAN_POINT('Ctrl Pts',(7.64383018956121,12.2,8.20368867464392));
#210060=CARTESIAN_POINT('Ctrl Pts',(7.6407093174674,12.2,8.20228467752817));
#210061=CARTESIAN_POINT('Ctrl Pts',(7.63759673159069,12.2,8.2008799767973));
#210062=CARTESIAN_POINT('Ctrl Pts',(7.63449245392437,12.2,8.19947461198641));
#210063=CARTESIAN_POINT('Ctrl Pts',(7.63138817625805,12.2,8.19806924717553));
#210064=CARTESIAN_POINT('Ctrl Pts',(7.62829220711722,12.2,8.19666321812894));
#210065=CARTESIAN_POINT('Ctrl Pts',(7.62520456668847,12.2,8.19525656788832));
#210066=CARTESIAN_POINT('Ctrl Pts',(7.62211692625973,12.2,8.19384991764772));
#210067=CARTESIAN_POINT('Ctrl Pts',(7.61903761517164,12.2,8.19244264523217));
#210068=CARTESIAN_POINT('Ctrl Pts',(7.61596665519988,12.2,8.19103479303333));
#210069=CARTESIAN_POINT('Ctrl Pts',(7.61289569522812,12.2,8.18962694083447));
#210070=CARTESIAN_POINT('Ctrl Pts',(7.60983308597269,12.2,8.18821850803565));
#210071=CARTESIAN_POINT('Ctrl Pts',(7.60677884804128,12.2,8.18680953742023));
#210072=CARTESIAN_POINT('Ctrl Pts',(7.60372461010986,12.2,8.18540056680481));
#210073=CARTESIAN_POINT('Ctrl Pts',(7.60067874519667,12.2,8.18399105870861));
#210074=CARTESIAN_POINT('Ctrl Pts',(7.59764127257098,12.2,8.18258105498112));
#210075=CARTESIAN_POINT('Ctrl Pts',(7.59460379994529,12.2,8.18117105125363));
#210076=CARTESIAN_POINT('Ctrl Pts',(7.59157472121646,12.2,8.17976055197292));
#210077=CARTESIAN_POINT('Ctrl Pts',(7.58855405670006,12.2,8.17834959981591));
#210078=CARTESIAN_POINT('Ctrl Pts',(7.58452650364569,12.2,8.17646833010235));
#210079=CARTESIAN_POINT('Ctrl Pts',(7.58051390929275,12.2,8.17458625549982));
#210080=CARTESIAN_POINT('Ctrl Pts',(7.57651632624155,12.2,8.17270347900832));
#210081=CARTESIAN_POINT('Ctrl Pts',(7.57251874319034,12.2,8.17082070251681));
#210082=CARTESIAN_POINT('Ctrl Pts',(7.56853617010479,12.2,8.16893722303636));
#210083=CARTESIAN_POINT('Ctrl Pts',(7.56456865833454,12.2,8.16705314343361));
#210084=CARTESIAN_POINT('Ctrl Pts',(7.56060114710487,12.2,8.16516906408757));
#210085=CARTESIAN_POINT('Ctrl Pts',(7.55664869510975,12.2,8.16328438574739));
#210086=CARTESIAN_POINT('Ctrl Pts',(7.55271135596924,12.2,8.16139921172627));
#210087=CARTESIAN_POINT('Ctrl Pts',(7.54778968164126,12.2,8.15904274400723));
#210088=CARTESIAN_POINT('Ctrl Pts',(7.542891619961,12.2,8.1566855032111));
#210089=CARTESIAN_POINT('Ctrl Pts',(7.53801727051655,12.2,8.15432769376665));
#210090=CARTESIAN_POINT('Ctrl Pts',(7.53411779074846,12.2,8.1524414461083));
#210091=CARTESIAN_POINT('Ctrl Pts',(7.53023348539883,12.2,8.1505548338999));
#210092=CARTESIAN_POINT('Ctrl Pts',(7.52636440763396,12.2,8.14866796490815));
#210093=CARTESIAN_POINT('Ctrl Pts',(7.52249533039625,12.2,8.14678109617349));
#210094=CARTESIAN_POINT('Ctrl Pts',(7.51864147712563,12.2,8.14489397024166));
#210095=CARTESIAN_POINT('Ctrl Pts',(7.5148029044775,12.2,8.14300669477627));
#210096=CARTESIAN_POINT('Ctrl Pts',(7.51096433130638,12.2,8.14111941905374));
#210097=CARTESIAN_POINT('Ctrl Pts',(7.50714103536659,12.2,8.13923199363592));
#210098=CARTESIAN_POINT('Ctrl Pts',(7.50333306782729,12.2,8.13734452669972));
#210099=CARTESIAN_POINT('Ctrl Pts',(7.49952510080683,12.2,8.13545706002067));
#210100=CARTESIAN_POINT('Ctrl Pts',(7.49573246366214,12.2,8.1335695518222));
#210101=CARTESIAN_POINT('Ctrl Pts',(7.49195520652549,12.2,8.13168211242095));
#210102=CARTESIAN_POINT('Ctrl Pts',(7.48817794887418,12.2,8.12979467276254));
#210103=CARTESIAN_POINT('Ctrl Pts',(7.4844160713158,12.2,8.12790730122882));
#210104=CARTESIAN_POINT('Ctrl Pts',(7.48066962598134,12.2,8.12602010947614));
#210105=CARTESIAN_POINT('Ctrl Pts',(7.47692318115733,12.2,8.12413291798059));
#210106=CARTESIAN_POINT('Ctrl Pts',(7.47319216701493,12.2,8.122245904425));
#210107=CARTESIAN_POINT('Ctrl Pts',(7.46947663659545,12.2,8.12035918241256));
#210108=CARTESIAN_POINT('Ctrl Pts',(7.46576110566972,12.2,8.11847246014305));
#210109=CARTESIAN_POINT('Ctrl Pts',(7.4620610583875,12.2,8.11658603009579));
#210110=CARTESIAN_POINT('Ctrl Pts',(7.45837654596549,12.2,8.11470000260414));
#210111=CARTESIAN_POINT('Ctrl Pts',(7.4546920340455,12.2,8.11281397536946));
#210112=CARTESIAN_POINT('Ctrl Pts',(7.45102305555418,12.2,8.11092835311085));
#210113=CARTESIAN_POINT('Ctrl Pts',(7.4473696647801,12.2,8.10904324778186));
#210114=CARTESIAN_POINT('Ctrl Pts',(7.44280292593917,12.2,8.10668686592799));
#210115=CARTESIAN_POINT('Ctrl Pts',(7.43826054062456,12.2,8.10433129402626));
#210116=CARTESIAN_POINT('Ctrl Pts',(7.43374261055384,12.2,8.10197675638731));
#210117=CARTESIAN_POINT('Ctrl Pts',(7.42922468048313,12.2,8.09962221874837));
#210118=CARTESIAN_POINT('Ctrl Pts',(7.42473120554358,12.2,8.09726871679834));
#210119=CARTESIAN_POINT('Ctrl Pts',(7.42026228700063,12.2,8.09491647735383));
#210120=CARTESIAN_POINT('Ctrl Pts',(7.41668715197141,12.2,8.09303468569566));
#210121=CARTESIAN_POINT('Ctrl Pts',(7.41312773254409,12.2,8.09115370204313));
#210122=CARTESIAN_POINT('Ctrl Pts',(7.40958408218534,12.2,8.08927364582963));
#210123=CARTESIAN_POINT('Ctrl Pts',(7.40604043230941,12.2,8.08739358987228));
#210124=CARTESIAN_POINT('Ctrl Pts',(7.40251254992986,12.2,8.08551446027678));
#210125=CARTESIAN_POINT('Ctrl Pts',(7.39900048798459,12.2,8.08363637628084));
#210126=CARTESIAN_POINT('Ctrl Pts',(7.3954884255608,12.2,8.08175829202902));
#210127=CARTESIAN_POINT('Ctrl Pts',(7.39199218376249,12.2,8.07988125432658));
#210128=CARTESIAN_POINT('Ctrl Pts',(7.38851181474051,12.2,8.0780053841133));
#210129=CARTESIAN_POINT('Ctrl Pts',(7.38503144619273,12.2,8.07612951415561));
#210130=CARTESIAN_POINT('Ctrl Pts',(7.38156695127788,12.2,8.07425480986715));
#210131=CARTESIAN_POINT('Ctrl Pts',(7.37811838011373,12.2,8.07238139529795));
#210132=CARTESIAN_POINT('Ctrl Pts',(7.37466980847971,12.2,8.0705079804735));
#210133=CARTESIAN_POINT('Ctrl Pts',(7.37123716157424,12.2,8.06863585487305));
#210134=CARTESIAN_POINT('Ctrl Pts',(7.36782049253923,12.2,8.06676514070704));
#210135=CARTESIAN_POINT('Ctrl Pts',(7.36440382396974,12.2,8.06489442679591));
#210136=CARTESIAN_POINT('Ctrl Pts',(7.36100313115045,12.2,8.06302512548616));
#210137=CARTESIAN_POINT('Ctrl Pts',(7.35761847053661,12.2,8.06115736097203));
#210138=CARTESIAN_POINT('Ctrl Pts',(7.35423380946162,12.2,8.05928959620341));
#210139=CARTESIAN_POINT('Ctrl Pts',(7.3508651769437,12.2,8.05742336837106));
#210140=CARTESIAN_POINT('Ctrl Pts',(7.34751262798321,12.2,8.05555880299165));
#210141=CARTESIAN_POINT('Ctrl Pts',(7.34416007902272,12.2,8.05369423761223));
#210142=CARTESIAN_POINT('Ctrl Pts',(7.34082361337521,12.2,8.05183133561638));
#210143=CARTESIAN_POINT('Ctrl Pts',(7.33750328297369,12.2,8.04997022290402));
#210144=CARTESIAN_POINT('Ctrl Pts',(7.33418295302456,12.2,8.04810911044525));
#210145=CARTESIAN_POINT('Ctrl Pts',(7.3308787572122,12.2,8.04624978857173));
#210146=CARTESIAN_POINT('Ctrl Pts',(7.32759075074379,12.2,8.04439238599291));
#210147=CARTESIAN_POINT('Ctrl Pts',(7.32430274382739,12.2,8.04253498316102));
#210148=CARTESIAN_POINT('Ctrl Pts',(7.32103092687394,12.2,8.0406794974283));
#210149=CARTESIAN_POINT('Ctrl Pts',(7.31777534997593,12.2,8.03882606193861));
#210150=CARTESIAN_POINT('Ctrl Pts',(7.3145197735215,12.2,8.03697262670143));
#210151=CARTESIAN_POINT('Ctrl Pts',(7.31128043879833,12.2,8.03512124026681));
#210152=CARTESIAN_POINT('Ctrl Pts',(7.30805739900519,12.2,8.03327203441784));
#210153=CARTESIAN_POINT('Ctrl Pts',(7.3048343587729,12.2,8.0314228283169));
#210154=CARTESIAN_POINT('Ctrl Pts',(7.30162761399941,12.2,8.02957580092479));
#210155=CARTESIAN_POINT('Ctrl Pts',(7.29843721627869,12.2,8.02773108873231));
#210156=CARTESIAN_POINT('Ctrl Pts',(7.29524681899266,12.2,8.02588637679116));
#210157=CARTESIAN_POINT('Ctrl Pts',(7.29207277096222,12.2,8.02404397850571));
#210158=CARTESIAN_POINT('Ctrl Pts',(7.28891512377484,12.2,8.02220402743375));
#210159=CARTESIAN_POINT('Ctrl Pts',(7.28496806446794,12.2,8.01990408840578));
#210160=CARTESIAN_POINT('Ctrl Pts',(7.28104663162282,12.2,8.01760797478344));
#210161=CARTESIAN_POINT('Ctrl Pts',(7.27715093224648,12.2,8.01531595165823));
#210162=CARTESIAN_POINT('Ctrl Pts',(7.27403437257556,12.2,8.01348233305813));
#210163=CARTESIAN_POINT('Ctrl Pts',(7.27093428065097,12.2,8.01165133336154));
#210164=CARTESIAN_POINT('Ctrl Pts',(7.26785071155252,12.2,8.00982308922637));
#210165=CARTESIAN_POINT('Ctrl Pts',(7.26476714287421,12.2,8.00799484534028));
#210166=CARTESIAN_POINT('Ctrl Pts',(7.26170009711222,12.2,8.00616935722518));
#210167=CARTESIAN_POINT('Ctrl Pts',(7.25864962724941,12.2,8.004346764874));
#210168=CARTESIAN_POINT('Ctrl Pts',(7.25559915697098,12.2,8.00252417227449));
#210169=CARTESIAN_POINT('Ctrl Pts',(7.25256526281118,12.2,8.00070447630863));
#210170=CARTESIAN_POINT('Ctrl Pts',(7.24954799920337,12.2,7.99888781637649));
#210171=CARTESIAN_POINT('Ctrl Pts',(7.24653073600668,12.2,7.99707115669187));
#210172=CARTESIAN_POINT('Ctrl Pts',(7.24353010407009,12.2,7.99525753293597));
#210173=CARTESIAN_POINT('Ctrl Pts',(7.24054615544128,12.2,7.99344709027103));
#210174=CARTESIAN_POINT('Ctrl Pts',(7.23756220640591,12.2,7.99163664735941));
#210175=CARTESIAN_POINT('Ctrl Pts',(7.23459494211575,12.2,7.98982938229229));
#210176=CARTESIAN_POINT('Ctrl Pts',(7.23164441723382,12.2,7.98802544236086));
#210177=CARTESIAN_POINT('Ctrl Pts',(7.2286938927539,12.2,7.98622150267522));
#210178=CARTESIAN_POINT('Ctrl Pts',(7.22576010761784,12.2,7.9844208865778));
#210179=CARTESIAN_POINT('Ctrl Pts',(7.22284311574349,12.2,7.98262374033548));
#210180=CARTESIAN_POINT('Ctrl Pts',(7.21992612347169,12.2,7.98082659384829));
#210181=CARTESIAN_POINT('Ctrl Pts',(7.21702592461531,12.2,7.97903291817943));
#210182=CARTESIAN_POINT('Ctrl Pts',(7.21414257372292,12.2,7.97724286024042));
#210183=CARTESIAN_POINT('Ctrl Pts',(7.21125922322339,12.2,7.97545280254531));
#210184=CARTESIAN_POINT('Ctrl Pts',(7.20839272224845,12.2,7.97366636282386));
#210185=CARTESIAN_POINT('Ctrl Pts',(7.20554312375747,12.2,7.97188369052478));
#210186=CARTESIAN_POINT('Ctrl Pts',(7.20269352487822,12.2,7.9701010179828));
#210187=CARTESIAN_POINT('Ctrl Pts',(7.19986082836445,12.2,7.96832211230504));
#210188=CARTESIAN_POINT('Ctrl Pts',(7.19704509076654,12.2,7.96654712704164));
#210189=CARTESIAN_POINT('Ctrl Pts',(7.19352541896098,12.2,7.9643283955833));
#210190=CARTESIAN_POINT('Ctrl Pts',(7.19003224428033,12.2,7.96211578575877));
#210191=CARTESIAN_POINT('Ctrl Pts',(7.18656567426466,12.2,7.95990959949877));
#210192=CARTESIAN_POINT('Ctrl Pts',(7.18309910424899,12.2,7.95770341323877));
#210193=CARTESIAN_POINT('Ctrl Pts',(7.17965914028098,12.2,7.95550365009514));
#210194=CARTESIAN_POINT('Ctrl Pts',(7.17624588931015,12.2,7.95331061537325));
#210195=CARTESIAN_POINT('Ctrl Pts',(7.17283263833932,12.2,7.95111758065137));
#210196=CARTESIAN_POINT('Ctrl Pts',(7.1694461011067,12.2,7.94893127249602));
#210197=CARTESIAN_POINT('Ctrl Pts',(7.16608638603865,12.2,7.94675200131582));
#210198=CARTESIAN_POINT('Ctrl Pts',(7.16272667097059,12.2,7.94457273013561));
#210199=CARTESIAN_POINT('Ctrl Pts',(7.15939377867686,12.2,7.94240049478027));
#210200=CARTESIAN_POINT('Ctrl Pts',(7.1560878177755,12.2,7.9402356111001));
#210201=CARTESIAN_POINT('Ctrl Pts',(7.15278185687413,12.2,7.93807072741993));
#210202=CARTESIAN_POINT('Ctrl Pts',(7.14950282748861,12.2,7.93591319379618));
#210203=CARTESIAN_POINT('Ctrl Pts',(7.14625083968913,12.2,7.93376333000876));
#210204=CARTESIAN_POINT('Ctrl Pts',(7.14299885188964,12.2,7.93161346622133));
#210205=CARTESIAN_POINT('Ctrl Pts',(7.13977390627385,12.2,7.92947127234795));
#210206=CARTESIAN_POINT('Ctrl Pts',(7.13657611203995,12.2,7.92733707123748));
#210207=CARTESIAN_POINT('Ctrl Pts',(7.13337831780604,12.2,7.92520287012701));
#210208=CARTESIAN_POINT('Ctrl Pts',(7.13020767530872,12.2,7.9230766632167));
#210209=CARTESIAN_POINT('Ctrl Pts',(7.12706429600539,12.2,7.92095877877295));
#210210=CARTESIAN_POINT('Ctrl Pts',(7.12392091704471,12.2,7.91884089456003));
#210211=CARTESIAN_POINT('Ctrl Pts',(7.12080480014722,12.2,7.91673133285203));
#210212=CARTESIAN_POINT('Ctrl Pts',(7.11771605791223,12.2,7.91463042877477));
#210213=CARTESIAN_POINT('Ctrl Pts',(7.11462731534056,12.2,7.91252952446851));
#210214=CARTESIAN_POINT('Ctrl Pts',(7.11156594752674,12.2,7.91043727756208));
#210215=CARTESIAN_POINT('Ctrl Pts',(7.10853206641338,12.2,7.90835402825578));
#210216=CARTESIAN_POINT('Ctrl Pts',(7.10549818530004,12.2,7.9062707789495));
#210217=CARTESIAN_POINT('Ctrl Pts',(7.10249178837982,12.2,7.90419652754905));
#210218=CARTESIAN_POINT('Ctrl Pts',(7.09951299156243,12.2,7.90213161897303));
#210219=CARTESIAN_POINT('Ctrl Pts',(7.09653419474505,12.2,7.90006671039701));
#210220=CARTESIAN_POINT('Ctrl Pts',(7.09358299699269,12.2,7.89801114594546));
#210221=CARTESIAN_POINT('Ctrl Pts',(7.0906595111579,12.2,7.89596527587549));
#210222=CARTESIAN_POINT('Ctrl Pts',(7.08773602532311,12.2,7.89391940580553));
#210223=CARTESIAN_POINT('Ctrl Pts',(7.08484025172794,12.2,7.89188323109972));
#210224=CARTESIAN_POINT('Ctrl Pts',(7.08197230492094,12.2,7.8898571085992));
#210225=CARTESIAN_POINT('Ctrl Pts',(7.07910435811394,12.2,7.88783098609868));
#210226=CARTESIAN_POINT('Ctrl Pts',(7.0762642354865,12.2,7.8858149176491));
#210227=CARTESIAN_POINT('Ctrl Pts',(7.07345205450141,12.2,7.88380926500105));
#210228=CARTESIAN_POINT('Ctrl Pts',(7.0700774374419,12.2,7.88140248191085));
#210229=CARTESIAN_POINT('Ctrl Pts',(7.06674305432533,12.2,7.87901069728202));
#210230=CARTESIAN_POINT('Ctrl Pts',(7.06344910610892,12.2,7.87663455345063));
#210231=CARTESIAN_POINT('Ctrl Pts',(7.06070414916219,12.2,7.87465443351919));
#210232=CARTESIAN_POINT('Ctrl Pts',(7.05798726968171,12.2,7.87268517585367));
#210233=CARTESIAN_POINT('Ctrl Pts',(7.05529858683709,12.2,7.87072715672729));
#210234=CARTESIAN_POINT('Ctrl Pts',(7.0520721672477,12.2,7.86837753364757));
#210235=CARTESIAN_POINT('Ctrl Pts',(7.04888634615096,12.2,7.86604409633942));
#210236=CARTESIAN_POINT('Ctrl Pts',(7.04574132989866,12.2,7.86372750921406));
#210237=CARTESIAN_POINT('Ctrl Pts',(7.04259631393203,12.2,7.86141092229912));
#210238=CARTESIAN_POINT('Ctrl Pts',(7.03949210049268,12.2,7.85911118625966));
#210239=CARTESIAN_POINT('Ctrl Pts',(7.03642889350682,12.2,7.85682898149892));
#210240=CARTESIAN_POINT('Ctrl Pts',(7.03336568652096,12.2,7.85454677673819));
#210241=CARTESIAN_POINT('Ctrl Pts',(7.030343486381,12.2,7.8522821026083));
#210242=CARTESIAN_POINT('Ctrl Pts',(7.02736249840418,12.2,7.8500356568558));
#210243=CARTESIAN_POINT('Ctrl Pts',(7.02438151015659,12.2,7.84778921089926));
#210244=CARTESIAN_POINT('Ctrl Pts',(7.02144173382242,12.2,7.84556099131991));
#210245=CARTESIAN_POINT('Ctrl Pts',(7.0185433766673,12.2,7.84335171145081));
#210246=CARTESIAN_POINT('Ctrl Pts',(7.01564501977544,12.2,7.84114243178239));
#210247=CARTESIAN_POINT('Ctrl Pts',(7.0127880823342,12.2,7.8389520900187));
#210248=CARTESIAN_POINT('Ctrl Pts',(7.00997277335495,12.2,7.8367814145984));
#210249=CARTESIAN_POINT('Ctrl Pts',(7.00715746437569,12.2,7.83461073917812));
#210250=CARTESIAN_POINT('Ctrl Pts',(7.00438378362651,12.2,7.83245973096464));
#210251=CARTESIAN_POINT('Ctrl Pts',(7.0016519426406,12.2,7.83032913262448));
#210252=CARTESIAN_POINT('Ctrl Pts',(6.99892010165468,12.2,7.82819853428435));
#210253=CARTESIAN_POINT('Ctrl Pts',(6.99623009952015,12.2,7.82608834790319));
#210254=CARTESIAN_POINT('Ctrl Pts',(6.99358215153017,12.2,7.82399933447765));
#210255=CARTESIAN_POINT('Ctrl Pts',(6.99093420329967,12.2,7.82191032086237));
#210256=CARTESIAN_POINT('Ctrl Pts',(6.98832830629821,12.2,7.8198424802241));
#210257=CARTESIAN_POINT('Ctrl Pts',(6.98576467732702,12.2,7.81779659186356));
#210258=CARTESIAN_POINT('Ctrl Pts',(6.98320104858868,12.2,7.81575070368886));
#210259=CARTESIAN_POINT('Ctrl Pts',(6.98067968938863,12.2,7.81372677060407));
#210260=CARTESIAN_POINT('Ctrl Pts',(6.97820081539348,12.2,7.81172558934244));
#210261=CARTESIAN_POINT('Ctrl Pts',(6.97572194139835,12.2,7.80972440808081));
#210262=CARTESIAN_POINT('Ctrl Pts',(6.97328555258509,12.2,7.80774597872696));
#210263=CARTESIAN_POINT('Ctrl Pts',(6.97089186975247,12.2,7.80579112346304));
#210264=CARTESIAN_POINT('Ctrl Pts',(6.96849818670243,12.2,7.80383626802155));
#210265=CARTESIAN_POINT('Ctrl Pts',(6.96614721079818,12.2,7.80190498224898));
#210266=CARTESIAN_POINT('Ctrl Pts',(6.96383916184092,12.2,7.79999810914611));
#210267=CARTESIAN_POINT('Ctrl Pts',(6.96153111309331,12.2,7.79809123621645));
#210268=CARTESIAN_POINT('Ctrl Pts',(6.95926599407201,12.2,7.7962087743418));
#210269=CARTESIAN_POINT('Ctrl Pts',(6.95704402822588,12.2,7.79435158723412));
#210270=CARTESIAN_POINT('Ctrl Pts',(6.95482206237975,12.2,7.79249440012643));
#210271=CARTESIAN_POINT('Ctrl Pts',(6.95264324974966,12.2,7.79066248473294));
#210272=CARTESIAN_POINT('Ctrl Pts',(6.95050782074098,12.2,7.78885672596344));
#210273=CARTESIAN_POINT('Ctrl Pts',(6.94837239153831,12.2,7.78705096702992));
#210274=CARTESIAN_POINT('Ctrl Pts',(6.94628034338827,12.2,7.78527136550364));
#210275=CARTESIAN_POINT('Ctrl Pts',(6.94423190826015,12.2,7.78351882657214));
#210276=CARTESIAN_POINT('Ctrl Pts',(6.9421834733181,12.2,7.78176628779983));
#210277=CARTESIAN_POINT('Ctrl Pts',(6.94017865297863,12.2,7.78004081407993));
#210278=CARTESIAN_POINT('Ctrl Pts',(6.93821767921653,12.2,7.77834333372493));
#210279=CARTESIAN_POINT('Ctrl Pts',(6.93625670545443,12.2,7.77664585336993));
#210280=CARTESIAN_POINT('Ctrl Pts',(6.93433957997591,12.2,7.77497636927441));
#210281=CARTESIAN_POINT('Ctrl Pts',(6.93246653994784,12.2,7.77333583766704));
#210282=CARTESIAN_POINT('Ctrl Pts',(6.93059349974963,12.2,7.77169530591067));
#210283=CARTESIAN_POINT('Ctrl Pts',(6.92876454473291,12.2,7.77008372582003));
#210284=CARTESIAN_POINT('Ctrl Pts',(6.92697991580536,12.2,7.76850208231921));
#210285=CARTESIAN_POINT('Ctrl Pts',(6.92519528703991,12.2,7.76692043896207));
#210286=CARTESIAN_POINT('Ctrl Pts',(6.92345498657842,12.2,7.76536873156749));
#210287=CARTESIAN_POINT('Ctrl Pts',(6.92175925679911,12.2,7.76384797328258));
#210288=CARTESIAN_POINT('Ctrl Pts',(6.9200635270198,12.2,7.76232721499769));
#210289=CARTESIAN_POINT('Ctrl Pts',(6.91841236845617,12.2,7.76083740255294));
#210290=CARTESIAN_POINT('Ctrl Pts',(6.91680603159594,12.2,7.75937958152118));
#210291=CARTESIAN_POINT('Ctrl Pts',(6.91519969458979,12.2,7.75792176035702));
#210292=CARTESIAN_POINT('Ctrl Pts',(6.91363817867246,12.2,7.75649592919676));
#210293=CARTESIAN_POINT('Ctrl Pts',(6.91212173584292,12.2,7.75510315837313));
#210294=CARTESIAN_POINT('Ctrl Pts',(6.91060529315112,12.2,7.75371038767601));
#210295=CARTESIAN_POINT('Ctrl Pts',(6.90913392473523,12.2,7.75235068106152));
#210296=CARTESIAN_POINT('Ctrl Pts',(6.90770788712233,12.2,7.75102513844449));
#210297=CARTESIAN_POINT('Ctrl Pts',(6.90581334753501,12.2,7.74926410988541));
#210298=CARTESIAN_POINT('Ctrl Pts',(6.90399882477399,12.2,7.74756337736256));
#210299=CARTESIAN_POINT('Ctrl Pts',(6.90226491999994,12.2,7.74592563799998));
#210300=CARTESIAN_POINT('Ctrl Pts',(6.90226491999994,15.2,7.74592563799998));
#210301=CARTESIAN_POINT('Ctrl Pts',(6.90356378263743,15.2,7.74715246342883));
#210302=CARTESIAN_POINT('Ctrl Pts',(6.90490788344662,15.2,7.74841464105156));
#210303=CARTESIAN_POINT('Ctrl Pts',(6.90629697055607,15.2,7.74971102712461));
#210304=CARTESIAN_POINT('Ctrl Pts',(6.90769275654571,15.2,7.75101366502659));
#210305=CARTESIAN_POINT('Ctrl Pts',(6.90913396266922,15.2,7.75235084439584));
#210306=CARTESIAN_POINT('Ctrl Pts',(6.91062032766044,15.2,7.7537214504576));
#210307=CARTESIAN_POINT('Ctrl Pts',(6.91210669251663,15.2,7.75509205639487));
#210308=CARTESIAN_POINT('Ctrl Pts',(6.91363821531548,15.2,7.75649608787712));
#210309=CARTESIAN_POINT('Ctrl Pts',(6.9152146440082,15.2,7.75793246374159));
#210310=CARTESIAN_POINT('Ctrl Pts',(6.91679107270092,15.2,7.75936883960606));
#210311=CARTESIAN_POINT('Ctrl Pts',(6.91841240633538,15.2,7.76083755757795));
#210312=CARTESIAN_POINT('Ctrl Pts',(6.92007839335548,15.2,7.76233756884657));
#210313=CARTESIAN_POINT('Ctrl Pts',(6.92174438052691,15.2,7.76383758025143));
#210314=CARTESIAN_POINT('Ctrl Pts',(6.92345502357584,15.2,7.76536888328299));
#210315=CARTESIAN_POINT('Ctrl Pts',(6.92521007267451,15.2,7.76693045587015));
#210316=CARTESIAN_POINT('Ctrl Pts',(6.92696512161377,15.2,7.76849202831548));
#210317=CARTESIAN_POINT('Ctrl Pts',(6.92876458061756,15.2,7.77008387331881));
#210318=CARTESIAN_POINT('Ctrl Pts',(6.93060820347571,15.2,7.77170499376734));
#210319=CARTESIAN_POINT('Ctrl Pts',(6.93245182633386,15.2,7.77332611421586));
#210320=CARTESIAN_POINT('Ctrl Pts',(6.93433961447518,15.2,7.77497651200411));
#210321=CARTESIAN_POINT('Ctrl Pts',(6.93627133015311,15.2,7.7766552214419));
#210322=CARTESIAN_POINT('Ctrl Pts',(6.93820304600649,15.2,7.77833393103218));
#210323=CARTESIAN_POINT('Ctrl Pts',(6.94017868713198,15.2,7.78004095115929));
#210324=CARTESIAN_POINT('Ctrl Pts',(6.94219802016165,15.2,7.78177534392233));
#210325=CARTESIAN_POINT('Ctrl Pts',(6.9442173530079,15.2,7.78350973652782));
#210326=CARTESIAN_POINT('Ctrl Pts',(6.94628037724782,15.2,7.78527149982797));
#210327=CARTESIAN_POINT('Ctrl Pts',(6.94838686008986,15.2,7.78705971959751));
#210328=CARTESIAN_POINT('Ctrl Pts',(6.95049334293191,15.2,7.78884793936704));
#210329=CARTESIAN_POINT('Ctrl Pts',(6.95264328337871,15.2,7.79066261469271));
#210330=CARTESIAN_POINT('Ctrl Pts',(6.95483645513052,15.2,7.79250285637475));
#210331=CARTESIAN_POINT('Ctrl Pts',(6.95702962688232,15.2,7.79434309805681));
#210332=CARTESIAN_POINT('Ctrl Pts',(6.95926602758718,15.2,7.79620890483925));
#210333=CARTESIAN_POINT('Ctrl Pts',(6.96154543150143,15.2,7.79809940601888));
#210334=CARTESIAN_POINT('Ctrl Pts',(6.96382483562273,15.2,7.79998990737024));
#210335=CARTESIAN_POINT('Ctrl Pts',(6.9661472434982,15.2,7.80190510779901));
#210336=CARTESIAN_POINT('Ctrl Pts',(6.96851243062895,15.2,7.80384415607239));
#210337=CARTESIAN_POINT('Ctrl Pts',(6.97127181529257,15.2,7.80610637879379));
#210338=CARTESIAN_POINT('Ctrl Pts',(6.97408942933038,15.2,7.80840106193489));
#210339=CARTESIAN_POINT('Ctrl Pts',(6.97696491948123,15.2,7.81072689831598));
#210340=CARTESIAN_POINT('Ctrl Pts',(6.97942962561266,15.2,7.81272047258974));
#210341=CARTESIAN_POINT('Ctrl Pts',(6.98193685458154,15.2,7.81473693384074));
#210342=CARTESIAN_POINT('Ctrl Pts',(6.984486386889,15.2,7.81677548136947));
#210343=CARTESIAN_POINT('Ctrl Pts',(6.98746084113191,15.2,7.81915378672707));
#210344=CARTESIAN_POINT('Ctrl Pts',(6.99049287871483,15.2,7.82156215202135));
#210345=CARTESIAN_POINT('Ctrl Pts',(6.99358215153017,15.2,7.82399933447766));
#210346=CARTESIAN_POINT('Ctrl Pts',(6.99623009952018,15.2,7.8260883479032));
#210347=CARTESIAN_POINT('Ctrl Pts',(6.99892010165468,15.2,7.82819853428434));
#210348=CARTESIAN_POINT('Ctrl Pts',(7.0016519426406,15.2,7.83032913262448));
#210349=CARTESIAN_POINT('Ctrl Pts',(7.00438378362652,15.2,7.83245973096464));
#210350=CARTESIAN_POINT('Ctrl Pts',(7.00715746437572,15.2,7.83461073917814));
#210351=CARTESIAN_POINT('Ctrl Pts',(7.00997277335495,15.2,7.8367814145984));
#210352=CARTESIAN_POINT('Ctrl Pts',(7.01278808233417,15.2,7.83895209001868));
#210353=CARTESIAN_POINT('Ctrl Pts',(7.01564501977542,15.2,7.84114243178237));
#210354=CARTESIAN_POINT('Ctrl Pts',(7.01854337666729,15.2,7.84335171145081));
#210355=CARTESIAN_POINT('Ctrl Pts',(7.02144173382244,15.2,7.84556099131992));
#210356=CARTESIAN_POINT('Ctrl Pts',(7.02438151015657,15.2,7.84778921089924));
#210357=CARTESIAN_POINT('Ctrl Pts',(7.02736249840418,15.2,7.8500356568558));
#210358=CARTESIAN_POINT('Ctrl Pts',(7.03034348638102,15.2,7.85228210260832));
#210359=CARTESIAN_POINT('Ctrl Pts',(7.03336568652096,15.2,7.85454677673819));
#210360=CARTESIAN_POINT('Ctrl Pts',(7.03642889350682,15.2,7.85682898149892));
#210361=CARTESIAN_POINT('Ctrl Pts',(7.03949210049268,15.2,7.85911118625966));
#210362=CARTESIAN_POINT('Ctrl Pts',(7.04259631393244,15.2,7.86141092229942));
#210363=CARTESIAN_POINT('Ctrl Pts',(7.04574132989874,15.2,7.86372750921412));
#210364=CARTESIAN_POINT('Ctrl Pts',(7.04888634615073,15.2,7.86604409633925));
#210365=CARTESIAN_POINT('Ctrl Pts',(7.05207216724769,15.2,7.86837753364757));
#210366=CARTESIAN_POINT('Ctrl Pts',(7.05529858683709,15.2,7.87072715672729));
#210367=CARTESIAN_POINT('Ctrl Pts',(7.05798726968171,15.2,7.87268517585368));
#210368=CARTESIAN_POINT('Ctrl Pts',(7.0607041491622,15.2,7.87465443351919));
#210369=CARTESIAN_POINT('Ctrl Pts',(7.06344910610893,15.2,7.87663455345063));
#210370=CARTESIAN_POINT('Ctrl Pts',(7.06619406305566,15.2,7.87861467338206));
#210371=CARTESIAN_POINT('Ctrl Pts',(7.06896710005286,15.2,7.88060565486091));
#210372=CARTESIAN_POINT('Ctrl Pts',(7.07176810012459,15.2,7.88260712652842));
#210373=CARTESIAN_POINT('Ctrl Pts',(7.07456909989099,15.2,7.88460859797777));
#210374=CARTESIAN_POINT('Ctrl Pts',(7.077398064901,15.2,7.88662055850115));
#210375=CARTESIAN_POINT('Ctrl Pts',(7.08025487639288,15.2,7.88864264425214));
#210376=CARTESIAN_POINT('Ctrl Pts',(7.08311168819617,15.2,7.89066473022354));
#210377=CARTESIAN_POINT('Ctrl Pts',(7.08599634966565,15.2,7.89269694209479));
#210378=CARTESIAN_POINT('Ctrl Pts',(7.08890874563561,15.2,7.89473891973287));
#210379=CARTESIAN_POINT('Ctrl Pts',(7.09182114160556,15.2,7.89678089737096));
#210380=CARTESIAN_POINT('Ctrl Pts',(7.09476127381467,15.2,7.89883264054175));
#210381=CARTESIAN_POINT('Ctrl Pts',(7.09772902590546,15.2,7.90089379751906));
#210382=CARTESIAN_POINT('Ctrl Pts',(7.10069677799626,15.2,7.90295495449638));
#210383=CARTESIAN_POINT('Ctrl Pts',(7.10369215273713,15.2,7.90502552475338));
#210384=CARTESIAN_POINT('Ctrl Pts',(7.10671503606901,15.2,7.90710516086401));
#210385=CARTESIAN_POINT('Ctrl Pts',(7.11034249626498,15.2,7.90960072433278));
#210386=CARTESIAN_POINT('Ctrl Pts',(7.11400956662419,15.2,7.91210934346984));
#210387=CARTESIAN_POINT('Ctrl Pts',(7.11771605791223,15.2,7.91463042877477));
#210388=CARTESIAN_POINT('Ctrl Pts',(7.12080480014725,15.2,7.91673133285204));
#210389=CARTESIAN_POINT('Ctrl Pts',(7.12392091704472,15.2,7.91884089456004));
#210390=CARTESIAN_POINT('Ctrl Pts',(7.1270642960054,15.2,7.92095877877295));
#210391=CARTESIAN_POINT('Ctrl Pts',(7.13020767530871,15.2,7.9230766632167));
#210392=CARTESIAN_POINT('Ctrl Pts',(7.13337831780605,15.2,7.92520287012702));
#210393=CARTESIAN_POINT('Ctrl Pts',(7.13657611203995,15.2,7.92733707123748));
#210394=CARTESIAN_POINT('Ctrl Pts',(7.13977390627383,15.2,7.92947127234794));
#210395=CARTESIAN_POINT('Ctrl Pts',(7.14299885188965,15.2,7.93161346622134));
#210396=CARTESIAN_POINT('Ctrl Pts',(7.14625083968913,15.2,7.93376333000876));
#210397=CARTESIAN_POINT('Ctrl Pts',(7.1495028274886,15.2,7.93591319379618));
#210398=CARTESIAN_POINT('Ctrl Pts',(7.15278185687412,15.2,7.93807072741992));
#210399=CARTESIAN_POINT('Ctrl Pts',(7.1560878177755,15.2,7.9402356111001));
#210400=CARTESIAN_POINT('Ctrl Pts',(7.15939377867686,15.2,7.94240049478027));
#210401=CARTESIAN_POINT('Ctrl Pts',(7.1627266709706,15.2,7.94457273013562));
#210402=CARTESIAN_POINT('Ctrl Pts',(7.16608638603865,15.2,7.94675200131582));
#210403=CARTESIAN_POINT('Ctrl Pts',(7.16944610110669,15.2,7.94893127249602));
#210404=CARTESIAN_POINT('Ctrl Pts',(7.17283263833933,15.2,7.95111758065138));
#210405=CARTESIAN_POINT('Ctrl Pts',(7.17624588931015,15.2,7.95331061537325));
#210406=CARTESIAN_POINT('Ctrl Pts',(7.17965914028097,15.2,7.95550365009513));
#210407=CARTESIAN_POINT('Ctrl Pts',(7.183099104249,15.2,7.95770341323877));
#210408=CARTESIAN_POINT('Ctrl Pts',(7.18656567426466,15.2,7.95990959949877));
#210409=CARTESIAN_POINT('Ctrl Pts',(7.19003224428033,15.2,7.96211578575877));
#210410=CARTESIAN_POINT('Ctrl Pts',(7.19352541896098,15.2,7.9643283955833));
#210411=CARTESIAN_POINT('Ctrl Pts',(7.19704509076654,15.2,7.96654712704164));
#210412=CARTESIAN_POINT('Ctrl Pts',(7.19986082836445,15.2,7.96832211230504));
#210413=CARTESIAN_POINT('Ctrl Pts',(7.2026935248782,15.2,7.97010101798279));
#210414=CARTESIAN_POINT('Ctrl Pts',(7.20554312375746,15.2,7.97188369052478));
#210415=CARTESIAN_POINT('Ctrl Pts',(7.20839272224847,15.2,7.97366636282387));
#210416=CARTESIAN_POINT('Ctrl Pts',(7.21125922322337,15.2,7.9754528025453));
#210417=CARTESIAN_POINT('Ctrl Pts',(7.21414257372292,15.2,7.97724286024042));
#210418=CARTESIAN_POINT('Ctrl Pts',(7.21702592461532,15.2,7.97903291817944));
#210419=CARTESIAN_POINT('Ctrl Pts',(7.21992612347168,15.2,7.98082659384829));
#210420=CARTESIAN_POINT('Ctrl Pts',(7.22284311574349,15.2,7.98262374033548));
#210421=CARTESIAN_POINT('Ctrl Pts',(7.22576010761785,15.2,7.9844208865778));
#210422=CARTESIAN_POINT('Ctrl Pts',(7.22869389275389,15.2,7.98622150267522));
#210423=CARTESIAN_POINT('Ctrl Pts',(7.23164441723383,15.2,7.98802544236086));
#210424=CARTESIAN_POINT('Ctrl Pts',(7.23459494211577,15.2,7.9898293822923));
#210425=CARTESIAN_POINT('Ctrl Pts',(7.23756220640593,15.2,7.99163664735943));
#210426=CARTESIAN_POINT('Ctrl Pts',(7.2405461554413,15.2,7.99344709027103));
#210427=CARTESIAN_POINT('Ctrl Pts',(7.24427609153222,15.2,7.99571014378721));
#210428=CARTESIAN_POINT('Ctrl Pts',(7.24803209579799,15.2,7.99797816725241));
#210429=CARTESIAN_POINT('Ctrl Pts',(7.25181406503624,15.2,8.00025087878058));
#210430=CARTESIAN_POINT('Ctrl Pts',(7.2548396401795,15.2,8.00206904785448));
#210431=CARTESIAN_POINT('Ctrl Pts',(7.25788183197334,15.2,8.00389021819185));
#210432=CARTESIAN_POINT('Ctrl Pts',(7.26094058649998,15.2,8.00571424987588));
#210433=CARTESIAN_POINT('Ctrl Pts',(7.26399934144337,15.2,8.00753828180843));
#210434=CARTESIAN_POINT('Ctrl Pts',(7.26707465909644,15.2,8.00936517352968));
#210435=CARTESIAN_POINT('Ctrl Pts',(7.27016648619862,15.2,8.01119478749881));
#210436=CARTESIAN_POINT('Ctrl Pts',(7.2740312698657,15.2,8.01348180483557));
#210437=CARTESIAN_POINT('Ctrl Pts',(7.27792184776561,15.2,8.01577307310544));
#210438=CARTESIAN_POINT('Ctrl Pts',(7.2818381170038,15.2,8.0180683263002));
#210439=CARTESIAN_POINT('Ctrl Pts',(7.28497113213824,15.2,8.01990452870589));
#210440=CARTESIAN_POINT('Ctrl Pts',(7.28812058870667,15.2,8.02174328086405));
#210441=CARTESIAN_POINT('Ctrl Pts',(7.29128643322456,15.2,8.02358444732448));
#210442=CARTESIAN_POINT('Ctrl Pts',(7.2944522781738,15.2,8.02542561403577));
#210443=CARTESIAN_POINT('Ctrl Pts',(7.29763451133135,15.2,8.02726919383593));
#210444=CARTESIAN_POINT('Ctrl Pts',(7.30083307972244,15.2,8.02911505525117));
#210445=CARTESIAN_POINT('Ctrl Pts',(7.30403164767773,15.2,8.03096091641491));
#210446=CARTESIAN_POINT('Ctrl Pts',(7.30724654915665,15.2,8.03280905748347));
#210447=CARTESIAN_POINT('Ctrl Pts',(7.31047773300255,15.2,8.03465934533207));
#210448=CARTESIAN_POINT('Ctrl Pts',(7.3137089172887,15.2,8.03650963343278));
#210449=CARTESIAN_POINT('Ctrl Pts',(7.31695638384625,15.2,8.03836206872818));
#210450=CARTESIAN_POINT('Ctrl Pts',(7.32022007752517,15.2,8.04021652138493));
#210451=CARTESIAN_POINT('Ctrl Pts',(7.32511561759888,15.2,8.04299820011739));
#210452=CARTESIAN_POINT('Ctrl Pts',(7.33004767192233,15.2,8.04578441368743));
#210453=CARTESIAN_POINT('Ctrl Pts',(7.33501606176429,15.2,8.04857472676538));
#210454=CARTESIAN_POINT('Ctrl Pts',(7.3383283219598,15.2,8.05043493565298));
#210455=CARTESIAN_POINT('Ctrl Pts',(7.34165672980724,15.2,8.05229696780573));
#210456=CARTESIAN_POINT('Ctrl Pts',(7.34500123354672,15.2,8.05416069329637));
#210457=CARTESIAN_POINT('Ctrl Pts',(7.34918186299321,15.2,8.05649035003269));
#210458=CARTESIAN_POINT('Ctrl Pts',(7.35338764442345,15.2,8.0588226551385));
#210459=CARTESIAN_POINT('Ctrl Pts',(7.35761847053662,15.2,8.06115736097203));
#210460=CARTESIAN_POINT('Ctrl Pts',(7.36100313115045,15.2,8.06302512548616));
#210461=CARTESIAN_POINT('Ctrl Pts',(7.36440382396975,15.2,8.06489442679592));
#210462=CARTESIAN_POINT('Ctrl Pts',(7.36782049253922,15.2,8.06676514070704));
#210463=CARTESIAN_POINT('Ctrl Pts',(7.37209132860021,15.2,8.06910353328709));
#210464=CARTESIAN_POINT('Ctrl Pts',(7.37638713024987,15.2,8.07144413099999));
#210465=CARTESIAN_POINT('Ctrl Pts',(7.38070779295821,15.2,8.07378669599998));
#210466=CARTESIAN_POINT('Ctrl Pts',(7.38416432331326,15.2,8.07566074810212));
#210467=CARTESIAN_POINT('Ctrl Pts',(7.38763676491183,15.2,8.07753605782662));
#210468=CARTESIAN_POINT('Ctrl Pts',(7.39112506777023,15.2,8.07941250404011));
#210469=CARTESIAN_POINT('Ctrl Pts',(7.39461337015335,15.2,8.08128894999794));
#210470=CARTESIAN_POINT('Ctrl Pts',(7.39811753065544,15.2,8.08316653394931));
#210471=CARTESIAN_POINT('Ctrl Pts',(7.40163749977249,15.2,8.0850451332487));
#210472=CARTESIAN_POINT('Ctrl Pts',(7.40515746936914,15.2,8.08692373280405));
#210473=CARTESIAN_POINT('Ctrl Pts',(7.40869324495761,15.2,8.0888033480632));
#210474=CARTESIAN_POINT('Ctrl Pts',(7.41224477659724,15.2,8.09068386033245));
#210475=CARTESIAN_POINT('Ctrl Pts',(7.41845995624073,15.2,8.09397475641931));
#210476=CARTESIAN_POINT('Ctrl Pts',(7.42472338657279,15.2,8.0972683997419));
#210477=CARTESIAN_POINT('Ctrl Pts',(7.43103478713523,15.2,8.10056415946707));
#210478=CARTESIAN_POINT('Ctrl Pts',(7.43464130216352,15.2,8.10244745095854));
#210479=CARTESIAN_POINT('Ctrl Pts',(7.43826348147363,15.2,8.10433143449833));
#210480=CARTESIAN_POINT('Ctrl Pts',(7.44190127374403,15.2,8.10621599277627));
#210481=CARTESIAN_POINT('Ctrl Pts',(7.44553906551878,15.2,8.10810055079744));
#210482=CARTESIAN_POINT('Ctrl Pts',(7.44919246907098,15.2,8.10998568487366));
#210483=CARTESIAN_POINT('Ctrl Pts',(7.45286143415835,15.2,8.11187127894169));
#210484=CARTESIAN_POINT('Ctrl Pts',(7.45653039974561,15.2,8.11375687326663));
#210485=CARTESIAN_POINT('Ctrl Pts',(7.4602149251899,15.2,8.1156429294083));
#210486=CARTESIAN_POINT('Ctrl Pts',(7.46391495955821,15.2,8.11752933173332));
#210487=CARTESIAN_POINT('Ctrl Pts',(7.46761499392653,15.2,8.11941573405834));
#210488=CARTESIAN_POINT('Ctrl Pts',(7.47133053725778,15.2,8.1213024847612));
#210489=CARTESIAN_POINT('Ctrl Pts',(7.47506153885158,15.2,8.12318947030851));
#210490=CARTESIAN_POINT('Ctrl Pts',(7.47879253993703,15.2,8.12507645559871));
#210491=CARTESIAN_POINT('Ctrl Pts',(7.48253899765449,15.2,8.12696367438608));
#210492=CARTESIAN_POINT('Ctrl Pts',(7.48630086203066,15.2,8.12885101774037));
#210493=CARTESIAN_POINT('Ctrl Pts',(7.49006272691937,15.2,8.1307383613518));
#210494=CARTESIAN_POINT('Ctrl Pts',(7.49383999707006,15.2,8.13262582863072));
#210495=CARTESIAN_POINT('Ctrl Pts',(7.49763262211165,15.2,8.13451330956692));
#210496=CARTESIAN_POINT('Ctrl Pts',(7.50142524663651,15.2,8.13640079024596));
#210497=CARTESIAN_POINT('Ctrl Pts',(7.50523322634269,15.2,8.13828828401109));
#210498=CARTESIAN_POINT('Ctrl Pts',(7.50905650886248,15.2,8.14017568207903));
#210499=CARTESIAN_POINT('Ctrl Pts',(7.51287979190317,15.2,8.14206308040412));
#210500=CARTESIAN_POINT('Ctrl Pts',(7.51671837775807,15.2,8.14395038339893));
#210501=CARTESIAN_POINT('Ctrl Pts',(7.52057221755085,15.2,8.14583748304048));
#210502=CARTESIAN_POINT('Ctrl Pts',(7.52442605681854,15.2,8.14772458242492));
#210503=CARTESIAN_POINT('Ctrl Pts',(7.52829514618711,15.2,8.14961147781384));
#210504=CARTESIAN_POINT('Ctrl Pts',(7.53217943792415,15.2,8.15149806260409));
#210505=CARTESIAN_POINT('Ctrl Pts',(7.53703480299238,15.2,8.15385629378468));
#210506=CARTESIAN_POINT('Ctrl Pts',(7.54191391844172,15.2,8.15621403873468));
#210507=CARTESIAN_POINT('Ctrl Pts',(7.54681668691272,15.2,8.15857109234583));
#210508=CARTESIAN_POINT('Ctrl Pts',(7.55270000886414,15.2,8.16139955657645));
#210509=CARTESIAN_POINT('Ctrl Pts',(7.55861739121975,15.2,8.1642270242862));
#210510=CARTESIAN_POINT('Ctrl Pts',(7.56456865833454,15.2,8.16705314343361));
#210511=CARTESIAN_POINT('Ctrl Pts',(7.56952804777705,15.2,8.16940824280868));
#210512=CARTESIAN_POINT('Ctrl Pts',(7.57451097031365,15.2,8.17176240398658));
#210513=CARTESIAN_POINT('Ctrl Pts',(7.57951732635339,15.2,8.17411542766721));
#210514=CARTESIAN_POINT('Ctrl Pts',(7.58352241140346,15.2,8.17599784671432));
#210515=CARTESIAN_POINT('Ctrl Pts',(7.58754249534214,15.2,8.17787953823468));
#210516=CARTESIAN_POINT('Ctrl Pts',(7.5915775244693,15.2,8.1797603992346));
#210517=CARTESIAN_POINT('Ctrl Pts',(7.59460379603979,15.2,8.18117104485641));
#210518=CARTESIAN_POINT('Ctrl Pts',(7.59763847602724,15.2,8.18258122312686));
#210519=CARTESIAN_POINT('Ctrl Pts',(7.60068154151379,15.2,8.18399089179038));
#210520=CARTESIAN_POINT('Ctrl Pts',(7.60372460700035,15.2,8.1854005604539));
#210521=CARTESIAN_POINT('Ctrl Pts',(7.60677605856173,15.2,8.18680971964756));
#210522=CARTESIAN_POINT('Ctrl Pts',(7.60983587544984,15.2,8.18821832684644));
#210523=CARTESIAN_POINT('Ctrl Pts',(7.61289569233794,15.2,8.18962693404532));
#210524=CARTESIAN_POINT('Ctrl Pts',(7.61596387265879,15.2,8.19103498917755));
#210525=CARTESIAN_POINT('Ctrl Pts',(7.61904039762921,15.2,8.19244244991816));
#210526=CARTESIAN_POINT('Ctrl Pts',(7.62211692315853,15.2,8.19384991091447));
#210527=CARTESIAN_POINT('Ctrl Pts',(7.62520179255686,15.2,8.19525677830226));
#210528=CARTESIAN_POINT('Ctrl Pts',(7.62829498367421,15.2,8.19666300975655));
#210529=CARTESIAN_POINT('Ctrl Pts',(7.63345030089196,15.2,8.19900672825094));
#210530=CARTESIAN_POINT('Ctrl Pts',(7.63862873644949,15.2,8.20134867962105));
#210531=CARTESIAN_POINT('Ctrl Pts',(7.64383018956121,15.2,8.20368867464392));
#210532=CARTESIAN_POINT('Ctrl Pts',(7.64799135273094,15.2,8.20556067096829));
#210533=CARTESIAN_POINT('Ctrl Pts',(7.65216724861038,15.2,8.20743141318144));
#210534=CARTESIAN_POINT('Ctrl Pts',(7.65635782628322,15.2,8.20930080628332));
#210535=CARTESIAN_POINT('Ctrl Pts',(7.65950075925237,15.2,8.21070285098238));
#210536=CARTESIAN_POINT('Ctrl Pts',(7.66265195108782,15.2,8.21210413679813));
#210537=CARTESIAN_POINT('Ctrl Pts',(7.66581137963899,15.2,8.21350462158066));
#210538=CARTESIAN_POINT('Ctrl Pts',(7.67002395142318,15.2,8.21537193479364));
#210539=CARTESIAN_POINT('Ctrl Pts',(7.67425116663779,15.2,8.21723782594256));
#210540=CARTESIAN_POINT('Ctrl Pts',(7.67849297708215,15.2,8.21910219980385));
#210541=CARTESIAN_POINT('Ctrl Pts',(7.68273478694857,15.2,8.22096657341112));
#210542=CARTESIAN_POINT('Ctrl Pts',(7.68699118905654,15.2,8.2228294300832));
#210543=CARTESIAN_POINT('Ctrl Pts',(7.69126213615087,15.2,8.22469067359782));
#210544=CARTESIAN_POINT('Ctrl Pts',(7.6944653466171,15.2,8.22608660629717));
#210545=CARTESIAN_POINT('Ctrl Pts',(7.69767673809946,15.2,8.22748163149661));
#210546=CARTESIAN_POINT('Ctrl Pts',(7.7008962890647,15.2,8.22887571073775));
#210547=CARTESIAN_POINT('Ctrl Pts',(7.70411584061482,15.2,8.23026979023215));
#210548=CARTESIAN_POINT('Ctrl Pts',(7.7073435517006,15.2,8.23166292400129));
#210549=CARTESIAN_POINT('Ctrl Pts',(7.71057940175531,15.2,8.23305507103681));
#210550=CARTESIAN_POINT('Ctrl Pts',(7.71381525122218,15.2,8.23444721781943));
#210551=CARTESIAN_POINT('Ctrl Pts',(7.71705923895058,15.2,8.23583837846679));
#210552=CARTESIAN_POINT('Ctrl Pts',(7.72031134462084,15.2,8.23722851473561));
#210553=CARTESIAN_POINT('Ctrl Pts',(7.72573152093486,15.2,8.23954540860116));
#210554=CARTESIAN_POINT('Ctrl Pts',(7.73117424467958,15.2,8.24185945493586));
#210555=CARTESIAN_POINT('Ctrl Pts',(7.73663942072308,15.2,8.24417047535227));
#210556=CARTESIAN_POINT('Ctrl Pts',(7.73991852623003,15.2,8.24555708755174));
#210557=CARTESIAN_POINT('Ctrl Pts',(7.74320571439489,15.2,8.24694260940127));
#210558=CARTESIAN_POINT('Ctrl Pts',(7.74650096385921,15.2,8.24832700460087));
#210559=CARTESIAN_POINT('Ctrl Pts',(7.74979621332352,15.2,8.24971139980047));
#210560=CARTESIAN_POINT('Ctrl Pts',(7.75309952323687,15.2,8.25109466731688));
#210561=CARTESIAN_POINT('Ctrl Pts',(7.75641087424155,15.2,8.25247676851666));
#210562=CARTESIAN_POINT('Ctrl Pts',(7.75972222524624,15.2,8.25385886971644));
#210563=CARTESIAN_POINT('Ctrl Pts',(7.76304161755893,15.2,8.25523980386629));
#210564=CARTESIAN_POINT('Ctrl Pts',(7.76636902814567,15.2,8.25661953556625));
#210565=CARTESIAN_POINT('Ctrl Pts',(7.76969643873239,15.2,8.25799926726622));
#210566=CARTESIAN_POINT('Ctrl Pts',(7.77303186940848,15.2,8.25937779563126));
#210567=CARTESIAN_POINT('Ctrl Pts',(7.7763752985781,15.2,8.26075508152518));
#210568=CARTESIAN_POINT('Ctrl Pts',(7.77971872774771,15.2,8.26213236741908));
#210569=CARTESIAN_POINT('Ctrl Pts',(7.78307015524069,15.2,8.26350841260007));
#210570=CARTESIAN_POINT('Ctrl Pts',(7.78642955978421,15.2,8.26488317846696));
#210571=CARTESIAN_POINT('Ctrl Pts',(7.79202856756017,15.2,8.26717445499503));
#210572=CARTESIAN_POINT('Ctrl Pts',(7.79764973525801,15.2,8.26946218059539));
#210573=CARTESIAN_POINT('Ctrl Pts',(7.80329296622843,15.2,8.27174618198458));
#210574=CARTESIAN_POINT('Ctrl Pts',(7.80667890530277,15.2,8.27311658301726));
#210575=CARTESIAN_POINT('Ctrl Pts',(7.8100727864627,15.2,8.27448564326624));
#210576=CARTESIAN_POINT('Ctrl Pts',(7.81347458999982,15.2,8.27585332679815));
#210577=CARTESIAN_POINT('Ctrl Pts',(7.81801032701934,15.2,8.27767690442659));
#210578=CARTESIAN_POINT('Ctrl Pts',(7.82256014663809,15.2,8.27949803396138));
#210579=CARTESIAN_POINT('Ctrl Pts',(7.82712399973012,15.2,8.28131662826542));
#210580=CARTESIAN_POINT('Ctrl Pts',(7.83054688970459,15.2,8.2826805740554));
#210581=CARTESIAN_POINT('Ctrl Pts',(7.83397767315083,15.2,8.28404309425095));
#210582=CARTESIAN_POINT('Ctrl Pts',(7.83741632965021,15.2,8.28540415211828));
#210583=CARTESIAN_POINT('Ctrl Pts',(7.84200120539916,15.2,8.28721889610623));
#210584=CARTESIAN_POINT('Ctrl Pts',(7.84660007774703,15.2,8.28903104099945));
#210585=CARTESIAN_POINT('Ctrl Pts',(7.85121289811045,15.2,8.2908405040979));
#210586=CARTESIAN_POINT('Ctrl Pts',(7.85467251306877,15.2,8.29219760129846));
#210587=CARTESIAN_POINT('Ctrl Pts',(7.85813997353016,15.2,8.29355318896095));
#210588=CARTESIAN_POINT('Ctrl Pts',(7.86161525800305,15.2,8.29490723070956));
#210589=CARTESIAN_POINT('Ctrl Pts',(7.86509054247594,15.2,8.29626127245817));
#210590=CARTESIAN_POINT('Ctrl Pts',(7.86857365102441,15.2,8.29761376882504));
#210591=CARTESIAN_POINT('Ctrl Pts',(7.87206456249672,15.2,8.2989646830321));
#210592=CARTESIAN_POINT('Ctrl Pts',(7.87555547396903,15.2,8.30031559723915));
#210593=CARTESIAN_POINT('Ctrl Pts',(7.87905418756256,15.2,8.30166492785189));
#210594=CARTESIAN_POINT('Ctrl Pts',(7.88256068510115,15.2,8.3030126456364));
#210595=CARTESIAN_POINT('Ctrl Pts',(7.88606718263973,15.2,8.30436036342091));
#210596=CARTESIAN_POINT('Ctrl Pts',(7.88958146472778,15.2,8.30570646745553));
#210597=CARTESIAN_POINT('Ctrl Pts',(7.89310351022376,15.2,8.30705092374024));
#210598=CARTESIAN_POINT('Ctrl Pts',(7.89662555635957,15.2,8.3083953802692));
#210599=CARTESIAN_POINT('Ctrl Pts',(7.90015536668925,15.2,8.30973818933102));
#210600=CARTESIAN_POINT('Ctrl Pts',(7.90369291574608,15.2,8.3110793087757));
#210601=CARTESIAN_POINT('Ctrl Pts',(7.90723046416027,15.2,8.31242042797673));
#210602=CARTESIAN_POINT('Ctrl Pts',(7.91077575090475,15.2,8.31375985704076));
#210603=CARTESIAN_POINT('Ctrl Pts',(7.91432875270405,15.2,8.31509755705879));
#210604=CARTESIAN_POINT('Ctrl Pts',(7.91788175450336,15.2,8.31643525707682));
#210605=CARTESIAN_POINT('Ctrl Pts',(7.92144247234112,15.2,8.31777122784645));
#210606=CARTESIAN_POINT('Ctrl Pts',(7.92501089566236,15.2,8.31910545566979));
#210607=CARTESIAN_POINT('Ctrl Pts',(7.92857931898359,15.2,8.32043968349314));
#210608=CARTESIAN_POINT('Ctrl Pts',(7.93215544959198,15.2,8.32177216810586));
#210609=CARTESIAN_POINT('Ctrl Pts',(7.93573928199995,15.2,8.32310290899999));
#210610=CARTESIAN_POINT('Origin',(-5.66257110645729E-14,15.2,-1.77635683940025E-14));
#210611=CARTESIAN_POINT('',(6.57080831899994,15.2,8.02901631899999));
#210612=CARTESIAN_POINT('',(6.57080831899994,12.2,8.02901631899999));
#210613=CARTESIAN_POINT('',(6.57080831899994,15.2,8.02901631899999));
#210614=CARTESIAN_POINT('Origin',(-5.66257110645729E-14,12.2,-1.77635683940025E-14));
#210615=CARTESIAN_POINT('Origin',(-5.66257110645729E-14,15.2,-1.77635683940025E-14));
#210616=CARTESIAN_POINT('Origin',(-5.66257110645729E-14,15.2,-1.77635683940025E-14));
#210617=CARTESIAN_POINT('',(6.97920857099994,15.2,9.14005731499999));
#210618=CARTESIAN_POINT('',(6.67046385465267,15.2,9.36775917498041));
#210619=CARTESIAN_POINT('Origin',(-5.66257110645729E-14,15.2,-1.77635683940025E-14));
#210620=CARTESIAN_POINT('',(6.67046385465267,12.2,9.36775917498041));
#210621=CARTESIAN_POINT('',(6.67046385499994,15.2,9.36775917499999));
#210622=CARTESIAN_POINT('',(6.97920857099994,12.2,9.14005731499999));
#210623=CARTESIAN_POINT('Origin',(-5.66257110645729E-14,12.2,-1.77635683940025E-14));
#210624=CARTESIAN_POINT('',(6.97920857099994,15.2,9.14005731499999));
#210625=CARTESIAN_POINT('Ctrl Pts',(6.67046385399994,15.2,9.36775917499999));
#210626=CARTESIAN_POINT('Ctrl Pts',(6.67046385399994,11.6,9.36775917499999));
#210627=CARTESIAN_POINT('Ctrl Pts',(6.66979225999994,15.2,9.36739372899999));
#210628=CARTESIAN_POINT('Ctrl Pts',(6.66979225999994,11.6,9.36739372899999));
#210629=CARTESIAN_POINT('Ctrl Pts',(6.66844959599994,15.2,9.36666279599999));
#210630=CARTESIAN_POINT('Ctrl Pts',(6.66844959599994,11.6,9.36666279599999));
#210631=CARTESIAN_POINT('Ctrl Pts',(6.66643717599994,15.2,9.36556626999998));
#210632=CARTESIAN_POINT('Ctrl Pts',(6.66643717599994,11.6,9.36556626999998));
#210633=CARTESIAN_POINT('Ctrl Pts',(6.66375709799994,15.2,9.36410398399998));
#210634=CARTESIAN_POINT('Ctrl Pts',(6.66375709799994,11.6,9.36410398399998));
#210635=CARTESIAN_POINT('Ctrl Pts',(6.66041225099994,15.2,9.36227570699998));
#210636=CARTESIAN_POINT('Ctrl Pts',(6.66041225099994,11.6,9.36227570699998));
#210637=CARTESIAN_POINT('Ctrl Pts',(6.65707265499995,15.2,9.36044700999999));
#210638=CARTESIAN_POINT('Ctrl Pts',(6.65707265499995,11.6,9.36044700999999));
#210639=CARTESIAN_POINT('Ctrl Pts',(6.65373830999994,15.2,9.35861789599999));
#210640=CARTESIAN_POINT('Ctrl Pts',(6.65373830999994,11.6,9.35861789599999));
#210641=CARTESIAN_POINT('Ctrl Pts',(6.65040921899994,15.2,9.35678837099999));
#210642=CARTESIAN_POINT('Ctrl Pts',(6.65040921899994,11.6,9.35678837099999));
#210643=CARTESIAN_POINT('Ctrl Pts',(6.64708538299994,15.2,9.35495843699999));
#210644=CARTESIAN_POINT('Ctrl Pts',(6.64708538299994,11.6,9.35495843699999));
#210645=CARTESIAN_POINT('Ctrl Pts',(6.64376680599994,15.2,9.35312810399999));
#210646=CARTESIAN_POINT('Ctrl Pts',(6.64376680599994,11.6,9.35312810399999));
#210647=CARTESIAN_POINT('Ctrl Pts',(6.64045349299994,15.2,9.35129737899998));
#210648=CARTESIAN_POINT('Ctrl Pts',(6.64045349299994,11.6,9.35129737899998));
#210649=CARTESIAN_POINT('Ctrl Pts',(6.63714544599994,15.2,9.34946627399999));
#210650=CARTESIAN_POINT('Ctrl Pts',(6.63714544599994,11.6,9.34946627399999));
#210651=CARTESIAN_POINT('Ctrl Pts',(6.63384266999994,15.2,9.34763479799999));
#210652=CARTESIAN_POINT('Ctrl Pts',(6.63384266999994,11.6,9.34763479799999));
#210653=CARTESIAN_POINT('Ctrl Pts',(6.63054516999994,15.2,9.34580296099998));
#210654=CARTESIAN_POINT('Ctrl Pts',(6.63054516999994,11.6,9.34580296099998));
#210655=CARTESIAN_POINT('Ctrl Pts',(6.62725294799994,15.2,9.34397077399998));
#210656=CARTESIAN_POINT('Ctrl Pts',(6.62725294799994,11.6,9.34397077399998));
#210657=CARTESIAN_POINT('Ctrl Pts',(6.62396601099994,15.2,9.34213824399999));
#210658=CARTESIAN_POINT('Ctrl Pts',(6.62396601099994,11.6,9.34213824399999));
#210659=CARTESIAN_POINT('Ctrl Pts',(6.62068435999994,15.2,9.34030537999998));
#210660=CARTESIAN_POINT('Ctrl Pts',(6.62068435999994,11.6,9.34030537999998));
#210661=CARTESIAN_POINT('Ctrl Pts',(6.61740799799994,15.2,9.33847218999999));
#210662=CARTESIAN_POINT('Ctrl Pts',(6.61740799799994,11.6,9.33847218999999));
#210663=CARTESIAN_POINT('Ctrl Pts',(6.61413692799995,15.2,9.33663867999999));
#210664=CARTESIAN_POINT('Ctrl Pts',(6.61413692799995,11.6,9.33663867999999));
#210665=CARTESIAN_POINT('Ctrl Pts',(6.61087115499994,15.2,9.33480485999999));
#210666=CARTESIAN_POINT('Ctrl Pts',(6.61087115499994,11.6,9.33480485999999));
#210667=CARTESIAN_POINT('Ctrl Pts',(6.60761068099994,15.2,9.33297073499999));
#210668=CARTESIAN_POINT('Ctrl Pts',(6.60761068099994,11.6,9.33297073499999));
#210669=CARTESIAN_POINT('Ctrl Pts',(6.60435550799994,15.2,9.33113631499998));
#210670=CARTESIAN_POINT('Ctrl Pts',(6.60435550799994,11.6,9.33113631499998));
#210671=CARTESIAN_POINT('Ctrl Pts',(6.60110564199995,15.2,9.32930160899998));
#210672=CARTESIAN_POINT('Ctrl Pts',(6.60110564199995,11.6,9.32930160899998));
#210673=CARTESIAN_POINT('Ctrl Pts',(6.59786108499994,15.2,9.32746662499999));
#210674=CARTESIAN_POINT('Ctrl Pts',(6.59786108499994,11.6,9.32746662499999));
#210675=CARTESIAN_POINT('Ctrl Pts',(6.59462184299994,15.2,9.32563137199999));
#210676=CARTESIAN_POINT('Ctrl Pts',(6.59462184299994,11.6,9.32563137199999));
#210677=CARTESIAN_POINT('Ctrl Pts',(6.59138791599994,15.2,9.32379585899999));
#210678=CARTESIAN_POINT('Ctrl Pts',(6.59138791599994,11.6,9.32379585899999));
#210679=CARTESIAN_POINT('Ctrl Pts',(6.58815930899994,15.2,9.32196009399998));
#210680=CARTESIAN_POINT('Ctrl Pts',(6.58815930899994,11.6,9.32196009399998));
#210681=CARTESIAN_POINT('Ctrl Pts',(6.58493602699994,15.2,9.32012408699999));
#210682=CARTESIAN_POINT('Ctrl Pts',(6.58493602699994,11.6,9.32012408699999));
#210683=CARTESIAN_POINT('Ctrl Pts',(6.58171807199994,15.2,9.31828784399999));
#210684=CARTESIAN_POINT('Ctrl Pts',(6.58171807199994,11.6,9.31828784399999));
#210685=CARTESIAN_POINT('Ctrl Pts',(6.57850544799994,15.2,9.31645137699999));
#210686=CARTESIAN_POINT('Ctrl Pts',(6.57850544799994,11.6,9.31645137699999));
#210687=CARTESIAN_POINT('Ctrl Pts',(6.57529815699994,15.2,9.31461469099998));
#210688=CARTESIAN_POINT('Ctrl Pts',(6.57529815699994,11.6,9.31461469099998));
#210689=CARTESIAN_POINT('Ctrl Pts',(6.57209620299994,15.2,9.31277779599998));
#210690=CARTESIAN_POINT('Ctrl Pts',(6.57209620299994,11.6,9.31277779599998));
#210691=CARTESIAN_POINT('Ctrl Pts',(6.56889959099995,15.2,9.31094069999999));
#210692=CARTESIAN_POINT('Ctrl Pts',(6.56889959099995,11.6,9.31094069999999));
#210693=CARTESIAN_POINT('Ctrl Pts',(6.56570832199994,15.2,9.30910341199999));
#210694=CARTESIAN_POINT('Ctrl Pts',(6.56570832199994,11.6,9.30910341199999));
#210695=CARTESIAN_POINT('Ctrl Pts',(6.56252240099994,15.2,9.30726594099998));
#210696=CARTESIAN_POINT('Ctrl Pts',(6.56252240099994,11.6,9.30726594099998));
#210697=CARTESIAN_POINT('Ctrl Pts',(6.55934183199994,15.2,9.30542829599998));
#210698=CARTESIAN_POINT('Ctrl Pts',(6.55934183199994,11.6,9.30542829599998));
#210699=CARTESIAN_POINT('Ctrl Pts',(6.55616661699994,15.2,9.30359048399998));
#210700=CARTESIAN_POINT('Ctrl Pts',(6.55616661699994,11.6,9.30359048399998));
#210701=CARTESIAN_POINT('Ctrl Pts',(6.55299675999995,15.2,9.30175251599999));
#210702=CARTESIAN_POINT('Ctrl Pts',(6.55299675999995,11.6,9.30175251599999));
#210703=CARTESIAN_POINT('Ctrl Pts',(6.54983226499994,15.2,9.29991439899998));
#210704=CARTESIAN_POINT('Ctrl Pts',(6.54983226499994,11.6,9.29991439899998));
#210705=CARTESIAN_POINT('Ctrl Pts',(6.54667313399995,15.2,9.29807614199999));
#210706=CARTESIAN_POINT('Ctrl Pts',(6.54667313399995,11.6,9.29807614199999));
#210707=CARTESIAN_POINT('Ctrl Pts',(6.54351937199994,15.2,9.29623775399998));
#210708=CARTESIAN_POINT('Ctrl Pts',(6.54351937199994,11.6,9.29623775399998));
#210709=CARTESIAN_POINT('Ctrl Pts',(6.54037098099994,15.2,9.29439924499999));
#210710=CARTESIAN_POINT('Ctrl Pts',(6.54037098099994,11.6,9.29439924499999));
#210711=CARTESIAN_POINT('Ctrl Pts',(6.53722796599994,15.2,9.29256062199999));
#210712=CARTESIAN_POINT('Ctrl Pts',(6.53722796599994,11.6,9.29256062199999));
#210713=CARTESIAN_POINT('Ctrl Pts',(6.53409032999994,15.2,9.29072189399999));
#210714=CARTESIAN_POINT('Ctrl Pts',(6.53409032999994,11.6,9.29072189399999));
#210715=CARTESIAN_POINT('Ctrl Pts',(6.53095807499994,15.2,9.28888306999998));
#210716=CARTESIAN_POINT('Ctrl Pts',(6.53095807499994,11.6,9.28888306999998));
#210717=CARTESIAN_POINT('Ctrl Pts',(6.52783120599994,15.2,9.28704415999999));
#210718=CARTESIAN_POINT('Ctrl Pts',(6.52783120599994,11.6,9.28704415999999));
#210719=CARTESIAN_POINT('Ctrl Pts',(6.52470972599994,15.2,9.28520517099999));
#210720=CARTESIAN_POINT('Ctrl Pts',(6.52470972599994,11.6,9.28520517099999));
#210721=CARTESIAN_POINT('Ctrl Pts',(6.52159363899995,15.2,9.28336611399999));
#210722=CARTESIAN_POINT('Ctrl Pts',(6.52159363899995,11.6,9.28336611399999));
#210723=CARTESIAN_POINT('Ctrl Pts',(6.51848294799994,15.2,9.28152699599998));
#210724=CARTESIAN_POINT('Ctrl Pts',(6.51848294799994,11.6,9.28152699599998));
#210725=CARTESIAN_POINT('Ctrl Pts',(6.51537765399994,15.2,9.27968782599999));
#210726=CARTESIAN_POINT('Ctrl Pts',(6.51537765399994,11.6,9.27968782599999));
#210727=CARTESIAN_POINT('Ctrl Pts',(6.51227776499994,15.2,9.27784861499998));
#210728=CARTESIAN_POINT('Ctrl Pts',(6.51227776499994,11.6,9.27784861499998));
#210729=CARTESIAN_POINT('Ctrl Pts',(6.50918327999994,15.2,9.27600936999998));
#210730=CARTESIAN_POINT('Ctrl Pts',(6.50918327999994,11.6,9.27600936999998));
#210731=CARTESIAN_POINT('Ctrl Pts',(6.50609420699994,15.2,9.27417009999999));
#210732=CARTESIAN_POINT('Ctrl Pts',(6.50609420699994,11.6,9.27417009999999));
#210733=CARTESIAN_POINT('Ctrl Pts',(6.50301054499994,15.2,9.27233081499999));
#210734=CARTESIAN_POINT('Ctrl Pts',(6.50301054499994,11.6,9.27233081499999));
#210735=CARTESIAN_POINT('Ctrl Pts',(6.49993229999994,15.2,9.27049152299999));
#210736=CARTESIAN_POINT('Ctrl Pts',(6.49993229999994,11.6,9.27049152299999));
#210737=CARTESIAN_POINT('Ctrl Pts',(6.49685947499994,15.2,9.26865223299998));
#210738=CARTESIAN_POINT('Ctrl Pts',(6.49685947499994,11.6,9.26865223299998));
#210739=CARTESIAN_POINT('Ctrl Pts',(6.49379207299994,15.2,9.26681295599998));
#210740=CARTESIAN_POINT('Ctrl Pts',(6.49379207299994,11.6,9.26681295599998));
#210741=CARTESIAN_POINT('Ctrl Pts',(6.49073009699994,15.2,9.26497369899998));
#210742=CARTESIAN_POINT('Ctrl Pts',(6.49073009699994,11.6,9.26497369899998));
#210743=CARTESIAN_POINT('Ctrl Pts',(6.48767355099994,15.2,9.26313447199998));
#210744=CARTESIAN_POINT('Ctrl Pts',(6.48767355099994,11.6,9.26313447199998));
#210745=CARTESIAN_POINT('Ctrl Pts',(6.48462243899994,15.2,9.26129528299998));
#210746=CARTESIAN_POINT('Ctrl Pts',(6.48462243899994,11.6,9.26129528299998));
#210747=CARTESIAN_POINT('Ctrl Pts',(6.48157676399994,15.2,9.25945614199998));
#210748=CARTESIAN_POINT('Ctrl Pts',(6.48157676399994,11.6,9.25945614199998));
#210749=CARTESIAN_POINT('Ctrl Pts',(6.47853652899994,15.2,9.25761705899999));
#210750=CARTESIAN_POINT('Ctrl Pts',(6.47853652899994,11.6,9.25761705899999));
#210751=CARTESIAN_POINT('Ctrl Pts',(6.47550173799995,15.2,9.25577804099999));
#210752=CARTESIAN_POINT('Ctrl Pts',(6.47550173799995,11.6,9.25577804099999));
#210753=CARTESIAN_POINT('Ctrl Pts',(6.47247239299994,15.2,9.25393909899999));
#210754=CARTESIAN_POINT('Ctrl Pts',(6.47247239299994,11.6,9.25393909899999));
#210755=CARTESIAN_POINT('Ctrl Pts',(6.46944849899994,15.2,9.25210024199998));
#210756=CARTESIAN_POINT('Ctrl Pts',(6.46944849899994,11.6,9.25210024199998));
#210757=CARTESIAN_POINT('Ctrl Pts',(6.46643005899994,15.2,9.25026147899998));
#210758=CARTESIAN_POINT('Ctrl Pts',(6.46643005899994,11.6,9.25026147899998));
#210759=CARTESIAN_POINT('Ctrl Pts',(6.46341707499994,15.2,9.24842281899998));
#210760=CARTESIAN_POINT('Ctrl Pts',(6.46341707499994,11.6,9.24842281899998));
#210761=CARTESIAN_POINT('Ctrl Pts',(6.46040955299994,15.2,9.24658427099999));
#210762=CARTESIAN_POINT('Ctrl Pts',(6.46040955299994,11.6,9.24658427099999));
#210763=CARTESIAN_POINT('Ctrl Pts',(6.45740749499994,15.2,9.24474584499999));
#210764=CARTESIAN_POINT('Ctrl Pts',(6.45740749499994,11.6,9.24474584499999));
#210765=CARTESIAN_POINT('Ctrl Pts',(6.45441090399994,15.2,9.24290754999999));
#210766=CARTESIAN_POINT('Ctrl Pts',(6.45441090399994,11.6,9.24290754999999));
#210767=CARTESIAN_POINT('Ctrl Pts',(6.45141978499994,15.2,9.24106939399999));
#210768=CARTESIAN_POINT('Ctrl Pts',(6.45141978499994,11.6,9.24106939399999));
#210769=CARTESIAN_POINT('Ctrl Pts',(6.44843413899994,15.2,9.23923138899998));
#210770=CARTESIAN_POINT('Ctrl Pts',(6.44843413899994,11.6,9.23923138899998));
#210771=CARTESIAN_POINT('Ctrl Pts',(6.44545397099994,15.2,9.23739354299999));
#210772=CARTESIAN_POINT('Ctrl Pts',(6.44545397099994,11.6,9.23739354299999));
#210773=CARTESIAN_POINT('Ctrl Pts',(6.44247928399994,15.2,9.23555586399999));
#210774=CARTESIAN_POINT('Ctrl Pts',(6.44247928399994,11.6,9.23555586399999));
#210775=CARTESIAN_POINT('Ctrl Pts',(6.43951008099994,15.2,9.23371836299999));
#210776=CARTESIAN_POINT('Ctrl Pts',(6.43951008099994,11.6,9.23371836299999));
#210777=CARTESIAN_POINT('Ctrl Pts',(6.43654636599994,15.2,9.23188105099998));
#210778=CARTESIAN_POINT('Ctrl Pts',(6.43654636599994,11.6,9.23188105099998));
#210779=CARTESIAN_POINT('Ctrl Pts',(6.43358814399994,15.2,9.23004393399999));
#210780=CARTESIAN_POINT('Ctrl Pts',(6.43358814399994,11.6,9.23004393399999));
#210781=CARTESIAN_POINT('Ctrl Pts',(6.43063541499994,15.2,9.22820702299998));
#210782=CARTESIAN_POINT('Ctrl Pts',(6.43063541499994,11.6,9.22820702299998));
#210783=CARTESIAN_POINT('Ctrl Pts',(6.42768818399994,15.2,9.22637032699999));
#210784=CARTESIAN_POINT('Ctrl Pts',(6.42768818399994,11.6,9.22637032699999));
#210785=CARTESIAN_POINT('Ctrl Pts',(6.42474645399994,15.2,9.22453385799999));
#210786=CARTESIAN_POINT('Ctrl Pts',(6.42474645399994,11.6,9.22453385799999));
#210787=CARTESIAN_POINT('Ctrl Pts',(6.42181022999995,15.2,9.22269762299998));
#210788=CARTESIAN_POINT('Ctrl Pts',(6.42181022999995,11.6,9.22269762299998));
#210789=CARTESIAN_POINT('Ctrl Pts',(6.41887951299994,15.2,9.22086163099999));
#210790=CARTESIAN_POINT('Ctrl Pts',(6.41887951299994,11.6,9.22086163099999));
#210791=CARTESIAN_POINT('Ctrl Pts',(6.41595430799994,15.2,9.21902589299999));
#210792=CARTESIAN_POINT('Ctrl Pts',(6.41595430799994,11.6,9.21902589299999));
#210793=CARTESIAN_POINT('Ctrl Pts',(6.41303461899994,15.2,9.21719041899999));
#210794=CARTESIAN_POINT('Ctrl Pts',(6.41303461899994,11.6,9.21719041899999));
#210795=CARTESIAN_POINT('Ctrl Pts',(6.41012044699994,15.2,9.21535521599999));
#210796=CARTESIAN_POINT('Ctrl Pts',(6.41012044699994,11.6,9.21535521599999));
#210797=CARTESIAN_POINT('Ctrl Pts',(6.40721179599994,15.2,9.21352029699998));
#210798=CARTESIAN_POINT('Ctrl Pts',(6.40721179599994,11.6,9.21352029699998));
#210799=CARTESIAN_POINT('Ctrl Pts',(6.40430867099994,15.2,9.21168566999999));
#210800=CARTESIAN_POINT('Ctrl Pts',(6.40430867099994,11.6,9.21168566999999));
#210801=CARTESIAN_POINT('Ctrl Pts',(6.40141107399994,15.2,9.20985134399999));
#210802=CARTESIAN_POINT('Ctrl Pts',(6.40141107399994,11.6,9.20985134399999));
#210803=CARTESIAN_POINT('Ctrl Pts',(6.39851900999994,15.2,9.20801732999998));
#210804=CARTESIAN_POINT('Ctrl Pts',(6.39851900999994,11.6,9.20801732999998));
#210805=CARTESIAN_POINT('Ctrl Pts',(6.39563247999994,15.2,9.20618363799999));
#210806=CARTESIAN_POINT('Ctrl Pts',(6.39563247999994,11.6,9.20618363799999));
#210807=CARTESIAN_POINT('Ctrl Pts',(6.39275148899995,15.2,9.20435027499998));
#210808=CARTESIAN_POINT('Ctrl Pts',(6.39275148899995,11.6,9.20435027499998));
#210809=CARTESIAN_POINT('Ctrl Pts',(6.38987603999994,15.2,9.20251725399999));
#210810=CARTESIAN_POINT('Ctrl Pts',(6.38987603999994,11.6,9.20251725399999));
#210811=CARTESIAN_POINT('Ctrl Pts',(6.38700613599994,15.2,9.20068458399999));
#210812=CARTESIAN_POINT('Ctrl Pts',(6.38700613599994,11.6,9.20068458399999));
#210813=CARTESIAN_POINT('Ctrl Pts',(6.38414177999994,15.2,9.19885227399998));
#210814=CARTESIAN_POINT('Ctrl Pts',(6.38414177999994,11.6,9.19885227399998));
#210815=CARTESIAN_POINT('Ctrl Pts',(6.38128297699994,15.2,9.19702033299998));
#210816=CARTESIAN_POINT('Ctrl Pts',(6.38128297699994,11.6,9.19702033299998));
#210817=CARTESIAN_POINT('Ctrl Pts',(6.37842972899994,15.2,9.19518877199998));
#210818=CARTESIAN_POINT('Ctrl Pts',(6.37842972899994,11.6,9.19518877199998));
#210819=CARTESIAN_POINT('Ctrl Pts',(6.37558203999994,15.2,9.19335760099998));
#210820=CARTESIAN_POINT('Ctrl Pts',(6.37558203999994,11.6,9.19335760099998));
#210821=CARTESIAN_POINT('Ctrl Pts',(6.37273991299994,15.2,9.19152682999999));
#210822=CARTESIAN_POINT('Ctrl Pts',(6.37273991299994,11.6,9.19152682999999));
#210823=CARTESIAN_POINT('Ctrl Pts',(6.36990335099994,15.2,9.18969646699999));
#210824=CARTESIAN_POINT('Ctrl Pts',(6.36990335099994,11.6,9.18969646699999));
#210825=CARTESIAN_POINT('Ctrl Pts',(6.36707235799994,15.2,9.18786652599999));
#210826=CARTESIAN_POINT('Ctrl Pts',(6.36707235799994,11.6,9.18786652599999));
#210827=CARTESIAN_POINT('Ctrl Pts',(6.36424693799994,15.2,9.18603701199999));
#210828=CARTESIAN_POINT('Ctrl Pts',(6.36424693799994,11.6,9.18603701199999));
#210829=CARTESIAN_POINT('Ctrl Pts',(6.36142709299994,15.2,9.18420793799999));
#210830=CARTESIAN_POINT('Ctrl Pts',(6.36142709299994,11.6,9.18420793799999));
#210831=CARTESIAN_POINT('Ctrl Pts',(6.35861282699994,15.2,9.18237931399998));
#210832=CARTESIAN_POINT('Ctrl Pts',(6.35861282699994,11.6,9.18237931399998));
#210833=CARTESIAN_POINT('Ctrl Pts',(6.35580414299994,15.2,9.18055114999999));
#210834=CARTESIAN_POINT('Ctrl Pts',(6.35580414299994,11.6,9.18055114999999));
#210835=CARTESIAN_POINT('Ctrl Pts',(6.35300104399994,15.2,9.17872345399999));
#210836=CARTESIAN_POINT('Ctrl Pts',(6.35300104399994,11.6,9.17872345399999));
#210837=CARTESIAN_POINT('Ctrl Pts',(6.35020353499994,15.2,9.17689623799999));
#210838=CARTESIAN_POINT('Ctrl Pts',(6.35020353499994,11.6,9.17689623799999));
#210839=CARTESIAN_POINT('Ctrl Pts',(6.34741161699995,15.2,9.17506951099998));
#210840=CARTESIAN_POINT('Ctrl Pts',(6.34741161699995,11.6,9.17506951099998));
#210841=CARTESIAN_POINT('Ctrl Pts',(6.34462529599994,15.2,9.17324328399998));
#210842=CARTESIAN_POINT('Ctrl Pts',(6.34462529599994,11.6,9.17324328399998));
#210843=CARTESIAN_POINT('Ctrl Pts',(6.34184457399994,15.2,9.17141756699999));
#210844=CARTESIAN_POINT('Ctrl Pts',(6.34184457399994,11.6,9.17141756699999));
#210845=CARTESIAN_POINT('Ctrl Pts',(6.33906945299994,15.2,9.16959236999999));
#210846=CARTESIAN_POINT('Ctrl Pts',(6.33906945299994,11.6,9.16959236999999));
#210847=CARTESIAN_POINT('Ctrl Pts',(6.33629993899994,15.2,9.16776770199998));
#210848=CARTESIAN_POINT('Ctrl Pts',(6.33629993899994,11.6,9.16776770199998));
#210849=CARTESIAN_POINT('Ctrl Pts',(6.33353603299994,15.2,9.16594357499999));
#210850=CARTESIAN_POINT('Ctrl Pts',(6.33353603299994,11.6,9.16594357499999));
#210851=CARTESIAN_POINT('Ctrl Pts',(6.33077773999994,15.2,9.16411999899999));
#210852=CARTESIAN_POINT('Ctrl Pts',(6.33077773999994,11.6,9.16411999899999));
#210853=CARTESIAN_POINT('Ctrl Pts',(6.32802506299995,15.2,9.16229698299999));
#210854=CARTESIAN_POINT('Ctrl Pts',(6.32802506299995,11.6,9.16229698299999));
#210855=CARTESIAN_POINT('Ctrl Pts',(6.32527800399994,15.2,9.16047453899999));
#210856=CARTESIAN_POINT('Ctrl Pts',(6.32527800399994,11.6,9.16047453899999));
#210857=CARTESIAN_POINT('Ctrl Pts',(6.32253656799994,15.2,9.15865267499999));
#210858=CARTESIAN_POINT('Ctrl Pts',(6.32253656799994,11.6,9.15865267499999));
#210859=CARTESIAN_POINT('Ctrl Pts',(6.31980075799994,15.2,9.15683140299999));
#210860=CARTESIAN_POINT('Ctrl Pts',(6.31980075799994,11.6,9.15683140299999));
#210861=CARTESIAN_POINT('Ctrl Pts',(6.31707057599994,15.2,9.15501073299998));
#210862=CARTESIAN_POINT('Ctrl Pts',(6.31707057599994,11.6,9.15501073299998));
#210863=CARTESIAN_POINT('Ctrl Pts',(6.31434602699994,15.2,9.15319067599999));
#210864=CARTESIAN_POINT('Ctrl Pts',(6.31434602699994,11.6,9.15319067599999));
#210865=CARTESIAN_POINT('Ctrl Pts',(6.31162711399995,15.2,9.15137123999998));
#210866=CARTESIAN_POINT('Ctrl Pts',(6.31162711399995,11.6,9.15137123999998));
#210867=CARTESIAN_POINT('Ctrl Pts',(6.30891383899994,15.2,9.14955243799999));
#210868=CARTESIAN_POINT('Ctrl Pts',(6.30891383899994,11.6,9.14955243799999));
#210869=CARTESIAN_POINT('Ctrl Pts',(6.30620620699994,15.2,9.14773428099998));
#210870=CARTESIAN_POINT('Ctrl Pts',(6.30620620699994,11.6,9.14773428099998));
#210871=CARTESIAN_POINT('Ctrl Pts',(6.30350422099994,15.2,9.14591677599999));
#210872=CARTESIAN_POINT('Ctrl Pts',(6.30350422099994,11.6,9.14591677599999));
#210873=CARTESIAN_POINT('Ctrl Pts',(6.30080788399994,15.2,9.14409993499999));
#210874=CARTESIAN_POINT('Ctrl Pts',(6.30080788399994,11.6,9.14409993499999));
#210875=CARTESIAN_POINT('Ctrl Pts',(6.29811719899994,15.2,9.14228377099998));
#210876=CARTESIAN_POINT('Ctrl Pts',(6.29811719899994,11.6,9.14228377099998));
#210877=CARTESIAN_POINT('Ctrl Pts',(6.29543216899994,15.2,9.14046829099998));
#210878=CARTESIAN_POINT('Ctrl Pts',(6.29543216899994,11.6,9.14046829099998));
#210879=CARTESIAN_POINT('Ctrl Pts',(6.29275279799994,15.2,9.13865350699999));
#210880=CARTESIAN_POINT('Ctrl Pts',(6.29275279799994,11.6,9.13865350699999));
#210881=CARTESIAN_POINT('Ctrl Pts',(6.29007908999994,15.2,9.13683942999998));
#210882=CARTESIAN_POINT('Ctrl Pts',(6.29007908999994,11.6,9.13683942999998));
#210883=CARTESIAN_POINT('Ctrl Pts',(6.28741104799994,15.2,9.13502606899998));
#210884=CARTESIAN_POINT('Ctrl Pts',(6.28741104799994,11.6,9.13502606899998));
#210885=CARTESIAN_POINT('Ctrl Pts',(6.28474867399994,15.2,9.13321343699998));
#210886=CARTESIAN_POINT('Ctrl Pts',(6.28474867399994,11.6,9.13321343699998));
#210887=CARTESIAN_POINT('Ctrl Pts',(6.28209197199994,15.2,9.13140154299998));
#210888=CARTESIAN_POINT('Ctrl Pts',(6.28209197199994,11.6,9.13140154299998));
#210889=CARTESIAN_POINT('Ctrl Pts',(6.27944094699994,15.2,9.12959039799999));
#210890=CARTESIAN_POINT('Ctrl Pts',(6.27944094699994,11.6,9.12959039799999));
#210891=CARTESIAN_POINT('Ctrl Pts',(6.27679559899994,15.2,9.12778001299999));
#210892=CARTESIAN_POINT('Ctrl Pts',(6.27679559899994,11.6,9.12778001299999));
#210893=CARTESIAN_POINT('Ctrl Pts',(6.27415593399994,15.2,9.12597039899998));
#210894=CARTESIAN_POINT('Ctrl Pts',(6.27415593399994,11.6,9.12597039899998));
#210895=CARTESIAN_POINT('Ctrl Pts',(6.27152195499994,15.2,9.12416156499999));
#210896=CARTESIAN_POINT('Ctrl Pts',(6.27152195499994,11.6,9.12416156499999));
#210897=CARTESIAN_POINT('Ctrl Pts',(6.26889366399994,15.2,9.12235352399998));
#210898=CARTESIAN_POINT('Ctrl Pts',(6.26889366399994,11.6,9.12235352399998));
#210899=CARTESIAN_POINT('Ctrl Pts',(6.26627106499994,15.2,9.12054628599999));
#210900=CARTESIAN_POINT('Ctrl Pts',(6.26627106499994,11.6,9.12054628599999));
#210901=CARTESIAN_POINT('Ctrl Pts',(6.26365416199994,15.2,9.11873985999998));
#210902=CARTESIAN_POINT('Ctrl Pts',(6.26365416199994,11.6,9.11873985999998));
#210903=CARTESIAN_POINT('Ctrl Pts',(6.26104295599994,15.2,9.11693425999999));
#210904=CARTESIAN_POINT('Ctrl Pts',(6.26104295599994,11.6,9.11693425999999));
#210905=CARTESIAN_POINT('Ctrl Pts',(6.25843745399994,15.2,9.11512949599998));
#210906=CARTESIAN_POINT('Ctrl Pts',(6.25843745399994,11.6,9.11512949599998));
#210907=CARTESIAN_POINT('Ctrl Pts',(6.25583765699994,15.2,9.11332557699998));
#210908=CARTESIAN_POINT('Ctrl Pts',(6.25583765699994,11.6,9.11332557699998));
#210909=CARTESIAN_POINT('Ctrl Pts',(6.25324356799994,15.2,9.11152251499999));
#210910=CARTESIAN_POINT('Ctrl Pts',(6.25324356799994,11.6,9.11152251499999));
#210911=CARTESIAN_POINT('Ctrl Pts',(6.25065519099994,15.2,9.10972032199999));
#210912=CARTESIAN_POINT('Ctrl Pts',(6.25065519099994,11.6,9.10972032199999));
#210913=CARTESIAN_POINT('Ctrl Pts',(6.24807252799994,15.2,9.10791900599998));
#210914=CARTESIAN_POINT('Ctrl Pts',(6.24807252799994,11.6,9.10791900599998));
#210915=CARTESIAN_POINT('Ctrl Pts',(6.24549558499995,15.2,9.10611858299998));
#210916=CARTESIAN_POINT('Ctrl Pts',(6.24549558499995,11.6,9.10611858299998));
#210917=CARTESIAN_POINT('Ctrl Pts',(6.24292436299994,15.2,9.10431905899999));
#210918=CARTESIAN_POINT('Ctrl Pts',(6.24292436299994,11.6,9.10431905899999));
#210919=CARTESIAN_POINT('Ctrl Pts',(6.24035886599994,15.2,9.10252044899998));
#210920=CARTESIAN_POINT('Ctrl Pts',(6.24035886599994,11.6,9.10252044899998));
#210921=CARTESIAN_POINT('Ctrl Pts',(6.23779909799994,15.2,9.10072276099999));
#210922=CARTESIAN_POINT('Ctrl Pts',(6.23779909799994,11.6,9.10072276099999));
#210923=CARTESIAN_POINT('Ctrl Pts',(6.23524505999994,15.2,9.09892600699998));
#210924=CARTESIAN_POINT('Ctrl Pts',(6.23524505999994,11.6,9.09892600699998));
#210925=CARTESIAN_POINT('Ctrl Pts',(6.23269675799994,15.2,9.09713019899998));
#210926=CARTESIAN_POINT('Ctrl Pts',(6.23269675799994,11.6,9.09713019899998));
#210927=CARTESIAN_POINT('Ctrl Pts',(6.23015419399994,15.2,9.09533534799999));
#210928=CARTESIAN_POINT('Ctrl Pts',(6.23015419399994,11.6,9.09533534799999));
#210929=CARTESIAN_POINT('Ctrl Pts',(6.22761737199995,15.2,9.09354146399998));
#210930=CARTESIAN_POINT('Ctrl Pts',(6.22761737199995,11.6,9.09354146399998));
#210931=CARTESIAN_POINT('Ctrl Pts',(6.22508629399994,15.2,9.09174855899998));
#210932=CARTESIAN_POINT('Ctrl Pts',(6.22508629399994,11.6,9.09174855899998));
#210933=CARTESIAN_POINT('Ctrl Pts',(6.22256096399994,15.2,9.08995664499999));
#210934=CARTESIAN_POINT('Ctrl Pts',(6.22256096399994,11.6,9.08995664499999));
#210935=CARTESIAN_POINT('Ctrl Pts',(6.22004138599995,15.2,9.08816573299998));
#210936=CARTESIAN_POINT('Ctrl Pts',(6.22004138599995,11.6,9.08816573299998));
#210937=CARTESIAN_POINT('Ctrl Pts',(6.21752756199994,15.2,9.08637583199998));
#210938=CARTESIAN_POINT('Ctrl Pts',(6.21752756199994,11.6,9.08637583199998));
#210939=CARTESIAN_POINT('Ctrl Pts',(6.21501949499994,15.2,9.08458695699998));
#210940=CARTESIAN_POINT('Ctrl Pts',(6.21501949499994,11.6,9.08458695699998));
#210941=CARTESIAN_POINT('Ctrl Pts',(6.21251718999994,15.2,9.08279911699999));
#210942=CARTESIAN_POINT('Ctrl Pts',(6.21251718999994,11.6,9.08279911699999));
#210943=CARTESIAN_POINT('Ctrl Pts',(6.21002064899994,15.2,9.08101232299998));
#210944=CARTESIAN_POINT('Ctrl Pts',(6.21002064899994,11.6,9.08101232299998));
#210945=CARTESIAN_POINT('Ctrl Pts',(6.20752987599994,15.2,9.07922658799999));
#210946=CARTESIAN_POINT('Ctrl Pts',(6.20752987599994,11.6,9.07922658799999));
#210947=CARTESIAN_POINT('Ctrl Pts',(6.20504487399994,15.2,9.07744192299998));
#210948=CARTESIAN_POINT('Ctrl Pts',(6.20504487399994,11.6,9.07744192299998));
#210949=CARTESIAN_POINT('Ctrl Pts',(6.20256564499994,15.2,9.07565833799998));
#210950=CARTESIAN_POINT('Ctrl Pts',(6.20256564499994,11.6,9.07565833799998));
#210951=CARTESIAN_POINT('Ctrl Pts',(6.20009219499994,15.2,9.07387584599999));
#210952=CARTESIAN_POINT('Ctrl Pts',(6.20009219499994,11.6,9.07387584599999));
#210953=CARTESIAN_POINT('Ctrl Pts',(6.19762452399995,15.2,9.07209445799998));
#210954=CARTESIAN_POINT('Ctrl Pts',(6.19762452399995,11.6,9.07209445799998));
#210955=CARTESIAN_POINT('Ctrl Pts',(6.19516263699994,15.2,9.07031418699999));
#210956=CARTESIAN_POINT('Ctrl Pts',(6.19516263699994,11.6,9.07031418699999));
#210957=CARTESIAN_POINT('Ctrl Pts',(6.19270653899994,15.2,9.06853504199999));
#210958=CARTESIAN_POINT('Ctrl Pts',(6.19270653899994,11.6,9.06853504199999));
#210959=CARTESIAN_POINT('Ctrl Pts',(6.19025622999994,15.2,9.06675703599999));
#210960=CARTESIAN_POINT('Ctrl Pts',(6.19025622999994,11.6,9.06675703599999));
#210961=CARTESIAN_POINT('Ctrl Pts',(6.18781171499994,15.2,9.06498017999999));
#210962=CARTESIAN_POINT('Ctrl Pts',(6.18781171499994,11.6,9.06498017999999));
#210963=CARTESIAN_POINT('Ctrl Pts',(6.18537299699994,15.2,9.06320448699999));
#210964=CARTESIAN_POINT('Ctrl Pts',(6.18537299699994,11.6,9.06320448699999));
#210965=CARTESIAN_POINT('Ctrl Pts',(6.18294007899994,15.2,9.06142996799998));
#210966=CARTESIAN_POINT('Ctrl Pts',(6.18294007899994,11.6,9.06142996799998));
#210967=CARTESIAN_POINT('Ctrl Pts',(6.18051296399994,15.2,9.05965663499998));
#210968=CARTESIAN_POINT('Ctrl Pts',(6.18051296399994,11.6,9.05965663499998));
#210969=CARTESIAN_POINT('Ctrl Pts',(6.17809165599994,15.2,9.05788449699998));
#210970=CARTESIAN_POINT('Ctrl Pts',(6.17809165599994,11.6,9.05788449699998));
#210971=CARTESIAN_POINT('Ctrl Pts',(6.17567615899994,15.2,9.05611356999999));
#210972=CARTESIAN_POINT('Ctrl Pts',(6.17567615899994,11.6,9.05611356999999));
#210973=CARTESIAN_POINT('Ctrl Pts',(6.17326647299994,15.2,9.05434386299999));
#210974=CARTESIAN_POINT('Ctrl Pts',(6.17326647299994,11.6,9.05434386299999));
#210975=CARTESIAN_POINT('Ctrl Pts',(6.17086260499994,15.2,9.05257538899999));
#210976=CARTESIAN_POINT('Ctrl Pts',(6.17086260499994,11.6,9.05257538899999));
#210977=CARTESIAN_POINT('Ctrl Pts',(6.16846455699994,15.2,9.05080815899998));
#210978=CARTESIAN_POINT('Ctrl Pts',(6.16846455699994,11.6,9.05080815899998));
#210979=CARTESIAN_POINT('Ctrl Pts',(6.16607233099994,15.2,9.04904218599999));
#210980=CARTESIAN_POINT('Ctrl Pts',(6.16607233099994,11.6,9.04904218599999));
#210981=CARTESIAN_POINT('Ctrl Pts',(6.16368593199994,15.2,9.04727748099998));
#210982=CARTESIAN_POINT('Ctrl Pts',(6.16368593199994,11.6,9.04727748099998));
#210983=CARTESIAN_POINT('Ctrl Pts',(6.16130536099995,15.2,9.04551405599998));
#210984=CARTESIAN_POINT('Ctrl Pts',(6.16130536099995,11.6,9.04551405599998));
#210985=CARTESIAN_POINT('Ctrl Pts',(6.15893062299994,15.2,9.04375192399998));
#210986=CARTESIAN_POINT('Ctrl Pts',(6.15893062299994,11.6,9.04375192399998));
#210987=CARTESIAN_POINT('Ctrl Pts',(6.15656172199994,15.2,9.04199109599999));
#210988=CARTESIAN_POINT('Ctrl Pts',(6.15656172199994,11.6,9.04199109599999));
#210989=CARTESIAN_POINT('Ctrl Pts',(6.15419865899994,15.2,9.04023158399998));
#210990=CARTESIAN_POINT('Ctrl Pts',(6.15419865899994,11.6,9.04023158399998));
#210991=CARTESIAN_POINT('Ctrl Pts',(6.15184143899994,15.2,9.03847339999999));
#210992=CARTESIAN_POINT('Ctrl Pts',(6.15184143899994,11.6,9.03847339999999));
#210993=CARTESIAN_POINT('Ctrl Pts',(6.14949006299994,15.2,9.03671655699998));
#210994=CARTESIAN_POINT('Ctrl Pts',(6.14949006299994,11.6,9.03671655699998));
#210995=CARTESIAN_POINT('Ctrl Pts',(6.14714453699994,15.2,9.03496106599999));
#210996=CARTESIAN_POINT('Ctrl Pts',(6.14714453699994,11.6,9.03496106599999));
#210997=CARTESIAN_POINT('Ctrl Pts',(6.14480486199994,15.2,9.03320694099998));
#210998=CARTESIAN_POINT('Ctrl Pts',(6.14480486199994,11.6,9.03320694099998));
#210999=CARTESIAN_POINT('Ctrl Pts',(6.14247104399994,15.2,9.03145419099998));
#211000=CARTESIAN_POINT('Ctrl Pts',(6.14247104399994,11.6,9.03145419099998));
#211001=CARTESIAN_POINT('Ctrl Pts',(6.14014308399994,15.2,9.02970283199998));
#211002=CARTESIAN_POINT('Ctrl Pts',(6.14014308399994,11.6,9.02970283199998));
#211003=CARTESIAN_POINT('Ctrl Pts',(6.13782098399994,15.2,9.02795287399999));
#211004=CARTESIAN_POINT('Ctrl Pts',(6.13782098399994,11.6,9.02795287399999));
#211005=CARTESIAN_POINT('Ctrl Pts',(6.13550474899994,15.2,9.02620432899998));
#211006=CARTESIAN_POINT('Ctrl Pts',(6.13550474899994,11.6,9.02620432899998));
#211007=CARTESIAN_POINT('Ctrl Pts',(6.13319438299994,15.2,9.02445720999999));
#211008=CARTESIAN_POINT('Ctrl Pts',(6.13319438299994,11.6,9.02445720999999));
#211009=CARTESIAN_POINT('Ctrl Pts',(6.13088988899994,15.2,9.02271152899999));
#211010=CARTESIAN_POINT('Ctrl Pts',(6.13088988899994,11.6,9.02271152899999));
#211011=CARTESIAN_POINT('Ctrl Pts',(6.12859126799994,15.2,9.02096729899998));
#211012=CARTESIAN_POINT('Ctrl Pts',(6.12859126799994,11.6,9.02096729899998));
#211013=CARTESIAN_POINT('Ctrl Pts',(6.12629852499994,15.2,9.01922453199998));
#211014=CARTESIAN_POINT('Ctrl Pts',(6.12629852499994,11.6,9.01922453199998));
#211015=CARTESIAN_POINT('Ctrl Pts',(6.12401166399994,15.2,9.01748324099999));
#211016=CARTESIAN_POINT('Ctrl Pts',(6.12401166399994,11.6,9.01748324099999));
#211017=CARTESIAN_POINT('Ctrl Pts',(6.12173068599994,15.2,9.01574343799999));
#211018=CARTESIAN_POINT('Ctrl Pts',(6.12173068599994,11.6,9.01574343799999));
#211019=CARTESIAN_POINT('Ctrl Pts',(6.11945559599994,15.2,9.01400513499999));
#211020=CARTESIAN_POINT('Ctrl Pts',(6.11945559599994,11.6,9.01400513499999));
#211021=CARTESIAN_POINT('Ctrl Pts',(6.11718639499994,15.2,9.01226834599999));
#211022=CARTESIAN_POINT('Ctrl Pts',(6.11718639499994,11.6,9.01226834599999));
#211023=CARTESIAN_POINT('Ctrl Pts',(6.11492308999994,15.2,9.01053308099998));
#211024=CARTESIAN_POINT('Ctrl Pts',(6.11492308999994,11.6,9.01053308099998));
#211025=CARTESIAN_POINT('Ctrl Pts',(6.11266567999994,15.2,9.00879935599999));
#211026=CARTESIAN_POINT('Ctrl Pts',(6.11266567999994,11.6,9.00879935599999));
#211027=CARTESIAN_POINT('Ctrl Pts',(6.11041416999995,15.2,9.00706718099999));
#211028=CARTESIAN_POINT('Ctrl Pts',(6.11041416999995,11.6,9.00706718099999));
#211029=CARTESIAN_POINT('Ctrl Pts',(6.10816856499994,15.2,9.00533656899999));
#211030=CARTESIAN_POINT('Ctrl Pts',(6.10816856499994,11.6,9.00533656899999));
#211031=CARTESIAN_POINT('Ctrl Pts',(6.10592886499994,15.2,9.00360753399998));
#211032=CARTESIAN_POINT('Ctrl Pts',(6.10592886499994,11.6,9.00360753399998));
#211033=CARTESIAN_POINT('Ctrl Pts',(6.10369507599994,15.2,9.00188008699999));
#211034=CARTESIAN_POINT('Ctrl Pts',(6.10369507599994,11.6,9.00188008699999));
#211035=CARTESIAN_POINT('Ctrl Pts',(6.10146719899994,15.2,9.00015424299998));
#211036=CARTESIAN_POINT('Ctrl Pts',(6.10146719899994,11.6,9.00015424299998));
#211037=CARTESIAN_POINT('Ctrl Pts',(6.09924523799994,15.2,8.99843001299999));
#211038=CARTESIAN_POINT('Ctrl Pts',(6.09924523799994,11.6,8.99843001299999));
#211039=CARTESIAN_POINT('Ctrl Pts',(6.09702919599994,15.2,8.99670740999999));
#211040=CARTESIAN_POINT('Ctrl Pts',(6.09702919599994,11.6,8.99670740999999));
#211041=CARTESIAN_POINT('Ctrl Pts',(6.09481907699994,15.2,8.99498644799999));
#211042=CARTESIAN_POINT('Ctrl Pts',(6.09481907699994,11.6,8.99498644799999));
#211043=CARTESIAN_POINT('Ctrl Pts',(6.09261488399994,15.2,8.99326713799999));
#211044=CARTESIAN_POINT('Ctrl Pts',(6.09261488399994,11.6,8.99326713799999));
#211045=CARTESIAN_POINT('Ctrl Pts',(6.09041661899994,15.2,8.99154949399998));
#211046=CARTESIAN_POINT('Ctrl Pts',(6.09041661899994,11.6,8.99154949399998));
#211047=CARTESIAN_POINT('Ctrl Pts',(6.08822428599994,15.2,8.98983352999998));
#211048=CARTESIAN_POINT('Ctrl Pts',(6.08822428599994,11.6,8.98983352999998));
#211049=CARTESIAN_POINT('Ctrl Pts',(6.08603788899994,15.2,8.98811925799999));
#211050=CARTESIAN_POINT('Ctrl Pts',(6.08603788899994,11.6,8.98811925799999));
#211051=CARTESIAN_POINT('Ctrl Pts',(6.08385742999994,15.2,8.98640669099999));
#211052=CARTESIAN_POINT('Ctrl Pts',(6.08385742999994,11.6,8.98640669099999));
#211053=CARTESIAN_POINT('Ctrl Pts',(6.08168291099994,15.2,8.98469584199999));
#211054=CARTESIAN_POINT('Ctrl Pts',(6.08168291099994,11.6,8.98469584199999));
#211055=CARTESIAN_POINT('Ctrl Pts',(6.07951433799995,15.2,8.98298672299998));
#211056=CARTESIAN_POINT('Ctrl Pts',(6.07951433799995,11.6,8.98298672299998));
#211057=CARTESIAN_POINT('Ctrl Pts',(6.07735171299994,15.2,8.98127934999999));
#211058=CARTESIAN_POINT('Ctrl Pts',(6.07735171299994,11.6,8.98127934999999));
#211059=CARTESIAN_POINT('Ctrl Pts',(6.07519503899994,15.2,8.97957373399999));
#211060=CARTESIAN_POINT('Ctrl Pts',(6.07519503899994,11.6,8.97957373399999));
#211061=CARTESIAN_POINT('Ctrl Pts',(6.07304431899995,15.2,8.97786988899998));
#211062=CARTESIAN_POINT('Ctrl Pts',(6.07304431899995,11.6,8.97786988899998));
#211063=CARTESIAN_POINT('Ctrl Pts',(6.07089955599994,15.2,8.97616782699998));
#211064=CARTESIAN_POINT('Ctrl Pts',(6.07089955599994,11.6,8.97616782699998));
#211065=CARTESIAN_POINT('Ctrl Pts',(6.06876075399994,15.2,8.97446756299999));
#211066=CARTESIAN_POINT('Ctrl Pts',(6.06876075399994,11.6,8.97446756299999));
#211067=CARTESIAN_POINT('Ctrl Pts',(6.06662791499994,15.2,8.97276910999998));
#211068=CARTESIAN_POINT('Ctrl Pts',(6.06662791499994,11.6,8.97276910999998));
#211069=CARTESIAN_POINT('Ctrl Pts',(6.06450104399994,15.2,8.97107248099999));
#211070=CARTESIAN_POINT('Ctrl Pts',(6.06450104399994,11.6,8.97107248099999));
#211071=CARTESIAN_POINT('Ctrl Pts',(6.06238014199994,15.2,8.96937768799998));
#211072=CARTESIAN_POINT('Ctrl Pts',(6.06238014199994,11.6,8.96937768799998));
#211073=CARTESIAN_POINT('Ctrl Pts',(6.06026521299994,15.2,8.96768474699999));
#211074=CARTESIAN_POINT('Ctrl Pts',(6.06026521299994,11.6,8.96768474699999));
#211075=CARTESIAN_POINT('Ctrl Pts',(6.05815626099994,15.2,8.96599366899999));
#211076=CARTESIAN_POINT('Ctrl Pts',(6.05815626099994,11.6,8.96599366899999));
#211077=CARTESIAN_POINT('Ctrl Pts',(6.05605328699995,15.2,8.96430446999998));
#211078=CARTESIAN_POINT('Ctrl Pts',(6.05605328699995,11.6,8.96430446999998));
#211079=CARTESIAN_POINT('Ctrl Pts',(6.05395629799994,15.2,8.96261716199999));
#211080=CARTESIAN_POINT('Ctrl Pts',(6.05395629799994,11.6,8.96261716199999));
#211081=CARTESIAN_POINT('Ctrl Pts',(6.05186529299995,15.2,8.96093175899999));
#211082=CARTESIAN_POINT('Ctrl Pts',(6.05186529299995,11.6,8.96093175899999));
#211083=CARTESIAN_POINT('Ctrl Pts',(6.04978027699994,15.2,8.95924827399998));
#211084=CARTESIAN_POINT('Ctrl Pts',(6.04978027699994,11.6,8.95924827399998));
#211085=CARTESIAN_POINT('Ctrl Pts',(6.04770125299994,15.2,8.95756672099999));
#211086=CARTESIAN_POINT('Ctrl Pts',(6.04770125299994,11.6,8.95756672099999));
#211087=CARTESIAN_POINT('Ctrl Pts',(6.04562822499994,15.2,8.95588711399999));
#211088=CARTESIAN_POINT('Ctrl Pts',(6.04562822499994,11.6,8.95588711399999));
#211089=CARTESIAN_POINT('Ctrl Pts',(6.04356119499994,15.2,8.95420946599998));
#211090=CARTESIAN_POINT('Ctrl Pts',(6.04356119499994,11.6,8.95420946599998));
#211091=CARTESIAN_POINT('Ctrl Pts',(6.04150016599994,15.2,8.95253379199998));
#211092=CARTESIAN_POINT('Ctrl Pts',(6.04150016599994,11.6,8.95253379199998));
#211093=CARTESIAN_POINT('Ctrl Pts',(6.03944514199994,15.2,8.95086010499998));
#211094=CARTESIAN_POINT('Ctrl Pts',(6.03944514199994,11.6,8.95086010499998));
#211095=CARTESIAN_POINT('Ctrl Pts',(6.03739612599994,15.2,8.94918841899998));
#211096=CARTESIAN_POINT('Ctrl Pts',(6.03739612599994,11.6,8.94918841899998));
#211097=CARTESIAN_POINT('Ctrl Pts',(6.03535311999994,15.2,8.94751874799999));
#211098=CARTESIAN_POINT('Ctrl Pts',(6.03535311999994,11.6,8.94751874799999));
#211099=CARTESIAN_POINT('Ctrl Pts',(6.03331612799994,15.2,8.94585110499998));
#211100=CARTESIAN_POINT('Ctrl Pts',(6.03331612799994,11.6,8.94585110499998));
#211101=CARTESIAN_POINT('Ctrl Pts',(6.03128515299994,15.2,8.94418550499999));
#211102=CARTESIAN_POINT('Ctrl Pts',(6.03128515299994,11.6,8.94418550499999));
#211103=CARTESIAN_POINT('Ctrl Pts',(6.02926019899994,15.2,8.94252196099998));
#211104=CARTESIAN_POINT('Ctrl Pts',(6.02926019899994,11.6,8.94252196099998));
#211105=CARTESIAN_POINT('Ctrl Pts',(6.02724126899994,15.2,8.94086048899998));
#211106=CARTESIAN_POINT('Ctrl Pts',(6.02724126899994,11.6,8.94086048899998));
#211107=CARTESIAN_POINT('Ctrl Pts',(6.02522836399994,15.2,8.93920110099998));
#211108=CARTESIAN_POINT('Ctrl Pts',(6.02522836399994,11.6,8.93920110099998));
#211109=CARTESIAN_POINT('Ctrl Pts',(6.02322148899994,15.2,8.93754381099999));
#211110=CARTESIAN_POINT('Ctrl Pts',(6.02322148899994,11.6,8.93754381099999));
#211111=CARTESIAN_POINT('Ctrl Pts',(6.02122064699994,15.2,8.93588863499998));
#211112=CARTESIAN_POINT('Ctrl Pts',(6.02122064699994,11.6,8.93588863499998));
#211113=CARTESIAN_POINT('Ctrl Pts',(6.01922584099994,15.2,8.93423558599999));
#211114=CARTESIAN_POINT('Ctrl Pts',(6.01922584099994,11.6,8.93423558599999));
#211115=CARTESIAN_POINT('Ctrl Pts',(6.01723707399994,15.2,8.93258467799999));
#211116=CARTESIAN_POINT('Ctrl Pts',(6.01723707399994,11.6,8.93258467799999));
#211117=CARTESIAN_POINT('Ctrl Pts',(6.01525434799994,15.2,8.93093592599998));
#211118=CARTESIAN_POINT('Ctrl Pts',(6.01525434799994,11.6,8.93093592599998));
#211119=CARTESIAN_POINT('Ctrl Pts',(6.01327766799994,15.2,8.92928934399999));
#211120=CARTESIAN_POINT('Ctrl Pts',(6.01327766799994,11.6,8.92928934399999));
#211121=CARTESIAN_POINT('Ctrl Pts',(6.01130703699994,15.2,8.92764494699998));
#211122=CARTESIAN_POINT('Ctrl Pts',(6.01130703699994,11.6,8.92764494699998));
#211123=CARTESIAN_POINT('Ctrl Pts',(6.00934245599994,15.2,8.92600274699999));
#211124=CARTESIAN_POINT('Ctrl Pts',(6.00934245599994,11.6,8.92600274699999));
#211125=CARTESIAN_POINT('Ctrl Pts',(6.00738392999994,15.2,8.92436276099998));
#211126=CARTESIAN_POINT('Ctrl Pts',(6.00738392999994,11.6,8.92436276099998));
#211127=CARTESIAN_POINT('Ctrl Pts',(6.00543146199994,15.2,8.92272500299999));
#211128=CARTESIAN_POINT('Ctrl Pts',(6.00543146199994,11.6,8.92272500299999));
#211129=CARTESIAN_POINT('Ctrl Pts',(6.00348505499994,15.2,8.92108948699999));
#211130=CARTESIAN_POINT('Ctrl Pts',(6.00348505499994,11.6,8.92108948699999));
#211131=CARTESIAN_POINT('Ctrl Pts',(6.00154470999994,15.2,8.91945622799999));
#211132=CARTESIAN_POINT('Ctrl Pts',(6.00154470999994,11.6,8.91945622799999));
#211133=CARTESIAN_POINT('Ctrl Pts',(5.99961043399994,15.2,8.91782523899998));
#211134=CARTESIAN_POINT('Ctrl Pts',(5.99961043399994,11.6,8.91782523899998));
#211135=CARTESIAN_POINT('Ctrl Pts',(5.99768222699995,15.2,8.91619653699999));
#211136=CARTESIAN_POINT('Ctrl Pts',(5.99768222699995,11.6,8.91619653699999));
#211137=CARTESIAN_POINT('Ctrl Pts',(5.99576009299994,15.2,8.91457013599998));
#211138=CARTESIAN_POINT('Ctrl Pts',(5.99576009299994,11.6,8.91457013599998));
#211139=CARTESIAN_POINT('Ctrl Pts',(5.99384403599994,15.2,8.91294604999998));
#211140=CARTESIAN_POINT('Ctrl Pts',(5.99384403599994,11.6,8.91294604999998));
#211141=CARTESIAN_POINT('Ctrl Pts',(5.99193405699994,15.2,8.91132429299999));
#211142=CARTESIAN_POINT('Ctrl Pts',(5.99193405699994,11.6,8.91132429299999));
#211143=CARTESIAN_POINT('Ctrl Pts',(5.99003016199994,15.2,8.90970488199999));
#211144=CARTESIAN_POINT('Ctrl Pts',(5.99003016199994,11.6,8.90970488199999));
#211145=CARTESIAN_POINT('Ctrl Pts',(5.98813235099994,15.2,8.90808782999999));
#211146=CARTESIAN_POINT('Ctrl Pts',(5.98813235099994,11.6,8.90808782999999));
#211147=CARTESIAN_POINT('Ctrl Pts',(5.98624062899995,15.2,8.90647315299999));
#211148=CARTESIAN_POINT('Ctrl Pts',(5.98624062899995,11.6,8.90647315299999));
#211149=CARTESIAN_POINT('Ctrl Pts',(5.98435499899994,15.2,8.90486086599999));
#211150=CARTESIAN_POINT('Ctrl Pts',(5.98435499899994,11.6,8.90486086599999));
#211151=CARTESIAN_POINT('Ctrl Pts',(5.98247546299995,15.2,8.90325098299999));
#211152=CARTESIAN_POINT('Ctrl Pts',(5.98247546299995,11.6,8.90325098299999));
#211153=CARTESIAN_POINT('Ctrl Pts',(5.98060202599994,15.2,8.90164351999999));
#211154=CARTESIAN_POINT('Ctrl Pts',(5.98060202599994,11.6,8.90164351999999));
#211155=CARTESIAN_POINT('Ctrl Pts',(5.97873468799994,15.2,8.90003849199999));
#211156=CARTESIAN_POINT('Ctrl Pts',(5.97873468799994,11.6,8.90003849199999));
#211157=CARTESIAN_POINT('Ctrl Pts',(5.97687345599994,15.2,8.89843591199998));
#211158=CARTESIAN_POINT('Ctrl Pts',(5.97687345599994,11.6,8.89843591199998));
#211159=CARTESIAN_POINT('Ctrl Pts',(5.97501832899995,15.2,8.89683579899998));
#211160=CARTESIAN_POINT('Ctrl Pts',(5.97501832899995,11.6,8.89683579899998));
#211161=CARTESIAN_POINT('Ctrl Pts',(5.97316931399994,15.2,8.89523816499998));
#211162=CARTESIAN_POINT('Ctrl Pts',(5.97316931399994,11.6,8.89523816499998));
#211163=CARTESIAN_POINT('Ctrl Pts',(5.97132640999994,15.2,8.89364302699999));
#211164=CARTESIAN_POINT('Ctrl Pts',(5.97132640999994,11.6,8.89364302699999));
#211165=CARTESIAN_POINT('Ctrl Pts',(5.96948962499994,15.2,8.89205039899998));
#211166=CARTESIAN_POINT('Ctrl Pts',(5.96948962499994,11.6,8.89205039899998));
#211167=CARTESIAN_POINT('Ctrl Pts',(5.96765895599994,15.2,8.89046029799999));
#211168=CARTESIAN_POINT('Ctrl Pts',(5.96765895599994,11.6,8.89046029799999));
#211169=CARTESIAN_POINT('Ctrl Pts',(5.96583441199994,15.2,8.88887273699999));
#211170=CARTESIAN_POINT('Ctrl Pts',(5.96583441199994,11.6,8.88887273699999));
#211171=CARTESIAN_POINT('Ctrl Pts',(5.96401599199995,15.2,8.88728773299999));
#211172=CARTESIAN_POINT('Ctrl Pts',(5.96401599199995,11.6,8.88728773299999));
#211173=CARTESIAN_POINT('Ctrl Pts',(5.96220370099994,15.2,8.88570530199999));
#211174=CARTESIAN_POINT('Ctrl Pts',(5.96220370099994,11.6,8.88570530199999));
#211175=CARTESIAN_POINT('Ctrl Pts',(5.96039754099994,15.2,8.88412545899998));
#211176=CARTESIAN_POINT('Ctrl Pts',(5.96039754099994,11.6,8.88412545899998));
#211177=CARTESIAN_POINT('Ctrl Pts',(5.95859751599994,15.2,8.88254821899999));
#211178=CARTESIAN_POINT('Ctrl Pts',(5.95859751599994,11.6,8.88254821899999));
#211179=CARTESIAN_POINT('Ctrl Pts',(5.95680362799994,15.2,8.88097359799998));
#211180=CARTESIAN_POINT('Ctrl Pts',(5.95680362799994,11.6,8.88097359799998));
#211181=CARTESIAN_POINT('Ctrl Pts',(5.95501588199995,15.2,8.87940161199998));
#211182=CARTESIAN_POINT('Ctrl Pts',(5.95501588199995,11.6,8.87940161199998));
#211183=CARTESIAN_POINT('Ctrl Pts',(5.95323427899994,15.2,8.87783227599999));
#211184=CARTESIAN_POINT('Ctrl Pts',(5.95323427899994,11.6,8.87783227599999));
#211185=CARTESIAN_POINT('Ctrl Pts',(5.95145882199994,15.2,8.87626560599998));
#211186=CARTESIAN_POINT('Ctrl Pts',(5.95145882199994,11.6,8.87626560599998));
#211187=CARTESIAN_POINT('Ctrl Pts',(5.94968951499995,15.2,8.87470161799998));
#211188=CARTESIAN_POINT('Ctrl Pts',(5.94968951499995,11.6,8.87470161799998));
#211189=CARTESIAN_POINT('Ctrl Pts',(5.94792636199994,15.2,8.87314032899998));
#211190=CARTESIAN_POINT('Ctrl Pts',(5.94792636199994,11.6,8.87314032899998));
#211191=CARTESIAN_POINT('Ctrl Pts',(5.94616936399994,15.2,8.87158175299999));
#211192=CARTESIAN_POINT('Ctrl Pts',(5.94616936399994,11.6,8.87158175299999));
#211193=CARTESIAN_POINT('Ctrl Pts',(5.94441852499994,15.2,8.87002590499998));
#211194=CARTESIAN_POINT('Ctrl Pts',(5.94441852499994,11.6,8.87002590499998));
#211195=CARTESIAN_POINT('Ctrl Pts',(5.94267384799994,15.2,8.86847280399999));
#211196=CARTESIAN_POINT('Ctrl Pts',(5.94267384799994,11.6,8.86847280399999));
#211197=CARTESIAN_POINT('Ctrl Pts',(5.94093533599994,15.2,8.86692246499998));
#211198=CARTESIAN_POINT('Ctrl Pts',(5.94093533599994,11.6,8.86692246499998));
#211199=CARTESIAN_POINT('Ctrl Pts',(5.93920299199994,15.2,8.86537490399999));
#211200=CARTESIAN_POINT('Ctrl Pts',(5.93920299199994,11.6,8.86537490399999));
#211201=CARTESIAN_POINT('Ctrl Pts',(5.93747681899995,15.2,8.86383013699999));
#211202=CARTESIAN_POINT('Ctrl Pts',(5.93747681899995,11.6,8.86383013699999));
#211203=CARTESIAN_POINT('Ctrl Pts',(5.93575681999994,15.2,8.86228817899998));
#211204=CARTESIAN_POINT('Ctrl Pts',(5.93575681999994,11.6,8.86228817899998));
#211205=CARTESIAN_POINT('Ctrl Pts',(5.93404299799994,15.2,8.86074904799998));
#211206=CARTESIAN_POINT('Ctrl Pts',(5.93404299799994,11.6,8.86074904799998));
#211207=CARTESIAN_POINT('Ctrl Pts',(5.93233535699994,15.2,8.85921275999999));
#211208=CARTESIAN_POINT('Ctrl Pts',(5.93233535699994,11.6,8.85921275999999));
#211209=CARTESIAN_POINT('Ctrl Pts',(5.93063389799994,15.2,8.85767933099999));
#211210=CARTESIAN_POINT('Ctrl Pts',(5.93063389799994,11.6,8.85767933099999));
#211211=CARTESIAN_POINT('Ctrl Pts',(5.92893862599994,15.2,8.85614877699999));
#211212=CARTESIAN_POINT('Ctrl Pts',(5.92893862599994,11.6,8.85614877699999));
#211213=CARTESIAN_POINT('Ctrl Pts',(5.92724954299994,15.2,8.85462111499999));
#211214=CARTESIAN_POINT('Ctrl Pts',(5.92724954299994,11.6,8.85462111499999));
#211215=CARTESIAN_POINT('Ctrl Pts',(5.92556665199995,15.2,8.85309636099999));
#211216=CARTESIAN_POINT('Ctrl Pts',(5.92556665199995,11.6,8.85309636099999));
#211217=CARTESIAN_POINT('Ctrl Pts',(5.92388995599994,15.2,8.85157453299998));
#211218=CARTESIAN_POINT('Ctrl Pts',(5.92388995599994,11.6,8.85157453299998));
#211219=CARTESIAN_POINT('Ctrl Pts',(5.92221945899994,15.2,8.85005564699998));
#211220=CARTESIAN_POINT('Ctrl Pts',(5.92221945899994,11.6,8.85005564699998));
#211221=CARTESIAN_POINT('Ctrl Pts',(5.92055516299995,15.2,8.84853971799998));
#211222=CARTESIAN_POINT('Ctrl Pts',(5.92055516299995,11.6,8.84853971799998));
#211223=CARTESIAN_POINT('Ctrl Pts',(5.91889706999994,15.2,8.84702676499998));
#211224=CARTESIAN_POINT('Ctrl Pts',(5.91889706999994,11.6,8.84702676499998));
#211225=CARTESIAN_POINT('Ctrl Pts',(5.91724518499994,15.2,8.84551680299998));
#211226=CARTESIAN_POINT('Ctrl Pts',(5.91724518499994,11.6,8.84551680299998));
#211227=CARTESIAN_POINT('Ctrl Pts',(5.91559951099994,15.2,8.84400984899998));
#211228=CARTESIAN_POINT('Ctrl Pts',(5.91559951099994,11.6,8.84400984899998));
#211229=CARTESIAN_POINT('Ctrl Pts',(5.91396004999994,15.2,8.84250592099999));
#211230=CARTESIAN_POINT('Ctrl Pts',(5.91396004999994,11.6,8.84250592099999));
#211231=CARTESIAN_POINT('Ctrl Pts',(5.91232680399995,15.2,8.84100503599999));
#211232=CARTESIAN_POINT('Ctrl Pts',(5.91232680399995,11.6,8.84100503599999));
#211233=CARTESIAN_POINT('Ctrl Pts',(5.91069977899994,15.2,8.83950720899998));
#211234=CARTESIAN_POINT('Ctrl Pts',(5.91069977899994,11.6,8.83950720899998));
#211235=CARTESIAN_POINT('Ctrl Pts',(5.90907897499994,15.2,8.83801245899999));
#211236=CARTESIAN_POINT('Ctrl Pts',(5.90907897499994,11.6,8.83801245899999));
#211237=CARTESIAN_POINT('Ctrl Pts',(5.90746439699994,15.2,8.83652080299999));
#211238=CARTESIAN_POINT('Ctrl Pts',(5.90746439699994,11.6,8.83652080299999));
#211239=CARTESIAN_POINT('Ctrl Pts',(5.90585604599994,15.2,8.83503225699998));
#211240=CARTESIAN_POINT('Ctrl Pts',(5.90585604599994,11.6,8.83503225699998));
#211241=CARTESIAN_POINT('Ctrl Pts',(5.90425392799995,15.2,8.83354683899999));
#211242=CARTESIAN_POINT('Ctrl Pts',(5.90425392799995,11.6,8.83354683899999));
#211243=CARTESIAN_POINT('Ctrl Pts',(5.90265804299994,15.2,8.83206456499998));
#211244=CARTESIAN_POINT('Ctrl Pts',(5.90265804299994,11.6,8.83206456499998));
#211245=CARTESIAN_POINT('Ctrl Pts',(5.90106839599994,15.2,8.83058545499999));
#211246=CARTESIAN_POINT('Ctrl Pts',(5.90106839599994,11.6,8.83058545499999));
#211247=CARTESIAN_POINT('Ctrl Pts',(5.89948498799994,15.2,8.82910952399998));
#211248=CARTESIAN_POINT('Ctrl Pts',(5.89948498799994,11.6,8.82910952399998));
#211249=CARTESIAN_POINT('Ctrl Pts',(5.89790782399994,15.2,8.82763678999999));
#211250=CARTESIAN_POINT('Ctrl Pts',(5.89790782399994,11.6,8.82763678999999));
#211251=CARTESIAN_POINT('Ctrl Pts',(5.89633690599994,15.2,8.82616727099998));
#211252=CARTESIAN_POINT('Ctrl Pts',(5.89633690599994,11.6,8.82616727099998));
#211253=CARTESIAN_POINT('Ctrl Pts',(5.89477223699994,15.2,8.82470098399999));
#211254=CARTESIAN_POINT('Ctrl Pts',(5.89477223699994,11.6,8.82470098399999));
#211255=CARTESIAN_POINT('Ctrl Pts',(5.89321381999994,15.2,8.82323794699998));
#211256=CARTESIAN_POINT('Ctrl Pts',(5.89321381999994,11.6,8.82323794699998));
#211257=CARTESIAN_POINT('Ctrl Pts',(5.89166165899995,15.2,8.82177817599998));
#211258=CARTESIAN_POINT('Ctrl Pts',(5.89166165899995,11.6,8.82177817599998));
#211259=CARTESIAN_POINT('Ctrl Pts',(5.89011575399994,15.2,8.82032169099999));
#211260=CARTESIAN_POINT('Ctrl Pts',(5.89011575399994,11.6,8.82032169099999));
#211261=CARTESIAN_POINT('Ctrl Pts',(5.88857611199994,15.2,8.81886850999998));
#211262=CARTESIAN_POINT('Ctrl Pts',(5.88857611199994,11.6,8.81886850999998));
#211263=CARTESIAN_POINT('Ctrl Pts',(5.88704273199995,15.2,8.81741864899999));
#211264=CARTESIAN_POINT('Ctrl Pts',(5.88704273199995,11.6,8.81741864899999));
#211265=CARTESIAN_POINT('Ctrl Pts',(5.88551561999994,15.2,8.81597212599999));
#211266=CARTESIAN_POINT('Ctrl Pts',(5.88551561999994,11.6,8.81597212599999));
#211267=CARTESIAN_POINT('Ctrl Pts',(5.88399477899994,15.2,8.81452895999999));
#211268=CARTESIAN_POINT('Ctrl Pts',(5.88399477899994,11.6,8.81452895999999));
#211269=CARTESIAN_POINT('Ctrl Pts',(5.88248020899995,15.2,8.81308916799998));
#211270=CARTESIAN_POINT('Ctrl Pts',(5.88248020899995,11.6,8.81308916799998));
#211271=CARTESIAN_POINT('Ctrl Pts',(5.88097191599994,15.2,8.81165276999998));
#211272=CARTESIAN_POINT('Ctrl Pts',(5.88097191599994,11.6,8.81165276999998));
#211273=CARTESIAN_POINT('Ctrl Pts',(5.87946990099995,15.2,8.81021978199998));
#211274=CARTESIAN_POINT('Ctrl Pts',(5.87946990099995,11.6,8.81021978199998));
#211275=CARTESIAN_POINT('Ctrl Pts',(5.87797416699994,15.2,8.80879022299998));
#211276=CARTESIAN_POINT('Ctrl Pts',(5.87797416699994,11.6,8.80879022299998));
#211277=CARTESIAN_POINT('Ctrl Pts',(5.87648471999994,15.2,8.80736411099999));
#211278=CARTESIAN_POINT('Ctrl Pts',(5.87648471999994,11.6,8.80736411099999));
#211279=CARTESIAN_POINT('Ctrl Pts',(5.87500155899994,15.2,8.80594146499998));
#211280=CARTESIAN_POINT('Ctrl Pts',(5.87500155899994,11.6,8.80594146499998));
#211281=CARTESIAN_POINT('Ctrl Pts',(5.87352468899994,15.2,8.80452230299999));
#211282=CARTESIAN_POINT('Ctrl Pts',(5.87352468899994,11.6,8.80452230299999));
#211283=CARTESIAN_POINT('Ctrl Pts',(5.87205411099994,15.2,8.80310664299999));
#211284=CARTESIAN_POINT('Ctrl Pts',(5.87205411099994,11.6,8.80310664299999));
#211285=CARTESIAN_POINT('Ctrl Pts',(5.87058983199994,15.2,8.80169450299999));
#211286=CARTESIAN_POINT('Ctrl Pts',(5.87058983199994,11.6,8.80169450299999));
#211287=CARTESIAN_POINT('Ctrl Pts',(5.86913184999994,15.2,8.80028590299998));
#211288=CARTESIAN_POINT('Ctrl Pts',(5.86913184999994,11.6,8.80028590299998));
#211289=CARTESIAN_POINT('Ctrl Pts',(5.86768017199994,15.2,8.79888086199998));
#211290=CARTESIAN_POINT('Ctrl Pts',(5.86768017199994,11.6,8.79888086199998));
#211291=CARTESIAN_POINT('Ctrl Pts',(5.86623479799995,15.2,8.79747939699998));
#211292=CARTESIAN_POINT('Ctrl Pts',(5.86623479799995,11.6,8.79747939699998));
#211293=CARTESIAN_POINT('Ctrl Pts',(5.86479573299994,15.2,8.79608152699999));
#211294=CARTESIAN_POINT('Ctrl Pts',(5.86479573299994,11.6,8.79608152699999));
#211295=CARTESIAN_POINT('Ctrl Pts',(5.86336297799994,15.2,8.79468727199999));
#211296=CARTESIAN_POINT('Ctrl Pts',(5.86336297799994,11.6,8.79468727199999));
#211297=CARTESIAN_POINT('Ctrl Pts',(5.86193653799994,15.2,8.79329664999998));
#211298=CARTESIAN_POINT('Ctrl Pts',(5.86193653799994,11.6,8.79329664999998));
#211299=CARTESIAN_POINT('Ctrl Pts',(5.86051641599994,15.2,8.79190967999998));
#211300=CARTESIAN_POINT('Ctrl Pts',(5.86051641599994,11.6,8.79190967999998));
#211301=CARTESIAN_POINT('Ctrl Pts',(5.85910261199994,15.2,8.79052638199998));
#211302=CARTESIAN_POINT('Ctrl Pts',(5.85910261199994,11.6,8.79052638199998));
#211303=CARTESIAN_POINT('Ctrl Pts',(5.85769513199994,15.2,8.78914677199998));
#211304=CARTESIAN_POINT('Ctrl Pts',(5.85769513199994,11.6,8.78914677199998));
#211305=CARTESIAN_POINT('Ctrl Pts',(5.85629397699994,15.2,8.78777087299999));
#211306=CARTESIAN_POINT('Ctrl Pts',(5.85629397699994,11.6,8.78777087299999));
#211307=CARTESIAN_POINT('Ctrl Pts',(5.85489915099994,15.2,8.78639870299999));
#211308=CARTESIAN_POINT('Ctrl Pts',(5.85489915099994,11.6,8.78639870299999));
#211309=CARTESIAN_POINT('Ctrl Pts',(5.85351065599995,15.2,8.78503028099999));
#211310=CARTESIAN_POINT('Ctrl Pts',(5.85351065599995,11.6,8.78503028099999));
#211311=CARTESIAN_POINT('Ctrl Pts',(5.85212849599994,15.2,8.78366562499998));
#211312=CARTESIAN_POINT('Ctrl Pts',(5.85212849599994,11.6,8.78366562499998));
#211313=CARTESIAN_POINT('Ctrl Pts',(5.85075267399994,15.2,8.78230475599998));
#211314=CARTESIAN_POINT('Ctrl Pts',(5.85075267399994,11.6,8.78230475599998));
#211315=CARTESIAN_POINT('Ctrl Pts',(5.84938319199994,15.2,8.78094769299998));
#211316=CARTESIAN_POINT('Ctrl Pts',(5.84938319199994,11.6,8.78094769299998));
#211317=CARTESIAN_POINT('Ctrl Pts',(5.84802005299994,15.2,8.77959445599998));
#211318=CARTESIAN_POINT('Ctrl Pts',(5.84802005299994,11.6,8.77959445599998));
#211319=CARTESIAN_POINT('Ctrl Pts',(5.84666325999994,15.2,8.77824506499999));
#211320=CARTESIAN_POINT('Ctrl Pts',(5.84666325999994,11.6,8.77824506499999));
#211321=CARTESIAN_POINT('Ctrl Pts',(5.84531281599994,15.2,8.77689953899999));
#211322=CARTESIAN_POINT('Ctrl Pts',(5.84531281599994,11.6,8.77689953899999));
#211323=CARTESIAN_POINT('Ctrl Pts',(5.84396872499994,15.2,8.77555789599998));
#211324=CARTESIAN_POINT('Ctrl Pts',(5.84396872499994,11.6,8.77555789599998));
#211325=CARTESIAN_POINT('Ctrl Pts',(5.84263098699994,15.2,8.77422015899998));
#211326=CARTESIAN_POINT('Ctrl Pts',(5.84263098699994,11.6,8.77422015899998));
#211327=CARTESIAN_POINT('Ctrl Pts',(5.84129960799994,15.2,8.77288634599999));
#211328=CARTESIAN_POINT('Ctrl Pts',(5.84129960799994,11.6,8.77288634599999));
#211329=CARTESIAN_POINT('Ctrl Pts',(5.83997458899995,15.2,8.77155647799999));
#211330=CARTESIAN_POINT('Ctrl Pts',(5.83997458899995,11.6,8.77155647799999));
#211331=CARTESIAN_POINT('Ctrl Pts',(5.83865593499994,15.2,8.77023057399999));
#211332=CARTESIAN_POINT('Ctrl Pts',(5.83865593499994,11.6,8.77023057399999));
#211333=CARTESIAN_POINT('Ctrl Pts',(5.83734364599994,15.2,8.76890865499998));
#211334=CARTESIAN_POINT('Ctrl Pts',(5.83734364599994,11.6,8.76890865499998));
#211335=CARTESIAN_POINT('Ctrl Pts',(5.83603772599995,15.2,8.76759074099999));
#211336=CARTESIAN_POINT('Ctrl Pts',(5.83603772599995,11.6,8.76759074099999));
#211337=CARTESIAN_POINT('Ctrl Pts',(5.83473817899995,15.2,8.76627685199999));
#211338=CARTESIAN_POINT('Ctrl Pts',(5.83473817899995,11.6,8.76627685199999));
#211339=CARTESIAN_POINT('Ctrl Pts',(5.83344500599994,15.2,8.76496700899999));
#211340=CARTESIAN_POINT('Ctrl Pts',(5.83344500599994,11.6,8.76496700899999));
#211341=CARTESIAN_POINT('Ctrl Pts',(5.83215821299994,15.2,8.76366122999999));
#211342=CARTESIAN_POINT('Ctrl Pts',(5.83215821299994,11.6,8.76366122999999));
#211343=CARTESIAN_POINT('Ctrl Pts',(5.83087779899994,15.2,8.76235953999998));
#211344=CARTESIAN_POINT('Ctrl Pts',(5.83087779899994,11.6,8.76235953999998));
#211345=CARTESIAN_POINT('Ctrl Pts',(5.82960376999995,15.2,8.76106195499998));
#211346=CARTESIAN_POINT('Ctrl Pts',(5.82960376999995,11.6,8.76106195499998));
#211347=CARTESIAN_POINT('Ctrl Pts',(5.82833612699994,15.2,8.75976849799999));
#211348=CARTESIAN_POINT('Ctrl Pts',(5.82833612699994,11.6,8.75976849799999));
#211349=CARTESIAN_POINT('Ctrl Pts',(5.82707487299994,15.2,8.75847918999998));
#211350=CARTESIAN_POINT('Ctrl Pts',(5.82707487299994,11.6,8.75847918999998));
#211351=CARTESIAN_POINT('Ctrl Pts',(5.82582001199994,15.2,8.75719405099998));
#211352=CARTESIAN_POINT('Ctrl Pts',(5.82582001199994,11.6,8.75719405099998));
#211353=CARTESIAN_POINT('Ctrl Pts',(5.82457154599994,15.2,8.75591310099999));
#211354=CARTESIAN_POINT('Ctrl Pts',(5.82457154599994,11.6,8.75591310099999));
#211355=CARTESIAN_POINT('Ctrl Pts',(5.82332947799994,15.2,8.75463636299998));
#211356=CARTESIAN_POINT('Ctrl Pts',(5.82332947799994,11.6,8.75463636299998));
#211357=CARTESIAN_POINT('Ctrl Pts',(5.82209381199994,15.2,8.75336385699999));
#211358=CARTESIAN_POINT('Ctrl Pts',(5.82209381199994,11.6,8.75336385699999));
#211359=CARTESIAN_POINT('Ctrl Pts',(5.82086454899994,15.2,8.75209560299999));
#211360=CARTESIAN_POINT('Ctrl Pts',(5.82086454899994,11.6,8.75209560299999));
#211361=CARTESIAN_POINT('Ctrl Pts',(5.81964169299994,15.2,8.75083162499998));
#211362=CARTESIAN_POINT('Ctrl Pts',(5.81964169299994,11.6,8.75083162499998));
#211363=CARTESIAN_POINT('Ctrl Pts',(5.81842524599995,15.2,8.74957194099999));
#211364=CARTESIAN_POINT('Ctrl Pts',(5.81842524599995,11.6,8.74957194099999));
#211365=CARTESIAN_POINT('Ctrl Pts',(5.81721521199994,15.2,8.74831657499998));
#211366=CARTESIAN_POINT('Ctrl Pts',(5.81721521199994,11.6,8.74831657499998));
#211367=CARTESIAN_POINT('Ctrl Pts',(5.81601159299994,15.2,8.74706554699999));
#211368=CARTESIAN_POINT('Ctrl Pts',(5.81601159299994,11.6,8.74706554699999));
#211369=CARTESIAN_POINT('Ctrl Pts',(5.81481439199995,15.2,8.74581887799999));
#211370=CARTESIAN_POINT('Ctrl Pts',(5.81481439199995,11.6,8.74581887799999));
#211371=CARTESIAN_POINT('Ctrl Pts',(5.81362361299995,15.2,8.74457659099999));
#211372=CARTESIAN_POINT('Ctrl Pts',(5.81362361299995,11.6,8.74457659099999));
#211373=CARTESIAN_POINT('Ctrl Pts',(5.81243925699994,15.2,8.74333870699999));
#211374=CARTESIAN_POINT('Ctrl Pts',(5.81243925699994,11.6,8.74333870699999));
#211375=CARTESIAN_POINT('Ctrl Pts',(5.81126132699994,15.2,8.74210524899999));
#211376=CARTESIAN_POINT('Ctrl Pts',(5.81126132699994,11.6,8.74210524899999));
#211377=CARTESIAN_POINT('Ctrl Pts',(5.81008982699994,15.2,8.74087623599999));
#211378=CARTESIAN_POINT('Ctrl Pts',(5.81008982699994,11.6,8.74087623599999));
#211379=CARTESIAN_POINT('Ctrl Pts',(5.80892475999994,15.2,8.73965169199998));
#211380=CARTESIAN_POINT('Ctrl Pts',(5.80892475999994,11.6,8.73965169199998));
#211381=CARTESIAN_POINT('Ctrl Pts',(5.80776612699994,15.2,8.73843163899998));
#211382=CARTESIAN_POINT('Ctrl Pts',(5.80776612699994,11.6,8.73843163899998));
#211383=CARTESIAN_POINT('Ctrl Pts',(5.80661393399994,15.2,8.73721609899999));
#211384=CARTESIAN_POINT('Ctrl Pts',(5.80661393399994,11.6,8.73721609899999));
#211385=CARTESIAN_POINT('Ctrl Pts',(5.80546818099994,15.2,8.73600509399999));
#211386=CARTESIAN_POINT('Ctrl Pts',(5.80546818099994,11.6,8.73600509399999));
#211387=CARTESIAN_POINT('Ctrl Pts',(5.80432887199994,15.2,8.73479864499998));
#211388=CARTESIAN_POINT('Ctrl Pts',(5.80432887199994,11.6,8.73479864499998));
#211389=CARTESIAN_POINT('Ctrl Pts',(5.80319600899994,15.2,8.73359677599998));
#211390=CARTESIAN_POINT('Ctrl Pts',(5.80319600899994,11.6,8.73359677599998));
#211391=CARTESIAN_POINT('Ctrl Pts',(5.80206959599994,15.2,8.73239950899999));
#211392=CARTESIAN_POINT('Ctrl Pts',(5.80206959599994,11.6,8.73239950899999));
#211393=CARTESIAN_POINT('Ctrl Pts',(5.80094963499994,15.2,8.73120686599999));
#211394=CARTESIAN_POINT('Ctrl Pts',(5.80094963499994,11.6,8.73120686599999));
#211395=CARTESIAN_POINT('Ctrl Pts',(5.79983612799994,15.2,8.73001887099999));
#211396=CARTESIAN_POINT('Ctrl Pts',(5.79983612799994,11.6,8.73001887099999));
#211397=CARTESIAN_POINT('Ctrl Pts',(5.79872907999994,15.2,8.72883554599999));
#211398=CARTESIAN_POINT('Ctrl Pts',(5.79872907999994,11.6,8.72883554599999));
#211399=CARTESIAN_POINT('Ctrl Pts',(5.79762849299994,15.2,8.72765691299998));
#211400=CARTESIAN_POINT('Ctrl Pts',(5.79762849299994,11.6,8.72765691299998));
#211401=CARTESIAN_POINT('Ctrl Pts',(5.79653436899994,15.2,8.72648299499998));
#211402=CARTESIAN_POINT('Ctrl Pts',(5.79653436899994,11.6,8.72648299499998));
#211403=CARTESIAN_POINT('Ctrl Pts',(5.79544671099995,15.2,8.72531381599998));
#211404=CARTESIAN_POINT('Ctrl Pts',(5.79544671099995,11.6,8.72531381599998));
#211405=CARTESIAN_POINT('Ctrl Pts',(5.79436552299994,15.2,8.72414939899999));
#211406=CARTESIAN_POINT('Ctrl Pts',(5.79436552299994,11.6,8.72414939899999));
#211407=CARTESIAN_POINT('Ctrl Pts',(5.79329080699994,15.2,8.72298976599998));
#211408=CARTESIAN_POINT('Ctrl Pts',(5.79329080699994,11.6,8.72298976599998));
#211409=CARTESIAN_POINT('Ctrl Pts',(5.79222256599994,15.2,8.72183494199999));
#211410=CARTESIAN_POINT('Ctrl Pts',(5.79222256599994,11.6,8.72183494199999));
#211411=CARTESIAN_POINT('Ctrl Pts',(5.79116080199994,15.2,8.72068494799999));
#211412=CARTESIAN_POINT('Ctrl Pts',(5.79116080199994,11.6,8.72068494799999));
#211413=CARTESIAN_POINT('Ctrl Pts',(5.79010551899994,15.2,8.71953980899999));
#211414=CARTESIAN_POINT('Ctrl Pts',(5.79010551899994,11.6,8.71953980899999));
#211415=CARTESIAN_POINT('Ctrl Pts',(5.78905671899995,15.2,8.71839954799999));
#211416=CARTESIAN_POINT('Ctrl Pts',(5.78905671899995,11.6,8.71839954799999));
#211417=CARTESIAN_POINT('Ctrl Pts',(5.78801440499994,15.2,8.71726418999998));
#211418=CARTESIAN_POINT('Ctrl Pts',(5.78801440499994,11.6,8.71726418999998));
#211419=CARTESIAN_POINT('Ctrl Pts',(5.78697857999994,15.2,8.71613375699998));
#211420=CARTESIAN_POINT('Ctrl Pts',(5.78697857999994,11.6,8.71613375699998));
#211421=CARTESIAN_POINT('Ctrl Pts',(5.78594924699994,15.2,8.71500827299998));
#211422=CARTESIAN_POINT('Ctrl Pts',(5.78594924699994,11.6,8.71500827299998));
#211423=CARTESIAN_POINT('Ctrl Pts',(5.78492640799994,15.2,8.71388776199998));
#211424=CARTESIAN_POINT('Ctrl Pts',(5.78492640799994,11.6,8.71388776199998));
#211425=CARTESIAN_POINT('Ctrl Pts',(5.78391006599994,15.2,8.71277224899998));
#211426=CARTESIAN_POINT('Ctrl Pts',(5.78391006599994,11.6,8.71277224899998));
#211427=CARTESIAN_POINT('Ctrl Pts',(5.78290022499995,15.2,8.71166175799999));
#211428=CARTESIAN_POINT('Ctrl Pts',(5.78290022499995,11.6,8.71166175799999));
#211429=CARTESIAN_POINT('Ctrl Pts',(5.78189688599994,15.2,8.71055631299999));
#211430=CARTESIAN_POINT('Ctrl Pts',(5.78189688599994,11.6,8.71055631299999));
#211431=CARTESIAN_POINT('Ctrl Pts',(5.78090005399994,15.2,8.70945593699999));
#211432=CARTESIAN_POINT('Ctrl Pts',(5.78090005399994,11.6,8.70945593699999));
#211433=CARTESIAN_POINT('Ctrl Pts',(5.77990972899994,15.2,8.70836065599999));
#211434=CARTESIAN_POINT('Ctrl Pts',(5.77990972899994,11.6,8.70836065599999));
#211435=CARTESIAN_POINT('Ctrl Pts',(5.77892591699994,15.2,8.70727049299998));
#211436=CARTESIAN_POINT('Ctrl Pts',(5.77892591699994,11.6,8.70727049299998));
#211437=CARTESIAN_POINT('Ctrl Pts',(5.77794861699994,15.2,8.70618547499999));
#211438=CARTESIAN_POINT('Ctrl Pts',(5.77794861699994,11.6,8.70618547499999));
#211439=CARTESIAN_POINT('Ctrl Pts',(5.77697783599994,15.2,8.70510562499998));
#211440=CARTESIAN_POINT('Ctrl Pts',(5.77697783599994,11.6,8.70510562499998));
#211441=CARTESIAN_POINT('Ctrl Pts',(5.77601357299995,15.2,8.70403096699999));
#211442=CARTESIAN_POINT('Ctrl Pts',(5.77601357299995,11.6,8.70403096699999));
#211443=CARTESIAN_POINT('Ctrl Pts',(5.77505583299994,15.2,8.70296152799998));
#211444=CARTESIAN_POINT('Ctrl Pts',(5.77505583299994,11.6,8.70296152799998));
#211445=CARTESIAN_POINT('Ctrl Pts',(5.77410461799994,15.2,8.70189733199998));
#211446=CARTESIAN_POINT('Ctrl Pts',(5.77410461799994,11.6,8.70189733199998));
#211447=CARTESIAN_POINT('Ctrl Pts',(5.77315993099995,15.2,8.70083840499999));
#211448=CARTESIAN_POINT('Ctrl Pts',(5.77315993099995,11.6,8.70083840499999));
#211449=CARTESIAN_POINT('Ctrl Pts',(5.77222177499994,15.2,8.69978477099998));
#211450=CARTESIAN_POINT('Ctrl Pts',(5.77222177499994,11.6,8.69978477099998));
#211451=CARTESIAN_POINT('Ctrl Pts',(5.77129015299994,15.2,8.69873645499998));
#211452=CARTESIAN_POINT('Ctrl Pts',(5.77129015299994,11.6,8.69873645499998));
#211453=CARTESIAN_POINT('Ctrl Pts',(5.77036506699995,15.2,8.69769348399998));
#211454=CARTESIAN_POINT('Ctrl Pts',(5.77036506699995,11.6,8.69769348399998));
#211455=CARTESIAN_POINT('Ctrl Pts',(5.76944651999994,15.2,8.69665588399998));
#211456=CARTESIAN_POINT('Ctrl Pts',(5.76944651999994,11.6,8.69665588399998));
#211457=CARTESIAN_POINT('Ctrl Pts',(5.76853451499994,15.2,8.69562367799999));
#211458=CARTESIAN_POINT('Ctrl Pts',(5.76853451499994,11.6,8.69562367799999));
#211459=CARTESIAN_POINT('Ctrl Pts',(5.76762905499995,15.2,8.69459689299998));
#211460=CARTESIAN_POINT('Ctrl Pts',(5.76762905499995,11.6,8.69459689299998));
#211461=CARTESIAN_POINT('Ctrl Pts',(5.76673014099994,15.2,8.69357555699998));
#211462=CARTESIAN_POINT('Ctrl Pts',(5.76673014099994,11.6,8.69357555699998));
#211463=CARTESIAN_POINT('Ctrl Pts',(5.76583777899994,15.2,8.69255969399998));
#211464=CARTESIAN_POINT('Ctrl Pts',(5.76583777899994,11.6,8.69255969399998));
#211465=CARTESIAN_POINT('Ctrl Pts',(5.76495196899995,15.2,8.69154932999999));
#211466=CARTESIAN_POINT('Ctrl Pts',(5.76495196899995,11.6,8.69154932999999));
#211467=CARTESIAN_POINT('Ctrl Pts',(5.76407271499994,15.2,8.69054449199999));
#211468=CARTESIAN_POINT('Ctrl Pts',(5.76407271499994,11.6,8.69054449199999));
#211469=CARTESIAN_POINT('Ctrl Pts',(5.76320001899995,15.2,8.68954520599999));
#211470=CARTESIAN_POINT('Ctrl Pts',(5.76320001899995,11.6,8.68954520599999));
#211471=CARTESIAN_POINT('Ctrl Pts',(5.76233388499994,15.2,8.68855149899998));
#211472=CARTESIAN_POINT('Ctrl Pts',(5.76233388499994,11.6,8.68855149899998));
#211473=CARTESIAN_POINT('Ctrl Pts',(5.76147431499995,15.2,8.68756339699999));
#211474=CARTESIAN_POINT('Ctrl Pts',(5.76147431499995,11.6,8.68756339699999));
#211475=CARTESIAN_POINT('Ctrl Pts',(5.76062131199994,15.2,8.68658092599999));
#211476=CARTESIAN_POINT('Ctrl Pts',(5.76062131199994,11.6,8.68658092599999));
#211477=CARTESIAN_POINT('Ctrl Pts',(5.75977487799994,15.2,8.68560411499999));
#211478=CARTESIAN_POINT('Ctrl Pts',(5.75977487799994,11.6,8.68560411499999));
#211479=CARTESIAN_POINT('Ctrl Pts',(5.75893501599994,15.2,8.68463298899999));
#211480=CARTESIAN_POINT('Ctrl Pts',(5.75893501599994,11.6,8.68463298899999));
#211481=CARTESIAN_POINT('Ctrl Pts',(5.75810172999994,15.2,8.68366757599999));
#211482=CARTESIAN_POINT('Ctrl Pts',(5.75810172999994,11.6,8.68366757599999));
#211483=CARTESIAN_POINT('Ctrl Pts',(5.75727501999994,15.2,8.68270790299999));
#211484=CARTESIAN_POINT('Ctrl Pts',(5.75727501999994,11.6,8.68270790299999));
#211485=CARTESIAN_POINT('Ctrl Pts',(5.75645489199994,15.2,8.68175399699999));
#211486=CARTESIAN_POINT('Ctrl Pts',(5.75645489199994,11.6,8.68175399699999));
#211487=CARTESIAN_POINT('Ctrl Pts',(5.75564134699994,15.2,8.68080588599998));
#211488=CARTESIAN_POINT('Ctrl Pts',(5.75564134699994,11.6,8.68080588599998));
#211489=CARTESIAN_POINT('Ctrl Pts',(5.75483438799995,15.2,8.67986359699999));
#211490=CARTESIAN_POINT('Ctrl Pts',(5.75483438799995,11.6,8.67986359699999));
#211491=CARTESIAN_POINT('Ctrl Pts',(5.75403401799995,15.2,8.67892715799999));
#211492=CARTESIAN_POINT('Ctrl Pts',(5.75403401799995,11.6,8.67892715799999));
#211493=CARTESIAN_POINT('Ctrl Pts',(5.75324023999994,15.2,8.67799659699998));
#211494=CARTESIAN_POINT('Ctrl Pts',(5.75324023999994,11.6,8.67799659699998));
#211495=CARTESIAN_POINT('Ctrl Pts',(5.75245305499994,15.2,8.67707194299999));
#211496=CARTESIAN_POINT('Ctrl Pts',(5.75245305499994,11.6,8.67707194299999));
#211497=CARTESIAN_POINT('Ctrl Pts',(5.75167246799994,15.2,8.67615322099999));
#211498=CARTESIAN_POINT('Ctrl Pts',(5.75167246799994,11.6,8.67615322099999));
#211499=CARTESIAN_POINT('Ctrl Pts',(5.75089847999994,15.2,8.67524046099999));
#211500=CARTESIAN_POINT('Ctrl Pts',(5.75089847999994,11.6,8.67524046099999));
#211501=CARTESIAN_POINT('Ctrl Pts',(5.75013109599994,15.2,8.67433369199999));
#211502=CARTESIAN_POINT('Ctrl Pts',(5.75013109599994,11.6,8.67433369199999));
#211503=CARTESIAN_POINT('Ctrl Pts',(5.74937031599994,15.2,8.67343294199999));
#211504=CARTESIAN_POINT('Ctrl Pts',(5.74937031599994,11.6,8.67343294199999));
#211505=CARTESIAN_POINT('Ctrl Pts',(5.74861614399994,15.2,8.67253823899999));
#211506=CARTESIAN_POINT('Ctrl Pts',(5.74861614399994,11.6,8.67253823899999));
#211507=CARTESIAN_POINT('Ctrl Pts',(5.74786858399994,15.2,8.67164961299999));
#211508=CARTESIAN_POINT('Ctrl Pts',(5.74786858399994,11.6,8.67164961299999));
#211509=CARTESIAN_POINT('Ctrl Pts',(5.74712763499994,15.2,8.67076709099998));
#211510=CARTESIAN_POINT('Ctrl Pts',(5.74712763499994,11.6,8.67076709099998));
#211511=CARTESIAN_POINT('Ctrl Pts',(5.74639330499994,15.2,8.66989070399999));
#211512=CARTESIAN_POINT('Ctrl Pts',(5.74639330499994,11.6,8.66989070399999));
#211513=CARTESIAN_POINT('Ctrl Pts',(5.74566559199994,15.2,8.66902047899998));
#211514=CARTESIAN_POINT('Ctrl Pts',(5.74566559199994,11.6,8.66902047899998));
#211515=CARTESIAN_POINT('Ctrl Pts',(5.74494450099994,15.2,8.66815644699999));
#211516=CARTESIAN_POINT('Ctrl Pts',(5.74494450099994,11.6,8.66815644699999));
#211517=CARTESIAN_POINT('Ctrl Pts',(5.74423003499994,15.2,8.66729863599998));
#211518=CARTESIAN_POINT('Ctrl Pts',(5.74423003499994,11.6,8.66729863599998));
#211519=CARTESIAN_POINT('Ctrl Pts',(5.74352219599994,15.2,8.66644707799999));
#211520=CARTESIAN_POINT('Ctrl Pts',(5.74352219599994,11.6,8.66644707799999));
#211521=CARTESIAN_POINT('Ctrl Pts',(5.74282098799995,15.2,8.66560179999999));
#211522=CARTESIAN_POINT('Ctrl Pts',(5.74282098799995,11.6,8.66560179999999));
#211523=CARTESIAN_POINT('Ctrl Pts',(5.74212640999994,15.2,8.66476283199999));
#211524=CARTESIAN_POINT('Ctrl Pts',(5.74212640999994,11.6,8.66476283199999));
#211525=CARTESIAN_POINT('Ctrl Pts',(5.74143846899994,15.2,8.66393020599999));
#211526=CARTESIAN_POINT('Ctrl Pts',(5.74143846899994,11.6,8.66393020599999));
#211527=CARTESIAN_POINT('Ctrl Pts',(5.74075716599994,15.2,8.66310394999999));
#211528=CARTESIAN_POINT('Ctrl Pts',(5.74075716599994,11.6,8.66310394999999));
#211529=CARTESIAN_POINT('Ctrl Pts',(5.74008250299994,15.2,8.66228409699998));
#211530=CARTESIAN_POINT('Ctrl Pts',(5.74008250299994,11.6,8.66228409699998));
#211531=CARTESIAN_POINT('Ctrl Pts',(5.73941448499995,15.2,8.66147067399999));
#211532=CARTESIAN_POINT('Ctrl Pts',(5.73941448499995,11.6,8.66147067399999));
#211533=CARTESIAN_POINT('Ctrl Pts',(5.73875311199994,15.2,8.66066371299999));
#211534=CARTESIAN_POINT('Ctrl Pts',(5.73875311199994,11.6,8.66066371299999));
#211535=CARTESIAN_POINT('Ctrl Pts',(5.73809838799994,15.2,8.65986324599999));
#211536=CARTESIAN_POINT('Ctrl Pts',(5.73809838799994,11.6,8.65986324599999));
#211537=CARTESIAN_POINT('Ctrl Pts',(5.73745031599994,15.2,8.65906930299998));
#211538=CARTESIAN_POINT('Ctrl Pts',(5.73745031599994,11.6,8.65906930299998));
#211539=CARTESIAN_POINT('Ctrl Pts',(5.73680889799995,15.2,8.65828191399999));
#211540=CARTESIAN_POINT('Ctrl Pts',(5.73680889799995,11.6,8.65828191399999));
#211541=CARTESIAN_POINT('Ctrl Pts',(5.73617413699995,15.2,8.65750111099998));
#211542=CARTESIAN_POINT('Ctrl Pts',(5.73617413699995,11.6,8.65750111099998));
#211543=CARTESIAN_POINT('Ctrl Pts',(5.73554603599994,15.2,8.65672692399999));
#211544=CARTESIAN_POINT('Ctrl Pts',(5.73554603599994,11.6,8.65672692399999));
#211545=CARTESIAN_POINT('Ctrl Pts',(5.73492459799994,15.2,8.65595938799999));
#211546=CARTESIAN_POINT('Ctrl Pts',(5.73492459799994,11.6,8.65595938799999));
#211547=CARTESIAN_POINT('Ctrl Pts',(5.73430982499994,15.2,8.65519853099999));
#211548=CARTESIAN_POINT('Ctrl Pts',(5.73430982499994,11.6,8.65519853099999));
#211549=CARTESIAN_POINT('Ctrl Pts',(5.73370172099994,15.2,8.65444438599998));
#211550=CARTESIAN_POINT('Ctrl Pts',(5.73370172099994,11.6,8.65444438599998));
#211551=CARTESIAN_POINT('Ctrl Pts',(5.73310028599994,15.2,8.65369698599999));
#211552=CARTESIAN_POINT('Ctrl Pts',(5.73310028599994,11.6,8.65369698599999));
#211553=CARTESIAN_POINT('Ctrl Pts',(5.73250552599994,15.2,8.65295636199999));
#211554=CARTESIAN_POINT('Ctrl Pts',(5.73250552599994,11.6,8.65295636199999));
#211555=CARTESIAN_POINT('Ctrl Pts',(5.73191744099995,15.2,8.65222254499999));
#211556=CARTESIAN_POINT('Ctrl Pts',(5.73191744099995,11.6,8.65222254499999));
#211557=CARTESIAN_POINT('Ctrl Pts',(5.73133603499994,15.2,8.65149556999998));
#211558=CARTESIAN_POINT('Ctrl Pts',(5.73133603499994,11.6,8.65149556999998));
#211559=CARTESIAN_POINT('Ctrl Pts',(5.73076461999994,15.2,8.65077961499999));
#211560=CARTESIAN_POINT('Ctrl Pts',(5.73076461999994,11.6,8.65077961499999));
#211561=CARTESIAN_POINT('Ctrl Pts',(5.73031342099994,15.2,8.65021312599998));
#211562=CARTESIAN_POINT('Ctrl Pts',(5.73031342099994,11.6,8.65021312599998));
#211563=CARTESIAN_POINT('Ctrl Pts',(5.72997879099994,15.2,8.64979234999998));
#211564=CARTESIAN_POINT('Ctrl Pts',(5.72997879099994,11.6,8.64979234999998));
#211565=CARTESIAN_POINT('Ctrl Pts',(5.72975808699995,15.2,8.64951454399998));
#211566=CARTESIAN_POINT('Ctrl Pts',(5.72975808699995,11.6,8.64951454399998));
#211567=CARTESIAN_POINT('Ctrl Pts',(5.72964966099994,15.2,8.64937799999998));
#211568=CARTESIAN_POINT('Ctrl Pts',(5.72964966099994,11.6,8.64937799999998));
#211569=CARTESIAN_POINT('',(5.72964966093445,12.2,8.64937799923444));
#211570=CARTESIAN_POINT('',(5.72964966093445,15.2,8.64937799923444));
#211571=CARTESIAN_POINT('',(5.72964966099994,12.2,8.64937799899998));
#211572=CARTESIAN_POINT('Ctrl Pts',(6.67046385399994,12.2,9.36775917499999));
#211573=CARTESIAN_POINT('Ctrl Pts',(6.6671058818474,12.2,9.36593194382869));
#211574=CARTESIAN_POINT('Ctrl Pts',(6.66375578545945,12.2,9.36410408905281));
#211575=CARTESIAN_POINT('Ctrl Pts',(6.66041356410863,12.2,9.36227560222762));
#211576=CARTESIAN_POINT('Ctrl Pts',(6.65707134275782,12.2,9.36044711540242));
#211577=CARTESIAN_POINT('Ctrl Pts',(6.65373699675645,12.2,9.35861799819552));
#211578=CARTESIAN_POINT('Ctrl Pts',(6.65041053341856,12.2,9.35678826917066));
#211579=CARTESIAN_POINT('Ctrl Pts',(6.64597524856516,12.2,9.35434863024926));
#211580=CARTESIAN_POINT('Ctrl Pts',(6.64155397840679,12.2,9.35190790080295));
#211581=CARTESIAN_POINT('Ctrl Pts',(6.63714676338973,12.2,9.34946618105871));
#211582=CARTESIAN_POINT('Ctrl Pts',(6.63384135242718,12.2,9.34763489141686));
#211583=CARTESIAN_POINT('Ctrl Pts',(6.63054384824704,12.2,9.34580304603342));
#211584=CARTESIAN_POINT('Ctrl Pts',(6.62725426919988,12.2,9.34397068826666));
#211585=CARTESIAN_POINT('Ctrl Pts',(6.62396469015272,12.2,9.34213833049989));
#211586=CARTESIAN_POINT('Ctrl Pts',(6.62068303692194,12.2,9.34030545949983));
#211587=CARTESIAN_POINT('Ctrl Pts',(6.61740932137352,12.2,9.33847211023315));
#211588=CARTESIAN_POINT('Ctrl Pts',(6.61413560582511,12.2,9.33663876096647));
#211589=CARTESIAN_POINT('Ctrl Pts',(6.61086983012559,12.2,9.33480493332982));
#211590=CARTESIAN_POINT('Ctrl Pts',(6.60761200691361,12.2,9.33297066159654));
#211591=CARTESIAN_POINT('Ctrl Pts',(6.60435418370163,12.2,9.33113638986326));
#211592=CARTESIAN_POINT('Ctrl Pts',(6.60110431353991,12.2,9.32930167583331));
#211593=CARTESIAN_POINT('Ctrl Pts',(6.59786241440663,12.2,9.32746655815004));
#211594=CARTESIAN_POINT('Ctrl Pts',(6.59462051468439,12.2,9.3256314401334));
#211595=CARTESIAN_POINT('Ctrl Pts',(6.59138658419773,12.2,9.32379591866663));
#211596=CARTESIAN_POINT('Ctrl Pts',(6.58816063952165,12.2,9.32196003306644));
#211597=CARTESIAN_POINT('Ctrl Pts',(6.58493469543161,12.2,9.32012414779976));
#211598=CARTESIAN_POINT('Ctrl Pts',(6.58171673804949,12.2,9.31828789789976));
#211599=CARTESIAN_POINT('Ctrl Pts',(6.5785067809168,12.2,9.31645132209146));
#211600=CARTESIAN_POINT('Ctrl Pts',(6.57422683826761,12.2,9.31400255445826));
#211601=CARTESIAN_POINT('Ctrl Pts',(6.56996111897463,12.2,9.31155320486088));
#211602=CARTESIAN_POINT('Ctrl Pts',(6.56570965960855,12.2,9.30910336660547));
#211603=CARTESIAN_POINT('Ctrl Pts',(6.56039533496649,12.2,9.30604106853587));
#211604=CARTESIAN_POINT('Ctrl Pts',(6.55510329421805,12.2,9.30297800795032));
#211605=CARTESIAN_POINT('Ctrl Pts',(6.54983360636966,12.2,9.29991436420034));
#211606=CARTESIAN_POINT('Ctrl Pts',(6.54667179377551,12.2,9.29807617801715));
#211607=CARTESIAN_POINT('Ctrl Pts',(6.54351802822246,12.2,9.29623778218396));
#211608=CARTESIAN_POINT('Ctrl Pts',(6.54037232566899,12.2,9.29439921691746));
#211609=CARTESIAN_POINT('Ctrl Pts',(6.53722662254404,12.2,9.29256065131694));
#211610=CARTESIAN_POINT('Ctrl Pts',(6.53408898292138,12.2,9.29072191463304));
#211611=CARTESIAN_POINT('Ctrl Pts',(6.53095942080099,12.2,9.28888304807412));
#211612=CARTESIAN_POINT('Ctrl Pts',(6.52782985924913,12.2,9.28704418184924));
#211613=CARTESIAN_POINT('Ctrl Pts',(6.52470837625576,12.2,9.28520518526925));
#211614=CARTESIAN_POINT('Ctrl Pts',(6.52159498738094,12.2,9.28336609841083));
#211615=CARTESIAN_POINT('Ctrl Pts',(6.51848159850612,12.2,9.28152701155243));
#211616=CARTESIAN_POINT('Ctrl Pts',(6.51537630233253,12.2,9.27968783358269));
#211617=CARTESIAN_POINT('Ctrl Pts',(6.51227911573743,12.2,9.27784860631618));
#211618=CARTESIAN_POINT('Ctrl Pts',(6.50918192914233,12.2,9.27600937904966));
#211619=CARTESIAN_POINT('Ctrl Pts',(6.50609285223794,12.2,9.27417010098316));
#211620=CARTESIAN_POINT('Ctrl Pts',(6.50301189922488,12.2,9.27233081325832));
#211621=CARTESIAN_POINT('Ctrl Pts',(6.49993094621182,12.2,9.27049152553348));
#211622=CARTESIAN_POINT('Ctrl Pts',(6.4968581184401,12.2,9.2686522274503));
#211623=CARTESIAN_POINT('Ctrl Pts',(6.49379342984241,12.2,9.26681296122546));
#211624=CARTESIAN_POINT('Ctrl Pts',(6.49072874124472,12.2,9.26497369500062));
#211625=CARTESIAN_POINT('Ctrl Pts',(6.4876721920548,12.2,9.26313445950077));
#211626=CARTESIAN_POINT('Ctrl Pts',(6.48462379891444,12.2,9.26129529540092));
#211627=CARTESIAN_POINT('Ctrl Pts',(6.48157540522029,12.2,9.25945613096695));
#211628=CARTESIAN_POINT('Ctrl Pts',(6.47853516701179,12.2,9.25761703901634));
#211629=CARTESIAN_POINT('Ctrl Pts',(6.4755030988639,12.2,9.25577805958242));
#211630=CARTESIAN_POINT('Ctrl Pts',(6.47247103126683,12.2,9.25393908048258));
#211631=CARTESIAN_POINT('Ctrl Pts',(6.46944713415664,12.2,9.25210021516928));
#211632=CARTESIAN_POINT('Ctrl Pts',(6.46643142244985,12.2,9.25026150439425));
#211633=CARTESIAN_POINT('Ctrl Pts',(6.46341571074305,12.2,9.24842279361922));
#211634=CARTESIAN_POINT('Ctrl Pts',(6.46040818549674,12.2,9.24658423726613));
#211635=CARTESIAN_POINT('Ctrl Pts',(6.45740886143977,12.2,9.24474587754128));
#211636=CARTESIAN_POINT('Ctrl Pts',(6.4544095373828,12.2,9.24290751781643));
#211637=CARTESIAN_POINT('Ctrl Pts',(6.45141841504151,12.2,9.24106935351654));
#211638=CARTESIAN_POINT('Ctrl Pts',(6.44843550848322,12.2,9.23923142874998));
#211639=CARTESIAN_POINT('Ctrl Pts',(6.44545260192492,12.2,9.23739350398342));
#211640=CARTESIAN_POINT('Ctrl Pts',(6.44247791184965,12.2,9.23555581613354));
#211641=CARTESIAN_POINT('Ctrl Pts',(6.4395114533317,12.2,9.2337184104086));
#211642=CARTESIAN_POINT('Ctrl Pts',(6.43654499481376,12.2,9.23188100468366));
#211643=CARTESIAN_POINT('Ctrl Pts',(6.43358676976188,12.2,9.23004387978044));
#211644=CARTESIAN_POINT('Ctrl Pts',(6.43063679005406,12.2,9.22820707713037));
#211645=CARTESIAN_POINT('Ctrl Pts',(6.42768681034623,12.2,9.22637027448029));
#211646=CARTESIAN_POINT('Ctrl Pts',(6.42474507756727,12.2,9.22453379676693));
#211647=CARTESIAN_POINT('Ctrl Pts',(6.42181160742272,12.2,9.22269768416692));
#211648=CARTESIAN_POINT('Ctrl Pts',(6.41887813674525,12.2,9.22086157123335));
#211649=CARTESIAN_POINT('Ctrl Pts',(6.41595292835348,12.2,9.21902582433324));
#211650=CARTESIAN_POINT('Ctrl Pts',(6.413035997639,12.2,9.21719048639988));
#211651=CARTESIAN_POINT('Ctrl Pts',(6.40914675756954,12.2,9.21474336971111));
#211652=CARTESIAN_POINT('Ctrl Pts',(6.40527223088432,12.2,9.21229698082504));
#211653=CARTESIAN_POINT('Ctrl Pts',(6.40141245753223,12.2,9.20985142219158));
#211654=CARTESIAN_POINT('Ctrl Pts',(6.39851762738668,12.2,9.20801725313317));
#211655=CARTESIAN_POINT('Ctrl Pts',(6.395631094847,12.2,9.20618355192969));
#211656=CARTESIAN_POINT('Ctrl Pts',(6.39275287505683,12.2,9.20435036082133));
#211657=CARTESIAN_POINT('Ctrl Pts',(6.38987465526665,12.2,9.20251716971296));
#211658=CARTESIAN_POINT('Ctrl Pts',(6.38700474795421,12.2,9.20068449126623));
#211659=CARTESIAN_POINT('Ctrl Pts',(6.38414316884872,12.2,9.19885236666605));
#211660=CARTESIAN_POINT('Ctrl Pts',(6.38128158922337,12.2,9.19702024173304));
#211661=CARTESIAN_POINT('Ctrl Pts',(6.37842833804203,12.2,9.19518867110018));
#211662=CARTESIAN_POINT('Ctrl Pts',(6.37558342987971,12.2,9.19335770058416));
#211663=CARTESIAN_POINT('Ctrl Pts',(6.3727385222342,12.2,9.19152673040077));
#211664=CARTESIAN_POINT('Ctrl Pts',(6.3699019570716,12.2,9.18969635930069));
#211665=CARTESIAN_POINT('Ctrl Pts',(6.36707375092509,12.2,9.18786663261722));
#211666=CARTESIAN_POINT('Ctrl Pts',(6.36424554477857,12.2,9.18603690593375));
#211667=CARTESIAN_POINT('Ctrl Pts',(6.3614256971579,12.2,9.18420782217351));
#211668=CARTESIAN_POINT('Ctrl Pts',(6.35861422249733,12.2,9.18237942898165));
#211669=CARTESIAN_POINT('Ctrl Pts',(6.35580274783677,12.2,9.18055103578979));
#211670=CARTESIAN_POINT('Ctrl Pts',(6.35299964591362,12.2,9.1787233308769));
#211671=CARTESIAN_POINT('Ctrl Pts',(6.35020493279409,12.2,9.17689636026831));
#211672=CARTESIAN_POINT('Ctrl Pts',(6.34647864829625,12.2,9.17446039923558));
#211673=CARTESIAN_POINT('Ctrl Pts',(6.34276727724823,12.2,9.17202574417628));
#211674=CARTESIAN_POINT('Ctrl Pts',(6.33907085410387,12.2,9.16959250187715));
#211675=CARTESIAN_POINT('Ctrl Pts',(6.33537443146315,12.2,9.16715925990955));
#211676=CARTESIAN_POINT('Ctrl Pts',(6.33169295780377,12.2,9.16472743152231));
#211677=CARTESIAN_POINT('Ctrl Pts',(6.32802646782476,12.2,9.16229712616534));
#211678=CARTESIAN_POINT('Ctrl Pts',(6.32435997734619,12.2,9.15986682047724));
#211679=CARTESIAN_POINT('Ctrl Pts',(6.32070847097307,12.2,9.15743803640397));
#211680=CARTESIAN_POINT('Ctrl Pts',(6.31707198370562,12.2,9.15501088587279));
#211681=CARTESIAN_POINT('Ctrl Pts',(6.31252637486905,12.2,9.15197694787417));
#211682=CARTESIAN_POINT('Ctrl Pts',(6.30800423474288,12.2,9.1489455615425));
#211683=CARTESIAN_POINT('Ctrl Pts',(6.30350563266148,12.2,9.14591694161217));
#211684=CARTESIAN_POINT('Ctrl Pts',(6.29990675129056,12.2,9.14349404586599));
#211685=CARTESIAN_POINT('Ctrl Pts',(6.29632293268712,12.2,9.14107292328902));
#211686=CARTESIAN_POINT('Ctrl Pts',(6.29275421403344,12.2,9.1386536839311));
#211687=CARTESIAN_POINT('Ctrl Pts',(6.28918549489351,12.2,9.13623444424358));
#211688=CARTESIAN_POINT('Ctrl Pts',(6.28563187545207,12.2,9.13381708826275));
#211689=CARTESIAN_POINT('Ctrl Pts',(6.28209339069486,12.2,9.13140172989951));
#211690=CARTESIAN_POINT('Ctrl Pts',(6.27855490641977,12.2,9.12898637186537));
#211691=CARTESIAN_POINT('Ctrl Pts',(6.27503155668436,12.2,9.12657301194737));
#211692=CARTESIAN_POINT('Ctrl Pts',(6.27152337730349,12.2,9.12416176342212));
#211693=CARTESIAN_POINT('Ctrl Pts',(6.26801519744462,12.2,9.12175051456834));
#211694=CARTESIAN_POINT('Ctrl Pts',(6.26452218674315,12.2,9.11934137720371));
#211695=CARTESIAN_POINT('Ctrl Pts',(6.26104438166573,12.2,9.11693446879491));
#211696=CARTESIAN_POINT('Ctrl Pts',(6.25756657706216,12.2,9.11452756071404));
#211697=CARTESIAN_POINT('Ctrl Pts',(6.2541039794808,12.2,9.11212287958908));
#211698=CARTESIAN_POINT('Ctrl Pts',(6.25065662003354,12.2,9.10972054166525));
#211699=CARTESIAN_POINT('Ctrl Pts',(6.24634742037217,12.2,9.10671761901499));
#211700=CARTESIAN_POINT('Ctrl Pts',(6.24206203533554,12.2,9.10371836136277));
#211701=CARTESIAN_POINT('Ctrl Pts',(6.23780053082039,12.2,9.10072299469589));
#211702=CARTESIAN_POINT('Ctrl Pts',(6.23439132702247,12.2,9.09832670123178));
#211703=CARTESIAN_POINT('Ctrl Pts',(6.23099740759029,12.2,9.095932900018));
#211704=CARTESIAN_POINT('Ctrl Pts',(6.22761880774049,12.2,9.09354170855452));
#211705=CARTESIAN_POINT('Ctrl Pts',(6.22424020835103,12.2,9.09115051741683));
#211706=CARTESIAN_POINT('Ctrl Pts',(6.22087692853601,12.2,9.08876193805375));
#211707=CARTESIAN_POINT('Ctrl Pts',(6.21752900175238,12.2,9.08637608879615));
#211708=CARTESIAN_POINT('Ctrl Pts',(6.21418107451258,12.2,9.08399023921346));
#211709=CARTESIAN_POINT('Ctrl Pts',(6.21084850170585,12.2,9.08160712092661));
#211710=CARTESIAN_POINT('Ctrl Pts',(6.20753131847051,12.2,9.07922685529708));
#211711=CARTESIAN_POINT('Ctrl Pts',(6.20421413568714,12.2,9.07684658999184));
#211712=CARTESIAN_POINT('Ctrl Pts',(6.20091234171459,12.2,9.07446917552217));
#211713=CARTESIAN_POINT('Ctrl Pts',(6.19762597053721,12.2,9.07209473760486));
#211714=CARTESIAN_POINT('Ctrl Pts',(6.19433959891206,12.2,9.06972029936403));
#211715=CARTESIAN_POINT('Ctrl Pts',(6.19106865276064,12.2,9.06734883552906));
#211716=CARTESIAN_POINT('Ctrl Pts',(6.18781316424988,12.2,9.06498047073331));
#211717=CARTESIAN_POINT('Ctrl Pts',(6.18455767573913,12.2,9.06261210593757));
#211718=CARTESIAN_POINT('Ctrl Pts',(6.18131764480794,12.2,9.06024684137829));
#211719=CARTESIAN_POINT('Ctrl Pts',(6.17809310818935,12.2,9.05788479930545));
#211720=CARTESIAN_POINT('Ctrl Pts',(6.1748685720101,12.2,9.05552275755444));
#211721=CARTESIAN_POINT('Ctrl Pts',(6.17165952789167,12.2,9.05316394038639));
#211722=CARTESIAN_POINT('Ctrl Pts',(6.16846601252706,12.2,9.05080847323491));
#211723=CARTESIAN_POINT('Ctrl Pts',(6.16447411799498,12.2,9.04786413905486));
#211724=CARTESIAN_POINT('Ctrl Pts',(6.16050648444987,12.2,9.04492503999997));
#211725=CARTESIAN_POINT('Ctrl Pts',(6.15656318153321,12.2,9.04199142499997));
#211726=CARTESIAN_POINT('Ctrl Pts',(6.15340853902796,12.2,9.03964453287206));
#211727=CARTESIAN_POINT('Ctrl Pts',(6.15026946639395,12.2,9.03730114992513));
#211728=CARTESIAN_POINT('Ctrl Pts',(6.14714599928086,12.2,9.03496140707575));
#211729=CARTESIAN_POINT('Ctrl Pts',(6.14402253259335,12.2,9.03262166454518));
#211730=CARTESIAN_POINT('Ctrl Pts',(6.1409146728383,12.2,9.03028556102427));
#211731=CARTESIAN_POINT('Ctrl Pts',(6.13782245024366,12.2,9.0279532272599));
#211732=CARTESIAN_POINT('Ctrl Pts',(6.13473022722772,12.2,9.02562089317774));
#211733=CARTESIAN_POINT('Ctrl Pts',(6.13165364598967,12.2,9.02329232778231));
#211734=CARTESIAN_POINT('Ctrl Pts',(6.1285927369911,12.2,9.02096766437823));
#211735=CARTESIAN_POINT('Ctrl Pts',(6.12553182840959,12.2,9.01864300129088));
#211736=CARTESIAN_POINT('Ctrl Pts',(6.12248659518995,12.2,9.0163222401336));
#211737=CARTESIAN_POINT('Ctrl Pts',(6.11945706854769,12.2,9.01400551365607));
#211738=CARTESIAN_POINT('Ctrl Pts',(6.11642754149265,12.2,9.01168878686287));
#211739=CARTESIAN_POINT('Ctrl Pts',(6.11341372247396,12.2,9.0093760948308));
#211740=CARTESIAN_POINT('Ctrl Pts',(6.11041564577326,12.2,9.00706757142334));
#211741=CARTESIAN_POINT('Ctrl Pts',(6.10741756948106,12.2,9.00475904833043));
#211742=CARTESIAN_POINT('Ctrl Pts',(6.10443523627051,12.2,9.00245469451696));
#211743=CARTESIAN_POINT('Ctrl Pts',(6.10146867823422,12.2,9.00015464670471));
#211744=CARTESIAN_POINT('Ctrl Pts',(6.09850211979372,12.2,8.99785459857906));
#211745=CARTESIAN_POINT('Ctrl Pts',(6.09555133760237,12.2,8.99555885554841));
#211746=CARTESIAN_POINT('Ctrl Pts',(6.09261636577676,12.2,8.9932675543127));
#211747=CARTESIAN_POINT('Ctrl Pts',(6.08968139435104,12.2,8.99097625338917));
#211748=CARTESIAN_POINT('Ctrl Pts',(6.08676223358588,12.2,8.98868939669511));
#211749=CARTESIAN_POINT('Ctrl Pts',(6.08385891545459,12.2,8.98640712082283));
#211750=CARTESIAN_POINT('Ctrl Pts',(6.08095559692772,12.2,8.9841248446396));
#211751=CARTESIAN_POINT('Ctrl Pts',(6.07806812308744,12.2,8.98184714922667));
#211752=CARTESIAN_POINT('Ctrl Pts',(6.07519652726528,12.2,8.97957417654753));
#211753=CARTESIAN_POINT('Ctrl Pts',(6.07232493183439,12.2,8.97730120417809));
#211754=CARTESIAN_POINT('Ctrl Pts',(6.06946921353368,12.2,8.97503295278828));
#211755=CARTESIAN_POINT('Ctrl Pts',(6.06662940743087,12.2,8.9727695663617));
#211756=CARTESIAN_POINT('Ctrl Pts',(6.06378960094111,12.2,8.97050617962672));
#211757=CARTESIAN_POINT('Ctrl Pts',(6.06096570593593,12.2,8.96824765529258));
#211758=CARTESIAN_POINT('Ctrl Pts',(6.05815775554798,12.2,8.9659941387151));
#211759=CARTESIAN_POINT('Ctrl Pts',(6.0553498055426,12.2,8.96374062244466));
#211760=CARTESIAN_POINT('Ctrl Pts',(6.05255780151458,12.2,8.961492114295));
#211761=CARTESIAN_POINT('Ctrl Pts',(6.04978177546211,12.2,8.95924875736676));
#211762=CARTESIAN_POINT('Ctrl Pts',(6.0470057490314,12.2,8.95700540013286));
#211763=CARTESIAN_POINT('Ctrl Pts',(6.04424570233554,12.2,8.95476719471332));
#211764=CARTESIAN_POINT('Ctrl Pts',(6.04150166724154,12.2,8.95253428875829));
#211765=CARTESIAN_POINT('Ctrl Pts',(6.03875763214755,12.2,8.95030138280327));
#211766=CARTESIAN_POINT('Ctrl Pts',(6.03602960957208,12.2,8.94807377593496));
#211767=CARTESIAN_POINT('Ctrl Pts',(6.03331763181482,12.2,8.94585161536998));
#211768=CARTESIAN_POINT('Ctrl Pts',(6.03060565442707,12.2,8.94362945510777));
#211769=CARTESIAN_POINT('Ctrl Pts',(6.02790972416707,12.2,8.94141274234743));
#211770=CARTESIAN_POINT('Ctrl Pts',(6.02522987148504,12.2,8.93920162551813));
#211771=CARTESIAN_POINT('Ctrl Pts',(6.02255001843789,12.2,8.93699050838758));
#211772=CARTESIAN_POINT('Ctrl Pts',(6.01988624559575,12.2,8.93478498847348));
#211773=CARTESIAN_POINT('Ctrl Pts',(6.017238583842,12.2,8.93258521663197));
#211774=CARTESIAN_POINT('Ctrl Pts',(6.014590922449,12.2,8.93038544509017));
#211775=CARTESIAN_POINT('Ctrl Pts',(6.01195937395665,12.2,8.92819142275318));
#211776=CARTESIAN_POINT('Ctrl Pts',(6.00934396994718,12.2,8.9260033006539));
#211777=CARTESIAN_POINT('Ctrl Pts',(6.00672856558136,12.2,8.92381517825648));
#211778=CARTESIAN_POINT('Ctrl Pts',(6.00412930736298,12.2,8.92163295911099));
#211779=CARTESIAN_POINT('Ctrl Pts',(6.00154622681681,12.2,8.91945679521755));
#211780=CARTESIAN_POINT('Ctrl Pts',(5.99896314662258,12.2,8.9172806316206));
#211781=CARTESIAN_POINT('Ctrl Pts',(5.99639624582055,12.2,8.91511052588654));
#211782=CARTESIAN_POINT('Ctrl Pts',(5.99384555575022,12.2,8.91294663245192));
#211783=CARTESIAN_POINT('Ctrl Pts',(5.99065719290165,12.2,8.91024176543752));
#211784=CARTESIAN_POINT('Ctrl Pts',(5.98749416057878,12.2,8.90754660677615));
#211785=CARTESIAN_POINT('Ctrl Pts',(5.98435652273024,12.2,8.9048614671923));
#211786=CARTESIAN_POINT('Ctrl Pts',(5.9812188848817,12.2,8.90217632760845));
#211787=CARTESIAN_POINT('Ctrl Pts',(5.97810664153232,12.2,8.89950120595799));
#211788=CARTESIAN_POINT('Ctrl Pts',(5.9750198569349,12.2,8.89683641879307));
#211789=CARTESIAN_POINT('Ctrl Pts',(5.97193307233748,12.2,8.89417163162817));
#211790=CARTESIAN_POINT('Ctrl Pts',(5.96887174610543,12.2,8.89151717811661));
#211791=CARTESIAN_POINT('Ctrl Pts',(5.96583594304987,12.2,8.88887337624163));
#211792=CARTESIAN_POINT('Ctrl Pts',(5.96280013999433,12.2,8.88622957436663));
#211793=CARTESIAN_POINT('Ctrl Pts',(5.95978985804985,12.2,8.88359642708883));
#211794=CARTESIAN_POINT('Ctrl Pts',(5.95680516346653,12.2,8.88097425674161));
#211795=CARTESIAN_POINT('Ctrl Pts',(5.95382046888323,12.2,8.87835208639441));
#211796=CARTESIAN_POINT('Ctrl Pts',(5.95086135960598,12.2,8.87574089275476));
#211797=CARTESIAN_POINT('Ctrl Pts',(5.94792790077328,12.2,8.87314100725687));
#211798=CARTESIAN_POINT('Ctrl Pts',(5.94499444194058,12.2,8.87054112175899));
#211799=CARTESIAN_POINT('Ctrl Pts',(5.94208663164353,12.2,8.86795254016976));
#211800=CARTESIAN_POINT('Ctrl Pts',(5.93920453456154,12.2,8.86537560232316));
#211801=CARTESIAN_POINT('Ctrl Pts',(5.93632243747956,12.2,8.86279866447657));
#211802=CARTESIAN_POINT('Ctrl Pts',(5.93346605321914,12.2,8.86023336646575));
#211803=CARTESIAN_POINT('Ctrl Pts',(5.93063544453991,12.2,8.85768004959138));
#211804=CARTESIAN_POINT('Ctrl Pts',(5.92780483586069,12.2,8.85512673271699));
#211805=CARTESIAN_POINT('Ctrl Pts',(5.92500000295331,12.2,8.85258539625413));
#211806=CARTESIAN_POINT('Ctrl Pts',(5.92222100892737,12.2,8.85005638598975));
#211807=CARTESIAN_POINT('Ctrl Pts',(5.91944201490143,12.2,8.84752737572535));
#211808=CARTESIAN_POINT('Ctrl Pts',(5.91668885870217,12.2,8.84501069001584));
#211809=CARTESIAN_POINT('Ctrl Pts',(5.9139616034265,12.2,8.84250668140577));
#211810=CARTESIAN_POINT('Ctrl Pts',(5.91123434815083,12.2,8.84000267279569));
#211811=CARTESIAN_POINT('Ctrl Pts',(5.90853299426447,12.2,8.83751133963026));
#211812=CARTESIAN_POINT('Ctrl Pts',(5.90585760384995,12.2,8.83503303865913));
#211813=CARTESIAN_POINT('Ctrl Pts',(5.90318221372705,12.2,8.83255473795813));
#211814=CARTESIAN_POINT('Ctrl Pts',(5.90053278688699,12.2,8.83008946886562));
#211815=CARTESIAN_POINT('Ctrl Pts',(5.89790938585136,12.2,8.82763759406233));
#211816=CARTESIAN_POINT('Ctrl Pts',(5.89528598452978,12.2,8.82518571899178));
#211817=CARTESIAN_POINT('Ctrl Pts',(5.8926886087717,12.2,8.82274723660714));
#211818=CARTESIAN_POINT('Ctrl Pts',(5.89011732001954,12.2,8.82032251730044));
#211819=CARTESIAN_POINT('Ctrl Pts',(5.88754603126739,12.2,8.81789779799374));
#211820=CARTESIAN_POINT('Ctrl Pts',(5.88500083064228,12.2,8.81548683936562));
#211821=CARTESIAN_POINT('Ctrl Pts',(5.88248177850073,12.2,8.8130900167449));
#211822=CARTESIAN_POINT('Ctrl Pts',(5.87996272635918,12.2,8.81069319412419));
#211823=CARTESIAN_POINT('Ctrl Pts',(5.87746982396273,12.2,8.80831050698901));
#211824=CARTESIAN_POINT('Ctrl Pts',(5.87500313187802,12.2,8.80594233615491));
#211825=CARTESIAN_POINT('Ctrl Pts',(5.87253643979331,12.2,8.80357416532081));
#211826=CARTESIAN_POINT('Ctrl Pts',(5.87009595785373,12.2,8.80122050867043));
#211827=CARTESIAN_POINT('Ctrl Pts',(5.86768174819959,12.2,8.79888175616966));
#211828=CARTESIAN_POINT('Ctrl Pts',(5.86478469671989,12.2,8.79607525327071));
#211829=CARTESIAN_POINT('Ctrl Pts',(5.86192547658248,12.2,8.79329020901056));
#211830=CARTESIAN_POINT('Ctrl Pts',(5.85910419326574,12.2,8.79052730435944));
#211831=CARTESIAN_POINT('Ctrl Pts',(5.85628290969271,12.2,8.78776439945734));
#211832=CARTESIAN_POINT('Ctrl Pts',(5.85349956259004,12.2,8.78502363625738));
#211833=CARTESIAN_POINT('Ctrl Pts',(5.85075425885876,12.2,8.78230570736025));
#211834=CARTESIAN_POINT('Ctrl Pts',(5.84755140487964,12.2,8.77913479068393));
#211835=CARTESIAN_POINT('Ctrl Pts',(5.84440032854945,12.2,8.77599495627641));
#211836=CARTESIAN_POINT('Ctrl Pts',(5.84130119832276,12.2,8.77288733252362));
#211837=CARTESIAN_POINT('Ctrl Pts',(5.83864480067538,12.2,8.77022365471015));
#211838=CARTESIAN_POINT('Ctrl Pts',(5.83602656652335,12.2,8.76758364347395));
#211839=CARTESIAN_POINT('Ctrl Pts',(5.83344660080109,12.2,8.76496802491582));
#211840=CARTESIAN_POINT('Ctrl Pts',(5.83086663531318,12.2,8.76235240659527));
#211841=CARTESIAN_POINT('Ctrl Pts',(5.82832493726317,12.2,8.75976118361123));
#211842=CARTESIAN_POINT('Ctrl Pts',(5.82582161075935,12.2,8.7571950982761));
#211843=CARTESIAN_POINT('Ctrl Pts',(5.82331828425552,12.2,8.75462901294098));
#211844=CARTESIAN_POINT('Ctrl Pts',(5.82085332991217,12.2,8.75208806698448));
#211845=CARTESIAN_POINT('Ctrl Pts',(5.8184268494977,12.2,8.74957302074075));
#211846=CARTESIAN_POINT('Ctrl Pts',(5.81600036886283,12.2,8.74705797426858));
#211847=CARTESIAN_POINT('Ctrl Pts',(5.81361236392419,12.2,8.74456882772578));
#211848=CARTESIAN_POINT('Ctrl Pts',(5.81126293426436,12.2,8.74210636005346));
#211849=CARTESIAN_POINT('Ctrl Pts',(5.80891350481795,12.2,8.73964389260483));
#211850=CARTESIAN_POINT('Ctrl Pts',(5.80660265493396,12.2,8.73720810406243));
#211851=CARTESIAN_POINT('Ctrl Pts',(5.80433048351653,12.2,8.73479978998325));
#211852=CARTESIAN_POINT('Ctrl Pts',(5.80205831209908,12.2,8.73239147590408));
#211853=CARTESIAN_POINT('Ctrl Pts',(5.79982481950369,12.2,8.73001063901449));
#211854=CARTESIAN_POINT('Ctrl Pts',(5.79763010899744,12.2,8.7276580920147));
#211855=CARTESIAN_POINT('Ctrl Pts',(5.79543539829184,12.2,8.72530554480121));
#211856=CARTESIAN_POINT('Ctrl Pts',(5.79327946874741,12.2,8.72298129074938));
#211857=CARTESIAN_POINT('Ctrl Pts',(5.7911624220285,12.2,8.72068616151131));
#211858=CARTESIAN_POINT('Ctrl Pts',(5.7890453755019,12.2,8.71839103248172));
#211859=CARTESIAN_POINT('Ctrl Pts',(5.78696721260079,12.2,8.71612503132703));
#211860=CARTESIAN_POINT('Ctrl Pts',(5.78492803225821,12.2,8.7138890114916));
#211861=CARTESIAN_POINT('Ctrl Pts',(5.78288885191562,12.2,8.71165299165615));
#211862=CARTESIAN_POINT('Ctrl Pts',(5.78088865678534,12.2,8.70944695629186));
#211863=CARTESIAN_POINT('Ctrl Pts',(5.77892754525635,12.2,8.7072717794271));
#211864=CARTESIAN_POINT('Ctrl Pts',(5.77696643354925,12.2,8.70509660236476));
#211865=CARTESIAN_POINT('Ctrl Pts',(5.77504440614461,12.2,8.70295228505764));
#211866=CARTESIAN_POINT('Ctrl Pts',(5.77316156354465,12.2,8.700839728028));
#211867=CARTESIAN_POINT('Ctrl Pts',(5.77127872111573,12.2,8.69872717119023));
#211868=CARTESIAN_POINT('Ctrl Pts',(5.76943506489992,12.2,8.69664637181713));
#211869=CARTESIAN_POINT('Ctrl Pts',(5.76763069154072,12.2,8.69459825521566));
#211870=CARTESIAN_POINT('Ctrl Pts',(5.76582631818152,12.2,8.69255013861418));
#211871=CARTESIAN_POINT('Ctrl Pts',(5.76406122962478,12.2,8.69053470495421));
#211872=CARTESIAN_POINT('Ctrl Pts',(5.76233552610243,12.2,8.68855290035808));
#211873=CARTESIAN_POINT('Ctrl Pts',(5.76060982242332,12.2,8.68657109558192));
#211874=CARTESIAN_POINT('Ctrl Pts',(5.75892350278245,12.2,8.6846229190683));
#211875=CARTESIAN_POINT('Ctrl Pts',(5.75727666527871,12.2,8.68270934454968));
#211876=CARTESIAN_POINT('Ctrl Pts',(5.75562982792455,12.2,8.68079577020487));
#211877=CARTESIAN_POINT('Ctrl Pts',(5.75402247582258,12.2,8.67891679728942));
#211878=CARTESIAN_POINT('Ctrl Pts',(5.75245470438126,12.2,8.67707342594128));
#211879=CARTESIAN_POINT('Ctrl Pts',(5.75088693293994,12.2,8.67523005459314));
#211880=CARTESIAN_POINT('Ctrl Pts',(5.74935874527049,12.2,8.67342228223386));
#211881=CARTESIAN_POINT('Ctrl Pts',(5.74787023690616,12.2,8.67165113912993));
#211882=CARTESIAN_POINT('Ctrl Pts',(5.74638172854184,12.2,8.66987999602601));
#211883=CARTESIAN_POINT('Ctrl Pts',(5.74493290056333,12.2,8.66814547940082));
#211884=CARTESIAN_POINT('Ctrl Pts',(5.7435238538618,12.2,8.66644864820988));
#211885=CARTESIAN_POINT('Ctrl Pts',(5.74211480703228,12.2,8.66475181686481));
#211886=CARTESIAN_POINT('Ctrl Pts',(5.74074553694831,12.2,8.66309266816506));
#211887=CARTESIAN_POINT('Ctrl Pts',(5.73941614621092,12.2,8.66147228941177));
#211888=CARTESIAN_POINT('Ctrl Pts',(5.73808675559428,12.2,8.65985191080565));
#211889=CARTESIAN_POINT('Ctrl Pts',(5.7367972402858,12.2,8.65827030439334));
#211890=CARTESIAN_POINT('Ctrl Pts',(5.73554770174212,12.2,8.65672858669229));
#211891=CARTESIAN_POINT('Ctrl Pts',(5.7334711343,12.2,8.65416645621689));
#211892=CARTESIAN_POINT('Ctrl Pts',(5.73150497962641,12.2,8.65171445644522));
#211893=CARTESIAN_POINT('Ctrl Pts',(5.72964966099994,12.2,8.64937799999998));
#211894=CARTESIAN_POINT('Ctrl Pts',(5.72964966099994,15.2,8.64937799999998));
#211895=CARTESIAN_POINT('Ctrl Pts',(5.73076070896187,15.2,8.65077717485576));
#211896=CARTESIAN_POINT('Ctrl Pts',(5.731911500976,15.2,8.65221780246531));
#211897=CARTESIAN_POINT('Ctrl Pts',(5.7331019545695,15.2,8.65369867983773));
#211898=CARTESIAN_POINT('Ctrl Pts',(5.73429814913197,15.2,8.65518669874938));
#211899=CARTESIAN_POINT('Ctrl Pts',(5.73553438373783,15.2,8.65671537363565));
#211900=CARTESIAN_POINT('Ctrl Pts',(5.73681056237342,15.2,8.65828356063504));
#211901=CARTESIAN_POINT('Ctrl Pts',(5.73808674089308,15.2,8.65985174749198));
#211902=CARTESIAN_POINT('Ctrl Pts',(5.73940286065744,15.2,8.66145944675969));
#211903=CARTESIAN_POINT('Ctrl Pts',(5.74075882602487,15.2,8.66310555069991));
#211904=CARTESIAN_POINT('Ctrl Pts',(5.74211479139229,15.2,8.66475165464014));
#211905=CARTESIAN_POINT('Ctrl Pts',(5.74351060050216,15.2,8.66643616409547));
#211906=CARTESIAN_POINT('Ctrl Pts',(5.74494615710277,15.2,8.66815800211678));
#211907=CARTESIAN_POINT('Ctrl Pts',(5.74638171383377,15.2,8.6698798402945));
#211908=CARTESIAN_POINT('Ctrl Pts',(5.74785701674642,15.2,8.67163900569532));
#211909=CARTESIAN_POINT('Ctrl Pts',(5.74937196816501,15.2,8.6734344539623));
#211910=CARTESIAN_POINT('Ctrl Pts',(5.75088691944599,15.2,8.67522990206619));
#211911=CARTESIAN_POINT('Ctrl Pts',(5.75244151836787,15.2,8.6770616323184));
#211912=CARTESIAN_POINT('Ctrl Pts',(5.75403566598394,15.2,8.67892862750911));
#211913=CARTESIAN_POINT('Ctrl Pts',(5.7556298136,15.2,8.68079562269983));
#211914=CARTESIAN_POINT('Ctrl Pts',(5.75726351227137,15.2,8.68269788279138));
#211915=CARTESIAN_POINT('Ctrl Pts',(5.75893665987552,15.2,8.6846344171362));
#211916=CARTESIAN_POINT('Ctrl Pts',(5.76060980763166,15.2,8.68657095165691));
#211917=CARTESIAN_POINT('Ctrl Pts',(5.76232240510937,15.2,8.68854176053192));
#211918=CARTESIAN_POINT('Ctrl Pts',(5.76407435470751,15.2,8.69054588022672));
#211919=CARTESIAN_POINT('Ctrl Pts',(5.76582630414653,15.2,8.69254999973948));
#211920=CARTESIAN_POINT('Ctrl Pts',(5.76761760416457,15.2,8.69458743088663));
#211921=CARTESIAN_POINT('Ctrl Pts',(5.76944815559981,15.2,8.6966572326462));
#211922=CARTESIAN_POINT('Ctrl Pts',(5.77127870703505,15.2,8.69872703440579));
#211923=CARTESIAN_POINT('Ctrl Pts',(5.77314850964208,15.2,8.70082920789601));
#211924=CARTESIAN_POINT('Ctrl Pts',(5.77505746415434,15.2,8.70296283865045));
#211925=CARTESIAN_POINT('Ctrl Pts',(5.77696641866661,15.2,8.70509646940489));
#211926=CARTESIAN_POINT('Ctrl Pts',(5.77891452415813,15.2,8.70726155765079));
#211927=CARTESIAN_POINT('Ctrl Pts',(5.78090168058329,15.2,8.70945721048562));
#211928=CARTESIAN_POINT('Ctrl Pts',(5.78288883718896,15.2,8.7116528635199));
#211929=CARTESIAN_POINT('Ctrl Pts',(5.78491504540668,15.2,8.71387908124878));
#211930=CARTESIAN_POINT('Ctrl Pts',(5.78698020310426,15.2,8.716134994373));
#211931=CARTESIAN_POINT('Ctrl Pts',(5.78938955347004,15.2,8.71876689271056));
#211932=CARTESIAN_POINT('Ctrl Pts',(5.79185192008576,15.2,8.72143920784557));
#211933=CARTESIAN_POINT('Ctrl Pts',(5.79436714077323,15.2,8.72415059477162));
#211934=CARTESIAN_POINT('Ctrl Pts',(5.79652304447141,15.2,8.72647464097966));
#211935=CARTESIAN_POINT('Ctrl Pts',(5.79871778110668,15.2,8.7288273938155));
#211936=CARTESIAN_POINT('Ctrl Pts',(5.80095124864676,15.2,8.73120802811313));
#211937=CARTESIAN_POINT('Ctrl Pts',(5.80318471598397,15.2,8.73358866219452));
#211938=CARTESIAN_POINT('Ctrl Pts',(5.80545691140975,15.2,8.73599717787366));
#211939=CARTESIAN_POINT('Ctrl Pts',(5.8077677368241,15.2,8.73843276711731));
#211940=CARTESIAN_POINT('Ctrl Pts',(5.81123397515551,15.2,8.74208615120402));
#211941=CARTESIAN_POINT('Ctrl Pts',(5.81478712865559,15.2,8.74580045114671));
#211942=CARTESIAN_POINT('Ctrl Pts',(5.8184268494977,15.2,8.74957302074075));
#211943=CARTESIAN_POINT('Ctrl Pts',(5.82085332991218,15.2,8.75208806698448));
#211944=CARTESIAN_POINT('Ctrl Pts',(5.82331828425553,15.2,8.75462901294099));
#211945=CARTESIAN_POINT('Ctrl Pts',(5.82582161075935,15.2,8.75719509827611));
#211946=CARTESIAN_POINT('Ctrl Pts',(5.82832493726318,15.2,8.75976118361123));
#211947=CARTESIAN_POINT('Ctrl Pts',(5.83086663531317,15.2,8.76235240659527));
#211948=CARTESIAN_POINT('Ctrl Pts',(5.8334466008011,15.2,8.76496802491582));
#211949=CARTESIAN_POINT('Ctrl Pts',(5.83602656652336,15.2,8.76758364347396));
#211950=CARTESIAN_POINT('Ctrl Pts',(5.83864480067538,15.2,8.77022365471015));
#211951=CARTESIAN_POINT('Ctrl Pts',(5.84130119832277,15.2,8.77288733252363));
#211952=CARTESIAN_POINT('Ctrl Pts',(5.84395759572888,15.2,8.77555101009516));
#211953=CARTESIAN_POINT('Ctrl Pts',(5.84665215749663,15.2,8.77823835307859));
#211954=CARTESIAN_POINT('Ctrl Pts',(5.84938477789897,15.2,8.78094864964775));
#211955=CARTESIAN_POINT('Ctrl Pts',(5.85211739830131,15.2,8.78365894621693));
#211956=CARTESIAN_POINT('Ctrl Pts',(5.8548880786423,15.2,8.78639219407594));
#211957=CARTESIAN_POINT('Ctrl Pts',(5.85769671312197,15.2,8.7891476995582));
#211958=CARTESIAN_POINT('Ctrl Pts',(5.86050534760164,15.2,8.79190320504047));
#211959=CARTESIAN_POINT('Ctrl Pts',(5.86335193650951,15.2,8.79468096380633));
#211960=CARTESIAN_POINT('Ctrl Pts',(5.86623637490215,15.2,8.79748029545316));
#211961=CARTESIAN_POINT('Ctrl Pts',(5.86864007365003,15.2,8.79981307191029));
#211962=CARTESIAN_POINT('Ctrl Pts',(5.87107005561963,15.2,8.80216082902547));
#211963=CARTESIAN_POINT('Ctrl Pts',(5.87352626172862,15.2,8.80452317819096));
#211964=CARTESIAN_POINT('Ctrl Pts',(5.87598246783761,15.2,8.80688552735646));
#211965=CARTESIAN_POINT('Ctrl Pts',(5.87846489537969,15.2,8.8092624695595));
#211966=CARTESIAN_POINT('Ctrl Pts',(5.88097348522543,15.2,8.81165362224742));
#211967=CARTESIAN_POINT('Ctrl Pts',(5.88348207507117,15.2,8.81404477493533));
#211968=CARTESIAN_POINT('Ctrl Pts',(5.88601682607281,15.2,8.81645014055365));
#211969=CARTESIAN_POINT('Ctrl Pts',(5.88857767739089,15.2,8.81886933985848));
#211970=CARTESIAN_POINT('Ctrl Pts',(5.89113852870896,15.2,8.82128853916331));
#211971=CARTESIAN_POINT('Ctrl Pts',(5.89372547933051,15.2,8.82372157627962));
#211972=CARTESIAN_POINT('Ctrl Pts',(5.89633846807914,15.2,8.82616807884836));
#211973=CARTESIAN_POINT('Ctrl Pts',(5.89895145682779,15.2,8.82861458141711));
#211974=CARTESIAN_POINT('Ctrl Pts',(5.90159048412528,15.2,8.83107455085408));
#211975=CARTESIAN_POINT('Ctrl Pts',(5.9042554862901,15.2,8.83354762503194));
#211976=CARTESIAN_POINT('Ctrl Pts',(5.90745348877168,15.2,8.83651531393756));
#211977=CARTESIAN_POINT('Ctrl Pts',(5.9106888972146,15.2,8.83950187118285));
#211978=CARTESIAN_POINT('Ctrl Pts',(5.9139616034265,15.2,8.84250668140577));
#211979=CARTESIAN_POINT('Ctrl Pts',(5.91668885870217,15.2,8.84501069001585));
#211980=CARTESIAN_POINT('Ctrl Pts',(5.91944201490142,15.2,8.84752737572535));
#211981=CARTESIAN_POINT('Ctrl Pts',(5.92222100892737,15.2,8.85005638598975));
#211982=CARTESIAN_POINT('Ctrl Pts',(5.92500000295333,15.2,8.85258539625415));
#211983=CARTESIAN_POINT('Ctrl Pts',(5.9278048358607,15.2,8.85512673271699));
#211984=CARTESIAN_POINT('Ctrl Pts',(5.93063544453991,15.2,8.85768004959138));
#211985=CARTESIAN_POINT('Ctrl Pts',(5.93346605321913,15.2,8.86023336646575));
#211986=CARTESIAN_POINT('Ctrl Pts',(5.93632243747956,15.2,8.86279866447656));
#211987=CARTESIAN_POINT('Ctrl Pts',(5.93920453456154,15.2,8.86537560232316));
#211988=CARTESIAN_POINT('Ctrl Pts',(5.94266305093427,15.2,8.86846792762673));
#211989=CARTESIAN_POINT('Ctrl Pts',(5.94615859363737,15.2,8.87157701808228));
#211990=CARTESIAN_POINT('Ctrl Pts',(5.94969105308986,15.2,8.87470229238431));
#211991=CARTESIAN_POINT('Ctrl Pts',(5.95322351286323,15.2,8.87782756697023));
#211992=CARTESIAN_POINT('Ctrl Pts',(5.95679289023178,15.2,8.88096902934102));
#211993=CARTESIAN_POINT('Ctrl Pts',(5.96039907492991,15.2,8.88412610993042));
#211994=CARTESIAN_POINT('Ctrl Pts',(5.96340422868123,15.2,8.88675701027819));
#211995=CARTESIAN_POINT('Ctrl Pts',(5.96643494304858,15.2,8.88939875880627));
#211996=CARTESIAN_POINT('Ctrl Pts',(5.96949115429991,15.2,8.89205103089015));
#211997=CARTESIAN_POINT('Ctrl Pts',(5.97254736555123,15.2,8.89470330297401));
#211998=CARTESIAN_POINT('Ctrl Pts',(5.97562907338701,15.2,8.8973660997816));
#211999=CARTESIAN_POINT('Ctrl Pts',(5.978736214794,15.2,8.90003910436029));
#212000=CARTESIAN_POINT('Ctrl Pts',(5.98184335620099,15.2,8.90271210893899));
#212001=CARTESIAN_POINT('Ctrl Pts',(5.98497593003309,15.2,8.90539531874586));
#212002=CARTESIAN_POINT('Ctrl Pts',(5.98813387364629,15.2,8.9080884240939));
#212003=CARTESIAN_POINT('Ctrl Pts',(5.99066022833032,15.2,8.91024290819619));
#212004=CARTESIAN_POINT('Ctrl Pts',(5.99320281850387,15.2,8.91240372497264));
#212005=CARTESIAN_POINT('Ctrl Pts',(5.99576161201585,15.2,8.91457071457287));
#212006=CARTESIAN_POINT('Ctrl Pts',(5.99832040587646,15.2,8.91673770446834));
#212007=CARTESIAN_POINT('Ctrl Pts',(6.00089540309832,15.2,8.9189108695436));
#212008=CARTESIAN_POINT('Ctrl Pts',(6.00348657092596,15.2,8.92109005154954));
#212009=CARTESIAN_POINT('Ctrl Pts',(6.00607773840056,15.2,8.92326923325856));
#212010=CARTESIAN_POINT('Ctrl Pts',(6.00868507520109,15.2,8.92545443323651));
#212011=CARTESIAN_POINT('Ctrl Pts',(6.0113085493189,15.2,8.92764549611256));
#212012=CARTESIAN_POINT('Ctrl Pts',(6.01393202379415,15.2,8.92983655928714));
#212013=CARTESIAN_POINT('Ctrl Pts',(6.01657163575746,15.2,8.93203348492911));
#212014=CARTESIAN_POINT('Ctrl Pts',(6.01922735095881,15.2,8.93423612143842));
#212015=CARTESIAN_POINT('Ctrl Pts',(6.02188306579832,15.2,8.93643875764762));
#212016=CARTESIAN_POINT('Ctrl Pts',(6.02455488531346,15.2,8.93864710454405));
#212017=CARTESIAN_POINT('Ctrl Pts',(6.02724277489327,15.2,8.94086100969541));
#212018=CARTESIAN_POINT('Ctrl Pts',(6.03060263714272,15.2,8.94362839136083));
#212019=CARTESIAN_POINT('Ctrl Pts',(6.03398761037835,15.2,8.94640446026837));
#212020=CARTESIAN_POINT('Ctrl Pts',(6.03739762829368,15.2,8.94918892255957));
#212021=CARTESIAN_POINT('Ctrl Pts',(6.04012564277461,15.2,8.95141649251393));
#212022=CARTESIAN_POINT('Ctrl Pts',(6.04286968619365,15.2,8.95364943538289));
#212023=CARTESIAN_POINT('Ctrl Pts',(6.045629724734,15.2,8.95588760394965));
#212024=CARTESIAN_POINT('Ctrl Pts',(6.04976978216848,15.2,8.95924485649484));
#212025=CARTESIAN_POINT('Ctrl Pts',(6.05394583034862,15.2,8.96261386415592));
#212026=CARTESIAN_POINT('Ctrl Pts',(6.05815775554797,15.2,8.9659941387151));
#212027=CARTESIAN_POINT('Ctrl Pts',(6.06096570593592,15.2,8.96824765529257));
#212028=CARTESIAN_POINT('Ctrl Pts',(6.06378960094112,15.2,8.97050617962673));
#212029=CARTESIAN_POINT('Ctrl Pts',(6.06662940743087,15.2,8.9727695663617));
#212030=CARTESIAN_POINT('Ctrl Pts',(6.07017916534957,15.2,8.97559879962621));
#212031=CARTESIAN_POINT('Ctrl Pts',(6.07375378580201,15.2,8.9784356338825));
#212032=CARTESIAN_POINT('Ctrl Pts',(6.0773532012207,15.2,8.98127978964699));
#212033=CARTESIAN_POINT('Ctrl Pts',(6.08023273332025,15.2,8.98355511407257));
#212034=CARTESIAN_POINT('Ctrl Pts',(6.08312813661161,15.2,8.98583512653592));
#212035=CARTESIAN_POINT('Ctrl Pts',(6.0860393734979,15.2,8.98811968424841));
#212036=CARTESIAN_POINT('Ctrl Pts',(6.08895061078086,15.2,8.99040424227218));
#212037=CARTESIAN_POINT('Ctrl Pts',(6.09187768442181,15.2,8.99269334799673));
#212038=CARTESIAN_POINT('Ctrl Pts',(6.09482055897272,15.2,8.99498686139996));
#212039=CARTESIAN_POINT('Ctrl Pts',(6.09849915196087,15.2,8.99785375299776));
#212040=CARTESIAN_POINT('Ctrl Pts',(6.10220243617994,15.2,9.00072753154841));
#212041=CARTESIAN_POINT('Ctrl Pts',(6.10593034319584,15.2,9.00360793141007));
#212042=CARTESIAN_POINT('Ctrl Pts',(6.1096582498054,15.2,9.00648833095775));
#212043=CARTESIAN_POINT('Ctrl Pts',(6.11341078093621,15.2,9.00937535045964));
#212044=CARTESIAN_POINT('Ctrl Pts',(6.11718786843918,15.2,9.01226872667151));
#212045=CARTESIAN_POINT('Ctrl Pts',(6.12020953893558,15.2,9.01458342801947));
#212046=CARTESIAN_POINT('Ctrl Pts',(6.12324692625293,15.2,9.01690219692061));
#212047=CARTESIAN_POINT('Ctrl Pts',(6.12629999547488,15.2,9.01922490099164));
#212048=CARTESIAN_POINT('Ctrl Pts',(6.13011633179433,15.2,9.0221282809222));
#212049=CARTESIAN_POINT('Ctrl Pts',(6.13395717168436,15.2,9.02503780981607));
#212050=CARTESIAN_POINT('Ctrl Pts',(6.13782245024366,15.2,9.02795322725989));
#212051=CARTESIAN_POINT('Ctrl Pts',(6.14323384031094,15.2,9.03203481174479));
#212052=CARTESIAN_POINT('Ctrl Pts',(6.14869312389253,15.2,9.03612794009108));
#212053=CARTESIAN_POINT('Ctrl Pts',(6.15420012023107,15.2,9.04023191639174));
#212054=CARTESIAN_POINT('Ctrl Pts',(6.15734697497541,15.2,9.04257704547816));
#212055=CARTESIAN_POINT('Ctrl Pts',(6.16050940936771,15.2,9.04492571573077));
#212056=CARTESIAN_POINT('Ctrl Pts',(6.16368738877356,15.2,9.04727780081605));
#212057=CARTESIAN_POINT('Ctrl Pts',(6.16765986335562,15.2,9.050217907413));
#212058=CARTESIAN_POINT('Ctrl Pts',(6.17165662644063,15.2,9.05316334821277));
#212059=CARTESIAN_POINT('Ctrl Pts',(6.17567761180603,15.2,9.0561138750317));
#212060=CARTESIAN_POINT('Ctrl Pts',(6.17889440027367,15.2,9.05847429661549));
#212061=CARTESIAN_POINT('Ctrl Pts',(6.18212669035232,15.2,9.06083797404374));
#212062=CARTESIAN_POINT('Ctrl Pts',(6.1853744475309,15.2,9.06320478089528));
#212063=CARTESIAN_POINT('Ctrl Pts',(6.19024608285629,15.2,9.06675499085012));
#212064=CARTESIAN_POINT('Ctrl Pts',(6.19515251938776,15.2,9.07031224414614));
#212065=CARTESIAN_POINT('Ctrl Pts',(6.20009363979154,15.2,9.07387612201664));
#212066=CARTESIAN_POINT('Ctrl Pts',(6.20421124027763,15.2,9.07684602034995));
#212067=CARTESIAN_POINT('Ctrl Pts',(6.20835292641652,15.2,9.07982051850473));
#212068=CARTESIAN_POINT('Ctrl Pts',(6.21251863101882,15.2,9.08279937851827));
#212069=CARTESIAN_POINT('Ctrl Pts',(6.21585119442823,15.2,9.08518246633427));
#212070=CARTESIAN_POINT('Ctrl Pts',(6.21919913004318,15.2,9.08756834573277));
#212071=CARTESIAN_POINT('Ctrl Pts',(6.22256240143333,15.2,9.08995689509278));
#212072=CARTESIAN_POINT('Ctrl Pts',(6.22592567328172,15.2,9.09234544477823));
#212073=CARTESIAN_POINT('Ctrl Pts',(6.22930428199803,15.2,9.09473666661102));
#212074=CARTESIAN_POINT('Ctrl Pts',(6.23269819251648,15.2,9.0971304382416));
#212075=CARTESIAN_POINT('Ctrl Pts',(6.23694058043335,15.2,9.10012265261674));
#212076=CARTESIAN_POINT('Ctrl Pts',(6.2412068781049,15.2,9.10311885343798));
#212077=CARTESIAN_POINT('Ctrl Pts',(6.24549701527722,15.2,9.10611880782661));
#212078=CARTESIAN_POINT('Ctrl Pts',(6.24892912473451,15.2,9.10851877114132));
#212079=CARTESIAN_POINT('Ctrl Pts',(6.25237649344894,15.2,9.11092113838697));
#212080=CARTESIAN_POINT('Ctrl Pts',(6.25583908344209,15.2,9.11332579085681));
#212081=CARTESIAN_POINT('Ctrl Pts',(6.25930167390702,15.2,9.1157304436543));
#212082=CARTESIAN_POINT('Ctrl Pts',(6.26277948772895,15.2,9.11813738085479));
#212083=CARTESIAN_POINT('Ctrl Pts',(6.26627248897488,15.2,9.12054648904165));
#212084=CARTESIAN_POINT('Ctrl Pts',(6.27063874029432,15.2,9.1235578741111));
#212085=CARTESIAN_POINT('Ctrl Pts',(6.27502872253217,15.2,9.12657264784901));
#212086=CARTESIAN_POINT('Ctrl Pts',(6.27944236630229,15.2,9.12959058800162));
#212087=CARTESIAN_POINT('Ctrl Pts',(6.28297328102973,15.2,9.13200493992634));
#212088=CARTESIAN_POINT('Ctrl Pts',(6.2865193398131,15.2,9.13442131805804));
#212089=CARTESIAN_POINT('Ctrl Pts',(6.2900805059093,15.2,9.13683960863792));
#212090=CARTESIAN_POINT('Ctrl Pts',(6.29364167249071,15.2,9.13925789954729));
#212091=CARTESIAN_POINT('Ctrl Pts',(6.29721794913749,15.2,9.14167810184575));
#212092=CARTESIAN_POINT('Ctrl Pts',(6.30080929699988,15.2,9.14410010419998));
#212093=CARTESIAN_POINT('Ctrl Pts',(6.30529848158322,15.2,9.14712760697777));
#212094=CARTESIAN_POINT('Ctrl Pts',(6.30981121798725,15.2,9.15015792190452));
#212095=CARTESIAN_POINT('Ctrl Pts',(6.31434743599403,15.2,9.1531908312933));
#212096=CARTESIAN_POINT('Ctrl Pts',(6.31797641010277,15.2,9.15561715860597));
#212097=CARTESIAN_POINT('Ctrl Pts',(6.32162041321341,15.2,9.1580451462793));
#212098=CARTESIAN_POINT('Ctrl Pts',(6.32527940913498,15.2,9.16047468363608));
#212099=CARTESIAN_POINT('Ctrl Pts',(6.32893840555508,15.2,9.16290422132388));
#212100=CARTESIAN_POINT('Ctrl Pts',(6.33261239449883,15.2,9.16533530832297));
#212101=CARTESIAN_POINT('Ctrl Pts',(6.33630134103322,15.2,9.16776783723332));
#212102=CARTESIAN_POINT('Ctrl Pts',(6.3399902875676,15.2,9.17020036614366));
#212103=CARTESIAN_POINT('Ctrl Pts',(6.34369419106484,15.2,9.17263433475696));
#212104=CARTESIAN_POINT('Ctrl Pts',(6.34741301682459,15.2,9.17506963638982));
#212105=CARTESIAN_POINT('Ctrl Pts',(6.35113184207766,15.2,9.17750493769088));
#212106=CARTESIAN_POINT('Ctrl Pts',(6.35486558978681,15.2,9.17994157150321));
#212107=CARTESIAN_POINT('Ctrl Pts',(6.35861422249733,15.2,9.18237942898165));
#212108=CARTESIAN_POINT('Ctrl Pts',(6.36142569715791,15.2,9.18420782217352));
#212109=CARTESIAN_POINT('Ctrl Pts',(6.36424554477858,15.2,9.18603690593376));
#212110=CARTESIAN_POINT('Ctrl Pts',(6.36707375092508,15.2,9.18786663261722));
#212111=CARTESIAN_POINT('Ctrl Pts',(6.36990195707159,15.2,9.18969635930068));
#212112=CARTESIAN_POINT('Ctrl Pts',(6.3727385222342,15.2,9.19152673040077));
#212113=CARTESIAN_POINT('Ctrl Pts',(6.3755834298797,15.2,9.19335770058416));
#212114=CARTESIAN_POINT('Ctrl Pts',(6.37937664041824,15.2,9.19579899438376));
#212115=CARTESIAN_POINT('Ctrl Pts',(6.38318468323784,15.2,9.19824135485738));
#212116=CARTESIAN_POINT('Ctrl Pts',(6.38700752301916,15.2,9.20068467400165));
#212117=CARTESIAN_POINT('Ctrl Pts',(6.38987465259472,15.2,9.2025171631934));
#212118=CARTESIAN_POINT('Ctrl Pts',(6.39275010465566,15.2,9.20435019368994));
#212119=CARTESIAN_POINT('Ctrl Pts',(6.3956338647306,15.2,9.20618372029832));
#212120=CARTESIAN_POINT('Ctrl Pts',(6.39851762480555,15.2,9.20801724690669));
#212121=CARTESIAN_POINT('Ctrl Pts',(6.40140969210666,15.2,9.20985126946672));
#212122=CARTESIAN_POINT('Ctrl Pts',(6.40431005270888,15.2,9.2116857450667));
#212123=CARTESIAN_POINT('Ctrl Pts',(6.40914398722156,15.2,9.21474320451106));
#212124=CARTESIAN_POINT('Ctrl Pts',(6.41400095629875,15.2,9.21780192074995));
#212125=CARTESIAN_POINT('Ctrl Pts',(6.41888089067255,15.2,9.22086169429155));
#212126=CARTESIAN_POINT('Ctrl Pts',(6.42180885119044,15.2,9.22269755834981));
#212127=CARTESIAN_POINT('Ctrl Pts',(6.42474507849111,15.2,9.22453380161966));
#212128=CARTESIAN_POINT('Ctrl Pts',(6.42768955869695,15.2,9.22637038335299));
#212129=CARTESIAN_POINT('Ctrl Pts',(6.43063403890278,15.2,9.22820696508631));
#212130=CARTESIAN_POINT('Ctrl Pts',(6.43358677037976,15.2,9.23004388566625));
#212131=CARTESIAN_POINT('Ctrl Pts',(6.43654773856273,15.2,9.23188109939114));
#212132=CARTESIAN_POINT('Ctrl Pts',(6.44148268571366,15.2,9.23494312237719));
#212133=CARTESIAN_POINT('Ctrl Pts',(6.44644051555031,15.2,9.2380059652049));
#212134=CARTESIAN_POINT('Ctrl Pts',(6.45142115263176,15.2,9.24106943131595));
#212135=CARTESIAN_POINT('Ctrl Pts',(6.45440953531495,15.2,9.24290751124971));
#212136=CARTESIAN_POINT('Ctrl Pts',(6.45740612943379,15.2,9.24474581541689));
#212137=CARTESIAN_POINT('Ctrl Pts',(6.46041091966327,15.2,9.24658430189244));
#212138=CARTESIAN_POINT('Ctrl Pts',(6.46441730572614,15.2,9.24903561663653));
#212139=CARTESIAN_POINT('Ctrl Pts',(6.46843826381987,15.2,9.25148725543762));
#212140=CARTESIAN_POINT('Ctrl Pts',(6.47247375573047,15.2,9.25393912024831));
#212141=CARTESIAN_POINT('Ctrl Pts',(6.47550037480087,15.2,9.25577801893985));
#212142=CARTESIAN_POINT('Ctrl Pts',(6.47853516907962,15.2,9.25761704504969));
#212143=CARTESIAN_POINT('Ctrl Pts',(6.48157812367667,15.2,9.25945615627452));
#212144=CARTESIAN_POINT('Ctrl Pts',(6.48462107827373,15.2,9.26129526749935));
#212145=CARTESIAN_POINT('Ctrl Pts',(6.48767219327857,15.2,9.26313446489919));
#212146=CARTESIAN_POINT('Ctrl Pts',(6.49073145383298,15.2,9.26497370608236));
#212147=CARTESIAN_POINT('Ctrl Pts',(6.49379071494315,15.2,9.26681294759966));
#212148=CARTESIAN_POINT('Ctrl Pts',(6.49685812047229,15.2,9.26865223348365));
#212149=CARTESIAN_POINT('Ctrl Pts',(6.49993365567036,15.2,9.27049152391762));
#212150=CARTESIAN_POINT('Ctrl Pts',(6.50300919030972,15.2,9.27233081401745));
#212151=CARTESIAN_POINT('Ctrl Pts',(6.50609285466531,15.2,9.27417010731729));
#212152=CARTESIAN_POINT('Ctrl Pts',(6.50918463326203,15.2,9.2760093639588));
#212153=CARTESIAN_POINT('Ctrl Pts',(6.51433759777712,15.2,9.27907479180602));
#212154=CARTESIAN_POINT('Ctrl Pts',(6.51951310256993,15.2,9.28214011708603));
#212155=CARTESIAN_POINT('Ctrl Pts',(6.52471107484504,15.2,9.28520515432246));
#212156=CARTESIAN_POINT('Ctrl Pts',(6.5278298580968,15.2,9.2870441765975));
#212157=CARTESIAN_POINT('Ctrl Pts',(6.5309567305216,15.2,9.28888309506723));
#212158=CARTESIAN_POINT('Ctrl Pts',(6.53409167561673,15.2,9.29072187020875));
#212159=CARTESIAN_POINT('Ctrl Pts',(6.53827160222041,15.2,9.29317357028608));
#212160=CARTESIAN_POINT('Ctrl Pts',(6.54246588093787,15.2,9.2956250134468));
#212161=CARTESIAN_POINT('Ctrl Pts',(6.54667447553679,15.2,9.29807610885757));
#212162=CARTESIAN_POINT('Ctrl Pts',(6.55088307070914,15.2,9.30052720460229));
#212163=CARTESIAN_POINT('Ctrl Pts',(6.55510598126924,15.2,9.30297795047366));
#212164=CARTESIAN_POINT('Ctrl Pts',(6.55934317051944,15.2,9.30542825428499));
#212165=CARTESIAN_POINT('Ctrl Pts',(6.56358035919234,15.2,9.30787855776247));
#212166=CARTESIAN_POINT('Ctrl Pts',(6.56783182778595,15.2,9.31032841916913));
#212167=CARTESIAN_POINT('Ctrl Pts',(6.57209753776912,15.2,9.31277774535785));
#212168=CARTESIAN_POINT('Ctrl Pts',(6.57636324833349,15.2,9.31522707188029));
#212169=CARTESIAN_POINT('Ctrl Pts',(6.58064320086586,15.2,9.31767586224991));
#212170=CARTESIAN_POINT('Ctrl Pts',(6.58493735876655,15.2,9.32012402804999));
#212171=CARTESIAN_POINT('Ctrl Pts',(6.58815797689953,15.2,9.32196015223327));
#212172=CARTESIAN_POINT('Ctrl Pts',(6.59138658726553,15.2,9.32379592456658));
#212173=CARTESIAN_POINT('Ctrl Pts',(6.5946231714389,15.2,9.32563130679159));
#212174=CARTESIAN_POINT('Ctrl Pts',(6.59785975561227,15.2,9.3274666890166));
#212175=CARTESIAN_POINT('Ctrl Pts',(6.60110431487729,15.2,9.32930168082));
#212176=CARTESIAN_POINT('Ctrl Pts',(6.60435683408735,15.2,9.33113624313671));
#212177=CARTESIAN_POINT('Ctrl Pts',(6.60760935329742,15.2,9.33297080545342));
#212178=CARTESIAN_POINT('Ctrl Pts',(6.61086983042388,15.2,9.33480493775014));
#212179=CARTESIAN_POINT('Ctrl Pts',(6.61413825151238,15.2,9.33663860205858));
#212180=CARTESIAN_POINT('Ctrl Pts',(6.61740667319464,15.2,9.33847226670014));
#212181=CARTESIAN_POINT('Ctrl Pts',(6.62068303892081,15.2,9.34030546433323));
#212182=CARTESIAN_POINT('Ctrl Pts',(6.62396733323254,15.2,9.34213816089119));
#212183=CARTESIAN_POINT('Ctrl Pts',(6.62725162694763,15.2,9.3439708571162));
#212184=CARTESIAN_POINT('Ctrl Pts',(6.6305438517456,15.2,9.34580305239956));
#212185=CARTESIAN_POINT('Ctrl Pts',(6.63384398933474,15.2,9.34763470795797));
#212186=CARTESIAN_POINT('Ctrl Pts',(6.63934421884978,15.2,9.35068746733289));
#212187=CARTESIAN_POINT('Ctrl Pts',(6.64486642765394,15.2,9.3537387206851));
#212188=CARTESIAN_POINT('Ctrl Pts',(6.65041053341855,15.2,9.35678826917066));
#212189=CARTESIAN_POINT('Ctrl Pts',(6.65373699675646,15.2,9.35861799819552));
#212190=CARTESIAN_POINT('Ctrl Pts',(6.65707134275782,15.2,9.36044711540242));
#212191=CARTESIAN_POINT('Ctrl Pts',(6.66041356410864,15.2,9.36227560222762));
#212192=CARTESIAN_POINT('Ctrl Pts',(6.66375578545946,15.2,9.36410408905281));
#212193=CARTESIAN_POINT('Ctrl Pts',(6.6671058818474,15.2,9.36593194382869));
#212194=CARTESIAN_POINT('Ctrl Pts',(6.67046385399994,15.2,9.36775917499999));
#212195=CARTESIAN_POINT('Ctrl Pts',(6.57080831899994,15.2,8.02901631899999));
#212196=CARTESIAN_POINT('Ctrl Pts',(6.57080831899994,11.6,8.02901631899999));
#212197=CARTESIAN_POINT('Ctrl Pts',(6.57090674099994,15.2,8.02916024099999));
#212198=CARTESIAN_POINT('Ctrl Pts',(6.57090674099994,11.6,8.02916024099999));
#212199=CARTESIAN_POINT('Ctrl Pts',(6.57110695099994,15.2,8.02945316199999));
#212200=CARTESIAN_POINT('Ctrl Pts',(6.57110695099994,11.6,8.02945316199999));
#212201=CARTESIAN_POINT('Ctrl Pts',(6.57141009899994,15.2,8.02989715799999));
#212202=CARTESIAN_POINT('Ctrl Pts',(6.57141009899994,11.6,8.02989715799999));
#212203=CARTESIAN_POINT('Ctrl Pts',(6.57181801899994,15.2,8.03049556499998));
#212204=CARTESIAN_POINT('Ctrl Pts',(6.57181801899994,11.6,8.03049556499998));
#212205=CARTESIAN_POINT('Ctrl Pts',(6.57233322399994,15.2,8.03125297399998));
#212206=CARTESIAN_POINT('Ctrl Pts',(6.57233322399994,11.6,8.03125297399998));
#212207=CARTESIAN_POINT('Ctrl Pts',(6.57285600599994,15.2,8.03202318499999));
#212208=CARTESIAN_POINT('Ctrl Pts',(6.57285600599994,11.6,8.03202318499999));
#212209=CARTESIAN_POINT('Ctrl Pts',(6.57338334999994,15.2,8.03280179799999));
#212210=CARTESIAN_POINT('Ctrl Pts',(6.57338334999994,11.6,8.03280179799999));
#212211=CARTESIAN_POINT('Ctrl Pts',(6.57391522699994,15.2,8.03358879999998));
#212212=CARTESIAN_POINT('Ctrl Pts',(6.57391522699994,11.6,8.03358879999998));
#212213=CARTESIAN_POINT('Ctrl Pts',(6.57445160499995,15.2,8.03438417899999));
#212214=CARTESIAN_POINT('Ctrl Pts',(6.57445160499995,11.6,8.03438417899999));
#212215=CARTESIAN_POINT('Ctrl Pts',(6.57499245699994,15.2,8.03518792399998));
#212216=CARTESIAN_POINT('Ctrl Pts',(6.57499245699994,11.6,8.03518792399998));
#212217=CARTESIAN_POINT('Ctrl Pts',(6.57553775199994,15.2,8.03600002099999));
#212218=CARTESIAN_POINT('Ctrl Pts',(6.57553775199994,11.6,8.03600002099999));
#212219=CARTESIAN_POINT('Ctrl Pts',(6.57608745899994,15.2,8.03682046099999));
#212220=CARTESIAN_POINT('Ctrl Pts',(6.57608745899994,11.6,8.03682046099999));
#212221=CARTESIAN_POINT('Ctrl Pts',(6.57664155099994,15.2,8.03764922899998));
#212222=CARTESIAN_POINT('Ctrl Pts',(6.57664155099994,11.6,8.03764922899998));
#212223=CARTESIAN_POINT('Ctrl Pts',(6.57719999699995,15.2,8.03848631499999));
#212224=CARTESIAN_POINT('Ctrl Pts',(6.57719999699995,11.6,8.03848631499999));
#212225=CARTESIAN_POINT('Ctrl Pts',(6.57776276799994,15.2,8.03933170599999));
#212226=CARTESIAN_POINT('Ctrl Pts',(6.57776276799994,11.6,8.03933170599999));
#212227=CARTESIAN_POINT('Ctrl Pts',(6.57832983599994,15.2,8.04018538999999));
#212228=CARTESIAN_POINT('Ctrl Pts',(6.57832983599994,11.6,8.04018538999999));
#212229=CARTESIAN_POINT('Ctrl Pts',(6.57890117199995,15.2,8.04104735799999));
#212230=CARTESIAN_POINT('Ctrl Pts',(6.57890117199995,11.6,8.04104735799999));
#212231=CARTESIAN_POINT('Ctrl Pts',(6.57947674699995,15.2,8.04191759399998));
#212232=CARTESIAN_POINT('Ctrl Pts',(6.57947674699995,11.6,8.04191759399998));
#212233=CARTESIAN_POINT('Ctrl Pts',(6.58005653199995,15.2,8.04279608999998));
#212234=CARTESIAN_POINT('Ctrl Pts',(6.58005653199995,11.6,8.04279608999998));
#212235=CARTESIAN_POINT('Ctrl Pts',(6.58064049899994,15.2,8.04368283299999));
#212236=CARTESIAN_POINT('Ctrl Pts',(6.58064049899994,11.6,8.04368283299999));
#212237=CARTESIAN_POINT('Ctrl Pts',(6.58122861999995,15.2,8.04457781099998));
#212238=CARTESIAN_POINT('Ctrl Pts',(6.58122861999995,11.6,8.04457781099998));
#212239=CARTESIAN_POINT('Ctrl Pts',(6.58182086699994,15.2,8.04548101299999));
#212240=CARTESIAN_POINT('Ctrl Pts',(6.58182086699994,11.6,8.04548101299999));
#212241=CARTESIAN_POINT('Ctrl Pts',(6.58241721199994,15.2,8.04639242699999));
#212242=CARTESIAN_POINT('Ctrl Pts',(6.58241721199994,11.6,8.04639242699999));
#212243=CARTESIAN_POINT('Ctrl Pts',(6.58301762599995,15.2,8.04731204199998));
#212244=CARTESIAN_POINT('Ctrl Pts',(6.58301762599995,11.6,8.04731204199998));
#212245=CARTESIAN_POINT('Ctrl Pts',(6.58362208299994,15.2,8.04823984599999));
#212246=CARTESIAN_POINT('Ctrl Pts',(6.58362208299994,11.6,8.04823984599999));
#212247=CARTESIAN_POINT('Ctrl Pts',(6.58423055399994,15.2,8.04917582899999));
#212248=CARTESIAN_POINT('Ctrl Pts',(6.58423055399994,11.6,8.04917582899999));
#212249=CARTESIAN_POINT('Ctrl Pts',(6.58484301299994,15.2,8.05011997899998));
#212250=CARTESIAN_POINT('Ctrl Pts',(6.58484301299994,11.6,8.05011997899998));
#212251=CARTESIAN_POINT('Ctrl Pts',(6.58545943099995,15.2,8.05107228299999));
#212252=CARTESIAN_POINT('Ctrl Pts',(6.58545943099995,11.6,8.05107228299999));
#212253=CARTESIAN_POINT('Ctrl Pts',(6.58607978199995,15.2,8.05203273199999));
#212254=CARTESIAN_POINT('Ctrl Pts',(6.58607978199995,11.6,8.05203273199999));
#212255=CARTESIAN_POINT('Ctrl Pts',(6.58670403999994,15.2,8.05300131399999));
#212256=CARTESIAN_POINT('Ctrl Pts',(6.58670403999994,11.6,8.05300131399999));
#212257=CARTESIAN_POINT('Ctrl Pts',(6.58733217599995,15.2,8.05397801699998));
#212258=CARTESIAN_POINT('Ctrl Pts',(6.58733217599995,11.6,8.05397801699998));
#212259=CARTESIAN_POINT('Ctrl Pts',(6.58796416399994,15.2,8.05496283099998));
#212260=CARTESIAN_POINT('Ctrl Pts',(6.58796416399994,11.6,8.05496283099998));
#212261=CARTESIAN_POINT('Ctrl Pts',(6.58859997799994,15.2,8.05595574499998));
#212262=CARTESIAN_POINT('Ctrl Pts',(6.58859997799994,11.6,8.05595574499998));
#212263=CARTESIAN_POINT('Ctrl Pts',(6.58923958999994,15.2,8.05695674699999));
#212264=CARTESIAN_POINT('Ctrl Pts',(6.58923958999994,11.6,8.05695674699999));
#212265=CARTESIAN_POINT('Ctrl Pts',(6.58988297499994,15.2,8.05796582699998));
#212266=CARTESIAN_POINT('Ctrl Pts',(6.58988297499994,11.6,8.05796582699998));
#212267=CARTESIAN_POINT('Ctrl Pts',(6.59053010699994,15.2,8.05898297299999));
#212268=CARTESIAN_POINT('Ctrl Pts',(6.59053010699994,11.6,8.05898297299999));
#212269=CARTESIAN_POINT('Ctrl Pts',(6.59118095799994,15.2,8.06000817499999));
#212270=CARTESIAN_POINT('Ctrl Pts',(6.59118095799994,11.6,8.06000817499999));
#212271=CARTESIAN_POINT('Ctrl Pts',(6.59183550399994,15.2,8.06104142099999));
#212272=CARTESIAN_POINT('Ctrl Pts',(6.59183550399994,11.6,8.06104142099999));
#212273=CARTESIAN_POINT('Ctrl Pts',(6.59249371899994,15.2,8.06208270099999));
#212274=CARTESIAN_POINT('Ctrl Pts',(6.59249371899994,11.6,8.06208270099999));
#212275=CARTESIAN_POINT('Ctrl Pts',(6.59315557499994,15.2,8.06313200399998));
#212276=CARTESIAN_POINT('Ctrl Pts',(6.59315557499994,11.6,8.06313200399998));
#212277=CARTESIAN_POINT('Ctrl Pts',(6.59382104899994,15.2,8.06418931799998));
#212278=CARTESIAN_POINT('Ctrl Pts',(6.59382104899994,11.6,8.06418931799998));
#212279=CARTESIAN_POINT('Ctrl Pts',(6.59449011399994,15.2,8.06525463399998));
#212280=CARTESIAN_POINT('Ctrl Pts',(6.59449011399994,11.6,8.06525463399998));
#212281=CARTESIAN_POINT('Ctrl Pts',(6.59516274499994,15.2,8.06632794099999));
#212282=CARTESIAN_POINT('Ctrl Pts',(6.59516274499994,11.6,8.06632794099999));
#212283=CARTESIAN_POINT('Ctrl Pts',(6.59583891699994,15.2,8.06740922799998));
#212284=CARTESIAN_POINT('Ctrl Pts',(6.59583891699994,11.6,8.06740922799998));
#212285=CARTESIAN_POINT('Ctrl Pts',(6.59651860399994,15.2,8.06849848399998));
#212286=CARTESIAN_POINT('Ctrl Pts',(6.59651860399994,11.6,8.06849848399998));
#212287=CARTESIAN_POINT('Ctrl Pts',(6.59720178199994,15.2,8.06959569799999));
#212288=CARTESIAN_POINT('Ctrl Pts',(6.59720178199994,11.6,8.06959569799999));
#212289=CARTESIAN_POINT('Ctrl Pts',(6.59788842499994,15.2,8.07070086099999));
#212290=CARTESIAN_POINT('Ctrl Pts',(6.59788842499994,11.6,8.07070086099999));
#212291=CARTESIAN_POINT('Ctrl Pts',(6.59857850999994,15.2,8.07181396099999));
#212292=CARTESIAN_POINT('Ctrl Pts',(6.59857850999994,11.6,8.07181396099999));
#212293=CARTESIAN_POINT('Ctrl Pts',(6.59927200899994,15.2,8.07293498699998));
#212294=CARTESIAN_POINT('Ctrl Pts',(6.59927200899994,11.6,8.07293498699998));
#212295=CARTESIAN_POINT('Ctrl Pts',(6.59996890099994,15.2,8.07406392999999));
#212296=CARTESIAN_POINT('Ctrl Pts',(6.59996890099994,11.6,8.07406392999999));
#212297=CARTESIAN_POINT('Ctrl Pts',(6.60066915899994,15.2,8.07520077899999));
#212298=CARTESIAN_POINT('Ctrl Pts',(6.60066915899994,11.6,8.07520077899999));
#212299=CARTESIAN_POINT('Ctrl Pts',(6.60137275999994,15.2,8.07634552299999));
#212300=CARTESIAN_POINT('Ctrl Pts',(6.60137275999994,11.6,8.07634552299999));
#212301=CARTESIAN_POINT('Ctrl Pts',(6.60207967899994,15.2,8.07749815299999));
#212302=CARTESIAN_POINT('Ctrl Pts',(6.60207967899994,11.6,8.07749815299999));
#212303=CARTESIAN_POINT('Ctrl Pts',(6.60278989199995,15.2,8.07865865699998));
#212304=CARTESIAN_POINT('Ctrl Pts',(6.60278989199995,11.6,8.07865865699998));
#212305=CARTESIAN_POINT('Ctrl Pts',(6.60350337599994,15.2,8.07982702499999));
#212306=CARTESIAN_POINT('Ctrl Pts',(6.60350337599994,11.6,8.07982702499999));
#212307=CARTESIAN_POINT('Ctrl Pts',(6.60422010499994,15.2,8.08100324799998));
#212308=CARTESIAN_POINT('Ctrl Pts',(6.60422010499994,11.6,8.08100324799998));
#212309=CARTESIAN_POINT('Ctrl Pts',(6.60494005699994,15.2,8.08218731499998));
#212310=CARTESIAN_POINT('Ctrl Pts',(6.60494005699994,11.6,8.08218731499998));
#212311=CARTESIAN_POINT('Ctrl Pts',(6.60566320699994,15.2,8.08337921499999));
#212312=CARTESIAN_POINT('Ctrl Pts',(6.60566320699994,11.6,8.08337921499999));
#212313=CARTESIAN_POINT('Ctrl Pts',(6.60638953399994,15.2,8.08457893799999));
#212314=CARTESIAN_POINT('Ctrl Pts',(6.60638953399994,11.6,8.08457893799999));
#212315=CARTESIAN_POINT('Ctrl Pts',(6.60711900899994,15.2,8.08578647499999));
#212316=CARTESIAN_POINT('Ctrl Pts',(6.60711900899994,11.6,8.08578647499999));
#212317=CARTESIAN_POINT('Ctrl Pts',(6.60785161499994,15.2,8.08700181499999));
#212318=CARTESIAN_POINT('Ctrl Pts',(6.60785161499994,11.6,8.08700181499999));
#212319=CARTESIAN_POINT('Ctrl Pts',(6.60858732499994,15.2,8.08822494799998));
#212320=CARTESIAN_POINT('Ctrl Pts',(6.60858732499994,11.6,8.08822494799998));
#212321=CARTESIAN_POINT('Ctrl Pts',(6.60932611599995,15.2,8.08945586299998));
#212322=CARTESIAN_POINT('Ctrl Pts',(6.60932611599995,11.6,8.08945586299998));
#212323=CARTESIAN_POINT('Ctrl Pts',(6.61006796499994,15.2,8.09069455199998));
#212324=CARTESIAN_POINT('Ctrl Pts',(6.61006796499994,11.6,8.09069455199998));
#212325=CARTESIAN_POINT('Ctrl Pts',(6.61081285099994,15.2,8.09194100299998));
#212326=CARTESIAN_POINT('Ctrl Pts',(6.61081285099994,11.6,8.09194100299998));
#212327=CARTESIAN_POINT('Ctrl Pts',(6.61156074799995,15.2,8.09319520799999));
#212328=CARTESIAN_POINT('Ctrl Pts',(6.61156074799995,11.6,8.09319520799999));
#212329=CARTESIAN_POINT('Ctrl Pts',(6.61231163599994,15.2,8.09445715399999));
#212330=CARTESIAN_POINT('Ctrl Pts',(6.61231163599994,11.6,8.09445715399999));
#212331=CARTESIAN_POINT('Ctrl Pts',(6.61306548999994,15.2,8.09572683299999));
#212332=CARTESIAN_POINT('Ctrl Pts',(6.61306548999994,11.6,8.09572683299999));
#212333=CARTESIAN_POINT('Ctrl Pts',(6.61382228899994,15.2,8.09700423699999));
#212334=CARTESIAN_POINT('Ctrl Pts',(6.61382228899994,11.6,8.09700423699999));
#212335=CARTESIAN_POINT('Ctrl Pts',(6.61458201099994,15.2,8.09828935199998));
#212336=CARTESIAN_POINT('Ctrl Pts',(6.61458201099994,11.6,8.09828935199998));
#212337=CARTESIAN_POINT('Ctrl Pts',(6.61534463099994,15.2,8.09958217099998));
#212338=CARTESIAN_POINT('Ctrl Pts',(6.61534463099994,11.6,8.09958217099998));
#212339=CARTESIAN_POINT('Ctrl Pts',(6.61611012899994,15.2,8.10088268299998));
#212340=CARTESIAN_POINT('Ctrl Pts',(6.61611012899994,11.6,8.10088268299998));
#212341=CARTESIAN_POINT('Ctrl Pts',(6.61687848099994,15.2,8.10219087899998));
#212342=CARTESIAN_POINT('Ctrl Pts',(6.61687848099994,11.6,8.10219087899998));
#212343=CARTESIAN_POINT('Ctrl Pts',(6.61764966699994,15.2,8.10350674899999));
#212344=CARTESIAN_POINT('Ctrl Pts',(6.61764966699994,11.6,8.10350674899999));
#212345=CARTESIAN_POINT('Ctrl Pts',(6.61842366399994,15.2,8.10483028299998));
#212346=CARTESIAN_POINT('Ctrl Pts',(6.61842366399994,11.6,8.10483028299998));
#212347=CARTESIAN_POINT('Ctrl Pts',(6.61920044999994,15.2,8.10616147099999));
#212348=CARTESIAN_POINT('Ctrl Pts',(6.61920044999994,11.6,8.10616147099999));
#212349=CARTESIAN_POINT('Ctrl Pts',(6.61998000099994,15.2,8.10750030399999));
#212350=CARTESIAN_POINT('Ctrl Pts',(6.61998000099994,11.6,8.10750030399999));
#212351=CARTESIAN_POINT('Ctrl Pts',(6.62076229999994,15.2,8.10884677099999));
#212352=CARTESIAN_POINT('Ctrl Pts',(6.62076229999994,11.6,8.10884677099999));
#212353=CARTESIAN_POINT('Ctrl Pts',(6.62154732099994,15.2,8.11020086499998));
#212354=CARTESIAN_POINT('Ctrl Pts',(6.62154732099994,11.6,8.11020086499998));
#212355=CARTESIAN_POINT('Ctrl Pts',(6.62233504499994,15.2,8.11156257399999));
#212356=CARTESIAN_POINT('Ctrl Pts',(6.62233504499994,11.6,8.11156257399999));
#212357=CARTESIAN_POINT('Ctrl Pts',(6.62312544999994,15.2,8.11293188899998));
#212358=CARTESIAN_POINT('Ctrl Pts',(6.62312544999994,11.6,8.11293188899998));
#212359=CARTESIAN_POINT('Ctrl Pts',(6.62391851399994,15.2,8.11430880099999));
#212360=CARTESIAN_POINT('Ctrl Pts',(6.62391851399994,11.6,8.11430880099999));
#212361=CARTESIAN_POINT('Ctrl Pts',(6.62471421499994,15.2,8.11569329899999));
#212362=CARTESIAN_POINT('Ctrl Pts',(6.62471421499994,11.6,8.11569329899999));
#212363=CARTESIAN_POINT('Ctrl Pts',(6.62551253299994,15.2,8.11708537599999));
#212364=CARTESIAN_POINT('Ctrl Pts',(6.62551253299994,11.6,8.11708537599999));
#212365=CARTESIAN_POINT('Ctrl Pts',(6.62631344799994,15.2,8.11848501999999));
#212366=CARTESIAN_POINT('Ctrl Pts',(6.62631344799994,11.6,8.11848501999999));
#212367=CARTESIAN_POINT('Ctrl Pts',(6.62711693599995,15.2,8.11989222299999));
#212368=CARTESIAN_POINT('Ctrl Pts',(6.62711693599995,11.6,8.11989222299999));
#212369=CARTESIAN_POINT('Ctrl Pts',(6.62792297799994,15.2,8.12130697599999));
#212370=CARTESIAN_POINT('Ctrl Pts',(6.62792297799994,11.6,8.12130697599999));
#212371=CARTESIAN_POINT('Ctrl Pts',(6.62873155399994,15.2,8.12272926799999));
#212372=CARTESIAN_POINT('Ctrl Pts',(6.62873155399994,11.6,8.12272926799999));
#212373=CARTESIAN_POINT('Ctrl Pts',(6.62954264199994,15.2,8.12415908999998));
#212374=CARTESIAN_POINT('Ctrl Pts',(6.62954264199994,11.6,8.12415908999998));
#212375=CARTESIAN_POINT('Ctrl Pts',(6.63035622099994,15.2,8.12559643399998));
#212376=CARTESIAN_POINT('Ctrl Pts',(6.63035622099994,11.6,8.12559643399998));
#212377=CARTESIAN_POINT('Ctrl Pts',(6.63117226999994,15.2,8.12704128899998));
#212378=CARTESIAN_POINT('Ctrl Pts',(6.63117226999994,11.6,8.12704128899998));
#212379=CARTESIAN_POINT('Ctrl Pts',(6.63199076999994,15.2,8.12849364699998));
#212380=CARTESIAN_POINT('Ctrl Pts',(6.63199076999994,11.6,8.12849364699998));
#212381=CARTESIAN_POINT('Ctrl Pts',(6.63281169999994,15.2,8.12995349699998));
#212382=CARTESIAN_POINT('Ctrl Pts',(6.63281169999994,11.6,8.12995349699998));
#212383=CARTESIAN_POINT('Ctrl Pts',(6.63363503799994,15.2,8.13142083199999));
#212384=CARTESIAN_POINT('Ctrl Pts',(6.63363503799994,11.6,8.13142083199999));
#212385=CARTESIAN_POINT('Ctrl Pts',(6.63446076799994,15.2,8.13289564099998));
#212386=CARTESIAN_POINT('Ctrl Pts',(6.63446076799994,11.6,8.13289564099998));
#212387=CARTESIAN_POINT('Ctrl Pts',(6.63528886399994,15.2,8.13437791499998));
#212388=CARTESIAN_POINT('Ctrl Pts',(6.63528886399994,11.6,8.13437791499998));
#212389=CARTESIAN_POINT('Ctrl Pts',(6.63611931099994,15.2,8.13586764599999));
#212390=CARTESIAN_POINT('Ctrl Pts',(6.63611931099994,11.6,8.13586764599999));
#212391=CARTESIAN_POINT('Ctrl Pts',(6.63695208599994,15.2,8.13736482299999));
#212392=CARTESIAN_POINT('Ctrl Pts',(6.63695208599994,11.6,8.13736482299999));
#212393=CARTESIAN_POINT('Ctrl Pts',(6.63778716999994,15.2,8.13886943899998));
#212394=CARTESIAN_POINT('Ctrl Pts',(6.63778716999994,11.6,8.13886943899998));
#212395=CARTESIAN_POINT('Ctrl Pts',(6.63862454399994,15.2,8.14038148399998));
#212396=CARTESIAN_POINT('Ctrl Pts',(6.63862454399994,11.6,8.14038148399998));
#212397=CARTESIAN_POINT('Ctrl Pts',(6.63946418699994,15.2,8.14190094699999));
#212398=CARTESIAN_POINT('Ctrl Pts',(6.63946418699994,11.6,8.14190094699999));
#212399=CARTESIAN_POINT('Ctrl Pts',(6.64030607799994,15.2,8.14342782199999));
#212400=CARTESIAN_POINT('Ctrl Pts',(6.64030607799994,11.6,8.14342782199999));
#212401=CARTESIAN_POINT('Ctrl Pts',(6.64115019999994,15.2,8.14496209799999));
#212402=CARTESIAN_POINT('Ctrl Pts',(6.64115019999994,11.6,8.14496209799999));
#212403=CARTESIAN_POINT('Ctrl Pts',(6.64199653299994,15.2,8.14650376599998));
#212404=CARTESIAN_POINT('Ctrl Pts',(6.64199653299994,11.6,8.14650376599998));
#212405=CARTESIAN_POINT('Ctrl Pts',(6.64284505599994,15.2,8.14805281799998));
#212406=CARTESIAN_POINT('Ctrl Pts',(6.64284505599994,11.6,8.14805281799998));
#212407=CARTESIAN_POINT('Ctrl Pts',(6.64369575099995,15.2,8.14960924399998));
#212408=CARTESIAN_POINT('Ctrl Pts',(6.64369575099995,11.6,8.14960924399998));
#212409=CARTESIAN_POINT('Ctrl Pts',(6.64454859899994,15.2,8.15117303499999));
#212410=CARTESIAN_POINT('Ctrl Pts',(6.64454859899994,11.6,8.15117303499999));
#212411=CARTESIAN_POINT('Ctrl Pts',(6.64540357999994,15.2,8.15274418299998));
#212412=CARTESIAN_POINT('Ctrl Pts',(6.64540357999994,11.6,8.15274418299998));
#212413=CARTESIAN_POINT('Ctrl Pts',(6.64626067299994,15.2,8.15432267999999));
#212414=CARTESIAN_POINT('Ctrl Pts',(6.64626067299994,11.6,8.15432267999999));
#212415=CARTESIAN_POINT('Ctrl Pts',(6.64711986199994,15.2,8.15590851399998));
#212416=CARTESIAN_POINT('Ctrl Pts',(6.64711986199994,11.6,8.15590851399998));
#212417=CARTESIAN_POINT('Ctrl Pts',(6.64798112699994,15.2,8.15750167699999));
#212418=CARTESIAN_POINT('Ctrl Pts',(6.64798112699994,11.6,8.15750167699999));
#212419=CARTESIAN_POINT('Ctrl Pts',(6.64884444799994,15.2,8.15910216299999));
#212420=CARTESIAN_POINT('Ctrl Pts',(6.64884444799994,11.6,8.15910216299999));
#212421=CARTESIAN_POINT('Ctrl Pts',(6.64970980799994,15.2,8.16070995999999));
#212422=CARTESIAN_POINT('Ctrl Pts',(6.64970980799994,11.6,8.16070995999999));
#212423=CARTESIAN_POINT('Ctrl Pts',(6.65057718599994,15.2,8.16232506099999));
#212424=CARTESIAN_POINT('Ctrl Pts',(6.65057718599994,11.6,8.16232506099999));
#212425=CARTESIAN_POINT('Ctrl Pts',(6.65144656499994,15.2,8.16394745499998));
#212426=CARTESIAN_POINT('Ctrl Pts',(6.65144656499994,11.6,8.16394745499998));
#212427=CARTESIAN_POINT('Ctrl Pts',(6.65231792499994,15.2,8.16557713599998));
#212428=CARTESIAN_POINT('Ctrl Pts',(6.65231792499994,11.6,8.16557713599998));
#212429=CARTESIAN_POINT('Ctrl Pts',(6.65319124899994,15.2,8.16721409299999));
#212430=CARTESIAN_POINT('Ctrl Pts',(6.65319124899994,11.6,8.16721409299999));
#212431=CARTESIAN_POINT('Ctrl Pts',(6.65406651699994,15.2,8.16885831899998));
#212432=CARTESIAN_POINT('Ctrl Pts',(6.65406651699994,11.6,8.16885831899998));
#212433=CARTESIAN_POINT('Ctrl Pts',(6.65494371099994,15.2,8.17050980299998));
#212434=CARTESIAN_POINT('Ctrl Pts',(6.65494371099994,11.6,8.17050980299998));
#212435=CARTESIAN_POINT('Ctrl Pts',(6.65582281299994,15.2,8.17216853899998));
#212436=CARTESIAN_POINT('Ctrl Pts',(6.65582281299994,11.6,8.17216853899998));
#212437=CARTESIAN_POINT('Ctrl Pts',(6.65670380499994,15.2,8.17383451699998));
#212438=CARTESIAN_POINT('Ctrl Pts',(6.65670380499994,11.6,8.17383451699998));
#212439=CARTESIAN_POINT('Ctrl Pts',(6.65758666799994,15.2,8.17550772799999));
#212440=CARTESIAN_POINT('Ctrl Pts',(6.65758666799994,11.6,8.17550772799999));
#212441=CARTESIAN_POINT('Ctrl Pts',(6.65847138399994,15.2,8.17718816299998));
#212442=CARTESIAN_POINT('Ctrl Pts',(6.65847138399994,11.6,8.17718816299998));
#212443=CARTESIAN_POINT('Ctrl Pts',(6.65935793499994,15.2,8.17887581499999));
#212444=CARTESIAN_POINT('Ctrl Pts',(6.65935793499994,11.6,8.17887581499999));
#212445=CARTESIAN_POINT('Ctrl Pts',(6.66024630299995,15.2,8.18057067299998));
#212446=CARTESIAN_POINT('Ctrl Pts',(6.66024630299995,11.6,8.18057067299998));
#212447=CARTESIAN_POINT('Ctrl Pts',(6.66113646899994,15.2,8.18227273199999));
#212448=CARTESIAN_POINT('Ctrl Pts',(6.66113646899994,11.6,8.18227273199999));
#212449=CARTESIAN_POINT('Ctrl Pts',(6.66202841699994,15.2,8.18398197899998));
#212450=CARTESIAN_POINT('Ctrl Pts',(6.66202841699994,11.6,8.18398197899998));
#212451=CARTESIAN_POINT('Ctrl Pts',(6.66292212899994,15.2,8.18569840899999));
#212452=CARTESIAN_POINT('Ctrl Pts',(6.66292212899994,11.6,8.18569840899999));
#212453=CARTESIAN_POINT('Ctrl Pts',(6.66381758599995,15.2,8.18742201199999));
#212454=CARTESIAN_POINT('Ctrl Pts',(6.66381758599995,11.6,8.18742201199999));
#212455=CARTESIAN_POINT('Ctrl Pts',(6.66471477099994,15.2,8.18915277999999));
#212456=CARTESIAN_POINT('Ctrl Pts',(6.66471477099994,11.6,8.18915277999999));
#212457=CARTESIAN_POINT('Ctrl Pts',(6.66561366699994,15.2,8.19089070399999));
#212458=CARTESIAN_POINT('Ctrl Pts',(6.66561366699994,11.6,8.19089070399999));
#212459=CARTESIAN_POINT('Ctrl Pts',(6.66651425399994,15.2,8.19263577599998));
#212460=CARTESIAN_POINT('Ctrl Pts',(6.66651425399994,11.6,8.19263577599998));
#212461=CARTESIAN_POINT('Ctrl Pts',(6.66741651699994,15.2,8.19438798599998));
#212462=CARTESIAN_POINT('Ctrl Pts',(6.66741651699994,11.6,8.19438798599998));
#212463=CARTESIAN_POINT('Ctrl Pts',(6.66832043699995,15.2,8.19614732799998));
#212464=CARTESIAN_POINT('Ctrl Pts',(6.66832043699995,11.6,8.19614732799998));
#212465=CARTESIAN_POINT('Ctrl Pts',(6.66922599799994,15.2,8.19791379099998));
#212466=CARTESIAN_POINT('Ctrl Pts',(6.66922599799994,11.6,8.19791379099998));
#212467=CARTESIAN_POINT('Ctrl Pts',(6.67013318299994,15.2,8.19968736899998));
#212468=CARTESIAN_POINT('Ctrl Pts',(6.67013318299994,11.6,8.19968736899998));
#212469=CARTESIAN_POINT('Ctrl Pts',(6.67104197299994,15.2,8.20146805199998));
#212470=CARTESIAN_POINT('Ctrl Pts',(6.67104197299994,11.6,8.20146805199998));
#212471=CARTESIAN_POINT('Ctrl Pts',(6.67195235199994,15.2,8.20325583299999));
#212472=CARTESIAN_POINT('Ctrl Pts',(6.67195235199994,11.6,8.20325583299999));
#212473=CARTESIAN_POINT('Ctrl Pts',(6.67286430199994,15.2,8.20505070199999));
#212474=CARTESIAN_POINT('Ctrl Pts',(6.67286430199994,11.6,8.20505070199999));
#212475=CARTESIAN_POINT('Ctrl Pts',(6.67377780699994,15.2,8.20685265099998));
#212476=CARTESIAN_POINT('Ctrl Pts',(6.67377780699994,11.6,8.20685265099998));
#212477=CARTESIAN_POINT('Ctrl Pts',(6.67469284899994,15.2,8.20866167399998));
#212478=CARTESIAN_POINT('Ctrl Pts',(6.67469284899994,11.6,8.20866167399998));
#212479=CARTESIAN_POINT('Ctrl Pts',(6.67560941099994,15.2,8.21047775899999));
#212480=CARTESIAN_POINT('Ctrl Pts',(6.67560941099994,11.6,8.21047775899999));
#212481=CARTESIAN_POINT('Ctrl Pts',(6.67652747899995,15.2,8.21230089999998));
#212482=CARTESIAN_POINT('Ctrl Pts',(6.67652747899995,11.6,8.21230089999998));
#212483=CARTESIAN_POINT('Ctrl Pts',(6.67744703199994,15.2,8.21413108799998));
#212484=CARTESIAN_POINT('Ctrl Pts',(6.67744703199994,11.6,8.21413108799998));
#212485=CARTESIAN_POINT('Ctrl Pts',(6.67836805499994,15.2,8.21596831599999));
#212486=CARTESIAN_POINT('Ctrl Pts',(6.67836805499994,11.6,8.21596831599999));
#212487=CARTESIAN_POINT('Ctrl Pts',(6.67929053299994,15.2,8.21781257299998));
#212488=CARTESIAN_POINT('Ctrl Pts',(6.67929053299994,11.6,8.21781257299998));
#212489=CARTESIAN_POINT('Ctrl Pts',(6.68021444599994,15.2,8.21966385399998));
#212490=CARTESIAN_POINT('Ctrl Pts',(6.68021444599994,11.6,8.21966385399998));
#212491=CARTESIAN_POINT('Ctrl Pts',(6.68113978099995,15.2,8.22152214899998));
#212492=CARTESIAN_POINT('Ctrl Pts',(6.68113978099995,11.6,8.22152214899998));
#212493=CARTESIAN_POINT('Ctrl Pts',(6.68206651899995,15.2,8.22338744899999));
#212494=CARTESIAN_POINT('Ctrl Pts',(6.68206651899995,11.6,8.22338744899999));
#212495=CARTESIAN_POINT('Ctrl Pts',(6.68299464399994,15.2,8.22525974799999));
#212496=CARTESIAN_POINT('Ctrl Pts',(6.68299464399994,11.6,8.22525974799999));
#212497=CARTESIAN_POINT('Ctrl Pts',(6.68392413999994,15.2,8.22713903699999));
#212498=CARTESIAN_POINT('Ctrl Pts',(6.68392413999994,11.6,8.22713903699999));
#212499=CARTESIAN_POINT('Ctrl Pts',(6.68485499199994,15.2,8.22902530699999));
#212500=CARTESIAN_POINT('Ctrl Pts',(6.68485499199994,11.6,8.22902530699999));
#212501=CARTESIAN_POINT('Ctrl Pts',(6.68578717999995,15.2,8.23091854999999));
#212502=CARTESIAN_POINT('Ctrl Pts',(6.68578717999995,11.6,8.23091854999999));
#212503=CARTESIAN_POINT('Ctrl Pts',(6.68672069299994,15.2,8.23281875899998));
#212504=CARTESIAN_POINT('Ctrl Pts',(6.68672069299994,11.6,8.23281875899998));
#212505=CARTESIAN_POINT('Ctrl Pts',(6.68765550999994,15.2,8.23472592499999));
#212506=CARTESIAN_POINT('Ctrl Pts',(6.68765550999994,11.6,8.23472592499999));
#212507=CARTESIAN_POINT('Ctrl Pts',(6.68859161699995,15.2,8.23664004199999));
#212508=CARTESIAN_POINT('Ctrl Pts',(6.68859161699995,11.6,8.23664004199999));
#212509=CARTESIAN_POINT('Ctrl Pts',(6.68952899899995,15.2,8.23856109799999));
#212510=CARTESIAN_POINT('Ctrl Pts',(6.68952899899995,11.6,8.23856109799999));
#212511=CARTESIAN_POINT('Ctrl Pts',(6.69046763699994,15.2,8.24048908699999));
#212512=CARTESIAN_POINT('Ctrl Pts',(6.69046763699994,11.6,8.24048908699999));
#212513=CARTESIAN_POINT('Ctrl Pts',(6.69140751799994,15.2,8.24242400199999));
#212514=CARTESIAN_POINT('Ctrl Pts',(6.69140751799994,11.6,8.24242400199999));
#212515=CARTESIAN_POINT('Ctrl Pts',(6.69234862499994,15.2,8.24436583299999));
#212516=CARTESIAN_POINT('Ctrl Pts',(6.69234862499994,11.6,8.24436583299999));
#212517=CARTESIAN_POINT('Ctrl Pts',(6.69329094199994,15.2,8.24631457399999));
#212518=CARTESIAN_POINT('Ctrl Pts',(6.69329094199994,11.6,8.24631457399999));
#212519=CARTESIAN_POINT('Ctrl Pts',(6.69423445299994,15.2,8.24827021499999));
#212520=CARTESIAN_POINT('Ctrl Pts',(6.69423445299994,11.6,8.24827021499999));
#212521=CARTESIAN_POINT('Ctrl Pts',(6.69517914399994,15.2,8.25023274999998));
#212522=CARTESIAN_POINT('Ctrl Pts',(6.69517914399994,11.6,8.25023274999998));
#212523=CARTESIAN_POINT('Ctrl Pts',(6.69612499799995,15.2,8.25220216899999));
#212524=CARTESIAN_POINT('Ctrl Pts',(6.69612499799995,11.6,8.25220216899999));
#212525=CARTESIAN_POINT('Ctrl Pts',(6.69707199899994,15.2,8.25417846599999));
#212526=CARTESIAN_POINT('Ctrl Pts',(6.69707199899994,11.6,8.25417846599999));
#212527=CARTESIAN_POINT('Ctrl Pts',(6.69802013099994,15.2,8.25616163199999));
#212528=CARTESIAN_POINT('Ctrl Pts',(6.69802013099994,11.6,8.25616163199999));
#212529=CARTESIAN_POINT('Ctrl Pts',(6.69896938099994,15.2,8.25815165899999));
#212530=CARTESIAN_POINT('Ctrl Pts',(6.69896938099994,11.6,8.25815165899999));
#212531=CARTESIAN_POINT('Ctrl Pts',(6.69991973099994,15.2,8.26014853899999));
#212532=CARTESIAN_POINT('Ctrl Pts',(6.69991973099994,11.6,8.26014853899999));
#212533=CARTESIAN_POINT('Ctrl Pts',(6.70087116699994,15.2,8.26215226499999));
#212534=CARTESIAN_POINT('Ctrl Pts',(6.70087116699994,11.6,8.26215226499999));
#212535=CARTESIAN_POINT('Ctrl Pts',(6.70182367299994,15.2,8.26416282799999));
#212536=CARTESIAN_POINT('Ctrl Pts',(6.70182367299994,11.6,8.26416282799999));
#212537=CARTESIAN_POINT('Ctrl Pts',(6.70277723299994,15.2,8.26618022199998));
#212538=CARTESIAN_POINT('Ctrl Pts',(6.70277723299994,11.6,8.26618022199998));
#212539=CARTESIAN_POINT('Ctrl Pts',(6.70373183299994,15.2,8.26820443599999));
#212540=CARTESIAN_POINT('Ctrl Pts',(6.70373183299994,11.6,8.26820443599999));
#212541=CARTESIAN_POINT('Ctrl Pts',(6.70468745899995,15.2,8.27023546499999));
#212542=CARTESIAN_POINT('Ctrl Pts',(6.70468745899995,11.6,8.27023546499999));
#212543=CARTESIAN_POINT('Ctrl Pts',(6.70564409299995,15.2,8.27227329999998));
#212544=CARTESIAN_POINT('Ctrl Pts',(6.70564409299995,11.6,8.27227329999998));
#212545=CARTESIAN_POINT('Ctrl Pts',(6.70660172299994,15.2,8.27431793299999));
#212546=CARTESIAN_POINT('Ctrl Pts',(6.70660172299994,11.6,8.27431793299999));
#212547=CARTESIAN_POINT('Ctrl Pts',(6.70756033099994,15.2,8.27636935799998));
#212548=CARTESIAN_POINT('Ctrl Pts',(6.70756033099994,11.6,8.27636935799998));
#212549=CARTESIAN_POINT('Ctrl Pts',(6.70851990399994,15.2,8.27842756399999));
#212550=CARTESIAN_POINT('Ctrl Pts',(6.70851990399994,11.6,8.27842756399999));
#212551=CARTESIAN_POINT('Ctrl Pts',(6.70948042599994,15.2,8.28049254499999));
#212552=CARTESIAN_POINT('Ctrl Pts',(6.70948042599994,11.6,8.28049254499999));
#212553=CARTESIAN_POINT('Ctrl Pts',(6.71044188299994,15.2,8.28256429499999));
#212554=CARTESIAN_POINT('Ctrl Pts',(6.71044188299994,11.6,8.28256429499999));
#212555=CARTESIAN_POINT('Ctrl Pts',(6.71140425899994,15.2,8.28464280299999));
#212556=CARTESIAN_POINT('Ctrl Pts',(6.71140425899994,11.6,8.28464280299999));
#212557=CARTESIAN_POINT('Ctrl Pts',(6.71236754099994,15.2,8.28672806399998));
#212558=CARTESIAN_POINT('Ctrl Pts',(6.71236754099994,11.6,8.28672806399998));
#212559=CARTESIAN_POINT('Ctrl Pts',(6.71333171199994,15.2,8.28882006799999));
#212560=CARTESIAN_POINT('Ctrl Pts',(6.71333171199994,11.6,8.28882006799999));
#212561=CARTESIAN_POINT('Ctrl Pts',(6.71429675799994,15.2,8.29091880899998));
#212562=CARTESIAN_POINT('Ctrl Pts',(6.71429675799994,11.6,8.29091880899998));
#212563=CARTESIAN_POINT('Ctrl Pts',(6.71526266699995,15.2,8.29302427799998));
#212564=CARTESIAN_POINT('Ctrl Pts',(6.71526266699995,11.6,8.29302427799998));
#212565=CARTESIAN_POINT('Ctrl Pts',(6.71622941999994,15.2,8.29513646899999));
#212566=CARTESIAN_POINT('Ctrl Pts',(6.71622941999994,11.6,8.29513646899999));
#212567=CARTESIAN_POINT('Ctrl Pts',(6.71719700699994,15.2,8.29725537299998));
#212568=CARTESIAN_POINT('Ctrl Pts',(6.71719700699994,11.6,8.29725537299998));
#212569=CARTESIAN_POINT('Ctrl Pts',(6.71816540999994,15.2,8.29938098199998));
#212570=CARTESIAN_POINT('Ctrl Pts',(6.71816540999994,11.6,8.29938098199998));
#212571=CARTESIAN_POINT('Ctrl Pts',(6.71913461599994,15.2,8.30151328999998));
#212572=CARTESIAN_POINT('Ctrl Pts',(6.71913461599994,11.6,8.30151328999998));
#212573=CARTESIAN_POINT('Ctrl Pts',(6.72010461099994,15.2,8.30365228699998));
#212574=CARTESIAN_POINT('Ctrl Pts',(6.72010461099994,11.6,8.30365228699998));
#212575=CARTESIAN_POINT('Ctrl Pts',(6.72107537999994,15.2,8.30579796799999));
#212576=CARTESIAN_POINT('Ctrl Pts',(6.72107537999994,11.6,8.30579796799999));
#212577=CARTESIAN_POINT('Ctrl Pts',(6.72204690799994,15.2,8.30795032399998));
#212578=CARTESIAN_POINT('Ctrl Pts',(6.72204690799994,11.6,8.30795032399998));
#212579=CARTESIAN_POINT('Ctrl Pts',(6.72301918199994,15.2,8.31010934699999));
#212580=CARTESIAN_POINT('Ctrl Pts',(6.72301918199994,11.6,8.31010934699999));
#212581=CARTESIAN_POINT('Ctrl Pts',(6.72399218799994,15.2,8.31227503099999));
#212582=CARTESIAN_POINT('Ctrl Pts',(6.72399218799994,11.6,8.31227503099999));
#212583=CARTESIAN_POINT('Ctrl Pts',(6.72496590999994,15.2,8.31444736699999));
#212584=CARTESIAN_POINT('Ctrl Pts',(6.72496590999994,11.6,8.31444736699999));
#212585=CARTESIAN_POINT('Ctrl Pts',(6.72594033699994,15.2,8.31662634799999));
#212586=CARTESIAN_POINT('Ctrl Pts',(6.72594033699994,11.6,8.31662634799999));
#212587=CARTESIAN_POINT('Ctrl Pts',(6.72691545099994,15.2,8.31881196599999));
#212588=CARTESIAN_POINT('Ctrl Pts',(6.72691545099994,11.6,8.31881196599999));
#212589=CARTESIAN_POINT('Ctrl Pts',(6.72789124099994,15.2,8.32100421499998));
#212590=CARTESIAN_POINT('Ctrl Pts',(6.72789124099994,11.6,8.32100421499998));
#212591=CARTESIAN_POINT('Ctrl Pts',(6.72886769299994,15.2,8.32320308499998));
#212592=CARTESIAN_POINT('Ctrl Pts',(6.72886769299994,11.6,8.32320308499998));
#212593=CARTESIAN_POINT('Ctrl Pts',(6.72984478999994,15.2,8.32540856999999));
#212594=CARTESIAN_POINT('Ctrl Pts',(6.72984478999994,11.6,8.32540856999999));
#212595=CARTESIAN_POINT('Ctrl Pts',(6.73082252199994,15.2,8.32762066199999));
#212596=CARTESIAN_POINT('Ctrl Pts',(6.73082252199994,11.6,8.32762066199999));
#212597=CARTESIAN_POINT('Ctrl Pts',(6.73180087299994,15.2,8.32983935599999));
#212598=CARTESIAN_POINT('Ctrl Pts',(6.73180087299994,11.6,8.32983935599999));
#212599=CARTESIAN_POINT('Ctrl Pts',(6.73277982899994,15.2,8.33206463999998));
#212600=CARTESIAN_POINT('Ctrl Pts',(6.73277982899994,11.6,8.33206463999998));
#212601=CARTESIAN_POINT('Ctrl Pts',(6.73375937699995,15.2,8.33429650999998));
#212602=CARTESIAN_POINT('Ctrl Pts',(6.73375937699995,11.6,8.33429650999998));
#212603=CARTESIAN_POINT('Ctrl Pts',(6.73473950299995,15.2,8.33653495699998));
#212604=CARTESIAN_POINT('Ctrl Pts',(6.73473950299995,11.6,8.33653495699998));
#212605=CARTESIAN_POINT('Ctrl Pts',(6.73572019399994,15.2,8.33877997399998));
#212606=CARTESIAN_POINT('Ctrl Pts',(6.73572019399994,11.6,8.33877997399998));
#212607=CARTESIAN_POINT('Ctrl Pts',(6.73670143599994,15.2,8.34103155399998));
#212608=CARTESIAN_POINT('Ctrl Pts',(6.73670143599994,11.6,8.34103155399998));
#212609=CARTESIAN_POINT('Ctrl Pts',(6.73768321599994,15.2,8.34328968899998));
#212610=CARTESIAN_POINT('Ctrl Pts',(6.73768321599994,11.6,8.34328968899998));
#212611=CARTESIAN_POINT('Ctrl Pts',(6.73866551799994,15.2,8.34555437199998));
#212612=CARTESIAN_POINT('Ctrl Pts',(6.73866551799994,11.6,8.34555437199998));
#212613=CARTESIAN_POINT('Ctrl Pts',(6.73964833099994,15.2,8.34782559399999));
#212614=CARTESIAN_POINT('Ctrl Pts',(6.73964833099994,11.6,8.34782559399999));
#212615=CARTESIAN_POINT('Ctrl Pts',(6.74063164199994,15.2,8.35010335099999));
#212616=CARTESIAN_POINT('Ctrl Pts',(6.74063164199994,11.6,8.35010335099999));
#212617=CARTESIAN_POINT('Ctrl Pts',(6.74161543499994,15.2,8.35238763299999));
#212618=CARTESIAN_POINT('Ctrl Pts',(6.74161543499994,11.6,8.35238763299999));
#212619=CARTESIAN_POINT('Ctrl Pts',(6.74259969899994,15.2,8.35467843299998));
#212620=CARTESIAN_POINT('Ctrl Pts',(6.74259969899994,11.6,8.35467843299998));
#212621=CARTESIAN_POINT('Ctrl Pts',(6.74358441899994,15.2,8.35697574399998));
#212622=CARTESIAN_POINT('Ctrl Pts',(6.74358441899994,11.6,8.35697574399998));
#212623=CARTESIAN_POINT('Ctrl Pts',(6.74456958199994,15.2,8.35927955899999));
#212624=CARTESIAN_POINT('Ctrl Pts',(6.74456958199994,11.6,8.35927955899999));
#212625=CARTESIAN_POINT('Ctrl Pts',(6.74555517699994,15.2,8.36158986999998));
#212626=CARTESIAN_POINT('Ctrl Pts',(6.74555517699994,11.6,8.36158986999998));
#212627=CARTESIAN_POINT('Ctrl Pts',(6.74654118699994,15.2,8.36390667099998));
#212628=CARTESIAN_POINT('Ctrl Pts',(6.74654118699994,11.6,8.36390667099998));
#212629=CARTESIAN_POINT('Ctrl Pts',(6.74752760399994,15.2,8.36622995199999));
#212630=CARTESIAN_POINT('Ctrl Pts',(6.74752760399994,11.6,8.36622995199999));
#212631=CARTESIAN_POINT('Ctrl Pts',(6.74851440899995,15.2,8.36855970899999));
#212632=CARTESIAN_POINT('Ctrl Pts',(6.74851440899995,11.6,8.36855970899999));
#212633=CARTESIAN_POINT('Ctrl Pts',(6.74950159299994,15.2,8.37089593199998));
#212634=CARTESIAN_POINT('Ctrl Pts',(6.74950159299994,11.6,8.37089593199998));
#212635=CARTESIAN_POINT('Ctrl Pts',(6.75048914099994,15.2,8.37323861399998));
#212636=CARTESIAN_POINT('Ctrl Pts',(6.75048914099994,11.6,8.37323861399998));
#212637=CARTESIAN_POINT('Ctrl Pts',(6.75147703999994,15.2,8.37558774999999));
#212638=CARTESIAN_POINT('Ctrl Pts',(6.75147703999994,11.6,8.37558774999999));
#212639=CARTESIAN_POINT('Ctrl Pts',(6.75246527899994,15.2,8.37794333099998));
#212640=CARTESIAN_POINT('Ctrl Pts',(6.75246527899994,11.6,8.37794333099998));
#212641=CARTESIAN_POINT('Ctrl Pts',(6.75345384399994,15.2,8.38030534999999));
#212642=CARTESIAN_POINT('Ctrl Pts',(6.75345384399994,11.6,8.38030534999999));
#212643=CARTESIAN_POINT('Ctrl Pts',(6.75444272099995,15.2,8.38267379999999));
#212644=CARTESIAN_POINT('Ctrl Pts',(6.75444272099995,11.6,8.38267379999999));
#212645=CARTESIAN_POINT('Ctrl Pts',(6.75543189899994,15.2,8.38504867299999));
#212646=CARTESIAN_POINT('Ctrl Pts',(6.75543189899994,11.6,8.38504867299999));
#212647=CARTESIAN_POINT('Ctrl Pts',(6.75642136399994,15.2,8.38742996299998));
#212648=CARTESIAN_POINT('Ctrl Pts',(6.75642136399994,11.6,8.38742996299998));
#212649=CARTESIAN_POINT('Ctrl Pts',(6.75741110399994,15.2,8.38981766199998));
#212650=CARTESIAN_POINT('Ctrl Pts',(6.75741110399994,11.6,8.38981766199998));
#212651=CARTESIAN_POINT('Ctrl Pts',(6.75840110499994,15.2,8.39221176299999));
#212652=CARTESIAN_POINT('Ctrl Pts',(6.75840110499994,11.6,8.39221176299999));
#212653=CARTESIAN_POINT('Ctrl Pts',(6.75939135499994,15.2,8.39461225999998));
#212654=CARTESIAN_POINT('Ctrl Pts',(6.75939135499994,11.6,8.39461225999998));
#212655=CARTESIAN_POINT('Ctrl Pts',(6.76038184399994,15.2,8.39701914299999));
#212656=CARTESIAN_POINT('Ctrl Pts',(6.76038184399994,11.6,8.39701914299999));
#212657=CARTESIAN_POINT('Ctrl Pts',(6.76137255499994,15.2,8.39943240699998));
#212658=CARTESIAN_POINT('Ctrl Pts',(6.76137255499994,11.6,8.39943240699998));
#212659=CARTESIAN_POINT('Ctrl Pts',(6.76236347699994,15.2,8.40185204399998));
#212660=CARTESIAN_POINT('Ctrl Pts',(6.76236347699994,11.6,8.40185204399998));
#212661=CARTESIAN_POINT('Ctrl Pts',(6.76335459899994,15.2,8.40427804899999));
#212662=CARTESIAN_POINT('Ctrl Pts',(6.76335459899994,11.6,8.40427804899999));
#212663=CARTESIAN_POINT('Ctrl Pts',(6.76434590699994,15.2,8.40671041199998));
#212664=CARTESIAN_POINT('Ctrl Pts',(6.76434590699994,11.6,8.40671041199998));
#212665=CARTESIAN_POINT('Ctrl Pts',(6.76533738899994,15.2,8.40914912599998));
#212666=CARTESIAN_POINT('Ctrl Pts',(6.76533738899994,11.6,8.40914912599998));
#212667=CARTESIAN_POINT('Ctrl Pts',(6.76632903299994,15.2,8.41159418599998));
#212668=CARTESIAN_POINT('Ctrl Pts',(6.76632903299994,11.6,8.41159418599998));
#212669=CARTESIAN_POINT('Ctrl Pts',(6.76732082599995,15.2,8.41404558399999));
#212670=CARTESIAN_POINT('Ctrl Pts',(6.76732082599995,11.6,8.41404558399999));
#212671=CARTESIAN_POINT('Ctrl Pts',(6.76831275599994,15.2,8.41650331199999));
#212672=CARTESIAN_POINT('Ctrl Pts',(6.76831275599994,11.6,8.41650331199999));
#212673=CARTESIAN_POINT('Ctrl Pts',(6.76930481099994,15.2,8.41896736399999));
#212674=CARTESIAN_POINT('Ctrl Pts',(6.76930481099994,11.6,8.41896736399999));
#212675=CARTESIAN_POINT('Ctrl Pts',(6.77029697699994,15.2,8.42143773199999));
#212676=CARTESIAN_POINT('Ctrl Pts',(6.77029697699994,11.6,8.42143773199999));
#212677=CARTESIAN_POINT('Ctrl Pts',(6.77128924399995,15.2,8.42391440999998));
#212678=CARTESIAN_POINT('Ctrl Pts',(6.77128924399995,11.6,8.42391440999998));
#212679=CARTESIAN_POINT('Ctrl Pts',(6.77228159899994,15.2,8.42639739099998));
#212680=CARTESIAN_POINT('Ctrl Pts',(6.77228159899994,11.6,8.42639739099998));
#212681=CARTESIAN_POINT('Ctrl Pts',(6.77327402999994,15.2,8.42888666499999));
#212682=CARTESIAN_POINT('Ctrl Pts',(6.77327402999994,11.6,8.42888666499999));
#212683=CARTESIAN_POINT('Ctrl Pts',(6.77426652499994,15.2,8.43138222999999));
#212684=CARTESIAN_POINT('Ctrl Pts',(6.77426652499994,11.6,8.43138222999999));
#212685=CARTESIAN_POINT('Ctrl Pts',(6.77525906999994,15.2,8.43388407499998));
#212686=CARTESIAN_POINT('Ctrl Pts',(6.77525906999994,11.6,8.43388407499998));
#212687=CARTESIAN_POINT('Ctrl Pts',(6.77625165599994,15.2,8.43639219399999));
#212688=CARTESIAN_POINT('Ctrl Pts',(6.77625165599994,11.6,8.43639219399999));
#212689=CARTESIAN_POINT('Ctrl Pts',(6.77724426899994,15.2,8.43890658099999));
#212690=CARTESIAN_POINT('Ctrl Pts',(6.77724426899994,11.6,8.43890658099999));
#212691=CARTESIAN_POINT('Ctrl Pts',(6.77823689699995,15.2,8.44142722899999));
#212692=CARTESIAN_POINT('Ctrl Pts',(6.77823689699995,11.6,8.44142722899999));
#212693=CARTESIAN_POINT('Ctrl Pts',(6.77922952999994,15.2,8.44395412899999));
#212694=CARTESIAN_POINT('Ctrl Pts',(6.77922952999994,11.6,8.44395412899999));
#212695=CARTESIAN_POINT('Ctrl Pts',(6.78022215399994,15.2,8.44648727499998));
#212696=CARTESIAN_POINT('Ctrl Pts',(6.78022215399994,11.6,8.44648727499998));
#212697=CARTESIAN_POINT('Ctrl Pts',(6.78121475799994,15.2,8.44902666199999));
#212698=CARTESIAN_POINT('Ctrl Pts',(6.78121475799994,11.6,8.44902666199999));
#212699=CARTESIAN_POINT('Ctrl Pts',(6.78220733099994,15.2,8.45157227999999));
#212700=CARTESIAN_POINT('Ctrl Pts',(6.78220733099994,11.6,8.45157227999999));
#212701=CARTESIAN_POINT('Ctrl Pts',(6.78319985999994,15.2,8.45412412399998));
#212702=CARTESIAN_POINT('Ctrl Pts',(6.78319985999994,11.6,8.45412412399998));
#212703=CARTESIAN_POINT('Ctrl Pts',(6.78419233199994,15.2,8.45668218599998));
#212704=CARTESIAN_POINT('Ctrl Pts',(6.78419233199994,11.6,8.45668218599998));
#212705=CARTESIAN_POINT('Ctrl Pts',(6.78518473799994,15.2,8.45924645999999));
#212706=CARTESIAN_POINT('Ctrl Pts',(6.78518473799994,11.6,8.45924645999999));
#212707=CARTESIAN_POINT('Ctrl Pts',(6.78617706499994,15.2,8.46181693899998));
#212708=CARTESIAN_POINT('Ctrl Pts',(6.78617706499994,11.6,8.46181693899998));
#212709=CARTESIAN_POINT('Ctrl Pts',(6.78716930199994,15.2,8.46439361399998));
#212710=CARTESIAN_POINT('Ctrl Pts',(6.78716930199994,11.6,8.46439361399998));
#212711=CARTESIAN_POINT('Ctrl Pts',(6.78816143599994,15.2,8.46697648099998));
#212712=CARTESIAN_POINT('Ctrl Pts',(6.78816143599994,11.6,8.46697648099998));
#212713=CARTESIAN_POINT('Ctrl Pts',(6.78915345799994,15.2,8.46956553199998));
#212714=CARTESIAN_POINT('Ctrl Pts',(6.78915345799994,11.6,8.46956553199998));
#212715=CARTESIAN_POINT('Ctrl Pts',(6.79014535299994,15.2,8.47216075999999));
#212716=CARTESIAN_POINT('Ctrl Pts',(6.79014535299994,11.6,8.47216075999999));
#212717=CARTESIAN_POINT('Ctrl Pts',(6.79113711199994,15.2,8.47476215799999));
#212718=CARTESIAN_POINT('Ctrl Pts',(6.79113711199994,11.6,8.47476215799999));
#212719=CARTESIAN_POINT('Ctrl Pts',(6.79212872199995,15.2,8.47736971999998));
#212720=CARTESIAN_POINT('Ctrl Pts',(6.79212872199995,11.6,8.47736971999998));
#212721=CARTESIAN_POINT('Ctrl Pts',(6.79312017299995,15.2,8.47998343599999));
#212722=CARTESIAN_POINT('Ctrl Pts',(6.79312017299995,11.6,8.47998343599999));
#212723=CARTESIAN_POINT('Ctrl Pts',(6.79411145299994,15.2,8.48260330499999));
#212724=CARTESIAN_POINT('Ctrl Pts',(6.79411145299994,11.6,8.48260330499999));
#212725=CARTESIAN_POINT('Ctrl Pts',(6.79510254999995,15.2,8.48522931399999));
#212726=CARTESIAN_POINT('Ctrl Pts',(6.79510254999995,11.6,8.48522931399999));
#212727=CARTESIAN_POINT('Ctrl Pts',(6.79609345299995,15.2,8.48786145899999));
#212728=CARTESIAN_POINT('Ctrl Pts',(6.79609345299995,11.6,8.48786145899999));
#212729=CARTESIAN_POINT('Ctrl Pts',(6.79708415199994,15.2,8.49049973299999));
#212730=CARTESIAN_POINT('Ctrl Pts',(6.79708415199994,11.6,8.49049973299999));
#212731=CARTESIAN_POINT('Ctrl Pts',(6.79807463299994,15.2,8.49314413099999));
#212732=CARTESIAN_POINT('Ctrl Pts',(6.79807463299994,11.6,8.49314413099999));
#212733=CARTESIAN_POINT('Ctrl Pts',(6.79906488699995,15.2,8.49579464199999));
#212734=CARTESIAN_POINT('Ctrl Pts',(6.79906488699995,11.6,8.49579464199999));
#212735=CARTESIAN_POINT('Ctrl Pts',(6.80005490199994,15.2,8.49845126299999));
#212736=CARTESIAN_POINT('Ctrl Pts',(6.80005490199994,11.6,8.49845126299999));
#212737=CARTESIAN_POINT('Ctrl Pts',(6.80104466699994,15.2,8.50111398499998));
#212738=CARTESIAN_POINT('Ctrl Pts',(6.80104466699994,11.6,8.50111398499998));
#212739=CARTESIAN_POINT('Ctrl Pts',(6.80203416999994,15.2,8.50378280199998));
#212740=CARTESIAN_POINT('Ctrl Pts',(6.80203416999994,11.6,8.50378280199998));
#212741=CARTESIAN_POINT('Ctrl Pts',(6.80302340199994,15.2,8.50645770699998));
#212742=CARTESIAN_POINT('Ctrl Pts',(6.80302340199994,11.6,8.50645770699998));
#212743=CARTESIAN_POINT('Ctrl Pts',(6.80401234899994,15.2,8.50913869399999));
#212744=CARTESIAN_POINT('Ctrl Pts',(6.80401234899994,11.6,8.50913869399999));
#212745=CARTESIAN_POINT('Ctrl Pts',(6.80500100199994,15.2,8.51182575499998));
#212746=CARTESIAN_POINT('Ctrl Pts',(6.80500100199994,11.6,8.51182575499998));
#212747=CARTESIAN_POINT('Ctrl Pts',(6.80598934999994,15.2,8.51451888299999));
#212748=CARTESIAN_POINT('Ctrl Pts',(6.80598934999994,11.6,8.51451888299999));
#212749=CARTESIAN_POINT('Ctrl Pts',(6.80697738099994,15.2,8.51721807399999));
#212750=CARTESIAN_POINT('Ctrl Pts',(6.80697738099994,11.6,8.51721807399999));
#212751=CARTESIAN_POINT('Ctrl Pts',(6.80796508399995,15.2,8.51992331899999));
#212752=CARTESIAN_POINT('Ctrl Pts',(6.80796508399995,11.6,8.51992331899999));
#212753=CARTESIAN_POINT('Ctrl Pts',(6.80895244899994,15.2,8.52263460999998));
#212754=CARTESIAN_POINT('Ctrl Pts',(6.80895244899994,11.6,8.52263460999998));
#212755=CARTESIAN_POINT('Ctrl Pts',(6.80993946499994,15.2,8.52535194399999));
#212756=CARTESIAN_POINT('Ctrl Pts',(6.80993946499994,11.6,8.52535194399999));
#212757=CARTESIAN_POINT('Ctrl Pts',(6.81092611999994,15.2,8.52807530999998));
#212758=CARTESIAN_POINT('Ctrl Pts',(6.81092611999994,11.6,8.52807530999998));
#212759=CARTESIAN_POINT('Ctrl Pts',(6.81191240399994,15.2,8.53080470399998));
#212760=CARTESIAN_POINT('Ctrl Pts',(6.81191240399994,11.6,8.53080470399998));
#212761=CARTESIAN_POINT('Ctrl Pts',(6.81289830599995,15.2,8.53354011999999));
#212762=CARTESIAN_POINT('Ctrl Pts',(6.81289830599995,11.6,8.53354011999999));
#212763=CARTESIAN_POINT('Ctrl Pts',(6.81388381499994,15.2,8.53628154899998));
#212764=CARTESIAN_POINT('Ctrl Pts',(6.81388381499994,11.6,8.53628154899998));
#212765=CARTESIAN_POINT('Ctrl Pts',(6.81486892199994,15.2,8.53902898499998));
#212766=CARTESIAN_POINT('Ctrl Pts',(6.81486892199994,11.6,8.53902898499998));
#212767=CARTESIAN_POINT('Ctrl Pts',(6.81585361299994,15.2,8.54178242199998));
#212768=CARTESIAN_POINT('Ctrl Pts',(6.81585361299994,11.6,8.54178242199998));
#212769=CARTESIAN_POINT('Ctrl Pts',(6.81683788099994,15.2,8.54454185299998));
#212770=CARTESIAN_POINT('Ctrl Pts',(6.81683788099994,11.6,8.54454185299998));
#212771=CARTESIAN_POINT('Ctrl Pts',(6.81782171199995,15.2,8.54730727199998));
#212772=CARTESIAN_POINT('Ctrl Pts',(6.81782171199995,11.6,8.54730727199998));
#212773=CARTESIAN_POINT('Ctrl Pts',(6.81880509699995,15.2,8.55007867099999));
#212774=CARTESIAN_POINT('Ctrl Pts',(6.81880509699995,11.6,8.55007867099999));
#212775=CARTESIAN_POINT('Ctrl Pts',(6.81978802599994,15.2,8.55285604299999));
#212776=CARTESIAN_POINT('Ctrl Pts',(6.81978802599994,11.6,8.55285604299999));
#212777=CARTESIAN_POINT('Ctrl Pts',(6.82077048599994,15.2,8.55563938299999));
#212778=CARTESIAN_POINT('Ctrl Pts',(6.82077048599994,11.6,8.55563938299999));
#212779=CARTESIAN_POINT('Ctrl Pts',(6.82175246999994,15.2,8.55842868399998));
#212780=CARTESIAN_POINT('Ctrl Pts',(6.82175246999994,11.6,8.55842868399998));
#212781=CARTESIAN_POINT('Ctrl Pts',(6.82273396499994,15.2,8.56122393999998));
#212782=CARTESIAN_POINT('Ctrl Pts',(6.82273396499994,11.6,8.56122393999998));
#212783=CARTESIAN_POINT('Ctrl Pts',(6.82371496099995,15.2,8.56402514099998));
#212784=CARTESIAN_POINT('Ctrl Pts',(6.82371496099995,11.6,8.56402514099998));
#212785=CARTESIAN_POINT('Ctrl Pts',(6.82469544599994,15.2,8.56683228399999));
#212786=CARTESIAN_POINT('Ctrl Pts',(6.82469544599994,11.6,8.56683228399999));
#212787=CARTESIAN_POINT('Ctrl Pts',(6.82567541399994,15.2,8.56964536099999));
#212788=CARTESIAN_POINT('Ctrl Pts',(6.82567541399994,11.6,8.56964536099999));
#212789=CARTESIAN_POINT('Ctrl Pts',(6.82665484999994,15.2,8.57246436599999));
#212790=CARTESIAN_POINT('Ctrl Pts',(6.82665484999994,11.6,8.57246436599999));
#212791=CARTESIAN_POINT('Ctrl Pts',(6.82763374599994,15.2,8.57528929199999));
#212792=CARTESIAN_POINT('Ctrl Pts',(6.82763374599994,11.6,8.57528929199999));
#212793=CARTESIAN_POINT('Ctrl Pts',(6.82861209099995,15.2,8.57812013199998));
#212794=CARTESIAN_POINT('Ctrl Pts',(6.82861209099995,11.6,8.57812013199998));
#212795=CARTESIAN_POINT('Ctrl Pts',(6.82958987399994,15.2,8.58095687999998));
#212796=CARTESIAN_POINT('Ctrl Pts',(6.82958987399994,11.6,8.58095687999998));
#212797=CARTESIAN_POINT('Ctrl Pts',(6.83056708699994,15.2,8.58379952899998));
#212798=CARTESIAN_POINT('Ctrl Pts',(6.83056708699994,11.6,8.58379952899998));
#212799=CARTESIAN_POINT('Ctrl Pts',(6.83154371799994,15.2,8.58664807299999));
#212800=CARTESIAN_POINT('Ctrl Pts',(6.83154371799994,11.6,8.58664807299999));
#212801=CARTESIAN_POINT('Ctrl Pts',(6.83251975599994,15.2,8.58950250499999));
#212802=CARTESIAN_POINT('Ctrl Pts',(6.83251975599994,11.6,8.58950250499999));
#212803=CARTESIAN_POINT('Ctrl Pts',(6.83349519199994,15.2,8.59236281799999));
#212804=CARTESIAN_POINT('Ctrl Pts',(6.83349519199994,11.6,8.59236281799999));
#212805=CARTESIAN_POINT('Ctrl Pts',(6.83447001599994,15.2,8.59522900599998));
#212806=CARTESIAN_POINT('Ctrl Pts',(6.83447001599994,11.6,8.59522900599998));
#212807=CARTESIAN_POINT('Ctrl Pts',(6.83544421899994,15.2,8.59810106299999));
#212808=CARTESIAN_POINT('Ctrl Pts',(6.83544421899994,11.6,8.59810106299999));
#212809=CARTESIAN_POINT('Ctrl Pts',(6.83641778699994,15.2,8.60097898199999));
#212810=CARTESIAN_POINT('Ctrl Pts',(6.83641778699994,11.6,8.60097898199999));
#212811=CARTESIAN_POINT('Ctrl Pts',(6.83739071399994,15.2,8.60386275599998));
#212812=CARTESIAN_POINT('Ctrl Pts',(6.83739071399994,11.6,8.60386275599998));
#212813=CARTESIAN_POINT('Ctrl Pts',(6.83836298699994,15.2,8.60675237899999));
#212814=CARTESIAN_POINT('Ctrl Pts',(6.83836298699994,11.6,8.60675237899999));
#212815=CARTESIAN_POINT('Ctrl Pts',(6.83933459699994,15.2,8.60964784399999));
#212816=CARTESIAN_POINT('Ctrl Pts',(6.83933459699994,11.6,8.60964784399999));
#212817=CARTESIAN_POINT('Ctrl Pts',(6.84030553599994,15.2,8.61254914499998));
#212818=CARTESIAN_POINT('Ctrl Pts',(6.84030553599994,11.6,8.61254914499998));
#212819=CARTESIAN_POINT('Ctrl Pts',(6.84127578999994,15.2,8.61545627499999));
#212820=CARTESIAN_POINT('Ctrl Pts',(6.84127578999994,11.6,8.61545627499999));
#212821=CARTESIAN_POINT('Ctrl Pts',(6.84224535299994,15.2,8.61836922799998));
#212822=CARTESIAN_POINT('Ctrl Pts',(6.84224535299994,11.6,8.61836922799998));
#212823=CARTESIAN_POINT('Ctrl Pts',(6.84321421299994,15.2,8.62128799799999));
#212824=CARTESIAN_POINT('Ctrl Pts',(6.84321421299994,11.6,8.62128799799999));
#212825=CARTESIAN_POINT('Ctrl Pts',(6.84418235899994,15.2,8.62421257699998));
#212826=CARTESIAN_POINT('Ctrl Pts',(6.84418235899994,11.6,8.62421257699998));
#212827=CARTESIAN_POINT('Ctrl Pts',(6.84514978399994,15.2,8.62714295999999));
#212828=CARTESIAN_POINT('Ctrl Pts',(6.84514978399994,11.6,8.62714295999999));
#212829=CARTESIAN_POINT('Ctrl Pts',(6.84611647599994,15.2,8.63007913899999));
#212830=CARTESIAN_POINT('Ctrl Pts',(6.84611647599994,11.6,8.63007913899999));
#212831=CARTESIAN_POINT('Ctrl Pts',(6.84708242699994,15.2,8.63302110999999));
#212832=CARTESIAN_POINT('Ctrl Pts',(6.84708242699994,11.6,8.63302110999999));
#212833=CARTESIAN_POINT('Ctrl Pts',(6.84804762499994,15.2,8.63596886399998));
#212834=CARTESIAN_POINT('Ctrl Pts',(6.84804762499994,11.6,8.63596886399998));
#212835=CARTESIAN_POINT('Ctrl Pts',(6.84901206199994,15.2,8.63892239499998));
#212836=CARTESIAN_POINT('Ctrl Pts',(6.84901206199994,11.6,8.63892239499998));
#212837=CARTESIAN_POINT('Ctrl Pts',(6.84997572699994,15.2,8.64188169799998));
#212838=CARTESIAN_POINT('Ctrl Pts',(6.84997572699994,11.6,8.64188169799998));
#212839=CARTESIAN_POINT('Ctrl Pts',(6.85093861099995,15.2,8.64484676499998));
#212840=CARTESIAN_POINT('Ctrl Pts',(6.85093861099995,11.6,8.64484676499998));
#212841=CARTESIAN_POINT('Ctrl Pts',(6.85190070399995,15.2,8.64781759099999));
#212842=CARTESIAN_POINT('Ctrl Pts',(6.85190070399995,11.6,8.64781759099999));
#212843=CARTESIAN_POINT('Ctrl Pts',(6.85286199699994,15.2,8.65079416799999));
#212844=CARTESIAN_POINT('Ctrl Pts',(6.85286199699994,11.6,8.65079416799999));
#212845=CARTESIAN_POINT('Ctrl Pts',(6.85382247899994,15.2,8.65377649199999));
#212846=CARTESIAN_POINT('Ctrl Pts',(6.85382247899994,11.6,8.65377649199999));
#212847=CARTESIAN_POINT('Ctrl Pts',(6.85478214199994,15.2,8.65676455299998));
#212848=CARTESIAN_POINT('Ctrl Pts',(6.85478214199994,11.6,8.65676455299998));
#212849=CARTESIAN_POINT('Ctrl Pts',(6.85574097599994,15.2,8.65975834699999));
#212850=CARTESIAN_POINT('Ctrl Pts',(6.85574097599994,11.6,8.65975834699999));
#212851=CARTESIAN_POINT('Ctrl Pts',(6.85669896999994,15.2,8.66275786799999));
#212852=CARTESIAN_POINT('Ctrl Pts',(6.85669896999994,11.6,8.66275786799999));
#212853=CARTESIAN_POINT('Ctrl Pts',(6.85765611699994,15.2,8.66576310799999));
#212854=CARTESIAN_POINT('Ctrl Pts',(6.85765611699994,11.6,8.66576310799999));
#212855=CARTESIAN_POINT('Ctrl Pts',(6.85861240499994,15.2,8.66877406199999));
#212856=CARTESIAN_POINT('Ctrl Pts',(6.85861240499994,11.6,8.66877406199999));
#212857=CARTESIAN_POINT('Ctrl Pts',(6.85956782499994,15.2,8.67179072199999));
#212858=CARTESIAN_POINT('Ctrl Pts',(6.85956782499994,11.6,8.67179072199999));
#212859=CARTESIAN_POINT('Ctrl Pts',(6.86052236999994,15.2,8.67481308299999));
#212860=CARTESIAN_POINT('Ctrl Pts',(6.86052236999994,11.6,8.67481308299999));
#212861=CARTESIAN_POINT('Ctrl Pts',(6.86147602799994,15.2,8.67784113899998));
#212862=CARTESIAN_POINT('Ctrl Pts',(6.86147602799994,11.6,8.67784113899998));
#212863=CARTESIAN_POINT('Ctrl Pts',(6.86242878899994,15.2,8.68087488199999));
#212864=CARTESIAN_POINT('Ctrl Pts',(6.86242878899994,11.6,8.68087488199999));
#212865=CARTESIAN_POINT('Ctrl Pts',(6.86338064599994,15.2,8.68391430699998));
#212866=CARTESIAN_POINT('Ctrl Pts',(6.86338064599994,11.6,8.68391430699998));
#212867=CARTESIAN_POINT('Ctrl Pts',(6.86433158899994,15.2,8.68695940699999));
#212868=CARTESIAN_POINT('Ctrl Pts',(6.86433158899994,11.6,8.68695940699999));
#212869=CARTESIAN_POINT('Ctrl Pts',(6.86528160599994,15.2,8.69001017499999));
#212870=CARTESIAN_POINT('Ctrl Pts',(6.86528160599994,11.6,8.69001017499999));
#212871=CARTESIAN_POINT('Ctrl Pts',(6.86623069199994,15.2,8.69306660699999));
#212872=CARTESIAN_POINT('Ctrl Pts',(6.86623069199994,11.6,8.69306660699999));
#212873=CARTESIAN_POINT('Ctrl Pts',(6.86717883499994,15.2,8.69612869499999));
#212874=CARTESIAN_POINT('Ctrl Pts',(6.86717883499994,11.6,8.69612869499999));
#212875=CARTESIAN_POINT('Ctrl Pts',(6.86812602599994,15.2,8.69919643199999));
#212876=CARTESIAN_POINT('Ctrl Pts',(6.86812602599994,11.6,8.69919643199999));
#212877=CARTESIAN_POINT('Ctrl Pts',(6.86907225599994,15.2,8.70226981399998));
#212878=CARTESIAN_POINT('Ctrl Pts',(6.86907225599994,11.6,8.70226981399998));
#212879=CARTESIAN_POINT('Ctrl Pts',(6.87001751699994,15.2,8.70534883199999));
#212880=CARTESIAN_POINT('Ctrl Pts',(6.87001751699994,11.6,8.70534883199999));
#212881=CARTESIAN_POINT('Ctrl Pts',(6.87096179699994,15.2,8.70843347999998));
#212882=CARTESIAN_POINT('Ctrl Pts',(6.87096179699994,11.6,8.70843347999998));
#212883=CARTESIAN_POINT('Ctrl Pts',(6.87190508999994,15.2,8.71152375499998));
#212884=CARTESIAN_POINT('Ctrl Pts',(6.87190508999994,11.6,8.71152375499998));
#212885=CARTESIAN_POINT('Ctrl Pts',(6.87284738499994,15.2,8.71461964699999));
#212886=CARTESIAN_POINT('Ctrl Pts',(6.87284738499994,11.6,8.71461964699999));
#212887=CARTESIAN_POINT('Ctrl Pts',(6.87378867299994,15.2,8.71772115099999));
#212888=CARTESIAN_POINT('Ctrl Pts',(6.87378867299994,11.6,8.71772115099999));
#212889=CARTESIAN_POINT('Ctrl Pts',(6.87472894499995,15.2,8.72082825999998));
#212890=CARTESIAN_POINT('Ctrl Pts',(6.87472894499995,11.6,8.72082825999998));
#212891=CARTESIAN_POINT('Ctrl Pts',(6.87566819199994,15.2,8.72394096899999));
#212892=CARTESIAN_POINT('Ctrl Pts',(6.87566819199994,11.6,8.72394096899999));
#212893=CARTESIAN_POINT('Ctrl Pts',(6.87660640499994,15.2,8.72705927199998));
#212894=CARTESIAN_POINT('Ctrl Pts',(6.87660640499994,11.6,8.72705927199998));
#212895=CARTESIAN_POINT('Ctrl Pts',(6.87754357599994,15.2,8.73018315999998));
#212896=CARTESIAN_POINT('Ctrl Pts',(6.87754357599994,11.6,8.73018315999998));
#212897=CARTESIAN_POINT('Ctrl Pts',(6.87847969399995,15.2,8.73331262999999));
#212898=CARTESIAN_POINT('Ctrl Pts',(6.87847969399995,11.6,8.73331262999999));
#212899=CARTESIAN_POINT('Ctrl Pts',(6.87941475099994,15.2,8.73644767499999));
#212900=CARTESIAN_POINT('Ctrl Pts',(6.87941475099994,11.6,8.73644767499999));
#212901=CARTESIAN_POINT('Ctrl Pts',(6.88034873899994,15.2,8.73958828699998));
#212902=CARTESIAN_POINT('Ctrl Pts',(6.88034873899994,11.6,8.73958828699998));
#212903=CARTESIAN_POINT('Ctrl Pts',(6.88128164699994,15.2,8.74273446099998));
#212904=CARTESIAN_POINT('Ctrl Pts',(6.88128164699994,11.6,8.74273446099998));
#212905=CARTESIAN_POINT('Ctrl Pts',(6.88221346799994,15.2,8.74588618999999));
#212906=CARTESIAN_POINT('Ctrl Pts',(6.88221346799994,11.6,8.74588618999999));
#212907=CARTESIAN_POINT('Ctrl Pts',(6.88314419099994,15.2,8.74904346999998));
#212908=CARTESIAN_POINT('Ctrl Pts',(6.88314419099994,11.6,8.74904346999998));
#212909=CARTESIAN_POINT('Ctrl Pts',(6.88407380999994,15.2,8.75220629299999));
#212910=CARTESIAN_POINT('Ctrl Pts',(6.88407380999994,11.6,8.75220629299999));
#212911=CARTESIAN_POINT('Ctrl Pts',(6.88500231399994,15.2,8.75537465099999));
#212912=CARTESIAN_POINT('Ctrl Pts',(6.88500231399994,11.6,8.75537465099999));
#212913=CARTESIAN_POINT('Ctrl Pts',(6.88592969499994,15.2,8.75854854099998));
#212914=CARTESIAN_POINT('Ctrl Pts',(6.88592969499994,11.6,8.75854854099998));
#212915=CARTESIAN_POINT('Ctrl Pts',(6.88685594399994,15.2,8.76172795599999));
#212916=CARTESIAN_POINT('Ctrl Pts',(6.88685594399994,11.6,8.76172795599999));
#212917=CARTESIAN_POINT('Ctrl Pts',(6.88778105099995,15.2,8.76491288799999));
#212918=CARTESIAN_POINT('Ctrl Pts',(6.88778105099995,11.6,8.76491288799999));
#212919=CARTESIAN_POINT('Ctrl Pts',(6.88870501099994,15.2,8.76810333299998));
#212920=CARTESIAN_POINT('Ctrl Pts',(6.88870501099994,11.6,8.76810333299998));
#212921=CARTESIAN_POINT('Ctrl Pts',(6.88962781099994,15.2,8.77129928399999));
#212922=CARTESIAN_POINT('Ctrl Pts',(6.88962781099994,11.6,8.77129928399999));
#212923=CARTESIAN_POINT('Ctrl Pts',(6.89054944499994,15.2,8.77450073399999));
#212924=CARTESIAN_POINT('Ctrl Pts',(6.89054944499994,11.6,8.77450073399999));
#212925=CARTESIAN_POINT('Ctrl Pts',(6.89146990199994,15.2,8.77770767799999));
#212926=CARTESIAN_POINT('Ctrl Pts',(6.89146990199994,11.6,8.77770767799999));
#212927=CARTESIAN_POINT('Ctrl Pts',(6.89238917499994,15.2,8.78092010899999));
#212928=CARTESIAN_POINT('Ctrl Pts',(6.89238917499994,11.6,8.78092010899999));
#212929=CARTESIAN_POINT('Ctrl Pts',(6.89330725499994,15.2,8.78413802199999));
#212930=CARTESIAN_POINT('Ctrl Pts',(6.89330725499994,11.6,8.78413802199999));
#212931=CARTESIAN_POINT('Ctrl Pts',(6.89422413499994,15.2,8.78736140899999));
#212932=CARTESIAN_POINT('Ctrl Pts',(6.89422413499994,11.6,8.78736140899999));
#212933=CARTESIAN_POINT('Ctrl Pts',(6.89513980299994,15.2,8.79059026499998));
#212934=CARTESIAN_POINT('Ctrl Pts',(6.89513980299994,11.6,8.79059026499998));
#212935=CARTESIAN_POINT('Ctrl Pts',(6.89605425299994,15.2,8.79382458399999));
#212936=CARTESIAN_POINT('Ctrl Pts',(6.89605425299994,11.6,8.79382458399999));
#212937=CARTESIAN_POINT('Ctrl Pts',(6.89696747599994,15.2,8.79706435899998));
#212938=CARTESIAN_POINT('Ctrl Pts',(6.89696747599994,11.6,8.79706435899998));
#212939=CARTESIAN_POINT('Ctrl Pts',(6.89787946299995,15.2,8.80030958399999));
#212940=CARTESIAN_POINT('Ctrl Pts',(6.89787946299995,11.6,8.80030958399999));
#212941=CARTESIAN_POINT('Ctrl Pts',(6.89879020599995,15.2,8.80356025499999));
#212942=CARTESIAN_POINT('Ctrl Pts',(6.89879020599995,11.6,8.80356025499999));
#212943=CARTESIAN_POINT('Ctrl Pts',(6.89969969499994,15.2,8.80681636199999));
#212944=CARTESIAN_POINT('Ctrl Pts',(6.89969969499994,11.6,8.80681636199999));
#212945=CARTESIAN_POINT('Ctrl Pts',(6.90060792399994,15.2,8.81007790299999));
#212946=CARTESIAN_POINT('Ctrl Pts',(6.90060792399994,11.6,8.81007790299999));
#212947=CARTESIAN_POINT('Ctrl Pts',(6.90151488199994,15.2,8.81334486799998));
#212948=CARTESIAN_POINT('Ctrl Pts',(6.90151488199994,11.6,8.81334486799998));
#212949=CARTESIAN_POINT('Ctrl Pts',(6.90242056299994,15.2,8.81661725299999));
#212950=CARTESIAN_POINT('Ctrl Pts',(6.90242056299994,11.6,8.81661725299999));
#212951=CARTESIAN_POINT('Ctrl Pts',(6.90332495699994,15.2,8.81989505199999));
#212952=CARTESIAN_POINT('Ctrl Pts',(6.90332495699994,11.6,8.81989505199999));
#212953=CARTESIAN_POINT('Ctrl Pts',(6.90422805599994,15.2,8.82317825799999));
#212954=CARTESIAN_POINT('Ctrl Pts',(6.90422805599994,11.6,8.82317825799999));
#212955=CARTESIAN_POINT('Ctrl Pts',(6.90512985199994,15.2,8.82646686599998));
#212956=CARTESIAN_POINT('Ctrl Pts',(6.90512985199994,11.6,8.82646686599998));
#212957=CARTESIAN_POINT('Ctrl Pts',(6.90603033499994,15.2,8.82976086899999));
#212958=CARTESIAN_POINT('Ctrl Pts',(6.90603033499994,11.6,8.82976086899999));
#212959=CARTESIAN_POINT('Ctrl Pts',(6.90692949899994,15.2,8.83306025999998));
#212960=CARTESIAN_POINT('Ctrl Pts',(6.90692949899994,11.6,8.83306025999998));
#212961=CARTESIAN_POINT('Ctrl Pts',(6.90782733599994,15.2,8.83636503599998));
#212962=CARTESIAN_POINT('Ctrl Pts',(6.90782733599994,11.6,8.83636503599998));
#212963=CARTESIAN_POINT('Ctrl Pts',(6.90872383499994,15.2,8.83967518699999));
#212964=CARTESIAN_POINT('Ctrl Pts',(6.90872383499994,11.6,8.83967518699999));
#212965=CARTESIAN_POINT('Ctrl Pts',(6.90961898899995,15.2,8.84299070899999));
#212966=CARTESIAN_POINT('Ctrl Pts',(6.90961898899995,11.6,8.84299070899999));
#212967=CARTESIAN_POINT('Ctrl Pts',(6.91051278999994,15.2,8.84631159699998));
#212968=CARTESIAN_POINT('Ctrl Pts',(6.91051278999994,11.6,8.84631159699998));
#212969=CARTESIAN_POINT('Ctrl Pts',(6.91140523099994,15.2,8.84963784299998));
#212970=CARTESIAN_POINT('Ctrl Pts',(6.91140523099994,11.6,8.84963784299998));
#212971=CARTESIAN_POINT('Ctrl Pts',(6.91229630099994,15.2,8.85296944199998));
#212972=CARTESIAN_POINT('Ctrl Pts',(6.91229630099994,11.6,8.85296944199998));
#212973=CARTESIAN_POINT('Ctrl Pts',(6.91318599399994,15.2,8.85630638799999));
#212974=CARTESIAN_POINT('Ctrl Pts',(6.91318599399994,11.6,8.85630638799999));
#212975=CARTESIAN_POINT('Ctrl Pts',(6.91407430099994,15.2,8.85964867299998));
#212976=CARTESIAN_POINT('Ctrl Pts',(6.91407430099994,11.6,8.85964867299998));
#212977=CARTESIAN_POINT('Ctrl Pts',(6.91496121499994,15.2,8.86299629399998));
#212978=CARTESIAN_POINT('Ctrl Pts',(6.91496121499994,11.6,8.86299629399998));
#212979=CARTESIAN_POINT('Ctrl Pts',(6.91584672499994,15.2,8.86634924299998));
#212980=CARTESIAN_POINT('Ctrl Pts',(6.91584672499994,11.6,8.86634924299998));
#212981=CARTESIAN_POINT('Ctrl Pts',(6.91673082599995,15.2,8.86970751299998));
#212982=CARTESIAN_POINT('Ctrl Pts',(6.91673082599995,11.6,8.86970751299998));
#212983=CARTESIAN_POINT('Ctrl Pts',(6.91761350799994,15.2,8.87307110099999));
#212984=CARTESIAN_POINT('Ctrl Pts',(6.91761350799994,11.6,8.87307110099999));
#212985=CARTESIAN_POINT('Ctrl Pts',(6.91849476599994,15.2,8.87643999799998));
#212986=CARTESIAN_POINT('Ctrl Pts',(6.91849476599994,11.6,8.87643999799998));
#212987=CARTESIAN_POINT('Ctrl Pts',(6.91937458799995,15.2,8.87981419999999));
#212988=CARTESIAN_POINT('Ctrl Pts',(6.91937458799995,11.6,8.87981419999999));
#212989=CARTESIAN_POINT('Ctrl Pts',(6.92025296699994,15.2,8.88319369999999));
#212990=CARTESIAN_POINT('Ctrl Pts',(6.92025296699994,11.6,8.88319369999999));
#212991=CARTESIAN_POINT('Ctrl Pts',(6.92112989699995,15.2,8.88657849199999));
#212992=CARTESIAN_POINT('Ctrl Pts',(6.92112989699995,11.6,8.88657849199999));
#212993=CARTESIAN_POINT('Ctrl Pts',(6.92200536799994,15.2,8.88996856999999));
#212994=CARTESIAN_POINT('Ctrl Pts',(6.92200536799994,11.6,8.88996856999999));
#212995=CARTESIAN_POINT('Ctrl Pts',(6.92287937299994,15.2,8.89336392899999));
#212996=CARTESIAN_POINT('Ctrl Pts',(6.92287937299994,11.6,8.89336392899999));
#212997=CARTESIAN_POINT('Ctrl Pts',(6.92375190399994,15.2,8.89676456099998));
#212998=CARTESIAN_POINT('Ctrl Pts',(6.92375190399994,11.6,8.89676456099998));
#212999=CARTESIAN_POINT('Ctrl Pts',(6.92462295199994,15.2,8.90017046199999));
#213000=CARTESIAN_POINT('Ctrl Pts',(6.92462295199994,11.6,8.90017046199999));
#213001=CARTESIAN_POINT('Ctrl Pts',(6.92549251099994,15.2,8.90358162499999));
#213002=CARTESIAN_POINT('Ctrl Pts',(6.92549251099994,11.6,8.90358162499999));
#213003=CARTESIAN_POINT('Ctrl Pts',(6.92636057199994,15.2,8.90699804499998));
#213004=CARTESIAN_POINT('Ctrl Pts',(6.92636057199994,11.6,8.90699804499998));
#213005=CARTESIAN_POINT('Ctrl Pts',(6.92722712699994,15.2,8.91041971399999));
#213006=CARTESIAN_POINT('Ctrl Pts',(6.92722712699994,11.6,8.91041971399999));
#213007=CARTESIAN_POINT('Ctrl Pts',(6.92809216799994,15.2,8.91384662599998));
#213008=CARTESIAN_POINT('Ctrl Pts',(6.92809216799994,11.6,8.91384662599998));
#213009=CARTESIAN_POINT('Ctrl Pts',(6.92895568699995,15.2,8.91727877899999));
#213010=CARTESIAN_POINT('Ctrl Pts',(6.92895568699995,11.6,8.91727877899999));
#213011=CARTESIAN_POINT('Ctrl Pts',(6.92981767799994,15.2,8.92071616199999));
#213012=CARTESIAN_POINT('Ctrl Pts',(6.92981767799994,11.6,8.92071616199999));
#213013=CARTESIAN_POINT('Ctrl Pts',(6.93067813199994,15.2,8.92415877199999));
#213014=CARTESIAN_POINT('Ctrl Pts',(6.93067813199994,11.6,8.92415877199999));
#213015=CARTESIAN_POINT('Ctrl Pts',(6.93153704099994,15.2,8.92760660299999));
#213016=CARTESIAN_POINT('Ctrl Pts',(6.93153704099994,11.6,8.92760660299999));
#213017=CARTESIAN_POINT('Ctrl Pts',(6.93239439699994,15.2,8.93105964699998));
#213018=CARTESIAN_POINT('Ctrl Pts',(6.93239439699994,11.6,8.93105964699998));
#213019=CARTESIAN_POINT('Ctrl Pts',(6.93325019299994,15.2,8.93451789999999));
#213020=CARTESIAN_POINT('Ctrl Pts',(6.93325019299994,11.6,8.93451789999999));
#213021=CARTESIAN_POINT('Ctrl Pts',(6.93410442099994,15.2,8.93798135499999));
#213022=CARTESIAN_POINT('Ctrl Pts',(6.93410442099994,11.6,8.93798135499999));
#213023=CARTESIAN_POINT('Ctrl Pts',(6.93495707299994,15.2,8.94145000699999));
#213024=CARTESIAN_POINT('Ctrl Pts',(6.93495707299994,11.6,8.94145000699999));
#213025=CARTESIAN_POINT('Ctrl Pts',(6.93580814299994,15.2,8.94492384899999));
#213026=CARTESIAN_POINT('Ctrl Pts',(6.93580814299994,11.6,8.94492384899999));
#213027=CARTESIAN_POINT('Ctrl Pts',(6.93665761999994,15.2,8.94840287599998));
#213028=CARTESIAN_POINT('Ctrl Pts',(6.93665761999994,11.6,8.94840287599998));
#213029=CARTESIAN_POINT('Ctrl Pts',(6.93750550099994,15.2,8.95188708099998));
#213030=CARTESIAN_POINT('Ctrl Pts',(6.93750550099994,11.6,8.95188708099998));
#213031=CARTESIAN_POINT('Ctrl Pts',(6.93835177299994,15.2,8.95537645999998));
#213032=CARTESIAN_POINT('Ctrl Pts',(6.93835177299994,11.6,8.95537645999998));
#213033=CARTESIAN_POINT('Ctrl Pts',(6.93919643299994,15.2,8.95887100399998));
#213034=CARTESIAN_POINT('Ctrl Pts',(6.93919643299994,11.6,8.95887100399998));
#213035=CARTESIAN_POINT('Ctrl Pts',(6.94003947099994,15.2,8.96237070999998));
#213036=CARTESIAN_POINT('Ctrl Pts',(6.94003947099994,11.6,8.96237070999998));
#213037=CARTESIAN_POINT('Ctrl Pts',(6.94088087899994,15.2,8.96587557099998));
#213038=CARTESIAN_POINT('Ctrl Pts',(6.94088087899994,11.6,8.96587557099998));
#213039=CARTESIAN_POINT('Ctrl Pts',(6.94172065299994,15.2,8.96938558099999));
#213040=CARTESIAN_POINT('Ctrl Pts',(6.94172065299994,11.6,8.96938558099999));
#213041=CARTESIAN_POINT('Ctrl Pts',(6.94255878099994,15.2,8.97290073299999));
#213042=CARTESIAN_POINT('Ctrl Pts',(6.94255878099994,11.6,8.97290073299999));
#213043=CARTESIAN_POINT('Ctrl Pts',(6.94339525799994,15.2,8.97642102299999));
#213044=CARTESIAN_POINT('Ctrl Pts',(6.94339525799994,11.6,8.97642102299999));
#213045=CARTESIAN_POINT('Ctrl Pts',(6.94423007699994,15.2,8.97994644399999));
#213046=CARTESIAN_POINT('Ctrl Pts',(6.94423007699994,11.6,8.97994644399999));
#213047=CARTESIAN_POINT('Ctrl Pts',(6.94506322799994,15.2,8.98347699099999));
#213048=CARTESIAN_POINT('Ctrl Pts',(6.94506322799994,11.6,8.98347699099999));
#213049=CARTESIAN_POINT('Ctrl Pts',(6.94589470499994,15.2,8.98701265699999));
#213050=CARTESIAN_POINT('Ctrl Pts',(6.94589470499994,11.6,8.98701265699999));
#213051=CARTESIAN_POINT('Ctrl Pts',(6.94672450099994,15.2,8.99055343599999));
#213052=CARTESIAN_POINT('Ctrl Pts',(6.94672450099994,11.6,8.99055343599999));
#213053=CARTESIAN_POINT('Ctrl Pts',(6.94755260899995,15.2,8.99409932399998));
#213054=CARTESIAN_POINT('Ctrl Pts',(6.94755260899995,11.6,8.99409932399998));
#213055=CARTESIAN_POINT('Ctrl Pts',(6.94837901999994,15.2,8.99765031299999));
#213056=CARTESIAN_POINT('Ctrl Pts',(6.94837901999994,11.6,8.99765031299999));
#213057=CARTESIAN_POINT('Ctrl Pts',(6.94920372699994,15.2,9.00120639899999));
#213058=CARTESIAN_POINT('Ctrl Pts',(6.94920372699994,11.6,9.00120639899999));
#213059=CARTESIAN_POINT('Ctrl Pts',(6.95002672299994,15.2,9.00476757299998));
#213060=CARTESIAN_POINT('Ctrl Pts',(6.95002672299994,11.6,9.00476757299998));
#213061=CARTESIAN_POINT('Ctrl Pts',(6.95084800199994,15.2,9.00833383299998));
#213062=CARTESIAN_POINT('Ctrl Pts',(6.95084800199994,11.6,9.00833383299998));
#213063=CARTESIAN_POINT('Ctrl Pts',(6.95166755399995,15.2,9.01190517099998));
#213064=CARTESIAN_POINT('Ctrl Pts',(6.95166755399995,11.6,9.01190517099998));
#213065=CARTESIAN_POINT('Ctrl Pts',(6.95248537399995,15.2,9.01548158099999));
#213066=CARTESIAN_POINT('Ctrl Pts',(6.95248537399995,11.6,9.01548158099999));
#213067=CARTESIAN_POINT('Ctrl Pts',(6.95330145399994,15.2,9.01906305799999));
#213068=CARTESIAN_POINT('Ctrl Pts',(6.95330145399994,11.6,9.01906305799999));
#213069=CARTESIAN_POINT('Ctrl Pts',(6.95411578499994,15.2,9.02264959699998));
#213070=CARTESIAN_POINT('Ctrl Pts',(6.95411578499994,11.6,9.02264959699998));
#213071=CARTESIAN_POINT('Ctrl Pts',(6.95492836299994,15.2,9.02624118899999));
#213072=CARTESIAN_POINT('Ctrl Pts',(6.95492836299994,11.6,9.02624118899999));
#213073=CARTESIAN_POINT('Ctrl Pts',(6.95573917799994,15.2,9.02983783099998));
#213074=CARTESIAN_POINT('Ctrl Pts',(6.95573917799994,11.6,9.02983783099998));
#213075=CARTESIAN_POINT('Ctrl Pts',(6.95654822399994,15.2,9.03343951599999));
#213076=CARTESIAN_POINT('Ctrl Pts',(6.95654822399994,11.6,9.03343951599999));
#213077=CARTESIAN_POINT('Ctrl Pts',(6.95735549299994,15.2,9.03704623899999));
#213078=CARTESIAN_POINT('Ctrl Pts',(6.95735549299994,11.6,9.03704623899999));
#213079=CARTESIAN_POINT('Ctrl Pts',(6.95816097799994,15.2,9.04065799199999));
#213080=CARTESIAN_POINT('Ctrl Pts',(6.95816097799994,11.6,9.04065799199999));
#213081=CARTESIAN_POINT('Ctrl Pts',(6.95896467299994,15.2,9.04427477199999));
#213082=CARTESIAN_POINT('Ctrl Pts',(6.95896467299994,11.6,9.04427477199999));
#213083=CARTESIAN_POINT('Ctrl Pts',(6.95976656999994,15.2,9.04789657199998));
#213084=CARTESIAN_POINT('Ctrl Pts',(6.95976656999994,11.6,9.04789657199998));
#213085=CARTESIAN_POINT('Ctrl Pts',(6.96056666199994,15.2,9.05152338599999));
#213086=CARTESIAN_POINT('Ctrl Pts',(6.96056666199994,11.6,9.05152338599999));
#213087=CARTESIAN_POINT('Ctrl Pts',(6.96136494299994,15.2,9.05515520899998));
#213088=CARTESIAN_POINT('Ctrl Pts',(6.96136494299994,11.6,9.05515520899998));
#213089=CARTESIAN_POINT('Ctrl Pts',(6.96216140399994,15.2,9.05879203399999));
#213090=CARTESIAN_POINT('Ctrl Pts',(6.96216140399994,11.6,9.05879203399999));
#213091=CARTESIAN_POINT('Ctrl Pts',(6.96295603899994,15.2,9.06243385699998));
#213092=CARTESIAN_POINT('Ctrl Pts',(6.96295603899994,11.6,9.06243385699998));
#213093=CARTESIAN_POINT('Ctrl Pts',(6.96374883999994,15.2,9.06608066999999));
#213094=CARTESIAN_POINT('Ctrl Pts',(6.96374883999994,11.6,9.06608066999999));
#213095=CARTESIAN_POINT('Ctrl Pts',(6.96453979999994,15.2,9.06973246599998));
#213096=CARTESIAN_POINT('Ctrl Pts',(6.96453979999994,11.6,9.06973246599998));
#213097=CARTESIAN_POINT('Ctrl Pts',(6.96532891099994,15.2,9.07338924299999));
#213098=CARTESIAN_POINT('Ctrl Pts',(6.96532891099994,11.6,9.07338924299999));
#213099=CARTESIAN_POINT('Ctrl Pts',(6.96611616599994,15.2,9.07705099099999));
#213100=CARTESIAN_POINT('Ctrl Pts',(6.96611616599994,11.6,9.07705099099999));
#213101=CARTESIAN_POINT('Ctrl Pts',(6.96690156099994,15.2,9.08071770699999));
#213102=CARTESIAN_POINT('Ctrl Pts',(6.96690156099994,11.6,9.08071770699999));
#213103=CARTESIAN_POINT('Ctrl Pts',(6.96768508599994,15.2,9.08438938599998));
#213104=CARTESIAN_POINT('Ctrl Pts',(6.96768508599994,11.6,9.08438938599998));
#213105=CARTESIAN_POINT('Ctrl Pts',(6.96846673699994,15.2,9.08806602099999));
#213106=CARTESIAN_POINT('Ctrl Pts',(6.96846673699994,11.6,9.08806602099999));
#213107=CARTESIAN_POINT('Ctrl Pts',(6.96924650799994,15.2,9.09174760899998));
#213108=CARTESIAN_POINT('Ctrl Pts',(6.96924650799994,11.6,9.09174760899998));
#213109=CARTESIAN_POINT('Ctrl Pts',(6.97002438999994,15.2,9.09543414099998));
#213110=CARTESIAN_POINT('Ctrl Pts',(6.97002438999994,11.6,9.09543414099998));
#213111=CARTESIAN_POINT('Ctrl Pts',(6.97080037899994,15.2,9.09912561499999));
#213112=CARTESIAN_POINT('Ctrl Pts',(6.97080037899994,11.6,9.09912561499999));
#213113=CARTESIAN_POINT('Ctrl Pts',(6.97157446399994,15.2,9.10282202199999));
#213114=CARTESIAN_POINT('Ctrl Pts',(6.97157446399994,11.6,9.10282202199999));
#213115=CARTESIAN_POINT('Ctrl Pts',(6.97234663699994,15.2,9.10652335599998));
#213116=CARTESIAN_POINT('Ctrl Pts',(6.97234663699994,11.6,9.10652335599998));
#213117=CARTESIAN_POINT('Ctrl Pts',(6.97311689199994,15.2,9.11022960899999));
#213118=CARTESIAN_POINT('Ctrl Pts',(6.97311689199994,11.6,9.11022960899999));
#213119=CARTESIAN_POINT('Ctrl Pts',(6.97388521799994,15.2,9.11394077399999));
#213120=CARTESIAN_POINT('Ctrl Pts',(6.97388521799994,11.6,9.11394077399999));
#213121=CARTESIAN_POINT('Ctrl Pts',(6.97465160699994,15.2,9.11765684499999));
#213122=CARTESIAN_POINT('Ctrl Pts',(6.97465160699994,11.6,9.11765684499999));
#213123=CARTESIAN_POINT('Ctrl Pts',(6.97541605599994,15.2,9.12137781699998));
#213124=CARTESIAN_POINT('Ctrl Pts',(6.97541605599994,11.6,9.12137781699998));
#213125=CARTESIAN_POINT('Ctrl Pts',(6.97617855799994,15.2,9.12510368599998));
#213126=CARTESIAN_POINT('Ctrl Pts',(6.97617855799994,11.6,9.12510368599998));
#213127=CARTESIAN_POINT('Ctrl Pts',(6.97693911099995,15.2,9.12883444899999));
#213128=CARTESIAN_POINT('Ctrl Pts',(6.97693911099995,11.6,9.12883444899999));
#213129=CARTESIAN_POINT('Ctrl Pts',(6.97769771099994,15.2,9.13257010499999));
#213130=CARTESIAN_POINT('Ctrl Pts',(6.97769771099994,11.6,9.13257010499999));
#213131=CARTESIAN_POINT('Ctrl Pts',(6.97830303199994,15.2,9.13556254299999));
#213132=CARTESIAN_POINT('Ctrl Pts',(6.97830303199994,11.6,9.13556254299999));
#213133=CARTESIAN_POINT('Ctrl Pts',(6.97875614299994,15.2,9.13780907399998));
#213134=CARTESIAN_POINT('Ctrl Pts',(6.97875614299994,11.6,9.13780907399998));
#213135=CARTESIAN_POINT('Ctrl Pts',(6.97905782599994,15.2,9.13930773799999));
#213136=CARTESIAN_POINT('Ctrl Pts',(6.97905782599994,11.6,9.13930773799999));
#213137=CARTESIAN_POINT('Ctrl Pts',(6.97920857099994,15.2,9.14005731499999));
#213138=CARTESIAN_POINT('Ctrl Pts',(6.97920857099994,11.6,9.14005731499999));
#213139=CARTESIAN_POINT('Ctrl Pts',(6.57080831899994,15.2,8.02901631899999));
#213140=CARTESIAN_POINT('Ctrl Pts',(6.57181685709479,15.2,8.03049109922884));
#213141=CARTESIAN_POINT('Ctrl Pts',(6.57285322895298,15.2,8.03201610932772));
#213142=CARTESIAN_POINT('Ctrl Pts',(6.57391635217513,15.2,8.03359089408577));
#213143=CARTESIAN_POINT('Ctrl Pts',(6.57498460231485,15.2,8.03517327325192));
#213144=CARTESIAN_POINT('Ctrl Pts',(6.57607986599813,15.2,8.03680591632581));
#213145=CARTESIAN_POINT('Ctrl Pts',(6.57720107836676,15.2,8.03848839142112));
#213146=CARTESIAN_POINT('Ctrl Pts',(6.57850915931071,15.2,8.04045127880305));
#213147=CARTESIAN_POINT('Ctrl Pts',(6.57985256090342,15.2,8.0424819924996));
#213148=CARTESIAN_POINT('Ctrl Pts',(6.58122965137125,15.2,8.04457986679557));
#213149=CARTESIAN_POINT('Ctrl Pts',(6.58241001476725,15.2,8.04637804497357));
#213150=CARTESIAN_POINT('Ctrl Pts',(6.5836151303474,15.2,8.04822556534917));
#213151=CARTESIAN_POINT('Ctrl Pts',(6.58484400289384,15.2,8.05012201771681));
#213152=CARTESIAN_POINT('Ctrl Pts',(6.58607287532866,15.2,8.05201846991219));
#213153=CARTESIAN_POINT('Ctrl Pts',(6.5873255059879,15.2,8.05396385292234));
#213154=CARTESIAN_POINT('Ctrl Pts',(6.5886009275249,15.2,8.05595776701655));
#213155=CARTESIAN_POINT('Ctrl Pts',(6.58987634906188,15.2,8.05795168111077));
#213156=CARTESIAN_POINT('Ctrl Pts',(6.59117456239721,15.2,8.05999412543044));
#213157=CARTESIAN_POINT('Ctrl Pts',(6.59249462916393,15.2,8.06208470653945));
#213158=CARTESIAN_POINT('Ctrl Pts',(6.59381469605055,15.2,8.06417528783836));
#213159=CARTESIAN_POINT('Ctrl Pts',(6.59515661597275,15.2,8.06631400529914));
#213160=CARTESIAN_POINT('Ctrl Pts',(6.59651947688179,15.2,8.06850047375489));
#213161=CARTESIAN_POINT('Ctrl Pts',(6.59788233766702,15.2,8.07068694201203));
#213162=CARTESIAN_POINT('Ctrl Pts',(6.59926613977845,15.2,8.07292116150669));
#213163=CARTESIAN_POINT('Ctrl Pts',(6.60066999473389,15.2,8.07520275276762));
#213164=CARTESIAN_POINT('Ctrl Pts',(6.60207384968932,15.2,8.07748434402855));
#213165=CARTESIAN_POINT('Ctrl Pts',(6.60349775834128,15.2,8.07981330796732));
#213166=CARTESIAN_POINT('Ctrl Pts',(6.60494085645468,15.2,8.08218927312894));
#213167=CARTESIAN_POINT('Ctrl Pts',(6.60638395469915,15.2,8.08456523850639));
#213168=CARTESIAN_POINT('Ctrl Pts',(6.6078462442627,15.2,8.08698820426467));
#213169=CARTESIAN_POINT('Ctrl Pts',(6.60932688067797,15.2,8.08945780673577));
#213170=CARTESIAN_POINT('Ctrl Pts',(6.61080751695876,15.2,8.09192740898253));
#213171=CARTESIAN_POINT('Ctrl Pts',(6.61230650277865,15.2,8.09444364778919));
#213172=CARTESIAN_POINT('Ctrl Pts',(6.61382301980764,15.2,8.09700616494809));
#213173=CARTESIAN_POINT('Ctrl Pts',(6.61533953683664,15.2,8.09956868210699));
#213174=CARTESIAN_POINT('Ctrl Pts',(6.61687358203922,15.2,8.10217747604554));
#213175=CARTESIAN_POINT('Ctrl Pts',(6.6184243611488,15.2,8.10483219636375));
#213176=CARTESIAN_POINT('Ctrl Pts',(6.6199751402584,15.2,8.10748691668196));
#213177=CARTESIAN_POINT('Ctrl Pts',(6.62154264930262,15.2,8.11018756270347));
#213178=CARTESIAN_POINT('Ctrl Pts',(6.62312611457732,15.2,8.11293378793391));
#213179=CARTESIAN_POINT('Ctrl Pts',(6.62523740180204,15.2,8.1165954219071));
#213180=CARTESIAN_POINT('Ctrl Pts',(6.62737704680761,15.2,8.12033808468612));
#213181=CARTESIAN_POINT('Ctrl Pts',(6.62954326492701,15.2,8.12416097078744));
#213182=CARTESIAN_POINT('Ctrl Pts',(6.631167928369,15.2,8.127028135103));
#213183=CARTESIAN_POINT('Ctrl Pts',(6.63280753706155,15.2,8.12994042577014));
#213184=CARTESIAN_POINT('Ctrl Pts',(6.63446135959234,15.2,8.13289750725959));
#213185=CARTESIAN_POINT('Ctrl Pts',(6.63611518212314,15.2,8.13585458874903));
#213186=CARTESIAN_POINT('Ctrl Pts',(6.63778321817001,15.2,8.13885646332167));
#213187=CARTESIAN_POINT('Ctrl Pts',(6.63946474894167,15.2,8.1419027997924));
#213188=CARTESIAN_POINT('Ctrl Pts',(6.64114627986605,15.2,8.14494913653984));
#213189=CARTESIAN_POINT('Ctrl Pts',(6.64284130675046,15.2,8.14803993675109));
#213190=CARTESIAN_POINT('Ctrl Pts',(6.64454913242775,15.2,8.15117487459163));
#213191=CARTESIAN_POINT('Ctrl Pts',(6.64625695794992,15.2,8.15430981214742));
#213192=CARTESIAN_POINT('Ctrl Pts',(6.64797757785682,15.2,8.15748888975759));
#213193=CARTESIAN_POINT('Ctrl Pts',(6.64971031262775,15.2,8.16071178614242));
#213194=CARTESIAN_POINT('Ctrl Pts',(6.65144304739867,15.2,8.16393468252726));
#213195=CARTESIAN_POINT('Ctrl Pts',(6.65318789496859,15.2,8.16720139724187));
#213196=CARTESIAN_POINT('Ctrl Pts',(6.65494418790425,15.2,8.17051161578635));
#213197=CARTESIAN_POINT('Ctrl Pts',(6.65670048083992,15.2,8.17382183433081));
#213198=CARTESIAN_POINT('Ctrl Pts',(6.65846822131309,15.2,8.17717555743936));
#213199=CARTESIAN_POINT('Ctrl Pts',(6.66024675233107,15.2,8.18057247281299));
#213200=CARTESIAN_POINT('Ctrl Pts',(6.66202528351059,15.2,8.18396938849518));
#213201=CARTESIAN_POINT('Ctrl Pts',(6.66381460970786,15.2,8.18740949648156));
#213202=CARTESIAN_POINT('Ctrl Pts',(6.66561408988971,15.2,8.19089249117325));
#213203=CARTESIAN_POINT('Ctrl Pts',(6.66741356990811,15.2,8.19437548554857));
#213204=CARTESIAN_POINT('Ctrl Pts',(6.66922320412363,15.2,8.1979013640035));
#213205=CARTESIAN_POINT('Ctrl Pts',(6.67104237023243,15.2,8.20146982647329));
#213206=CARTESIAN_POINT('Ctrl Pts',(6.67255834204486,15.2,8.20444354530617));
#213207=CARTESIAN_POINT('Ctrl Pts',(6.67408093153883,15.2,8.20744683568326));
#213208=CARTESIAN_POINT('Ctrl Pts',(6.67560978744159,15.2,8.2104795229749));
#213209=CARTESIAN_POINT('Ctrl Pts',(6.67713864334436,15.2,8.21351221026653));
#213210=CARTESIAN_POINT('Ctrl Pts',(6.67867376366598,15.2,8.21657429548192));
#213211=CARTESIAN_POINT('Ctrl Pts',(6.68021480145077,15.2,8.21966560750993));
#213212=CARTESIAN_POINT('Ctrl Pts',(6.68175583923556,15.2,8.22275691953794));
#213213=CARTESIAN_POINT('Ctrl Pts',(6.68330279499564,15.2,8.22587745733786));
#213214=CARTESIAN_POINT('Ctrl Pts',(6.6848553261765,15.2,8.2290270504644));
#213215=CARTESIAN_POINT('Ctrl Pts',(6.68671836352583,15.2,8.23280656207892));
#213216=CARTESIAN_POINT('Ctrl Pts',(6.68858943118284,15.2,8.23662791582342));
#213217=CARTESIAN_POINT('Ctrl Pts',(6.69046794761425,15.2,8.24049081826456));
#213218=CARTESIAN_POINT('Ctrl Pts',(6.69203337803064,15.2,8.24370990374914));
#213219=CARTESIAN_POINT('Ctrl Pts',(6.69360398287526,15.2,8.24695784379444));
#213220=CARTESIAN_POINT('Ctrl Pts',(6.69517943475741,15.2,8.25023447103147));
#213221=CARTESIAN_POINT('Ctrl Pts',(6.69675488663955,15.2,8.25351109826849));
#213222=CARTESIAN_POINT('Ctrl Pts',(6.69833518289994,15.2,8.25681641326103));
#213223=CARTESIAN_POINT('Ctrl Pts',(6.69992000248326,15.2,8.26015025048324));
#213224=CARTESIAN_POINT('Ctrl Pts',(6.70150482206659,15.2,8.26348408770544));
#213225=CARTESIAN_POINT('Ctrl Pts',(6.70309416312688,15.2,8.26684644767516));
#213226=CARTESIAN_POINT('Ctrl Pts',(6.7046877110508,15.2,8.2702371665101));
#213227=CARTESIAN_POINT('Ctrl Pts',(6.70659996849003,15.2,8.27430602896418));
#213228=CARTESIAN_POINT('Ctrl Pts',(6.70851828215691,15.2,8.2784157278098));
#213229=CARTESIAN_POINT('Ctrl Pts',(6.71044211267011,15.2,8.28256598432389));
#213230=CARTESIAN_POINT('Ctrl Pts',(6.71204530482267,15.2,8.28602453154462));
#213231=CARTESIAN_POINT('Ctrl Pts',(6.71365232831704,15.2,8.28951124262168));
#213232=CARTESIAN_POINT('Ctrl Pts',(6.71526287796963,15.2,8.29302595824522));
#213233=CARTESIAN_POINT('Ctrl Pts',(6.71687342762222,15.2,8.29654067386875));
#213234=CARTESIAN_POINT('Ctrl Pts',(6.71848750324171,15.2,8.30008339392071));
#213235=CARTESIAN_POINT('Ctrl Pts',(6.72010480449905,15.2,8.30365395796463));
#213236=CARTESIAN_POINT('Ctrl Pts',(6.72172210575639,15.2,8.30722452200856));
#213237=CARTESIAN_POINT('Ctrl Pts',(6.72334263070549,15.2,8.31082293178325));
#213238=CARTESIAN_POINT('Ctrl Pts',(6.72496608619161,15.2,8.31444902824158));
#213239=CARTESIAN_POINT('Ctrl Pts',(6.72658954167772,15.2,8.31807512469992));
#213240=CARTESIAN_POINT('Ctrl Pts',(6.72821592633883,15.2,8.32172890851102));
#213241=CARTESIAN_POINT('Ctrl Pts',(6.72984494869994,15.2,8.32541022177491));
#213242=CARTESIAN_POINT('Ctrl Pts',(6.73147397106104,15.2,8.32909153503879));
#213243=CARTESIAN_POINT('Ctrl Pts',(6.7331056319434,15.2,8.33280038045713));
#213244=CARTESIAN_POINT('Ctrl Pts',(6.7347396442425,15.2,8.33653659950195));
#213245=CARTESIAN_POINT('Ctrl Pts',(6.73637365654159,15.2,8.34027281854678));
#213246=CARTESIAN_POINT('Ctrl Pts',(6.73801002092921,15.2,8.34403641308545));
#213247=CARTESIAN_POINT('Ctrl Pts',(6.73964845558211,15.2,8.347827227948));
#213248=CARTESIAN_POINT('Ctrl Pts',(6.741286890235,15.2,8.35161804281056));
#213249=CARTESIAN_POINT('Ctrl Pts',(6.74292739366837,15.2,8.355436079239));
#213250=CARTESIAN_POINT('Ctrl Pts',(6.74456969005736,15.2,8.35928118326822));
#213251=CARTESIAN_POINT('Ctrl Pts',(6.74588352706115,15.2,8.36235726624014));
#213252=CARTESIAN_POINT('Ctrl Pts',(6.7471985122176,15.2,8.36545067278518));
#213253=CARTESIAN_POINT('Ctrl Pts',(6.74851450350898,15.2,8.36856132507363));
#213254=CARTESIAN_POINT('Ctrl Pts',(6.74983049497967,15.2,8.3716719777859));
#213255=CARTESIAN_POINT('Ctrl Pts',(6.75114749275803,15.2,8.37479987469578));
#213256=CARTESIAN_POINT('Ctrl Pts',(6.75246536060769,15.2,8.37794494075719));
#213257=CARTESIAN_POINT('Ctrl Pts',(6.75378322827778,15.2,8.38109000639009));
#213258=CARTESIAN_POINT('Ctrl Pts',(6.75510196406992,15.2,8.38425223983344));
#213259=CARTESIAN_POINT('Ctrl Pts',(6.75642143251754,15.2,8.38743156473844));
#213260=CARTESIAN_POINT('Ctrl Pts',(6.75774090114493,15.2,8.39061089007662));
#213261=CARTESIAN_POINT('Ctrl Pts',(6.75906110102841,15.2,8.39380730742622));
#213262=CARTESIAN_POINT('Ctrl Pts',(6.76038189955084,15.2,8.39702073822711));
#213263=CARTESIAN_POINT('Ctrl Pts',(6.76170269789331,15.2,8.40023416859018));
#213264=CARTESIAN_POINT('Ctrl Pts',(6.76302409172527,15.2,8.40346461550287));
#213265=CARTESIAN_POINT('Ctrl Pts',(6.76434595028382,15.2,8.40671199923564));
#213266=CARTESIAN_POINT('Ctrl Pts',(6.76566780902246,15.2,8.40995938341087));
#213267=CARTESIAN_POINT('Ctrl Pts',(6.76699013193896,15.2,8.41322370691553));
#213268=CARTESIAN_POINT('Ctrl Pts',(6.76831278723328,15.2,8.41650489298325));
#213269=CARTESIAN_POINT('Ctrl Pts',(6.76963544252758,15.2,8.41978607905095));
#213270=CARTESIAN_POINT('Ctrl Pts',(6.77095842881082,15.2,8.4230841286762));
#213271=CARTESIAN_POINT('Ctrl Pts',(6.77228161821629,15.2,8.42639896485858));
#213272=CARTESIAN_POINT('Ctrl Pts',(6.77360480744148,15.2,8.42971380058932));
#213273=CARTESIAN_POINT('Ctrl Pts',(6.77492819831234,15.2,8.43304542463676));
#213274=CARTESIAN_POINT('Ctrl Pts',(6.77625166276571,15.2,8.43639376098931));
#213275=CARTESIAN_POINT('Ctrl Pts',(6.77823685953593,15.2,8.44141626574624));
#213276=CARTESIAN_POINT('Ctrl Pts',(6.78022222002234,15.2,8.44647637519039));
#213277=CARTESIAN_POINT('Ctrl Pts',(6.78220731978357,15.2,8.45157383591931));
#213278=CARTESIAN_POINT('Ctrl Pts',(6.7838615696447,15.2,8.45582172001441));
#213279=CARTESIAN_POINT('Ctrl Pts',(6.78551563503645,15.2,8.46009554375456));
#213280=CARTESIAN_POINT('Ctrl Pts',(6.78716927609131,15.2,8.46439516146755));
#213281=CARTESIAN_POINT('Ctrl Pts',(6.7884921890073,15.2,8.4678348558254));
#213282=CARTESIAN_POINT('Ctrl Pts',(6.78981483008878,15.2,8.4712910599492));
#213283=CARTESIAN_POINT('Ctrl Pts',(6.79113707488304,15.2,8.47476369925064));
#213284=CARTESIAN_POINT('Ctrl Pts',(6.79245931949714,15.2,8.47823633807893));
#213285=CARTESIAN_POINT('Ctrl Pts',(6.79378116923355,15.2,8.48172541230115));
#213286=CARTESIAN_POINT('Ctrl Pts',(6.79510250129224,15.2,8.48523084740179));
#213287=CARTESIAN_POINT('Ctrl Pts',(6.79675416650063,15.2,8.4896126416358));
#213288=CARTESIAN_POINT('Ctrl Pts',(6.79840502414815,15.2,8.4940200027491));
#213289=CARTESIAN_POINT('Ctrl Pts',(6.80005483930009,15.2,8.49845278776043));
#213290=CARTESIAN_POINT('Ctrl Pts',(6.80170465445202,15.2,8.50288557277178));
#213291=CARTESIAN_POINT('Ctrl Pts',(6.80335342639768,15.2,8.50734378141373));
#213292=CARTESIAN_POINT('Ctrl Pts',(6.80500092563386,15.2,8.51182727148185));
#213293=CARTESIAN_POINT('Ctrl Pts',(6.80664842487003,15.2,8.51631076154996));
#213294=CARTESIAN_POINT('Ctrl Pts',(6.80829465035342,15.2,8.52081953613825));
#213295=CARTESIAN_POINT('Ctrl Pts',(6.80993937465904,15.2,8.52535345176188));
#213296=CARTESIAN_POINT('Ctrl Pts',(6.81125515417524,15.2,8.52898058445846));
#213297=CARTESIAN_POINT('Ctrl Pts',(6.81256997178956,15.2,8.53262380823073));
#213298=CARTESIAN_POINT('Ctrl Pts',(6.81388371464891,15.2,8.53628305128099));
#213299=CARTESIAN_POINT('Ctrl Pts',(6.81519745732926,15.2,8.53994229383269));
#213300=CARTESIAN_POINT('Ctrl Pts',(6.81651012421375,15.2,8.54361755584278));
#213301=CARTESIAN_POINT('Ctrl Pts',(6.81782160038439,15.2,8.54730876670666));
#213302=CARTESIAN_POINT('Ctrl Pts',(6.81913307673373,15.2,8.55099997807347));
#213303=CARTESIAN_POINT('Ctrl Pts',(6.82044336308847,15.2,8.55470713570607));
#213304=CARTESIAN_POINT('Ctrl Pts',(6.82175234788195,15.2,8.5584301730211));
#213305=CARTESIAN_POINT('Ctrl Pts',(6.82338857878461,15.2,8.56308396941128));
#213306=CARTESIAN_POINT('Ctrl Pts',(6.82502277306912,15.2,8.56776257169818));
#213307=CARTESIAN_POINT('Ctrl Pts',(6.82665471516439,15.2,8.572465846796));
#213308=CARTESIAN_POINT('Ctrl Pts',(6.82796026873388,15.2,8.57622846656667));
#213309=CARTESIAN_POINT('Ctrl Pts',(6.82926438011927,15.2,8.58000687479833));
#213310=CARTESIAN_POINT('Ctrl Pts',(6.83056694140179,15.2,8.58380100243157));
#213311=CARTESIAN_POINT('Ctrl Pts',(6.83186950286176,15.2,8.58759513058177));
#213312=CARTESIAN_POINT('Ctrl Pts',(6.83317051068823,15.2,8.59140497740054));
#213313=CARTESIAN_POINT('Ctrl Pts',(6.83446986081449,15.2,8.59523047355448));
#213314=CARTESIAN_POINT('Ctrl Pts',(6.83576921076371,15.2,8.59905596918719));
#213315=CARTESIAN_POINT('Ctrl Pts',(6.8370669000966,15.2,8.60289711458346));
#213316=CARTESIAN_POINT('Ctrl Pts',(6.8383628210464,15.2,8.60675383887768));
#213317=CARTESIAN_POINT('Ctrl Pts',(6.83965874217276,15.2,8.61061056369739));
#213318=CARTESIAN_POINT('Ctrl Pts',(6.84095289646064,15.2,8.61448286745074));
#213319=CARTESIAN_POINT('Ctrl Pts',(6.84224517725917,15.2,8.61837068223592));
#213320=CARTESIAN_POINT('Ctrl Pts',(6.84353745788162,15.2,8.62225849649138));
#213321=CARTESIAN_POINT('Ctrl Pts',(6.84482786305553,15.2,8.62616182069504));
#213322=CARTESIAN_POINT('Ctrl Pts',(6.84611629050596,15.2,8.63008058631755));
#213323=CARTESIAN_POINT('Ctrl Pts',(6.84772682495066,15.2,8.63497904374613));
#213324=CARTESIAN_POINT('Ctrl Pts',(6.84933426686765,15.2,8.6399016274827));
#213325=CARTESIAN_POINT('Ctrl Pts',(6.85093841304846,15.2,8.64484820407792));
#213326=CARTESIAN_POINT('Ctrl Pts',(6.85254255922927,15.2,8.64979478067313));
#213327=CARTESIAN_POINT('Ctrl Pts',(6.85414341035111,15.2,8.65476534971123));
#213328=CARTESIAN_POINT('Ctrl Pts',(6.85574076584785,15.2,8.65975977815357));
#213329=CARTESIAN_POINT('Ctrl Pts',(6.85701865031487,15.2,8.6637553211252));
#213330=CARTESIAN_POINT('Ctrl Pts',(6.85829429729866,15.2,8.66776613396156));
#213331=CARTESIAN_POINT('Ctrl Pts',(6.85956760631236,15.2,8.67179214757087));
#213332=CARTESIAN_POINT('Ctrl Pts',(6.86115924249273,15.2,8.67682466430823));
#213333=CARTESIAN_POINT('Ctrl Pts',(6.86274722550929,15.2,8.68188093511996));
#213334=CARTESIAN_POINT('Ctrl Pts',(6.86433135766187,15.2,8.6869608243573));
#213335=CARTESIAN_POINT('Ctrl Pts',(6.86559866328032,15.2,8.69102473541494));
#213336=CARTESIAN_POINT('Ctrl Pts',(6.86686350589278,15.2,8.69510376413461));
#213337=CARTESIAN_POINT('Ctrl Pts',(6.86812578557511,15.2,8.69919784261427));
#213338=CARTESIAN_POINT('Ctrl Pts',(6.869703635307,15.2,8.70431544113219));
#213339=CARTESIAN_POINT('Ctrl Pts',(6.87127748189704,15.2,8.7094565538135));
#213340=CARTESIAN_POINT('Ctrl Pts',(6.87284713314727,15.2,8.71462104964565));
#213341=CARTESIAN_POINT('Ctrl Pts',(6.87410285421589,15.2,8.71875264653653));
#213342=CARTESIAN_POINT('Ctrl Pts',(6.87535588956473,15.2,8.7228992084125));
#213343=CARTESIAN_POINT('Ctrl Pts',(6.87660614457714,15.2,8.72706066864027));
#213344=CARTESIAN_POINT('Ctrl Pts',(6.87785639941919,15.2,8.73122212830105));
#213345=CARTESIAN_POINT('Ctrl Pts',(6.87910387255866,15.2,8.73539848700974));
#213346=CARTESIAN_POINT('Ctrl Pts',(6.88034846885267,15.2,8.73958967687517));
#213347=CARTESIAN_POINT('Ctrl Pts',(6.88159306531626,15.2,8.74378086731166));
#213348=CARTESIAN_POINT('Ctrl Pts',(6.88283478369778,15.2,8.74798689018359));
#213349=CARTESIAN_POINT('Ctrl Pts',(6.8840735313762,15.2,8.75220767713678));
#213350=CARTESIAN_POINT('Ctrl Pts',(6.88531227888583,15.2,8.7564284635149));
#213351=CARTESIAN_POINT('Ctrl Pts',(6.88654805374886,15.2,8.76066401515675));
#213352=CARTESIAN_POINT('Ctrl Pts',(6.88778076398174,15.2,8.76491426553001));
#213353=CARTESIAN_POINT('Ctrl Pts',(6.88901347438257,15.2,8.76916451648237));
#213354=CARTESIAN_POINT('Ctrl Pts',(6.89024312013394,15.2,8.77342946685009));
#213355=CARTESIAN_POINT('Ctrl Pts',(6.89146960598412,15.2,8.77770904976951));
#213356=CARTESIAN_POINT('Ctrl Pts',(6.89238947028821,15.2,8.78091873666753));
#213357=CARTESIAN_POINT('Ctrl Pts',(6.89330755882824,15.2,8.78413665529961));
#213358=CARTESIAN_POINT('Ctrl Pts',(6.89422383204912,15.2,8.78736277623867));
#213359=CARTESIAN_POINT('Ctrl Pts',(6.8957509541394,15.2,8.7927396446658));
#213360=CARTESIAN_POINT('Ctrl Pts',(6.89727303364441,15.2,8.79813929989994));
#213361=CARTESIAN_POINT('Ctrl Pts',(6.89878989253329,15.2,8.80356161406659));
#213362=CARTESIAN_POINT('Ctrl Pts',(6.89970000783355,15.2,8.80681500244837));
#213363=CARTESIAN_POINT('Ctrl Pts',(6.90060824381724,15.2,8.81007654816319));
#213364=CARTESIAN_POINT('Ctrl Pts',(6.9015145626178,15.2,8.81334622262701));
#213365=CARTESIAN_POINT('Ctrl Pts',(6.90242088141836,15.2,8.81661589709082));
#213366=CARTESIAN_POINT('Ctrl Pts',(6.90332528329616,15.2,8.81989370130379));
#213367=CARTESIAN_POINT('Ctrl Pts',(6.90422773005867,15.2,8.8231796078476));
#213368=CARTESIAN_POINT('Ctrl Pts',(6.90513017682119,15.2,8.82646551439141));
#213369=CARTESIAN_POINT('Ctrl Pts',(6.90603066735313,15.2,8.82975952263449));
#213370=CARTESIAN_POINT('Ctrl Pts',(6.90692916702908,15.2,8.83306160547174));
#213371=CARTESIAN_POINT('Ctrl Pts',(6.90782766686827,15.2,8.83636368890887));
#213372=CARTESIAN_POINT('Ctrl Pts',(6.90872417394857,15.2,8.83967384625665));
#213373=CARTESIAN_POINT('Ctrl Pts',(6.90961865095329,15.2,8.84299205119831));
#213374=CARTESIAN_POINT('Ctrl Pts',(6.91051312779551,15.2,8.84631025553717));
#213375=CARTESIAN_POINT('Ctrl Pts',(6.91140557597951,15.2,8.84963650730062));
#213376=CARTESIAN_POINT('Ctrl Pts',(6.91229595682197,15.2,8.85297077909683));
#213377=CARTESIAN_POINT('Ctrl Pts',(6.91318633766444,15.2,8.85630505089304));
#213378=CARTESIAN_POINT('Ctrl Pts',(6.91407465274561,15.2,8.85964734174278));
#213379=CARTESIAN_POINT('Ctrl Pts',(6.91496086405076,15.2,8.86299762601131));
#213380=CARTESIAN_POINT('Ctrl Pts',(6.91614247907064,15.2,8.86746467149981));
#213381=CARTESIAN_POINT('Ctrl Pts',(6.91732035466747,15.2,8.87194592513662));
#213382=CARTESIAN_POINT('Ctrl Pts',(6.91849440684967,15.2,8.87644132348994));
#213383=CARTESIAN_POINT('Ctrl Pts',(6.91937494618627,15.2,8.87981287302055));
#213384=CARTESIAN_POINT('Ctrl Pts',(6.92025333254726,15.2,8.88319237921167));
#213385=CARTESIAN_POINT('Ctrl Pts',(6.92112953246597,15.2,8.88657981424674));
#213386=CARTESIAN_POINT('Ctrl Pts',(6.9220057322255,15.2,8.88996724866642));
#213387=CARTESIAN_POINT('Ctrl Pts',(6.92287974452682,15.2,8.89336261267731));
#213388=CARTESIAN_POINT('Ctrl Pts',(6.92375153336995,15.2,8.89676587859603));
#213389=CARTESIAN_POINT('Ctrl Pts',(6.92520451482796,15.2,8.90243798866665));
#213390=CARTESIAN_POINT('Ctrl Pts',(6.92665132191786,15.2,8.90813204995426));
#213391=CARTESIAN_POINT('Ctrl Pts',(6.92809178768382,15.2,8.91384793683853));
#213392=CARTESIAN_POINT('Ctrl Pts',(6.92895606711199,15.2,8.9172774688445));
#213393=CARTESIAN_POINT('Ctrl Pts',(6.92981806504173,15.2,8.92071485781676));
#213394=CARTESIAN_POINT('Ctrl Pts',(6.93067774584363,15.2,8.92416007760892));
#213395=CARTESIAN_POINT('Ctrl Pts',(6.93153742664552,15.2,8.92760529740109));
#213396=CARTESIAN_POINT('Ctrl Pts',(6.93239478969769,15.2,8.93105834714234));
#213397=CARTESIAN_POINT('Ctrl Pts',(6.93324980099996,15.2,8.93451920051659));
#213398=CARTESIAN_POINT('Ctrl Pts',(6.93410481230223,15.2,8.93798005389085));
#213399=CARTESIAN_POINT('Ctrl Pts',(6.93495747183793,15.2,8.94144871098147));
#213400=CARTESIAN_POINT('Ctrl Pts',(6.93580774472391,15.2,8.94492514485446));
#213401=CARTESIAN_POINT('Ctrl Pts',(6.93665801760989,15.2,8.94840157872746));
#213402=CARTESIAN_POINT('Ctrl Pts',(6.93750590432937,15.2,8.95188578966663));
#213403=CARTESIAN_POINT('Ctrl Pts',(6.93835136975731,15.2,8.95537775053869));
#213404=CARTESIAN_POINT('Ctrl Pts',(6.93919683533885,15.2,8.95886971204513));
#213405=CARTESIAN_POINT('Ctrl Pts',(6.94003988016138,15.2,8.9623694235371));
#213406=CARTESIAN_POINT('Ctrl Pts',(6.94088047061654,15.2,8.96587685900623));
#213407=CARTESIAN_POINT('Ctrl Pts',(6.941721060919,15.2,8.96938429383817));
#213408=CARTESIAN_POINT('Ctrl Pts',(6.94255919633385,15.2,8.97289945139939));
#213409=CARTESIAN_POINT('Ctrl Pts',(6.94339484363661,15.2,8.97642230644826));
#213410=CARTESIAN_POINT('Ctrl Pts',(6.94423049093937,15.2,8.97994516149713));
#213411=CARTESIAN_POINT('Ctrl Pts',(6.94506364895419,15.2,8.98347571369694));
#213412=CARTESIAN_POINT('Ctrl Pts',(6.94589428484046,15.2,8.9870139356524));
#213413=CARTESIAN_POINT('Ctrl Pts',(6.94672492072673,15.2,8.99055215760786));
#213414=CARTESIAN_POINT('Ctrl Pts',(6.9475530356133,15.2,8.99409805037904));
#213415=CARTESIAN_POINT('Ctrl Pts',(6.94837859399996,15.2,8.99765158720827));
#213416=CARTESIAN_POINT('Ctrl Pts',(6.94920415238664,15.2,9.00120512403751));
#213417=CARTESIAN_POINT('Ctrl Pts',(6.95002715535674,15.2,9.00476630384141));
#213418=CARTESIAN_POINT('Ctrl Pts',(6.95084757020216,15.2,9.00833510212773));
#213419=CARTESIAN_POINT('Ctrl Pts',(6.95194145676207,15.2,9.01309350027503));
#213420=CARTESIAN_POINT('Ctrl Pts',(6.95303074152221,15.2,9.01786544049333));
#213421=CARTESIAN_POINT('Ctrl Pts',(6.95411534685732,15.2,9.02265086099441));
#213422=CARTESIAN_POINT('Ctrl Pts',(6.95492880078478,15.2,9.02623992604421));
#213423=CARTESIAN_POINT('Ctrl Pts',(6.95573962300094,15.2,9.0298365725399));
#213424=CARTESIAN_POINT('Ctrl Pts',(6.95654777984634,15.2,9.03344077586792));
#213425=CARTESIAN_POINT('Ctrl Pts',(6.95789470797095,15.2,9.03944778163286));
#213426=CARTESIAN_POINT('Ctrl Pts',(6.95923423285408,15.2,9.04547577529457));
#213427=CARTESIAN_POINT('Ctrl Pts',(6.96056620931203,15.2,9.05152463862899));
#213428=CARTESIAN_POINT('Ctrl Pts',(6.96136539515776,15.2,9.05515395649778));
#213429=CARTESIAN_POINT('Ctrl Pts',(6.96216186315926,15.2,9.05879078725241));
#213430=CARTESIAN_POINT('Ctrl Pts',(6.96295558050902,15.2,9.06243510451158));
#213431=CARTESIAN_POINT('Ctrl Pts',(6.96374929785877,15.2,9.06607942177076));
#213432=CARTESIAN_POINT('Ctrl Pts',(6.96454026450762,15.2,9.06973122396299));
#213433=CARTESIAN_POINT('Ctrl Pts',(6.96532844702425,15.2,9.07339048580495));
#213434=CARTESIAN_POINT('Ctrl Pts',(6.96637935714186,15.2,9.0782695020374));
#213435=CARTESIAN_POINT('Ctrl Pts',(6.96742531992227,15.2,9.08316177839994));
#213436=CARTESIAN_POINT('Ctrl Pts',(6.96846626714516,15.2,9.08806726000199));
#213437=CARTESIAN_POINT('Ctrl Pts',(6.96950721422621,15.2,9.09297274093567));
#213438=CARTESIAN_POINT('Ctrl Pts',(6.97054314812736,15.2,9.09789142717872));
#213439=CARTESIAN_POINT('Ctrl Pts',(6.97157398593231,15.2,9.10282325333021));
#213440=CARTESIAN_POINT('Ctrl Pts',(6.97234711432113,15.2,9.10652212311181));
#213441=CARTESIAN_POINT('Ctrl Pts',(6.97311737659069,15.2,9.11022838219846));
#213442=CARTESIAN_POINT('Ctrl Pts',(6.97388473364314,15.2,9.11394199978984));
#213443=CARTESIAN_POINT('Ctrl Pts',(6.97465209069559,15.2,9.11765561738122));
#213444=CARTESIAN_POINT('Ctrl Pts',(6.97541654334455,15.2,9.12137659300695));
#213445=CARTESIAN_POINT('Ctrl Pts',(6.97617807056728,15.2,9.12510490870382));
#213446=CARTESIAN_POINT('Ctrl Pts',(6.97719344028981,15.2,9.13007599675117));
#213447=CARTESIAN_POINT('Ctrl Pts',(6.97820360405943,15.2,9.13506013363826));
#213448=CARTESIAN_POINT('Ctrl Pts',(6.97920857099994,15.2,9.14005731499999));
#213449=CARTESIAN_POINT('Ctrl Pts',(6.57080831899994,12.2,8.02901631899999));
#213450=CARTESIAN_POINT('Ctrl Pts',(6.57181685709479,12.2,8.03049109922884));
#213451=CARTESIAN_POINT('Ctrl Pts',(6.57285322895298,12.2,8.03201610932772));
#213452=CARTESIAN_POINT('Ctrl Pts',(6.57391635217513,12.2,8.03359089408577));
#213453=CARTESIAN_POINT('Ctrl Pts',(6.57498460231485,12.2,8.03517327325192));
#213454=CARTESIAN_POINT('Ctrl Pts',(6.57607986599813,12.2,8.03680591632581));
#213455=CARTESIAN_POINT('Ctrl Pts',(6.57720107836676,12.2,8.03848839142112));
#213456=CARTESIAN_POINT('Ctrl Pts',(6.57850915931071,12.2,8.04045127880305));
#213457=CARTESIAN_POINT('Ctrl Pts',(6.57985256090342,12.2,8.0424819924996));
#213458=CARTESIAN_POINT('Ctrl Pts',(6.58122965137125,12.2,8.04457986679557));
#213459=CARTESIAN_POINT('Ctrl Pts',(6.58241001476725,12.2,8.04637804497357));
#213460=CARTESIAN_POINT('Ctrl Pts',(6.5836151303474,12.2,8.04822556534917));
#213461=CARTESIAN_POINT('Ctrl Pts',(6.58484400289384,12.2,8.05012201771681));
#213462=CARTESIAN_POINT('Ctrl Pts',(6.58607287532866,12.2,8.05201846991219));
#213463=CARTESIAN_POINT('Ctrl Pts',(6.5873255059879,12.2,8.05396385292234));
#213464=CARTESIAN_POINT('Ctrl Pts',(6.5886009275249,12.2,8.05595776701656));
#213465=CARTESIAN_POINT('Ctrl Pts',(6.58987634906188,12.2,8.05795168111077));
#213466=CARTESIAN_POINT('Ctrl Pts',(6.59117456239721,12.2,8.05999412543044));
#213467=CARTESIAN_POINT('Ctrl Pts',(6.59249462916393,12.2,8.06208470653945));
#213468=CARTESIAN_POINT('Ctrl Pts',(6.59381469605055,12.2,8.06417528783836));
#213469=CARTESIAN_POINT('Ctrl Pts',(6.59515661597275,12.2,8.06631400529914));
#213470=CARTESIAN_POINT('Ctrl Pts',(6.59651947688179,12.2,8.06850047375489));
#213471=CARTESIAN_POINT('Ctrl Pts',(6.59788233766702,12.2,8.07068694201203));
#213472=CARTESIAN_POINT('Ctrl Pts',(6.59926613977845,12.2,8.07292116150669));
#213473=CARTESIAN_POINT('Ctrl Pts',(6.60066999473389,12.2,8.07520275276762));
#213474=CARTESIAN_POINT('Ctrl Pts',(6.60207384968932,12.2,8.07748434402855));
#213475=CARTESIAN_POINT('Ctrl Pts',(6.60349775834128,12.2,8.07981330796732));
#213476=CARTESIAN_POINT('Ctrl Pts',(6.60494085645468,12.2,8.08218927312894));
#213477=CARTESIAN_POINT('Ctrl Pts',(6.60638395469915,12.2,8.08456523850638));
#213478=CARTESIAN_POINT('Ctrl Pts',(6.6078462442627,12.2,8.08698820426467));
#213479=CARTESIAN_POINT('Ctrl Pts',(6.60932688067797,12.2,8.08945780673577));
#213480=CARTESIAN_POINT('Ctrl Pts',(6.61080751695876,12.2,8.09192740898253));
#213481=CARTESIAN_POINT('Ctrl Pts',(6.61230650277865,12.2,8.09444364778919));
#213482=CARTESIAN_POINT('Ctrl Pts',(6.61382301980764,12.2,8.09700616494809));
#213483=CARTESIAN_POINT('Ctrl Pts',(6.61533953683664,12.2,8.09956868210699));
#213484=CARTESIAN_POINT('Ctrl Pts',(6.61687358203922,12.2,8.10217747604554));
#213485=CARTESIAN_POINT('Ctrl Pts',(6.6184243611488,12.2,8.10483219636375));
#213486=CARTESIAN_POINT('Ctrl Pts',(6.6199751402584,12.2,8.10748691668196));
#213487=CARTESIAN_POINT('Ctrl Pts',(6.62154264930262,12.2,8.11018756270347));
#213488=CARTESIAN_POINT('Ctrl Pts',(6.62312611457732,12.2,8.11293378793391));
#213489=CARTESIAN_POINT('Ctrl Pts',(6.62497349082704,12.2,8.11613771753573));
#213490=CARTESIAN_POINT('Ctrl Pts',(6.62684257807194,12.2,8.11940368562293));
#213491=CARTESIAN_POINT('Ctrl Pts',(6.62873218192006,12.2,8.12273115035301));
#213492=CARTESIAN_POINT('Ctrl Pts',(6.63035184242433,12.2,8.1255832630898));
#213493=CARTESIAN_POINT('Ctrl Pts',(6.63198657150547,12.2,8.12848055834052));
#213494=CARTESIAN_POINT('Ctrl Pts',(6.63363563609634,12.2,8.13142270083728));
#213495=CARTESIAN_POINT('Ctrl Pts',(6.63528470053742,12.2,8.1343648430668));
#213496=CARTESIAN_POINT('Ctrl Pts',(6.63694809790168,12.2,8.1373518322318));
#213497=CARTESIAN_POINT('Ctrl Pts',(6.63862511134138,12.2,8.14038333870698));
#213498=CARTESIAN_POINT('Ctrl Pts',(6.64030212478107,12.2,8.14341484518217));
#213499=CARTESIAN_POINT('Ctrl Pts',(6.64199274946127,12.2,8.14649086962036));
#213500=CARTESIAN_POINT('Ctrl Pts',(6.6436962891488,12.2,8.14961108508838));
#213501=CARTESIAN_POINT('Ctrl Pts',(6.64539982883633,12.2,8.15273130055639));
#213502=CARTESIAN_POINT('Ctrl Pts',(6.64711627975847,12.2,8.15589570914476));
#213503=CARTESIAN_POINT('Ctrl Pts',(6.64884495752816,12.2,8.15910399044188));
#213504=CARTESIAN_POINT('Ctrl Pts',(6.65057363545487,12.2,8.16231227203041));
#213505=CARTESIAN_POINT('Ctrl Pts',(6.65231453949944,12.2,8.1655644249565));
#213506=CARTESIAN_POINT('Ctrl Pts',(6.65406699859548,12.2,8.16886013372137));
#213507=CARTESIAN_POINT('Ctrl Pts',(6.65581945753233,12.2,8.17215584218689));
#213508=CARTESIAN_POINT('Ctrl Pts',(6.65758347338056,12.2,8.17549510798934));
#213509=CARTESIAN_POINT('Ctrl Pts',(6.65935838924079,12.2,8.17887761654838));
#213510=CARTESIAN_POINT('Ctrl Pts',(6.66113330510102,12.2,8.18226012510744));
#213511=CARTESIAN_POINT('Ctrl Pts',(6.66291912067844,12.2,8.18568587817577));
#213512=CARTESIAN_POINT('Ctrl Pts',(6.66471519852916,12.2,8.18915456863017));
#213513=CARTESIAN_POINT('Ctrl Pts',(6.66651127654302,12.2,8.19262325939965));
#213514=CARTESIAN_POINT('Ctrl Pts',(6.66831761217702,12.2,8.19613488566173));
#213515=CARTESIAN_POINT('Ctrl Pts',(6.67013358445062,12.2,8.19968914561884));
#213516=CARTESIAN_POINT('Ctrl Pts',(6.67164689459615,12.2,8.20265102875501));
#213517=CARTESIAN_POINT('Ctrl Pts',(6.67316689471018,12.2,8.20564251785934));
#213518=CARTESIAN_POINT('Ctrl Pts',(6.67469322922457,12.2,8.20866343994505));
#213519=CARTESIAN_POINT('Ctrl Pts',(6.67621956373898,12.2,8.21168436203077));
#213520=CARTESIAN_POINT('Ctrl Pts',(6.67775223513403,12.2,8.21473471540034));
#213521=CARTESIAN_POINT('Ctrl Pts',(6.67929089200952,12.2,8.21781432936106));
#213522=CARTESIAN_POINT('Ctrl Pts',(6.68082954871729,12.2,8.22089394298609));
#213523=CARTESIAN_POINT('Ctrl Pts',(6.68237419135549,12.2,8.22400281753944));
#213524=CARTESIAN_POINT('Ctrl Pts',(6.68392447875549,12.2,8.22714078184781));
#213525=CARTESIAN_POINT('Ctrl Pts',(6.68609488138585,12.2,8.23153393242677));
#213526=CARTESIAN_POINT('Ctrl Pts',(6.68827634499719,12.2,8.23598409851597));
#213527=CARTESIAN_POINT('Ctrl Pts',(6.69046794761425,12.2,8.24049081826456));
#213528=CARTESIAN_POINT('Ctrl Pts',(6.69203337803064,12.2,8.24370990374914));
#213529=CARTESIAN_POINT('Ctrl Pts',(6.69360398287526,12.2,8.24695784379444));
#213530=CARTESIAN_POINT('Ctrl Pts',(6.69517943475741,12.2,8.25023447103147));
#213531=CARTESIAN_POINT('Ctrl Pts',(6.69675488663955,12.2,8.25351109826849));
#213532=CARTESIAN_POINT('Ctrl Pts',(6.69833518289994,12.2,8.25681641326104));
#213533=CARTESIAN_POINT('Ctrl Pts',(6.69992000248327,12.2,8.26015025048325));
#213534=CARTESIAN_POINT('Ctrl Pts',(6.7015048220666,12.2,8.26348408770545));
#213535=CARTESIAN_POINT('Ctrl Pts',(6.70309416312688,12.2,8.26684644767516));
#213536=CARTESIAN_POINT('Ctrl Pts',(6.7046877110508,12.2,8.2702371665101));
#213537=CARTESIAN_POINT('Ctrl Pts',(6.70628125897473,12.2,8.27362788534503));
#213538=CARTESIAN_POINT('Ctrl Pts',(6.70787901275451,12.2,8.27704696277963));
#213539=CARTESIAN_POINT('Ctrl Pts',(6.70948065983804,12.2,8.28049423743388));
#213540=CARTESIAN_POINT('Ctrl Pts',(6.71108230692158,12.2,8.28394151208813));
#213541=CARTESIAN_POINT('Ctrl Pts',(6.71268784678278,12.2,8.28741698396107));
#213542=CARTESIAN_POINT('Ctrl Pts',(6.71429697379686,12.2,8.29092049125421));
#213543=CARTESIAN_POINT('Ctrl Pts',(6.7162279261436,12.2,8.29512469985322));
#213544=CARTESIAN_POINT('Ctrl Pts',(6.71816404306076,12.2,8.29936928126761));
#213545=CARTESIAN_POINT('Ctrl Pts',(6.72010480449906,12.2,8.30365395796463));
#213546=CARTESIAN_POINT('Ctrl Pts',(6.72172210575639,12.2,8.30722452200856));
#213547=CARTESIAN_POINT('Ctrl Pts',(6.72334263070548,12.2,8.31082293178325));
#213548=CARTESIAN_POINT('Ctrl Pts',(6.7249660861916,12.2,8.31444902824158));
#213549=CARTESIAN_POINT('Ctrl Pts',(6.72658954167771,12.2,8.31807512469991));
#213550=CARTESIAN_POINT('Ctrl Pts',(6.72821592633883,12.2,8.32172890851102));
#213551=CARTESIAN_POINT('Ctrl Pts',(6.72984494869994,12.2,8.32541022177491));
#213552=CARTESIAN_POINT('Ctrl Pts',(6.73147397106104,12.2,8.32909153503879));
#213553=CARTESIAN_POINT('Ctrl Pts',(6.7331056319434,12.2,8.33280038045713));
#213554=CARTESIAN_POINT('Ctrl Pts',(6.7347396442425,12.2,8.33653659950195));
#213555=CARTESIAN_POINT('Ctrl Pts',(6.73637365654159,12.2,8.34027281854678));
#213556=CARTESIAN_POINT('Ctrl Pts',(6.73801002092921,12.2,8.34403641308545));
#213557=CARTESIAN_POINT('Ctrl Pts',(6.73964845558211,12.2,8.347827227948));
#213558=CARTESIAN_POINT('Ctrl Pts',(6.741286890235,12.2,8.35161804281056));
#213559=CARTESIAN_POINT('Ctrl Pts',(6.74292739366837,12.2,8.355436079239));
#213560=CARTESIAN_POINT('Ctrl Pts',(6.74456969005736,12.2,8.35928118326822));
#213561=CARTESIAN_POINT('Ctrl Pts',(6.74588352706115,12.2,8.36235726624014));
#213562=CARTESIAN_POINT('Ctrl Pts',(6.7471985122176,12.2,8.36545067278518));
#213563=CARTESIAN_POINT('Ctrl Pts',(6.74851450350898,12.2,8.36856132507363));
#213564=CARTESIAN_POINT('Ctrl Pts',(6.74983049497967,12.2,8.3716719777859));
#213565=CARTESIAN_POINT('Ctrl Pts',(6.75114749275803,12.2,8.37479987469578));
#213566=CARTESIAN_POINT('Ctrl Pts',(6.75246536060769,12.2,8.37794494075719));
#213567=CARTESIAN_POINT('Ctrl Pts',(6.75378322827778,12.2,8.38109000639009));
#213568=CARTESIAN_POINT('Ctrl Pts',(6.75510196406992,12.2,8.38425223983344));
#213569=CARTESIAN_POINT('Ctrl Pts',(6.75642143251754,12.2,8.38743156473844));
#213570=CARTESIAN_POINT('Ctrl Pts',(6.75774090114493,12.2,8.39061089007662));
#213571=CARTESIAN_POINT('Ctrl Pts',(6.75906110102841,12.2,8.39380730742622));
#213572=CARTESIAN_POINT('Ctrl Pts',(6.76038189955084,12.2,8.39702073822711));
#213573=CARTESIAN_POINT('Ctrl Pts',(6.76170269789331,12.2,8.40023416859018));
#213574=CARTESIAN_POINT('Ctrl Pts',(6.76302409172527,12.2,8.40346461550287));
#213575=CARTESIAN_POINT('Ctrl Pts',(6.76434595028382,12.2,8.40671199923564));
#213576=CARTESIAN_POINT('Ctrl Pts',(6.76566780902246,12.2,8.40995938341088));
#213577=CARTESIAN_POINT('Ctrl Pts',(6.76699013193896,12.2,8.41322370691553));
#213578=CARTESIAN_POINT('Ctrl Pts',(6.76831278723328,12.2,8.41650489298325));
#213579=CARTESIAN_POINT('Ctrl Pts',(6.76963544252758,12.2,8.41978607905095));
#213580=CARTESIAN_POINT('Ctrl Pts',(6.77095842881082,12.2,8.4230841286762));
#213581=CARTESIAN_POINT('Ctrl Pts',(6.77228161821629,12.2,8.42639896485858));
#213582=CARTESIAN_POINT('Ctrl Pts',(6.77360480744148,12.2,8.42971380058932));
#213583=CARTESIAN_POINT('Ctrl Pts',(6.77492819831234,12.2,8.43304542463677));
#213584=CARTESIAN_POINT('Ctrl Pts',(6.77625166276571,12.2,8.43639376098931));
#213585=CARTESIAN_POINT('Ctrl Pts',(6.77757512739941,12.2,8.43974209779807));
#213586=CARTESIAN_POINT('Ctrl Pts',(6.77889866503309,12.2,8.44310714774182));
#213587=CARTESIAN_POINT('Ctrl Pts',(6.78022214921633,12.2,8.44648883576116));
#213588=CARTESIAN_POINT('Ctrl Pts',(6.78154563321924,12.2,8.44987052331975));
#213589=CARTESIAN_POINT('Ctrl Pts',(6.78286906468882,12.2,8.45326884904839));
#213590=CARTESIAN_POINT('Ctrl Pts',(6.78419231535843,12.2,8.45668373871257));
#213591=CARTESIAN_POINT('Ctrl Pts',(6.78551556620833,12.2,8.46009862884203));
#213592=CARTESIAN_POINT('Ctrl Pts',(6.78683863867041,12.2,8.46353008264707));
#213593=CARTESIAN_POINT('Ctrl Pts',(6.78816140814188,12.2,8.46697802750866));
#213594=CARTESIAN_POINT('Ctrl Pts',(6.78948417743313,12.2,8.47042597190047));
#213595=CARTESIAN_POINT('Ctrl Pts',(6.79080664278882,12.2,8.4738904071873));
#213596=CARTESIAN_POINT('Ctrl Pts',(6.7921286821252,12.2,8.47737125829051));
#213597=CARTESIAN_POINT('Ctrl Pts',(6.79345072164171,12.2,8.48085210986798));
#213598=CARTESIAN_POINT('Ctrl Pts',(6.79477233533599,12.2,8.48434937936146));
#213599=CARTESIAN_POINT('Ctrl Pts',(6.7960934020746,12.2,8.48786299155397));
#213600=CARTESIAN_POINT('Ctrl Pts',(6.79741446863322,12.2,8.49137660326776));
#213601=CARTESIAN_POINT('Ctrl Pts',(6.79873498728644,12.2,8.49490656004127));
#213602=CARTESIAN_POINT('Ctrl Pts',(6.80005483930009,12.2,8.49845278776043));
#213603=CARTESIAN_POINT('Ctrl Pts',(6.80170465445202,12.2,8.50288557277178));
#213604=CARTESIAN_POINT('Ctrl Pts',(6.80335342639768,12.2,8.50734378141373));
#213605=CARTESIAN_POINT('Ctrl Pts',(6.80500092563386,12.2,8.51182727148185));
#213606=CARTESIAN_POINT('Ctrl Pts',(6.80631892509463,12.2,8.51541406373182));
#213607=CARTESIAN_POINT('Ctrl Pts',(6.80763610905532,12.2,8.51901703822544));
#213608=CARTESIAN_POINT('Ctrl Pts',(6.80895236184921,12.2,8.52263612097927));
#213609=CARTESIAN_POINT('Ctrl Pts',(6.81026861446377,12.2,8.52625520324002));
#213610=CARTESIAN_POINT('Ctrl Pts',(6.81158393472871,12.2,8.52989039369603));
#213611=CARTESIAN_POINT('Ctrl Pts',(6.8128982075759,12.2,8.53354162274519));
#213612=CARTESIAN_POINT('Ctrl Pts',(6.81421248060215,12.2,8.53719285229184));
#213613=CARTESIAN_POINT('Ctrl Pts',(6.81552570710522,12.2,8.54086011752718));
#213614=CARTESIAN_POINT('Ctrl Pts',(6.81683777189887,12.2,8.54454335028452));
#213615=CARTESIAN_POINT('Ctrl Pts',(6.81814983651375,12.2,8.54822658254003));
#213616=CARTESIAN_POINT('Ctrl Pts',(6.81946073862053,12.2,8.55192577967837));
#213617=CARTESIAN_POINT('Ctrl Pts',(6.82077036673582,12.2,8.55564087265085));
#213618=CARTESIAN_POINT('Ctrl Pts',(6.82207999502956,12.2,8.5593559661295));
#213619=CARTESIAN_POINT('Ctrl Pts',(6.82338834909869,12.2,8.56308695474234));
#213620=CARTESIAN_POINT('Ctrl Pts',(6.82469531667584,12.2,8.56683376751915));
#213621=CARTESIAN_POINT('Ctrl Pts',(6.82600228407492,12.2,8.57058057978546));
#213622=CARTESIAN_POINT('Ctrl Pts',(6.82730786614041,12.2,8.57434321740655));
#213623=CARTESIAN_POINT('Ctrl Pts',(6.82861195031173,12.2,8.57812160837383));
#213624=CARTESIAN_POINT('Ctrl Pts',(6.82991603466074,12.2,8.58189999985591));
#213625=CARTESIAN_POINT('Ctrl Pts',(6.8312186238096,12.2,8.58569414577284));
#213626=CARTESIAN_POINT('Ctrl Pts',(6.83251960549162,12.2,8.58950397525826));
#213627=CARTESIAN_POINT('Ctrl Pts',(6.83382058717364,12.2,8.59331380474367));
#213628=CARTESIAN_POINT('Ctrl Pts',(6.83511996455545,12.2,8.59713931823089));
#213629=CARTESIAN_POINT('Ctrl Pts',(6.83641762690379,12.2,8.6009804463863));
#213630=CARTESIAN_POINT('Ctrl Pts',(6.83771528907532,12.2,8.60482157401836));
#213631=CARTESIAN_POINT('Ctrl Pts',(6.83901123726094,12.2,8.60867831564833));
#213632=CARTESIAN_POINT('Ctrl Pts',(6.8403053647108,12.2,8.61255060194184));
#213633=CARTESIAN_POINT('Ctrl Pts',(6.84159949233701,12.2,8.61642288876295));
#213634=CARTESIAN_POINT('Ctrl Pts',(6.84289179914979,12.2,8.62031072085456));
#213635=CARTESIAN_POINT('Ctrl Pts',(6.84418217889552,12.2,8.62421402854141));
#213636=CARTESIAN_POINT('Ctrl Pts',(6.84547255846543,12.2,8.62811733569644));
#213637=CARTESIAN_POINT('Ctrl Pts',(6.84676101244702,12.2,8.63203611887053));
#213638=CARTESIAN_POINT('Ctrl Pts',(6.84804743461977,12.2,8.63597030793678));
#213639=CARTESIAN_POINT('Ctrl Pts',(6.84933385696779,12.2,8.63990449753907));
#213640=CARTESIAN_POINT('Ctrl Pts',(6.85061824779612,12.2,8.64385409422376));
#213641=CARTESIAN_POINT('Ctrl Pts',(6.85190050408809,12.2,8.64781902910754));
#213642=CARTESIAN_POINT('Ctrl Pts',(6.85318276020535,12.2,8.6517839634511));
#213643=CARTESIAN_POINT('Ctrl Pts',(6.85446288155493,12.2,8.65576423572633));
#213644=CARTESIAN_POINT('Ctrl Pts',(6.85574076584785,12.2,8.65975977815357));
#213645=CARTESIAN_POINT('Ctrl Pts',(6.85701865031487,12.2,8.6637553211252));
#213646=CARTESIAN_POINT('Ctrl Pts',(6.85829429729866,12.2,8.66776613396156));
#213647=CARTESIAN_POINT('Ctrl Pts',(6.85956760631236,12.2,8.67179214757087));
#213648=CARTESIAN_POINT('Ctrl Pts',(6.86084091515256,12.2,8.67581816063164));
#213649=CARTESIAN_POINT('Ctrl Pts',(6.86211188526822,12.2,8.67985937619763));
#213650=CARTESIAN_POINT('Ctrl Pts',(6.86338041727588,12.2,8.68391572508671));
#213651=CARTESIAN_POINT('Ctrl Pts',(6.86464894945638,12.2,8.68797207452847));
#213652=CARTESIAN_POINT('Ctrl Pts',(6.86591504192623,12.2,8.69204355764752));
#213653=CARTESIAN_POINT('Ctrl Pts',(6.86717859700082,12.2,8.69613010727772));
#213654=CARTESIAN_POINT('Ctrl Pts',(6.86844215190325,12.2,8.70021665635113));
#213655=CARTESIAN_POINT('Ctrl Pts',(6.86970316904958,12.2,8.7043182717455));
#213656=CARTESIAN_POINT('Ctrl Pts',(6.87096155000254,12.2,8.70843488601853));
#213657=CARTESIAN_POINT('Ctrl Pts',(6.87221993112694,12.2,8.71255150085243));
#213658=CARTESIAN_POINT('Ctrl Pts',(6.873475677015,12.2,8.71668311504338));
#213659=CARTESIAN_POINT('Ctrl Pts',(6.87472868874996,12.2,8.72082965999159));
#213660=CARTESIAN_POINT('Ctrl Pts',(6.87598170048491,12.2,8.72497620493979));
#213661=CARTESIAN_POINT('Ctrl Pts',(6.87723197977511,12.2,8.72913768169534));
#213662=CARTESIAN_POINT('Ctrl Pts',(6.87847942895391,12.2,8.73331402442444));
#213663=CARTESIAN_POINT('Ctrl Pts',(6.87972687796275,12.2,8.73749036658451));
#213664=CARTESIAN_POINT('Ctrl Pts',(6.88097149858108,12.2,8.74168157270519));
#213665=CARTESIAN_POINT('Ctrl Pts',(6.88221319354078,12.2,8.74588757771374));
#213666=CARTESIAN_POINT('Ctrl Pts',(6.88345488866965,12.2,8.75009358329535));
#213667=CARTESIAN_POINT('Ctrl Pts',(6.88469365984886,12.2,8.75431438686847));
#213668=CARTESIAN_POINT('Ctrl Pts',(6.88592941219367,12.2,8.75854992293411));
#213669=CARTESIAN_POINT('Ctrl Pts',(6.88716516437011,12.2,8.76278545842266));
#213670=CARTESIAN_POINT('Ctrl Pts',(6.88839789773583,12.2,8.76703572543434));
#213671=CARTESIAN_POINT('Ctrl Pts',(6.88962751935774,12.2,8.77130065841808));
#213672=CARTESIAN_POINT('Ctrl Pts',(6.89054973561605,12.2,8.77449935830115));
#213673=CARTESIAN_POINT('Ctrl Pts',(6.89147020074281,12.2,8.77770630735176));
#213674=CARTESIAN_POINT('Ctrl Pts',(6.89238887658886,12.2,8.78092147885295));
#213675=CARTESIAN_POINT('Ctrl Pts',(6.89330755243492,12.2,8.78413665035414));
#213676=CARTESIAN_POINT('Ctrl Pts',(6.89422443993347,12.2,8.78736004319732));
#213677=CARTESIAN_POINT('Ctrl Pts',(6.89513949827547,12.2,8.79059163003711));
#213678=CARTESIAN_POINT('Ctrl Pts',(6.89605455678372,12.2,8.79382321746398));
#213679=CARTESIAN_POINT('Ctrl Pts',(6.89696778779977,12.2,8.79706299826816));
#213680=CARTESIAN_POINT('Ctrl Pts',(6.89787915218197,12.2,8.80031094615799));
#213681=CARTESIAN_POINT('Ctrl Pts',(6.89879051639861,12.2,8.80355889345778));
#213682=CARTESIAN_POINT('Ctrl Pts',(6.89970001363199,12.2,8.80681500710709));
#213683=CARTESIAN_POINT('Ctrl Pts',(6.90060760639052,12.2,8.81007925940587));
#213684=CARTESIAN_POINT('Ctrl Pts',(6.90151519914904,12.2,8.81334351170466));
#213685=CARTESIAN_POINT('Ctrl Pts',(6.90242088744619,12.2,8.81661590187384));
#213686=CARTESIAN_POINT('Ctrl Pts',(6.90332463325078,12.2,8.81989640376958));
#213687=CARTESIAN_POINT('Ctrl Pts',(6.90422837905537,12.2,8.82317690566531));
#213688=CARTESIAN_POINT('Ctrl Pts',(6.90513018234441,12.2,8.82646551955179));
#213689=CARTESIAN_POINT('Ctrl Pts',(6.90603000523247,12.2,8.82976221603026));
#213690=CARTESIAN_POINT('Ctrl Pts',(6.90692982812054,12.2,8.83305891250873));
#213691=CARTESIAN_POINT('Ctrl Pts',(6.90782767280132,12.2,8.83636369337671));
#213692=CARTESIAN_POINT('Ctrl Pts',(6.90872349864395,12.2,8.83967652938063));
#213693=CARTESIAN_POINT('Ctrl Pts',(6.90961932448657,12.2,8.84298936538455));
#213694=CARTESIAN_POINT('Ctrl Pts',(6.91051313333768,12.2,8.8463102585963));
#213695=CARTESIAN_POINT('Ctrl Pts',(6.91140488809722,12.2,8.8496391805159));
#213696=CARTESIAN_POINT('Ctrl Pts',(6.91229664301877,12.2,8.85296810304025));
#213697=CARTESIAN_POINT('Ctrl Pts',(6.91318634303141,12.2,8.85630505465857));
#213698=CARTESIAN_POINT('Ctrl Pts',(6.91407395291013,12.2,8.85965000768748));
#213699=CARTESIAN_POINT('Ctrl Pts',(6.9149615626276,12.2,8.86299496010873));
#213700=CARTESIAN_POINT('Ctrl Pts',(6.91584708057573,12.2,8.86634791455353));
#213701=CARTESIAN_POINT('Ctrl Pts',(6.91673047146252,12.2,8.86970884310027));
#213702=CARTESIAN_POINT('Ctrl Pts',(6.91761386234932,12.2,8.873069771647));
#213703=CARTESIAN_POINT('Ctrl Pts',(6.91849512742788,12.2,8.87643867454014));
#213704=CARTESIAN_POINT('Ctrl Pts',(6.91937422735408,12.2,8.87981552487648));
#213705=CARTESIAN_POINT('Ctrl Pts',(6.92025332728029,12.2,8.88319237521282));
#213706=CARTESIAN_POINT('Ctrl Pts',(6.92113026414842,12.2,8.88657717238988));
#213707=CARTESIAN_POINT('Ctrl Pts',(6.92200500149163,12.2,8.88996989022494));
#213708=CARTESIAN_POINT('Ctrl Pts',(6.92287973883485,12.2,8.89336260806001));
#213709=CARTESIAN_POINT('Ctrl Pts',(6.92375227678649,12.2,8.89676324576975));
#213710=CARTESIAN_POINT('Ctrl Pts',(6.92462257963006,12.2,8.9001717771452));
#213711=CARTESIAN_POINT('Ctrl Pts',(6.92549288247362,12.2,8.90358030852063));
#213712=CARTESIAN_POINT('Ctrl Pts',(6.92636095098704,12.2,8.90699673390843));
#213713=CARTESIAN_POINT('Ctrl Pts',(6.92722674833243,12.2,8.91042102412082));
#213714=CARTESIAN_POINT('Ctrl Pts',(6.92809254567781,12.2,8.91384531433321));
#213715=CARTESIAN_POINT('Ctrl Pts',(6.92895607180986,12.2,8.91727747197607));
#213716=CARTESIAN_POINT('Ctrl Pts',(6.92981729357054,12.2,8.92071746797501));
#213717=CARTESIAN_POINT('Ctrl Pts',(6.93067851548769,12.2,8.92415746459888));
#213718=CARTESIAN_POINT('Ctrl Pts',(6.93153743167919,12.2,8.92760530143334));
#213719=CARTESIAN_POINT('Ctrl Pts',(6.93239400717836,12.2,8.93106094997828));
#213720=CARTESIAN_POINT('Ctrl Pts',(6.93325058252192,12.2,8.93451659789544));
#213721=CARTESIAN_POINT('Ctrl Pts',(6.93410481729059,12.2,8.93798005852054));
#213722=CARTESIAN_POINT('Ctrl Pts',(6.93495667755111,12.2,8.9414513048951));
#213723=CARTESIAN_POINT('Ctrl Pts',(6.93580853781162,12.2,8.94492255126966));
#213724=CARTESIAN_POINT('Ctrl Pts',(6.93665802303074,12.2,8.94840158312663));
#213725=CARTESIAN_POINT('Ctrl Pts',(6.9375050988333,12.2,8.95188837445826));
#213726=CARTESIAN_POINT('Ctrl Pts',(6.93835217463585,12.2,8.9553751657899));
#213727=CARTESIAN_POINT('Ctrl Pts',(6.93919684097184,12.2,8.95886971554625));
#213728=CARTESIAN_POINT('Ctrl Pts',(6.94003906344145,12.2,8.96237199837663));
#213729=CARTESIAN_POINT('Ctrl Pts',(6.94088128591105,12.2,8.96587428120702));
#213730=CARTESIAN_POINT('Ctrl Pts',(6.94172106605958,12.2,8.96938429620575));
#213731=CARTESIAN_POINT('Ctrl Pts',(6.94255836807128,12.2,8.97290201679442));
#213732=CARTESIAN_POINT('Ctrl Pts',(6.94339567008296,12.2,8.9764197373831));
#213733=CARTESIAN_POINT('Ctrl Pts',(6.94423049588175,12.2,8.97994516415916));
#213734=CARTESIAN_POINT('Ctrl Pts',(6.94506280931018,12.2,8.98347826998806));
#213735=CARTESIAN_POINT('Ctrl Pts',(6.94617256064889,12.2,8.98818907818783));
#213736=CARTESIAN_POINT('Ctrl Pts',(6.94727784938442,12.2,8.99291353767225));
#213737=CARTESIAN_POINT('Ctrl Pts',(6.94837859399996,12.2,8.99765158720827));
#213738=CARTESIAN_POINT('Ctrl Pts',(6.94920415238664,12.2,9.00120512403751));
#213739=CARTESIAN_POINT('Ctrl Pts',(6.95002715535674,12.2,9.0047663038414));
#213740=CARTESIAN_POINT('Ctrl Pts',(6.95084757020216,12.2,9.00833510212772));
#213741=CARTESIAN_POINT('Ctrl Pts',(6.95166798504757,12.2,9.01190390041404));
#213742=CARTESIAN_POINT('Ctrl Pts',(6.95248581166414,12.2,9.01548031530866));
#213743=CARTESIAN_POINT('Ctrl Pts',(6.95330101663388,12.2,9.01906432277325));
#213744=CARTESIAN_POINT('Ctrl Pts',(6.95411622160362,12.2,9.02264833023785));
#213745=CARTESIAN_POINT('Ctrl Pts',(6.95492880566913,12.2,9.02623992811379));
#213746=CARTESIAN_POINT('Ctrl Pts',(6.95573873555673,12.2,9.02983909098199));
#213747=CARTESIAN_POINT('Ctrl Pts',(6.95654866559146,12.2,9.03343825450403));
#213748=CARTESIAN_POINT('Ctrl Pts',(6.95735594112546,12.2,9.03704498289489));
#213749=CARTESIAN_POINT('Ctrl Pts',(6.95816053065869,12.2,9.04065924950451));
#213750=CARTESIAN_POINT('Ctrl Pts',(6.95896512004576,12.2,9.04427351545755));
#213751=CARTESIAN_POINT('Ctrl Pts',(6.9597670234663,12.2,9.0478953207602));
#213752=CARTESIAN_POINT('Ctrl Pts',(6.96056620931203,12.2,9.05152463862899));
#213753=CARTESIAN_POINT('Ctrl Pts',(6.96136539515776,12.2,9.05515395649778));
#213754=CARTESIAN_POINT('Ctrl Pts',(6.96216186315926,12.2,9.05879078725241));
#213755=CARTESIAN_POINT('Ctrl Pts',(6.96295558050902,12.2,9.06243510451158));
#213756=CARTESIAN_POINT('Ctrl Pts',(6.96374929785877,12.2,9.06607942177076));
#213757=CARTESIAN_POINT('Ctrl Pts',(6.96454026450762,12.2,9.06973122396299));
#213758=CARTESIAN_POINT('Ctrl Pts',(6.96532844702425,12.2,9.07339048580495));
#213759=CARTESIAN_POINT('Ctrl Pts',(6.96637935714186,12.2,9.0782695020374));
#213760=CARTESIAN_POINT('Ctrl Pts',(6.96742531992227,12.2,9.08316177839994));
#213761=CARTESIAN_POINT('Ctrl Pts',(6.96846626714516,12.2,9.08806726000199));
#213762=CARTESIAN_POINT('Ctrl Pts',(6.96924697749141,12.2,9.09174637086934));
#213763=CARTESIAN_POINT('Ctrl Pts',(6.97002486692947,12.2,9.09543290893625));
#213764=CARTESIAN_POINT('Ctrl Pts',(6.97079990310939,12.2,9.0991268486777));
#213765=CARTESIAN_POINT('Ctrl Pts',(6.9718332846357,12.2,9.1040521014426));
#213766=CARTESIAN_POINT('Ctrl Pts',(6.972861590953,12.2,9.10899050989288));
#213767=CARTESIAN_POINT('Ctrl Pts',(6.97388473364314,12.2,9.11394199978984));
#213768=CARTESIAN_POINT('Ctrl Pts',(6.97465209069559,12.2,9.11765561738122));
#213769=CARTESIAN_POINT('Ctrl Pts',(6.97541654334455,12.2,9.12137659300695));
#213770=CARTESIAN_POINT('Ctrl Pts',(6.97617807056728,12.2,9.12510490870382));
#213771=CARTESIAN_POINT('Ctrl Pts',(6.97719344028981,12.2,9.13007599675117));
#213772=CARTESIAN_POINT('Ctrl Pts',(6.97820360405943,12.2,9.13506013363826));
#213773=CARTESIAN_POINT('Ctrl Pts',(6.97920857099994,12.2,9.14005731499999));
#213774=CARTESIAN_POINT('Origin',(-5.66257110645729E-14,15.2,-1.77635683940025E-14));
#213775=CARTESIAN_POINT('',(5.36127880565669,15.2,8.88241603231688));
#213776=CARTESIAN_POINT('',(5.36127880565669,12.2,8.88241603231688));
#213777=CARTESIAN_POINT('',(5.36127880599994,15.2,8.88241603199998));
#213778=CARTESIAN_POINT('Origin',(-5.66257110645729E-14,12.2,-1.77635683940025E-14));
#213779=CARTESIAN_POINT('Origin',(-5.66257110645729E-14,15.2,-1.77635683940025E-14));
#213780=CARTESIAN_POINT('Origin',(-5.66257110645729E-14,15.2,-1.77635683940025E-14));
#213781=CARTESIAN_POINT('',(5.60740451299995,15.2,10.04026965));
#213782=CARTESIAN_POINT('',(5.2693970185908,15.2,10.2217148785196));
#213783=CARTESIAN_POINT('Origin',(-5.66257110645729E-14,15.2,-1.77635683940025E-14));
#213784=CARTESIAN_POINT('',(5.2693970185908,12.2,10.2217148785196));
#213785=CARTESIAN_POINT('',(5.26939701899994,15.2,10.221714879));
#213786=CARTESIAN_POINT('',(5.60740451299995,12.2,10.04026965));
#213787=CARTESIAN_POINT('Origin',(-5.66257110645729E-14,12.2,-1.77635683940025E-14));
#213788=CARTESIAN_POINT('',(5.60740451299995,15.2,10.04026965));
#213789=CARTESIAN_POINT('Ctrl Pts',(5.36127880499994,15.2,8.88241603299999));
#213790=CARTESIAN_POINT('Ctrl Pts',(5.36127880499994,11.6,8.88241603299999));
#213791=CARTESIAN_POINT('Ctrl Pts',(5.36135574299994,15.2,8.88257249699999));
#213792=CARTESIAN_POINT('Ctrl Pts',(5.36135574299994,11.6,8.88257249699999));
#213793=CARTESIAN_POINT('Ctrl Pts',(5.36151222899994,15.2,8.88289092999998));
#213794=CARTESIAN_POINT('Ctrl Pts',(5.36151222899994,11.6,8.88289092999998));
#213795=CARTESIAN_POINT('Ctrl Pts',(5.36174910299994,15.2,8.88337354899999));
#213796=CARTESIAN_POINT('Ctrl Pts',(5.36174910299994,11.6,8.88337354899999));
#213797=CARTESIAN_POINT('Ctrl Pts',(5.36206770999994,15.2,8.88402391699999));
#213798=CARTESIAN_POINT('Ctrl Pts',(5.36206770999994,11.6,8.88402391699999));
#213799=CARTESIAN_POINT('Ctrl Pts',(5.36246987999994,15.2,8.88484693899999));
#213800=CARTESIAN_POINT('Ctrl Pts',(5.36246987999994,11.6,8.88484693899999));
#213801=CARTESIAN_POINT('Ctrl Pts',(5.36287772799994,15.2,8.88568370999998));
#213802=CARTESIAN_POINT('Ctrl Pts',(5.36287772799994,11.6,8.88568370999998));
#213803=CARTESIAN_POINT('Ctrl Pts',(5.36328889699995,15.2,8.88652944599999));
#213804=CARTESIAN_POINT('Ctrl Pts',(5.36328889699995,11.6,8.88652944599999));
#213805=CARTESIAN_POINT('Ctrl Pts',(5.36370335799995,15.2,8.88738413199999));
#213806=CARTESIAN_POINT('Ctrl Pts',(5.36370335799995,11.6,8.88738413199999));
#213807=CARTESIAN_POINT('Ctrl Pts',(5.36412108299994,15.2,8.88824774999998));
#213808=CARTESIAN_POINT('Ctrl Pts',(5.36412108299994,11.6,8.88824774999998));
#213809=CARTESIAN_POINT('Ctrl Pts',(5.36454204499995,15.2,8.88912028399999));
#213810=CARTESIAN_POINT('Ctrl Pts',(5.36454204499995,11.6,8.88912028399999));
#213811=CARTESIAN_POINT('Ctrl Pts',(5.36496621399994,15.2,8.89000171999999));
#213812=CARTESIAN_POINT('Ctrl Pts',(5.36496621399994,11.6,8.89000171999999));
#213813=CARTESIAN_POINT('Ctrl Pts',(5.36539356699994,15.2,8.89089203999998));
#213814=CARTESIAN_POINT('Ctrl Pts',(5.36539356699994,11.6,8.89089203999998));
#213815=CARTESIAN_POINT('Ctrl Pts',(5.36582407199995,15.2,8.89179122799998));
#213816=CARTESIAN_POINT('Ctrl Pts',(5.36582407199995,11.6,8.89179122799998));
#213817=CARTESIAN_POINT('Ctrl Pts',(5.36625770499994,15.2,8.89269926899999));
#213818=CARTESIAN_POINT('Ctrl Pts',(5.36625770499994,11.6,8.89269926899999));
#213819=CARTESIAN_POINT('Ctrl Pts',(5.36669443599994,15.2,8.89361614499999));
#213820=CARTESIAN_POINT('Ctrl Pts',(5.36669443599994,11.6,8.89361614499999));
#213821=CARTESIAN_POINT('Ctrl Pts',(5.36713423999994,15.2,8.89454184299998));
#213822=CARTESIAN_POINT('Ctrl Pts',(5.36713423999994,11.6,8.89454184299998));
#213823=CARTESIAN_POINT('Ctrl Pts',(5.36757708999994,15.2,8.89547634599998));
#213824=CARTESIAN_POINT('Ctrl Pts',(5.36757708999994,11.6,8.89547634599998));
#213825=CARTESIAN_POINT('Ctrl Pts',(5.36802295899994,15.2,8.89641963799999));
#213826=CARTESIAN_POINT('Ctrl Pts',(5.36802295899994,11.6,8.89641963799999));
#213827=CARTESIAN_POINT('Ctrl Pts',(5.36847181899994,15.2,8.89737170399999));
#213828=CARTESIAN_POINT('Ctrl Pts',(5.36847181899994,11.6,8.89737170399999));
#213829=CARTESIAN_POINT('Ctrl Pts',(5.36892364499994,15.2,8.89833252799999));
#213830=CARTESIAN_POINT('Ctrl Pts',(5.36892364499994,11.6,8.89833252799999));
#213831=CARTESIAN_POINT('Ctrl Pts',(5.36937841199994,15.2,8.89930209499998));
#213832=CARTESIAN_POINT('Ctrl Pts',(5.36937841199994,11.6,8.89930209499998));
#213833=CARTESIAN_POINT('Ctrl Pts',(5.36983609099994,15.2,8.90028038899998));
#213834=CARTESIAN_POINT('Ctrl Pts',(5.36983609099994,11.6,8.90028038899998));
#213835=CARTESIAN_POINT('Ctrl Pts',(5.37029665799994,15.2,8.90126739499999));
#213836=CARTESIAN_POINT('Ctrl Pts',(5.37029665799994,11.6,8.90126739499999));
#213837=CARTESIAN_POINT('Ctrl Pts',(5.37076008699994,15.2,8.90226309799999));
#213838=CARTESIAN_POINT('Ctrl Pts',(5.37076008699994,11.6,8.90226309799999));
#213839=CARTESIAN_POINT('Ctrl Pts',(5.37122634999994,15.2,8.90326748199998));
#213840=CARTESIAN_POINT('Ctrl Pts',(5.37122634999994,11.6,8.90326748199998));
#213841=CARTESIAN_POINT('Ctrl Pts',(5.37169542399995,15.2,8.90428053199999));
#213842=CARTESIAN_POINT('Ctrl Pts',(5.37169542399995,11.6,8.90428053199999));
#213843=CARTESIAN_POINT('Ctrl Pts',(5.37216728199994,15.2,8.90530223299999));
#213844=CARTESIAN_POINT('Ctrl Pts',(5.37216728199994,11.6,8.90530223299999));
#213845=CARTESIAN_POINT('Ctrl Pts',(5.37264189899994,15.2,8.90633256999998));
#213846=CARTESIAN_POINT('Ctrl Pts',(5.37264189899994,11.6,8.90633256999998));
#213847=CARTESIAN_POINT('Ctrl Pts',(5.37311924999995,15.2,8.90737152799998));
#213848=CARTESIAN_POINT('Ctrl Pts',(5.37311924999995,11.6,8.90737152799998));
#213849=CARTESIAN_POINT('Ctrl Pts',(5.37359930999994,15.2,8.90841909199998));
#213850=CARTESIAN_POINT('Ctrl Pts',(5.37359930999994,11.6,8.90841909199998));
#213851=CARTESIAN_POINT('Ctrl Pts',(5.37408205299994,15.2,8.90947524699998));
#213852=CARTESIAN_POINT('Ctrl Pts',(5.37408205299994,11.6,8.90947524699998));
#213853=CARTESIAN_POINT('Ctrl Pts',(5.37456745499994,15.2,8.91053997799998));
#213854=CARTESIAN_POINT('Ctrl Pts',(5.37456745499994,11.6,8.91053997799998));
#213855=CARTESIAN_POINT('Ctrl Pts',(5.37505548999994,15.2,8.91161327199999));
#213856=CARTESIAN_POINT('Ctrl Pts',(5.37505548999994,11.6,8.91161327199999));
#213857=CARTESIAN_POINT('Ctrl Pts',(5.37554613599994,15.2,8.91269511099999));
#213858=CARTESIAN_POINT('Ctrl Pts',(5.37554613599994,11.6,8.91269511099999));
#213859=CARTESIAN_POINT('Ctrl Pts',(5.37603936499995,15.2,8.91378548299999));
#213860=CARTESIAN_POINT('Ctrl Pts',(5.37603936499995,11.6,8.91378548299999));
#213861=CARTESIAN_POINT('Ctrl Pts',(5.37653515399994,15.2,8.91488437299999));
#213862=CARTESIAN_POINT('Ctrl Pts',(5.37653515399994,11.6,8.91488437299999));
#213863=CARTESIAN_POINT('Ctrl Pts',(5.37703347999994,15.2,8.91599176499999));
#213864=CARTESIAN_POINT('Ctrl Pts',(5.37703347999994,11.6,8.91599176499999));
#213865=CARTESIAN_POINT('Ctrl Pts',(5.37753431699994,15.2,8.91710764599999));
#213866=CARTESIAN_POINT('Ctrl Pts',(5.37753431699994,11.6,8.91710764599999));
#213867=CARTESIAN_POINT('Ctrl Pts',(5.37803764199994,15.2,8.91823200099999));
#213868=CARTESIAN_POINT('Ctrl Pts',(5.37803764199994,11.6,8.91823200099999));
#213869=CARTESIAN_POINT('Ctrl Pts',(5.37854343099994,15.2,8.91936481499998));
#213870=CARTESIAN_POINT('Ctrl Pts',(5.37854343099994,11.6,8.91936481499998));
#213871=CARTESIAN_POINT('Ctrl Pts',(5.37905165999994,15.2,8.92050607499998));
#213872=CARTESIAN_POINT('Ctrl Pts',(5.37905165999994,11.6,8.92050607499998));
#213873=CARTESIAN_POINT('Ctrl Pts',(5.37956230399994,15.2,8.92165576499998));
#213874=CARTESIAN_POINT('Ctrl Pts',(5.37956230399994,11.6,8.92165576499998));
#213875=CARTESIAN_POINT('Ctrl Pts',(5.38007534199994,15.2,8.92281387299998));
#213876=CARTESIAN_POINT('Ctrl Pts',(5.38007534199994,11.6,8.92281387299998));
#213877=CARTESIAN_POINT('Ctrl Pts',(5.38059074799994,15.2,8.92398038299999));
#213878=CARTESIAN_POINT('Ctrl Pts',(5.38059074799994,11.6,8.92398038299999));
#213879=CARTESIAN_POINT('Ctrl Pts',(5.38110849899994,15.2,8.92515528099998));
#213880=CARTESIAN_POINT('Ctrl Pts',(5.38110849899994,11.6,8.92515528099998));
#213881=CARTESIAN_POINT('Ctrl Pts',(5.38162857399994,15.2,8.92633855399998));
#213882=CARTESIAN_POINT('Ctrl Pts',(5.38162857399994,11.6,8.92633855399998));
#213883=CARTESIAN_POINT('Ctrl Pts',(5.38215094699994,15.2,8.92753018699998));
#213884=CARTESIAN_POINT('Ctrl Pts',(5.38215094699994,11.6,8.92753018699998));
#213885=CARTESIAN_POINT('Ctrl Pts',(5.38267559599994,15.2,8.92873016599999));
#213886=CARTESIAN_POINT('Ctrl Pts',(5.38267559599994,11.6,8.92873016599999));
#213887=CARTESIAN_POINT('Ctrl Pts',(5.38320249799994,15.2,8.92993847799998));
#213888=CARTESIAN_POINT('Ctrl Pts',(5.38320249799994,11.6,8.92993847799998));
#213889=CARTESIAN_POINT('Ctrl Pts',(5.38373163099994,15.2,8.93115510699998));
#213890=CARTESIAN_POINT('Ctrl Pts',(5.38373163099994,11.6,8.93115510699998));
#213891=CARTESIAN_POINT('Ctrl Pts',(5.38426297099994,15.2,8.93238004199999));
#213892=CARTESIAN_POINT('Ctrl Pts',(5.38426297099994,11.6,8.93238004199999));
#213893=CARTESIAN_POINT('Ctrl Pts',(5.38479649699994,15.2,8.93361326699999));
#213894=CARTESIAN_POINT('Ctrl Pts',(5.38479649699994,11.6,8.93361326699999));
#213895=CARTESIAN_POINT('Ctrl Pts',(5.38533218399994,15.2,8.93485476999999));
#213896=CARTESIAN_POINT('Ctrl Pts',(5.38533218399994,11.6,8.93485476999999));
#213897=CARTESIAN_POINT('Ctrl Pts',(5.38587001199994,15.2,8.93610453599998));
#213898=CARTESIAN_POINT('Ctrl Pts',(5.38587001199994,11.6,8.93610453599998));
#213899=CARTESIAN_POINT('Ctrl Pts',(5.38640995699994,15.2,8.93736255199999));
#213900=CARTESIAN_POINT('Ctrl Pts',(5.38640995699994,11.6,8.93736255199999));
#213901=CARTESIAN_POINT('Ctrl Pts',(5.38695199599994,15.2,8.93862880299999));
#213902=CARTESIAN_POINT('Ctrl Pts',(5.38695199599994,11.6,8.93862880299999));
#213903=CARTESIAN_POINT('Ctrl Pts',(5.38749611099994,15.2,8.93990327699999));
#213904=CARTESIAN_POINT('Ctrl Pts',(5.38749611099994,11.6,8.93990327699999));
#213905=CARTESIAN_POINT('Ctrl Pts',(5.38804227499995,15.2,8.94118596099998));
#213906=CARTESIAN_POINT('Ctrl Pts',(5.38804227499995,11.6,8.94118596099998));
#213907=CARTESIAN_POINT('Ctrl Pts',(5.38859046899994,15.2,8.94247683999998));
#213908=CARTESIAN_POINT('Ctrl Pts',(5.38859046899994,11.6,8.94247683999998));
#213909=CARTESIAN_POINT('Ctrl Pts',(5.38914067099994,15.2,8.94377590099998));
#213910=CARTESIAN_POINT('Ctrl Pts',(5.38914067099994,11.6,8.94377590099998));
#213911=CARTESIAN_POINT('Ctrl Pts',(5.38969285799995,15.2,8.94508313099998));
#213912=CARTESIAN_POINT('Ctrl Pts',(5.38969285799995,11.6,8.94508313099998));
#213913=CARTESIAN_POINT('Ctrl Pts',(5.39024700899994,15.2,8.94639851699999));
#213914=CARTESIAN_POINT('Ctrl Pts',(5.39024700899994,11.6,8.94639851699999));
#213915=CARTESIAN_POINT('Ctrl Pts',(5.39080310299994,15.2,8.94772204399998));
#213916=CARTESIAN_POINT('Ctrl Pts',(5.39080310299994,11.6,8.94772204399998));
#213917=CARTESIAN_POINT('Ctrl Pts',(5.39136111799994,15.2,8.94905370099998));
#213918=CARTESIAN_POINT('Ctrl Pts',(5.39136111799994,11.6,8.94905370099998));
#213919=CARTESIAN_POINT('Ctrl Pts',(5.39192103299994,15.2,8.95039347299999));
#213920=CARTESIAN_POINT('Ctrl Pts',(5.39192103299994,11.6,8.95039347299999));
#213921=CARTESIAN_POINT('Ctrl Pts',(5.39248282599995,15.2,8.95174134799999));
#213922=CARTESIAN_POINT('Ctrl Pts',(5.39248282599995,11.6,8.95174134799999));
#213923=CARTESIAN_POINT('Ctrl Pts',(5.39304647699994,15.2,8.95309731199998));
#213924=CARTESIAN_POINT('Ctrl Pts',(5.39304647699994,11.6,8.95309731199998));
#213925=CARTESIAN_POINT('Ctrl Pts',(5.39361196299994,15.2,8.95446135399999));
#213926=CARTESIAN_POINT('Ctrl Pts',(5.39361196299994,11.6,8.95446135399999));
#213927=CARTESIAN_POINT('Ctrl Pts',(5.39417926699994,15.2,8.95583345799999));
#213928=CARTESIAN_POINT('Ctrl Pts',(5.39417926699994,11.6,8.95583345799999));
#213929=CARTESIAN_POINT('Ctrl Pts',(5.39474836399994,15.2,8.95721361199998));
#213930=CARTESIAN_POINT('Ctrl Pts',(5.39474836399994,11.6,8.95721361199998));
#213931=CARTESIAN_POINT('Ctrl Pts',(5.39531923399994,15.2,8.95860180399998));
#213932=CARTESIAN_POINT('Ctrl Pts',(5.39531923399994,11.6,8.95860180399998));
#213933=CARTESIAN_POINT('Ctrl Pts',(5.39589185799994,15.2,8.95999802199999));
#213934=CARTESIAN_POINT('Ctrl Pts',(5.39589185799994,11.6,8.95999802199999));
#213935=CARTESIAN_POINT('Ctrl Pts',(5.39646621499994,15.2,8.96140224899998));
#213936=CARTESIAN_POINT('Ctrl Pts',(5.39646621499994,11.6,8.96140224899998));
#213937=CARTESIAN_POINT('Ctrl Pts',(5.39704228299994,15.2,8.96281447699998));
#213938=CARTESIAN_POINT('Ctrl Pts',(5.39704228299994,11.6,8.96281447699998));
#213939=CARTESIAN_POINT('Ctrl Pts',(5.39762004199994,15.2,8.96423468999998));
#213940=CARTESIAN_POINT('Ctrl Pts',(5.39762004199994,11.6,8.96423468999998));
#213941=CARTESIAN_POINT('Ctrl Pts',(5.39819947299994,15.2,8.96566287699999));
#213942=CARTESIAN_POINT('Ctrl Pts',(5.39819947299994,11.6,8.96566287699999));
#213943=CARTESIAN_POINT('Ctrl Pts',(5.39878055599995,15.2,8.96709902399999));
#213944=CARTESIAN_POINT('Ctrl Pts',(5.39878055599995,11.6,8.96709902399999));
#213945=CARTESIAN_POINT('Ctrl Pts',(5.39936326899994,15.2,8.96854311899999));
#213946=CARTESIAN_POINT('Ctrl Pts',(5.39936326899994,11.6,8.96854311899999));
#213947=CARTESIAN_POINT('Ctrl Pts',(5.39994759199994,15.2,8.96999514999998));
#213948=CARTESIAN_POINT('Ctrl Pts',(5.39994759199994,11.6,8.96999514999998));
#213949=CARTESIAN_POINT('Ctrl Pts',(5.40053350699995,15.2,8.97145510299998));
#213950=CARTESIAN_POINT('Ctrl Pts',(5.40053350699995,11.6,8.97145510299998));
#213951=CARTESIAN_POINT('Ctrl Pts',(5.40112099199994,15.2,8.97292296699998));
#213952=CARTESIAN_POINT('Ctrl Pts',(5.40112099199994,11.6,8.97292296699998));
#213953=CARTESIAN_POINT('Ctrl Pts',(5.40171002799994,15.2,8.97439872899999));
#213954=CARTESIAN_POINT('Ctrl Pts',(5.40171002799994,11.6,8.97439872899999));
#213955=CARTESIAN_POINT('Ctrl Pts',(5.40230059699994,15.2,8.97588237599999));
#213956=CARTESIAN_POINT('Ctrl Pts',(5.40230059699994,11.6,8.97588237599999));
#213957=CARTESIAN_POINT('Ctrl Pts',(5.40289267599994,15.2,8.97737389499999));
#213958=CARTESIAN_POINT('Ctrl Pts',(5.40289267599994,11.6,8.97737389499999));
#213959=CARTESIAN_POINT('Ctrl Pts',(5.40348624899995,15.2,8.97887327499999));
#213960=CARTESIAN_POINT('Ctrl Pts',(5.40348624899995,11.6,8.97887327499999));
#213961=CARTESIAN_POINT('Ctrl Pts',(5.40408129299994,15.2,8.98038050299999));
#213962=CARTESIAN_POINT('Ctrl Pts',(5.40408129299994,11.6,8.98038050299999));
#213963=CARTESIAN_POINT('Ctrl Pts',(5.40467779099994,15.2,8.98189556699998));
#213964=CARTESIAN_POINT('Ctrl Pts',(5.40467779099994,11.6,8.98189556699998));
#213965=CARTESIAN_POINT('Ctrl Pts',(5.40527572299994,15.2,8.98341845499999));
#213966=CARTESIAN_POINT('Ctrl Pts',(5.40527572299994,11.6,8.98341845499999));
#213967=CARTESIAN_POINT('Ctrl Pts',(5.40587506999994,15.2,8.98494915299998));
#213968=CARTESIAN_POINT('Ctrl Pts',(5.40587506999994,11.6,8.98494915299998));
#213969=CARTESIAN_POINT('Ctrl Pts',(5.40647581199994,15.2,8.98648765099999));
#213970=CARTESIAN_POINT('Ctrl Pts',(5.40647581199994,11.6,8.98648765099999));
#213971=CARTESIAN_POINT('Ctrl Pts',(5.40707793099994,15.2,8.98803393599999));
#213972=CARTESIAN_POINT('Ctrl Pts',(5.40707793099994,11.6,8.98803393599999));
#213973=CARTESIAN_POINT('Ctrl Pts',(5.40768140799995,15.2,8.98958799599999));
#213974=CARTESIAN_POINT('Ctrl Pts',(5.40768140799995,11.6,8.98958799599999));
#213975=CARTESIAN_POINT('Ctrl Pts',(5.40828622299994,15.2,8.99114981699999));
#213976=CARTESIAN_POINT('Ctrl Pts',(5.40828622299994,11.6,8.99114981699999));
#213977=CARTESIAN_POINT('Ctrl Pts',(5.40889235899994,15.2,8.99271938999998));
#213978=CARTESIAN_POINT('Ctrl Pts',(5.40889235899994,11.6,8.99271938999998));
#213979=CARTESIAN_POINT('Ctrl Pts',(5.40949979499994,15.2,8.99429669999999));
#213980=CARTESIAN_POINT('Ctrl Pts',(5.40949979499994,11.6,8.99429669999999));
#213981=CARTESIAN_POINT('Ctrl Pts',(5.41010851399994,15.2,8.99588173799999));
#213982=CARTESIAN_POINT('Ctrl Pts',(5.41010851399994,11.6,8.99588173799999));
#213983=CARTESIAN_POINT('Ctrl Pts',(5.41071849599994,15.2,8.99747448999998));
#213984=CARTESIAN_POINT('Ctrl Pts',(5.41071849599994,11.6,8.99747448999998));
#213985=CARTESIAN_POINT('Ctrl Pts',(5.41132972499994,15.2,8.99907494599999));
#213986=CARTESIAN_POINT('Ctrl Pts',(5.41132972499994,11.6,8.99907494599999));
#213987=CARTESIAN_POINT('Ctrl Pts',(5.41194217999994,15.2,9.00068309099998));
#213988=CARTESIAN_POINT('Ctrl Pts',(5.41194217999994,11.6,9.00068309099998));
#213989=CARTESIAN_POINT('Ctrl Pts',(5.41255584299994,15.2,9.00229891499999));
#213990=CARTESIAN_POINT('Ctrl Pts',(5.41255584299994,11.6,9.00229891499999));
#213991=CARTESIAN_POINT('Ctrl Pts',(5.41317069799994,15.2,9.00392240699999));
#213992=CARTESIAN_POINT('Ctrl Pts',(5.41317069799994,11.6,9.00392240699999));
#213993=CARTESIAN_POINT('Ctrl Pts',(5.41378672399994,15.2,9.00555355399998));
#213994=CARTESIAN_POINT('Ctrl Pts',(5.41378672399994,11.6,9.00555355399998));
#213995=CARTESIAN_POINT('Ctrl Pts',(5.41440390399995,15.2,9.00719234399999));
#213996=CARTESIAN_POINT('Ctrl Pts',(5.41440390399995,11.6,9.00719234399999));
#213997=CARTESIAN_POINT('Ctrl Pts',(5.41502221999994,15.2,9.00883876599998));
#213998=CARTESIAN_POINT('Ctrl Pts',(5.41502221999994,11.6,9.00883876599998));
#213999=CARTESIAN_POINT('Ctrl Pts',(5.41564165299994,15.2,9.01049280899999));
#214000=CARTESIAN_POINT('Ctrl Pts',(5.41564165299994,11.6,9.01049280899999));
#214001=CARTESIAN_POINT('Ctrl Pts',(5.41626218699994,15.2,9.01215445799998));
#214002=CARTESIAN_POINT('Ctrl Pts',(5.41626218699994,11.6,9.01215445799998));
#214003=CARTESIAN_POINT('Ctrl Pts',(5.41688380299994,15.2,9.01382370599999));
#214004=CARTESIAN_POINT('Ctrl Pts',(5.41688380299994,11.6,9.01382370599999));
#214005=CARTESIAN_POINT('Ctrl Pts',(5.41750648299994,15.2,9.01550053899999));
#214006=CARTESIAN_POINT('Ctrl Pts',(5.41750648299994,11.6,9.01550053899999));
#214007=CARTESIAN_POINT('Ctrl Pts',(5.41813020999994,15.2,9.01718494499999));
#214008=CARTESIAN_POINT('Ctrl Pts',(5.41813020999994,11.6,9.01718494499999));
#214009=CARTESIAN_POINT('Ctrl Pts',(5.41875496599994,15.2,9.01887691399999));
#214010=CARTESIAN_POINT('Ctrl Pts',(5.41875496599994,11.6,9.01887691399999));
#214011=CARTESIAN_POINT('Ctrl Pts',(5.41938073299994,15.2,9.02057643199999));
#214012=CARTESIAN_POINT('Ctrl Pts',(5.41938073299994,11.6,9.02057643199999));
#214013=CARTESIAN_POINT('Ctrl Pts',(5.42000749399994,15.2,9.02228348999999));
#214014=CARTESIAN_POINT('Ctrl Pts',(5.42000749399994,11.6,9.02228348999999));
#214015=CARTESIAN_POINT('Ctrl Pts',(5.42063523199994,15.2,9.02399807499998));
#214016=CARTESIAN_POINT('Ctrl Pts',(5.42063523199994,11.6,9.02399807499998));
#214017=CARTESIAN_POINT('Ctrl Pts',(5.42126392899994,15.2,9.02572017699999));
#214018=CARTESIAN_POINT('Ctrl Pts',(5.42126392899994,11.6,9.02572017699999));
#214019=CARTESIAN_POINT('Ctrl Pts',(5.42189356699994,15.2,9.02744978399999));
#214020=CARTESIAN_POINT('Ctrl Pts',(5.42189356699994,11.6,9.02744978399999));
#214021=CARTESIAN_POINT('Ctrl Pts',(5.42252413099994,15.2,9.02918688399998));
#214022=CARTESIAN_POINT('Ctrl Pts',(5.42252413099994,11.6,9.02918688399998));
#214023=CARTESIAN_POINT('Ctrl Pts',(5.42315560199994,15.2,9.03093146599998));
#214024=CARTESIAN_POINT('Ctrl Pts',(5.42315560199994,11.6,9.03093146599998));
#214025=CARTESIAN_POINT('Ctrl Pts',(5.42378796399994,15.2,9.03268351899998));
#214026=CARTESIAN_POINT('Ctrl Pts',(5.42378796399994,11.6,9.03268351899998));
#214027=CARTESIAN_POINT('Ctrl Pts',(5.42442119799994,15.2,9.03444303199999));
#214028=CARTESIAN_POINT('Ctrl Pts',(5.42442119799994,11.6,9.03444303199999));
#214029=CARTESIAN_POINT('Ctrl Pts',(5.42505528999994,15.2,9.03620999399998));
#214030=CARTESIAN_POINT('Ctrl Pts',(5.42505528999994,11.6,9.03620999399998));
#214031=CARTESIAN_POINT('Ctrl Pts',(5.42569022099994,15.2,9.03798439299998));
#214032=CARTESIAN_POINT('Ctrl Pts',(5.42569022099994,11.6,9.03798439299998));
#214033=CARTESIAN_POINT('Ctrl Pts',(5.42632597499994,15.2,9.03976621599998));
#214034=CARTESIAN_POINT('Ctrl Pts',(5.42632597499994,11.6,9.03976621599998));
#214035=CARTESIAN_POINT('Ctrl Pts',(5.42696253499994,15.2,9.04155545599998));
#214036=CARTESIAN_POINT('Ctrl Pts',(5.42696253499994,11.6,9.04155545599998));
#214037=CARTESIAN_POINT('Ctrl Pts',(5.42759988399994,15.2,9.04335209899998));
#214038=CARTESIAN_POINT('Ctrl Pts',(5.42759988399994,11.6,9.04335209899998));
#214039=CARTESIAN_POINT('Ctrl Pts',(5.42823800599994,15.2,9.04515613499999));
#214040=CARTESIAN_POINT('Ctrl Pts',(5.42823800599994,11.6,9.04515613499999));
#214041=CARTESIAN_POINT('Ctrl Pts',(5.42887688399994,15.2,9.04696755199998));
#214042=CARTESIAN_POINT('Ctrl Pts',(5.42887688399994,11.6,9.04696755199998));
#214043=CARTESIAN_POINT('Ctrl Pts',(5.42951650299995,15.2,9.04878633999999));
#214044=CARTESIAN_POINT('Ctrl Pts',(5.42951650299995,11.6,9.04878633999999));
#214045=CARTESIAN_POINT('Ctrl Pts',(5.43015684399994,15.2,9.05061248799999));
#214046=CARTESIAN_POINT('Ctrl Pts',(5.43015684399994,11.6,9.05061248799999));
#214047=CARTESIAN_POINT('Ctrl Pts',(5.43079789199994,15.2,9.05244598399998));
#214048=CARTESIAN_POINT('Ctrl Pts',(5.43079789199994,11.6,9.05244598399998));
#214049=CARTESIAN_POINT('Ctrl Pts',(5.43143963199994,15.2,9.05428681699998));
#214050=CARTESIAN_POINT('Ctrl Pts',(5.43143963199994,11.6,9.05428681699998));
#214051=CARTESIAN_POINT('Ctrl Pts',(5.43208204399994,15.2,9.05613497799998));
#214052=CARTESIAN_POINT('Ctrl Pts',(5.43208204399994,11.6,9.05613497799998));
#214053=CARTESIAN_POINT('Ctrl Pts',(5.43272511499994,15.2,9.05799045399998));
#214054=CARTESIAN_POINT('Ctrl Pts',(5.43272511499994,11.6,9.05799045399998));
#214055=CARTESIAN_POINT('Ctrl Pts',(5.43336882899994,15.2,9.05985323499999));
#214056=CARTESIAN_POINT('Ctrl Pts',(5.43336882899994,11.6,9.05985323499999));
#214057=CARTESIAN_POINT('Ctrl Pts',(5.43401316899994,15.2,9.06172330999999));
#214058=CARTESIAN_POINT('Ctrl Pts',(5.43401316899994,11.6,9.06172330999999));
#214059=CARTESIAN_POINT('Ctrl Pts',(5.43465811899994,15.2,9.06360066899998));
#214060=CARTESIAN_POINT('Ctrl Pts',(5.43465811899994,11.6,9.06360066899998));
#214061=CARTESIAN_POINT('Ctrl Pts',(5.43530366199994,15.2,9.06548529999998));
#214062=CARTESIAN_POINT('Ctrl Pts',(5.43530366199994,11.6,9.06548529999998));
#214063=CARTESIAN_POINT('Ctrl Pts',(5.43594978499994,15.2,9.06737719299999));
#214064=CARTESIAN_POINT('Ctrl Pts',(5.43594978499994,11.6,9.06737719299999));
#214065=CARTESIAN_POINT('Ctrl Pts',(5.43659646899994,15.2,9.06927633599998));
#214066=CARTESIAN_POINT('Ctrl Pts',(5.43659646899994,11.6,9.06927633599998));
#214067=CARTESIAN_POINT('Ctrl Pts',(5.43724370099994,15.2,9.07118272099999));
#214068=CARTESIAN_POINT('Ctrl Pts',(5.43724370099994,11.6,9.07118272099999));
#214069=CARTESIAN_POINT('Ctrl Pts',(5.43789146399994,15.2,9.07309633499998));
#214070=CARTESIAN_POINT('Ctrl Pts',(5.43789146399994,11.6,9.07309633499998));
#214071=CARTESIAN_POINT('Ctrl Pts',(5.43853974099994,15.2,9.07501716699999));
#214072=CARTESIAN_POINT('Ctrl Pts',(5.43853974099994,11.6,9.07501716699999));
#214073=CARTESIAN_POINT('Ctrl Pts',(5.43918851899994,15.2,9.07694520799998));
#214074=CARTESIAN_POINT('Ctrl Pts',(5.43918851899994,11.6,9.07694520799998));
#214075=CARTESIAN_POINT('Ctrl Pts',(5.43983778099994,15.2,9.07888044599999));
#214076=CARTESIAN_POINT('Ctrl Pts',(5.43983778099994,11.6,9.07888044599999));
#214077=CARTESIAN_POINT('Ctrl Pts',(5.44048751099994,15.2,9.08082287099998));
#214078=CARTESIAN_POINT('Ctrl Pts',(5.44048751099994,11.6,9.08082287099998));
#214079=CARTESIAN_POINT('Ctrl Pts',(5.44113769599995,15.2,9.08277247399998));
#214080=CARTESIAN_POINT('Ctrl Pts',(5.44113769599995,11.6,9.08277247399998));
#214081=CARTESIAN_POINT('Ctrl Pts',(5.44178831799995,15.2,9.08472924199998));
#214082=CARTESIAN_POINT('Ctrl Pts',(5.44178831799995,11.6,9.08472924199998));
#214083=CARTESIAN_POINT('Ctrl Pts',(5.44243936299995,15.2,9.08669316599998));
#214084=CARTESIAN_POINT('Ctrl Pts',(5.44243936299995,11.6,9.08669316599998));
#214085=CARTESIAN_POINT('Ctrl Pts',(5.44309081699994,15.2,9.08866423499998));
#214086=CARTESIAN_POINT('Ctrl Pts',(5.44309081699994,11.6,9.08866423499998));
#214087=CARTESIAN_POINT('Ctrl Pts',(5.44374266099994,15.2,9.09064243899999));
#214088=CARTESIAN_POINT('Ctrl Pts',(5.44374266099994,11.6,9.09064243899999));
#214089=CARTESIAN_POINT('Ctrl Pts',(5.44439488399994,15.2,9.09262776599999));
#214090=CARTESIAN_POINT('Ctrl Pts',(5.44439488399994,11.6,9.09262776599999));
#214091=CARTESIAN_POINT('Ctrl Pts',(5.44504746899994,15.2,9.09462020699999));
#214092=CARTESIAN_POINT('Ctrl Pts',(5.44504746899994,11.6,9.09462020699999));
#214093=CARTESIAN_POINT('Ctrl Pts',(5.44570040099994,15.2,9.09661975099999));
#214094=CARTESIAN_POINT('Ctrl Pts',(5.44570040099994,11.6,9.09661975099999));
#214095=CARTESIAN_POINT('Ctrl Pts',(5.44635366499994,15.2,9.09862638899998));
#214096=CARTESIAN_POINT('Ctrl Pts',(5.44635366499994,11.6,9.09862638899998));
#214097=CARTESIAN_POINT('Ctrl Pts',(5.44700724699994,15.2,9.10064010899998));
#214098=CARTESIAN_POINT('Ctrl Pts',(5.44700724699994,11.6,9.10064010899998));
#214099=CARTESIAN_POINT('Ctrl Pts',(5.44766113199994,15.2,9.10266090099999));
#214100=CARTESIAN_POINT('Ctrl Pts',(5.44766113199994,11.6,9.10266090099999));
#214101=CARTESIAN_POINT('Ctrl Pts',(5.44831530399994,15.2,9.10468875599998));
#214102=CARTESIAN_POINT('Ctrl Pts',(5.44831530399994,11.6,9.10468875599998));
#214103=CARTESIAN_POINT('Ctrl Pts',(5.44896974899994,15.2,9.10672366199999));
#214104=CARTESIAN_POINT('Ctrl Pts',(5.44896974899994,11.6,9.10672366199999));
#214105=CARTESIAN_POINT('Ctrl Pts',(5.44962445199995,15.2,9.10876560899998));
#214106=CARTESIAN_POINT('Ctrl Pts',(5.44962445199995,11.6,9.10876560899998));
#214107=CARTESIAN_POINT('Ctrl Pts',(5.45027939899994,15.2,9.11081458899999));
#214108=CARTESIAN_POINT('Ctrl Pts',(5.45027939899994,11.6,9.11081458899999));
#214109=CARTESIAN_POINT('Ctrl Pts',(5.45093457599994,15.2,9.11287058899998));
#214110=CARTESIAN_POINT('Ctrl Pts',(5.45093457599994,11.6,9.11287058899998));
#214111=CARTESIAN_POINT('Ctrl Pts',(5.45158996599994,15.2,9.11493359899998));
#214112=CARTESIAN_POINT('Ctrl Pts',(5.45158996599994,11.6,9.11493359899998));
#214113=CARTESIAN_POINT('Ctrl Pts',(5.45224555799994,15.2,9.11700361099999));
#214114=CARTESIAN_POINT('Ctrl Pts',(5.45224555799994,11.6,9.11700361099999));
#214115=CARTESIAN_POINT('Ctrl Pts',(5.45290133399994,15.2,9.11908061299999));
#214116=CARTESIAN_POINT('Ctrl Pts',(5.45290133399994,11.6,9.11908061299999));
#214117=CARTESIAN_POINT('Ctrl Pts',(5.45355728299994,15.2,9.12116459599999));
#214118=CARTESIAN_POINT('Ctrl Pts',(5.45355728299994,11.6,9.12116459599999));
#214119=CARTESIAN_POINT('Ctrl Pts',(5.45421338799994,15.2,9.12325554899999));
#214120=CARTESIAN_POINT('Ctrl Pts',(5.45421338799994,11.6,9.12325554899999));
#214121=CARTESIAN_POINT('Ctrl Pts',(5.45486963699994,15.2,9.12535346199999));
#214122=CARTESIAN_POINT('Ctrl Pts',(5.45486963699994,11.6,9.12535346199999));
#214123=CARTESIAN_POINT('Ctrl Pts',(5.45552601299994,15.2,9.12745832599999));
#214124=CARTESIAN_POINT('Ctrl Pts',(5.45552601299994,11.6,9.12745832599999));
#214125=CARTESIAN_POINT('Ctrl Pts',(5.45618250499994,15.2,9.12957012999998));
#214126=CARTESIAN_POINT('Ctrl Pts',(5.45618250499994,11.6,9.12957012999998));
#214127=CARTESIAN_POINT('Ctrl Pts',(5.45683909599994,15.2,9.13168886499999));
#214128=CARTESIAN_POINT('Ctrl Pts',(5.45683909599994,11.6,9.13168886499999));
#214129=CARTESIAN_POINT('Ctrl Pts',(5.45749577399994,15.2,9.13381451899999));
#214130=CARTESIAN_POINT('Ctrl Pts',(5.45749577399994,11.6,9.13381451899999));
#214131=CARTESIAN_POINT('Ctrl Pts',(5.45815252399994,15.2,9.13594708299998));
#214132=CARTESIAN_POINT('Ctrl Pts',(5.45815252399994,11.6,9.13594708299998));
#214133=CARTESIAN_POINT('Ctrl Pts',(5.45880933199994,15.2,9.13808654799999));
#214134=CARTESIAN_POINT('Ctrl Pts',(5.45880933199994,11.6,9.13808654799999));
#214135=CARTESIAN_POINT('Ctrl Pts',(5.45946618499994,15.2,9.14023290499999));
#214136=CARTESIAN_POINT('Ctrl Pts',(5.45946618499994,11.6,9.14023290499999));
#214137=CARTESIAN_POINT('Ctrl Pts',(5.46012306899994,15.2,9.14238613999999));
#214138=CARTESIAN_POINT('Ctrl Pts',(5.46012306899994,11.6,9.14238613999999));
#214139=CARTESIAN_POINT('Ctrl Pts',(5.46077996899994,15.2,9.14454624699999));
#214140=CARTESIAN_POINT('Ctrl Pts',(5.46077996899994,11.6,9.14454624699999));
#214141=CARTESIAN_POINT('Ctrl Pts',(5.46143687199994,15.2,9.14671321499998));
#214142=CARTESIAN_POINT('Ctrl Pts',(5.46143687199994,11.6,9.14671321499998));
#214143=CARTESIAN_POINT('Ctrl Pts',(5.46209376399994,15.2,9.14888703299999));
#214144=CARTESIAN_POINT('Ctrl Pts',(5.46209376399994,11.6,9.14888703299999));
#214145=CARTESIAN_POINT('Ctrl Pts',(5.46275063199994,15.2,9.15106769299998));
#214146=CARTESIAN_POINT('Ctrl Pts',(5.46275063199994,11.6,9.15106769299998));
#214147=CARTESIAN_POINT('Ctrl Pts',(5.46340746199994,15.2,9.15325518399998));
#214148=CARTESIAN_POINT('Ctrl Pts',(5.46340746199994,11.6,9.15325518399998));
#214149=CARTESIAN_POINT('Ctrl Pts',(5.46406423999994,15.2,9.15544949699999));
#214150=CARTESIAN_POINT('Ctrl Pts',(5.46406423999994,11.6,9.15544949699999));
#214151=CARTESIAN_POINT('Ctrl Pts',(5.46472095299994,15.2,9.15765062199998));
#214152=CARTESIAN_POINT('Ctrl Pts',(5.46472095299994,11.6,9.15765062199998));
#214153=CARTESIAN_POINT('Ctrl Pts',(5.46537758699994,15.2,9.15985854799998));
#214154=CARTESIAN_POINT('Ctrl Pts',(5.46537758699994,11.6,9.15985854799998));
#214155=CARTESIAN_POINT('Ctrl Pts',(5.46603412999994,15.2,9.16207326799999));
#214156=CARTESIAN_POINT('Ctrl Pts',(5.46603412999994,11.6,9.16207326799999));
#214157=CARTESIAN_POINT('Ctrl Pts',(5.46669056599994,15.2,9.16429476899999));
#214158=CARTESIAN_POINT('Ctrl Pts',(5.46669056599994,11.6,9.16429476899999));
#214159=CARTESIAN_POINT('Ctrl Pts',(5.46734688499994,15.2,9.16652304399998));
#214160=CARTESIAN_POINT('Ctrl Pts',(5.46734688499994,11.6,9.16652304399998));
#214161=CARTESIAN_POINT('Ctrl Pts',(5.46800306999994,15.2,9.16875808199999));
#214162=CARTESIAN_POINT('Ctrl Pts',(5.46800306999994,11.6,9.16875808199999));
#214163=CARTESIAN_POINT('Ctrl Pts',(5.46865911099994,15.2,9.17099987499999));
#214164=CARTESIAN_POINT('Ctrl Pts',(5.46865911099994,11.6,9.17099987499999));
#214165=CARTESIAN_POINT('Ctrl Pts',(5.46931499299994,15.2,9.17324841099998));
#214166=CARTESIAN_POINT('Ctrl Pts',(5.46931499299994,11.6,9.17324841099998));
#214167=CARTESIAN_POINT('Ctrl Pts',(5.46997070299994,15.2,9.17550368099998));
#214168=CARTESIAN_POINT('Ctrl Pts',(5.46997070299994,11.6,9.17550368099998));
#214169=CARTESIAN_POINT('Ctrl Pts',(5.47062622799994,15.2,9.17776567599999));
#214170=CARTESIAN_POINT('Ctrl Pts',(5.47062622799994,11.6,9.17776567599999));
#214171=CARTESIAN_POINT('Ctrl Pts',(5.47128155699994,15.2,9.18003438799998));
#214172=CARTESIAN_POINT('Ctrl Pts',(5.47128155699994,11.6,9.18003438799998));
#214173=CARTESIAN_POINT('Ctrl Pts',(5.47193667299994,15.2,9.18230980399999));
#214174=CARTESIAN_POINT('Ctrl Pts',(5.47193667299994,11.6,9.18230980399999));
#214175=CARTESIAN_POINT('Ctrl Pts',(5.47259156599995,15.2,9.18459191699998));
#214176=CARTESIAN_POINT('Ctrl Pts',(5.47259156599995,11.6,9.18459191699998));
#214177=CARTESIAN_POINT('Ctrl Pts',(5.47324622199994,15.2,9.18688071699999));
#214178=CARTESIAN_POINT('Ctrl Pts',(5.47324622199994,11.6,9.18688071699999));
#214179=CARTESIAN_POINT('Ctrl Pts',(5.47390062799994,15.2,9.18917619399998));
#214180=CARTESIAN_POINT('Ctrl Pts',(5.47390062799994,11.6,9.18917619399998));
#214181=CARTESIAN_POINT('Ctrl Pts',(5.47455477099994,15.2,9.19147833999999));
#214182=CARTESIAN_POINT('Ctrl Pts',(5.47455477099994,11.6,9.19147833999999));
#214183=CARTESIAN_POINT('Ctrl Pts',(5.47520863999994,15.2,9.19378714299998));
#214184=CARTESIAN_POINT('Ctrl Pts',(5.47520863999994,11.6,9.19378714299998));
#214185=CARTESIAN_POINT('Ctrl Pts',(5.47586222099994,15.2,9.19610259599999));
#214186=CARTESIAN_POINT('Ctrl Pts',(5.47586222099994,11.6,9.19610259599999));
#214187=CARTESIAN_POINT('Ctrl Pts',(5.47651549999994,15.2,9.19842468799999));
#214188=CARTESIAN_POINT('Ctrl Pts',(5.47651549999994,11.6,9.19842468799999));
#214189=CARTESIAN_POINT('Ctrl Pts',(5.47716846599994,15.2,9.20075340999999));
#214190=CARTESIAN_POINT('Ctrl Pts',(5.47716846599994,11.6,9.20075340999999));
#214191=CARTESIAN_POINT('Ctrl Pts',(5.47782110499995,15.2,9.20308875299998));
#214192=CARTESIAN_POINT('Ctrl Pts',(5.47782110499995,11.6,9.20308875299998));
#214193=CARTESIAN_POINT('Ctrl Pts',(5.47847340599994,15.2,9.20543070799998));
#214194=CARTESIAN_POINT('Ctrl Pts',(5.47847340599994,11.6,9.20543070799998));
#214195=CARTESIAN_POINT('Ctrl Pts',(5.47912535699994,15.2,9.20777926499999));
#214196=CARTESIAN_POINT('Ctrl Pts',(5.47912535699994,11.6,9.20777926499999));
#214197=CARTESIAN_POINT('Ctrl Pts',(5.47977694299994,15.2,9.21013441399998));
#214198=CARTESIAN_POINT('Ctrl Pts',(5.47977694299994,11.6,9.21013441399998));
#214199=CARTESIAN_POINT('Ctrl Pts',(5.48042815199994,15.2,9.21249614799999));
#214200=CARTESIAN_POINT('Ctrl Pts',(5.48042815199994,11.6,9.21249614799999));
#214201=CARTESIAN_POINT('Ctrl Pts',(5.48107897199994,15.2,9.21486445499998));
#214202=CARTESIAN_POINT('Ctrl Pts',(5.48107897199994,11.6,9.21486445499998));
#214203=CARTESIAN_POINT('Ctrl Pts',(5.48172939199994,15.2,9.21723932699998));
#214204=CARTESIAN_POINT('Ctrl Pts',(5.48172939199994,11.6,9.21723932699998));
#214205=CARTESIAN_POINT('Ctrl Pts',(5.48237939899994,15.2,9.21962075499999));
#214206=CARTESIAN_POINT('Ctrl Pts',(5.48237939899994,11.6,9.21962075499999));
#214207=CARTESIAN_POINT('Ctrl Pts',(5.48302897899994,15.2,9.22200872899998));
#214208=CARTESIAN_POINT('Ctrl Pts',(5.48302897899994,11.6,9.22200872899998));
#214209=CARTESIAN_POINT('Ctrl Pts',(5.48367812199994,15.2,9.22440324099998));
#214210=CARTESIAN_POINT('Ctrl Pts',(5.48367812199994,11.6,9.22440324099998));
#214211=CARTESIAN_POINT('Ctrl Pts',(5.48432681499994,15.2,9.22680428099999));
#214212=CARTESIAN_POINT('Ctrl Pts',(5.48432681499994,11.6,9.22680428099999));
#214213=CARTESIAN_POINT('Ctrl Pts',(5.48497504599994,15.2,9.22921183899999));
#214214=CARTESIAN_POINT('Ctrl Pts',(5.48497504599994,11.6,9.22921183899999));
#214215=CARTESIAN_POINT('Ctrl Pts',(5.48562280099994,15.2,9.23162590799999));
#214216=CARTESIAN_POINT('Ctrl Pts',(5.48562280099994,11.6,9.23162590799999));
#214217=CARTESIAN_POINT('Ctrl Pts',(5.48627006999994,15.2,9.23404647599998));
#214218=CARTESIAN_POINT('Ctrl Pts',(5.48627006999994,11.6,9.23404647599998));
#214219=CARTESIAN_POINT('Ctrl Pts',(5.48691684099994,15.2,9.23647353599998));
#214220=CARTESIAN_POINT('Ctrl Pts',(5.48691684099994,11.6,9.23647353599998));
#214221=CARTESIAN_POINT('Ctrl Pts',(5.48756310199994,15.2,9.23890707899999));
#214222=CARTESIAN_POINT('Ctrl Pts',(5.48756310199994,11.6,9.23890707899999));
#214223=CARTESIAN_POINT('Ctrl Pts',(5.48820883899994,15.2,9.24134709399999));
#214224=CARTESIAN_POINT('Ctrl Pts',(5.48820883899994,11.6,9.24134709399999));
#214225=CARTESIAN_POINT('Ctrl Pts',(5.48885404099994,15.2,9.24379357399999));
#214226=CARTESIAN_POINT('Ctrl Pts',(5.48885404099994,11.6,9.24379357399999));
#214227=CARTESIAN_POINT('Ctrl Pts',(5.48949869799994,15.2,9.24624650799998));
#214228=CARTESIAN_POINT('Ctrl Pts',(5.48949869799994,11.6,9.24624650799998));
#214229=CARTESIAN_POINT('Ctrl Pts',(5.49014279599994,15.2,9.24870588899999));
#214230=CARTESIAN_POINT('Ctrl Pts',(5.49014279599994,11.6,9.24870588899999));
#214231=CARTESIAN_POINT('Ctrl Pts',(5.49078632299994,15.2,9.25117170699998));
#214232=CARTESIAN_POINT('Ctrl Pts',(5.49078632299994,11.6,9.25117170699998));
#214233=CARTESIAN_POINT('Ctrl Pts',(5.49142926899994,15.2,9.25364395199999));
#214234=CARTESIAN_POINT('Ctrl Pts',(5.49142926899994,11.6,9.25364395199999));
#214235=CARTESIAN_POINT('Ctrl Pts',(5.49207162099994,15.2,9.25612261599999));
#214236=CARTESIAN_POINT('Ctrl Pts',(5.49207162099994,11.6,9.25612261599999));
#214237=CARTESIAN_POINT('Ctrl Pts',(5.49271336799994,15.2,9.25860769099998));
#214238=CARTESIAN_POINT('Ctrl Pts',(5.49271336799994,11.6,9.25860769099998));
#214239=CARTESIAN_POINT('Ctrl Pts',(5.49335449699995,15.2,9.26109916599999));
#214240=CARTESIAN_POINT('Ctrl Pts',(5.49335449699995,11.6,9.26109916599999));
#214241=CARTESIAN_POINT('Ctrl Pts',(5.49399499799994,15.2,9.26359703299998));
#214242=CARTESIAN_POINT('Ctrl Pts',(5.49399499799994,11.6,9.26359703299998));
#214243=CARTESIAN_POINT('Ctrl Pts',(5.49463485899994,15.2,9.26610128399999));
#214244=CARTESIAN_POINT('Ctrl Pts',(5.49463485899994,11.6,9.26610128399999));
#214245=CARTESIAN_POINT('Ctrl Pts',(5.49527406699994,15.2,9.26861190799999));
#214246=CARTESIAN_POINT('Ctrl Pts',(5.49527406699994,11.6,9.26861190799999));
#214247=CARTESIAN_POINT('Ctrl Pts',(5.49591261199994,15.2,9.27112889799999));
#214248=CARTESIAN_POINT('Ctrl Pts',(5.49591261199994,11.6,9.27112889799999));
#214249=CARTESIAN_POINT('Ctrl Pts',(5.49655048199994,15.2,9.27365224499999));
#214250=CARTESIAN_POINT('Ctrl Pts',(5.49655048199994,11.6,9.27365224499999));
#214251=CARTESIAN_POINT('Ctrl Pts',(5.49718766599994,15.2,9.27618193799999));
#214252=CARTESIAN_POINT('Ctrl Pts',(5.49718766599994,11.6,9.27618193799999));
#214253=CARTESIAN_POINT('Ctrl Pts',(5.49782415299994,15.2,9.27871796999998));
#214254=CARTESIAN_POINT('Ctrl Pts',(5.49782415299994,11.6,9.27871796999998));
#214255=CARTESIAN_POINT('Ctrl Pts',(5.49845992999995,15.2,9.28126033199998));
#214256=CARTESIAN_POINT('Ctrl Pts',(5.49845992999995,11.6,9.28126033199998));
#214257=CARTESIAN_POINT('Ctrl Pts',(5.49909498699994,15.2,9.28380901499999));
#214258=CARTESIAN_POINT('Ctrl Pts',(5.49909498699994,11.6,9.28380901499999));
#214259=CARTESIAN_POINT('Ctrl Pts',(5.49972931199994,15.2,9.28636400999999));
#214260=CARTESIAN_POINT('Ctrl Pts',(5.49972931199994,11.6,9.28636400999999));
#214261=CARTESIAN_POINT('Ctrl Pts',(5.50036289399994,15.2,9.28892530799999));
#214262=CARTESIAN_POINT('Ctrl Pts',(5.50036289399994,11.6,9.28892530799999));
#214263=CARTESIAN_POINT('Ctrl Pts',(5.50099572099994,15.2,9.29149289999998));
#214264=CARTESIAN_POINT('Ctrl Pts',(5.50099572099994,11.6,9.29149289999998));
#214265=CARTESIAN_POINT('Ctrl Pts',(5.50162778299994,15.2,9.29406677899999));
#214266=CARTESIAN_POINT('Ctrl Pts',(5.50162778299994,11.6,9.29406677899999));
#214267=CARTESIAN_POINT('Ctrl Pts',(5.50225906899994,15.2,9.29664693499999));
#214268=CARTESIAN_POINT('Ctrl Pts',(5.50225906899994,11.6,9.29664693499999));
#214269=CARTESIAN_POINT('Ctrl Pts',(5.50288956699994,15.2,9.29923335799998));
#214270=CARTESIAN_POINT('Ctrl Pts',(5.50288956699994,11.6,9.29923335799998));
#214271=CARTESIAN_POINT('Ctrl Pts',(5.50351926699994,15.2,9.30182604099999));
#214272=CARTESIAN_POINT('Ctrl Pts',(5.50351926699994,11.6,9.30182604099999));
#214273=CARTESIAN_POINT('Ctrl Pts',(5.50414815599994,15.2,9.30442497499998));
#214274=CARTESIAN_POINT('Ctrl Pts',(5.50414815599994,11.6,9.30442497499998));
#214275=CARTESIAN_POINT('Ctrl Pts',(5.50477622399995,15.2,9.30703015099999));
#214276=CARTESIAN_POINT('Ctrl Pts',(5.50477622399995,11.6,9.30703015099999));
#214277=CARTESIAN_POINT('Ctrl Pts',(5.50540345999995,15.2,9.30964156099999));
#214278=CARTESIAN_POINT('Ctrl Pts',(5.50540345999995,11.6,9.30964156099999));
#214279=CARTESIAN_POINT('Ctrl Pts',(5.50602985399995,15.2,9.31225919499998));
#214280=CARTESIAN_POINT('Ctrl Pts',(5.50602985399995,11.6,9.31225919499998));
#214281=CARTESIAN_POINT('Ctrl Pts',(5.50665539399994,15.2,9.31488304499998));
#214282=CARTESIAN_POINT('Ctrl Pts',(5.50665539399994,11.6,9.31488304499998));
#214283=CARTESIAN_POINT('Ctrl Pts',(5.50728006899995,15.2,9.31751310199999));
#214284=CARTESIAN_POINT('Ctrl Pts',(5.50728006899995,11.6,9.31751310199999));
#214285=CARTESIAN_POINT('Ctrl Pts',(5.50790386899994,15.2,9.32014935899998));
#214286=CARTESIAN_POINT('Ctrl Pts',(5.50790386899994,11.6,9.32014935899998));
#214287=CARTESIAN_POINT('Ctrl Pts',(5.50852678199995,15.2,9.32279180499999));
#214288=CARTESIAN_POINT('Ctrl Pts',(5.50852678199995,11.6,9.32279180499999));
#214289=CARTESIAN_POINT('Ctrl Pts',(5.50914879799994,15.2,9.32544043399999));
#214290=CARTESIAN_POINT('Ctrl Pts',(5.50914879799994,11.6,9.32544043399999));
#214291=CARTESIAN_POINT('Ctrl Pts',(5.50976990699994,15.2,9.32809523399998));
#214292=CARTESIAN_POINT('Ctrl Pts',(5.50976990699994,11.6,9.32809523399998));
#214293=CARTESIAN_POINT('Ctrl Pts',(5.51039009699994,15.2,9.33075619999999));
#214294=CARTESIAN_POINT('Ctrl Pts',(5.51039009699994,11.6,9.33075619999999));
#214295=CARTESIAN_POINT('Ctrl Pts',(5.51100935799995,15.2,9.33342332199998));
#214296=CARTESIAN_POINT('Ctrl Pts',(5.51100935799995,11.6,9.33342332199998));
#214297=CARTESIAN_POINT('Ctrl Pts',(5.51162767899994,15.2,9.33609658999998));
#214298=CARTESIAN_POINT('Ctrl Pts',(5.51162767899994,11.6,9.33609658999998));
#214299=CARTESIAN_POINT('Ctrl Pts',(5.51224504999994,15.2,9.33877599699999));
#214300=CARTESIAN_POINT('Ctrl Pts',(5.51224504999994,11.6,9.33877599699999));
#214301=CARTESIAN_POINT('Ctrl Pts',(5.51286145799994,15.2,9.34146153499999));
#214302=CARTESIAN_POINT('Ctrl Pts',(5.51286145799994,11.6,9.34146153499999));
#214303=CARTESIAN_POINT('Ctrl Pts',(5.51347689599995,15.2,9.34415319399999));
#214304=CARTESIAN_POINT('Ctrl Pts',(5.51347689599995,11.6,9.34415319399999));
#214305=CARTESIAN_POINT('Ctrl Pts',(5.51409135199994,15.2,9.34685096699998));
#214306=CARTESIAN_POINT('Ctrl Pts',(5.51409135199994,11.6,9.34685096699998));
#214307=CARTESIAN_POINT('Ctrl Pts',(5.51470481499994,15.2,9.34955484399998));
#214308=CARTESIAN_POINT('Ctrl Pts',(5.51470481499994,11.6,9.34955484399998));
#214309=CARTESIAN_POINT('Ctrl Pts',(5.51531727499994,15.2,9.35226481699999));
#214310=CARTESIAN_POINT('Ctrl Pts',(5.51531727499994,11.6,9.35226481699999));
#214311=CARTESIAN_POINT('Ctrl Pts',(5.51592872199994,15.2,9.35498087899998));
#214312=CARTESIAN_POINT('Ctrl Pts',(5.51592872199994,11.6,9.35498087899998));
#214313=CARTESIAN_POINT('Ctrl Pts',(5.51653914399994,15.2,9.35770301999998));
#214314=CARTESIAN_POINT('Ctrl Pts',(5.51653914399994,11.6,9.35770301999998));
#214315=CARTESIAN_POINT('Ctrl Pts',(5.51714853299995,15.2,9.36043123099999));
#214316=CARTESIAN_POINT('Ctrl Pts',(5.51714853299995,11.6,9.36043123099999));
#214317=CARTESIAN_POINT('Ctrl Pts',(5.51775687699994,15.2,9.36316550599999));
#214318=CARTESIAN_POINT('Ctrl Pts',(5.51775687699994,11.6,9.36316550599999));
#214319=CARTESIAN_POINT('Ctrl Pts',(5.51836416599994,15.2,9.36590583399998));
#214320=CARTESIAN_POINT('Ctrl Pts',(5.51836416599994,11.6,9.36590583399998));
#214321=CARTESIAN_POINT('Ctrl Pts',(5.51897038999994,15.2,9.36865220899998));
#214322=CARTESIAN_POINT('Ctrl Pts',(5.51897038999994,11.6,9.36865220899998));
#214323=CARTESIAN_POINT('Ctrl Pts',(5.51957553899994,15.2,9.37140461999999));
#214324=CARTESIAN_POINT('Ctrl Pts',(5.51957553899994,11.6,9.37140461999999));
#214325=CARTESIAN_POINT('Ctrl Pts',(5.52017960199994,15.2,9.37416306199999));
#214326=CARTESIAN_POINT('Ctrl Pts',(5.52017960199994,11.6,9.37416306199999));
#214327=CARTESIAN_POINT('Ctrl Pts',(5.52078256999994,15.2,9.37692752199998));
#214328=CARTESIAN_POINT('Ctrl Pts',(5.52078256999994,11.6,9.37692752199998));
#214329=CARTESIAN_POINT('Ctrl Pts',(5.52138443099994,15.2,9.37969799599998));
#214330=CARTESIAN_POINT('Ctrl Pts',(5.52138443099994,11.6,9.37969799599998));
#214331=CARTESIAN_POINT('Ctrl Pts',(5.52198517699994,15.2,9.38247447399998));
#214332=CARTESIAN_POINT('Ctrl Pts',(5.52198517699994,11.6,9.38247447399998));
#214333=CARTESIAN_POINT('Ctrl Pts',(5.52258479599995,15.2,9.38525694799999));
#214334=CARTESIAN_POINT('Ctrl Pts',(5.52258479599995,11.6,9.38525694799999));
#214335=CARTESIAN_POINT('Ctrl Pts',(5.52318327999994,15.2,9.38804540799998));
#214336=CARTESIAN_POINT('Ctrl Pts',(5.52318327999994,11.6,9.38804540799998));
#214337=CARTESIAN_POINT('Ctrl Pts',(5.52378061699994,15.2,9.39083984899998));
#214338=CARTESIAN_POINT('Ctrl Pts',(5.52378061699994,11.6,9.39083984899998));
#214339=CARTESIAN_POINT('Ctrl Pts',(5.52437679899994,15.2,9.39364025899999));
#214340=CARTESIAN_POINT('Ctrl Pts',(5.52437679899994,11.6,9.39364025899999));
#214341=CARTESIAN_POINT('Ctrl Pts',(5.52497181399994,15.2,9.39644663299998));
#214342=CARTESIAN_POINT('Ctrl Pts',(5.52497181399994,11.6,9.39644663299998));
#214343=CARTESIAN_POINT('Ctrl Pts',(5.52556565399994,15.2,9.39925895999998));
#214344=CARTESIAN_POINT('Ctrl Pts',(5.52556565399994,11.6,9.39925895999998));
#214345=CARTESIAN_POINT('Ctrl Pts',(5.52615830699994,15.2,9.40207723399999));
#214346=CARTESIAN_POINT('Ctrl Pts',(5.52615830699994,11.6,9.40207723399999));
#214347=CARTESIAN_POINT('Ctrl Pts',(5.52674976499994,15.2,9.40490144499999));
#214348=CARTESIAN_POINT('Ctrl Pts',(5.52674976499994,11.6,9.40490144499999));
#214349=CARTESIAN_POINT('Ctrl Pts',(5.52734001699994,15.2,9.40773158699999));
#214350=CARTESIAN_POINT('Ctrl Pts',(5.52734001699994,11.6,9.40773158699999));
#214351=CARTESIAN_POINT('Ctrl Pts',(5.52792905399994,15.2,9.41056764999999));
#214352=CARTESIAN_POINT('Ctrl Pts',(5.52792905399994,11.6,9.41056764999999));
#214353=CARTESIAN_POINT('Ctrl Pts',(5.52851686599994,15.2,9.41340962499999));
#214354=CARTESIAN_POINT('Ctrl Pts',(5.52851686599994,11.6,9.41340962499999));
#214355=CARTESIAN_POINT('Ctrl Pts',(5.52910344299995,15.2,9.41625750699998));
#214356=CARTESIAN_POINT('Ctrl Pts',(5.52910344299995,11.6,9.41625750699998));
#214357=CARTESIAN_POINT('Ctrl Pts',(5.52968877499994,15.2,9.41911128399998));
#214358=CARTESIAN_POINT('Ctrl Pts',(5.52968877499994,11.6,9.41911128399998));
#214359=CARTESIAN_POINT('Ctrl Pts',(5.53027285299994,15.2,9.42197095099999));
#214360=CARTESIAN_POINT('Ctrl Pts',(5.53027285299994,11.6,9.42197095099999));
#214361=CARTESIAN_POINT('Ctrl Pts',(5.53085566699995,15.2,9.42483649799998));
#214362=CARTESIAN_POINT('Ctrl Pts',(5.53085566699995,11.6,9.42483649799998));
#214363=CARTESIAN_POINT('Ctrl Pts',(5.53143720799994,15.2,9.42770791799998));
#214364=CARTESIAN_POINT('Ctrl Pts',(5.53143720799994,11.6,9.42770791799998));
#214365=CARTESIAN_POINT('Ctrl Pts',(5.53201746599995,15.2,9.43058520199998));
#214366=CARTESIAN_POINT('Ctrl Pts',(5.53201746599995,11.6,9.43058520199998));
#214367=CARTESIAN_POINT('Ctrl Pts',(5.53259642999994,15.2,9.43346834199998));
#214368=CARTESIAN_POINT('Ctrl Pts',(5.53259642999994,11.6,9.43346834199998));
#214369=CARTESIAN_POINT('Ctrl Pts',(5.53317409299994,15.2,9.43635733099999));
#214370=CARTESIAN_POINT('Ctrl Pts',(5.53317409299994,11.6,9.43635733099999));
#214371=CARTESIAN_POINT('Ctrl Pts',(5.53375044299995,15.2,9.43925215999998));
#214372=CARTESIAN_POINT('Ctrl Pts',(5.53375044299995,11.6,9.43925215999998));
#214373=CARTESIAN_POINT('Ctrl Pts',(5.53432547199994,15.2,9.44215281999998));
#214374=CARTESIAN_POINT('Ctrl Pts',(5.53432547199994,11.6,9.44215281999998));
#214375=CARTESIAN_POINT('Ctrl Pts',(5.53489916999995,15.2,9.44505930399998));
#214376=CARTESIAN_POINT('Ctrl Pts',(5.53489916999995,11.6,9.44505930399998));
#214377=CARTESIAN_POINT('Ctrl Pts',(5.53547152799994,15.2,9.44797160399999));
#214378=CARTESIAN_POINT('Ctrl Pts',(5.53547152799994,11.6,9.44797160399999));
#214379=CARTESIAN_POINT('Ctrl Pts',(5.53604253599995,15.2,9.45088971299998));
#214380=CARTESIAN_POINT('Ctrl Pts',(5.53604253599995,11.6,9.45088971299998));
#214381=CARTESIAN_POINT('Ctrl Pts',(5.53661218599995,15.2,9.45381362099998));
#214382=CARTESIAN_POINT('Ctrl Pts',(5.53661218599995,11.6,9.45381362099998));
#214383=CARTESIAN_POINT('Ctrl Pts',(5.53718046699994,15.2,9.45674331999999));
#214384=CARTESIAN_POINT('Ctrl Pts',(5.53718046699994,11.6,9.45674331999999));
#214385=CARTESIAN_POINT('Ctrl Pts',(5.53774736999994,15.2,9.45967880399999));
#214386=CARTESIAN_POINT('Ctrl Pts',(5.53774736999994,11.6,9.45967880399999));
#214387=CARTESIAN_POINT('Ctrl Pts',(5.53831288599994,15.2,9.46262006299998));
#214388=CARTESIAN_POINT('Ctrl Pts',(5.53831288599994,11.6,9.46262006299998));
#214389=CARTESIAN_POINT('Ctrl Pts',(5.53887700599994,15.2,9.46556708999999));
#214390=CARTESIAN_POINT('Ctrl Pts',(5.53887700599994,11.6,9.46556708999999));
#214391=CARTESIAN_POINT('Ctrl Pts',(5.53943972199994,15.2,9.46851987699999));
#214392=CARTESIAN_POINT('Ctrl Pts',(5.53943972199994,11.6,9.46851987699999));
#214393=CARTESIAN_POINT('Ctrl Pts',(5.54000102099995,15.2,9.47147841499999));
#214394=CARTESIAN_POINT('Ctrl Pts',(5.54000102099995,11.6,9.47147841499999));
#214395=CARTESIAN_POINT('Ctrl Pts',(5.54056089699994,15.2,9.47444269799998));
#214396=CARTESIAN_POINT('Ctrl Pts',(5.54056089699994,11.6,9.47444269799998));
#214397=CARTESIAN_POINT('Ctrl Pts',(5.54111933899994,15.2,9.47741271699999));
#214398=CARTESIAN_POINT('Ctrl Pts',(5.54111933899994,11.6,9.47741271699999));
#214399=CARTESIAN_POINT('Ctrl Pts',(5.54167633999994,15.2,9.48038846399999));
#214400=CARTESIAN_POINT('Ctrl Pts',(5.54167633999994,11.6,9.48038846399999));
#214401=CARTESIAN_POINT('Ctrl Pts',(5.54223188899994,15.2,9.48336992999998));
#214402=CARTESIAN_POINT('Ctrl Pts',(5.54223188899994,11.6,9.48336992999998));
#214403=CARTESIAN_POINT('Ctrl Pts',(5.54278597899994,15.2,9.48635710899998));
#214404=CARTESIAN_POINT('Ctrl Pts',(5.54278597899994,11.6,9.48635710899998));
#214405=CARTESIAN_POINT('Ctrl Pts',(5.54333859799994,15.2,9.48934999299999));
#214406=CARTESIAN_POINT('Ctrl Pts',(5.54333859799994,11.6,9.48934999299999));
#214407=CARTESIAN_POINT('Ctrl Pts',(5.54388973899995,15.2,9.49234857099999));
#214408=CARTESIAN_POINT('Ctrl Pts',(5.54388973899995,11.6,9.49234857099999));
#214409=CARTESIAN_POINT('Ctrl Pts',(5.54443939299994,15.2,9.49535283999998));
#214410=CARTESIAN_POINT('Ctrl Pts',(5.54443939299994,11.6,9.49535283999998));
#214411=CARTESIAN_POINT('Ctrl Pts',(5.54498754999995,15.2,9.49836278799999));
#214412=CARTESIAN_POINT('Ctrl Pts',(5.54498754999995,11.6,9.49836278799999));
#214413=CARTESIAN_POINT('Ctrl Pts',(5.54553420099994,15.2,9.50137841099998));
#214414=CARTESIAN_POINT('Ctrl Pts',(5.54553420099994,11.6,9.50137841099998));
#214415=CARTESIAN_POINT('Ctrl Pts',(5.54607933799995,15.2,9.50439969699998));
#214416=CARTESIAN_POINT('Ctrl Pts',(5.54607933799995,11.6,9.50439969699998));
#214417=CARTESIAN_POINT('Ctrl Pts',(5.54662295099994,15.2,9.50742664099998));
#214418=CARTESIAN_POINT('Ctrl Pts',(5.54662295099994,11.6,9.50742664099998));
#214419=CARTESIAN_POINT('Ctrl Pts',(5.54716503399994,15.2,9.51045923399998));
#214420=CARTESIAN_POINT('Ctrl Pts',(5.54716503399994,11.6,9.51045923399998));
#214421=CARTESIAN_POINT('Ctrl Pts',(5.54770557399995,15.2,9.51349746899999));
#214422=CARTESIAN_POINT('Ctrl Pts',(5.54770557399995,11.6,9.51349746899999));
#214423=CARTESIAN_POINT('Ctrl Pts',(5.54824456499994,15.2,9.51654133699999));
#214424=CARTESIAN_POINT('Ctrl Pts',(5.54824456499994,11.6,9.51654133699999));
#214425=CARTESIAN_POINT('Ctrl Pts',(5.54878199699995,15.2,9.51959082999998));
#214426=CARTESIAN_POINT('Ctrl Pts',(5.54878199699995,11.6,9.51959082999998));
#214427=CARTESIAN_POINT('Ctrl Pts',(5.54931786199995,15.2,9.52264594299999));
#214428=CARTESIAN_POINT('Ctrl Pts',(5.54931786199995,11.6,9.52264594299999));
#214429=CARTESIAN_POINT('Ctrl Pts',(5.54985214999995,15.2,9.52570666499999));
#214430=CARTESIAN_POINT('Ctrl Pts',(5.54985214999995,11.6,9.52570666499999));
#214431=CARTESIAN_POINT('Ctrl Pts',(5.55038485399994,15.2,9.52877299099999));
#214432=CARTESIAN_POINT('Ctrl Pts',(5.55038485399994,11.6,9.52877299099999));
#214433=CARTESIAN_POINT('Ctrl Pts',(5.55091596399994,15.2,9.53184491099999));
#214434=CARTESIAN_POINT('Ctrl Pts',(5.55091596399994,11.6,9.53184491099999));
#214435=CARTESIAN_POINT('Ctrl Pts',(5.55144547199995,15.2,9.53492241799999));
#214436=CARTESIAN_POINT('Ctrl Pts',(5.55144547199995,11.6,9.53492241799999));
#214437=CARTESIAN_POINT('Ctrl Pts',(5.55197336999995,15.2,9.53800550399999));
#214438=CARTESIAN_POINT('Ctrl Pts',(5.55197336999995,11.6,9.53800550399999));
#214439=CARTESIAN_POINT('Ctrl Pts',(5.55249964699994,15.2,9.54109416199999));
#214440=CARTESIAN_POINT('Ctrl Pts',(5.55249964699994,11.6,9.54109416199999));
#214441=CARTESIAN_POINT('Ctrl Pts',(5.55302429599994,15.2,9.54418838299999));
#214442=CARTESIAN_POINT('Ctrl Pts',(5.55302429599994,11.6,9.54418838299999));
#214443=CARTESIAN_POINT('Ctrl Pts',(5.55354730899994,15.2,9.54728816199999));
#214444=CARTESIAN_POINT('Ctrl Pts',(5.55354730899994,11.6,9.54728816199999));
#214445=CARTESIAN_POINT('Ctrl Pts',(5.55406867599994,15.2,9.55039348799998));
#214446=CARTESIAN_POINT('Ctrl Pts',(5.55406867599994,11.6,9.55039348799998));
#214447=CARTESIAN_POINT('Ctrl Pts',(5.55458838999994,15.2,9.55350435599998));
#214448=CARTESIAN_POINT('Ctrl Pts',(5.55458838999994,11.6,9.55350435599998));
#214449=CARTESIAN_POINT('Ctrl Pts',(5.55510644099994,15.2,9.55662075599999));
#214450=CARTESIAN_POINT('Ctrl Pts',(5.55510644099994,11.6,9.55662075599999));
#214451=CARTESIAN_POINT('Ctrl Pts',(5.55562282199994,15.2,9.55974268199999));
#214452=CARTESIAN_POINT('Ctrl Pts',(5.55562282199994,11.6,9.55974268199999));
#214453=CARTESIAN_POINT('Ctrl Pts',(5.55613752299994,15.2,9.56287012499999));
#214454=CARTESIAN_POINT('Ctrl Pts',(5.55613752299994,11.6,9.56287012499999));
#214455=CARTESIAN_POINT('Ctrl Pts',(5.55665053699995,15.2,9.56600307999998));
#214456=CARTESIAN_POINT('Ctrl Pts',(5.55665053699995,11.6,9.56600307999998));
#214457=CARTESIAN_POINT('Ctrl Pts',(5.55716185399994,15.2,9.56914153499999));
#214458=CARTESIAN_POINT('Ctrl Pts',(5.55716185399994,11.6,9.56914153499999));
#214459=CARTESIAN_POINT('Ctrl Pts',(5.55767146699995,15.2,9.57228548699998));
#214460=CARTESIAN_POINT('Ctrl Pts',(5.55767146699995,11.6,9.57228548699998));
#214461=CARTESIAN_POINT('Ctrl Pts',(5.55817936699994,15.2,9.57543492499998));
#214462=CARTESIAN_POINT('Ctrl Pts',(5.55817936699994,11.6,9.57543492499998));
#214463=CARTESIAN_POINT('Ctrl Pts',(5.55868554599994,15.2,9.57858984399999));
#214464=CARTESIAN_POINT('Ctrl Pts',(5.55868554599994,11.6,9.57858984399999));
#214465=CARTESIAN_POINT('Ctrl Pts',(5.55918999599994,15.2,9.58175023399999));
#214466=CARTESIAN_POINT('Ctrl Pts',(5.55918999599994,11.6,9.58175023399999));
#214467=CARTESIAN_POINT('Ctrl Pts',(5.55969270799994,15.2,9.58491608999999));
#214468=CARTESIAN_POINT('Ctrl Pts',(5.55969270799994,11.6,9.58491608999999));
#214469=CARTESIAN_POINT('Ctrl Pts',(5.56019367299994,15.2,9.58808740099999));
#214470=CARTESIAN_POINT('Ctrl Pts',(5.56019367299994,11.6,9.58808740099999));
#214471=CARTESIAN_POINT('Ctrl Pts',(5.56069288399994,15.2,9.59126416199998));
#214472=CARTESIAN_POINT('Ctrl Pts',(5.56069288399994,11.6,9.59126416199998));
#214473=CARTESIAN_POINT('Ctrl Pts',(5.56119033299994,15.2,9.59444636499999));
#214474=CARTESIAN_POINT('Ctrl Pts',(5.56119033299994,11.6,9.59444636499999));
#214475=CARTESIAN_POINT('Ctrl Pts',(5.56168601199994,15.2,9.59763400199999));
#214476=CARTESIAN_POINT('Ctrl Pts',(5.56168601199994,11.6,9.59763400199999));
#214477=CARTESIAN_POINT('Ctrl Pts',(5.56217990999994,15.2,9.60082706499998));
#214478=CARTESIAN_POINT('Ctrl Pts',(5.56217990999994,11.6,9.60082706499998));
#214479=CARTESIAN_POINT('Ctrl Pts',(5.56267202299994,15.2,9.60402554799998));
#214480=CARTESIAN_POINT('Ctrl Pts',(5.56267202299994,11.6,9.60402554799998));
#214481=CARTESIAN_POINT('Ctrl Pts',(5.56316233999994,15.2,9.60722944199999));
#214482=CARTESIAN_POINT('Ctrl Pts',(5.56316233999994,11.6,9.60722944199999));
#214483=CARTESIAN_POINT('Ctrl Pts',(5.56365085299994,15.2,9.61043873999999));
#214484=CARTESIAN_POINT('Ctrl Pts',(5.56365085299994,11.6,9.61043873999999));
#214485=CARTESIAN_POINT('Ctrl Pts',(5.56413755499994,15.2,9.61365343599999));
#214486=CARTESIAN_POINT('Ctrl Pts',(5.56413755499994,11.6,9.61365343599999));
#214487=CARTESIAN_POINT('Ctrl Pts',(5.56462243899994,15.2,9.61687351999998));
#214488=CARTESIAN_POINT('Ctrl Pts',(5.56462243899994,11.6,9.61687351999998));
#214489=CARTESIAN_POINT('Ctrl Pts',(5.56510549399994,15.2,9.62009898599998));
#214490=CARTESIAN_POINT('Ctrl Pts',(5.56510549399994,11.6,9.62009898599998));
#214491=CARTESIAN_POINT('Ctrl Pts',(5.56558671399994,15.2,9.62332982499999));
#214492=CARTESIAN_POINT('Ctrl Pts',(5.56558671399994,11.6,9.62332982499999));
#214493=CARTESIAN_POINT('Ctrl Pts',(5.56606608999994,15.2,9.62656603199999));
#214494=CARTESIAN_POINT('Ctrl Pts',(5.56606608999994,11.6,9.62656603199999));
#214495=CARTESIAN_POINT('Ctrl Pts',(5.56654361499994,15.2,9.62980759699999));
#214496=CARTESIAN_POINT('Ctrl Pts',(5.56654361499994,11.6,9.62980759699999));
#214497=CARTESIAN_POINT('Ctrl Pts',(5.56701928099995,15.2,9.63305451399999));
#214498=CARTESIAN_POINT('Ctrl Pts',(5.56701928099995,11.6,9.63305451399999));
#214499=CARTESIAN_POINT('Ctrl Pts',(5.56749307999994,15.2,9.63630677599999));
#214500=CARTESIAN_POINT('Ctrl Pts',(5.56749307999994,11.6,9.63630677599999));
#214501=CARTESIAN_POINT('Ctrl Pts',(5.56796500199994,15.2,9.63956437499998));
#214502=CARTESIAN_POINT('Ctrl Pts',(5.56796500199994,11.6,9.63956437499998));
#214503=CARTESIAN_POINT('Ctrl Pts',(5.56843504199994,15.2,9.64282730199999));
#214504=CARTESIAN_POINT('Ctrl Pts',(5.56843504199994,11.6,9.64282730199999));
#214505=CARTESIAN_POINT('Ctrl Pts',(5.56890318999995,15.2,9.64609555199999));
#214506=CARTESIAN_POINT('Ctrl Pts',(5.56890318999995,11.6,9.64609555199999));
#214507=CARTESIAN_POINT('Ctrl Pts',(5.56936943999994,15.2,9.64936911699999));
#214508=CARTESIAN_POINT('Ctrl Pts',(5.56936943999994,11.6,9.64936911699999));
#214509=CARTESIAN_POINT('Ctrl Pts',(5.56983378399994,15.2,9.65264798799998));
#214510=CARTESIAN_POINT('Ctrl Pts',(5.56983378399994,11.6,9.65264798799998));
#214511=CARTESIAN_POINT('Ctrl Pts',(5.57029621199994,15.2,9.65593215999998));
#214512=CARTESIAN_POINT('Ctrl Pts',(5.57029621199994,11.6,9.65593215999998));
#214513=CARTESIAN_POINT('Ctrl Pts',(5.57075671899995,15.2,9.65922162299999));
#214514=CARTESIAN_POINT('Ctrl Pts',(5.57075671899995,11.6,9.65922162299999));
#214515=CARTESIAN_POINT('Ctrl Pts',(5.57121529499994,15.2,9.66251637199999));
#214516=CARTESIAN_POINT('Ctrl Pts',(5.57121529499994,11.6,9.66251637199999));
#214517=CARTESIAN_POINT('Ctrl Pts',(5.57167193299994,15.2,9.66581639899999));
#214518=CARTESIAN_POINT('Ctrl Pts',(5.57167193299994,11.6,9.66581639899999));
#214519=CARTESIAN_POINT('Ctrl Pts',(5.57212662699994,15.2,9.66912169499999));
#214520=CARTESIAN_POINT('Ctrl Pts',(5.57212662699994,11.6,9.66912169499999));
#214521=CARTESIAN_POINT('Ctrl Pts',(5.57257936599994,15.2,9.67243225399999));
#214522=CARTESIAN_POINT('Ctrl Pts',(5.57257936599994,11.6,9.67243225399999));
#214523=CARTESIAN_POINT('Ctrl Pts',(5.57303014599994,15.2,9.67574806999998));
#214524=CARTESIAN_POINT('Ctrl Pts',(5.57303014599994,11.6,9.67574806999998));
#214525=CARTESIAN_POINT('Ctrl Pts',(5.57347895599994,15.2,9.67906913199998));
#214526=CARTESIAN_POINT('Ctrl Pts',(5.57347895599994,11.6,9.67906913199998));
#214527=CARTESIAN_POINT('Ctrl Pts',(5.57392578999995,15.2,9.68239543699998));
#214528=CARTESIAN_POINT('Ctrl Pts',(5.57392578999995,11.6,9.68239543699998));
#214529=CARTESIAN_POINT('Ctrl Pts',(5.57437064099994,15.2,9.68572697499999));
#214530=CARTESIAN_POINT('Ctrl Pts',(5.57437064099994,11.6,9.68572697499999));
#214531=CARTESIAN_POINT('Ctrl Pts',(5.57481349999994,15.2,9.68906373899999));
#214532=CARTESIAN_POINT('Ctrl Pts',(5.57481349999994,11.6,9.68906373899999));
#214533=CARTESIAN_POINT('Ctrl Pts',(5.57525436099994,15.2,9.69240572199999));
#214534=CARTESIAN_POINT('Ctrl Pts',(5.57525436099994,11.6,9.69240572199999));
#214535=CARTESIAN_POINT('Ctrl Pts',(5.57569321399994,15.2,9.69575291799998));
#214536=CARTESIAN_POINT('Ctrl Pts',(5.57569321399994,11.6,9.69575291799998));
#214537=CARTESIAN_POINT('Ctrl Pts',(5.57613005399994,15.2,9.69910531599999));
#214538=CARTESIAN_POINT('Ctrl Pts',(5.57613005399994,11.6,9.69910531599999));
#214539=CARTESIAN_POINT('Ctrl Pts',(5.57656487299995,15.2,9.70246291299999));
#214540=CARTESIAN_POINT('Ctrl Pts',(5.57656487299995,11.6,9.70246291299999));
#214541=CARTESIAN_POINT('Ctrl Pts',(5.57699766199995,15.2,9.70582569899998));
#214542=CARTESIAN_POINT('Ctrl Pts',(5.57699766199995,11.6,9.70582569899998));
#214543=CARTESIAN_POINT('Ctrl Pts',(5.57742841599994,15.2,9.70919366799999));
#214544=CARTESIAN_POINT('Ctrl Pts',(5.57742841599994,11.6,9.70919366799999));
#214545=CARTESIAN_POINT('Ctrl Pts',(5.57785712399995,15.2,9.71256681299998));
#214546=CARTESIAN_POINT('Ctrl Pts',(5.57785712399995,11.6,9.71256681299998));
#214547=CARTESIAN_POINT('Ctrl Pts',(5.57828378199994,15.2,9.71594512399999));
#214548=CARTESIAN_POINT('Ctrl Pts',(5.57828378199994,11.6,9.71594512399999));
#214549=CARTESIAN_POINT('Ctrl Pts',(5.57870838199994,15.2,9.71932859799999));
#214550=CARTESIAN_POINT('Ctrl Pts',(5.57870838199994,11.6,9.71932859799999));
#214551=CARTESIAN_POINT('Ctrl Pts',(5.57913091399994,15.2,9.72271722499999));
#214552=CARTESIAN_POINT('Ctrl Pts',(5.57913091399994,11.6,9.72271722499999));
#214553=CARTESIAN_POINT('Ctrl Pts',(5.57955137399994,15.2,9.72611099799998));
#214554=CARTESIAN_POINT('Ctrl Pts',(5.57955137399994,11.6,9.72611099799998));
#214555=CARTESIAN_POINT('Ctrl Pts',(5.57996975299995,15.2,9.72950991099999));
#214556=CARTESIAN_POINT('Ctrl Pts',(5.57996975299995,11.6,9.72950991099999));
#214557=CARTESIAN_POINT('Ctrl Pts',(5.58038604299995,15.2,9.73291395399999));
#214558=CARTESIAN_POINT('Ctrl Pts',(5.58038604299995,11.6,9.73291395399999));
#214559=CARTESIAN_POINT('Ctrl Pts',(5.58080023799994,15.2,9.73632312399998));
#214560=CARTESIAN_POINT('Ctrl Pts',(5.58080023799994,11.6,9.73632312399998));
#214561=CARTESIAN_POINT('Ctrl Pts',(5.58121232999994,15.2,9.73973741099999));
#214562=CARTESIAN_POINT('Ctrl Pts',(5.58121232999994,11.6,9.73973741099999));
#214563=CARTESIAN_POINT('Ctrl Pts',(5.58162231199995,15.2,9.74315680799998));
#214564=CARTESIAN_POINT('Ctrl Pts',(5.58162231199995,11.6,9.74315680799998));
#214565=CARTESIAN_POINT('Ctrl Pts',(5.58203017699994,15.2,9.74658130799998));
#214566=CARTESIAN_POINT('Ctrl Pts',(5.58203017699994,11.6,9.74658130799998));
#214567=CARTESIAN_POINT('Ctrl Pts',(5.58243591799994,15.2,9.75001090499998));
#214568=CARTESIAN_POINT('Ctrl Pts',(5.58243591799994,11.6,9.75001090499998));
#214569=CARTESIAN_POINT('Ctrl Pts',(5.58283952599995,15.2,9.75344558999998));
#214570=CARTESIAN_POINT('Ctrl Pts',(5.58283952599995,11.6,9.75344558999998));
#214571=CARTESIAN_POINT('Ctrl Pts',(5.58324099499995,15.2,9.75688535799998));
#214572=CARTESIAN_POINT('Ctrl Pts',(5.58324099499995,11.6,9.75688535799998));
#214573=CARTESIAN_POINT('Ctrl Pts',(5.58364031899995,15.2,9.76033019899998));
#214574=CARTESIAN_POINT('Ctrl Pts',(5.58364031899995,11.6,9.76033019899998));
#214575=CARTESIAN_POINT('Ctrl Pts',(5.58403748899994,15.2,9.76378010799999));
#214576=CARTESIAN_POINT('Ctrl Pts',(5.58403748899994,11.6,9.76378010799999));
#214577=CARTESIAN_POINT('Ctrl Pts',(5.58443249899994,15.2,9.76723507899998));
#214578=CARTESIAN_POINT('Ctrl Pts',(5.58443249899994,11.6,9.76723507899998));
#214579=CARTESIAN_POINT('Ctrl Pts',(5.58482534199994,15.2,9.77069510199998));
#214580=CARTESIAN_POINT('Ctrl Pts',(5.58482534199994,11.6,9.77069510199998));
#214581=CARTESIAN_POINT('Ctrl Pts',(5.58521600899994,15.2,9.77416016999998));
#214582=CARTESIAN_POINT('Ctrl Pts',(5.58521600899994,11.6,9.77416016999998));
#214583=CARTESIAN_POINT('Ctrl Pts',(5.58560449599995,15.2,9.77763027899999));
#214584=CARTESIAN_POINT('Ctrl Pts',(5.58560449599995,11.6,9.77763027899999));
#214585=CARTESIAN_POINT('Ctrl Pts',(5.58599079299994,15.2,9.78110541899999));
#214586=CARTESIAN_POINT('Ctrl Pts',(5.58599079299994,11.6,9.78110541899999));
#214587=CARTESIAN_POINT('Ctrl Pts',(5.58637489499994,15.2,9.78458558299998));
#214588=CARTESIAN_POINT('Ctrl Pts',(5.58637489499994,11.6,9.78458558299998));
#214589=CARTESIAN_POINT('Ctrl Pts',(5.58675679299995,15.2,9.78807076599999));
#214590=CARTESIAN_POINT('Ctrl Pts',(5.58675679299995,11.6,9.78807076599999));
#214591=CARTESIAN_POINT('Ctrl Pts',(5.58713648299995,15.2,9.79156095899998));
#214592=CARTESIAN_POINT('Ctrl Pts',(5.58713648299995,11.6,9.79156095899998));
#214593=CARTESIAN_POINT('Ctrl Pts',(5.58751395599995,15.2,9.79505615499999));
#214594=CARTESIAN_POINT('Ctrl Pts',(5.58751395599995,11.6,9.79505615499999));
#214595=CARTESIAN_POINT('Ctrl Pts',(5.58788920299994,15.2,9.79855634899998));
#214596=CARTESIAN_POINT('Ctrl Pts',(5.58788920299994,11.6,9.79855634899998));
#214597=CARTESIAN_POINT('Ctrl Pts',(5.58826222199994,15.2,9.80206153099999));
#214598=CARTESIAN_POINT('Ctrl Pts',(5.58826222199994,11.6,9.80206153099999));
#214599=CARTESIAN_POINT('Ctrl Pts',(5.58863300199994,15.2,9.80557169599999));
#214600=CARTESIAN_POINT('Ctrl Pts',(5.58863300199994,11.6,9.80557169599999));
#214601=CARTESIAN_POINT('Ctrl Pts',(5.58900153799994,15.2,9.80908683699998));
#214602=CARTESIAN_POINT('Ctrl Pts',(5.58900153799994,11.6,9.80908683699998));
#214603=CARTESIAN_POINT('Ctrl Pts',(5.58936782299994,15.2,9.81260694599998));
#214604=CARTESIAN_POINT('Ctrl Pts',(5.58936782299994,11.6,9.81260694599998));
#214605=CARTESIAN_POINT('Ctrl Pts',(5.58973184799994,15.2,9.81613201599998));
#214606=CARTESIAN_POINT('Ctrl Pts',(5.58973184799994,11.6,9.81613201599998));
#214607=CARTESIAN_POINT('Ctrl Pts',(5.59009360999994,15.2,9.81966203999999));
#214608=CARTESIAN_POINT('Ctrl Pts',(5.59009360999994,11.6,9.81966203999999));
#214609=CARTESIAN_POINT('Ctrl Pts',(5.59045309799994,15.2,9.82319701299998));
#214610=CARTESIAN_POINT('Ctrl Pts',(5.59045309799994,11.6,9.82319701299998));
#214611=CARTESIAN_POINT('Ctrl Pts',(5.59081030799994,15.2,9.82673692399998));
#214612=CARTESIAN_POINT('Ctrl Pts',(5.59081030799994,11.6,9.82673692399998));
#214613=CARTESIAN_POINT('Ctrl Pts',(5.59116523299994,15.2,9.83028176999999));
#214614=CARTESIAN_POINT('Ctrl Pts',(5.59116523299994,11.6,9.83028176999999));
#214615=CARTESIAN_POINT('Ctrl Pts',(5.59151786499994,15.2,9.83383154199998));
#214616=CARTESIAN_POINT('Ctrl Pts',(5.59151786499994,11.6,9.83383154199998));
#214617=CARTESIAN_POINT('Ctrl Pts',(5.59186819799995,15.2,9.83738623299999));
#214618=CARTESIAN_POINT('Ctrl Pts',(5.59186819799995,11.6,9.83738623299999));
#214619=CARTESIAN_POINT('Ctrl Pts',(5.59221622499994,15.2,9.84094583599998));
#214620=CARTESIAN_POINT('Ctrl Pts',(5.59221622499994,11.6,9.84094583599998));
#214621=CARTESIAN_POINT('Ctrl Pts',(5.59256193999994,15.2,9.84451034399999));
#214622=CARTESIAN_POINT('Ctrl Pts',(5.59256193999994,11.6,9.84451034399999));
#214623=CARTESIAN_POINT('Ctrl Pts',(5.59290533499994,15.2,9.84807975199999));
#214624=CARTESIAN_POINT('Ctrl Pts',(5.59290533499994,11.6,9.84807975199999));
#214625=CARTESIAN_POINT('Ctrl Pts',(5.59324640499995,15.2,9.85165404999999));
#214626=CARTESIAN_POINT('Ctrl Pts',(5.59324640499995,11.6,9.85165404999999));
#214627=CARTESIAN_POINT('Ctrl Pts',(5.59358513999994,15.2,9.85523323299999));
#214628=CARTESIAN_POINT('Ctrl Pts',(5.59358513999994,11.6,9.85523323299999));
#214629=CARTESIAN_POINT('Ctrl Pts',(5.59392153799994,15.2,9.85881729399999));
#214630=CARTESIAN_POINT('Ctrl Pts',(5.59392153799994,11.6,9.85881729399999));
#214631=CARTESIAN_POINT('Ctrl Pts',(5.59425558899994,15.2,9.86240622499999));
#214632=CARTESIAN_POINT('Ctrl Pts',(5.59425558899994,11.6,9.86240622499999));
#214633=CARTESIAN_POINT('Ctrl Pts',(5.59458728699994,15.2,9.86600001999999));
#214634=CARTESIAN_POINT('Ctrl Pts',(5.59458728699994,11.6,9.86600001999999));
#214635=CARTESIAN_POINT('Ctrl Pts',(5.59491662599994,15.2,9.86959867199998));
#214636=CARTESIAN_POINT('Ctrl Pts',(5.59491662599994,11.6,9.86959867199998));
#214637=CARTESIAN_POINT('Ctrl Pts',(5.59524359999994,15.2,9.87320217299999));
#214638=CARTESIAN_POINT('Ctrl Pts',(5.59524359999994,11.6,9.87320217299999));
#214639=CARTESIAN_POINT('Ctrl Pts',(5.59556819999995,15.2,9.87681051799999));
#214640=CARTESIAN_POINT('Ctrl Pts',(5.59556819999995,11.6,9.87681051799999));
#214641=CARTESIAN_POINT('Ctrl Pts',(5.59589042199995,15.2,9.88042369799999));
#214642=CARTESIAN_POINT('Ctrl Pts',(5.59589042199995,11.6,9.88042369799999));
#214643=CARTESIAN_POINT('Ctrl Pts',(5.59621025999995,15.2,9.88404170799999));
#214644=CARTESIAN_POINT('Ctrl Pts',(5.59621025999995,11.6,9.88404170799999));
#214645=CARTESIAN_POINT('Ctrl Pts',(5.59652770299994,15.2,9.88766453999999));
#214646=CARTESIAN_POINT('Ctrl Pts',(5.59652770299994,11.6,9.88766453999999));
#214647=CARTESIAN_POINT('Ctrl Pts',(5.59684274999994,15.2,9.89129218699999));
#214648=CARTESIAN_POINT('Ctrl Pts',(5.59684274999994,11.6,9.89129218699999));
#214649=CARTESIAN_POINT('Ctrl Pts',(5.59715539099994,15.2,9.89492464299998));
#214650=CARTESIAN_POINT('Ctrl Pts',(5.59715539099994,11.6,9.89492464299998));
#214651=CARTESIAN_POINT('Ctrl Pts',(5.59746561999994,15.2,9.89856189999998));
#214652=CARTESIAN_POINT('Ctrl Pts',(5.59746561999994,11.6,9.89856189999998));
#214653=CARTESIAN_POINT('Ctrl Pts',(5.59777343199994,15.2,9.90220395299998));
#214654=CARTESIAN_POINT('Ctrl Pts',(5.59777343199994,11.6,9.90220395299998));
#214655=CARTESIAN_POINT('Ctrl Pts',(5.59807881899995,15.2,9.90585079299999));
#214656=CARTESIAN_POINT('Ctrl Pts',(5.59807881899995,11.6,9.90585079299999));
#214657=CARTESIAN_POINT('Ctrl Pts',(5.59838177599995,15.2,9.90950241499998));
#214658=CARTESIAN_POINT('Ctrl Pts',(5.59838177599995,11.6,9.90950241499998));
#214659=CARTESIAN_POINT('Ctrl Pts',(5.59868229399994,15.2,9.91315880999998));
#214660=CARTESIAN_POINT('Ctrl Pts',(5.59868229399994,11.6,9.91315880999998));
#214661=CARTESIAN_POINT('Ctrl Pts',(5.59898037099994,15.2,9.91681997299998));
#214662=CARTESIAN_POINT('Ctrl Pts',(5.59898037099994,11.6,9.91681997299998));
#214663=CARTESIAN_POINT('Ctrl Pts',(5.59927599599994,15.2,9.92048589699999));
#214664=CARTESIAN_POINT('Ctrl Pts',(5.59927599599994,11.6,9.92048589699999));
#214665=CARTESIAN_POINT('Ctrl Pts',(5.59956916499995,15.2,9.92415657399999));
#214666=CARTESIAN_POINT('Ctrl Pts',(5.59956916499995,11.6,9.92415657399999));
#214667=CARTESIAN_POINT('Ctrl Pts',(5.59985987199994,15.2,9.92783199799998));
#214668=CARTESIAN_POINT('Ctrl Pts',(5.59985987199994,11.6,9.92783199799998));
#214669=CARTESIAN_POINT('Ctrl Pts',(5.60014810899994,15.2,9.93151216299999));
#214670=CARTESIAN_POINT('Ctrl Pts',(5.60014810899994,11.6,9.93151216299999));
#214671=CARTESIAN_POINT('Ctrl Pts',(5.60043387199994,15.2,9.93519705999999));
#214672=CARTESIAN_POINT('Ctrl Pts',(5.60043387199994,11.6,9.93519705999999));
#214673=CARTESIAN_POINT('Ctrl Pts',(5.60071715199995,15.2,9.93888668399999));
#214674=CARTESIAN_POINT('Ctrl Pts',(5.60071715199995,11.6,9.93888668399999));
#214675=CARTESIAN_POINT('Ctrl Pts',(5.60099794499994,15.2,9.94258102799999));
#214676=CARTESIAN_POINT('Ctrl Pts',(5.60099794499994,11.6,9.94258102799999));
#214677=CARTESIAN_POINT('Ctrl Pts',(5.60127624499994,15.2,9.94628008399999));
#214678=CARTESIAN_POINT('Ctrl Pts',(5.60127624499994,11.6,9.94628008399999));
#214679=CARTESIAN_POINT('Ctrl Pts',(5.60155204299994,15.2,9.94998384799998));
#214680=CARTESIAN_POINT('Ctrl Pts',(5.60155204299994,11.6,9.94998384799998));
#214681=CARTESIAN_POINT('Ctrl Pts',(5.60182533599995,15.2,9.95369231099998));
#214682=CARTESIAN_POINT('Ctrl Pts',(5.60182533599995,11.6,9.95369231099998));
#214683=CARTESIAN_POINT('Ctrl Pts',(5.60209611699994,15.2,9.95740546799999));
#214684=CARTESIAN_POINT('Ctrl Pts',(5.60209611699994,11.6,9.95740546799999));
#214685=CARTESIAN_POINT('Ctrl Pts',(5.60236437799994,15.2,9.96112330999999));
#214686=CARTESIAN_POINT('Ctrl Pts',(5.60236437799994,11.6,9.96112330999999));
#214687=CARTESIAN_POINT('Ctrl Pts',(5.60263011399995,15.2,9.96484582999998));
#214688=CARTESIAN_POINT('Ctrl Pts',(5.60263011399995,11.6,9.96484582999998));
#214689=CARTESIAN_POINT('Ctrl Pts',(5.60289331799994,15.2,9.96857302299999));
#214690=CARTESIAN_POINT('Ctrl Pts',(5.60289331799994,11.6,9.96857302299999));
#214691=CARTESIAN_POINT('Ctrl Pts',(5.60315398399994,15.2,9.97230487999998));
#214692=CARTESIAN_POINT('Ctrl Pts',(5.60315398399994,11.6,9.97230487999998));
#214693=CARTESIAN_POINT('Ctrl Pts',(5.60341210499995,15.2,9.97604139599999));
#214694=CARTESIAN_POINT('Ctrl Pts',(5.60341210499995,11.6,9.97604139599999));
#214695=CARTESIAN_POINT('Ctrl Pts',(5.60366767599994,15.2,9.97978256399998));
#214696=CARTESIAN_POINT('Ctrl Pts',(5.60366767599994,11.6,9.97978256399998));
#214697=CARTESIAN_POINT('Ctrl Pts',(5.60392069199994,15.2,9.98352837599998));
#214698=CARTESIAN_POINT('Ctrl Pts',(5.60392069199994,11.6,9.98352837599998));
#214699=CARTESIAN_POINT('Ctrl Pts',(5.60417114799994,15.2,9.98727882899999));
#214700=CARTESIAN_POINT('Ctrl Pts',(5.60417114799994,11.6,9.98727882899999));
#214701=CARTESIAN_POINT('Ctrl Pts',(5.60441903599994,15.2,9.99103391699999));
#214702=CARTESIAN_POINT('Ctrl Pts',(5.60441903599994,11.6,9.99103391699999));
#214703=CARTESIAN_POINT('Ctrl Pts',(5.60466435299994,15.2,9.99479363099999));
#214704=CARTESIAN_POINT('Ctrl Pts',(5.60466435299994,11.6,9.99479363099999));
#214705=CARTESIAN_POINT('Ctrl Pts',(5.60490709099994,15.2,9.99855796499999));
#214706=CARTESIAN_POINT('Ctrl Pts',(5.60490709099994,11.6,9.99855796499999));
#214707=CARTESIAN_POINT('Ctrl Pts',(5.60514724499994,15.2,10.002326911));
#214708=CARTESIAN_POINT('Ctrl Pts',(5.60514724499994,11.6,10.002326911));
#214709=CARTESIAN_POINT('Ctrl Pts',(5.60538480399994,15.2,10.006100462));
#214710=CARTESIAN_POINT('Ctrl Pts',(5.60538480399994,11.6,10.006100462));
#214711=CARTESIAN_POINT('Ctrl Pts',(5.60561976299994,15.2,10.009878609));
#214712=CARTESIAN_POINT('Ctrl Pts',(5.60561976299994,11.6,10.009878609));
#214713=CARTESIAN_POINT('Ctrl Pts',(5.60585211499995,15.2,10.013661345));
#214714=CARTESIAN_POINT('Ctrl Pts',(5.60585211499995,11.6,10.013661345));
#214715=CARTESIAN_POINT('Ctrl Pts',(5.60608185199994,15.2,10.01744866));
#214716=CARTESIAN_POINT('Ctrl Pts',(5.60608185199994,11.6,10.01744866));
#214717=CARTESIAN_POINT('Ctrl Pts',(5.60630896899994,15.2,10.021240551));
#214718=CARTESIAN_POINT('Ctrl Pts',(5.60630896899994,11.6,10.021240551));
#214719=CARTESIAN_POINT('Ctrl Pts',(5.60653346399994,15.2,10.025037011));
#214720=CARTESIAN_POINT('Ctrl Pts',(5.60653346399994,11.6,10.025037011));
#214721=CARTESIAN_POINT('Ctrl Pts',(5.60675533299994,15.2,10.028838039));
#214722=CARTESIAN_POINT('Ctrl Pts',(5.60675533299994,11.6,10.028838039));
#214723=CARTESIAN_POINT('Ctrl Pts',(5.60697457299995,15.2,10.032643632));
#214724=CARTESIAN_POINT('Ctrl Pts',(5.60697457299995,11.6,10.032643632));
#214725=CARTESIAN_POINT('Ctrl Pts',(5.60714786199994,15.2,10.035691756));
#214726=CARTESIAN_POINT('Ctrl Pts',(5.60714786199994,11.6,10.035691756));
#214727=CARTESIAN_POINT('Ctrl Pts',(5.60727664699994,15.2,10.037979905));
#214728=CARTESIAN_POINT('Ctrl Pts',(5.60727664699994,11.6,10.037979905));
#214729=CARTESIAN_POINT('Ctrl Pts',(5.60736197799995,15.2,10.039506249));
#214730=CARTESIAN_POINT('Ctrl Pts',(5.60736197799995,11.6,10.039506249));
#214731=CARTESIAN_POINT('Ctrl Pts',(5.60740451299995,15.2,10.04026965));
#214732=CARTESIAN_POINT('Ctrl Pts',(5.60740451299995,11.6,10.04026965));
#214733=CARTESIAN_POINT('Ctrl Pts',(5.36127880499994,15.2,8.88241603299999));
#214734=CARTESIAN_POINT('Ctrl Pts',(5.36206719568413,15.2,8.88401933383977));
#214735=CARTESIAN_POINT('Ctrl Pts',(5.3628759863957,15.2,8.88567631031983));
#214736=CARTESIAN_POINT('Ctrl Pts',(5.36370417391754,15.2,8.88738636482928));
#214737=CARTESIAN_POINT('Ctrl Pts',(5.36453635537823,15.2,8.88910466608596));
#214738=CARTESIAN_POINT('Ctrl Pts',(5.36538812011717,15.2,8.89087656335787));
#214739=CARTESIAN_POINT('Ctrl Pts',(5.36625847962582,15.2,8.89270147796823));
#214740=CARTESIAN_POINT('Ctrl Pts',(5.36712883905543,15.2,8.89452639241284));
#214741=CARTESIAN_POINT('Ctrl Pts',(5.36801779174953,15.2,8.89640432539507));
#214742=CARTESIAN_POINT('Ctrl Pts',(5.36892438021658,15.2,8.89833471374155));
#214743=CARTESIAN_POINT('Ctrl Pts',(5.36983096868362,15.2,8.90026510208804));
#214744=CARTESIAN_POINT('Ctrl Pts',(5.37075519224708,15.2,8.90224794602847));
#214745=CARTESIAN_POINT('Ctrl Pts',(5.3716961199256,15.2,8.90428269455318));
#214746=CARTESIAN_POINT('Ctrl Pts',(5.37263704768957,15.2,8.90631744326271));
#214747=CARTESIAN_POINT('Ctrl Pts',(5.37359468033524,15.2,8.9084040964046));
#214748=CARTESIAN_POINT('Ctrl Pts',(5.37456811338936,15.2,8.91054211894128));
#214749=CARTESIAN_POINT('Ctrl Pts',(5.37570378515322,15.2,8.91303647827611));
#214750=CARTESIAN_POINT('Ctrl Pts',(5.37686096291785,15.2,8.91560075447309));
#214751=CARTESIAN_POINT('Ctrl Pts',(5.37803825790234,15.2,8.91823411554835));
#214752=CARTESIAN_POINT('Ctrl Pts',(5.3790473680069,15.2,8.92049128244788));
#214753=CARTESIAN_POINT('Ctrl Pts',(5.38007125793053,15.2,8.92279920619165));
#214754=CARTESIAN_POINT('Ctrl Pts',(5.38110908007138,15.2,8.92515737499027));
#214755=CARTESIAN_POINT('Ctrl Pts',(5.38214690211796,15.2,8.92751554357471));
#214756=CARTESIAN_POINT('Ctrl Pts',(5.38319865533424,15.2,8.92992395694573));
#214757=CARTESIAN_POINT('Ctrl Pts',(5.38426351746707,15.2,8.93238211453435));
#214758=CARTESIAN_POINT('Ctrl Pts',(5.3853283795999,15.2,8.93484027212297));
#214759=CARTESIAN_POINT('Ctrl Pts',(5.3864063481307,15.2,8.93734817377245));
#214760=CARTESIAN_POINT('Ctrl Pts',(5.38749662325722,15.2,8.93990532934408));
#214761=CARTESIAN_POINT('Ctrl Pts',(5.38858689848278,15.2,8.94246248514798));
#214762=CARTESIAN_POINT('Ctrl Pts',(5.38968947790153,15.2,8.94506889477464));
#214763=CARTESIAN_POINT('Ctrl Pts',(5.39080358337969,15.2,8.94772407675599));
#214764=CARTESIAN_POINT('Ctrl Pts',(5.39191768875667,15.2,8.95037925849614));
#214765=CARTESIAN_POINT('Ctrl Pts',(5.39304331814439,15.2,8.95308321474799));
#214766=CARTESIAN_POINT('Ctrl Pts',(5.39417971535357,15.2,8.95583547065011));
#214767=CARTESIAN_POINT('Ctrl Pts',(5.39531611256277,15.2,8.95858772655223));
#214768=CARTESIAN_POINT('Ctrl Pts',(5.39646327322106,15.2,8.96138828550877));
#214769=CARTESIAN_POINT('Ctrl Pts',(5.39762045992857,15.2,8.96423668331986));
#214770=CARTESIAN_POINT('Ctrl Pts',(5.39877764663609,15.2,8.96708508113096));
#214771=CARTESIAN_POINT('Ctrl Pts',(5.39994486175675,15.2,8.96998131745591));
#214772=CARTESIAN_POINT('Ctrl Pts',(5.40112137963002,15.2,8.97292494117904));
#214773=CARTESIAN_POINT('Ctrl Pts',(5.40229789761017,15.2,8.97586856516956));
#214774=CARTESIAN_POINT('Ctrl Pts',(5.40348372275793,15.2,8.97885957314806));
#214775=CARTESIAN_POINT('Ctrl Pts',(5.40467814957339,15.2,8.981897523149));
#214776=CARTESIAN_POINT('Ctrl Pts',(5.40587257628037,15.2,8.98493547287399));
#214777=CARTESIAN_POINT('Ctrl Pts',(5.40707560536163,15.2,8.98802036289524));
#214778=CARTESIAN_POINT('Ctrl Pts',(5.40828655315064,15.2,8.99115175477944));
#214779=CARTESIAN_POINT('Ctrl Pts',(5.40949750093962,15.2,8.99428314666365));
#214780=CARTESIAN_POINT('Ctrl Pts',(5.41071636676135,15.2,8.99746104326049));
#214781=CARTESIAN_POINT('Ctrl Pts',(5.41194248188295,15.2,9.00068501039017));
#214782=CARTESIAN_POINT('Ctrl Pts',(5.41316859711593,15.2,9.00390897781269));
#214783=CARTESIAN_POINT('Ctrl Pts',(5.41440196414134,15.2,9.00717902039809));
#214784=CARTESIAN_POINT('Ctrl Pts',(5.41564192829254,15.2,9.01049471074747));
#214785=CARTESIAN_POINT('Ctrl Pts',(5.41688189233111,15.2,9.01381040079567));
#214786=CARTESIAN_POINT('Ctrl Pts',(5.41812845637254,15.2,9.01717174290682));
#214787=CARTESIAN_POINT('Ctrl Pts',(5.41938098149937,15.2,9.02057831696503));
#214788=CARTESIAN_POINT('Ctrl Pts',(5.42063350662618,15.2,9.02398489102326));
#214789=CARTESIAN_POINT('Ctrl Pts',(5.42189199455013,15.2,9.02743670033225));
#214790=CARTESIAN_POINT('Ctrl Pts',(5.42315582458718,15.2,9.03093333336878));
#214791=CARTESIAN_POINT('Ctrl Pts',(5.42441965473902,15.2,9.03442996672293));
#214792=CARTESIAN_POINT('Ctrl Pts',(5.42568882599815,15.2,9.03797142575305));
#214793=CARTESIAN_POINT('Ctrl Pts',(5.42696273238152,15.2,9.04155730713024));
#214794=CARTESIAN_POINT('Ctrl Pts',(5.42823663864917,15.2,9.04514318818172));
#214795=CARTESIAN_POINT('Ctrl Pts',(5.42951527992154,15.2,9.04877349106673));
#214796=CARTESIAN_POINT('Ctrl Pts',(5.43079806495827,15.2,9.05244781826656));
#214797=CARTESIAN_POINT('Ctrl Pts',(5.432080849995,15.2,9.0561221454664));
#214798=CARTESIAN_POINT('Ctrl Pts',(5.43336777664106,15.2,9.05984049843734));
#214799=CARTESIAN_POINT('Ctrl Pts',(5.43465826715844,15.2,9.06360248665276));
#214800=CARTESIAN_POINT('Ctrl Pts',(5.435733675962,15.2,9.06673747694619));
#214801=CARTESIAN_POINT('Ctrl Pts',(5.43681156121276,15.2,9.06990276903155));
#214802=CARTESIAN_POINT('Ctrl Pts',(5.43789159246265,15.2,9.07309813930779));
#214803=CARTESIAN_POINT('Ctrl Pts',(5.43897162371255,15.2,9.07629350958402));
#214804=CARTESIAN_POINT('Ctrl Pts',(5.44005380160138,15.2,9.0795189574332));
#214805=CARTESIAN_POINT('Ctrl Pts',(5.44113780521239,15.2,9.08277426507052));
#214806=CARTESIAN_POINT('Ctrl Pts',(5.44222180882341,15.2,9.08602957270784));
#214807=CARTESIAN_POINT('Ctrl Pts',(5.44330763673329,15.2,9.08931473918868));
#214808=CARTESIAN_POINT('Ctrl Pts',(5.44439497451602,15.2,9.09262954448144));
#214809=CARTESIAN_POINT('Ctrl Pts',(5.44548231229874,15.2,9.09594434977421));
#214810=CARTESIAN_POINT('Ctrl Pts',(5.44657115834994,15.2,9.09928879568325));
#214811=CARTESIAN_POINT('Ctrl Pts',(5.44766120376661,15.2,9.10266266672491));
#214812=CARTESIAN_POINT('Ctrl Pts',(5.44896925821909,15.2,9.1067113118278));
#214813=CARTESIAN_POINT('Ctrl Pts',(5.45027903671366,15.2,9.11080232867963));
#214814=CARTESIAN_POINT('Ctrl Pts',(5.45159001631479,15.2,9.11493534906686));
#214815=CARTESIAN_POINT('Ctrl Pts',(5.45268249935543,15.2,9.11837953284803));
#214816=CARTESIAN_POINT('Ctrl Pts',(5.45377581650622,15.2,9.12185288672812));
#214817=CARTESIAN_POINT('Ctrl Pts',(5.45486966872841,15.2,9.12535519950437));
#214818=CARTESIAN_POINT('Ctrl Pts',(5.45618229146657,15.2,9.12955797506492));
#214819=CARTESIAN_POINT('Ctrl Pts',(5.45749568456319,15.2,9.1338024511057));
#214820=CARTESIAN_POINT('Ctrl Pts',(5.4588093433848,15.2,9.13808827142541));
#214821=CARTESIAN_POINT('Ctrl Pts',(5.45990405889049,15.2,9.14165978777456));
#214822=CARTESIAN_POINT('Ctrl Pts',(5.46099895984273,15.2,9.14526001305091));
#214823=CARTESIAN_POINT('Ctrl Pts',(5.46209375784841,15.2,9.14888874300029));
#214824=CARTESIAN_POINT('Ctrl Pts',(5.46318855597342,15.2,9.1525174733452));
#214825=CARTESIAN_POINT('Ctrl Pts',(5.46428325185122,15.2,9.15617470902571));
#214826=CARTESIAN_POINT('Ctrl Pts',(5.46537756407347,15.2,9.15986024596785));
#214827=CARTESIAN_POINT('Ctrl Pts',(5.46647187629573,15.2,9.16354578290998));
#214828=CARTESIAN_POINT('Ctrl Pts',(5.46756580386281,15.2,9.16725962078066));
#214829=CARTESIAN_POINT('Ctrl Pts',(5.4686590711397,15.2,9.17100156034063));
#214830=CARTESIAN_POINT('Ctrl Pts',(5.46975233841657,15.2,9.1747434999006));
#214831=CARTESIAN_POINT('Ctrl Pts',(5.47084494464517,15.2,9.17851353832538));
#214832=CARTESIAN_POINT('Ctrl Pts',(5.47193661714521,15.2,9.1823114779767));
#214833=CARTESIAN_POINT('Ctrl Pts',(5.47302828964526,15.2,9.18610941762802));
#214834=CARTESIAN_POINT('Ctrl Pts',(5.4741190282064,15.2,9.18993525979951));
#214835=CARTESIAN_POINT('Ctrl Pts',(5.47520856792868,15.2,9.19378880521472));
#214836=CARTESIAN_POINT('Ctrl Pts',(5.47629810765096,15.2,9.19764235062994));
#214837=CARTESIAN_POINT('Ctrl Pts',(5.4773864436121,15.2,9.20152359963474));
#214838=CARTESIAN_POINT('Ctrl Pts',(5.47847331840386,15.2,9.20543235824444));
#214839=CARTESIAN_POINT('Ctrl Pts',(5.47956019319562,15.2,9.20934111685415));
#214840=CARTESIAN_POINT('Ctrl Pts',(5.48064560144443,15.2,9.21327738395761));
#214841=CARTESIAN_POINT('Ctrl Pts',(5.48172928874102,15.2,9.21724096598943));
#214842=CARTESIAN_POINT('Ctrl Pts',(5.4830297134497,15.2,9.2219972642548));
#214843=CARTESIAN_POINT('Ctrl Pts',(5.48432765722231,15.2,9.2267928970263));
#214844=CARTESIAN_POINT('Ctrl Pts',(5.48562267934213,15.2,9.23162753226462));
#214845=CARTESIAN_POINT('Ctrl Pts',(5.48648602750041,15.2,9.23485062271627));
#214846=CARTESIAN_POINT('Ctrl Pts',(5.48734808037473,15.2,9.23809104769311));
#214847=CARTESIAN_POINT('Ctrl Pts',(5.48820870525887,15.2,9.24134871021882));
#214848=CARTESIAN_POINT('Ctrl Pts',(5.48906933002574,15.2,9.24460637230066));
#214849=CARTESIAN_POINT('Ctrl Pts',(5.48992853026579,15.2,9.24788127249925));
#214850=CARTESIAN_POINT('Ctrl Pts',(5.49078617758473,15.2,9.25117331322835));
#214851=CARTESIAN_POINT('Ctrl Pts',(5.49164382502051,15.2,9.25446535440598));
#214852=CARTESIAN_POINT('Ctrl Pts',(5.49249992115894,15.2,9.25777453670752));
#214853=CARTESIAN_POINT('Ctrl Pts',(5.49335433998329,15.2,9.26110076399991));
#214854=CARTESIAN_POINT('Ctrl Pts',(5.49420875880763,15.2,9.2644269912923));
#214855=CARTESIAN_POINT('Ctrl Pts',(5.49506150129567,15.2,9.26777026404226));
#214856=CARTESIAN_POINT('Ctrl Pts',(5.49591244339741,15.2,9.27113048778265));
#214857=CARTESIAN_POINT('Ctrl Pts',(5.49676338538321,15.2,9.27449071106523));
#214858=CARTESIAN_POINT('Ctrl Pts',(5.49761252860366,15.2,9.27786788350966));
#214859=CARTESIAN_POINT('Ctrl Pts',(5.49845974998271,15.2,9.28126191224761));
#214860=CARTESIAN_POINT('Ctrl Pts',(5.49930697147719,15.2,9.28465594144798));
#214861=CARTESIAN_POINT('Ctrl Pts',(5.50015227166707,15.2,9.28806682570794));
#214862=CARTESIAN_POINT('Ctrl Pts',(5.50099552987949,15.2,9.29149447228535));
#214863=CARTESIAN_POINT('Ctrl Pts',(5.50183878797701,15.2,9.29492211839574));
#214864=CARTESIAN_POINT('Ctrl Pts',(5.50268000621923,15.2,9.29836652675115));
#214865=CARTESIAN_POINT('Ctrl Pts',(5.50351906420634,15.2,9.30182760346714));
#214866=CARTESIAN_POINT('Ctrl Pts',(5.50477765124416,15.2,9.30701921877689));
#214867=CARTESIAN_POINT('Ctrl Pts',(5.50603137697554,15.2,9.31224833908646));
#214868=CARTESIAN_POINT('Ctrl Pts',(5.5072798500972,15.2,9.31751465139257));
#214869=CARTESIAN_POINT('Ctrl Pts',(5.50811216558724,15.2,9.32102552658221));
#214870=CARTESIAN_POINT('Ctrl Pts',(5.50894214577708,15.2,9.32455293209843));
#214871=CARTESIAN_POINT('Ctrl Pts',(5.50976967726663,15.2,9.32809677545826));
#214872=CARTESIAN_POINT('Ctrl Pts',(5.51059720875617,15.2,9.33164061881809));
#214873=CARTESIAN_POINT('Ctrl Pts',(5.51142229116766,15.2,9.33520090112145));
#214874=CARTESIAN_POINT('Ctrl Pts',(5.51224480943444,15.2,9.33877753031806));
#214875=CARTESIAN_POINT('Ctrl Pts',(5.51306732758916,15.2,9.34235415902734));
#214876=CARTESIAN_POINT('Ctrl Pts',(5.51388728342361,15.2,9.34594713578453));
#214877=CARTESIAN_POINT('Ctrl Pts',(5.5147045642494,15.2,9.3495563680058));
#214878=CARTESIAN_POINT('Ctrl Pts',(5.51552184518655,15.2,9.35316560071883));
#214879=CARTESIAN_POINT('Ctrl Pts',(5.51633645107762,15.2,9.35679109096465));
#214880=CARTESIAN_POINT('Ctrl Pts',(5.51714827189936,15.2,9.36043274755369));
#214881=CARTESIAN_POINT('Ctrl Pts',(5.51796009261048,15.2,9.36407440364655));
#214882=CARTESIAN_POINT('Ctrl Pts',(5.51876912729418,15.2,9.36773222668446));
#214883=CARTESIAN_POINT('Ctrl Pts',(5.51957526745069,15.2,9.37140612738306));
#214884=CARTESIAN_POINT('Ctrl Pts',(5.52038140771703,15.2,9.37508002858223));
#214885=CARTESIAN_POINT('Ctrl Pts',(5.52118465309384,15.2,9.3787700061326));
#214886=CARTESIAN_POINT('Ctrl Pts',(5.52198489539939,15.2,9.38247597352111));
#214887=CARTESIAN_POINT('Ctrl Pts',(5.52278513759591,15.2,9.38618194040468));
#214888=CARTESIAN_POINT('Ctrl Pts',(5.52358237706084,15.2,9.38990389484001));
#214889=CARTESIAN_POINT('Ctrl Pts',(5.52437650721834,15.2,9.39364174964451));
#214890=CARTESIAN_POINT('Ctrl Pts',(5.52517063748404,15.2,9.39737960495828));
#214891=CARTESIAN_POINT('Ctrl Pts',(5.52596165798271,15.2,9.40113336004064));
#214892=CARTESIAN_POINT('Ctrl Pts',(5.526749463581,15.2,9.4049029280249));
#214893=CARTESIAN_POINT('Ctrl Pts',(5.52753726907194,15.2,9.40867249549554));
#214894=CARTESIAN_POINT('Ctrl Pts',(5.52832186005834,15.2,9.41245787532344));
#214895=CARTESIAN_POINT('Ctrl Pts',(5.5291031316449,15.2,9.41625898025678));
#214896=CARTESIAN_POINT('Ctrl Pts',(5.52988440333791,15.2,9.42006008570802));
#214897=CARTESIAN_POINT('Ctrl Pts',(5.53066235576293,15.2,9.42387691572295));
#214898=CARTESIAN_POINT('Ctrl Pts',(5.53143688730491,15.2,9.42770938432171));
#214899=CARTESIAN_POINT('Ctrl Pts',(5.53221141874136,15.2,9.4315418523983));
#214900=CARTESIAN_POINT('Ctrl Pts',(5.53298252767017,15.2,9.43538995900788));
#214901=CARTESIAN_POINT('Ctrl Pts',(5.53375011260779,15.2,9.43925361713489));
#214902=CARTESIAN_POINT('Ctrl Pts',(5.53451769764998,15.2,9.44311727578831));
#214903=CARTESIAN_POINT('Ctrl Pts',(5.53528175881948,15.2,9.44699648553922));
#214904=CARTESIAN_POINT('Ctrl Pts',(5.53604219647548,15.2,9.45089116276925));
#214905=CARTESIAN_POINT('Ctrl Pts',(5.53737296232167,15.2,9.45770684765646));
#214906=CARTESIAN_POINT('Ctrl Pts',(5.5386926294636,15.2,9.46456989538522));
#214907=CARTESIAN_POINT('Ctrl Pts',(5.5400006653305,15.2,9.47147985187053));
#214908=CARTESIAN_POINT('Ctrl Pts',(5.54112183887252,15.2,9.47740267140767));
#214909=CARTESIAN_POINT('Ctrl Pts',(5.54223446985674,15.2,9.48335995595096));
#214910=CARTESIAN_POINT('Ctrl Pts',(5.5433382284833,15.2,9.48935141656659));
#214911=CARTESIAN_POINT('Ctrl Pts',(5.54407406763451,15.2,9.49334572400649));
#214912=CARTESIAN_POINT('Ctrl Pts',(5.54480596489638,15.2,9.49735522218987));
#214913=CARTESIAN_POINT('Ctrl Pts',(5.5455338226023,15.2,9.50137982746629));
#214914=CARTESIAN_POINT('Ctrl Pts',(5.54626168020904,15.2,9.50540443219436));
#214915=CARTESIAN_POINT('Ctrl Pts',(5.54698550032724,15.2,9.50944414317971));
#214916=CARTESIAN_POINT('Ctrl Pts',(5.54770518671614,15.2,9.5134988772555));
#214917=CARTESIAN_POINT('Ctrl Pts',(5.54842487320309,15.2,9.51755361188376));
#214918=CARTESIAN_POINT('Ctrl Pts',(5.54914042699737,15.2,9.52162336856864));
#214919=CARTESIAN_POINT('Ctrl Pts',(5.54985175409126,15.2,9.52570806662612));
#214920=CARTESIAN_POINT('Ctrl Pts',(5.55056308108823,15.2,9.52979276412706));
#214921=CARTESIAN_POINT('Ctrl Pts',(5.55127018244964,15.2,9.53389240187326));
#214922=CARTESIAN_POINT('Ctrl Pts',(5.5519729647258,15.2,9.53800689664705));
#214923=CARTESIAN_POINT('Ctrl Pts',(5.55267574709771,15.2,9.54212139198143));
#214924=CARTESIAN_POINT('Ctrl Pts',(5.55337420969798,15.2,9.54625074512554));
#214925=CARTESIAN_POINT('Ctrl Pts',(5.55406826282565,15.2,9.55039487405968));
#214926=CARTESIAN_POINT('Ctrl Pts',(5.55476231585875,15.2,9.5545390024292));
#214927=CARTESIAN_POINT('Ctrl Pts',(5.55545195883573,15.2,9.55869790522049));
#214928=CARTESIAN_POINT('Ctrl Pts',(5.55613710116891,15.2,9.56287150260054));
#214929=CARTESIAN_POINT('Ctrl Pts',(5.55682224359543,15.2,9.56704510054923));
#214930=CARTESIAN_POINT('Ctrl Pts',(5.55750288499086,15.2,9.57123339148861));
#214931=CARTESIAN_POINT('Ctrl Pts',(5.55817893680519,15.2,9.57543629555199));
#214932=CARTESIAN_POINT('Ctrl Pts',(5.5588549885274,15.2,9.57963919904272));
#214933=CARTESIAN_POINT('Ctrl Pts',(5.55952645124896,15.2,9.58385671571892));
#214934=CARTESIAN_POINT('Ctrl Pts',(5.56019323439485,15.2,9.58808876286091));
#214935=CARTESIAN_POINT('Ctrl Pts',(5.56102671339534,15.2,9.59337882222087));
#214936=CARTESIAN_POINT('Ctrl Pts',(5.56185288362376,15.2,9.5986915873634));
#214937=CARTESIAN_POINT('Ctrl Pts',(5.56267157397138,15.2,9.60402690041779));
#214938=CARTESIAN_POINT('Ctrl Pts',(5.56349026431899,15.2,9.6093622134722));
#214939=CARTESIAN_POINT('Ctrl Pts',(5.56430147371364,15.2,9.61472007573824));
#214940=CARTESIAN_POINT('Ctrl Pts',(5.56510503517236,15.2,9.62010032893153));
#214941=CARTESIAN_POINT('Ctrl Pts',(5.5659085966311,15.2,9.6254805821248));
#214942=CARTESIAN_POINT('Ctrl Pts',(5.56670451099593,15.2,9.63088322722794));
#214943=CARTESIAN_POINT('Ctrl Pts',(5.5674926107912,15.2,9.63630811023865));
#214944=CARTESIAN_POINT('Ctrl Pts',(5.56812309066178,15.2,9.64064801688375));
#214945=CARTESIAN_POINT('Ctrl Pts',(5.56874856855144,15.2,9.64500215411906));
#214946=CARTESIAN_POINT('Ctrl Pts',(5.56936896358473,15.2,9.6493704442475));
#214947=CARTESIAN_POINT('Ctrl Pts',(5.57014445733409,15.2,9.65483080661045));
#214948=CARTESIAN_POINT('Ctrl Pts',(5.57091200490551,15.2,9.66031328220149));
#214949=CARTESIAN_POINT('Ctrl Pts',(5.57167144705763,15.2,9.66581771699492));
#214950=CARTESIAN_POINT('Ctrl Pts',(5.57227900072965,15.2,9.67022126446967));
#214951=CARTESIAN_POINT('Ctrl Pts',(5.57288136675953,15.2,9.674638865753));
#214952=CARTESIAN_POINT('Ctrl Pts',(5.57347846199122,15.2,9.67907044268858));
#214953=CARTESIAN_POINT('Ctrl Pts',(5.57407555730428,15.2,9.68350202022796));
#214954=CARTESIAN_POINT('Ctrl Pts',(5.57466738393944,15.2,9.68794757397072));
#214955=CARTESIAN_POINT('Ctrl Pts',(5.57525385913752,15.2,9.69240702593738));
#214956=CARTESIAN_POINT('Ctrl Pts',(5.57598695309516,15.2,9.69798134059192));
#214957=CARTESIAN_POINT('Ctrl Pts',(5.576711687361,15.2,9.70357736888849));
#214958=CARTESIAN_POINT('Ctrl Pts',(5.57742790465198,15.2,9.70919496270973));
#214959=CARTESIAN_POINT('Ctrl Pts',(5.57785763501095,15.2,9.71256551888001));
#214960=CARTESIAN_POINT('Ctrl Pts',(5.57828429970981,15.2,9.71594383709144));
#214961=CARTESIAN_POINT('Ctrl Pts',(5.57870786513189,15.2,9.71932988693013));
#214962=CARTESIAN_POINT('Ctrl Pts',(5.57941380752767,15.2,9.72497330353301));
#214963=CARTESIAN_POINT('Ctrl Pts',(5.58011114089075,15.2,9.73063819103081));
#214964=CARTESIAN_POINT('Ctrl Pts',(5.58079971234836,15.2,9.7363244040187));
#214965=CARTESIAN_POINT('Ctrl Pts',(5.58135056946943,15.2,9.74087337403714));
#214966=CARTESIAN_POINT('Ctrl Pts',(5.58189581960788,15.2,9.74543598981206));
#214967=CARTESIAN_POINT('Ctrl Pts',(5.5824353847308,15.2,9.75001217665929));
#214968=CARTESIAN_POINT('Ctrl Pts',(5.58284005859138,15.2,9.75344431695061));
#214969=CARTESIAN_POINT('Ctrl Pts',(5.58324153406708,15.2,9.75688409073694));
#214970=CARTESIAN_POINT('Ctrl Pts',(5.58363978044788,15.2,9.76033146532468));
#214971=CARTESIAN_POINT('Ctrl Pts',(5.58403802682868,15.2,9.76377883991242));
#214972=CARTESIAN_POINT('Ctrl Pts',(5.58443304351169,15.2,9.76723381760528));
#214973=CARTESIAN_POINT('Ctrl Pts',(5.58482479795623,15.2,9.7706963625201));
#214974=CARTESIAN_POINT('Ctrl Pts',(5.58521655247194,15.2,9.77415890806395));
#214975=CARTESIAN_POINT('Ctrl Pts',(5.5856050453284,15.2,9.77762902376828));
#214976=CARTESIAN_POINT('Ctrl Pts',(5.58599024430061,15.2,9.78110667577474));
#214977=CARTESIAN_POINT('Ctrl Pts',(5.58637544320283,15.2,9.78458432714942));
#214978=CARTESIAN_POINT('Ctrl Pts',(5.58675734805522,15.2,9.78806951627366));
#214979=CARTESIAN_POINT('Ctrl Pts',(5.58713592879118,15.2,9.79156221014743));
#214980=CARTESIAN_POINT('Ctrl Pts',(5.58776689670736,15.2,9.79738336681522));
#214981=CARTESIAN_POINT('Ctrl Pts',(5.58838862555219,15.2,9.80322537210294));
#214982=CARTESIAN_POINT('Ctrl Pts',(5.58900097530435,15.2,9.80908807968891));
#214983=CARTESIAN_POINT('Ctrl Pts',(5.58961332505651,15.2,9.81495078727488));
#214984=CARTESIAN_POINT('Ctrl Pts',(5.59021629202837,15.2,9.82083419513713));
#214985=CARTESIAN_POINT('Ctrl Pts',(5.59080973681925,15.2,9.82673815847218));
#214986=CARTESIAN_POINT('Ctrl Pts',(5.59116580368086,15.2,9.83028053634449));
#214987=CARTESIAN_POINT('Ctrl Pts',(5.59151844210096,15.2,9.83383031509972));
#214988=CARTESIAN_POINT('Ctrl Pts',(5.59186762154631,15.2,9.8373874613878));
#214989=CARTESIAN_POINT('Ctrl Pts',(5.59221680099165,15.2,9.84094460767589));
#214990=CARTESIAN_POINT('Ctrl Pts',(5.59256252184574,15.2,9.84450912229638));
#214991=CARTESIAN_POINT('Ctrl Pts',(5.59290475370831,15.2,9.84808097454161));
#214992=CARTESIAN_POINT('Ctrl Pts',(5.59324698557087,15.2,9.85165282678683));
#214993=CARTESIAN_POINT('Ctrl Pts',(5.59358572742524,15.2,9.85523201584012));
#214994=CARTESIAN_POINT('Ctrl Pts',(5.5939209512467,15.2,9.85881851112579));
#214995=CARTESIAN_POINT('Ctrl Pts',(5.59447965763609,15.2,9.86479600348576));
#214996=CARTESIAN_POINT('Ctrl Pts',(5.59502858784164,15.2,9.87079379022497));
#214997=CARTESIAN_POINT('Ctrl Pts',(5.59556760548301,15.2,9.87681172677999));
#214998=CARTESIAN_POINT('Ctrl Pts',(5.59589101605607,15.2,9.8804224885818));
#214999=CARTESIAN_POINT('Ctrl Pts',(5.59621085935995,15.2,9.88404050453726));
#215000=CARTESIAN_POINT('Ctrl Pts',(5.59652710389044,15.2,9.88766574336324));
#215001=CARTESIAN_POINT('Ctrl Pts',(5.59684334842093,15.2,9.89129098218923));
#215002=CARTESIAN_POINT('Ctrl Pts',(5.59715599571,15.2,9.89492344388971));
#215003=CARTESIAN_POINT('Ctrl Pts',(5.5974650156576,15.2,9.89856309817317));
#215004=CARTESIAN_POINT('Ctrl Pts',(5.59777403566135,15.2,9.90220275311783));
#215005=CARTESIAN_POINT('Ctrl Pts',(5.59807942928906,15.2,9.90584960063116));
#215006=CARTESIAN_POINT('Ctrl Pts',(5.59838116637408,15.2,9.90950360907985));
#215007=CARTESIAN_POINT('Ctrl Pts',(5.59878348239608,15.2,9.91437561923842));
#215008=CARTESIAN_POINT('Ctrl Pts',(5.59917929962418,15.2,9.91926036112476));
#215009=CARTESIAN_POINT('Ctrl Pts',(5.59956854948304,15.2,9.9241577607466));
#215010=CARTESIAN_POINT('Ctrl Pts',(5.59986048689044,15.2,9.92783081062981));
#215011=CARTESIAN_POINT('Ctrl Pts',(5.60014873031224,15.2,9.93151098146608));
#215012=CARTESIAN_POINT('Ctrl Pts',(5.60043325126056,15.2,9.93519824133148));
#215013=CARTESIAN_POINT('Ctrl Pts',(5.60071777220888,15.2,9.93888550119688));
#215014=CARTESIAN_POINT('Ctrl Pts',(5.60099857099912,15.2,9.9425798508285));
#215015=CARTESIAN_POINT('Ctrl Pts',(5.60127561948957,15.2,9.94628126015137));
#215016=CARTESIAN_POINT('Ctrl Pts',(5.60155266803035,15.2,9.94998267014666));
#215017=CARTESIAN_POINT('Ctrl Pts',(5.60182596658673,15.2,9.95369114070231));
#215018=CARTESIAN_POINT('Ctrl Pts',(5.60209548708372,15.2,9.9574066400766));
#215019=CARTESIAN_POINT('Ctrl Pts',(5.60245484766478,15.2,9.96236063811736));
#215020=CARTESIAN_POINT('Ctrl Pts',(5.60280749045975,15.2,9.96732713044767));
#215021=CARTESIAN_POINT('Ctrl Pts',(5.6031533477664,15.2,9.97230604472988));
#215022=CARTESIAN_POINT('Ctrl Pts',(5.60341274075817,15.2,9.97604023061113));
#215023=CARTESIAN_POINT('Ctrl Pts',(5.60366831649795,15.2,9.97978140382829));
#215024=CARTESIAN_POINT('Ctrl Pts',(5.60392005194747,15.2,9.98352953581651));
#215025=CARTESIAN_POINT('Ctrl Pts',(5.60417178739699,15.2,9.98727766780473));
#215026=CARTESIAN_POINT('Ctrl Pts',(5.60441968127177,15.2,9.99103276188411));
#215027=CARTESIAN_POINT('Ctrl Pts',(5.60466370822177,15.2,9.99479478516316));
#215028=CARTESIAN_POINT('Ctrl Pts',(5.6049077352161,15.2,9.99855680912564));
#215029=CARTESIAN_POINT('Ctrl Pts',(5.605147895501,15.2,10.0023257629567));
#215030=CARTESIAN_POINT('Ctrl Pts',(5.60538415403481,15.2,10.0061016118397));
#215031=CARTESIAN_POINT('Ctrl Pts',(5.60562041252569,15.2,10.0098774600368));
#215032=CARTESIAN_POINT('Ctrl Pts',(5.60585277035814,15.2,10.0136602020641));
#215033=CARTESIAN_POINT('Ctrl Pts',(5.60608119706913,15.2,10.0174498046999));
#215034=CARTESIAN_POINT('Ctrl Pts',(5.60630962378012,15.2,10.0212394073356));
#215035=CARTESIAN_POINT('Ctrl Pts',(5.60653412142436,15.2,10.0250358705591));
#215036=CARTESIAN_POINT('Ctrl Pts',(5.60675467580093,15.2,10.0288391806629));
#215037=CARTESIAN_POINT('Ctrl Pts',(5.6069752301775,15.2,10.0326424907666));
#215038=CARTESIAN_POINT('Ctrl Pts',(5.60719183796131,15.2,10.0364526443066));
#215039=CARTESIAN_POINT('Ctrl Pts',(5.60740451299995,15.2,10.04026965));
#215040=CARTESIAN_POINT('Ctrl Pts',(5.36127880499994,12.2,8.88241603299999));
#215041=CARTESIAN_POINT('Ctrl Pts',(5.36206719568413,12.2,8.88401933383977));
#215042=CARTESIAN_POINT('Ctrl Pts',(5.3628759863957,12.2,8.88567631031983));
#215043=CARTESIAN_POINT('Ctrl Pts',(5.36370417391754,12.2,8.88738636482928));
#215044=CARTESIAN_POINT('Ctrl Pts',(5.36453635537823,12.2,8.88910466608596));
#215045=CARTESIAN_POINT('Ctrl Pts',(5.36538812011717,12.2,8.89087656335787));
#215046=CARTESIAN_POINT('Ctrl Pts',(5.36625847962582,12.2,8.89270147796823));
#215047=CARTESIAN_POINT('Ctrl Pts',(5.36712883905543,12.2,8.89452639241284));
#215048=CARTESIAN_POINT('Ctrl Pts',(5.36801779174953,12.2,8.89640432539507));
#215049=CARTESIAN_POINT('Ctrl Pts',(5.36892438021658,12.2,8.89833471374155));
#215050=CARTESIAN_POINT('Ctrl Pts',(5.36983096868362,12.2,8.90026510208804));
#215051=CARTESIAN_POINT('Ctrl Pts',(5.37075519224708,12.2,8.90224794602847));
#215052=CARTESIAN_POINT('Ctrl Pts',(5.3716961199256,12.2,8.90428269455318));
#215053=CARTESIAN_POINT('Ctrl Pts',(5.37263704768957,12.2,8.90631744326271));
#215054=CARTESIAN_POINT('Ctrl Pts',(5.37359468033524,12.2,8.9084040964046));
#215055=CARTESIAN_POINT('Ctrl Pts',(5.37456811338936,12.2,8.91054211894128));
#215056=CARTESIAN_POINT('Ctrl Pts',(5.37570378515322,12.2,8.91303647827611));
#215057=CARTESIAN_POINT('Ctrl Pts',(5.37686096291785,12.2,8.91560075447309));
#215058=CARTESIAN_POINT('Ctrl Pts',(5.37803825790234,12.2,8.91823411554835));
#215059=CARTESIAN_POINT('Ctrl Pts',(5.3790473680069,12.2,8.92049128244788));
#215060=CARTESIAN_POINT('Ctrl Pts',(5.38007125793053,12.2,8.92279920619165));
#215061=CARTESIAN_POINT('Ctrl Pts',(5.38110908007138,12.2,8.92515737499027));
#215062=CARTESIAN_POINT('Ctrl Pts',(5.38214690211796,12.2,8.92751554357471));
#215063=CARTESIAN_POINT('Ctrl Pts',(5.38319865533422,12.2,8.9299239569457));
#215064=CARTESIAN_POINT('Ctrl Pts',(5.38426351746706,12.2,8.93238211453432));
#215065=CARTESIAN_POINT('Ctrl Pts',(5.38532837959989,12.2,8.93484027212294));
#215066=CARTESIAN_POINT('Ctrl Pts',(5.3864063481307,12.2,8.93734817377245));
#215067=CARTESIAN_POINT('Ctrl Pts',(5.38749662325722,12.2,8.93990532934408));
#215068=CARTESIAN_POINT('Ctrl Pts',(5.38858689848278,12.2,8.94246248514798));
#215069=CARTESIAN_POINT('Ctrl Pts',(5.38968947790153,12.2,8.94506889477464));
#215070=CARTESIAN_POINT('Ctrl Pts',(5.39080358337969,12.2,8.94772407675599));
#215071=CARTESIAN_POINT('Ctrl Pts',(5.39191768875667,12.2,8.95037925849614));
#215072=CARTESIAN_POINT('Ctrl Pts',(5.39304331814439,12.2,8.95308321474799));
#215073=CARTESIAN_POINT('Ctrl Pts',(5.39417971535357,12.2,8.95583547065011));
#215074=CARTESIAN_POINT('Ctrl Pts',(5.39531611256277,12.2,8.95858772655223));
#215075=CARTESIAN_POINT('Ctrl Pts',(5.39646327322106,12.2,8.96138828550877));
#215076=CARTESIAN_POINT('Ctrl Pts',(5.39762045992857,12.2,8.96423668331986));
#215077=CARTESIAN_POINT('Ctrl Pts',(5.39877764663609,12.2,8.96708508113096));
#215078=CARTESIAN_POINT('Ctrl Pts',(5.39994486175675,12.2,8.96998131745591));
#215079=CARTESIAN_POINT('Ctrl Pts',(5.40112137963002,12.2,8.97292494117905));
#215080=CARTESIAN_POINT('Ctrl Pts',(5.40229789761017,12.2,8.97586856516956));
#215081=CARTESIAN_POINT('Ctrl Pts',(5.40348372275793,12.2,8.97885957314806));
#215082=CARTESIAN_POINT('Ctrl Pts',(5.40467814957339,12.2,8.981897523149));
#215083=CARTESIAN_POINT('Ctrl Pts',(5.40587257628037,12.2,8.984935472874));
#215084=CARTESIAN_POINT('Ctrl Pts',(5.40707560536163,12.2,8.98802036289522));
#215085=CARTESIAN_POINT('Ctrl Pts',(5.40828655315063,12.2,8.99115175477942));
#215086=CARTESIAN_POINT('Ctrl Pts',(5.40949750093961,12.2,8.99428314666363));
#215087=CARTESIAN_POINT('Ctrl Pts',(5.41071636676135,12.2,8.99746104326049));
#215088=CARTESIAN_POINT('Ctrl Pts',(5.41194248188295,12.2,9.00068501039017));
#215089=CARTESIAN_POINT('Ctrl Pts',(5.41316859711593,12.2,9.00390897781269));
#215090=CARTESIAN_POINT('Ctrl Pts',(5.41440196414134,12.2,9.00717902039809));
#215091=CARTESIAN_POINT('Ctrl Pts',(5.41564192829254,12.2,9.01049471074747));
#215092=CARTESIAN_POINT('Ctrl Pts',(5.41688189233111,12.2,9.01381040079567));
#215093=CARTESIAN_POINT('Ctrl Pts',(5.41812845637254,12.2,9.01717174290682));
#215094=CARTESIAN_POINT('Ctrl Pts',(5.41938098149937,12.2,9.02057831696503));
#215095=CARTESIAN_POINT('Ctrl Pts',(5.42063350662618,12.2,9.02398489102326));
#215096=CARTESIAN_POINT('Ctrl Pts',(5.42189199455013,12.2,9.02743670033225));
#215097=CARTESIAN_POINT('Ctrl Pts',(5.42315582458718,12.2,9.03093333336878));
#215098=CARTESIAN_POINT('Ctrl Pts',(5.42441965473902,12.2,9.03442996672293));
#215099=CARTESIAN_POINT('Ctrl Pts',(5.42568882599815,12.2,9.03797142575305));
#215100=CARTESIAN_POINT('Ctrl Pts',(5.42696273238152,12.2,9.04155730713024));
#215101=CARTESIAN_POINT('Ctrl Pts',(5.42823663864917,12.2,9.04514318818172));
#215102=CARTESIAN_POINT('Ctrl Pts',(5.42951527992153,12.2,9.0487734910667));
#215103=CARTESIAN_POINT('Ctrl Pts',(5.43079806495826,12.2,9.05244781826653));
#215104=CARTESIAN_POINT('Ctrl Pts',(5.43208084999499,12.2,9.05612214546637));
#215105=CARTESIAN_POINT('Ctrl Pts',(5.43336777664106,12.2,9.05984049843734));
#215106=CARTESIAN_POINT('Ctrl Pts',(5.43465826715844,12.2,9.06360248665276));
#215107=CARTESIAN_POINT('Ctrl Pts',(5.435733675962,12.2,9.06673747694619));
#215108=CARTESIAN_POINT('Ctrl Pts',(5.43681156121276,12.2,9.06990276903155));
#215109=CARTESIAN_POINT('Ctrl Pts',(5.43789159246265,12.2,9.07309813930779));
#215110=CARTESIAN_POINT('Ctrl Pts',(5.43897162371255,12.2,9.07629350958402));
#215111=CARTESIAN_POINT('Ctrl Pts',(5.44005380160138,12.2,9.0795189574332));
#215112=CARTESIAN_POINT('Ctrl Pts',(5.44113780521239,12.2,9.08277426507052));
#215113=CARTESIAN_POINT('Ctrl Pts',(5.44222180882341,12.2,9.08602957270784));
#215114=CARTESIAN_POINT('Ctrl Pts',(5.44330763673329,12.2,9.08931473918867));
#215115=CARTESIAN_POINT('Ctrl Pts',(5.44439497451601,12.2,9.09262954448143));
#215116=CARTESIAN_POINT('Ctrl Pts',(5.44548231229873,12.2,9.09594434977421));
#215117=CARTESIAN_POINT('Ctrl Pts',(5.44657115834994,12.2,9.09928879568324));
#215118=CARTESIAN_POINT('Ctrl Pts',(5.44766120376661,12.2,9.10266266672491));
#215119=CARTESIAN_POINT('Ctrl Pts',(5.44875124918328,12.2,9.10603653776656));
#215120=CARTESIAN_POINT('Ctrl Pts',(5.44984249207336,12.2,9.10943983441946));
#215121=CARTESIAN_POINT('Ctrl Pts',(5.45093462930054,12.2,9.11287234151845));
#215122=CARTESIAN_POINT('Ctrl Pts',(5.45202676652772,12.2,9.11630484861744));
#215123=CARTESIAN_POINT('Ctrl Pts',(5.45311979771034,12.2,9.11976656888801));
#215124=CARTESIAN_POINT('Ctrl Pts',(5.4542134240298,12.2,9.12325728923671));
#215125=CARTESIAN_POINT('Ctrl Pts',(5.45530705034927,12.2,9.12674800958542));
#215126=CARTESIAN_POINT('Ctrl Pts',(5.45640127076041,12.2,9.13026773298068));
#215127=CARTESIAN_POINT('Ctrl Pts',(5.45749579207986,12.2,9.13381624673216));
#215128=CARTESIAN_POINT('Ctrl Pts',(5.45859031339931,12.2,9.13736476048364));
#215129=CARTESIAN_POINT('Ctrl Pts',(5.45968513585568,12.2,9.14094206818094));
#215130=CARTESIAN_POINT('Ctrl Pts',(5.4607799698687,12.2,9.14454796266859));
#215131=CARTESIAN_POINT('Ctrl Pts',(5.46187480388173,12.2,9.14815385715625));
#215132=CARTESIAN_POINT('Ctrl Pts',(5.46296964992647,12.2,9.1517883369267));
#215133=CARTESIAN_POINT('Ctrl Pts',(5.46406422388478,12.2,9.15545120047069));
#215134=CARTESIAN_POINT('Ctrl Pts',(5.4651587978431,12.2,9.15911406401468));
#215135=CARTESIAN_POINT('Ctrl Pts',(5.46625310024305,12.2,9.16280530907858));
#215136=CARTESIAN_POINT('Ctrl Pts',(5.46734685170134,12.2,9.16652473526142));
#215137=CARTESIAN_POINT('Ctrl Pts',(5.46844060304041,12.2,9.17024416103885));
#215138=CARTESIAN_POINT('Ctrl Pts',(5.46953380253719,12.2,9.17399176741993));
#215139=CARTESIAN_POINT('Ctrl Pts',(5.47062617880706,12.2,9.1777673547144));
#215140=CARTESIAN_POINT('Ctrl Pts',(5.471718555196,12.2,9.18154294242043));
#215141=CARTESIAN_POINT('Ctrl Pts',(5.47281010629056,12.2,9.18534650960661));
#215142=CARTESIAN_POINT('Ctrl Pts',(5.47390056212398,12.2,9.18917786071545));
#215143=CARTESIAN_POINT('Ctrl Pts',(5.47499101795739,12.2,9.19300921182428));
#215144=CARTESIAN_POINT('Ctrl Pts',(5.47608038170198,12.2,9.19686834516053));
#215145=CARTESIAN_POINT('Ctrl Pts',(5.47716838413264,12.2,9.20075506474153));
#215146=CARTESIAN_POINT('Ctrl Pts',(5.47825638656329,12.2,9.20464178432255));
#215147=CARTESIAN_POINT('Ctrl Pts',(5.47934303200856,12.2,9.20855609118631));
#215148=CARTESIAN_POINT('Ctrl Pts',(5.48042805463232,12.2,9.21249779082578));
#215149=CARTESIAN_POINT('Ctrl Pts',(5.48151307725608,12.2,9.21643949046523));
#215150=CARTESIAN_POINT('Ctrl Pts',(5.48259648117356,12.2,9.22040858079572));
#215151=CARTESIAN_POINT('Ctrl Pts',(5.48367800943754,12.2,9.22440487273872));
#215152=CARTESIAN_POINT('Ctrl Pts',(5.48475953770153,12.2,9.22840116468173));
#215153=CARTESIAN_POINT('Ctrl Pts',(5.48583918855158,12.2,9.23242465535882));
#215154=CARTESIAN_POINT('Ctrl Pts',(5.4869167134128,12.2,9.23647515646851));
#215155=CARTESIAN_POINT('Ctrl Pts',(5.48777873334876,12.2,9.23971555753287));
#215156=CARTESIAN_POINT('Ctrl Pts',(5.4886393897461,12.2,9.2429732441344));
#215157=CARTESIAN_POINT('Ctrl Pts',(5.48949855839128,12.2,9.24624812020022));
#215158=CARTESIAN_POINT('Ctrl Pts',(5.4903577269194,12.2,9.24952299581985));
#215159=CARTESIAN_POINT('Ctrl Pts',(5.4912154050665,12.2,9.25281506044842));
#215160=CARTESIAN_POINT('Ctrl Pts',(5.49207146966329,12.2,9.25612421845456));
#215161=CARTESIAN_POINT('Ctrl Pts',(5.49292753437671,12.2,9.25943337691156));
#215162=CARTESIAN_POINT('Ctrl Pts',(5.49378198440939,12.2,9.26275962837338));
#215163=CARTESIAN_POINT('Ctrl Pts',(5.49463469584464,12.2,9.26610287755673));
#215164=CARTESIAN_POINT('Ctrl Pts',(5.49548740716372,12.2,9.26944612628455));
#215165=CARTESIAN_POINT('Ctrl Pts',(5.49633837897022,12.2,9.27280637324101));
#215166=CARTESIAN_POINT('Ctrl Pts',(5.49718749161006,12.2,9.2761835222433));
#215167=CARTESIAN_POINT('Ctrl Pts',(5.4980366043656,12.2,9.27956067170573));
#215168=CARTESIAN_POINT('Ctrl Pts',(5.4988838562092,12.2,9.28295472484192));
#215169=CARTESIAN_POINT('Ctrl Pts',(5.4997291263107,12.2,9.28636558602892));
#215170=CARTESIAN_POINT('Ctrl Pts',(5.50057439629703,12.2,9.28977644675119));
#215171=CARTESIAN_POINT('Ctrl Pts',(5.50141768383653,12.2,9.29320411643952));
#215172=CARTESIAN_POINT('Ctrl Pts',(5.50225887187908,12.2,9.29664850121177));
#215173=CARTESIAN_POINT('Ctrl Pts',(5.50310006003624,12.2,9.3000928864533));
#215174=CARTESIAN_POINT('Ctrl Pts',(5.5039391477928,12.2,9.30355398628027));
#215175=CARTESIAN_POINT('Ctrl Pts',(5.50477601600886,12.2,9.30703170948562));
#215176=CARTESIAN_POINT('Ctrl Pts',(5.50561288411089,12.2,9.31050943221713));
#215177=CARTESIAN_POINT('Ctrl Pts',(5.50644753472056,12.2,9.31400377668128));
#215178=CARTESIAN_POINT('Ctrl Pts',(5.5072798500972,12.2,9.31751465139257));
#215179=CARTESIAN_POINT('Ctrl Pts',(5.50811216558724,12.2,9.32102552658221));
#215180=CARTESIAN_POINT('Ctrl Pts',(5.50894214577708,12.2,9.32455293209843));
#215181=CARTESIAN_POINT('Ctrl Pts',(5.50976967726663,12.2,9.32809677545826));
#215182=CARTESIAN_POINT('Ctrl Pts',(5.51059720875617,12.2,9.33164061881809));
#215183=CARTESIAN_POINT('Ctrl Pts',(5.51142229116766,12.2,9.33520090112145));
#215184=CARTESIAN_POINT('Ctrl Pts',(5.51224480943444,12.2,9.33877753031806));
#215185=CARTESIAN_POINT('Ctrl Pts',(5.51306732758916,12.2,9.34235415902734));
#215186=CARTESIAN_POINT('Ctrl Pts',(5.51388728342361,12.2,9.34594713578453));
#215187=CARTESIAN_POINT('Ctrl Pts',(5.5147045642494,12.2,9.3495563680058));
#215188=CARTESIAN_POINT('Ctrl Pts',(5.51552184518655,12.2,9.35316560071883));
#215189=CARTESIAN_POINT('Ctrl Pts',(5.51633645107762,12.2,9.35679109096465));
#215190=CARTESIAN_POINT('Ctrl Pts',(5.51714827189936,12.2,9.36043274755369));
#215191=CARTESIAN_POINT('Ctrl Pts',(5.51796009261048,12.2,9.36407440364655));
#215192=CARTESIAN_POINT('Ctrl Pts',(5.51876912729418,12.2,9.36773222668446));
#215193=CARTESIAN_POINT('Ctrl Pts',(5.51957526745069,12.2,9.37140612738306));
#215194=CARTESIAN_POINT('Ctrl Pts',(5.52038140771703,12.2,9.37508002858223));
#215195=CARTESIAN_POINT('Ctrl Pts',(5.52118465309384,12.2,9.3787700061326));
#215196=CARTESIAN_POINT('Ctrl Pts',(5.52198489539939,12.2,9.38247597352111));
#215197=CARTESIAN_POINT('Ctrl Pts',(5.52278513759591,12.2,9.38618194040468));
#215198=CARTESIAN_POINT('Ctrl Pts',(5.52358237706084,12.2,9.38990389484001));
#215199=CARTESIAN_POINT('Ctrl Pts',(5.52437650721834,12.2,9.39364174964451));
#215200=CARTESIAN_POINT('Ctrl Pts',(5.52517063748404,12.2,9.39737960495828));
#215201=CARTESIAN_POINT('Ctrl Pts',(5.52596165798271,12.2,9.40113336004065));
#215202=CARTESIAN_POINT('Ctrl Pts',(5.526749463581,12.2,9.4049029280249));
#215203=CARTESIAN_POINT('Ctrl Pts',(5.52753726907195,12.2,9.40867249549555));
#215204=CARTESIAN_POINT('Ctrl Pts',(5.52832186005834,12.2,9.41245787532344));
#215205=CARTESIAN_POINT('Ctrl Pts',(5.52910313164491,12.2,9.41625898025678));
#215206=CARTESIAN_POINT('Ctrl Pts',(5.52988440333791,12.2,9.42006008570802));
#215207=CARTESIAN_POINT('Ctrl Pts',(5.53066235576293,12.2,9.42387691572295));
#215208=CARTESIAN_POINT('Ctrl Pts',(5.53143688730491,12.2,9.42770938432171));
#215209=CARTESIAN_POINT('Ctrl Pts',(5.53221141874136,12.2,9.4315418523983));
#215210=CARTESIAN_POINT('Ctrl Pts',(5.53298252767017,12.2,9.43538995900788));
#215211=CARTESIAN_POINT('Ctrl Pts',(5.53375011260779,12.2,9.43925361713489));
#215212=CARTESIAN_POINT('Ctrl Pts',(5.53451769764998,12.2,9.44311727578831));
#215213=CARTESIAN_POINT('Ctrl Pts',(5.53528175881948,12.2,9.44699648553922));
#215214=CARTESIAN_POINT('Ctrl Pts',(5.53604219647548,12.2,9.45089116276925));
#215215=CARTESIAN_POINT('Ctrl Pts',(5.53680263402787,12.2,9.45478583946862));
#215216=CARTESIAN_POINT('Ctrl Pts',(5.53755944722412,12.2,9.45869598150561));
#215217=CARTESIAN_POINT('Ctrl Pts',(5.53831253688516,12.2,9.46262150434977));
#215218=CARTESIAN_POINT('Ctrl Pts',(5.5390656266488,12.2,9.46654702772878));
#215219=CARTESIAN_POINT('Ctrl Pts',(5.53981499415934,12.2,9.47048793140378));
#215220=CARTESIAN_POINT('Ctrl Pts',(5.54056053853329,12.2,9.47444413200825));
#215221=CARTESIAN_POINT('Ctrl Pts',(5.54149246894995,12.2,9.47938938249433));
#215222=CARTESIAN_POINT('Ctrl Pts',(5.54241842959441,12.2,9.48435853253883));
#215223=CARTESIAN_POINT('Ctrl Pts',(5.5433382284833,12.2,9.48935141656659));
#215224=CARTESIAN_POINT('Ctrl Pts',(5.54407406763451,12.2,9.49334572400649));
#215225=CARTESIAN_POINT('Ctrl Pts',(5.54480596489638,12.2,9.49735522218987));
#215226=CARTESIAN_POINT('Ctrl Pts',(5.5455338226023,12.2,9.50137982746629));
#215227=CARTESIAN_POINT('Ctrl Pts',(5.54626168020904,12.2,9.50540443219436));
#215228=CARTESIAN_POINT('Ctrl Pts',(5.54698550032724,12.2,9.50944414317971));
#215229=CARTESIAN_POINT('Ctrl Pts',(5.54770518671614,12.2,9.5134988772555));
#215230=CARTESIAN_POINT('Ctrl Pts',(5.54842487320309,12.2,9.51755361188376));
#215231=CARTESIAN_POINT('Ctrl Pts',(5.54914042699737,12.2,9.52162336856864));
#215232=CARTESIAN_POINT('Ctrl Pts',(5.54985175409126,12.2,9.52570806662612));
#215233=CARTESIAN_POINT('Ctrl Pts',(5.55056308108823,12.2,9.52979276412706));
#215234=CARTESIAN_POINT('Ctrl Pts',(5.55127018244964,12.2,9.53389240187326));
#215235=CARTESIAN_POINT('Ctrl Pts',(5.5519729647258,12.2,9.53800689664705));
#215236=CARTESIAN_POINT('Ctrl Pts',(5.55267574709771,12.2,9.54212139198143));
#215237=CARTESIAN_POINT('Ctrl Pts',(5.55337420969798,12.2,9.54625074512554));
#215238=CARTESIAN_POINT('Ctrl Pts',(5.55406826282565,12.2,9.55039487405968));
#215239=CARTESIAN_POINT('Ctrl Pts',(5.55476231585875,12.2,9.5545390024292));
#215240=CARTESIAN_POINT('Ctrl Pts',(5.55545195883573,12.2,9.55869790522049));
#215241=CARTESIAN_POINT('Ctrl Pts',(5.55613710116891,12.2,9.56287150260054));
#215242=CARTESIAN_POINT('Ctrl Pts',(5.55682224359543,12.2,9.56704510054923));
#215243=CARTESIAN_POINT('Ctrl Pts',(5.55750288499086,12.2,9.57123339148861));
#215244=CARTESIAN_POINT('Ctrl Pts',(5.55817893680519,12.2,9.57543629555199));
#215245=CARTESIAN_POINT('Ctrl Pts',(5.5588549885274,12.2,9.57963919904272));
#215246=CARTESIAN_POINT('Ctrl Pts',(5.55952645124896,12.2,9.58385671571892));
#215247=CARTESIAN_POINT('Ctrl Pts',(5.56019323439485,12.2,9.58808876286091));
#215248=CARTESIAN_POINT('Ctrl Pts',(5.56102671339534,12.2,9.59337882222087));
#215249=CARTESIAN_POINT('Ctrl Pts',(5.56185288362376,12.2,9.5986915873634));
#215250=CARTESIAN_POINT('Ctrl Pts',(5.56267157397138,12.2,9.6040269004178));
#215251=CARTESIAN_POINT('Ctrl Pts',(5.56332652628516,12.2,9.60829515109394));
#215252=CARTESIAN_POINT('Ctrl Pts',(5.56397669008727,12.2,9.61257783309124));
#215253=CARTESIAN_POINT('Ctrl Pts',(5.56462198184434,12.2,9.61687486582635));
#215254=CARTESIAN_POINT('Ctrl Pts',(5.56526727351349,12.2,9.621171897976));
#215255=CARTESIAN_POINT('Ctrl Pts',(5.56590769039972,12.2,9.6254832805583));
#215256=CARTESIAN_POINT('Ctrl Pts',(5.56654315015773,12.2,9.629808934364));
#215257=CARTESIAN_POINT('Ctrl Pts',(5.56717861000232,12.2,9.63413458875908));
#215258=CARTESIAN_POINT('Ctrl Pts',(5.56780911127284,12.2,9.63847451556499));
#215259=CARTESIAN_POINT('Ctrl Pts',(5.56843456908438,12.2,9.64282863308101));
#215260=CARTESIAN_POINT('Ctrl Pts',(5.5690600268107,12.2,9.64718275000377));
#215261=CARTESIAN_POINT('Ctrl Pts',(5.5696804424908,12.2,9.65155105993478));
#215262=CARTESIAN_POINT('Ctrl Pts',(5.57029573160769,12.2,9.65593348207507));
#215263=CARTESIAN_POINT('Ctrl Pts',(5.57091102080842,12.2,9.66031590481246));
#215264=CARTESIAN_POINT('Ctrl Pts',(5.57152118377301,12.2,9.66471244115915));
#215265=CARTESIAN_POINT('Ctrl Pts',(5.57212613830871,12.2,9.66912301075294));
#215266=CARTESIAN_POINT('Ctrl Pts',(5.57257985416927,12.2,9.67243093764781));
#215267=CARTESIAN_POINT('Ctrl Pts',(5.57303064054712,12.2,9.67574675983595));
#215268=CARTESIAN_POINT('Ctrl Pts',(5.57347846199122,12.2,9.67907044268858));
#215269=CARTESIAN_POINT('Ctrl Pts',(5.57392628343534,12.2,9.68239412554122));
#215270=CARTESIAN_POINT('Ctrl Pts',(5.57437114110088,12.2,9.68572567055809));
#215271=CARTESIAN_POINT('Ctrl Pts',(5.57481300041842,12.2,9.6890650433944));
#215272=CARTESIAN_POINT('Ctrl Pts',(5.57525485973595,12.2,9.69240441623071));
#215273=CARTESIAN_POINT('Ctrl Pts',(5.57569371987037,12.2,9.69575161812483));
#215274=CARTESIAN_POINT('Ctrl Pts',(5.57612954864662,12.2,9.69910661496022));
#215275=CARTESIAN_POINT('Ctrl Pts',(5.57656537750204,12.2,9.7024616124051));
#215276=CARTESIAN_POINT('Ctrl Pts',(5.57699817421494,12.2,9.70582440592713));
#215277=CARTESIAN_POINT('Ctrl Pts',(5.57742790465198,12.2,9.70919496270973));
#215278=CARTESIAN_POINT('Ctrl Pts',(5.57785763501095,12.2,9.71256551888001));
#215279=CARTESIAN_POINT('Ctrl Pts',(5.57828429970981,12.2,9.71594383709144));
#215280=CARTESIAN_POINT('Ctrl Pts',(5.57870786513189,12.2,9.71932988693013));
#215281=CARTESIAN_POINT('Ctrl Pts',(5.57913143055397,12.2,9.72271593676883));
#215282=CARTESIAN_POINT('Ctrl Pts',(5.57955189691084,12.2,9.72610971659373));
#215283=CARTESIAN_POINT('Ctrl Pts',(5.57996923081207,12.2,9.72951119392916));
#215284=CARTESIAN_POINT('Ctrl Pts',(5.5803865647133,12.2,9.73291267126461));
#215285=CARTESIAN_POINT('Ctrl Pts',(5.58080076609824,12.2,9.7363218472074));
#215286=CARTESIAN_POINT('Ctrl Pts',(5.58121180249997,12.2,9.73973868849992));
#215287=CARTESIAN_POINT('Ctrl Pts',(5.5816228389017,12.2,9.74315552979245));
#215288=CARTESIAN_POINT('Ctrl Pts',(5.58203071087023,12.2,9.74658003636799));
#215289=CARTESIAN_POINT('Ctrl Pts',(5.5824353847308,12.2,9.75001217665929));
#215290=CARTESIAN_POINT('Ctrl Pts',(5.58284005859138,12.2,9.75344431695061));
#215291=CARTESIAN_POINT('Ctrl Pts',(5.58324153406708,12.2,9.75688409073694));
#215292=CARTESIAN_POINT('Ctrl Pts',(5.58363978044788,12.2,9.76033146532468));
#215293=CARTESIAN_POINT('Ctrl Pts',(5.58403802682868,12.2,9.76377883991242));
#215294=CARTESIAN_POINT('Ctrl Pts',(5.58443304351169,12.2,9.76723381760528));
#215295=CARTESIAN_POINT('Ctrl Pts',(5.58482479795623,12.2,9.7706963625201));
#215296=CARTESIAN_POINT('Ctrl Pts',(5.58521655247194,12.2,9.77415890806395));
#215297=CARTESIAN_POINT('Ctrl Pts',(5.5856050453284,12.2,9.77762902376828));
#215298=CARTESIAN_POINT('Ctrl Pts',(5.58599024430061,12.2,9.78110667577474));
#215299=CARTESIAN_POINT('Ctrl Pts',(5.58637544320283,12.2,9.78458432714942));
#215300=CARTESIAN_POINT('Ctrl Pts',(5.58675734805522,12.2,9.78806951627366));
#215301=CARTESIAN_POINT('Ctrl Pts',(5.58713592879118,12.2,9.79156221014743));
#215302=CARTESIAN_POINT('Ctrl Pts',(5.58764070308286,12.2,9.79621913510096));
#215303=CARTESIAN_POINT('Ctrl Pts',(5.58813956426023,12.2,9.80088940296212));
#215304=CARTESIAN_POINT('Ctrl Pts',(5.58863244091175,12.2,9.80557293931206));
#215305=CARTESIAN_POINT('Ctrl Pts',(5.58900209841717,12.2,9.80908559173404));
#215306=CARTESIAN_POINT('Ctrl Pts',(5.58936838920025,12.2,9.81260570737679));
#215307=CARTESIAN_POINT('Ctrl Pts',(5.58973128210419,12.2,9.8161332537476));
#215308=CARTESIAN_POINT('Ctrl Pts',(5.59009417507406,12.2,9.81966080075924));
#215309=CARTESIAN_POINT('Ctrl Pts',(5.59045366989297,12.2,9.82319577995633));
#215310=CARTESIAN_POINT('Ctrl Pts',(5.59080973681925,12.2,9.82673815847218));
#215311=CARTESIAN_POINT('Ctrl Pts',(5.59116580368086,12.2,9.83028053634449));
#215312=CARTESIAN_POINT('Ctrl Pts',(5.59151844210096,12.2,9.83383031509972));
#215313=CARTESIAN_POINT('Ctrl Pts',(5.59186762154631,12.2,9.8373874613878));
#215314=CARTESIAN_POINT('Ctrl Pts',(5.59221680099165,12.2,9.84094460767589));
#215315=CARTESIAN_POINT('Ctrl Pts',(5.59256252184574,12.2,9.84450912229638));
#215316=CARTESIAN_POINT('Ctrl Pts',(5.59290475370831,12.2,9.84808097454161));
#215317=CARTESIAN_POINT('Ctrl Pts',(5.59324698557087,12.2,9.85165282678683));
#215318=CARTESIAN_POINT('Ctrl Pts',(5.59358572742524,12.2,9.85523201584012));
#215319=CARTESIAN_POINT('Ctrl Pts',(5.5939209512467,12.2,9.85881851112579));
#215320=CARTESIAN_POINT('Ctrl Pts',(5.59425617506815,12.2,9.86240500641146));
#215321=CARTESIAN_POINT('Ctrl Pts',(5.59458787878156,12.2,9.86599880757176));
#215322=CARTESIAN_POINT('Ctrl Pts',(5.59491603466144,12.2,9.86959988357828));
#215323=CARTESIAN_POINT('Ctrl Pts',(5.59524419054132,12.2,9.87320095958478));
#215324=CARTESIAN_POINT('Ctrl Pts',(5.59556879660783,12.2,9.87680931036078));
#215325=CARTESIAN_POINT('Ctrl Pts',(5.59588982588831,12.2,9.88042490468673));
#215326=CARTESIAN_POINT('Ctrl Pts',(5.59631786496785,12.2,9.88524569755923));
#215327=CARTESIAN_POINT('Ctrl Pts',(5.59673954193012,12.2,9.89007936839968));
#215328=CARTESIAN_POINT('Ctrl Pts',(5.59715478800831,12.2,9.89492584327494));
#215329=CARTESIAN_POINT('Ctrl Pts',(5.59746622253866,12.2,9.89856069910121));
#215330=CARTESIAN_POINT('Ctrl Pts',(5.59777404002748,12.2,9.9022027577855));
#215331=CARTESIAN_POINT('Ctrl Pts',(5.59807821143342,12.2,9.90585198806896));
#215332=CARTESIAN_POINT('Ctrl Pts',(5.59838238283935,12.2,9.90950121835242));
#215333=CARTESIAN_POINT('Ctrl Pts',(5.59868290762136,12.2,9.91315761960878));
#215334=CARTESIAN_POINT('Ctrl Pts',(5.59897975800084,12.2,9.91682116253287));
#215335=CARTESIAN_POINT('Ctrl Pts',(5.5992766083803,12.2,9.92048470545697));
#215336=CARTESIAN_POINT('Ctrl Pts',(5.59956978298021,12.2,9.92415538868278));
#215337=CARTESIAN_POINT('Ctrl Pts',(5.5998592544702,12.2,9.92783318242318));
#215338=CARTESIAN_POINT('Ctrl Pts',(5.60014872601277,12.2,9.9315109768317));
#215339=CARTESIAN_POINT('Ctrl Pts',(5.60043449417097,12.2,9.93519588088392));
#215340=CARTESIAN_POINT('Ctrl Pts',(5.60071653029478,12.2,9.93888786479647));
#215341=CARTESIAN_POINT('Ctrl Pts',(5.60109257837447,12.2,9.94381050889536));
#215342=CARTESIAN_POINT('Ctrl Pts',(5.60146199282447,12.2,9.94874573857864));
#215343=CARTESIAN_POINT('Ctrl Pts',(5.60182470796192,12.2,9.95369348406225));
#215344=CARTESIAN_POINT('Ctrl Pts',(5.60209674432737,12.2,9.95740429334348));
#215345=CARTESIAN_POINT('Ctrl Pts',(5.60236501149473,12.2,9.96112214152942));
#215346=CARTESIAN_POINT('Ctrl Pts',(5.6026294809571,12.2,9.964846997496));
#215347=CARTESIAN_POINT('Ctrl Pts',(5.60289395041948,12.2,9.96857185346258));
#215348=CARTESIAN_POINT('Ctrl Pts',(5.60315462186946,12.2,9.97230371693833));
#215349=CARTESIAN_POINT('Ctrl Pts',(5.60341146744397,12.2,9.97604255817653));
#215350=CARTESIAN_POINT('Ctrl Pts',(5.60366831306516,12.2,9.97978140009396));
#215351=CARTESIAN_POINT('Ctrl Pts',(5.6039213345186,12.2,9.9835272181217));
#215352=CARTESIAN_POINT('Ctrl Pts',(5.60417050609595,12.2,9.98727998854306));
#215353=CARTESIAN_POINT('Ctrl Pts',(5.60441967762805,12.2,9.99103275828267));
#215354=CARTESIAN_POINT('Ctrl Pts',(5.604664999652,12.2,9.99479247918021));
#215355=CARTESIAN_POINT('Ctrl Pts',(5.60490644497622,12.2,9.99855911841896));
#215356=CARTESIAN_POINT('Ctrl Pts',(5.60514789030045,12.2,10.0023257576577));
#215357=CARTESIAN_POINT('Ctrl Pts',(5.6053854563743,12.2,10.0060993155569));
#215358=CARTESIAN_POINT('Ctrl Pts',(5.60561911124185,12.2,10.0098797562284));
#215359=CARTESIAN_POINT('Ctrl Pts',(5.60585276610941,12.2,10.0136601968999));
#215360=CARTESIAN_POINT('Ctrl Pts',(5.60608250774026,12.2,10.0174475182505));
#215361=CARTESIAN_POINT('Ctrl Pts',(5.6063083134831,12.2,10.0212416932965));
#215362=CARTESIAN_POINT('Ctrl Pts',(5.6066846564015,12.2,10.0275653186029));
#215363=CARTESIAN_POINT('Ctrl Pts',(5.60705005458934,12.2,10.0339079736131));
#215364=CARTESIAN_POINT('Ctrl Pts',(5.60740451299995,12.2,10.04026965));
#215365=CARTESIAN_POINT('Ctrl Pts',(5.26939701799994,15.2,10.221714878));
#215366=CARTESIAN_POINT('Ctrl Pts',(5.26939701799994,11.6,10.221714878));
#215367=CARTESIAN_POINT('Ctrl Pts',(5.26878426899994,15.2,10.221257575));
#215368=CARTESIAN_POINT('Ctrl Pts',(5.26878426899994,11.6,10.221257575));
#215369=CARTESIAN_POINT('Ctrl Pts',(5.26755929399994,15.2,10.220343));
#215370=CARTESIAN_POINT('Ctrl Pts',(5.26755929399994,11.6,10.220343));
#215371=CARTESIAN_POINT('Ctrl Pts',(5.26572340899994,15.2,10.218971238));
#215372=CARTESIAN_POINT('Ctrl Pts',(5.26572340899994,11.6,10.218971238));
#215373=CARTESIAN_POINT('Ctrl Pts',(5.26327871499994,15.2,10.217142421));
#215374=CARTESIAN_POINT('Ctrl Pts',(5.26327871499994,11.6,10.217142421));
#215375=CARTESIAN_POINT('Ctrl Pts',(5.26022810499994,15.2,10.214856731));
#215376=CARTESIAN_POINT('Ctrl Pts',(5.26022810499994,11.6,10.214856731));
#215377=CARTESIAN_POINT('Ctrl Pts',(5.25718275199995,15.2,10.212571374));
#215378=CARTESIAN_POINT('Ctrl Pts',(5.25718275199995,11.6,10.212571374));
#215379=CARTESIAN_POINT('Ctrl Pts',(5.25414265599994,15.2,10.210286353));
#215380=CARTESIAN_POINT('Ctrl Pts',(5.25414265599994,11.6,10.210286353));
#215381=CARTESIAN_POINT('Ctrl Pts',(5.25110781899994,15.2,10.208001669));
#215382=CARTESIAN_POINT('Ctrl Pts',(5.25110781899994,11.6,10.208001669));
#215383=CARTESIAN_POINT('Ctrl Pts',(5.24807824099994,15.2,10.205717331));
#215384=CARTESIAN_POINT('Ctrl Pts',(5.24807824099994,11.6,10.205717331));
#215385=CARTESIAN_POINT('Ctrl Pts',(5.24505392599994,15.2,10.203433344));
#215386=CARTESIAN_POINT('Ctrl Pts',(5.24505392599994,11.6,10.203433344));
#215387=CARTESIAN_POINT('Ctrl Pts',(5.24203487699994,15.2,10.20114972));
#215388=CARTESIAN_POINT('Ctrl Pts',(5.24203487699994,11.6,10.20114972));
#215389=CARTESIAN_POINT('Ctrl Pts',(5.23902109399994,15.2,10.198866469));
#215390=CARTESIAN_POINT('Ctrl Pts',(5.23902109399994,11.6,10.198866469));
#215391=CARTESIAN_POINT('Ctrl Pts',(5.23601258199994,15.2,10.1965836));
#215392=CARTESIAN_POINT('Ctrl Pts',(5.23601258199994,11.6,10.1965836));
#215393=CARTESIAN_POINT('Ctrl Pts',(5.23300934399994,15.2,10.194301126));
#215394=CARTESIAN_POINT('Ctrl Pts',(5.23300934399994,11.6,10.194301126));
#215395=CARTESIAN_POINT('Ctrl Pts',(5.23001137999994,15.2,10.192019056));
#215396=CARTESIAN_POINT('Ctrl Pts',(5.23001137999994,11.6,10.192019056));
#215397=CARTESIAN_POINT('Ctrl Pts',(5.22701869399994,15.2,10.189737398));
#215398=CARTESIAN_POINT('Ctrl Pts',(5.22701869399994,11.6,10.189737398));
#215399=CARTESIAN_POINT('Ctrl Pts',(5.22403128899994,15.2,10.187456163));
#215400=CARTESIAN_POINT('Ctrl Pts',(5.22403128899994,11.6,10.187456163));
#215401=CARTESIAN_POINT('Ctrl Pts',(5.22104916599995,15.2,10.185175356));
#215402=CARTESIAN_POINT('Ctrl Pts',(5.22104916599995,11.6,10.185175356));
#215403=CARTESIAN_POINT('Ctrl Pts',(5.21807232699994,15.2,10.182894988));
#215404=CARTESIAN_POINT('Ctrl Pts',(5.21807232699994,11.6,10.182894988));
#215405=CARTESIAN_POINT('Ctrl Pts',(5.21510077399994,15.2,10.180615065));
#215406=CARTESIAN_POINT('Ctrl Pts',(5.21510077399994,11.6,10.180615065));
#215407=CARTESIAN_POINT('Ctrl Pts',(5.21213450999994,15.2,10.178335595));
#215408=CARTESIAN_POINT('Ctrl Pts',(5.21213450999994,11.6,10.178335595));
#215409=CARTESIAN_POINT('Ctrl Pts',(5.20917353599994,15.2,10.176056588));
#215410=CARTESIAN_POINT('Ctrl Pts',(5.20917353599994,11.6,10.176056588));
#215411=CARTESIAN_POINT('Ctrl Pts',(5.20621785499994,15.2,10.173778052));
#215412=CARTESIAN_POINT('Ctrl Pts',(5.20621785499994,11.6,10.173778052));
#215413=CARTESIAN_POINT('Ctrl Pts',(5.20326746799994,15.2,10.171499997));
#215414=CARTESIAN_POINT('Ctrl Pts',(5.20326746799994,11.6,10.171499997));
#215415=CARTESIAN_POINT('Ctrl Pts',(5.20032237999994,15.2,10.169222432));
#215416=CARTESIAN_POINT('Ctrl Pts',(5.20032237999994,11.6,10.169222432));
#215417=CARTESIAN_POINT('Ctrl Pts',(5.19738259199994,15.2,10.166945366));
#215418=CARTESIAN_POINT('Ctrl Pts',(5.19738259199994,11.6,10.166945366));
#215419=CARTESIAN_POINT('Ctrl Pts',(5.19444810399994,15.2,10.164668808));
#215420=CARTESIAN_POINT('Ctrl Pts',(5.19444810399994,11.6,10.164668808));
#215421=CARTESIAN_POINT('Ctrl Pts',(5.19151892099995,15.2,10.162392767));
#215422=CARTESIAN_POINT('Ctrl Pts',(5.19151892099995,11.6,10.162392767));
#215423=CARTESIAN_POINT('Ctrl Pts',(5.18859504499994,15.2,10.160117253));
#215424=CARTESIAN_POINT('Ctrl Pts',(5.18859504499994,11.6,10.160117253));
#215425=CARTESIAN_POINT('Ctrl Pts',(5.18567647699994,15.2,10.157842273));
#215426=CARTESIAN_POINT('Ctrl Pts',(5.18567647699994,11.6,10.157842273));
#215427=CARTESIAN_POINT('Ctrl Pts',(5.18276321899994,15.2,10.155567837));
#215428=CARTESIAN_POINT('Ctrl Pts',(5.18276321899994,11.6,10.155567837));
#215429=CARTESIAN_POINT('Ctrl Pts',(5.17985527399994,15.2,10.153293953));
#215430=CARTESIAN_POINT('Ctrl Pts',(5.17985527399994,11.6,10.153293953));
#215431=CARTESIAN_POINT('Ctrl Pts',(5.17695264399994,15.2,10.151020631));
#215432=CARTESIAN_POINT('Ctrl Pts',(5.17695264399994,11.6,10.151020631));
#215433=CARTESIAN_POINT('Ctrl Pts',(5.17405533099994,15.2,10.14874788));
#215434=CARTESIAN_POINT('Ctrl Pts',(5.17405533099994,11.6,10.14874788));
#215435=CARTESIAN_POINT('Ctrl Pts',(5.17116333899994,15.2,10.146475708));
#215436=CARTESIAN_POINT('Ctrl Pts',(5.17116333899994,11.6,10.146475708));
#215437=CARTESIAN_POINT('Ctrl Pts',(5.16827666699994,15.2,10.144204125));
#215438=CARTESIAN_POINT('Ctrl Pts',(5.16827666699994,11.6,10.144204125));
#215439=CARTESIAN_POINT('Ctrl Pts',(5.16539531799994,15.2,10.141933139));
#215440=CARTESIAN_POINT('Ctrl Pts',(5.16539531799994,11.6,10.141933139));
#215441=CARTESIAN_POINT('Ctrl Pts',(5.16251929599994,15.2,10.139662761));
#215442=CARTESIAN_POINT('Ctrl Pts',(5.16251929599994,11.6,10.139662761));
#215443=CARTESIAN_POINT('Ctrl Pts',(5.15964860199994,15.2,10.137392999));
#215444=CARTESIAN_POINT('Ctrl Pts',(5.15964860199994,11.6,10.137392999));
#215445=CARTESIAN_POINT('Ctrl Pts',(5.15678323799994,15.2,10.135123862));
#215446=CARTESIAN_POINT('Ctrl Pts',(5.15678323799994,11.6,10.135123862));
#215447=CARTESIAN_POINT('Ctrl Pts',(5.15392320699994,15.2,10.132855359));
#215448=CARTESIAN_POINT('Ctrl Pts',(5.15392320699994,11.6,10.132855359));
#215449=CARTESIAN_POINT('Ctrl Pts',(5.15106850999994,15.2,10.130587501));
#215450=CARTESIAN_POINT('Ctrl Pts',(5.15106850999994,11.6,10.130587501));
#215451=CARTESIAN_POINT('Ctrl Pts',(5.14821914899994,15.2,10.128320294));
#215452=CARTESIAN_POINT('Ctrl Pts',(5.14821914899994,11.6,10.128320294));
#215453=CARTESIAN_POINT('Ctrl Pts',(5.14537512799994,15.2,10.12605375));
#215454=CARTESIAN_POINT('Ctrl Pts',(5.14537512799994,11.6,10.12605375));
#215455=CARTESIAN_POINT('Ctrl Pts',(5.14253644699994,15.2,10.123787877));
#215456=CARTESIAN_POINT('Ctrl Pts',(5.14253644699994,11.6,10.123787877));
#215457=CARTESIAN_POINT('Ctrl Pts',(5.13970310899994,15.2,10.121522684));
#215458=CARTESIAN_POINT('Ctrl Pts',(5.13970310899994,11.6,10.121522684));
#215459=CARTESIAN_POINT('Ctrl Pts',(5.13687511699994,15.2,10.119258181));
#215460=CARTESIAN_POINT('Ctrl Pts',(5.13687511699994,11.6,10.119258181));
#215461=CARTESIAN_POINT('Ctrl Pts',(5.13405247199994,15.2,10.116994376));
#215462=CARTESIAN_POINT('Ctrl Pts',(5.13405247199994,11.6,10.116994376));
#215463=CARTESIAN_POINT('Ctrl Pts',(5.13123517599994,15.2,10.114731281));
#215464=CARTESIAN_POINT('Ctrl Pts',(5.13123517599994,11.6,10.114731281));
#215465=CARTESIAN_POINT('Ctrl Pts',(5.12842323199994,15.2,10.112468902));
#215466=CARTESIAN_POINT('Ctrl Pts',(5.12842323199994,11.6,10.112468902));
#215467=CARTESIAN_POINT('Ctrl Pts',(5.12561664199994,15.2,10.11020725));
#215468=CARTESIAN_POINT('Ctrl Pts',(5.12561664199994,11.6,10.11020725));
#215469=CARTESIAN_POINT('Ctrl Pts',(5.12281540699994,15.2,10.107946335));
#215470=CARTESIAN_POINT('Ctrl Pts',(5.12281540699994,11.6,10.107946335));
#215471=CARTESIAN_POINT('Ctrl Pts',(5.12001953099994,15.2,10.105686165));
#215472=CARTESIAN_POINT('Ctrl Pts',(5.12001953099994,11.6,10.105686165));
#215473=CARTESIAN_POINT('Ctrl Pts',(5.11722901399994,15.2,10.103426751));
#215474=CARTESIAN_POINT('Ctrl Pts',(5.11722901399994,11.6,10.103426751));
#215475=CARTESIAN_POINT('Ctrl Pts',(5.11444385999994,15.2,10.101168101));
#215476=CARTESIAN_POINT('Ctrl Pts',(5.11444385999994,11.6,10.101168101));
#215477=CARTESIAN_POINT('Ctrl Pts',(5.11166406899994,15.2,10.098910224));
#215478=CARTESIAN_POINT('Ctrl Pts',(5.11166406899994,11.6,10.098910224));
#215479=CARTESIAN_POINT('Ctrl Pts',(5.10888964499994,15.2,10.09665313));
#215480=CARTESIAN_POINT('Ctrl Pts',(5.10888964499994,11.6,10.09665313));
#215481=CARTESIAN_POINT('Ctrl Pts',(5.10612058999994,15.2,10.094396829));
#215482=CARTESIAN_POINT('Ctrl Pts',(5.10612058999994,11.6,10.094396829));
#215483=CARTESIAN_POINT('Ctrl Pts',(5.10335690499994,15.2,10.092141331));
#215484=CARTESIAN_POINT('Ctrl Pts',(5.10335690499994,11.6,10.092141331));
#215485=CARTESIAN_POINT('Ctrl Pts',(5.10059859199994,15.2,10.089886644));
#215486=CARTESIAN_POINT('Ctrl Pts',(5.10059859199994,11.6,10.089886644));
#215487=CARTESIAN_POINT('Ctrl Pts',(5.09784565399994,15.2,10.087632778));
#215488=CARTESIAN_POINT('Ctrl Pts',(5.09784565399994,11.6,10.087632778));
#215489=CARTESIAN_POINT('Ctrl Pts',(5.09509809299994,15.2,10.085379743));
#215490=CARTESIAN_POINT('Ctrl Pts',(5.09509809299994,11.6,10.085379743));
#215491=CARTESIAN_POINT('Ctrl Pts',(5.09235591199994,15.2,10.083127549));
#215492=CARTESIAN_POINT('Ctrl Pts',(5.09235591199994,11.6,10.083127549));
#215493=CARTESIAN_POINT('Ctrl Pts',(5.08961910999994,15.2,10.080876204));
#215494=CARTESIAN_POINT('Ctrl Pts',(5.08961910999994,11.6,10.080876204));
#215495=CARTESIAN_POINT('Ctrl Pts',(5.08688769099994,15.2,10.078625719));
#215496=CARTESIAN_POINT('Ctrl Pts',(5.08688769099994,11.6,10.078625719));
#215497=CARTESIAN_POINT('Ctrl Pts',(5.08416165799994,15.2,10.076376103));
#215498=CARTESIAN_POINT('Ctrl Pts',(5.08416165799994,11.6,10.076376103));
#215499=CARTESIAN_POINT('Ctrl Pts',(5.08144101099994,15.2,10.074127366));
#215500=CARTESIAN_POINT('Ctrl Pts',(5.08144101099994,11.6,10.074127366));
#215501=CARTESIAN_POINT('Ctrl Pts',(5.07872575399994,15.2,10.071879516));
#215502=CARTESIAN_POINT('Ctrl Pts',(5.07872575399994,11.6,10.071879516));
#215503=CARTESIAN_POINT('Ctrl Pts',(5.07601588799994,15.2,10.069632566));
#215504=CARTESIAN_POINT('Ctrl Pts',(5.07601588799994,11.6,10.069632566));
#215505=CARTESIAN_POINT('Ctrl Pts',(5.07331141499994,15.2,10.067386522));
#215506=CARTESIAN_POINT('Ctrl Pts',(5.07331141499994,11.6,10.067386522));
#215507=CARTESIAN_POINT('Ctrl Pts',(5.07061233699994,15.2,10.065141396));
#215508=CARTESIAN_POINT('Ctrl Pts',(5.07061233699994,11.6,10.065141396));
#215509=CARTESIAN_POINT('Ctrl Pts',(5.06791865699994,15.2,10.062897197));
#215510=CARTESIAN_POINT('Ctrl Pts',(5.06791865699994,11.6,10.062897197));
#215511=CARTESIAN_POINT('Ctrl Pts',(5.06523037499995,15.2,10.060653934));
#215512=CARTESIAN_POINT('Ctrl Pts',(5.06523037499995,11.6,10.060653934));
#215513=CARTESIAN_POINT('Ctrl Pts',(5.06254749499995,15.2,10.058411619));
#215514=CARTESIAN_POINT('Ctrl Pts',(5.06254749499995,11.6,10.058411619));
#215515=CARTESIAN_POINT('Ctrl Pts',(5.05987001799994,15.2,10.056170261));
#215516=CARTESIAN_POINT('Ctrl Pts',(5.05987001799994,11.6,10.056170261));
#215517=CARTESIAN_POINT('Ctrl Pts',(5.05719794699994,15.2,10.053929868));
#215518=CARTESIAN_POINT('Ctrl Pts',(5.05719794699994,11.6,10.053929868));
#215519=CARTESIAN_POINT('Ctrl Pts',(5.05453128299994,15.2,10.051690451));
#215520=CARTESIAN_POINT('Ctrl Pts',(5.05453128299994,11.6,10.051690451));
#215521=CARTESIAN_POINT('Ctrl Pts',(5.05187002799994,15.2,10.04945202));
#215522=CARTESIAN_POINT('Ctrl Pts',(5.05187002799994,11.6,10.04945202));
#215523=CARTESIAN_POINT('Ctrl Pts',(5.04921418499994,15.2,10.047214586));
#215524=CARTESIAN_POINT('Ctrl Pts',(5.04921418499994,11.6,10.047214586));
#215525=CARTESIAN_POINT('Ctrl Pts',(5.04656375499994,15.2,10.044978156));
#215526=CARTESIAN_POINT('Ctrl Pts',(5.04656375499994,11.6,10.044978156));
#215527=CARTESIAN_POINT('Ctrl Pts',(5.04391874099994,15.2,10.042742743));
#215528=CARTESIAN_POINT('Ctrl Pts',(5.04391874099994,11.6,10.042742743));
#215529=CARTESIAN_POINT('Ctrl Pts',(5.04127914399994,15.2,10.040508354));
#215530=CARTESIAN_POINT('Ctrl Pts',(5.04127914399994,11.6,10.040508354));
#215531=CARTESIAN_POINT('Ctrl Pts',(5.03864496599994,15.2,10.038275002));
#215532=CARTESIAN_POINT('Ctrl Pts',(5.03864496599994,11.6,10.038275002));
#215533=CARTESIAN_POINT('Ctrl Pts',(5.03601620899994,15.2,10.036042695));
#215534=CARTESIAN_POINT('Ctrl Pts',(5.03601620899994,11.6,10.036042695));
#215535=CARTESIAN_POINT('Ctrl Pts',(5.03339287499994,15.2,10.033811443));
#215536=CARTESIAN_POINT('Ctrl Pts',(5.03339287499994,11.6,10.033811443));
#215537=CARTESIAN_POINT('Ctrl Pts',(5.03077496799994,15.2,10.031581256));
#215538=CARTESIAN_POINT('Ctrl Pts',(5.03077496799994,11.6,10.031581256));
#215539=CARTESIAN_POINT('Ctrl Pts',(5.02816248699994,15.2,10.029352145));
#215540=CARTESIAN_POINT('Ctrl Pts',(5.02816248699994,11.6,10.029352145));
#215541=CARTESIAN_POINT('Ctrl Pts',(5.02555543499994,15.2,10.027124119));
#215542=CARTESIAN_POINT('Ctrl Pts',(5.02555543499994,11.6,10.027124119));
#215543=CARTESIAN_POINT('Ctrl Pts',(5.02295381499994,15.2,10.024897189));
#215544=CARTESIAN_POINT('Ctrl Pts',(5.02295381499994,11.6,10.024897189));
#215545=CARTESIAN_POINT('Ctrl Pts',(5.02035762799994,15.2,10.022671365));
#215546=CARTESIAN_POINT('Ctrl Pts',(5.02035762799994,11.6,10.022671365));
#215547=CARTESIAN_POINT('Ctrl Pts',(5.01776687499994,15.2,10.020446656));
#215548=CARTESIAN_POINT('Ctrl Pts',(5.01776687499994,11.6,10.020446656));
#215549=CARTESIAN_POINT('Ctrl Pts',(5.01518155999994,15.2,10.018223073));
#215550=CARTESIAN_POINT('Ctrl Pts',(5.01518155999994,11.6,10.018223073));
#215551=CARTESIAN_POINT('Ctrl Pts',(5.01260168399994,15.2,10.016000626));
#215552=CARTESIAN_POINT('Ctrl Pts',(5.01260168399994,11.6,10.016000626));
#215553=CARTESIAN_POINT('Ctrl Pts',(5.01002724899994,15.2,10.013779325));
#215554=CARTESIAN_POINT('Ctrl Pts',(5.01002724899994,11.6,10.013779325));
#215555=CARTESIAN_POINT('Ctrl Pts',(5.00745825699994,15.2,10.011559181));
#215556=CARTESIAN_POINT('Ctrl Pts',(5.00745825699994,11.6,10.011559181));
#215557=CARTESIAN_POINT('Ctrl Pts',(5.00489470899994,15.2,10.009340204));
#215558=CARTESIAN_POINT('Ctrl Pts',(5.00489470899994,11.6,10.009340204));
#215559=CARTESIAN_POINT('Ctrl Pts',(5.00233660699994,15.2,10.007122403));
#215560=CARTESIAN_POINT('Ctrl Pts',(5.00233660699994,11.6,10.007122403));
#215561=CARTESIAN_POINT('Ctrl Pts',(4.99978395499994,15.2,10.00490579));
#215562=CARTESIAN_POINT('Ctrl Pts',(4.99978395499994,11.6,10.00490579));
#215563=CARTESIAN_POINT('Ctrl Pts',(4.99723675399994,15.2,10.002690374));
#215564=CARTESIAN_POINT('Ctrl Pts',(4.99723675399994,11.6,10.002690374));
#215565=CARTESIAN_POINT('Ctrl Pts',(4.99469500299994,15.2,10.000476165));
#215566=CARTESIAN_POINT('Ctrl Pts',(4.99469500299994,11.6,10.000476165));
#215567=CARTESIAN_POINT('Ctrl Pts',(4.99215870799994,15.2,9.99826317399998));
#215568=CARTESIAN_POINT('Ctrl Pts',(4.99215870799994,11.6,9.99826317399998));
#215569=CARTESIAN_POINT('Ctrl Pts',(4.98962786999994,15.2,9.99605141199999));
#215570=CARTESIAN_POINT('Ctrl Pts',(4.98962786999994,11.6,9.99605141199999));
#215571=CARTESIAN_POINT('Ctrl Pts',(4.98710248999994,15.2,9.99384088899999));
#215572=CARTESIAN_POINT('Ctrl Pts',(4.98710248999994,11.6,9.99384088899999));
#215573=CARTESIAN_POINT('Ctrl Pts',(4.98458256799994,15.2,9.99163161499999));
#215574=CARTESIAN_POINT('Ctrl Pts',(4.98458256799994,11.6,9.99163161499999));
#215575=CARTESIAN_POINT('Ctrl Pts',(4.98206810999994,15.2,9.98942359999998));
#215576=CARTESIAN_POINT('Ctrl Pts',(4.98206810999994,11.6,9.98942359999998));
#215577=CARTESIAN_POINT('Ctrl Pts',(4.97955911499994,15.2,9.98721685499999));
#215578=CARTESIAN_POINT('Ctrl Pts',(4.97955911499994,11.6,9.98721685499999));
#215579=CARTESIAN_POINT('Ctrl Pts',(4.97705558599994,15.2,9.98501139099999));
#215580=CARTESIAN_POINT('Ctrl Pts',(4.97705558599994,11.6,9.98501139099999));
#215581=CARTESIAN_POINT('Ctrl Pts',(4.97455752499994,15.2,9.98280721799999));
#215582=CARTESIAN_POINT('Ctrl Pts',(4.97455752499994,11.6,9.98280721799999));
#215583=CARTESIAN_POINT('Ctrl Pts',(4.97206493199994,15.2,9.98060434499998));
#215584=CARTESIAN_POINT('Ctrl Pts',(4.97206493199994,11.6,9.98060434499998));
#215585=CARTESIAN_POINT('Ctrl Pts',(4.96957781099994,15.2,9.97840278399998));
#215586=CARTESIAN_POINT('Ctrl Pts',(4.96957781099994,11.6,9.97840278399998));
#215587=CARTESIAN_POINT('Ctrl Pts',(4.96709616399994,15.2,9.97620254699999));
#215588=CARTESIAN_POINT('Ctrl Pts',(4.96709616399994,11.6,9.97620254699999));
#215589=CARTESIAN_POINT('Ctrl Pts',(4.96461999099994,15.2,9.97400364199999));
#215590=CARTESIAN_POINT('Ctrl Pts',(4.96461999099994,11.6,9.97400364199999));
#215591=CARTESIAN_POINT('Ctrl Pts',(4.96214929499994,15.2,9.97180608099999));
#215592=CARTESIAN_POINT('Ctrl Pts',(4.96214929499994,11.6,9.97180608099999));
#215593=CARTESIAN_POINT('Ctrl Pts',(4.95968407799994,15.2,9.96960987399999));
#215594=CARTESIAN_POINT('Ctrl Pts',(4.95968407799994,11.6,9.96960987399999));
#215595=CARTESIAN_POINT('Ctrl Pts',(4.95722434099994,15.2,9.96741503199999));
#215596=CARTESIAN_POINT('Ctrl Pts',(4.95722434099994,11.6,9.96741503199999));
#215597=CARTESIAN_POINT('Ctrl Pts',(4.95477008699994,15.2,9.96522156599998));
#215598=CARTESIAN_POINT('Ctrl Pts',(4.95477008699994,11.6,9.96522156599998));
#215599=CARTESIAN_POINT('Ctrl Pts',(4.95232131799995,15.2,9.96302948599999));
#215600=CARTESIAN_POINT('Ctrl Pts',(4.95232131799995,11.6,9.96302948599999));
#215601=CARTESIAN_POINT('Ctrl Pts',(4.94987803399994,15.2,9.96083880199999));
#215602=CARTESIAN_POINT('Ctrl Pts',(4.94987803399994,11.6,9.96083880199999));
#215603=CARTESIAN_POINT('Ctrl Pts',(4.94744023799994,15.2,9.95864952599998));
#215604=CARTESIAN_POINT('Ctrl Pts',(4.94744023799994,11.6,9.95864952599998));
#215605=CARTESIAN_POINT('Ctrl Pts',(4.94500793199994,15.2,9.95646166799999));
#215606=CARTESIAN_POINT('Ctrl Pts',(4.94500793199994,11.6,9.95646166799999));
#215607=CARTESIAN_POINT('Ctrl Pts',(4.94258111699994,15.2,9.95427523999999));
#215608=CARTESIAN_POINT('Ctrl Pts',(4.94258111699994,11.6,9.95427523999999));
#215609=CARTESIAN_POINT('Ctrl Pts',(4.94015979599994,15.2,9.95209025199999));
#215610=CARTESIAN_POINT('Ctrl Pts',(4.94015979599994,11.6,9.95209025199999));
#215611=CARTESIAN_POINT('Ctrl Pts',(4.93774396999994,15.2,9.94990671399999));
#215612=CARTESIAN_POINT('Ctrl Pts',(4.93774396999994,11.6,9.94990671399999));
#215613=CARTESIAN_POINT('Ctrl Pts',(4.93533364099994,15.2,9.94772463799999));
#215614=CARTESIAN_POINT('Ctrl Pts',(4.93533364099994,11.6,9.94772463799999));
#215615=CARTESIAN_POINT('Ctrl Pts',(4.93292880999994,15.2,9.94554403399999));
#215616=CARTESIAN_POINT('Ctrl Pts',(4.93292880999994,11.6,9.94554403399999));
#215617=CARTESIAN_POINT('Ctrl Pts',(4.93052947999994,15.2,9.94336491299999));
#215618=CARTESIAN_POINT('Ctrl Pts',(4.93052947999994,11.6,9.94336491299999));
#215619=CARTESIAN_POINT('Ctrl Pts',(4.92813565299994,15.2,9.94118728699998));
#215620=CARTESIAN_POINT('Ctrl Pts',(4.92813565299994,11.6,9.94118728699998));
#215621=CARTESIAN_POINT('Ctrl Pts',(4.92574732899994,15.2,9.93901116599999));
#215622=CARTESIAN_POINT('Ctrl Pts',(4.92574732899994,11.6,9.93901116599999));
#215623=CARTESIAN_POINT('Ctrl Pts',(4.92336451099994,15.2,9.93683656199998));
#215624=CARTESIAN_POINT('Ctrl Pts',(4.92336451099994,11.6,9.93683656199998));
#215625=CARTESIAN_POINT('Ctrl Pts',(4.92098720099994,15.2,9.93466348399998));
#215626=CARTESIAN_POINT('Ctrl Pts',(4.92098720099994,11.6,9.93466348399998));
#215627=CARTESIAN_POINT('Ctrl Pts',(4.91861540099994,15.2,9.93249194499998));
#215628=CARTESIAN_POINT('Ctrl Pts',(4.91861540099994,11.6,9.93249194499998));
#215629=CARTESIAN_POINT('Ctrl Pts',(4.91624911099994,15.2,9.93032195499998));
#215630=CARTESIAN_POINT('Ctrl Pts',(4.91624911099994,11.6,9.93032195499998));
#215631=CARTESIAN_POINT('Ctrl Pts',(4.91388833399994,15.2,9.92815352399998));
#215632=CARTESIAN_POINT('Ctrl Pts',(4.91388833399994,11.6,9.92815352399998));
#215633=CARTESIAN_POINT('Ctrl Pts',(4.91153307199994,15.2,9.92598666599999));
#215634=CARTESIAN_POINT('Ctrl Pts',(4.91153307199994,11.6,9.92598666599999));
#215635=CARTESIAN_POINT('Ctrl Pts',(4.90918332699994,15.2,9.92382138899998));
#215636=CARTESIAN_POINT('Ctrl Pts',(4.90918332699994,11.6,9.92382138899998));
#215637=CARTESIAN_POINT('Ctrl Pts',(4.90683909899994,15.2,9.92165770599998));
#215638=CARTESIAN_POINT('Ctrl Pts',(4.90683909899994,11.6,9.92165770599998));
#215639=CARTESIAN_POINT('Ctrl Pts',(4.90450039099994,15.2,9.91949562899999));
#215640=CARTESIAN_POINT('Ctrl Pts',(4.90450039099994,11.6,9.91949562899999));
#215641=CARTESIAN_POINT('Ctrl Pts',(4.90216720599994,15.2,9.91733516599999));
#215642=CARTESIAN_POINT('Ctrl Pts',(4.90216720599994,11.6,9.91733516599999));
#215643=CARTESIAN_POINT('Ctrl Pts',(4.89983954199994,15.2,9.91517633099999));
#215644=CARTESIAN_POINT('Ctrl Pts',(4.89983954199994,11.6,9.91517633099999));
#215645=CARTESIAN_POINT('Ctrl Pts',(4.89751740499994,15.2,9.91301913399998));
#215646=CARTESIAN_POINT('Ctrl Pts',(4.89751740499994,11.6,9.91301913399998));
#215647=CARTESIAN_POINT('Ctrl Pts',(4.89520079399994,15.2,9.91086358699998));
#215648=CARTESIAN_POINT('Ctrl Pts',(4.89520079399994,11.6,9.91086358699998));
#215649=CARTESIAN_POINT('Ctrl Pts',(4.89288971099994,15.2,9.90870969999998));
#215650=CARTESIAN_POINT('Ctrl Pts',(4.89288971099994,11.6,9.90870969999998));
#215651=CARTESIAN_POINT('Ctrl Pts',(4.89058415899994,15.2,9.90655748699999));
#215652=CARTESIAN_POINT('Ctrl Pts',(4.89058415899994,11.6,9.90655748699999));
#215653=CARTESIAN_POINT('Ctrl Pts',(4.88828413899994,15.2,9.90440695499998));
#215654=CARTESIAN_POINT('Ctrl Pts',(4.88828413899994,11.6,9.90440695499998));
#215655=CARTESIAN_POINT('Ctrl Pts',(4.88598965099994,15.2,9.90225811999998));
#215656=CARTESIAN_POINT('Ctrl Pts',(4.88598965099994,11.6,9.90225811999998));
#215657=CARTESIAN_POINT('Ctrl Pts',(4.88370069999994,15.2,9.90011098999998));
#215658=CARTESIAN_POINT('Ctrl Pts',(4.88370069999994,11.6,9.90011098999998));
#215659=CARTESIAN_POINT('Ctrl Pts',(4.88141728599994,15.2,9.89796557799998));
#215660=CARTESIAN_POINT('Ctrl Pts',(4.88141728599994,11.6,9.89796557799998));
#215661=CARTESIAN_POINT('Ctrl Pts',(4.87913940899994,15.2,9.89582189499998));
#215662=CARTESIAN_POINT('Ctrl Pts',(4.87913940899994,11.6,9.89582189499998));
#215663=CARTESIAN_POINT('Ctrl Pts',(4.87686707299994,15.2,9.89367995299999));
#215664=CARTESIAN_POINT('Ctrl Pts',(4.87686707299994,11.6,9.89367995299999));
#215665=CARTESIAN_POINT('Ctrl Pts',(4.87460027899994,15.2,9.89153976199999));
#215666=CARTESIAN_POINT('Ctrl Pts',(4.87460027899994,11.6,9.89153976199999));
#215667=CARTESIAN_POINT('Ctrl Pts',(4.87233902799994,15.2,9.88940133499998));
#215668=CARTESIAN_POINT('Ctrl Pts',(4.87233902799994,11.6,9.88940133499998));
#215669=CARTESIAN_POINT('Ctrl Pts',(4.87008332399994,15.2,9.88726468299999));
#215670=CARTESIAN_POINT('Ctrl Pts',(4.87008332399994,11.6,9.88726468299999));
#215671=CARTESIAN_POINT('Ctrl Pts',(4.86783316499994,15.2,9.88512981799998));
#215672=CARTESIAN_POINT('Ctrl Pts',(4.86783316499994,11.6,9.88512981799998));
#215673=CARTESIAN_POINT('Ctrl Pts',(4.86558855599994,15.2,9.88299675099999));
#215674=CARTESIAN_POINT('Ctrl Pts',(4.86558855599994,11.6,9.88299675099999));
#215675=CARTESIAN_POINT('Ctrl Pts',(4.86334949599994,15.2,9.88086549299998));
#215676=CARTESIAN_POINT('Ctrl Pts',(4.86334949599994,11.6,9.88086549299998));
#215677=CARTESIAN_POINT('Ctrl Pts',(4.86111598899994,15.2,9.87873605699999));
#215678=CARTESIAN_POINT('Ctrl Pts',(4.86111598899994,11.6,9.87873605699999));
#215679=CARTESIAN_POINT('Ctrl Pts',(4.85888803499994,15.2,9.87660845499999));
#215680=CARTESIAN_POINT('Ctrl Pts',(4.85888803499994,11.6,9.87660845499999));
#215681=CARTESIAN_POINT('Ctrl Pts',(4.85666563599994,15.2,9.87448269699998));
#215682=CARTESIAN_POINT('Ctrl Pts',(4.85666563599994,11.6,9.87448269699998));
#215683=CARTESIAN_POINT('Ctrl Pts',(4.85444879299994,15.2,9.87235879599999));
#215684=CARTESIAN_POINT('Ctrl Pts',(4.85444879299994,11.6,9.87235879599999));
#215685=CARTESIAN_POINT('Ctrl Pts',(4.85223750899994,15.2,9.87023676299999));
#215686=CARTESIAN_POINT('Ctrl Pts',(4.85223750899994,11.6,9.87023676299999));
#215687=CARTESIAN_POINT('Ctrl Pts',(4.85003178499994,15.2,9.86811660999999));
#215688=CARTESIAN_POINT('Ctrl Pts',(4.85003178499994,11.6,9.86811660999999));
#215689=CARTESIAN_POINT('Ctrl Pts',(4.84783162099994,15.2,9.86599834899998));
#215690=CARTESIAN_POINT('Ctrl Pts',(4.84783162099994,11.6,9.86599834899998));
#215691=CARTESIAN_POINT('Ctrl Pts',(4.84563702199994,15.2,9.86388199099999));
#215692=CARTESIAN_POINT('Ctrl Pts',(4.84563702199994,11.6,9.86388199099999));
#215693=CARTESIAN_POINT('Ctrl Pts',(4.84344798699994,15.2,9.86176754899999));
#215694=CARTESIAN_POINT('Ctrl Pts',(4.84344798699994,11.6,9.86176754899999));
#215695=CARTESIAN_POINT('Ctrl Pts',(4.84126451799994,15.2,9.85965503499998));
#215696=CARTESIAN_POINT('Ctrl Pts',(4.84126451799994,11.6,9.85965503499998));
#215697=CARTESIAN_POINT('Ctrl Pts',(4.83908661699994,15.2,9.85754446099998));
#215698=CARTESIAN_POINT('Ctrl Pts',(4.83908661699994,11.6,9.85754446099998));
#215699=CARTESIAN_POINT('Ctrl Pts',(4.83691428499994,15.2,9.85543583699998));
#215700=CARTESIAN_POINT('Ctrl Pts',(4.83691428499994,11.6,9.85543583699998));
#215701=CARTESIAN_POINT('Ctrl Pts',(4.83474752499994,15.2,9.85332917699999));
#215702=CARTESIAN_POINT('Ctrl Pts',(4.83474752499994,11.6,9.85332917699999));
#215703=CARTESIAN_POINT('Ctrl Pts',(4.83258633699994,15.2,9.85122449099999));
#215704=CARTESIAN_POINT('Ctrl Pts',(4.83258633699994,11.6,9.85122449099999));
#215705=CARTESIAN_POINT('Ctrl Pts',(4.83043072399994,15.2,9.84912179399998));
#215706=CARTESIAN_POINT('Ctrl Pts',(4.83043072399994,11.6,9.84912179399998));
#215707=CARTESIAN_POINT('Ctrl Pts',(4.82828068499994,15.2,9.84702109599999));
#215708=CARTESIAN_POINT('Ctrl Pts',(4.82828068499994,11.6,9.84702109599999));
#215709=CARTESIAN_POINT('Ctrl Pts',(4.82613622399994,15.2,9.84492240899998));
#215710=CARTESIAN_POINT('Ctrl Pts',(4.82613622399994,11.6,9.84492240899998));
#215711=CARTESIAN_POINT('Ctrl Pts',(4.82399734199994,15.2,9.84282574499998));
#215712=CARTESIAN_POINT('Ctrl Pts',(4.82399734199994,11.6,9.84282574499998));
#215713=CARTESIAN_POINT('Ctrl Pts',(4.82186403999994,15.2,9.84073111799999));
#215714=CARTESIAN_POINT('Ctrl Pts',(4.82186403999994,11.6,9.84073111799999));
#215715=CARTESIAN_POINT('Ctrl Pts',(4.81973631899994,15.2,9.83863853799999));
#215716=CARTESIAN_POINT('Ctrl Pts',(4.81973631899994,11.6,9.83863853799999));
#215717=CARTESIAN_POINT('Ctrl Pts',(4.81761418199994,15.2,9.83654801799998));
#215718=CARTESIAN_POINT('Ctrl Pts',(4.81761418199994,11.6,9.83654801799998));
#215719=CARTESIAN_POINT('Ctrl Pts',(4.81549763099994,15.2,9.83445957099999));
#215720=CARTESIAN_POINT('Ctrl Pts',(4.81549763099994,11.6,9.83445957099999));
#215721=CARTESIAN_POINT('Ctrl Pts',(4.81338666499994,15.2,9.83237320799999));
#215722=CARTESIAN_POINT('Ctrl Pts',(4.81338666499994,11.6,9.83237320799999));
#215723=CARTESIAN_POINT('Ctrl Pts',(4.81128128599994,15.2,9.83028894199999));
#215724=CARTESIAN_POINT('Ctrl Pts',(4.81128128599994,11.6,9.83028894199999));
#215725=CARTESIAN_POINT('Ctrl Pts',(4.80918149799994,15.2,9.82820678499999));
#215726=CARTESIAN_POINT('Ctrl Pts',(4.80918149799994,11.6,9.82820678499999));
#215727=CARTESIAN_POINT('Ctrl Pts',(4.80708729999994,15.2,9.82612674999999));
#215728=CARTESIAN_POINT('Ctrl Pts',(4.80708729999994,11.6,9.82612674999999));
#215729=CARTESIAN_POINT('Ctrl Pts',(4.80499869399994,15.2,9.82404884799998));
#215730=CARTESIAN_POINT('Ctrl Pts',(4.80499869399994,11.6,9.82404884799998));
#215731=CARTESIAN_POINT('Ctrl Pts',(4.80291568299994,15.2,9.82197309199999));
#215732=CARTESIAN_POINT('Ctrl Pts',(4.80291568299994,11.6,9.82197309199999));
#215733=CARTESIAN_POINT('Ctrl Pts',(4.80083826599994,15.2,9.81989949599999));
#215734=CARTESIAN_POINT('Ctrl Pts',(4.80083826599994,11.6,9.81989949599999));
#215735=CARTESIAN_POINT('Ctrl Pts',(4.79876644599994,15.2,9.81782807099999));
#215736=CARTESIAN_POINT('Ctrl Pts',(4.79876644599994,11.6,9.81782807099999));
#215737=CARTESIAN_POINT('Ctrl Pts',(4.79670022499994,15.2,9.81575882899998));
#215738=CARTESIAN_POINT('Ctrl Pts',(4.79670022499994,11.6,9.81575882899998));
#215739=CARTESIAN_POINT('Ctrl Pts',(4.79463960199994,15.2,9.81369178299998));
#215740=CARTESIAN_POINT('Ctrl Pts',(4.79463960199994,11.6,9.81369178299998));
#215741=CARTESIAN_POINT('Ctrl Pts',(4.79258458199994,15.2,9.81162694599998));
#215742=CARTESIAN_POINT('Ctrl Pts',(4.79258458199994,11.6,9.81162694599998));
#215743=CARTESIAN_POINT('Ctrl Pts',(4.79053516299994,15.2,9.80956433099998));
#215744=CARTESIAN_POINT('Ctrl Pts',(4.79053516299994,11.6,9.80956433099998));
#215745=CARTESIAN_POINT('Ctrl Pts',(4.78849134899994,15.2,9.80750394899999));
#215746=CARTESIAN_POINT('Ctrl Pts',(4.78849134899994,11.6,9.80750394899999));
#215747=CARTESIAN_POINT('Ctrl Pts',(4.78645313999994,15.2,9.80544581399998));
#215748=CARTESIAN_POINT('Ctrl Pts',(4.78645313999994,11.6,9.80544581399998));
#215749=CARTESIAN_POINT('Ctrl Pts',(4.78442053799994,15.2,9.80338993799998));
#215750=CARTESIAN_POINT('Ctrl Pts',(4.78442053799994,11.6,9.80338993799998));
#215751=CARTESIAN_POINT('Ctrl Pts',(4.78239354399994,15.2,9.80133633399999));
#215752=CARTESIAN_POINT('Ctrl Pts',(4.78239354399994,11.6,9.80133633399999));
#215753=CARTESIAN_POINT('Ctrl Pts',(4.78037215899994,15.2,9.79928501499998));
#215754=CARTESIAN_POINT('Ctrl Pts',(4.78037215899994,11.6,9.79928501499998));
#215755=CARTESIAN_POINT('Ctrl Pts',(4.77835638599994,15.2,9.79723599399998));
#215756=CARTESIAN_POINT('Ctrl Pts',(4.77835638599994,11.6,9.79723599399998));
#215757=CARTESIAN_POINT('Ctrl Pts',(4.77634622499994,15.2,9.79518928099999));
#215758=CARTESIAN_POINT('Ctrl Pts',(4.77634622499994,11.6,9.79518928099999));
#215759=CARTESIAN_POINT('Ctrl Pts',(4.77434167799994,15.2,9.79314489299998));
#215760=CARTESIAN_POINT('Ctrl Pts',(4.77434167799994,11.6,9.79314489299998));
#215761=CARTESIAN_POINT('Ctrl Pts',(4.77234274699994,15.2,9.79110284099999));
#215762=CARTESIAN_POINT('Ctrl Pts',(4.77234274699994,11.6,9.79110284099999));
#215763=CARTESIAN_POINT('Ctrl Pts',(4.77034943099994,15.2,9.78906313699999));
#215764=CARTESIAN_POINT('Ctrl Pts',(4.77034943099994,11.6,9.78906313699999));
#215765=CARTESIAN_POINT('Ctrl Pts',(4.76836173399994,15.2,9.78702579499998));
#215766=CARTESIAN_POINT('Ctrl Pts',(4.76836173399994,11.6,9.78702579499998));
#215767=CARTESIAN_POINT('Ctrl Pts',(4.76637965599994,15.2,9.78499082799999));
#215768=CARTESIAN_POINT('Ctrl Pts',(4.76637965599994,11.6,9.78499082799999));
#215769=CARTESIAN_POINT('Ctrl Pts',(4.76440319899994,15.2,9.78295824899998));
#215770=CARTESIAN_POINT('Ctrl Pts',(4.76440319899994,11.6,9.78295824899998));
#215771=CARTESIAN_POINT('Ctrl Pts',(4.76243236299994,15.2,9.78092806999998));
#215772=CARTESIAN_POINT('Ctrl Pts',(4.76243236299994,11.6,9.78092806999998));
#215773=CARTESIAN_POINT('Ctrl Pts',(4.76046715199994,15.2,9.77890030499999));
#215774=CARTESIAN_POINT('Ctrl Pts',(4.76046715199994,11.6,9.77890030499999));
#215775=CARTESIAN_POINT('Ctrl Pts',(4.75850756399994,15.2,9.77687496799999));
#215776=CARTESIAN_POINT('Ctrl Pts',(4.75850756399994,11.6,9.77687496799999));
#215777=CARTESIAN_POINT('Ctrl Pts',(4.75655360399994,15.2,9.77485206899999));
#215778=CARTESIAN_POINT('Ctrl Pts',(4.75655360399994,11.6,9.77485206899999));
#215779=CARTESIAN_POINT('Ctrl Pts',(4.75460526999994,15.2,9.77283162499998));
#215780=CARTESIAN_POINT('Ctrl Pts',(4.75460526999994,11.6,9.77283162499998));
#215781=CARTESIAN_POINT('Ctrl Pts',(4.75266256599994,15.2,9.77081364599999));
#215782=CARTESIAN_POINT('Ctrl Pts',(4.75266256599994,11.6,9.77081364599999));
#215783=CARTESIAN_POINT('Ctrl Pts',(4.75072549099994,15.2,9.76879814799998));
#215784=CARTESIAN_POINT('Ctrl Pts',(4.75072549099994,11.6,9.76879814799998));
#215785=CARTESIAN_POINT('Ctrl Pts',(4.74879404699994,15.2,9.76678514099999));
#215786=CARTESIAN_POINT('Ctrl Pts',(4.74879404699994,11.6,9.76678514099999));
#215787=CARTESIAN_POINT('Ctrl Pts',(4.74686823599995,15.2,9.76477464199998));
#215788=CARTESIAN_POINT('Ctrl Pts',(4.74686823599995,11.6,9.76477464199998));
#215789=CARTESIAN_POINT('Ctrl Pts',(4.74494805999994,15.2,9.76276666099999));
#215790=CARTESIAN_POINT('Ctrl Pts',(4.74494805999994,11.6,9.76276666099999));
#215791=CARTESIAN_POINT('Ctrl Pts',(4.74303351799994,15.2,9.76076121399998));
#215792=CARTESIAN_POINT('Ctrl Pts',(4.74303351799994,11.6,9.76076121399998));
#215793=CARTESIAN_POINT('Ctrl Pts',(4.74112461299994,15.2,9.75875831199998));
#215794=CARTESIAN_POINT('Ctrl Pts',(4.74112461299994,11.6,9.75875831199998));
#215795=CARTESIAN_POINT('Ctrl Pts',(4.73922134499994,15.2,9.75675797099999));
#215796=CARTESIAN_POINT('Ctrl Pts',(4.73922134499994,11.6,9.75675797099999));
#215797=CARTESIAN_POINT('Ctrl Pts',(4.73732371699994,15.2,9.75476020199999));
#215798=CARTESIAN_POINT('Ctrl Pts',(4.73732371699994,11.6,9.75476020199999));
#215799=CARTESIAN_POINT('Ctrl Pts',(4.73543172899995,15.2,9.75276501999998));
#215800=CARTESIAN_POINT('Ctrl Pts',(4.73543172899995,11.6,9.75276501999998));
#215801=CARTESIAN_POINT('Ctrl Pts',(4.73354538299994,15.2,9.75077243799999));
#215802=CARTESIAN_POINT('Ctrl Pts',(4.73354538299994,11.6,9.75077243799999));
#215803=CARTESIAN_POINT('Ctrl Pts',(4.73166467999994,15.2,9.74878246999998));
#215804=CARTESIAN_POINT('Ctrl Pts',(4.73166467999994,11.6,9.74878246999998));
#215805=CARTESIAN_POINT('Ctrl Pts',(4.72978961999994,15.2,9.74679512799998));
#215806=CARTESIAN_POINT('Ctrl Pts',(4.72978961999994,11.6,9.74679512799998));
#215807=CARTESIAN_POINT('Ctrl Pts',(4.72792020499994,15.2,9.74481042899999));
#215808=CARTESIAN_POINT('Ctrl Pts',(4.72792020499994,11.6,9.74481042899999));
#215809=CARTESIAN_POINT('Ctrl Pts',(4.72605643799994,15.2,9.74282838299998));
#215810=CARTESIAN_POINT('Ctrl Pts',(4.72605643799994,11.6,9.74282838299998));
#215811=CARTESIAN_POINT('Ctrl Pts',(4.72419831899995,15.2,9.74084900499999));
#215812=CARTESIAN_POINT('Ctrl Pts',(4.72419831899995,11.6,9.74084900499999));
#215813=CARTESIAN_POINT('Ctrl Pts',(4.72234584699994,15.2,9.73887231099998));
#215814=CARTESIAN_POINT('Ctrl Pts',(4.72234584699994,11.6,9.73887231099998));
#215815=CARTESIAN_POINT('Ctrl Pts',(4.72049902599994,15.2,9.73689831099998));
#215816=CARTESIAN_POINT('Ctrl Pts',(4.72049902599994,11.6,9.73689831099998));
#215817=CARTESIAN_POINT('Ctrl Pts',(4.71865785699994,15.2,9.73492701999999));
#215818=CARTESIAN_POINT('Ctrl Pts',(4.71865785699994,11.6,9.73492701999999));
#215819=CARTESIAN_POINT('Ctrl Pts',(4.71682233899994,15.2,9.73295845299998));
#215820=CARTESIAN_POINT('Ctrl Pts',(4.71682233899994,11.6,9.73295845299998));
#215821=CARTESIAN_POINT('Ctrl Pts',(4.71499247599994,15.2,9.73099262399998));
#215822=CARTESIAN_POINT('Ctrl Pts',(4.71499247599994,11.6,9.73099262399998));
#215823=CARTESIAN_POINT('Ctrl Pts',(4.71316826799994,15.2,9.72902954599999));
#215824=CARTESIAN_POINT('Ctrl Pts',(4.71316826799994,11.6,9.72902954599999));
#215825=CARTESIAN_POINT('Ctrl Pts',(4.71134971599994,15.2,9.72706923299998));
#215826=CARTESIAN_POINT('Ctrl Pts',(4.71134971599994,11.6,9.72706923299998));
#215827=CARTESIAN_POINT('Ctrl Pts',(4.70953681999994,15.2,9.72511169999999));
#215828=CARTESIAN_POINT('Ctrl Pts',(4.70953681999994,11.6,9.72511169999999));
#215829=CARTESIAN_POINT('Ctrl Pts',(4.70772958299994,15.2,9.72315695899999));
#215830=CARTESIAN_POINT('Ctrl Pts',(4.70772958299994,11.6,9.72315695899999));
#215831=CARTESIAN_POINT('Ctrl Pts',(4.70592800699994,15.2,9.72120502599999));
#215832=CARTESIAN_POINT('Ctrl Pts',(4.70592800699994,11.6,9.72120502599999));
#215833=CARTESIAN_POINT('Ctrl Pts',(4.70413208999994,15.2,9.71925591399999));
#215834=CARTESIAN_POINT('Ctrl Pts',(4.70413208999994,11.6,9.71925591399999));
#215835=CARTESIAN_POINT('Ctrl Pts',(4.70234183499994,15.2,9.71730963799999));
#215836=CARTESIAN_POINT('Ctrl Pts',(4.70234183499994,11.6,9.71730963799999));
#215837=CARTESIAN_POINT('Ctrl Pts',(4.70055724399994,15.2,9.71536621099998));
#215838=CARTESIAN_POINT('Ctrl Pts',(4.70055724399994,11.6,9.71536621099998));
#215839=CARTESIAN_POINT('Ctrl Pts',(4.69877831599994,15.2,9.71342564899999));
#215840=CARTESIAN_POINT('Ctrl Pts',(4.69877831599994,11.6,9.71342564899999));
#215841=CARTESIAN_POINT('Ctrl Pts',(4.69700505299994,15.2,9.71148796399999));
#215842=CARTESIAN_POINT('Ctrl Pts',(4.69700505299994,11.6,9.71148796399999));
#215843=CARTESIAN_POINT('Ctrl Pts',(4.69523745699994,15.2,9.70955317299998));
#215844=CARTESIAN_POINT('Ctrl Pts',(4.69523745699994,11.6,9.70955317299998));
#215845=CARTESIAN_POINT('Ctrl Pts',(4.69347552899994,15.2,9.70762128699998));
#215846=CARTESIAN_POINT('Ctrl Pts',(4.69347552899994,11.6,9.70762128699998));
#215847=CARTESIAN_POINT('Ctrl Pts',(4.69171926699994,15.2,9.70569232299999));
#215848=CARTESIAN_POINT('Ctrl Pts',(4.69171926699994,11.6,9.70569232299999));
#215849=CARTESIAN_POINT('Ctrl Pts',(4.68996867699994,15.2,9.70376629399999));
#215850=CARTESIAN_POINT('Ctrl Pts',(4.68996867699994,11.6,9.70376629399999));
#215851=CARTESIAN_POINT('Ctrl Pts',(4.68822375699994,15.2,9.70184321599999));
#215852=CARTESIAN_POINT('Ctrl Pts',(4.68822375699994,11.6,9.70184321599999));
#215853=CARTESIAN_POINT('Ctrl Pts',(4.68648450799994,15.2,9.69992310099999));
#215854=CARTESIAN_POINT('Ctrl Pts',(4.68648450799994,11.6,9.69992310099999));
#215855=CARTESIAN_POINT('Ctrl Pts',(4.68475093199994,15.2,9.69800596699999));
#215856=CARTESIAN_POINT('Ctrl Pts',(4.68475093199994,11.6,9.69800596699999));
#215857=CARTESIAN_POINT('Ctrl Pts',(4.68302303099994,15.2,9.69609182599999));
#215858=CARTESIAN_POINT('Ctrl Pts',(4.68302303099994,11.6,9.69609182599999));
#215859=CARTESIAN_POINT('Ctrl Pts',(4.68130080299994,15.2,9.69418069199998));
#215860=CARTESIAN_POINT('Ctrl Pts',(4.68130080299994,11.6,9.69418069199998));
#215861=CARTESIAN_POINT('Ctrl Pts',(4.67958425099994,15.2,9.69227258199999));
#215862=CARTESIAN_POINT('Ctrl Pts',(4.67958425099994,11.6,9.69227258199999));
#215863=CARTESIAN_POINT('Ctrl Pts',(4.67787337699994,15.2,9.69036750899999));
#215864=CARTESIAN_POINT('Ctrl Pts',(4.67787337699994,11.6,9.69036750899999));
#215865=CARTESIAN_POINT('Ctrl Pts',(4.67616818099994,15.2,9.68846548899998));
#215866=CARTESIAN_POINT('Ctrl Pts',(4.67616818099994,11.6,9.68846548899998));
#215867=CARTESIAN_POINT('Ctrl Pts',(4.67446866299994,15.2,9.68656653599999));
#215868=CARTESIAN_POINT('Ctrl Pts',(4.67446866299994,11.6,9.68656653599999));
#215869=CARTESIAN_POINT('Ctrl Pts',(4.67277482599994,15.2,9.68467066399998));
#215870=CARTESIAN_POINT('Ctrl Pts',(4.67277482599994,11.6,9.68467066399998));
#215871=CARTESIAN_POINT('Ctrl Pts',(4.67108666899994,15.2,9.68277788899999));
#215872=CARTESIAN_POINT('Ctrl Pts',(4.67108666899994,11.6,9.68277788899999));
#215873=CARTESIAN_POINT('Ctrl Pts',(4.66940419399994,15.2,9.68088822599999));
#215874=CARTESIAN_POINT('Ctrl Pts',(4.66940419399994,11.6,9.68088822599999));
#215875=CARTESIAN_POINT('Ctrl Pts',(4.66772740199994,15.2,9.67900168899998));
#215876=CARTESIAN_POINT('Ctrl Pts',(4.66772740199994,11.6,9.67900168899998));
#215877=CARTESIAN_POINT('Ctrl Pts',(4.66605629399994,15.2,9.67711829299999));
#215878=CARTESIAN_POINT('Ctrl Pts',(4.66605629399994,11.6,9.67711829299999));
#215879=CARTESIAN_POINT('Ctrl Pts',(4.66439087099994,15.2,9.67523805499999));
#215880=CARTESIAN_POINT('Ctrl Pts',(4.66439087099994,11.6,9.67523805499999));
#215881=CARTESIAN_POINT('Ctrl Pts',(4.66273113299994,15.2,9.67336098699998));
#215882=CARTESIAN_POINT('Ctrl Pts',(4.66273113299994,11.6,9.67336098699998));
#215883=CARTESIAN_POINT('Ctrl Pts',(4.66107708199994,15.2,9.67148710599999));
#215884=CARTESIAN_POINT('Ctrl Pts',(4.66107708199994,11.6,9.67148710599999));
#215885=CARTESIAN_POINT('Ctrl Pts',(4.65942871899994,15.2,9.66961642799999));
#215886=CARTESIAN_POINT('Ctrl Pts',(4.65942871899994,11.6,9.66961642799999));
#215887=CARTESIAN_POINT('Ctrl Pts',(4.65778604399994,15.2,9.66774896599999));
#215888=CARTESIAN_POINT('Ctrl Pts',(4.65778604399994,11.6,9.66774896599999));
#215889=CARTESIAN_POINT('Ctrl Pts',(4.65614905999994,15.2,9.66588473699998));
#215890=CARTESIAN_POINT('Ctrl Pts',(4.65614905999994,11.6,9.66588473699998));
#215891=CARTESIAN_POINT('Ctrl Pts',(4.65451776499994,15.2,9.66402375399999));
#215892=CARTESIAN_POINT('Ctrl Pts',(4.65451776499994,11.6,9.66402375399999));
#215893=CARTESIAN_POINT('Ctrl Pts',(4.65289216199994,15.2,9.66216603499999));
#215894=CARTESIAN_POINT('Ctrl Pts',(4.65289216199994,11.6,9.66216603499999));
#215895=CARTESIAN_POINT('Ctrl Pts',(4.65127225199994,15.2,9.66031159299998));
#215896=CARTESIAN_POINT('Ctrl Pts',(4.65127225199994,11.6,9.66031159299998));
#215897=CARTESIAN_POINT('Ctrl Pts',(4.64965803299994,15.2,9.65846044499998));
#215898=CARTESIAN_POINT('Ctrl Pts',(4.64965803299994,11.6,9.65846044499998));
#215899=CARTESIAN_POINT('Ctrl Pts',(4.64804950999994,15.2,9.65661260499999));
#215900=CARTESIAN_POINT('Ctrl Pts',(4.64804950999994,11.6,9.65661260499999));
#215901=CARTESIAN_POINT('Ctrl Pts',(4.64644668199994,15.2,9.65476809099999));
#215902=CARTESIAN_POINT('Ctrl Pts',(4.64644668199994,11.6,9.65476809099999));
#215903=CARTESIAN_POINT('Ctrl Pts',(4.64484954799994,15.2,9.65292691699998));
#215904=CARTESIAN_POINT('Ctrl Pts',(4.64484954799994,11.6,9.65292691699998));
#215905=CARTESIAN_POINT('Ctrl Pts',(4.64325811199994,15.2,9.65108909799999));
#215906=CARTESIAN_POINT('Ctrl Pts',(4.64325811199994,11.6,9.65108909799999));
#215907=CARTESIAN_POINT('Ctrl Pts',(4.64167237399994,15.2,9.64925464899999));
#215908=CARTESIAN_POINT('Ctrl Pts',(4.64167237399994,11.6,9.64925464899999));
#215909=CARTESIAN_POINT('Ctrl Pts',(4.64009233299994,15.2,9.64742358899999));
#215910=CARTESIAN_POINT('Ctrl Pts',(4.64009233299994,11.6,9.64742358899999));
#215911=CARTESIAN_POINT('Ctrl Pts',(4.63851799199994,15.2,9.64559592999999));
#215912=CARTESIAN_POINT('Ctrl Pts',(4.63851799199994,11.6,9.64559592999999));
#215913=CARTESIAN_POINT('Ctrl Pts',(4.63694935099994,15.2,9.64377168999999));
#215914=CARTESIAN_POINT('Ctrl Pts',(4.63694935099994,11.6,9.64377168999999));
#215915=CARTESIAN_POINT('Ctrl Pts',(4.63538641099994,15.2,9.64195088399999));
#215916=CARTESIAN_POINT('Ctrl Pts',(4.63538641099994,11.6,9.64195088399999));
#215917=CARTESIAN_POINT('Ctrl Pts',(4.63382917099994,15.2,9.64013352699999));
#215918=CARTESIAN_POINT('Ctrl Pts',(4.63382917099994,11.6,9.64013352699999));
#215919=CARTESIAN_POINT('Ctrl Pts',(4.63227763499994,15.2,9.63831963699998));
#215920=CARTESIAN_POINT('Ctrl Pts',(4.63227763499994,11.6,9.63831963699998));
#215921=CARTESIAN_POINT('Ctrl Pts',(4.63073180199994,15.2,9.63650922899999));
#215922=CARTESIAN_POINT('Ctrl Pts',(4.63073180199994,11.6,9.63650922899999));
#215923=CARTESIAN_POINT('Ctrl Pts',(4.62919167299994,15.2,9.63470231799998));
#215924=CARTESIAN_POINT('Ctrl Pts',(4.62919167299994,11.6,9.63470231799998));
#215925=CARTESIAN_POINT('Ctrl Pts',(4.62765724799994,15.2,9.63289892099999));
#215926=CARTESIAN_POINT('Ctrl Pts',(4.62765724799994,11.6,9.63289892099999));
#215927=CARTESIAN_POINT('Ctrl Pts',(4.62612852999994,15.2,9.63109905299999));
#215928=CARTESIAN_POINT('Ctrl Pts',(4.62612852999994,11.6,9.63109905299999));
#215929=CARTESIAN_POINT('Ctrl Pts',(4.62460551699994,15.2,9.62930273299998));
#215930=CARTESIAN_POINT('Ctrl Pts',(4.62460551699994,11.6,9.62930273299998));
#215931=CARTESIAN_POINT('Ctrl Pts',(4.62308821099994,15.2,9.62750997299998));
#215932=CARTESIAN_POINT('Ctrl Pts',(4.62308821099994,11.6,9.62750997299998));
#215933=CARTESIAN_POINT('Ctrl Pts',(4.62157661299994,15.2,9.62572079199998));
#215934=CARTESIAN_POINT('Ctrl Pts',(4.62157661299994,11.6,9.62572079199998));
#215935=CARTESIAN_POINT('Ctrl Pts',(4.62007072299994,15.2,9.62393520599999));
#215936=CARTESIAN_POINT('Ctrl Pts',(4.62007072299994,11.6,9.62393520599999));
#215937=CARTESIAN_POINT('Ctrl Pts',(4.61857054399994,15.2,9.62215323199998));
#215938=CARTESIAN_POINT('Ctrl Pts',(4.61857054399994,11.6,9.62215323199998));
#215939=CARTESIAN_POINT('Ctrl Pts',(4.61707607299994,15.2,9.62037488299998));
#215940=CARTESIAN_POINT('Ctrl Pts',(4.61707607299994,11.6,9.62037488299998));
#215941=CARTESIAN_POINT('Ctrl Pts',(4.61558731299994,15.2,9.61860017899999));
#215942=CARTESIAN_POINT('Ctrl Pts',(4.61558731299994,11.6,9.61860017899999));
#215943=CARTESIAN_POINT('Ctrl Pts',(4.61410426499994,15.2,9.61682913599999));
#215944=CARTESIAN_POINT('Ctrl Pts',(4.61410426499994,11.6,9.61682913599999));
#215945=CARTESIAN_POINT('Ctrl Pts',(4.61262692899994,15.2,9.61506176899999));
#215946=CARTESIAN_POINT('Ctrl Pts',(4.61262692899994,11.6,9.61506176899999));
#215947=CARTESIAN_POINT('Ctrl Pts',(4.61115530499994,15.2,9.61329809499999));
#215948=CARTESIAN_POINT('Ctrl Pts',(4.61115530499994,11.6,9.61329809499999));
#215949=CARTESIAN_POINT('Ctrl Pts',(4.60968939499994,15.2,9.61153813099998));
#215950=CARTESIAN_POINT('Ctrl Pts',(4.60968939499994,11.6,9.61153813099998));
#215951=CARTESIAN_POINT('Ctrl Pts',(4.60822919899994,15.2,9.60978189399999));
#215952=CARTESIAN_POINT('Ctrl Pts',(4.60822919899994,11.6,9.60978189399999));
#215953=CARTESIAN_POINT('Ctrl Pts',(4.60677471599994,15.2,9.60802939999999));
#215954=CARTESIAN_POINT('Ctrl Pts',(4.60677471599994,11.6,9.60802939999999));
#215955=CARTESIAN_POINT('Ctrl Pts',(4.60532594999994,15.2,9.60628066599998));
#215956=CARTESIAN_POINT('Ctrl Pts',(4.60532594999994,11.6,9.60628066599998));
#215957=CARTESIAN_POINT('Ctrl Pts',(4.60388289999994,15.2,9.60453570899999));
#215958=CARTESIAN_POINT('Ctrl Pts',(4.60388289999994,11.6,9.60453570899999));
#215959=CARTESIAN_POINT('Ctrl Pts',(4.60244556499994,15.2,9.60279454499998));
#215960=CARTESIAN_POINT('Ctrl Pts',(4.60244556499994,11.6,9.60279454499998));
#215961=CARTESIAN_POINT('Ctrl Pts',(4.60101394899994,15.2,9.60105719299998));
#215962=CARTESIAN_POINT('Ctrl Pts',(4.60101394899994,11.6,9.60105719299998));
#215963=CARTESIAN_POINT('Ctrl Pts',(4.59958804899994,15.2,9.59932366799999));
#215964=CARTESIAN_POINT('Ctrl Pts',(4.59958804899994,11.6,9.59932366799999));
#215965=CARTESIAN_POINT('Ctrl Pts',(4.59816786799994,15.2,9.59759398699998));
#215966=CARTESIAN_POINT('Ctrl Pts',(4.59816786799994,11.6,9.59759398699998));
#215967=CARTESIAN_POINT('Ctrl Pts',(4.59675340599994,15.2,9.59586816899998));
#215968=CARTESIAN_POINT('Ctrl Pts',(4.59675340599994,11.6,9.59586816899998));
#215969=CARTESIAN_POINT('Ctrl Pts',(4.59534466399994,15.2,9.59414622899999));
#215970=CARTESIAN_POINT('Ctrl Pts',(4.59534466399994,11.6,9.59414622899999));
#215971=CARTESIAN_POINT('Ctrl Pts',(4.59394164099994,15.2,9.59242818499998));
#215972=CARTESIAN_POINT('Ctrl Pts',(4.59394164099994,11.6,9.59242818499998));
#215973=CARTESIAN_POINT('Ctrl Pts',(4.59254433799994,15.2,9.59071405499999));
#215974=CARTESIAN_POINT('Ctrl Pts',(4.59254433799994,11.6,9.59071405499999));
#215975=CARTESIAN_POINT('Ctrl Pts',(4.59115275799994,15.2,9.58900385399998));
#215976=CARTESIAN_POINT('Ctrl Pts',(4.59115275799994,11.6,9.58900385399998));
#215977=CARTESIAN_POINT('Ctrl Pts',(4.58976689799994,15.2,9.58729760299999));
#215978=CARTESIAN_POINT('Ctrl Pts',(4.58976689799994,11.6,9.58729760299999));
#215979=CARTESIAN_POINT('Ctrl Pts',(4.58838676199994,15.2,9.58559531599998));
#215980=CARTESIAN_POINT('Ctrl Pts',(4.58838676199994,11.6,9.58559531599998));
#215981=CARTESIAN_POINT('Ctrl Pts',(4.58701234599994,15.2,9.58389701199999));
#215982=CARTESIAN_POINT('Ctrl Pts',(4.58701234599994,11.6,9.58389701199999));
#215983=CARTESIAN_POINT('Ctrl Pts',(4.58564365499994,15.2,9.58220270799998));
#215984=CARTESIAN_POINT('Ctrl Pts',(4.58564365499994,11.6,9.58220270799998));
#215985=CARTESIAN_POINT('Ctrl Pts',(4.58428068699994,15.2,9.58051242199998));
#215986=CARTESIAN_POINT('Ctrl Pts',(4.58428068699994,11.6,9.58051242199998));
#215987=CARTESIAN_POINT('Ctrl Pts',(4.58292344399994,15.2,9.57882617199999));
#215988=CARTESIAN_POINT('Ctrl Pts',(4.58292344399994,11.6,9.57882617199999));
#215989=CARTESIAN_POINT('Ctrl Pts',(4.58157192499994,15.2,9.57714397399998));
#215990=CARTESIAN_POINT('Ctrl Pts',(4.58157192499994,11.6,9.57714397399998));
#215991=CARTESIAN_POINT('Ctrl Pts',(4.58022613099994,15.2,9.57546584699998));
#215992=CARTESIAN_POINT('Ctrl Pts',(4.58022613099994,11.6,9.57546584699998));
#215993=CARTESIAN_POINT('Ctrl Pts',(4.57888606199994,15.2,9.57379180899999));
#215994=CARTESIAN_POINT('Ctrl Pts',(4.57888606199994,11.6,9.57379180899999));
#215995=CARTESIAN_POINT('Ctrl Pts',(4.57755171999994,15.2,9.57212187799998));
#215996=CARTESIAN_POINT('Ctrl Pts',(4.57755171999994,11.6,9.57212187799998));
#215997=CARTESIAN_POINT('Ctrl Pts',(4.57622310299994,15.2,9.57045607099998));
#215998=CARTESIAN_POINT('Ctrl Pts',(4.57622310299994,11.6,9.57045607099998));
#215999=CARTESIAN_POINT('Ctrl Pts',(4.57490021399994,15.2,9.56879440499998));
#216000=CARTESIAN_POINT('Ctrl Pts',(4.57490021399994,11.6,9.56879440499998));
#216001=CARTESIAN_POINT('Ctrl Pts',(4.57358305099994,15.2,9.56713690099999));
#216002=CARTESIAN_POINT('Ctrl Pts',(4.57358305099994,11.6,9.56713690099999));
#216003=CARTESIAN_POINT('Ctrl Pts',(4.57227161699994,15.2,9.56548357499998));
#216004=CARTESIAN_POINT('Ctrl Pts',(4.57227161699994,11.6,9.56548357499998));
#216005=CARTESIAN_POINT('Ctrl Pts',(4.57096591099994,15.2,9.56383444499998));
#216006=CARTESIAN_POINT('Ctrl Pts',(4.57096591099994,11.6,9.56383444499998));
#216007=CARTESIAN_POINT('Ctrl Pts',(4.56966593299994,15.2,9.56218952999999));
#216008=CARTESIAN_POINT('Ctrl Pts',(4.56966593299994,11.6,9.56218952999999));
#216009=CARTESIAN_POINT('Ctrl Pts',(4.56837168299994,15.2,9.56054884799999));
#216010=CARTESIAN_POINT('Ctrl Pts',(4.56837168299994,11.6,9.56054884799999));
#216011=CARTESIAN_POINT('Ctrl Pts',(4.56708316199994,15.2,9.55891241699998));
#216012=CARTESIAN_POINT('Ctrl Pts',(4.56708316199994,11.6,9.55891241699998));
#216013=CARTESIAN_POINT('Ctrl Pts',(4.56580037199994,15.2,9.55728025599999));
#216014=CARTESIAN_POINT('Ctrl Pts',(4.56580037199994,11.6,9.55728025599999));
#216015=CARTESIAN_POINT('Ctrl Pts',(4.56452330999994,15.2,9.55565238299998));
#216016=CARTESIAN_POINT('Ctrl Pts',(4.56452330999994,11.6,9.55565238299998));
#216017=CARTESIAN_POINT('Ctrl Pts',(4.56325197899994,15.2,9.55402881599999));
#216018=CARTESIAN_POINT('Ctrl Pts',(4.56325197899994,11.6,9.55402881599999));
#216019=CARTESIAN_POINT('Ctrl Pts',(4.56198637899994,15.2,9.55240957399998));
#216020=CARTESIAN_POINT('Ctrl Pts',(4.56198637899994,11.6,9.55240957399998));
#216021=CARTESIAN_POINT('Ctrl Pts',(4.56072650899994,15.2,9.55079467699999));
#216022=CARTESIAN_POINT('Ctrl Pts',(4.56072650899994,11.6,9.55079467699999));
#216023=CARTESIAN_POINT('Ctrl Pts',(4.55947236999994,15.2,9.54918414099998));
#216024=CARTESIAN_POINT('Ctrl Pts',(4.55947236999994,11.6,9.54918414099998));
#216025=CARTESIAN_POINT('Ctrl Pts',(4.55822396199994,15.2,9.54757798599999));
#216026=CARTESIAN_POINT('Ctrl Pts',(4.55822396199994,11.6,9.54757798599999));
#216027=CARTESIAN_POINT('Ctrl Pts',(4.55698128499994,15.2,9.54597623199999));
#216028=CARTESIAN_POINT('Ctrl Pts',(4.55698128499994,11.6,9.54597623199999));
#216029=CARTESIAN_POINT('Ctrl Pts',(4.55574434099994,15.2,9.54437889699999));
#216030=CARTESIAN_POINT('Ctrl Pts',(4.55574434099994,11.6,9.54437889699999));
#216031=CARTESIAN_POINT('Ctrl Pts',(4.55451312799994,15.2,9.54278599799999));
#216032=CARTESIAN_POINT('Ctrl Pts',(4.55451312799994,11.6,9.54278599799999));
#216033=CARTESIAN_POINT('Ctrl Pts',(4.55328764899994,15.2,9.54119755699999));
#216034=CARTESIAN_POINT('Ctrl Pts',(4.55328764899994,11.6,9.54119755699999));
#216035=CARTESIAN_POINT('Ctrl Pts',(4.55206790099994,15.2,9.53961359099999));
#216036=CARTESIAN_POINT('Ctrl Pts',(4.55206790099994,11.6,9.53961359099999));
#216037=CARTESIAN_POINT('Ctrl Pts',(4.55085388599994,15.2,9.53803411999999));
#216038=CARTESIAN_POINT('Ctrl Pts',(4.55085388599994,11.6,9.53803411999999));
#216039=CARTESIAN_POINT('Ctrl Pts',(4.54964560399994,15.2,9.53645916199999));
#216040=CARTESIAN_POINT('Ctrl Pts',(4.54964560399994,11.6,9.53645916199999));
#216041=CARTESIAN_POINT('Ctrl Pts',(4.54844305499994,15.2,9.53488873799999));
#216042=CARTESIAN_POINT('Ctrl Pts',(4.54844305499994,11.6,9.53488873799999));
#216043=CARTESIAN_POINT('Ctrl Pts',(4.54724623999994,15.2,9.53332286699998));
#216044=CARTESIAN_POINT('Ctrl Pts',(4.54724623999994,11.6,9.53332286699998));
#216045=CARTESIAN_POINT('Ctrl Pts',(4.54605515799994,15.2,9.53176156799999));
#216046=CARTESIAN_POINT('Ctrl Pts',(4.54605515799994,11.6,9.53176156799999));
#216047=CARTESIAN_POINT('Ctrl Pts',(4.54486980899994,15.2,9.53020485899999));
#216048=CARTESIAN_POINT('Ctrl Pts',(4.54486980899994,11.6,9.53020485899999));
#216049=CARTESIAN_POINT('Ctrl Pts',(4.54369019399994,15.2,9.52865276099999));
#216050=CARTESIAN_POINT('Ctrl Pts',(4.54369019399994,11.6,9.52865276099999));
#216051=CARTESIAN_POINT('Ctrl Pts',(4.54251631299994,15.2,9.52710529499999));
#216052=CARTESIAN_POINT('Ctrl Pts',(4.54251631299994,11.6,9.52710529499999));
#216053=CARTESIAN_POINT('Ctrl Pts',(4.54134816699994,15.2,9.52556247699999));
#216054=CARTESIAN_POINT('Ctrl Pts',(4.54134816699994,11.6,9.52556247699999));
#216055=CARTESIAN_POINT('Ctrl Pts',(4.54018575499994,15.2,9.52402432999998));
#216056=CARTESIAN_POINT('Ctrl Pts',(4.54018575499994,11.6,9.52402432999998));
#216057=CARTESIAN_POINT('Ctrl Pts',(4.53902907599994,15.2,9.52249087299998));
#216058=CARTESIAN_POINT('Ctrl Pts',(4.53902907599994,11.6,9.52249087299998));
#216059=CARTESIAN_POINT('Ctrl Pts',(4.53787813099994,15.2,9.52096212399999));
#216060=CARTESIAN_POINT('Ctrl Pts',(4.53787813099994,11.6,9.52096212399999));
#216061=CARTESIAN_POINT('Ctrl Pts',(4.53673292199994,15.2,9.51943810399998));
#216062=CARTESIAN_POINT('Ctrl Pts',(4.53673292199994,11.6,9.51943810399998));
#216063=CARTESIAN_POINT('Ctrl Pts',(4.53559344599994,15.2,9.51791883399999));
#216064=CARTESIAN_POINT('Ctrl Pts',(4.53559344599994,11.6,9.51791883399999));
#216065=CARTESIAN_POINT('Ctrl Pts',(4.53445970499994,15.2,9.51640433299998));
#216066=CARTESIAN_POINT('Ctrl Pts',(4.53445970499994,11.6,9.51640433299998));
#216067=CARTESIAN_POINT('Ctrl Pts',(4.53333169799994,15.2,9.51489462199999));
#216068=CARTESIAN_POINT('Ctrl Pts',(4.53333169799994,11.6,9.51489462199999));
#216069=CARTESIAN_POINT('Ctrl Pts',(4.53220942699994,15.2,9.51338971999999));
#216070=CARTESIAN_POINT('Ctrl Pts',(4.53220942699994,11.6,9.51338971999999));
#216071=CARTESIAN_POINT('Ctrl Pts',(4.53109288899994,15.2,9.51188964799999));
#216072=CARTESIAN_POINT('Ctrl Pts',(4.53109288899994,11.6,9.51188964799999));
#216073=CARTESIAN_POINT('Ctrl Pts',(4.52998208699994,15.2,9.51039442599999));
#216074=CARTESIAN_POINT('Ctrl Pts',(4.52998208699994,11.6,9.51039442599999));
#216075=CARTESIAN_POINT('Ctrl Pts',(4.52887701799994,15.2,9.50890407399999));
#216076=CARTESIAN_POINT('Ctrl Pts',(4.52887701799994,11.6,9.50890407399999));
#216077=CARTESIAN_POINT('Ctrl Pts',(4.52777768499994,15.2,9.50741861399998));
#216078=CARTESIAN_POINT('Ctrl Pts',(4.52777768499994,11.6,9.50741861399998));
#216079=CARTESIAN_POINT('Ctrl Pts',(4.52668408499994,15.2,9.50593806499998));
#216080=CARTESIAN_POINT('Ctrl Pts',(4.52668408499994,11.6,9.50593806499998));
#216081=CARTESIAN_POINT('Ctrl Pts',(4.52559621999994,15.2,9.50446244899998));
#216082=CARTESIAN_POINT('Ctrl Pts',(4.52559621999994,11.6,9.50446244899998));
#216083=CARTESIAN_POINT('Ctrl Pts',(4.52451408999994,15.2,9.50299178399998));
#216084=CARTESIAN_POINT('Ctrl Pts',(4.52451408999994,11.6,9.50299178399998));
#216085=CARTESIAN_POINT('Ctrl Pts',(4.52343769299994,15.2,9.50152609499998));
#216086=CARTESIAN_POINT('Ctrl Pts',(4.52343769299994,11.6,9.50152609499998));
#216087=CARTESIAN_POINT('Ctrl Pts',(4.52236703099994,15.2,9.50006539899999));
#216088=CARTESIAN_POINT('Ctrl Pts',(4.52236703099994,11.6,9.50006539899999));
#216089=CARTESIAN_POINT('Ctrl Pts',(4.52130210399995,15.2,9.49860971899999));
#216090=CARTESIAN_POINT('Ctrl Pts',(4.52130210399995,11.6,9.49860971899999));
#216091=CARTESIAN_POINT('Ctrl Pts',(4.52024290899994,15.2,9.49715907499998));
#216092=CARTESIAN_POINT('Ctrl Pts',(4.52024290899994,11.6,9.49715907499998));
#216093=CARTESIAN_POINT('Ctrl Pts',(4.51918944899994,15.2,9.49571348899998));
#216094=CARTESIAN_POINT('Ctrl Pts',(4.51918944899994,11.6,9.49571348899998));
#216095=CARTESIAN_POINT('Ctrl Pts',(4.51814172299994,15.2,9.49427298099998));
#216096=CARTESIAN_POINT('Ctrl Pts',(4.51814172299994,11.6,9.49427298099998));
#216097=CARTESIAN_POINT('Ctrl Pts',(4.51709972999994,15.2,9.49283757399999));
#216098=CARTESIAN_POINT('Ctrl Pts',(4.51709972999994,11.6,9.49283757399999));
#216099=CARTESIAN_POINT('Ctrl Pts',(4.51606346999994,15.2,9.49140728699999));
#216100=CARTESIAN_POINT('Ctrl Pts',(4.51606346999994,11.6,9.49140728699999));
#216101=CARTESIAN_POINT('Ctrl Pts',(4.51503294399994,15.2,9.48998214299999));
#216102=CARTESIAN_POINT('Ctrl Pts',(4.51503294399994,11.6,9.48998214299999));
#216103=CARTESIAN_POINT('Ctrl Pts',(4.51400814999994,15.2,9.48856216299999));
#216104=CARTESIAN_POINT('Ctrl Pts',(4.51400814999994,11.6,9.48856216299999));
#216105=CARTESIAN_POINT('Ctrl Pts',(4.51298909099994,15.2,9.48714736799998));
#216106=CARTESIAN_POINT('Ctrl Pts',(4.51298909099994,11.6,9.48714736799998));
#216107=CARTESIAN_POINT('Ctrl Pts',(4.51197576199994,15.2,9.48573778099998));
#216108=CARTESIAN_POINT('Ctrl Pts',(4.51197576199994,11.6,9.48573778099998));
#216109=CARTESIAN_POINT('Ctrl Pts',(4.51096816599994,15.2,9.48433342299998));
#216110=CARTESIAN_POINT('Ctrl Pts',(4.51096816599994,11.6,9.48433342299998));
#216111=CARTESIAN_POINT('Ctrl Pts',(4.50996630399994,15.2,9.48293431499999));
#216112=CARTESIAN_POINT('Ctrl Pts',(4.50996630399994,11.6,9.48293431499999));
#216113=CARTESIAN_POINT('Ctrl Pts',(4.50897017099994,15.2,9.48154047899998));
#216114=CARTESIAN_POINT('Ctrl Pts',(4.50897017099994,11.6,9.48154047899998));
#216115=CARTESIAN_POINT('Ctrl Pts',(4.50797977099994,15.2,9.48015193799998));
#216116=CARTESIAN_POINT('Ctrl Pts',(4.50797977099994,11.6,9.48015193799998));
#216117=CARTESIAN_POINT('Ctrl Pts',(4.50699510299994,15.2,9.47876871399998));
#216118=CARTESIAN_POINT('Ctrl Pts',(4.50699510299994,11.6,9.47876871399998));
#216119=CARTESIAN_POINT('Ctrl Pts',(4.50601616399994,15.2,9.47739082699999));
#216120=CARTESIAN_POINT('Ctrl Pts',(4.50601616399994,11.6,9.47739082699999));
#216121=CARTESIAN_POINT('Ctrl Pts',(4.50504295699994,15.2,9.47601830199999));
#216122=CARTESIAN_POINT('Ctrl Pts',(4.50504295699994,11.6,9.47601830199999));
#216123=CARTESIAN_POINT('Ctrl Pts',(4.50407547999994,15.2,9.47465115999999));
#216124=CARTESIAN_POINT('Ctrl Pts',(4.50407547999994,11.6,9.47465115999999));
#216125=CARTESIAN_POINT('Ctrl Pts',(4.50311373299994,15.2,9.47328942299999));
#216126=CARTESIAN_POINT('Ctrl Pts',(4.50311373299994,11.6,9.47328942299999));
#216127=CARTESIAN_POINT('Ctrl Pts',(4.50215771599994,15.2,9.47193311399998));
#216128=CARTESIAN_POINT('Ctrl Pts',(4.50215771599994,11.6,9.47193311399998));
#216129=CARTESIAN_POINT('Ctrl Pts',(4.50120742799994,15.2,9.47058225599999));
#216130=CARTESIAN_POINT('Ctrl Pts',(4.50120742799994,11.6,9.47058225599999));
#216131=CARTESIAN_POINT('Ctrl Pts',(4.50026286899994,15.2,9.46923686999998));
#216132=CARTESIAN_POINT('Ctrl Pts',(4.50026286899994,11.6,9.46923686999998));
#216133=CARTESIAN_POINT('Ctrl Pts',(4.49932403799994,15.2,9.46789697899998));
#216134=CARTESIAN_POINT('Ctrl Pts',(4.49932403799994,11.6,9.46789697899998));
#216135=CARTESIAN_POINT('Ctrl Pts',(4.49839093499994,15.2,9.46656260799998));
#216136=CARTESIAN_POINT('Ctrl Pts',(4.49839093499994,11.6,9.46656260799998));
#216137=CARTESIAN_POINT('Ctrl Pts',(4.49746355999994,15.2,9.46523377799998));
#216138=CARTESIAN_POINT('Ctrl Pts',(4.49746355999994,11.6,9.46523377799998));
#216139=CARTESIAN_POINT('Ctrl Pts',(4.49654191199994,15.2,9.46391051099998));
#216140=CARTESIAN_POINT('Ctrl Pts',(4.49654191199994,11.6,9.46391051099998));
#216141=CARTESIAN_POINT('Ctrl Pts',(4.49562599099994,15.2,9.46259283199998));
#216142=CARTESIAN_POINT('Ctrl Pts',(4.49562599099994,11.6,9.46259283199998));
#216143=CARTESIAN_POINT('Ctrl Pts',(4.49471579599994,15.2,9.46128076399999));
#216144=CARTESIAN_POINT('Ctrl Pts',(4.49471579599994,11.6,9.46128076399999));
#216145=CARTESIAN_POINT('Ctrl Pts',(4.49381132699994,15.2,9.45997432999999));
#216146=CARTESIAN_POINT('Ctrl Pts',(4.49381132699994,11.6,9.45997432999999));
#216147=CARTESIAN_POINT('Ctrl Pts',(4.49291258199994,15.2,9.45867355199999));
#216148=CARTESIAN_POINT('Ctrl Pts',(4.49291258199994,11.6,9.45867355199999));
#216149=CARTESIAN_POINT('Ctrl Pts',(4.49201956299994,15.2,9.45737845499998));
#216150=CARTESIAN_POINT('Ctrl Pts',(4.49201956299994,11.6,9.45737845499998));
#216151=CARTESIAN_POINT('Ctrl Pts',(4.49113226699995,15.2,9.45608906199999));
#216152=CARTESIAN_POINT('Ctrl Pts',(4.49113226699995,11.6,9.45608906199999));
#216153=CARTESIAN_POINT('Ctrl Pts',(4.49025069599994,15.2,9.45480539599998));
#216154=CARTESIAN_POINT('Ctrl Pts',(4.49025069599994,11.6,9.45480539599998));
#216155=CARTESIAN_POINT('Ctrl Pts',(4.48937484699994,15.2,9.45352748299998));
#216156=CARTESIAN_POINT('Ctrl Pts',(4.48937484699994,11.6,9.45352748299998));
#216157=CARTESIAN_POINT('Ctrl Pts',(4.48850472099994,15.2,9.45225534399999));
#216158=CARTESIAN_POINT('Ctrl Pts',(4.48850472099994,11.6,9.45225534399999));
#216159=CARTESIAN_POINT('Ctrl Pts',(4.48764031599994,15.2,9.45098900299998));
#216160=CARTESIAN_POINT('Ctrl Pts',(4.48764031599994,11.6,9.45098900299998));
#216161=CARTESIAN_POINT('Ctrl Pts',(4.48678163299994,15.2,9.44972848599999));
#216162=CARTESIAN_POINT('Ctrl Pts',(4.48678163299994,11.6,9.44972848599999));
#216163=CARTESIAN_POINT('Ctrl Pts',(4.48592867099994,15.2,9.44847381599999));
#216164=CARTESIAN_POINT('Ctrl Pts',(4.48592867099994,11.6,9.44847381599999));
#216165=CARTESIAN_POINT('Ctrl Pts',(4.48508142799994,15.2,9.44722501699999));
#216166=CARTESIAN_POINT('Ctrl Pts',(4.48508142799994,11.6,9.44722501699999));
#216167=CARTESIAN_POINT('Ctrl Pts',(4.48423990499994,15.2,9.44598211299999));
#216168=CARTESIAN_POINT('Ctrl Pts',(4.48423990499994,11.6,9.44598211299999));
#216169=CARTESIAN_POINT('Ctrl Pts',(4.48340409999994,15.2,9.44474512999999));
#216170=CARTESIAN_POINT('Ctrl Pts',(4.48340409999994,11.6,9.44474512999999));
#216171=CARTESIAN_POINT('Ctrl Pts',(4.48257401299994,15.2,9.44351408899998));
#216172=CARTESIAN_POINT('Ctrl Pts',(4.48257401299994,11.6,9.44351408899998));
#216173=CARTESIAN_POINT('Ctrl Pts',(4.48174964399994,15.2,9.44228901799999));
#216174=CARTESIAN_POINT('Ctrl Pts',(4.48174964399994,11.6,9.44228901799999));
#216175=CARTESIAN_POINT('Ctrl Pts',(4.48093099099994,15.2,9.44106994099998));
#216176=CARTESIAN_POINT('Ctrl Pts',(4.48093099099994,11.6,9.44106994099998));
#216177=CARTESIAN_POINT('Ctrl Pts',(4.48011805399995,15.2,9.43985688299998));
#216178=CARTESIAN_POINT('Ctrl Pts',(4.48011805399995,11.6,9.43985688299998));
#216179=CARTESIAN_POINT('Ctrl Pts',(4.47931083199994,15.2,9.43864986699998));
#216180=CARTESIAN_POINT('Ctrl Pts',(4.47931083199994,11.6,9.43864986699998));
#216181=CARTESIAN_POINT('Ctrl Pts',(4.47850932399994,15.2,9.43744891999999));
#216182=CARTESIAN_POINT('Ctrl Pts',(4.47850932399994,11.6,9.43744891999999));
#216183=CARTESIAN_POINT('Ctrl Pts',(4.47771352899994,15.2,9.43625406599999));
#216184=CARTESIAN_POINT('Ctrl Pts',(4.47771352899994,11.6,9.43625406599999));
#216185=CARTESIAN_POINT('Ctrl Pts',(4.47692344799994,15.2,9.43506532899999));
#216186=CARTESIAN_POINT('Ctrl Pts',(4.47692344799994,11.6,9.43506532899999));
#216187=CARTESIAN_POINT('Ctrl Pts',(4.47613907699994,15.2,9.43388273699998));
#216188=CARTESIAN_POINT('Ctrl Pts',(4.47613907699994,11.6,9.43388273699998));
#216189=CARTESIAN_POINT('Ctrl Pts',(4.47536041799994,15.2,9.43270631399999));
#216190=CARTESIAN_POINT('Ctrl Pts',(4.47536041799994,11.6,9.43270631399999));
#216191=CARTESIAN_POINT('Ctrl Pts',(4.47458746999994,15.2,9.43153608499999));
#216192=CARTESIAN_POINT('Ctrl Pts',(4.47458746999994,11.6,9.43153608499999));
#216193=CARTESIAN_POINT('Ctrl Pts',(4.47382022999994,15.2,9.43037207699999));
#216194=CARTESIAN_POINT('Ctrl Pts',(4.47382022999994,11.6,9.43037207699999));
#216195=CARTESIAN_POINT('Ctrl Pts',(4.47305869799994,15.2,9.42921431399999));
#216196=CARTESIAN_POINT('Ctrl Pts',(4.47305869799994,11.6,9.42921431399999));
#216197=CARTESIAN_POINT('Ctrl Pts',(4.47230287399994,15.2,9.42806282299999));
#216198=CARTESIAN_POINT('Ctrl Pts',(4.47230287399994,11.6,9.42806282299999));
#216199=CARTESIAN_POINT('Ctrl Pts',(4.47155275699994,15.2,9.42691763099998));
#216200=CARTESIAN_POINT('Ctrl Pts',(4.47155275699994,11.6,9.42691763099998));
#216201=CARTESIAN_POINT('Ctrl Pts',(4.47080834499994,15.2,9.42577875999999));
#216202=CARTESIAN_POINT('Ctrl Pts',(4.47080834499994,11.6,9.42577875999999));
#216203=CARTESIAN_POINT('Ctrl Pts',(4.47006963599994,15.2,9.42464624099999));
#216204=CARTESIAN_POINT('Ctrl Pts',(4.47006963599994,11.6,9.42464624099999));
#216205=CARTESIAN_POINT('Ctrl Pts',(4.46933663299994,15.2,9.42352009699999));
#216206=CARTESIAN_POINT('Ctrl Pts',(4.46933663299994,11.6,9.42352009699999));
#216207=CARTESIAN_POINT('Ctrl Pts',(4.46860933199994,15.2,9.42240035599998));
#216208=CARTESIAN_POINT('Ctrl Pts',(4.46860933199994,11.6,9.42240035599998));
#216209=CARTESIAN_POINT('Ctrl Pts',(4.46788773299994,15.2,9.42128704399998));
#216210=CARTESIAN_POINT('Ctrl Pts',(4.46788773299994,11.6,9.42128704399998));
#216211=CARTESIAN_POINT('Ctrl Pts',(4.46717183399994,15.2,9.42018018699999));
#216212=CARTESIAN_POINT('Ctrl Pts',(4.46717183399994,11.6,9.42018018699999));
#216213=CARTESIAN_POINT('Ctrl Pts',(4.46646163399994,15.2,9.41907981299998));
#216214=CARTESIAN_POINT('Ctrl Pts',(4.46646163399994,11.6,9.41907981299998));
#216215=CARTESIAN_POINT('Ctrl Pts',(4.46575713299994,15.2,9.41798594799998));
#216216=CARTESIAN_POINT('Ctrl Pts',(4.46575713299994,11.6,9.41798594799998));
#216217=CARTESIAN_POINT('Ctrl Pts',(4.46505832899994,15.2,9.41689861899999));
#216218=CARTESIAN_POINT('Ctrl Pts',(4.46505832899994,11.6,9.41689861899999));
#216219=CARTESIAN_POINT('Ctrl Pts',(4.46436522199994,15.2,9.41581785299999));
#216220=CARTESIAN_POINT('Ctrl Pts',(4.46436522199994,11.6,9.41581785299999));
#216221=CARTESIAN_POINT('Ctrl Pts',(4.46367780899994,15.2,9.41474367799999));
#216222=CARTESIAN_POINT('Ctrl Pts',(4.46367780899994,11.6,9.41474367799999));
#216223=CARTESIAN_POINT('Ctrl Pts',(4.46299609099994,15.2,9.41367611999999));
#216224=CARTESIAN_POINT('Ctrl Pts',(4.46299609099994,11.6,9.41367611999999));
#216225=CARTESIAN_POINT('Ctrl Pts',(4.46232006499994,15.2,9.41261520599999));
#216226=CARTESIAN_POINT('Ctrl Pts',(4.46232006499994,11.6,9.41261520599999));
#216227=CARTESIAN_POINT('Ctrl Pts',(4.46164973199994,15.2,9.41156096599999));
#216228=CARTESIAN_POINT('Ctrl Pts',(4.46164973199994,11.6,9.41156096599999));
#216229=CARTESIAN_POINT('Ctrl Pts',(4.46098508699994,15.2,9.41051342599999));
#216230=CARTESIAN_POINT('Ctrl Pts',(4.46098508699994,11.6,9.41051342599999));
#216231=CARTESIAN_POINT('Ctrl Pts',(4.46032613299994,15.2,9.40947261499998));
#216232=CARTESIAN_POINT('Ctrl Pts',(4.46032613299994,11.6,9.40947261499998));
#216233=CARTESIAN_POINT('Ctrl Pts',(4.45967286699995,15.2,9.40843855999999));
#216234=CARTESIAN_POINT('Ctrl Pts',(4.45967286699995,11.6,9.40843855999999));
#216235=CARTESIAN_POINT('Ctrl Pts',(4.45902528699994,15.2,9.40741128699998));
#216236=CARTESIAN_POINT('Ctrl Pts',(4.45902528699994,11.6,9.40741128699998));
#216237=CARTESIAN_POINT('Ctrl Pts',(4.45838339299994,15.2,9.40639082799999));
#216238=CARTESIAN_POINT('Ctrl Pts',(4.45838339299994,11.6,9.40639082799999));
#216239=CARTESIAN_POINT('Ctrl Pts',(4.45774718199995,15.2,9.40537720999998));
#216240=CARTESIAN_POINT('Ctrl Pts',(4.45774718199995,11.6,9.40537720999998));
#216241=CARTESIAN_POINT('Ctrl Pts',(4.45711665599995,15.2,9.40437045999998));
#216242=CARTESIAN_POINT('Ctrl Pts',(4.45711665599995,11.6,9.40437045999998));
#216243=CARTESIAN_POINT('Ctrl Pts',(4.45649180899994,15.2,9.40337060799998));
#216244=CARTESIAN_POINT('Ctrl Pts',(4.45649180899994,11.6,9.40337060799998));
#216245=CARTESIAN_POINT('Ctrl Pts',(4.45587264399994,15.2,9.40237768199999));
#216246=CARTESIAN_POINT('Ctrl Pts',(4.45587264399994,11.6,9.40237768199999));
#216247=CARTESIAN_POINT('Ctrl Pts',(4.45525915699994,15.2,9.40139171099998));
#216248=CARTESIAN_POINT('Ctrl Pts',(4.45525915699994,11.6,9.40139171099998));
#216249=CARTESIAN_POINT('Ctrl Pts',(4.45465134699994,15.2,9.40041272399998));
#216250=CARTESIAN_POINT('Ctrl Pts',(4.45465134699994,11.6,9.40041272399998));
#216251=CARTESIAN_POINT('Ctrl Pts',(4.45404921299995,15.2,9.39944075099999));
#216252=CARTESIAN_POINT('Ctrl Pts',(4.45404921299995,11.6,9.39944075099999));
#216253=CARTESIAN_POINT('Ctrl Pts',(4.45345275399994,15.2,9.39847581999998));
#216254=CARTESIAN_POINT('Ctrl Pts',(4.45345275399994,11.6,9.39847581999998));
#216255=CARTESIAN_POINT('Ctrl Pts',(4.45286196799994,15.2,9.39751795999998));
#216256=CARTESIAN_POINT('Ctrl Pts',(4.45286196799994,11.6,9.39751795999998));
#216257=CARTESIAN_POINT('Ctrl Pts',(4.45227685199994,15.2,9.39656720199999));
#216258=CARTESIAN_POINT('Ctrl Pts',(4.45227685199994,11.6,9.39656720199999));
#216259=CARTESIAN_POINT('Ctrl Pts',(4.45169740799995,15.2,9.39562357499998));
#216260=CARTESIAN_POINT('Ctrl Pts',(4.45169740799995,11.6,9.39562357499998));
#216261=CARTESIAN_POINT('Ctrl Pts',(4.45112363199994,15.2,9.39468710799999));
#216262=CARTESIAN_POINT('Ctrl Pts',(4.45112363199994,11.6,9.39468710799999));
#216263=CARTESIAN_POINT('Ctrl Pts',(4.45055552199995,15.2,9.39375783199999));
#216264=CARTESIAN_POINT('Ctrl Pts',(4.45055552199995,11.6,9.39375783199999));
#216265=CARTESIAN_POINT('Ctrl Pts',(4.44999307799994,15.2,9.39283577599999));
#216266=CARTESIAN_POINT('Ctrl Pts',(4.44999307799994,11.6,9.39283577599999));
#216267=CARTESIAN_POINT('Ctrl Pts',(4.44943629699995,15.2,9.39192097099999));
#216268=CARTESIAN_POINT('Ctrl Pts',(4.44943629699995,11.6,9.39192097099999));
#216269=CARTESIAN_POINT('Ctrl Pts',(4.44888517999994,15.2,9.39101344799998));
#216270=CARTESIAN_POINT('Ctrl Pts',(4.44888517999994,11.6,9.39101344799998));
#216271=CARTESIAN_POINT('Ctrl Pts',(4.44833972299994,15.2,9.39011323599999));
#216272=CARTESIAN_POINT('Ctrl Pts',(4.44833972299994,11.6,9.39011323599999));
#216273=CARTESIAN_POINT('Ctrl Pts',(4.44779992399994,15.2,9.38922036599998));
#216274=CARTESIAN_POINT('Ctrl Pts',(4.44779992399994,11.6,9.38922036599998));
#216275=CARTESIAN_POINT('Ctrl Pts',(4.44726578199994,15.2,9.38833486899998));
#216276=CARTESIAN_POINT('Ctrl Pts',(4.44726578199994,11.6,9.38833486899998));
#216277=CARTESIAN_POINT('Ctrl Pts',(4.44673729699994,15.2,9.38745677599999));
#216278=CARTESIAN_POINT('Ctrl Pts',(4.44673729699994,11.6,9.38745677599999));
#216279=CARTESIAN_POINT('Ctrl Pts',(4.44621446499994,15.2,9.38658611899999));
#216280=CARTESIAN_POINT('Ctrl Pts',(4.44621446499994,11.6,9.38658611899999));
#216281=CARTESIAN_POINT('Ctrl Pts',(4.44569728499994,15.2,9.38572292699998));
#216282=CARTESIAN_POINT('Ctrl Pts',(4.44569728499994,11.6,9.38572292699998));
#216283=CARTESIAN_POINT('Ctrl Pts',(4.44518575599994,15.2,9.38486723299999));
#216284=CARTESIAN_POINT('Ctrl Pts',(4.44518575599994,11.6,9.38486723299999));
#216285=CARTESIAN_POINT('Ctrl Pts',(4.44467987499995,15.2,9.38401906899998));
#216286=CARTESIAN_POINT('Ctrl Pts',(4.44467987499995,11.6,9.38401906899998));
#216287=CARTESIAN_POINT('Ctrl Pts',(4.44417963999994,15.2,9.38317846499999));
#216288=CARTESIAN_POINT('Ctrl Pts',(4.44417963999994,11.6,9.38317846499999));
#216289=CARTESIAN_POINT('Ctrl Pts',(4.44368505199995,15.2,9.38234545399999));
#216290=CARTESIAN_POINT('Ctrl Pts',(4.44368505199995,11.6,9.38234545399999));
#216291=CARTESIAN_POINT('Ctrl Pts',(4.44319610499995,15.2,9.38152006799999));
#216292=CARTESIAN_POINT('Ctrl Pts',(4.44319610499995,11.6,9.38152006799999));
#216293=CARTESIAN_POINT('Ctrl Pts',(4.44271279899994,15.2,9.38070233899998));
#216294=CARTESIAN_POINT('Ctrl Pts',(4.44271279899994,11.6,9.38070233899998));
#216295=CARTESIAN_POINT('Ctrl Pts',(4.44223513299994,15.2,9.37989229799999));
#216296=CARTESIAN_POINT('Ctrl Pts',(4.44223513299994,11.6,9.37989229799999));
#216297=CARTESIAN_POINT('Ctrl Pts',(4.44176310499994,15.2,9.37908997999998));
#216298=CARTESIAN_POINT('Ctrl Pts',(4.44176310499994,11.6,9.37908997999998));
#216299=CARTESIAN_POINT('Ctrl Pts',(4.44129939799994,15.2,9.37829999199998));
#216300=CARTESIAN_POINT('Ctrl Pts',(4.44129939799994,11.6,9.37829999199998));
#216301=CARTESIAN_POINT('Ctrl Pts',(4.44093341099994,15.2,9.37767505799999));
#216302=CARTESIAN_POINT('Ctrl Pts',(4.44093341099994,11.6,9.37767505799999));
#216303=CARTESIAN_POINT('Ctrl Pts',(4.44066206999994,15.2,9.37721094199999));
#216304=CARTESIAN_POINT('Ctrl Pts',(4.44066206999994,11.6,9.37721094199999));
#216305=CARTESIAN_POINT('Ctrl Pts',(4.44048314699994,15.2,9.37690455399999));
#216306=CARTESIAN_POINT('Ctrl Pts',(4.44048314699994,11.6,9.37690455399999));
#216307=CARTESIAN_POINT('Ctrl Pts',(4.44039525799994,15.2,9.37675396799998));
#216308=CARTESIAN_POINT('Ctrl Pts',(4.44039525799994,11.6,9.37675396799998));
#216309=CARTESIAN_POINT('',(4.44039525799994,12.2,9.37675396699999));
#216310=CARTESIAN_POINT('',(4.44039525799994,15.2,9.37675396699999));
#216311=CARTESIAN_POINT('',(4.44039525799994,12.2,9.37675396699999));
#216312=CARTESIAN_POINT('Ctrl Pts',(5.26939701799994,12.2,10.221714878));
#216313=CARTESIAN_POINT('Ctrl Pts',(5.2653120205644,12.2,10.2186661882717));
#216314=CARTESIAN_POINT('Ctrl Pts',(5.26124103171183,12.2,10.2156183760956));
#216315=CARTESIAN_POINT('Ctrl Pts',(5.25718406560325,12.2,10.2125714574851));
#216316=CARTESIAN_POINT('Ctrl Pts',(5.25312710004742,12.2,10.2095245392899));
#216317=CARTESIAN_POINT('Ctrl Pts',(5.24908415133328,12.2,10.2064785072781));
#216318=CARTESIAN_POINT('Ctrl Pts',(5.24505524247764,12.2,10.2034334347354));
#216319=CARTESIAN_POINT('Ctrl Pts',(5.24203356069867,12.2,10.2011496302247));
#216320=CARTESIAN_POINT('Ctrl Pts',(5.23901977556914,12.2,10.1988663694659));
#216321=CARTESIAN_POINT('Ctrl Pts',(5.23601390080266,12.2,10.1965836989655));
#216322=CARTESIAN_POINT('Ctrl Pts',(5.23300802603618,12.2,10.194301028465));
#216323=CARTESIAN_POINT('Ctrl Pts',(5.23001006011084,12.2,10.1920189499479));
#216324=CARTESIAN_POINT('Ctrl Pts',(5.22702001488506,12.2,10.1897375041973));
#216325=CARTESIAN_POINT('Ctrl Pts',(5.22402996911608,12.2,10.1874560580323));
#216326=CARTESIAN_POINT('Ctrl Pts',(5.22104784408269,12.2,10.1851752440175));
#216327=CARTESIAN_POINT('Ctrl Pts',(5.21807364785986,12.2,10.1828950987696));
#216328=CARTESIAN_POINT('Ctrl Pts',(5.21509945217735,12.2,10.1806149539359));
#216329=CARTESIAN_POINT('Ctrl Pts',(5.21213318603366,12.2,10.1783354761067));
#216330=CARTESIAN_POINT('Ctrl Pts',(5.20917485866094,12.2,10.1760567053258));
#216331=CARTESIAN_POINT('Ctrl Pts',(5.20621653128821,12.2,10.1737779345448));
#216332=CARTESIAN_POINT('Ctrl Pts',(5.2032661425217,12.2,10.171499871169));
#216333=CARTESIAN_POINT('Ctrl Pts',(5.20032370467096,12.2,10.1692225565018));
#216334=CARTESIAN_POINT('Ctrl Pts',(5.19738126682022,12.2,10.1669452418346));
#216335=CARTESIAN_POINT('Ctrl Pts',(5.19444677701023,12.2,10.164668675434));
#216336=CARTESIAN_POINT('Ctrl Pts',(5.19152024774155,12.2,10.162392898725));
#216337=CARTESIAN_POINT('Ctrl Pts',(5.18859371847288,12.2,10.160117122016));
#216338=CARTESIAN_POINT('Ctrl Pts',(5.18567514874556,12.2,10.157842134432));
#216339=CARTESIAN_POINT('Ctrl Pts',(5.18276454755894,12.2,10.1555679752645));
#216340=CARTESIAN_POINT('Ctrl Pts',(5.17985394637232,12.2,10.1532938160971));
#216341=CARTESIAN_POINT('Ctrl Pts',(5.17695131418371,12.2,10.1510204859874));
#216342=CARTESIAN_POINT('Ctrl Pts',(5.17405666176834,12.2,10.1487480252063));
#216343=CARTESIAN_POINT('Ctrl Pts',(5.17019712486394,12.2,10.145718077223));
#216344=CARTESIAN_POINT('Ctrl Pts',(5.16635177173637,12.2,10.1426896739813));
#216345=CARTESIAN_POINT('Ctrl Pts',(5.16252062769516,12.2,10.1396629147609));
#216346=CARTESIAN_POINT('Ctrl Pts',(5.15964726992526,12.2,10.1373928455518));
#216347=CARTESIAN_POINT('Ctrl Pts',(5.1567819042794,12.2,10.1351236999176));
#216348=CARTESIAN_POINT('Ctrl Pts',(5.15392454050822,12.2,10.1328555202083));
#216349=CARTESIAN_POINT('Ctrl Pts',(5.15106717673703,12.2,10.130587340499));
#216350=CARTESIAN_POINT('Ctrl Pts',(5.14821781410719,12.2,10.1283201257148));
#216351=CARTESIAN_POINT('Ctrl Pts',(5.14537646333473,12.2,10.1260539180053));
#216352=CARTESIAN_POINT('Ctrl Pts',(5.14253511256228,12.2,10.1237877102959));
#216353=CARTESIAN_POINT('Ctrl Pts',(5.13970177271935,12.2,10.121522509169));
#216354=CARTESIAN_POINT('Ctrl Pts',(5.13687645430493,12.2,10.1192583559714));
#216355=CARTESIAN_POINT('Ctrl Pts',(5.13405113589052,12.2,10.1169942027738));
#216356=CARTESIAN_POINT('Ctrl Pts',(5.13123383787802,12.2,10.1147310987777));
#216357=CARTESIAN_POINT('Ctrl Pts',(5.12842457110398,12.2,10.1124690842348));
#216358=CARTESIAN_POINT('Ctrl Pts',(5.12561530381961,12.2,10.1102070692809));
#216359=CARTESIAN_POINT('Ctrl Pts',(5.1228140669125,12.2,10.1079461450189));
#216360=CARTESIAN_POINT('Ctrl Pts',(5.12002087017431,12.2,10.1056863534823));
#216361=CARTESIAN_POINT('Ctrl Pts',(5.11722767394355,12.2,10.1034265623563));
#216362=CARTESIAN_POINT('Ctrl Pts',(5.11444251757905,12.2,10.1011679040885));
#216363=CARTESIAN_POINT('Ctrl Pts',(5.11166541043065,12.2,10.0989104195039));
#216364=CARTESIAN_POINT('Ctrl Pts',(5.10888830328225,12.2,10.0966529349194));
#216365=CARTESIAN_POINT('Ctrl Pts',(5.10611924669956,12.2,10.0943966254347));
#216366=CARTESIAN_POINT('Ctrl Pts',(5.10335824800821,12.2,10.0921415337666));
#216367=CARTESIAN_POINT('Ctrl Pts',(5.10059724931687,12.2,10.0898864420986));
#216368=CARTESIAN_POINT('Ctrl Pts',(5.09784430908352,12.2,10.0876325671471));
#216369=CARTESIAN_POINT('Ctrl Pts',(5.09509943826588,12.2,10.0853799534789));
#216370=CARTESIAN_POINT('Ctrl Pts',(5.09235456744824,12.2,10.0831273398106));
#216371=CARTESIAN_POINT('Ctrl Pts',(5.08961776391601,12.2,10.0808759864328));
#216372=CARTESIAN_POINT('Ctrl Pts',(5.08688903800291,12.2,10.0786259366937));
#216373=CARTESIAN_POINT('Ctrl Pts',(5.0841603120898,12.2,10.0763758869545));
#216374=CARTESIAN_POINT('Ctrl Pts',(5.0814396636271,12.2,10.0741271405584));
#216375=CARTESIAN_POINT('Ctrl Pts',(5.07872710234957,12.2,10.0718797414316));
#216376=CARTESIAN_POINT('Ctrl Pts',(5.07601454057925,12.2,10.0696323418964));
#216377=CARTESIAN_POINT('Ctrl Pts',(5.07331006515285,12.2,10.0673862893367));
#216378=CARTESIAN_POINT('Ctrl Pts',(5.07061368588709,12.2,10.0651416272606));
#216379=CARTESIAN_POINT('Ctrl Pts',(5.06791730711117,12.2,10.0628969655924));
#216380=CARTESIAN_POINT('Ctrl Pts',(5.0652290237098,12.2,10.0606536937074));
#216381=CARTESIAN_POINT('Ctrl Pts',(5.06254884547455,12.2,10.0584118579973));
#216382=CARTESIAN_POINT('Ctrl Pts',(5.0598686672393,12.2,10.0561700222872));
#216383=CARTESIAN_POINT('Ctrl Pts',(5.05719659446274,12.2,10.0539296205601));
#216384=CARTESIAN_POINT('Ctrl Pts',(5.05453263525581,12.2,10.0516906975063));
#216385=CARTESIAN_POINT('Ctrl Pts',(5.05186867604886,12.2,10.0494517744525));
#216386=CARTESIAN_POINT('Ctrl Pts',(5.04921283073482,12.2,10.0472143307976));
#216387=CARTESIAN_POINT('Ctrl Pts',(5.04656510898563,12.2,10.044978410202));
#216388=CARTESIAN_POINT('Ctrl Pts',(5.04391738723644,12.2,10.0427424896064));
#216389=CARTESIAN_POINT('Ctrl Pts',(5.04127778877529,12.2,10.0405080921791));
#216390=CARTESIAN_POINT('Ctrl Pts',(5.03864632153685,12.2,10.03827526351));
#216391=CARTESIAN_POINT('Ctrl Pts',(5.03601485429843,12.2,10.036042434841));
#216392=CARTESIAN_POINT('Ctrl Pts',(5.03339151892609,12.2,10.0338111735552));
#216393=CARTESIAN_POINT('Ctrl Pts',(5.03077632510334,12.2,10.0315815254694));
#216394=CARTESIAN_POINT('Ctrl Pts',(5.02816113080549,12.2,10.0293518769784));
#216395=CARTESIAN_POINT('Ctrl Pts',(5.0255540764766,12.2,10.027123841538));
#216396=CARTESIAN_POINT('Ctrl Pts',(5.02295517268333,12.2,10.0248974650063));
#216397=CARTESIAN_POINT('Ctrl Pts',(5.01948996841253,12.2,10.0219289636381));
#216398=CARTESIAN_POINT('Ctrl Pts',(5.01603925109809,12.2,10.0189634097816));
#216399=CARTESIAN_POINT('Ctrl Pts',(5.01260304425224,12.2,10.0160009125103));
#216400=CARTESIAN_POINT('Ctrl Pts',(5.01002588900081,12.2,10.013779039456));
#216401=CARTESIAN_POINT('Ctrl Pts',(5.0074568954535,12.2,10.0115588863114));
#216402=CARTESIAN_POINT('Ctrl Pts',(5.00489607079582,12.2,10.0093404982668));
#216403=CARTESIAN_POINT('Ctrl Pts',(5.00233524613813,12.2,10.0071221102222));
#216404=CARTESIAN_POINT('Ctrl Pts',(4.99978259281325,12.2,10.0049054877859));
#216405=CARTESIAN_POINT('Ctrl Pts',(4.99723811711292,12.2,10.0026906762411));
#216406=CARTESIAN_POINT('Ctrl Pts',(4.99469364095034,12.2,10.000475864294));
#216407=CARTESIAN_POINT('Ctrl Pts',(4.99215734326508,12.2,9.99826286325572));
#216408=CARTESIAN_POINT('Ctrl Pts',(4.98962923394044,12.2,9.99605172126795));
#216409=CARTESIAN_POINT('Ctrl Pts',(4.98625842227304,12.2,9.9931035326204));
#216410=CARTESIAN_POINT('Ctrl Pts',(4.98290216362476,12.2,9.99015864651654));
#216411=CARTESIAN_POINT('Ctrl Pts',(4.97956048149383,12.2,9.98721717524364));
#216412=CARTESIAN_POINT('Ctrl Pts',(4.97621879890759,12.2,9.98427570356997));
#216413=CARTESIAN_POINT('Ctrl Pts',(4.97289169100956,12.2,9.9813376455353));
#216414=CARTESIAN_POINT('Ctrl Pts',(4.96957917894164,12.2,9.97840311448685));
#216415=CARTESIAN_POINT('Ctrl Pts',(4.96626666732504,12.2,9.97546858383822));
#216416=CARTESIAN_POINT('Ctrl Pts',(4.9629687504621,12.2,9.97253758002802));
#216417=CARTESIAN_POINT('Ctrl Pts',(4.9596854482851,12.2,9.96961021548932));
#216418=CARTESIAN_POINT('Ctrl Pts',(4.95640214566075,12.2,9.96668285055175));
#216419=CARTESIAN_POINT('Ctrl Pts',(4.95313345891366,12.2,9.96375912597543));
#216420=CARTESIAN_POINT('Ctrl Pts',(4.94987940551945,12.2,9.96083915355961));
#216421=CARTESIAN_POINT('Ctrl Pts',(4.9466253525686,12.2,9.95791918154165));
#216422=CARTESIAN_POINT('Ctrl Pts',(4.94338593425932,12.2,9.95500296396137));
#216423=CARTESIAN_POINT('Ctrl Pts',(4.94016117002198,12.2,9.95209061475476));
#216424=CARTESIAN_POINT('Ctrl Pts',(4.93693640534528,12.2,9.94917826515134));
#216425=CARTESIAN_POINT('Ctrl Pts',(4.93372629353421,12.2,9.94626978343171));
#216426=CARTESIAN_POINT('Ctrl Pts',(4.93053085547213,12.2,9.9433652864959));
#216427=CARTESIAN_POINT('Ctrl Pts',(4.92733541784544,12.2,9.94046078995584));
#216428=CARTESIAN_POINT('Ctrl Pts',(4.92415465206556,12.2,9.93756027910911));
#216429=CARTESIAN_POINT('Ctrl Pts',(4.92098857894272,12.2,9.93466386914528));
#216430=CARTESIAN_POINT('Ctrl Pts',(4.9178225053885,12.2,9.93176745878681));
#216431=CARTESIAN_POINT('Ctrl Pts',(4.91467112236914,12.2,9.92887515004603));
#216432=CARTESIAN_POINT('Ctrl Pts',(4.91153445097694,12.2,9.92598706105558));
#216433=CARTESIAN_POINT('Ctrl Pts',(4.90839778001212,12.2,9.92309897245864));
#216434=CARTESIAN_POINT('Ctrl Pts',(4.90527581901654,12.2,9.92021510386916));
#216435=CARTESIAN_POINT('Ctrl Pts',(4.9021685868246,12.2,9.91733557343745));
#216436=CARTESIAN_POINT('Ctrl Pts',(4.89906135420929,12.2,9.91445604261339));
#216437=CARTESIAN_POINT('Ctrl Pts',(4.89596885035724,12.2,9.91158085077582));
#216438=CARTESIAN_POINT('Ctrl Pts',(4.89289109373113,12.2,9.90871011843968));
#216439=CARTESIAN_POINT('Ctrl Pts',(4.88981333752437,12.2,9.90583938649468));
#216440=CARTESIAN_POINT('Ctrl Pts',(4.88675032783394,12.2,9.90297311305106));
#216441=CARTESIAN_POINT('Ctrl Pts',(4.88370208474828,12.2,9.90011141995119));
#216442=CARTESIAN_POINT('Ctrl Pts',(4.8806538412473,12.2,9.89724972646141));
#216443=CARTESIAN_POINT('Ctrl Pts',(4.87762036132828,12.2,9.89439261380542));
#216444=CARTESIAN_POINT('Ctrl Pts',(4.87460166477489,12.2,9.89154020298331));
#216445=CARTESIAN_POINT('Ctrl Pts',(4.87158296822151,12.2,9.88868779216121));
#216446=CARTESIAN_POINT('Ctrl Pts',(4.86857905546424,12.2,9.88584008495627));
#216447=CARTESIAN_POINT('Ctrl Pts',(4.86558994280284,12.2,9.88299720280183));
#216448=CARTESIAN_POINT('Ctrl Pts',(4.86110627421802,12.2,9.8787328799575));
#216449=CARTESIAN_POINT('Ctrl Pts',(4.8566559065057,12.2,9.87447941661418));
#216450=CARTESIAN_POINT('Ctrl Pts',(4.85223889875095,12.2,9.8702372327688));
#216451=CARTESIAN_POINT('Ctrl Pts',(4.84929422704819,12.2,9.86740911033366));
#216452=CARTESIAN_POINT('Ctrl Pts',(4.84636438118417,12.2,9.8645860005642));
#216453=CARTESIAN_POINT('Ctrl Pts',(4.8434493789765,12.2,9.86176803146071));
#216454=CARTESIAN_POINT('Ctrl Pts',(4.84053437637165,12.2,9.85895006197325));
#216455=CARTESIAN_POINT('Ctrl Pts',(4.83763421668213,12.2,9.85613723330575));
#216456=CARTESIAN_POINT('Ctrl Pts',(4.83474891802488,12.2,9.85332967054163));
#216457=CARTESIAN_POINT('Ctrl Pts',(4.83186361936764,12.2,9.85052210777752));
#216458=CARTESIAN_POINT('Ctrl Pts',(4.82899318032601,12.2,9.84771981368344));
#216459=CARTESIAN_POINT('Ctrl Pts',(4.82613761828301,12.2,9.84492291430934));
#216460=CARTESIAN_POINT('Ctrl Pts',(4.82328205662909,12.2,9.84212601531632));
#216461=CARTESIAN_POINT('Ctrl Pts',(4.82044137020316,12.2,9.8393345126868));
#216462=CARTESIAN_POINT('Ctrl Pts',(4.81761557847681,12.2,9.8365485362352));
#216463=CARTESIAN_POINT('Ctrl Pts',(4.81478978636546,12.2,9.83376255940399));
#216464=CARTESIAN_POINT('Ctrl Pts',(4.81197888582972,12.2,9.8309821085136));
#216465=CARTESIAN_POINT('Ctrl Pts',(4.80918289506775,12.2,9.82820731502962));
#216466=CARTESIAN_POINT('Ctrl Pts',(4.80638690468674,12.2,9.82543252192371));
#216467=CARTESIAN_POINT('Ctrl Pts',(4.80360582296489,12.2,9.82266338481429));
#216468=CARTESIAN_POINT('Ctrl Pts',(4.80083966546783,12.2,9.81990003898426));
#216469=CARTESIAN_POINT('Ctrl Pts',(4.79807350759388,12.2,9.81713669277772));
#216470=CARTESIAN_POINT('Ctrl Pts',(4.79532227474298,12.2,9.81437913470427));
#216471=CARTESIAN_POINT('Ctrl Pts',(4.79258598190291,12.2,9.81162750108404));
#216472=CARTESIAN_POINT('Ctrl Pts',(4.78984968943566,12.2,9.80887586783873));
#216473=CARTESIAN_POINT('Ctrl Pts',(4.78712833722324,12.2,9.80613015788931));
#216474=CARTESIAN_POINT('Ctrl Pts',(4.78442194022127,12.2,9.80339050622398));
#216475=CARTESIAN_POINT('Ctrl Pts',(4.78171554285056,12.2,9.80065085418537));
#216476=CARTESIAN_POINT('Ctrl Pts',(4.77902410020388,12.2,9.7979172612364));
#216477=CARTESIAN_POINT('Ctrl Pts',(4.77634762828123,12.2,9.79518986197706));
#216478=CARTESIAN_POINT('Ctrl Pts',(4.77367115672325,12.2,9.79246246308933));
#216479=CARTESIAN_POINT('Ctrl Pts',(4.77100965562339,12.2,9.7897412602804));
#216480=CARTESIAN_POINT('Ctrl Pts',(4.76836313915066,12.2,9.78702638914394));
#216481=CARTESIAN_POINT('Ctrl Pts',(4.76505499328931,12.2,9.78363279994593));
#216482=CARTESIAN_POINT('Ctrl Pts',(4.76177026094788,12.2,9.78024910590453));
#216483=CARTESIAN_POINT('Ctrl Pts',(4.75850897115498,12.2,9.77687557777898));
#216484=CARTESIAN_POINT('Ctrl Pts',(4.75589993917847,12.2,9.77417675513147));
#216485=CARTESIAN_POINT('Ctrl Pts',(4.75330591112321,12.2,9.77148443923473));
#216486=CARTESIAN_POINT('Ctrl Pts',(4.75072689853919,12.2,9.7687987705888));
#216487=CARTESIAN_POINT('Ctrl Pts',(4.74814788630656,12.2,9.76611310230878));
#216488=CARTESIAN_POINT('Ctrl Pts',(4.74558389201512,12.2,9.76343408176174));
#216489=CARTESIAN_POINT('Ctrl Pts',(4.74303492759484,12.2,9.76076185067942));
#216490=CARTESIAN_POINT('Ctrl Pts',(4.74048596282725,12.2,9.758089619233));
#216491=CARTESIAN_POINT('Ctrl Pts',(4.73795202858875,12.2,9.7554241777688));
#216492=CARTESIAN_POINT('Ctrl Pts',(4.73543313928577,12.2,9.75276566979102));
#216493=CARTESIAN_POINT('Ctrl Pts',(4.732914250326,12.2,9.75010716217546));
#216494=CARTESIAN_POINT('Ctrl Pts',(4.73041040501321,12.2,9.74745558778629));
#216495=CARTESIAN_POINT('Ctrl Pts',(4.72792161738181,12.2,9.744811092724));
#216496=CARTESIAN_POINT('Ctrl Pts',(4.72543282941131,12.2,9.74216659730139));
#216497=CARTESIAN_POINT('Ctrl Pts',(4.72295909912665,12.2,9.73952918073676));
#216498=CARTESIAN_POINT('Ctrl Pts',(4.72050043898155,12.2,9.73689898824816));
#216499=CARTESIAN_POINT('Ctrl Pts',(4.71804177917144,12.2,9.73426879611794));
#216500=CARTESIAN_POINT('Ctrl Pts',(4.71559818880275,12.2,9.73164582986177));
#216501=CARTESIAN_POINT('Ctrl Pts',(4.71316968238862,12.2,9.72903023768594));
#216502=CARTESIAN_POINT('Ctrl Pts',(4.71074117564361,12.2,9.72641464515374));
#216503=CARTESIAN_POINT('Ctrl Pts',(4.70832775053337,12.2,9.72380642651948));
#216504=CARTESIAN_POINT('Ctrl Pts',(4.70592942179155,12.2,9.72120573126663));
#216505=CARTESIAN_POINT('Ctrl Pts',(4.70353109304973,12.2,9.71860503601378));
#216506=CARTESIAN_POINT('Ctrl Pts',(4.70114785910134,12.2,9.71601186439792));
#216507=CARTESIAN_POINT('Ctrl Pts',(4.69877973186271,12.2,9.7134263678689));
#216508=CARTESIAN_POINT('Ctrl Pts',(4.69641160494673,12.2,9.71084087169215));
#216509=CARTESIAN_POINT('Ctrl Pts',(4.69405858586547,12.2,9.70826305030053));
#216510=CARTESIAN_POINT('Ctrl Pts',(4.69172068493481,12.2,9.70569305677671));
#216511=CARTESIAN_POINT('Ctrl Pts',(4.68938278368562,12.2,9.70312306290272));
#216512=CARTESIAN_POINT('Ctrl Pts',(4.68706000179682,12.2,9.7005608968763));
#216513=CARTESIAN_POINT('Ctrl Pts',(4.68475235033926,12.2,9.69800671484902));
#216514=CARTESIAN_POINT('Ctrl Pts',(4.68244469919612,12.2,9.69545253316975));
#216515=CARTESIAN_POINT('Ctrl Pts',(4.68015217650101,12.2,9.69290633256723));
#216516=CARTESIAN_POINT('Ctrl Pts',(4.67787479668621,12.2,9.69036827244086));
#216517=CARTESIAN_POINT('Ctrl Pts',(4.67559741656112,12.2,9.68783021196868));
#216518=CARTESIAN_POINT('Ctrl Pts',(4.67333517723231,12.2,9.68530029061066));
#216519=CARTESIAN_POINT('Ctrl Pts',(4.67108808916556,12.2,9.68277866662575));
#216520=CARTESIAN_POINT('Ctrl Pts',(4.66884100140499,12.2,9.68025704298442));
#216521=CARTESIAN_POINT('Ctrl Pts',(4.6666090661566,12.2,9.67774371659783));
#216522=CARTESIAN_POINT('Ctrl Pts',(4.66439229244791,12.2,9.67523884774647));
#216523=CARTESIAN_POINT('Ctrl Pts',(4.66162132508552,12.2,9.67210776142629));
#216524=CARTESIAN_POINT('Ctrl Pts',(4.65887404823495,12.2,9.66898988992599));
#216525=CARTESIAN_POINT('Ctrl Pts',(4.65615048246981,12.2,9.66588554874472));
#216526=CARTESIAN_POINT('Ctrl Pts',(4.65342691670467,12.2,9.66278120756344));
#216527=CARTESIAN_POINT('Ctrl Pts',(4.6507270597358,12.2,9.65969039592677));
#216528=CARTESIAN_POINT('Ctrl Pts',(4.64805093375135,12.2,9.6566134364683));
#216529=CARTESIAN_POINT('Ctrl Pts',(4.64537480776689,12.2,9.65353647700981));
#216530=CARTESIAN_POINT('Ctrl Pts',(4.64272240943322,12.2,9.65047336971662));
#216531=CARTESIAN_POINT('Ctrl Pts',(4.64009375797488,12.2,9.64742443929995));
#216532=CARTESIAN_POINT('Ctrl Pts',(4.63746510651654,12.2,9.64437550888329));
#216533=CARTESIAN_POINT('Ctrl Pts',(4.63486020159988,12.2,9.64134075374995));
#216534=CARTESIAN_POINT('Ctrl Pts',(4.63227906076654,12.2,9.63832050749994));
#216535=CARTESIAN_POINT('Ctrl Pts',(4.6296979199332,12.2,9.63530026124993));
#216536=CARTESIAN_POINT('Ctrl Pts',(4.62714054270995,12.2,9.63229452091742));
#216537=CARTESIAN_POINT('Ctrl Pts',(4.62460694374017,12.2,9.62930362305665));
#216538=CARTESIAN_POINT('Ctrl Pts',(4.62207334477039,12.2,9.62631272519588));
#216539=CARTESIAN_POINT('Ctrl Pts',(4.61956352612509,12.2,9.62333666902227));
#216540=CARTESIAN_POINT('Ctrl Pts',(4.61707750057077,12.2,9.62037579402306));
#216541=CARTESIAN_POINT('Ctrl Pts',(4.61459147501646,12.2,9.61741491902385));
#216542=CARTESIAN_POINT('Ctrl Pts',(4.61212924506708,12.2,9.61446922775758));
#216543=CARTESIAN_POINT('Ctrl Pts',(4.60969082333222,12.2,9.61153906255007));
#216544=CARTESIAN_POINT('Ctrl Pts',(4.60725240159737,12.2,9.60860889734257));
#216545=CARTESIAN_POINT('Ctrl Pts',(4.60483778696246,12.2,9.60569425874612));
#216546=CARTESIAN_POINT('Ctrl Pts',(4.6024469944141,12.2,9.60279549763016));
#216547=CARTESIAN_POINT('Ctrl Pts',(4.5995780434603,12.2,9.59931698441738));
#216548=CARTESIAN_POINT('Ctrl Pts',(4.59674339658148,12.2,9.59586133460025));
#216549=CARTESIAN_POINT('Ctrl Pts',(4.59394307101654,12.2,9.59242916347494));
#216550=CARTESIAN_POINT('Ctrl Pts',(4.59160946629431,12.2,9.5895690207666));
#216551=CARTESIAN_POINT('Ctrl Pts',(4.58929969949227,12.2,9.58672518292228));
#216552=CARTESIAN_POINT('Ctrl Pts',(4.58701377719031,12.2,9.58389801200673));
#216553=CARTESIAN_POINT('Ctrl Pts',(4.58472785488834,12.2,9.58107084109118));
#216554=CARTESIAN_POINT('Ctrl Pts',(4.58246578114682,12.2,9.57826033739977));
#216555=CARTESIAN_POINT('Ctrl Pts',(4.5802275621203,12.2,9.57546686906734));
#216556=CARTESIAN_POINT('Ctrl Pts',(4.57798934309378,12.2,9.5726734007349));
#216557=CARTESIAN_POINT('Ctrl Pts',(4.57577498043331,12.2,9.56989696797427));
#216558=CARTESIAN_POINT('Ctrl Pts',(4.57358448307344,12.2,9.56713794533627));
#216559=CARTESIAN_POINT('Ctrl Pts',(4.57139398571357,12.2,9.56437892269829));
#216560=CARTESIAN_POINT('Ctrl Pts',(4.56922735380106,12.2,9.56163730840754));
#216561=CARTESIAN_POINT('Ctrl Pts',(4.56708459445956,12.2,9.55891348417547));
#216562=CARTESIAN_POINT('Ctrl Pts',(4.56494183511805,12.2,9.5561896599434));
#216563=CARTESIAN_POINT('Ctrl Pts',(4.56282294889613,12.2,9.55348362526355));
#216564=CARTESIAN_POINT('Ctrl Pts',(4.56072794146753,12.2,9.55079576693171));
#216565=CARTESIAN_POINT('Ctrl Pts',(4.55863293403893,12.2,9.54810790859987));
#216566=CARTESIAN_POINT('Ctrl Pts',(4.55656180451348,12.2,9.54543822606832));
#216567=CARTESIAN_POINT('Ctrl Pts',(4.55451456118211,12.2,9.54278711211152));
#216568=CARTESIAN_POINT('Ctrl Pts',(4.55205786927373,12.2,9.53960577547894));
#216569=CARTESIAN_POINT('Ctrl Pts',(4.54963557012329,12.2,9.53645117662313));
#216570=CARTESIAN_POINT('Ctrl Pts',(4.54724767312822,12.2,9.53332400982129));
#216571=CARTESIAN_POINT('Ctrl Pts',(4.54485977613314,12.2,9.53019684301944));
#216572=CARTESIAN_POINT('Ctrl Pts',(4.54250627931032,12.2,9.52709710346541));
#216573=CARTESIAN_POINT('Ctrl Pts',(4.54018718839309,12.2,9.52402550265912));
#216574=CARTESIAN_POINT('Ctrl Pts',(4.53786809747585,12.2,9.52095390185282));
#216575=CARTESIAN_POINT('Ctrl Pts',(4.53558341020743,12.2,9.51791043415431));
#216576=CARTESIAN_POINT('Ctrl Pts',(4.53333313220351,12.2,9.5148958245952));
#216577=CARTESIAN_POINT('Ctrl Pts',(4.53070780772933,12.2,9.51137877992701));
#216578=CARTESIAN_POINT('Ctrl Pts',(4.52812931492057,12.2,9.50790101067677));
#216579=CARTESIAN_POINT('Ctrl Pts',(4.52559765385162,12.2,9.50446368696895));
#216580=CARTESIAN_POINT('Ctrl Pts',(4.52342765876229,12.2,9.50151740965803));
#216581=CARTESIAN_POINT('Ctrl Pts',(4.5212920688216,12.2,9.49860084915342));
#216582=CARTESIAN_POINT('Ctrl Pts',(4.51919088272892,12.2,9.49571475883952));
#216583=CARTESIAN_POINT('Ctrl Pts',(4.51708969644538,12.2,9.49282866826346));
#216584=CARTESIAN_POINT('Ctrl Pts',(4.51502291173186,12.2,9.48997304831535));
#216585=CARTESIAN_POINT('Ctrl Pts',(4.51299052345593,12.2,9.48714866982946));
#216586=CARTESIAN_POINT('Ctrl Pts',(4.5109581353646,12.2,9.48432429160011));
#216587=CARTESIAN_POINT('Ctrl Pts',(4.50896014223842,12.2,9.48153115545513));
#216588=CARTESIAN_POINT('Ctrl Pts',(4.50699653530078,12.2,9.47877004829285));
#216589=CARTESIAN_POINT('Ctrl Pts',(4.50503292836314,12.2,9.47600894113057));
#216590=CARTESIAN_POINT('Ctrl Pts',(4.50310370746493,12.2,9.4732798645481));
#216591=CARTESIAN_POINT('Ctrl Pts',(4.5012088604481,12.2,9.47058362431049));
#216592=CARTESIAN_POINT('Ctrl Pts',(4.49931401325915,12.2,9.46788738382798));
#216593=CARTESIAN_POINT('Ctrl Pts',(4.49745353859021,12.2,9.46522397791527));
#216594=CARTESIAN_POINT('Ctrl Pts',(4.49562742240884,12.2,9.46259423460674));
#216595=CARTESIAN_POINT('Ctrl Pts',(4.49380130639334,12.2,9.45996449153708));
#216596=CARTESIAN_POINT('Ctrl Pts',(4.49200954664489,12.2,9.4573684092114));
#216597=CARTESIAN_POINT('Ctrl Pts',(4.49025212653402,12.2,9.45480683420942));
#216598=CARTESIAN_POINT('Ctrl Pts',(4.48849470642314,12.2,9.45224525920745));
#216599=CARTESIAN_POINT('Ctrl Pts',(4.48677162418329,12.2,9.44971818978343));
#216600=CARTESIAN_POINT('Ctrl Pts',(4.48508285815897,12.2,9.44722649103819));
#216601=CARTESIAN_POINT('Ctrl Pts',(4.48339409198124,12.2,9.44473479206662));
#216602=CARTESIAN_POINT('Ctrl Pts',(4.48173964192714,12.2,9.44227846338324));
#216603=CARTESIAN_POINT('Ctrl Pts',(4.48011948259323,12.2,9.43985839329923));
#216604=CARTESIAN_POINT('Ctrl Pts',(4.47849932340649,12.2,9.43743832343503));
#216605=CARTESIAN_POINT('Ctrl Pts',(4.47691345301017,12.2,9.435054510098));
#216606=CARTESIAN_POINT('Ctrl Pts',(4.47536184573321,12.2,9.43270786251658));
#216607=CARTESIAN_POINT('Ctrl Pts',(4.47381023845626,12.2,9.43036121493518));
#216608=CARTESIAN_POINT('Ctrl Pts',(4.47229289187397,12.2,9.42805173368623));
#216609=CARTESIAN_POINT('Ctrl Pts',(4.47080977093511,12.2,9.42578034815307));
#216610=CARTESIAN_POINT('Ctrl Pts',(4.46932664986153,12.2,9.42350896241359));
#216611=CARTESIAN_POINT('Ctrl Pts',(4.46787775982046,12.2,9.42127567471935));
#216612=CARTESIAN_POINT('Ctrl Pts',(4.46646305857902,12.2,9.41908144001909));
#216613=CARTESIAN_POINT('Ctrl Pts',(4.46504835746609,12.2,9.41688720551812));
#216614=CARTESIAN_POINT('Ctrl Pts',(4.46366784748975,12.2,9.41473202373166));
#216615=CARTESIAN_POINT('Ctrl Pts',(4.46232148819927,12.2,9.41261687446562));
#216616=CARTESIAN_POINT('Ctrl Pts',(4.4609751289088,12.2,9.41050172519959));
#216617=CARTESIAN_POINT('Ctrl Pts',(4.45966291889973,12.2,9.40842661078881));
#216618=CARTESIAN_POINT('Ctrl Pts',(4.45838481386135,12.2,9.40639253836094));
#216619=CARTESIAN_POINT('Ctrl Pts',(4.45710670870688,12.2,9.40435846574831));
#216620=CARTESIAN_POINT('Ctrl Pts',(4.45586271009828,12.2,9.4023654325407));
#216621=CARTESIAN_POINT('Ctrl Pts',(4.45465276586801,12.2,9.4004144772706));
#216622=CARTESIAN_POINT('Ctrl Pts',(4.45344282174763,12.2,9.39846352217771));
#216623=CARTESIAN_POINT('Ctrl Pts',(4.45226693457815,12.2,9.39655464356205));
#216624=CARTESIAN_POINT('Ctrl Pts',(4.45112504845446,12.2,9.39468890563175));
#216625=CARTESIAN_POINT('Ctrl Pts',(4.44998316233077,12.2,9.39282316770143));
#216626=CARTESIAN_POINT('Ctrl Pts',(4.44887527936268,12.2,9.39100057111765));
#216627=CARTESIAN_POINT('Ctrl Pts',(4.44780133831689,12.2,9.38922220934701));
#216628=CARTESIAN_POINT('Ctrl Pts',(4.44672739727111,12.2,9.38744384757638));
#216629=CARTESIAN_POINT('Ctrl Pts',(4.44568740268365,12.2,9.38570972190072));
#216630=CARTESIAN_POINT('Ctrl Pts',(4.44468128663456,12.2,9.38402095920899));
#216631=CARTESIAN_POINT('Ctrl Pts',(4.44317694109225,12.2,9.38149591984635));
#216632=CARTESIAN_POINT('Ctrl Pts',(4.44174833406917,12.2,9.37907228215719));
#216633=CARTESIAN_POINT('Ctrl Pts',(4.44039525799994,12.2,9.37675396799998));
#216634=CARTESIAN_POINT('Ctrl Pts',(4.44039525799994,15.2,9.37675396799998));
#216635=CARTESIAN_POINT('Ctrl Pts',(4.44129586096445,15.2,9.37829703024913));
#216636=CARTESIAN_POINT('Ctrl Pts',(4.44222992819487,15.2,9.37988675810253));
#216637=CARTESIAN_POINT('Ctrl Pts',(4.44319751513558,15.2,9.38152198206248));
#216638=CARTESIAN_POINT('Ctrl Pts',(4.44416976826961,15.2,9.38316509189892));
#216639=CARTESIAN_POINT('Ctrl Pts',(4.4451758658233,15.2,9.38485414143403));
#216640=CARTESIAN_POINT('Ctrl Pts',(4.44621587810058,15.2,9.38658798545109));
#216641=CARTESIAN_POINT('Ctrl Pts',(4.4472558902834,15.2,9.38832182931068));
#216642=CARTESIAN_POINT('Ctrl Pts',(4.44832981474848,15.2,9.39010046854946));
#216643=CARTESIAN_POINT('Ctrl Pts',(4.44943771295822,15.2,9.39192279148324));
#216644=CARTESIAN_POINT('Ctrl Pts',(4.45054561116795,15.2,9.39374511441702));
#216645=CARTESIAN_POINT('Ctrl Pts',(4.45168748333048,15.2,9.39561112227516));
#216646=CARTESIAN_POINT('Ctrl Pts',(4.45286338542788,15.2,9.39751973529871));
#216647=CARTESIAN_POINT('Ctrl Pts',(4.45403928763209,15.2,9.39942834849564));
#216648=CARTESIAN_POINT('Ctrl Pts',(4.45524921742371,15.2,9.40137956636406));
#216649=CARTESIAN_POINT('Ctrl Pts',(4.45649322957716,15.2,9.40337233972547));
#216650=CARTESIAN_POINT('Ctrl Pts',(4.4577372416176,15.2,9.40536511290588));
#216651=CARTESIAN_POINT('Ctrl Pts',(4.45901533463377,15.2,9.40739944247505));
#216652=CARTESIAN_POINT('Ctrl Pts',(4.46032755500882,15.2,9.40947430399253));
#216653=CARTESIAN_POINT('Ctrl Pts',(4.46163977538387,15.2,9.41154916551003));
#216654=CARTESIAN_POINT('Ctrl Pts',(4.4629861253431,15.2,9.413664564196));
#216655=CARTESIAN_POINT('Ctrl Pts',(4.46436664545812,15.2,9.41581950061597));
#216656=CARTESIAN_POINT('Ctrl Pts',(4.46574716569854,15.2,9.41797443723169));
#216657=CARTESIAN_POINT('Ctrl Pts',(4.46716185739318,15.2,9.42016891470231));
#216658=CARTESIAN_POINT('Ctrl Pts',(4.46861075764116,15.2,9.42240196349333));
#216659=CARTESIAN_POINT('Ctrl Pts',(4.47005965775753,15.2,9.42463501208152));
#216660=CARTESIAN_POINT('Ctrl Pts',(4.47154276904471,15.2,9.42690663270821));
#216661=CARTESIAN_POINT('Ctrl Pts',(4.47306012507439,15.2,9.42921588212593));
#216662=CARTESIAN_POINT('Ctrl Pts',(4.47457748110407,15.2,9.43152513154365));
#216663=CARTESIAN_POINT('Ctrl Pts',(4.47612908118104,15.2,9.43387200857503));
#216664=CARTESIAN_POINT('Ctrl Pts',(4.47771495737194,15.2,9.43625559515351));
#216665=CARTESIAN_POINT('Ctrl Pts',(4.47930083356283,15.2,9.43863918173199));
#216666=CARTESIAN_POINT('Ctrl Pts',(4.48092098619868,15.2,9.4410594736239));
#216667=CARTESIAN_POINT('Ctrl Pts',(4.48257544230289,15.2,9.44351558119889));
#216668=CARTESIAN_POINT('Ctrl Pts',(4.48422989855739,15.2,9.44597168899697));
#216669=CARTESIAN_POINT('Ctrl Pts',(4.48591865848186,15.2,9.44846360505688));
#216670=CARTESIAN_POINT('Ctrl Pts',(4.48764174657727,15.2,9.45099045911279));
#216671=CARTESIAN_POINT('Ctrl Pts',(4.48936483451616,15.2,9.45351731293916));
#216672=CARTESIAN_POINT('Ctrl Pts',(4.49112224943113,15.2,9.4560791013147));
#216673=CARTESIAN_POINT('Ctrl Pts',(4.49291401345741,15.2,9.45867497223209));
#216674=CARTESIAN_POINT('Ctrl Pts',(4.49470577748369,15.2,9.46127084314946));
#216675=CARTESIAN_POINT('Ctrl Pts',(4.49653188877539,15.2,9.46390079565037));
#216676=CARTESIAN_POINT('Ctrl Pts',(4.49839236678877,15.2,9.46656399296798));
#216677=CARTESIAN_POINT('Ctrl Pts',(4.50025284497113,15.2,9.4692271905275));
#216678=CARTESIAN_POINT('Ctrl Pts',(4.50214768849854,15.2,9.47192363600699));
#216679=CARTESIAN_POINT('Ctrl Pts',(4.50407691260518,15.2,9.47465251140713));
#216680=CARTESIAN_POINT('Ctrl Pts',(4.50600613653657,15.2,9.47738138655938));
#216681=CARTESIAN_POINT('Ctrl Pts',(4.50796974130426,15.2,9.48014269284589));
#216682=CARTESIAN_POINT('Ctrl Pts',(4.50996773632398,15.2,9.482935633007));
#216683=CARTESIAN_POINT('Ctrl Pts',(4.51196573134371,15.2,9.48572857316812));
#216684=CARTESIAN_POINT('Ctrl Pts',(4.51399811724373,15.2,9.48855314519458));
#216685=CARTESIAN_POINT('Ctrl Pts',(4.51606490324962,15.2,9.49140857242204));
#216686=CARTESIAN_POINT('Ctrl Pts',(4.51813168944324,15.2,9.49426399990887));
#216687=CARTESIAN_POINT('Ctrl Pts',(4.52023287545651,15.2,9.49715028053412));
#216688=CARTESIAN_POINT('Ctrl Pts',(4.52236846493156,15.2,9.50006665325712));
#216689=CARTESIAN_POINT('Ctrl Pts',(4.52450405421262,15.2,9.50298302571523));
#216690=CARTESIAN_POINT('Ctrl Pts',(4.52667405002997,15.2,9.50592948849973));
#216691=CARTESIAN_POINT('Ctrl Pts',(4.52887845194988,15.2,9.50890529697493));
#216692=CARTESIAN_POINT('Ctrl Pts',(4.53108285386978,15.2,9.51188110545013));
#216693=CARTESIAN_POINT('Ctrl Pts',(4.53332166255942,15.2,9.51488625826685));
#216694=CARTESIAN_POINT('Ctrl Pts',(4.53559487950507,15.2,9.5179200259732));
#216695=CARTESIAN_POINT('Ctrl Pts',(4.53824696607933,15.2,9.52145942181432));
#216696=CARTESIAN_POINT('Ctrl Pts',(4.54094588222936,15.2,9.52503776449918));
#216697=CARTESIAN_POINT('Ctrl Pts',(4.54369162750822,15.2,9.52865391895827));
#216698=CARTESIAN_POINT('Ctrl Pts',(4.54604512333937,15.2,9.53175347976232));
#216699=CARTESIAN_POINT('Ctrl Pts',(4.54843302198461,15.2,9.53488082217843));
#216700=CARTESIAN_POINT('Ctrl Pts',(4.55085531901565,15.2,9.53803524796986));
#216701=CARTESIAN_POINT('Ctrl Pts',(4.55287389994818,15.2,9.5406639362249));
#216702=CARTESIAN_POINT('Ctrl Pts',(4.55491636724948,15.2,9.5433114314989));
#216703=CARTESIAN_POINT('Ctrl Pts',(4.55698271808156,15.2,9.54597733656737));
#216704=CARTESIAN_POINT('Ctrl Pts',(4.55904906891363,15.2,9.54864324163583));
#216705=CARTESIAN_POINT('Ctrl Pts',(4.56113930236859,15.2,9.55132755895761));
#216706=CARTESIAN_POINT('Ctrl Pts',(4.56325341160343,15.2,9.55402989708165));
#216707=CARTESIAN_POINT('Ctrl Pts',(4.56579034259306,15.2,9.55727270271265));
#216708=CARTESIAN_POINT('Ctrl Pts',(4.56836165881291,15.2,9.56054145658733));
#216709=CARTESIAN_POINT('Ctrl Pts',(4.57096734271587,15.2,9.56383549838256));
#216710=CARTESIAN_POINT('Ctrl Pts',(4.57313874604725,15.2,9.56658053331167));
#216711=CARTESIAN_POINT('Ctrl Pts',(4.57533401857269,15.2,9.56934312933219));
#216712=CARTESIAN_POINT('Ctrl Pts',(4.5775531510013,15.2,9.57212290863635));
#216713=CARTESIAN_POINT('Ctrl Pts',(4.57977228342991,15.2,9.57490268794052));
#216714=CARTESIAN_POINT('Ctrl Pts',(4.58201527541966,15.2,9.57769965287838));
#216715=CARTESIAN_POINT('Ctrl Pts',(4.58428211796182,15.2,9.5805134306567));
#216716=CARTESIAN_POINT('Ctrl Pts',(4.58654896050399,15.2,9.58332720843501));
#216717=CARTESIAN_POINT('Ctrl Pts',(4.58883965464435,15.2,9.58615780035358));
#216718=CARTESIAN_POINT('Ctrl Pts',(4.59115418790699,15.2,9.58900484125551));
#216719=CARTESIAN_POINT('Ctrl Pts',(4.59346872116964,15.2,9.59185188215743));
#216720=CARTESIAN_POINT('Ctrl Pts',(4.59580709517458,15.2,9.59471537239036));
#216721=CARTESIAN_POINT('Ctrl Pts',(4.59816929760388,15.2,9.59759495252839));
#216722=CARTESIAN_POINT('Ctrl Pts',(4.60053150003318,15.2,9.60047453266643));
#216723=CARTESIAN_POINT('Ctrl Pts',(4.60291753218211,15.2,9.60337020335182));
#216724=CARTESIAN_POINT('Ctrl Pts',(4.60532737899857,15.2,9.60628161024002));
#216725=CARTESIAN_POINT('Ctrl Pts',(4.60773722581503,15.2,9.60919301712823));
#216726=CARTESIAN_POINT('Ctrl Pts',(4.61017089048876,15.2,9.61212016044438));
#216727=CARTESIAN_POINT('Ctrl Pts',(4.61262835701655,15.2,9.61506269224995));
#216728=CARTESIAN_POINT('Ctrl Pts',(4.61606881020903,15.2,9.6191822368419));
#216729=CARTESIAN_POINT('Ctrl Pts',(4.61955591681464,15.2,9.62333194003229));
#216730=CARTESIAN_POINT('Ctrl Pts',(4.62308963828464,15.2,9.62751086807151));
#216731=CARTESIAN_POINT('Ctrl Pts',(4.62561372500964,15.2,9.63049581662447));
#216732=CARTESIAN_POINT('Ctrl Pts',(4.62816159339544,15.2,9.63349567338195));
#216733=CARTESIAN_POINT('Ctrl Pts',(4.63073322832793,15.2,9.6365101036609));
#216734=CARTESIAN_POINT('Ctrl Pts',(4.63330486326042,15.2,9.63952453393987));
#216735=CARTESIAN_POINT('Ctrl Pts',(4.63590026575164,15.2,9.64255353824684));
#216736=CARTESIAN_POINT('Ctrl Pts',(4.63851941735081,15.2,9.64559678512302));
#216737=CARTESIAN_POINT('Ctrl Pts',(4.64113856894998,15.2,9.64864003199919));
#216738=CARTESIAN_POINT('Ctrl Pts',(4.64378147109676,15.2,9.65169752175614));
#216739=CARTESIAN_POINT('Ctrl Pts',(4.64644810589035,15.2,9.65476892641003));
#216740=CARTESIAN_POINT('Ctrl Pts',(4.64911474039328,15.2,9.65784033072913));
#216741=CARTESIAN_POINT('Ctrl Pts',(4.65180510653709,15.2,9.66092565371126));
#216742=CARTESIAN_POINT('Ctrl Pts',(4.65451918762822,15.2,9.66402456955295));
#216743=CARTESIAN_POINT('Ctrl Pts',(4.65723326901519,15.2,9.66712348573241));
#216744=CARTESIAN_POINT('Ctrl Pts',(4.65997106375728,15.2,9.67023599479217));
#216745=CARTESIAN_POINT('Ctrl Pts',(4.66273255438036,15.2,9.67336178333277));
#216746=CARTESIAN_POINT('Ctrl Pts',(4.66494174699921,15.2,9.67586241430154));
#216747=CARTESIAN_POINT('Ctrl Pts',(4.66716610339692,15.2,9.67837154230579));
#216748=CARTESIAN_POINT('Ctrl Pts',(4.66940561475142,15.2,9.68088900751001));
#216749=CARTESIAN_POINT('Ctrl Pts',(4.67164512580078,15.2,9.68340647237122));
#216750=CARTESIAN_POINT('Ctrl Pts',(4.67389979117421,15.2,9.68593227509919));
#216751=CARTESIAN_POINT('Ctrl Pts',(4.67616960015378,15.2,9.68846625533565));
#216752=CARTESIAN_POINT('Ctrl Pts',(4.6784394094426,15.2,9.69100023591736));
#216753=CARTESIAN_POINT('Ctrl Pts',(4.68072436322175,15.2,9.69354239602485));
#216754=CARTESIAN_POINT('Ctrl Pts',(4.68302444929155,15.2,9.69609257777496));
#216755=CARTESIAN_POINT('Ctrl Pts',(4.6858995567221,15.2,9.69928030478884));
#216756=CARTESIAN_POINT('Ctrl Pts',(4.68879830853259,15.2,9.7024805646093));
#216757=CARTESIAN_POINT('Ctrl Pts',(4.69172068493481,15.2,9.70569305677671));
#216758=CARTESIAN_POINT('Ctrl Pts',(4.69405858586547,15.2,9.70826305030053));
#216759=CARTESIAN_POINT('Ctrl Pts',(4.69641160494672,15.2,9.71084087169215));
#216760=CARTESIAN_POINT('Ctrl Pts',(4.6987797318627,15.2,9.7134263678689));
#216761=CARTESIAN_POINT('Ctrl Pts',(4.70114785910134,15.2,9.71601186439792));
#216762=CARTESIAN_POINT('Ctrl Pts',(4.70353109304973,15.2,9.71860503601378));
#216763=CARTESIAN_POINT('Ctrl Pts',(4.70592942179154,15.2,9.72120573126662));
#216764=CARTESIAN_POINT('Ctrl Pts',(4.70892733255542,15.2,9.7244566001555));
#216765=CARTESIAN_POINT('Ctrl Pts',(4.71194883064877,15.2,9.72771922445351));
#216766=CARTESIAN_POINT('Ctrl Pts',(4.71499388975988,15.2,9.73099331176007));
#216767=CARTESIAN_POINT('Ctrl Pts',(4.71803894887099,15.2,9.73426739906664));
#216768=CARTESIAN_POINT('Ctrl Pts',(4.72110757203435,15.2,9.73755295130394));
#216769=CARTESIAN_POINT('Ctrl Pts',(4.72419973099392,15.2,9.74084967616563));
#216770=CARTESIAN_POINT('Ctrl Pts',(4.72667345795934,15.2,9.74348705583938));
#216771=CARTESIAN_POINT('Ctrl Pts',(4.72916224867453,15.2,9.7461315879367));
#216772=CARTESIAN_POINT('Ctrl Pts',(4.73166609035718,15.2,9.7487831261081));
#216773=CARTESIAN_POINT('Ctrl Pts',(4.73416993238098,15.2,9.75143466464077));
#216774=CARTESIAN_POINT('Ctrl Pts',(4.73668882432696,15.2,9.7540932086555));
#216775=CARTESIAN_POINT('Ctrl Pts',(4.73922275497661,15.2,9.75675861403511));
#216776=CARTESIAN_POINT('Ctrl Pts',(4.74175668528101,15.2,9.75942401905156));
#216777=CARTESIAN_POINT('Ctrl Pts',(4.74430565323905,15.2,9.76209628610942));
#216778=CARTESIAN_POINT('Ctrl Pts',(4.74686964430567,15.2,9.76477527111195));
#216779=CARTESIAN_POINT('Ctrl Pts',(4.74943363572164,15.2,9.76745425647947));
#216780=CARTESIAN_POINT('Ctrl Pts',(4.75201265215018,15.2,9.77013996059767));
#216781=CARTESIAN_POINT('Ctrl Pts',(4.75460667745821,15.2,9.77283224129996));
#216782=CARTESIAN_POINT('Ctrl Pts',(4.75720070276625,15.2,9.77552452200223));
#216783=CARTESIAN_POINT('Ctrl Pts',(4.75980973826216,15.2,9.77822337934974));
#216784=CARTESIAN_POINT('Ctrl Pts',(4.76243376962892,15.2,9.78092867394228));
#216785=CARTESIAN_POINT('Ctrl Pts',(4.76505780063815,15.2,9.78363396816621));
#216786=CARTESIAN_POINT('Ctrl Pts',(4.76769682747524,15.2,9.78634569853296));
#216787=CARTESIAN_POINT('Ctrl Pts',(4.77035083571475,15.2,9.78906372748978));
#216788=CARTESIAN_POINT('Ctrl Pts',(4.77300484431586,15.2,9.79178175681692));
#216789=CARTESIAN_POINT('Ctrl Pts',(4.77567383341869,15.2,9.79450608352196));
#216790=CARTESIAN_POINT('Ctrl Pts',(4.77835778945539,15.2,9.79723657150473));
#216791=CARTESIAN_POINT('Ctrl Pts',(4.7810417451264,15.2,9.79996705911548));
#216792=CARTESIAN_POINT('Ctrl Pts',(4.78374066790933,15.2,9.80270370614763));
#216793=CARTESIAN_POINT('Ctrl Pts',(4.78645454151983,15.2,9.80544637853414));
#216794=CARTESIAN_POINT('Ctrl Pts',(4.78984688381027,15.2,9.80887471929753));
#216795=CARTESIAN_POINT('Ctrl Pts',(4.79326258814358,15.2,9.81231247312135));
#216796=CARTESIAN_POINT('Ctrl Pts',(4.79670162454801,15.2,9.81575937799808));
#216797=CARTESIAN_POINT('Ctrl Pts',(4.79945285382151,15.2,9.81851690204976));
#216798=CARTESIAN_POINT('Ctrl Pts',(4.80221901512927,15.2,9.8212802809762));
#216799=CARTESIAN_POINT('Ctrl Pts',(4.80500009317127,15.2,9.82404938496105));
#216800=CARTESIAN_POINT('Ctrl Pts',(4.8084764405343,15.2,9.82751076475346));
#216801=CARTESIAN_POINT('Ctrl Pts',(4.81197609696989,15.2,9.83098108580431));
#216802=CARTESIAN_POINT('Ctrl Pts',(4.8154990277357,15.2,9.83446009247169));
#216803=CARTESIAN_POINT('Ctrl Pts',(4.8190219581175,15.2,9.83793909875986));
#216804=CARTESIAN_POINT('Ctrl Pts',(4.82256816631288,15.2,9.84142679066334));
#216805=CARTESIAN_POINT('Ctrl Pts',(4.82613761828301,15.2,9.84492291430934));
#216806=CARTESIAN_POINT('Ctrl Pts',(4.82899318032599,15.2,9.84771981368343));
#216807=CARTESIAN_POINT('Ctrl Pts',(4.83186361936764,15.2,9.85052210777751));
#216808=CARTESIAN_POINT('Ctrl Pts',(4.83474891802488,15.2,9.85332967054163));
#216809=CARTESIAN_POINT('Ctrl Pts',(4.83763421668212,15.2,9.85613723330575));
#216810=CARTESIAN_POINT('Ctrl Pts',(4.84053437637169,15.2,9.85895006197329));
#216811=CARTESIAN_POINT('Ctrl Pts',(4.8434493789765,15.2,9.86176803146071));
#216812=CARTESIAN_POINT('Ctrl Pts',(4.84636438118414,15.2,9.86458600056417));
#216813=CARTESIAN_POINT('Ctrl Pts',(4.8492942270482,15.2,9.86740911033366));
#216814=CARTESIAN_POINT('Ctrl Pts',(4.85223889875097,15.2,9.87023723276882));
#216815=CARTESIAN_POINT('Ctrl Pts',(4.85665590650573,15.2,9.87447941661421));
#216816=CARTESIAN_POINT('Ctrl Pts',(4.86110627421804,15.2,9.87873287995751));
#216817=CARTESIAN_POINT('Ctrl Pts',(4.86558994280284,15.2,9.88299720280182));
#216818=CARTESIAN_POINT('Ctrl Pts',(4.86932633342592,15.2,9.88655080530119));
#216819=CARTESIAN_POINT('Ctrl Pts',(4.87308584981257,15.2,9.89011194773937));
#216820=CARTESIAN_POINT('Ctrl Pts',(4.87686845800512,15.2,9.89368039030822));
#216821=CARTESIAN_POINT('Ctrl Pts',(4.88065106619768,15.2,9.89724883287706));
#216822=CARTESIAN_POINT('Ctrl Pts',(4.88445676508805,15.2,9.90082457442224));
#216823=CARTESIAN_POINT('Ctrl Pts',(4.88828552159717,15.2,9.90440737876741));
#216824=CARTESIAN_POINT('Ctrl Pts',(4.8913485269714,15.2,9.90727362239975));
#216825=CARTESIAN_POINT('Ctrl Pts',(4.89442628799722,15.2,9.91014438511696));
#216826=CARTESIAN_POINT('Ctrl Pts',(4.89751878677784,15.2,9.91301954671838));
#216827=CARTESIAN_POINT('Ctrl Pts',(4.90061128513711,15.2,9.91589470792809));
#216828=CARTESIAN_POINT('Ctrl Pts',(4.90371852174617,15.2,9.91877426834242));
#216829=CARTESIAN_POINT('Ctrl Pts',(4.90684047848945,15.2,9.92165810699513));
#216830=CARTESIAN_POINT('Ctrl Pts',(4.91074292473758,15.2,9.9252629056057));
#216831=CARTESIAN_POINT('Ctrl Pts',(4.91466836974595,15.2,9.92887439220526));
#216832=CARTESIAN_POINT('Ctrl Pts',(4.91861677806661,15.2,9.93249233183));
#216833=CARTESIAN_POINT('Ctrl Pts',(4.9217755048953,15.2,9.93538668368754));
#216834=CARTESIAN_POINT('Ctrl Pts',(4.92494892836094,15.2,9.93828516656772));
#216835=CARTESIAN_POINT('Ctrl Pts',(4.92813702903565,15.2,9.94118766350395));
#216836=CARTESIAN_POINT('Ctrl Pts',(4.93132512927599,15.2,9.94409016004472));
#216837=CARTESIAN_POINT('Ctrl Pts',(4.93452790748004,15.2,9.94699667113466));
#216838=CARTESIAN_POINT('Ctrl Pts',(4.93774534371551,15.2,9.94990707900746));
#216839=CARTESIAN_POINT('Ctrl Pts',(4.94096278038937,15.2,9.95281748727679));
#216840=CARTESIAN_POINT('Ctrl Pts',(4.94419487580203,15.2,9.95573179223521));
#216841=CARTESIAN_POINT('Ctrl Pts',(4.94744161049377,15.2,9.95864988051863));
#216842=CARTESIAN_POINT('Ctrl Pts',(4.95068834474315,15.2,9.96156796840446));
#216843=CARTESIAN_POINT('Ctrl Pts',(4.95394971775303,15.2,9.96448983825286));
#216844=CARTESIAN_POINT('Ctrl Pts',(4.95722571120594,15.2,9.96741537551332));
#216845=CARTESIAN_POINT('Ctrl Pts',(4.96132070335684,15.2,9.97107229738784));
#216846=CARTESIAN_POINT('Ctrl Pts',(4.96543853908239,15.2,9.97473495087619));
#216847=CARTESIAN_POINT('Ctrl Pts',(4.96957917894163,15.2,9.97840311448684));
#216848=CARTESIAN_POINT('Ctrl Pts',(4.97289169100955,15.2,9.98133764553529));
#216849=CARTESIAN_POINT('Ctrl Pts',(4.97621879890759,15.2,9.98427570356997));
#216850=CARTESIAN_POINT('Ctrl Pts',(4.97956048149383,15.2,9.98721717524365));
#216851=CARTESIAN_POINT('Ctrl Pts',(4.98290216362477,15.2,9.99015864651655));
#216852=CARTESIAN_POINT('Ctrl Pts',(4.98625842227304,15.2,9.99310353262039));
#216853=CARTESIAN_POINT('Ctrl Pts',(4.98962923394043,15.2,9.99605172126794));
#216854=CARTESIAN_POINT('Ctrl Pts',(4.99215734326506,15.2,9.99826286325571));
#216855=CARTESIAN_POINT('Ctrl Pts',(4.99469364095036,15.2,10.000475864294));
#216856=CARTESIAN_POINT('Ctrl Pts',(4.99723811711292,15.2,10.0026906762411));
#216857=CARTESIAN_POINT('Ctrl Pts',(4.99978259281324,15.2,10.0049054877859));
#216858=CARTESIAN_POINT('Ctrl Pts',(5.00233524613814,15.2,10.0071221102223));
#216859=CARTESIAN_POINT('Ctrl Pts',(5.00489607079583,15.2,10.0093404982668));
#216860=CARTESIAN_POINT('Ctrl Pts',(5.00916411204702,15.2,10.0130378118087));
#216861=CARTESIAN_POINT('Ctrl Pts',(5.01345484510585,15.2,10.0167400291948));
#216862=CARTESIAN_POINT('Ctrl Pts',(5.01776823497569,15.2,10.020446937922));
#216863=CARTESIAN_POINT('Ctrl Pts',(5.02121894658947,15.2,10.0234124646613));
#216864=CARTESIAN_POINT('Ctrl Pts',(5.02468415591764,15.2,10.0263809927113));
#216865=CARTESIAN_POINT('Ctrl Pts',(5.02816384396556,15.2,10.0293524160238));
#216866=CARTESIAN_POINT('Ctrl Pts',(5.03164353248757,15.2,10.0323238397411));
#216867=CARTESIAN_POINT('Ctrl Pts',(5.03513769823358,15.2,10.0352981583476));
#216868=CARTESIAN_POINT('Ctrl Pts',(5.03864632153686,15.2,10.03827526351));
#216869=CARTESIAN_POINT('Ctrl Pts',(5.04127778877529,15.2,10.0405080921791));
#216870=CARTESIAN_POINT('Ctrl Pts',(5.04391738723644,15.2,10.0427424896064));
#216871=CARTESIAN_POINT('Ctrl Pts',(5.04656510898563,15.2,10.044978410202));
#216872=CARTESIAN_POINT('Ctrl Pts',(5.04921283073482,15.2,10.0472143307976));
#216873=CARTESIAN_POINT('Ctrl Pts',(5.05186867604886,15.2,10.0494517744525));
#216874=CARTESIAN_POINT('Ctrl Pts',(5.0545326352558,15.2,10.0516906975063));
#216875=CARTESIAN_POINT('Ctrl Pts',(5.05719659446274,15.2,10.0539296205601));
#216876=CARTESIAN_POINT('Ctrl Pts',(5.0598686672393,15.2,10.0561700222872));
#216877=CARTESIAN_POINT('Ctrl Pts',(5.06254884547455,15.2,10.0584118579973));
#216878=CARTESIAN_POINT('Ctrl Pts',(5.0652290237098,15.2,10.0606536937074));
#216879=CARTESIAN_POINT('Ctrl Pts',(5.06791730711116,15.2,10.0628969655924));
#216880=CARTESIAN_POINT('Ctrl Pts',(5.07061368588708,15.2,10.0651416272606));
#216881=CARTESIAN_POINT('Ctrl Pts',(5.0751076506769,15.2,10.068882730177));
#216882=CARTESIAN_POINT('Ctrl Pts',(5.07962410405897,15.2,10.0726276958612));
#216883=CARTESIAN_POINT('Ctrl Pts',(5.0841630040064,15.2,10.0763763222982));
#216884=CARTESIAN_POINT('Ctrl Pts',(5.08688634387591,15.2,10.0786254980787));
#216885=CARTESIAN_POINT('Ctrl Pts',(5.08961776491998,15.2,10.0808759921577));
#216886=CARTESIAN_POINT('Ctrl Pts',(5.09235725619435,15.2,10.0831277607841));
#216887=CARTESIAN_POINT('Ctrl Pts',(5.09509674796639,15.2,10.0853795298195));
#216888=CARTESIAN_POINT('Ctrl Pts',(5.09784431064905,15.2,10.087632573747));
#216889=CARTESIAN_POINT('Ctrl Pts',(5.10059993634229,15.2,10.0898868497414));
#216890=CARTESIAN_POINT('Ctrl Pts',(5.10427410309893,15.2,10.0928925503848));
#216891=CARTESIAN_POINT('Ctrl Pts',(5.10796260106763,15.2,10.0959004401946));
#216892=CARTESIAN_POINT('Ctrl Pts',(5.11166541043065,15.2,10.0989104195039));
#216893=CARTESIAN_POINT('Ctrl Pts',(5.11444251757904,15.2,10.1011679040885));
#216894=CARTESIAN_POINT('Ctrl Pts',(5.11722767394358,15.2,10.1034265623563));
#216895=CARTESIAN_POINT('Ctrl Pts',(5.12002087017431,15.2,10.1056863534823));
#216896=CARTESIAN_POINT('Ctrl Pts',(5.12374513215358,15.2,10.1086994085908));
#216897=CARTESIAN_POINT('Ctrl Pts',(5.12748368738361,15.2,10.1117144781433));
#216898=CARTESIAN_POINT('Ctrl Pts',(5.13123651399412,15.2,10.1147314600437));
#216899=CARTESIAN_POINT('Ctrl Pts',(5.13405113369634,15.2,10.1169941962634));
#216900=CARTESIAN_POINT('Ctrl Pts',(5.13687378073734,15.2,10.1192580093033));
#216901=CARTESIAN_POINT('Ctrl Pts',(5.13970444548066,15.2,10.1215228564813));
#216902=CARTESIAN_POINT('Ctrl Pts',(5.14253511022397,15.2,10.1237877036593));
#216903=CARTESIAN_POINT('Ctrl Pts',(5.14537379292719,15.2,10.1260535848853));
#216904=CARTESIAN_POINT('Ctrl Pts',(5.1482204836564,15.2,10.1283204594696));
#216905=CARTESIAN_POINT('Ctrl Pts',(5.15106717438561,15.2,10.1305873340538));
#216906=CARTESIAN_POINT('Ctrl Pts',(5.15392187338094,15.2,10.1328552009379));
#216907=CARTESIAN_POINT('Ctrl Pts',(5.15678457060916,15.2,10.135124020022));
#216908=CARTESIAN_POINT('Ctrl Pts',(5.16060150059348,15.2,10.1381491124089));
#216909=CARTESIAN_POINT('Ctrl Pts',(5.16443265058931,15.2,10.1411758958205));
#216910=CARTESIAN_POINT('Ctrl Pts',(5.16827799776085,15.2,10.144204274277));
#216911=CARTESIAN_POINT('Ctrl Pts',(5.17212334440845,15.2,10.147232652321));
#216912=CARTESIAN_POINT('Ctrl Pts',(5.17598288599022,15.2,10.1502626236329));
#216913=CARTESIAN_POINT('Ctrl Pts',(5.17985660211654,15.2,10.153294092996));
#216914=CARTESIAN_POINT('Ctrl Pts',(5.18373031877066,15.2,10.1563255627722));
#216915=CARTESIAN_POINT('Ctrl Pts',(5.18761820836222,15.2,10.1593585295041));
#216916=CARTESIAN_POINT('Ctrl Pts',(5.19152024774155,15.2,10.162392898725));
#216917=CARTESIAN_POINT('Ctrl Pts',(5.19444677701023,15.2,10.164668675434));
#216918=CARTESIAN_POINT('Ctrl Pts',(5.19738126682024,15.2,10.1669452418346));
#216919=CARTESIAN_POINT('Ctrl Pts',(5.20032370467096,15.2,10.1692225565018));
#216920=CARTESIAN_POINT('Ctrl Pts',(5.20326614252168,15.2,10.171499871169));
#216921=CARTESIAN_POINT('Ctrl Pts',(5.2062165312882,15.2,10.1737779345448));
#216922=CARTESIAN_POINT('Ctrl Pts',(5.20917485866094,15.2,10.1760567053258));
#216923=CARTESIAN_POINT('Ctrl Pts',(5.21213318603366,15.2,10.1783354761067));
#216924=CARTESIAN_POINT('Ctrl Pts',(5.21509945217733,15.2,10.1806149539358));
#216925=CARTESIAN_POINT('Ctrl Pts',(5.21807364785985,15.2,10.1828950987696));
#216926=CARTESIAN_POINT('Ctrl Pts',(5.2210478440827,15.2,10.1851752440175));
#216927=CARTESIAN_POINT('Ctrl Pts',(5.22402996911609,15.2,10.1874560580323));
#216928=CARTESIAN_POINT('Ctrl Pts',(5.22702001488507,15.2,10.1897375041973));
#216929=CARTESIAN_POINT('Ctrl Pts',(5.23001006011085,15.2,10.1920189499479));
#216930=CARTESIAN_POINT('Ctrl Pts',(5.23300802603619,15.2,10.194301028465));
#216931=CARTESIAN_POINT('Ctrl Pts',(5.23601390080267,15.2,10.1965836989655));
#216932=CARTESIAN_POINT('Ctrl Pts',(5.24102369226215,15.2,10.2003881499378));
#216933=CARTESIAN_POINT('Ctrl Pts',(5.24605545522705,15.2,10.2041942383572));
#216934=CARTESIAN_POINT('Ctrl Pts',(5.25110913436996,15.2,10.2080017559086));
#216935=CARTESIAN_POINT('Ctrl Pts',(5.25414134174553,15.2,10.2102862663565));
#216936=CARTESIAN_POINT('Ctrl Pts',(5.25718143818119,15.2,10.2125712912946));
#216937=CARTESIAN_POINT('Ctrl Pts',(5.26022941958503,15.2,10.2148568145085));
#216938=CARTESIAN_POINT('Ctrl Pts',(5.26327740098887,15.2,10.2171423377224));
#216939=CARTESIAN_POINT('Ctrl Pts',(5.26633327020158,15.2,10.2194283609115));
#216940=CARTESIAN_POINT('Ctrl Pts',(5.26939701799994,15.2,10.221714878));
#216941=CARTESIAN_POINT('Origin',(-5.66257110645729E-14,15.2,-1.77635683940025E-14));
#216942=CARTESIAN_POINT('',(4.0426091163045,15.2,9.55499537093196));
#216943=CARTESIAN_POINT('',(4.0426091163045,12.2,9.55499537093196));
#216944=CARTESIAN_POINT('',(4.04260911599994,15.2,9.55499537099998));
#216945=CARTESIAN_POINT('Origin',(-5.66257110645729E-14,12.2,-1.77635683940025E-14));
#216946=CARTESIAN_POINT('Origin',(-5.66257110645729E-14,15.2,-1.77635683940025E-14));
#216947=CARTESIAN_POINT('Origin',(-5.66257110645729E-14,15.2,-1.77635683940025E-14));
#216948=CARTESIAN_POINT('',(4.12144986799994,15.2,10.736091048));
#216949=CARTESIAN_POINT('',(3.76106045499994,15.2,10.867585944));
#216950=CARTESIAN_POINT('Origin',(-5.66257110645729E-14,15.2,-1.77635683940025E-14));
#216951=CARTESIAN_POINT('',(3.76106045499994,12.2,10.867585944));
#216952=CARTESIAN_POINT('',(3.76106045499994,15.2,10.867585944));
#216953=CARTESIAN_POINT('',(4.12144986799994,12.2,10.736091048));
#216954=CARTESIAN_POINT('Origin',(-5.66257110645729E-14,12.2,-1.77635683940025E-14));
#216955=CARTESIAN_POINT('',(4.12144986799994,15.2,10.736091048));
#216956=CARTESIAN_POINT('Ctrl Pts',(3.76106045499994,15.2,10.867585944));
#216957=CARTESIAN_POINT('Ctrl Pts',(3.76106045499994,11.6,10.867585944));
#216958=CARTESIAN_POINT('Ctrl Pts',(3.76051902299994,15.2,10.867046091));
#216959=CARTESIAN_POINT('Ctrl Pts',(3.76051902299994,11.6,10.867046091));
#216960=CARTESIAN_POINT('Ctrl Pts',(3.75943667399994,15.2,10.865966495));
#216961=CARTESIAN_POINT('Ctrl Pts',(3.75943667399994,11.6,10.865966495));
#216962=CARTESIAN_POINT('Ctrl Pts',(3.75781469799994,15.2,10.864347421));
#216963=CARTESIAN_POINT('Ctrl Pts',(3.75781469799994,11.6,10.864347421));
#216964=CARTESIAN_POINT('Ctrl Pts',(3.75565515599994,15.2,10.862189302));
#216965=CARTESIAN_POINT('Ctrl Pts',(3.75565515599994,11.6,10.862189302));
#216966=CARTESIAN_POINT('Ctrl Pts',(3.75296088399994,15.2,10.85949273));
#216967=CARTESIAN_POINT('Ctrl Pts',(3.75296088399994,11.6,10.85949273));
#216968=CARTESIAN_POINT('Ctrl Pts',(3.75027176799994,15.2,10.856797236));
#216969=CARTESIAN_POINT('Ctrl Pts',(3.75027176799994,11.6,10.856797236));
#216970=CARTESIAN_POINT('Ctrl Pts',(3.74758780799994,15.2,10.854102822));
#216971=CARTESIAN_POINT('Ctrl Pts',(3.74758780799994,11.6,10.854102822));
#216972=CARTESIAN_POINT('Ctrl Pts',(3.74490900499994,15.2,10.85140949));
#216973=CARTESIAN_POINT('Ctrl Pts',(3.74490900499994,11.6,10.85140949));
#216974=CARTESIAN_POINT('Ctrl Pts',(3.74223535999994,15.2,10.84871725));
#216975=CARTESIAN_POINT('Ctrl Pts',(3.74223535999994,11.6,10.84871725));
#216976=CARTESIAN_POINT('Ctrl Pts',(3.73956687399994,15.2,10.846026106));
#216977=CARTESIAN_POINT('Ctrl Pts',(3.73956687399994,11.6,10.846026106));
#216978=CARTESIAN_POINT('Ctrl Pts',(3.73690354699994,15.2,10.843336071));
#216979=CARTESIAN_POINT('Ctrl Pts',(3.73690354699994,11.6,10.843336071));
#216980=CARTESIAN_POINT('Ctrl Pts',(3.73424538199994,15.2,10.840647153));
#216981=CARTESIAN_POINT('Ctrl Pts',(3.73424538199994,11.6,10.840647153));
#216982=CARTESIAN_POINT('Ctrl Pts',(3.73159237799995,15.2,10.837959365));
#216983=CARTESIAN_POINT('Ctrl Pts',(3.73159237799995,11.6,10.837959365));
#216984=CARTESIAN_POINT('Ctrl Pts',(3.72894453699994,15.2,10.835272717));
#216985=CARTESIAN_POINT('Ctrl Pts',(3.72894453699994,11.6,10.835272717));
#216986=CARTESIAN_POINT('Ctrl Pts',(3.72630186199994,15.2,10.832587221));
#216987=CARTESIAN_POINT('Ctrl Pts',(3.72630186199994,11.6,10.832587221));
#216988=CARTESIAN_POINT('Ctrl Pts',(3.72366435199994,15.2,10.829902884));
#216989=CARTESIAN_POINT('Ctrl Pts',(3.72366435199994,11.6,10.829902884));
#216990=CARTESIAN_POINT('Ctrl Pts',(3.72103200699994,15.2,10.827219716));
#216991=CARTESIAN_POINT('Ctrl Pts',(3.72103200699994,11.6,10.827219716));
#216992=CARTESIAN_POINT('Ctrl Pts',(3.71840482999994,15.2,10.824537725));
#216993=CARTESIAN_POINT('Ctrl Pts',(3.71840482999994,11.6,10.824537725));
#216994=CARTESIAN_POINT('Ctrl Pts',(3.71578282099994,15.2,10.821856919));
#216995=CARTESIAN_POINT('Ctrl Pts',(3.71578282099994,11.6,10.821856919));
#216996=CARTESIAN_POINT('Ctrl Pts',(3.71316598199994,15.2,10.819177306));
#216997=CARTESIAN_POINT('Ctrl Pts',(3.71316598199994,11.6,10.819177306));
#216998=CARTESIAN_POINT('Ctrl Pts',(3.71055431199994,15.2,10.816498895));
#216999=CARTESIAN_POINT('Ctrl Pts',(3.71055431199994,11.6,10.816498895));
#217000=CARTESIAN_POINT('Ctrl Pts',(3.70794781299994,15.2,10.813821695));
#217001=CARTESIAN_POINT('Ctrl Pts',(3.70794781299994,11.6,10.813821695));
#217002=CARTESIAN_POINT('Ctrl Pts',(3.70534648499994,15.2,10.811145713));
#217003=CARTESIAN_POINT('Ctrl Pts',(3.70534648499994,11.6,10.811145713));
#217004=CARTESIAN_POINT('Ctrl Pts',(3.70275033099994,15.2,10.808470961));
#217005=CARTESIAN_POINT('Ctrl Pts',(3.70275033099994,11.6,10.808470961));
#217006=CARTESIAN_POINT('Ctrl Pts',(3.70015935099994,15.2,10.805797449));
#217007=CARTESIAN_POINT('Ctrl Pts',(3.70015935099994,11.6,10.805797449));
#217008=CARTESIAN_POINT('Ctrl Pts',(3.69757354499994,15.2,10.803125184));
#217009=CARTESIAN_POINT('Ctrl Pts',(3.69757354499994,11.6,10.803125184));
#217010=CARTESIAN_POINT('Ctrl Pts',(3.69499291499995,15.2,10.800454179));
#217011=CARTESIAN_POINT('Ctrl Pts',(3.69499291499995,11.6,10.800454179));
#217012=CARTESIAN_POINT('Ctrl Pts',(3.69241746099994,15.2,10.797784438));
#217013=CARTESIAN_POINT('Ctrl Pts',(3.69241746099994,11.6,10.797784438));
#217014=CARTESIAN_POINT('Ctrl Pts',(3.68984718499994,15.2,10.795115974));
#217015=CARTESIAN_POINT('Ctrl Pts',(3.68984718499994,11.6,10.795115974));
#217016=CARTESIAN_POINT('Ctrl Pts',(3.68728208699994,15.2,10.792448794));
#217017=CARTESIAN_POINT('Ctrl Pts',(3.68728208699994,11.6,10.792448794));
#217018=CARTESIAN_POINT('Ctrl Pts',(3.68472216799994,15.2,10.789782909));
#217019=CARTESIAN_POINT('Ctrl Pts',(3.68472216799994,11.6,10.789782909));
#217020=CARTESIAN_POINT('Ctrl Pts',(3.68216742899994,15.2,10.787118327));
#217021=CARTESIAN_POINT('Ctrl Pts',(3.68216742899994,11.6,10.787118327));
#217022=CARTESIAN_POINT('Ctrl Pts',(3.67961787099994,15.2,10.784455057));
#217023=CARTESIAN_POINT('Ctrl Pts',(3.67961787099994,11.6,10.784455057));
#217024=CARTESIAN_POINT('Ctrl Pts',(3.67707349599994,15.2,10.781793108));
#217025=CARTESIAN_POINT('Ctrl Pts',(3.67707349599994,11.6,10.781793108));
#217026=CARTESIAN_POINT('Ctrl Pts',(3.67453430199994,15.2,10.77913249));
#217027=CARTESIAN_POINT('Ctrl Pts',(3.67453430199994,11.6,10.77913249));
#217028=CARTESIAN_POINT('Ctrl Pts',(3.67200029299994,15.2,10.776473211));
#217029=CARTESIAN_POINT('Ctrl Pts',(3.67200029299994,11.6,10.776473211));
#217030=CARTESIAN_POINT('Ctrl Pts',(3.66947146699994,15.2,10.773815282));
#217031=CARTESIAN_POINT('Ctrl Pts',(3.66947146699994,11.6,10.773815282));
#217032=CARTESIAN_POINT('Ctrl Pts',(3.66694782699994,15.2,10.771158713));
#217033=CARTESIAN_POINT('Ctrl Pts',(3.66694782699994,11.6,10.771158713));
#217034=CARTESIAN_POINT('Ctrl Pts',(3.66442937399994,15.2,10.768503511));
#217035=CARTESIAN_POINT('Ctrl Pts',(3.66442937399994,11.6,10.768503511));
#217036=CARTESIAN_POINT('Ctrl Pts',(3.66191610699994,15.2,10.765849687));
#217037=CARTESIAN_POINT('Ctrl Pts',(3.66191610699994,11.6,10.765849687));
#217038=CARTESIAN_POINT('Ctrl Pts',(3.65940802899994,15.2,10.76319725));
#217039=CARTESIAN_POINT('Ctrl Pts',(3.65940802899994,11.6,10.76319725));
#217040=CARTESIAN_POINT('Ctrl Pts',(3.65690513699994,15.2,10.760546208));
#217041=CARTESIAN_POINT('Ctrl Pts',(3.65690513699994,11.6,10.760546208));
#217042=CARTESIAN_POINT('Ctrl Pts',(3.65440743699994,15.2,10.757896573));
#217043=CARTESIAN_POINT('Ctrl Pts',(3.65440743699994,11.6,10.757896573));
#217044=CARTESIAN_POINT('Ctrl Pts',(3.65191492599994,15.2,10.755248353));
#217045=CARTESIAN_POINT('Ctrl Pts',(3.65191492599994,11.6,10.755248353));
#217046=CARTESIAN_POINT('Ctrl Pts',(3.64942760599994,15.2,10.752601556));
#217047=CARTESIAN_POINT('Ctrl Pts',(3.64942760599994,11.6,10.752601556));
#217048=CARTESIAN_POINT('Ctrl Pts',(3.64694547899994,15.2,10.749956194));
#217049=CARTESIAN_POINT('Ctrl Pts',(3.64694547899994,11.6,10.749956194));
#217050=CARTESIAN_POINT('Ctrl Pts',(3.64446854399994,15.2,10.747312275));
#217051=CARTESIAN_POINT('Ctrl Pts',(3.64446854399994,11.6,10.747312275));
#217052=CARTESIAN_POINT('Ctrl Pts',(3.64199680199994,15.2,10.744669808));
#217053=CARTESIAN_POINT('Ctrl Pts',(3.64199680199994,11.6,10.744669808));
#217054=CARTESIAN_POINT('Ctrl Pts',(3.63953025499994,15.2,10.742028805));
#217055=CARTESIAN_POINT('Ctrl Pts',(3.63953025499994,11.6,10.742028805));
#217056=CARTESIAN_POINT('Ctrl Pts',(3.63706890199994,15.2,10.739389272));
#217057=CARTESIAN_POINT('Ctrl Pts',(3.63706890199994,11.6,10.739389272));
#217058=CARTESIAN_POINT('Ctrl Pts',(3.63461274499994,15.2,10.736751222));
#217059=CARTESIAN_POINT('Ctrl Pts',(3.63461274499994,11.6,10.736751222));
#217060=CARTESIAN_POINT('Ctrl Pts',(3.63216178499994,15.2,10.734114662));
#217061=CARTESIAN_POINT('Ctrl Pts',(3.63216178499994,11.6,10.734114662));
#217062=CARTESIAN_POINT('Ctrl Pts',(3.62971602199994,15.2,10.731479602));
#217063=CARTESIAN_POINT('Ctrl Pts',(3.62971602199994,11.6,10.731479602));
#217064=CARTESIAN_POINT('Ctrl Pts',(3.62727545699994,15.2,10.728846054));
#217065=CARTESIAN_POINT('Ctrl Pts',(3.62727545699994,11.6,10.728846054));
#217066=CARTESIAN_POINT('Ctrl Pts',(3.62484009099994,15.2,10.726214025));
#217067=CARTESIAN_POINT('Ctrl Pts',(3.62484009099994,11.6,10.726214025));
#217068=CARTESIAN_POINT('Ctrl Pts',(3.62240992399994,15.2,10.723583524));
#217069=CARTESIAN_POINT('Ctrl Pts',(3.62240992399994,11.6,10.723583524));
#217070=CARTESIAN_POINT('Ctrl Pts',(3.61998495799994,15.2,10.720954563));
#217071=CARTESIAN_POINT('Ctrl Pts',(3.61998495799994,11.6,10.720954563));
#217072=CARTESIAN_POINT('Ctrl Pts',(3.61756519199994,15.2,10.718327151));
#217073=CARTESIAN_POINT('Ctrl Pts',(3.61756519199994,11.6,10.718327151));
#217074=CARTESIAN_POINT('Ctrl Pts',(3.61515062899994,15.2,10.715701296));
#217075=CARTESIAN_POINT('Ctrl Pts',(3.61515062899994,11.6,10.715701296));
#217076=CARTESIAN_POINT('Ctrl Pts',(3.61274126699994,15.2,10.71307701));
#217077=CARTESIAN_POINT('Ctrl Pts',(3.61274126699994,11.6,10.71307701));
#217078=CARTESIAN_POINT('Ctrl Pts',(3.61033710899994,15.2,10.710454302));
#217079=CARTESIAN_POINT('Ctrl Pts',(3.61033710899994,11.6,10.710454302));
#217080=CARTESIAN_POINT('Ctrl Pts',(3.60793815399994,15.2,10.707833181));
#217081=CARTESIAN_POINT('Ctrl Pts',(3.60793815399994,11.6,10.707833181));
#217082=CARTESIAN_POINT('Ctrl Pts',(3.60554440399994,15.2,10.705213657));
#217083=CARTESIAN_POINT('Ctrl Pts',(3.60554440399994,11.6,10.705213657));
#217084=CARTESIAN_POINT('Ctrl Pts',(3.60315585899994,15.2,10.702595741));
#217085=CARTESIAN_POINT('Ctrl Pts',(3.60315585899994,11.6,10.702595741));
#217086=CARTESIAN_POINT('Ctrl Pts',(3.60077251999994,15.2,10.699979441));
#217087=CARTESIAN_POINT('Ctrl Pts',(3.60077251999994,11.6,10.699979441));
#217088=CARTESIAN_POINT('Ctrl Pts',(3.59839438799994,15.2,10.697364767));
#217089=CARTESIAN_POINT('Ctrl Pts',(3.59839438799994,11.6,10.697364767));
#217090=CARTESIAN_POINT('Ctrl Pts',(3.59602146199994,15.2,10.694751731));
#217091=CARTESIAN_POINT('Ctrl Pts',(3.59602146199994,11.6,10.694751731));
#217092=CARTESIAN_POINT('Ctrl Pts',(3.59365374499994,15.2,10.692140339));
#217093=CARTESIAN_POINT('Ctrl Pts',(3.59365374499994,11.6,10.692140339));
#217094=CARTESIAN_POINT('Ctrl Pts',(3.59129123599994,15.2,10.689530605));
#217095=CARTESIAN_POINT('Ctrl Pts',(3.59129123599994,11.6,10.689530605));
#217096=CARTESIAN_POINT('Ctrl Pts',(3.58893393499994,15.2,10.686922536));
#217097=CARTESIAN_POINT('Ctrl Pts',(3.58893393499994,11.6,10.686922536));
#217098=CARTESIAN_POINT('Ctrl Pts',(3.58658184499994,15.2,10.684316143));
#217099=CARTESIAN_POINT('Ctrl Pts',(3.58658184499994,11.6,10.684316143));
#217100=CARTESIAN_POINT('Ctrl Pts',(3.58423496399995,15.2,10.681711437));
#217101=CARTESIAN_POINT('Ctrl Pts',(3.58423496399995,11.6,10.681711437));
#217102=CARTESIAN_POINT('Ctrl Pts',(3.58189329599994,15.2,10.679108425));
#217103=CARTESIAN_POINT('Ctrl Pts',(3.58189329599994,11.6,10.679108425));
#217104=CARTESIAN_POINT('Ctrl Pts',(3.57955683799994,15.2,10.67650712));
#217105=CARTESIAN_POINT('Ctrl Pts',(3.57955683799994,11.6,10.67650712));
#217106=CARTESIAN_POINT('Ctrl Pts',(3.57722559299994,15.2,10.673907531));
#217107=CARTESIAN_POINT('Ctrl Pts',(3.57722559299994,11.6,10.673907531));
#217108=CARTESIAN_POINT('Ctrl Pts',(3.57489956099994,15.2,10.671309666));
#217109=CARTESIAN_POINT('Ctrl Pts',(3.57489956099994,11.6,10.671309666));
#217110=CARTESIAN_POINT('Ctrl Pts',(3.57257874199994,15.2,10.668713538));
#217111=CARTESIAN_POINT('Ctrl Pts',(3.57257874199994,11.6,10.668713538));
#217112=CARTESIAN_POINT('Ctrl Pts',(3.57026313699994,15.2,10.666119155));
#217113=CARTESIAN_POINT('Ctrl Pts',(3.57026313699994,11.6,10.666119155));
#217114=CARTESIAN_POINT('Ctrl Pts',(3.56795274699994,15.2,10.663526528));
#217115=CARTESIAN_POINT('Ctrl Pts',(3.56795274699994,11.6,10.663526528));
#217116=CARTESIAN_POINT('Ctrl Pts',(3.56564757099994,15.2,10.660935667));
#217117=CARTESIAN_POINT('Ctrl Pts',(3.56564757099994,11.6,10.660935667));
#217118=CARTESIAN_POINT('Ctrl Pts',(3.56334761099994,15.2,10.658346581));
#217119=CARTESIAN_POINT('Ctrl Pts',(3.56334761099994,11.6,10.658346581));
#217120=CARTESIAN_POINT('Ctrl Pts',(3.56105286799994,15.2,10.655759282));
#217121=CARTESIAN_POINT('Ctrl Pts',(3.56105286799994,11.6,10.655759282));
#217122=CARTESIAN_POINT('Ctrl Pts',(3.55876334099994,15.2,10.653173779));
#217123=CARTESIAN_POINT('Ctrl Pts',(3.55876334099994,11.6,10.653173779));
#217124=CARTESIAN_POINT('Ctrl Pts',(3.55647903199994,15.2,10.650590083));
#217125=CARTESIAN_POINT('Ctrl Pts',(3.55647903199994,11.6,10.650590083));
#217126=CARTESIAN_POINT('Ctrl Pts',(3.55419994099994,15.2,10.648008202));
#217127=CARTESIAN_POINT('Ctrl Pts',(3.55419994099994,11.6,10.648008202));
#217128=CARTESIAN_POINT('Ctrl Pts',(3.55192606799994,15.2,10.645428149));
#217129=CARTESIAN_POINT('Ctrl Pts',(3.55192606799994,11.6,10.645428149));
#217130=CARTESIAN_POINT('Ctrl Pts',(3.54965741499994,15.2,10.642849932));
#217131=CARTESIAN_POINT('Ctrl Pts',(3.54965741499994,11.6,10.642849932));
#217132=CARTESIAN_POINT('Ctrl Pts',(3.54739397999994,15.2,10.640273563));
#217133=CARTESIAN_POINT('Ctrl Pts',(3.54739397999994,11.6,10.640273563));
#217134=CARTESIAN_POINT('Ctrl Pts',(3.54513576499994,15.2,10.637699051));
#217135=CARTESIAN_POINT('Ctrl Pts',(3.54513576499994,11.6,10.637699051));
#217136=CARTESIAN_POINT('Ctrl Pts',(3.54288277099994,15.2,10.635126406));
#217137=CARTESIAN_POINT('Ctrl Pts',(3.54288277099994,11.6,10.635126406));
#217138=CARTESIAN_POINT('Ctrl Pts',(3.54063499799994,15.2,10.632555639));
#217139=CARTESIAN_POINT('Ctrl Pts',(3.54063499799994,11.6,10.632555639));
#217140=CARTESIAN_POINT('Ctrl Pts',(3.53839244699994,15.2,10.62998676));
#217141=CARTESIAN_POINT('Ctrl Pts',(3.53839244699994,11.6,10.62998676));
#217142=CARTESIAN_POINT('Ctrl Pts',(3.53615511699994,15.2,10.62741978));
#217143=CARTESIAN_POINT('Ctrl Pts',(3.53615511699994,11.6,10.62741978));
#217144=CARTESIAN_POINT('Ctrl Pts',(3.53392300999994,15.2,10.624854709));
#217145=CARTESIAN_POINT('Ctrl Pts',(3.53392300999994,11.6,10.624854709));
#217146=CARTESIAN_POINT('Ctrl Pts',(3.53169612599994,15.2,10.622291557));
#217147=CARTESIAN_POINT('Ctrl Pts',(3.53169612599994,11.6,10.622291557));
#217148=CARTESIAN_POINT('Ctrl Pts',(3.52947446499994,15.2,10.619730334));
#217149=CARTESIAN_POINT('Ctrl Pts',(3.52947446499994,11.6,10.619730334));
#217150=CARTESIAN_POINT('Ctrl Pts',(3.52725802799994,15.2,10.617171051));
#217151=CARTESIAN_POINT('Ctrl Pts',(3.52725802799994,11.6,10.617171051));
#217152=CARTESIAN_POINT('Ctrl Pts',(3.52504681399994,15.2,10.61461372));
#217153=CARTESIAN_POINT('Ctrl Pts',(3.52504681399994,11.6,10.61461372));
#217154=CARTESIAN_POINT('Ctrl Pts',(3.52284082599994,15.2,10.612058349));
#217155=CARTESIAN_POINT('Ctrl Pts',(3.52284082599994,11.6,10.612058349));
#217156=CARTESIAN_POINT('Ctrl Pts',(3.52064006199994,15.2,10.609504948));
#217157=CARTESIAN_POINT('Ctrl Pts',(3.52064006199994,11.6,10.609504948));
#217158=CARTESIAN_POINT('Ctrl Pts',(3.51844452399994,15.2,10.606953531));
#217159=CARTESIAN_POINT('Ctrl Pts',(3.51844452399994,11.6,10.606953531));
#217160=CARTESIAN_POINT('Ctrl Pts',(3.51625421199994,15.2,10.604404106));
#217161=CARTESIAN_POINT('Ctrl Pts',(3.51625421199994,11.6,10.604404106));
#217162=CARTESIAN_POINT('Ctrl Pts',(3.51406912699994,15.2,10.601856683));
#217163=CARTESIAN_POINT('Ctrl Pts',(3.51406912699994,11.6,10.601856683));
#217164=CARTESIAN_POINT('Ctrl Pts',(3.51188926799994,15.2,10.599311274));
#217165=CARTESIAN_POINT('Ctrl Pts',(3.51188926799994,11.6,10.599311274));
#217166=CARTESIAN_POINT('Ctrl Pts',(3.50971463599994,15.2,10.596767889));
#217167=CARTESIAN_POINT('Ctrl Pts',(3.50971463599994,11.6,10.596767889));
#217168=CARTESIAN_POINT('Ctrl Pts',(3.50754523199994,15.2,10.594226538));
#217169=CARTESIAN_POINT('Ctrl Pts',(3.50754523199994,11.6,10.594226538));
#217170=CARTESIAN_POINT('Ctrl Pts',(3.50538105499994,15.2,10.591687233));
#217171=CARTESIAN_POINT('Ctrl Pts',(3.50538105499994,11.6,10.591687233));
#217172=CARTESIAN_POINT('Ctrl Pts',(3.50322210699994,15.2,10.589149983));
#217173=CARTESIAN_POINT('Ctrl Pts',(3.50322210699994,11.6,10.589149983));
#217174=CARTESIAN_POINT('Ctrl Pts',(3.50106838699995,15.2,10.5866148));
#217175=CARTESIAN_POINT('Ctrl Pts',(3.50106838699995,11.6,10.5866148));
#217176=CARTESIAN_POINT('Ctrl Pts',(3.49891989599994,15.2,10.584081694));
#217177=CARTESIAN_POINT('Ctrl Pts',(3.49891989599994,11.6,10.584081694));
#217178=CARTESIAN_POINT('Ctrl Pts',(3.49677663399994,15.2,10.581550676));
#217179=CARTESIAN_POINT('Ctrl Pts',(3.49677663399994,11.6,10.581550676));
#217180=CARTESIAN_POINT('Ctrl Pts',(3.49463860199994,15.2,10.579021758));
#217181=CARTESIAN_POINT('Ctrl Pts',(3.49463860199994,11.6,10.579021758));
#217182=CARTESIAN_POINT('Ctrl Pts',(3.49250580099994,15.2,10.576494948));
#217183=CARTESIAN_POINT('Ctrl Pts',(3.49250580099994,11.6,10.576494948));
#217184=CARTESIAN_POINT('Ctrl Pts',(3.49037822899994,15.2,10.573970259));
#217185=CARTESIAN_POINT('Ctrl Pts',(3.49037822899994,11.6,10.573970259));
#217186=CARTESIAN_POINT('Ctrl Pts',(3.48825588699994,15.2,10.571447699));
#217187=CARTESIAN_POINT('Ctrl Pts',(3.48825588699994,11.6,10.571447699));
#217188=CARTESIAN_POINT('Ctrl Pts',(3.48613877699994,15.2,10.568927282));
#217189=CARTESIAN_POINT('Ctrl Pts',(3.48613877699994,11.6,10.568927282));
#217190=CARTESIAN_POINT('Ctrl Pts',(3.48402689799994,15.2,10.566409018));
#217191=CARTESIAN_POINT('Ctrl Pts',(3.48402689799994,11.6,10.566409018));
#217192=CARTESIAN_POINT('Ctrl Pts',(3.48192024899994,15.2,10.563892917));
#217193=CARTESIAN_POINT('Ctrl Pts',(3.48192024899994,11.6,10.563892917));
#217194=CARTESIAN_POINT('Ctrl Pts',(3.47981883399994,15.2,10.561378991));
#217195=CARTESIAN_POINT('Ctrl Pts',(3.47981883399994,11.6,10.561378991));
#217196=CARTESIAN_POINT('Ctrl Pts',(3.47772264999994,15.2,10.558867249));
#217197=CARTESIAN_POINT('Ctrl Pts',(3.47772264999994,11.6,10.558867249));
#217198=CARTESIAN_POINT('Ctrl Pts',(3.47563169699994,15.2,10.556357703));
#217199=CARTESIAN_POINT('Ctrl Pts',(3.47563169699994,11.6,10.556357703));
#217200=CARTESIAN_POINT('Ctrl Pts',(3.47354597799994,15.2,10.553850365));
#217201=CARTESIAN_POINT('Ctrl Pts',(3.47354597799994,11.6,10.553850365));
#217202=CARTESIAN_POINT('Ctrl Pts',(3.47146549099994,15.2,10.551345244));
#217203=CARTESIAN_POINT('Ctrl Pts',(3.47146549099994,11.6,10.551345244));
#217204=CARTESIAN_POINT('Ctrl Pts',(3.46939023699994,15.2,10.548842353));
#217205=CARTESIAN_POINT('Ctrl Pts',(3.46939023699994,11.6,10.548842353));
#217206=CARTESIAN_POINT('Ctrl Pts',(3.46732021699995,15.2,10.546341702));
#217207=CARTESIAN_POINT('Ctrl Pts',(3.46732021699995,11.6,10.546341702));
#217208=CARTESIAN_POINT('Ctrl Pts',(3.46525542999994,15.2,10.543843302));
#217209=CARTESIAN_POINT('Ctrl Pts',(3.46525542999994,11.6,10.543843302));
#217210=CARTESIAN_POINT('Ctrl Pts',(3.46319587599994,15.2,10.541347163));
#217211=CARTESIAN_POINT('Ctrl Pts',(3.46319587599994,11.6,10.541347163));
#217212=CARTESIAN_POINT('Ctrl Pts',(3.46114155699994,15.2,10.538853298));
#217213=CARTESIAN_POINT('Ctrl Pts',(3.46114155699994,11.6,10.538853298));
#217214=CARTESIAN_POINT('Ctrl Pts',(3.45909247099994,15.2,10.536361718));
#217215=CARTESIAN_POINT('Ctrl Pts',(3.45909247099994,11.6,10.536361718));
#217216=CARTESIAN_POINT('Ctrl Pts',(3.45704861999995,15.2,10.533872432));
#217217=CARTESIAN_POINT('Ctrl Pts',(3.45704861999995,11.6,10.533872432));
#217218=CARTESIAN_POINT('Ctrl Pts',(3.45501000299994,15.2,10.531385453));
#217219=CARTESIAN_POINT('Ctrl Pts',(3.45501000299994,11.6,10.531385453));
#217220=CARTESIAN_POINT('Ctrl Pts',(3.45297662099994,15.2,10.528900792));
#217221=CARTESIAN_POINT('Ctrl Pts',(3.45297662099994,11.6,10.528900792));
#217222=CARTESIAN_POINT('Ctrl Pts',(3.45094847299994,15.2,10.526418461));
#217223=CARTESIAN_POINT('Ctrl Pts',(3.45094847299994,11.6,10.526418461));
#217224=CARTESIAN_POINT('Ctrl Pts',(3.44892555999994,15.2,10.523938468));
#217225=CARTESIAN_POINT('Ctrl Pts',(3.44892555999994,11.6,10.523938468));
#217226=CARTESIAN_POINT('Ctrl Pts',(3.44690788299994,15.2,10.521460827));
#217227=CARTESIAN_POINT('Ctrl Pts',(3.44690788299994,11.6,10.521460827));
#217228=CARTESIAN_POINT('Ctrl Pts',(3.44489543999994,15.2,10.51898555));
#217229=CARTESIAN_POINT('Ctrl Pts',(3.44489543999994,11.6,10.51898555));
#217230=CARTESIAN_POINT('Ctrl Pts',(3.44288823299994,15.2,10.516512645));
#217231=CARTESIAN_POINT('Ctrl Pts',(3.44288823299994,11.6,10.516512645));
#217232=CARTESIAN_POINT('Ctrl Pts',(3.44088626199994,15.2,10.514042126));
#217233=CARTESIAN_POINT('Ctrl Pts',(3.44088626199994,11.6,10.514042126));
#217234=CARTESIAN_POINT('Ctrl Pts',(3.43888952499994,15.2,10.511574004));
#217235=CARTESIAN_POINT('Ctrl Pts',(3.43888952499994,11.6,10.511574004));
#217236=CARTESIAN_POINT('Ctrl Pts',(3.43689802499994,15.2,10.50910829));
#217237=CARTESIAN_POINT('Ctrl Pts',(3.43689802499994,11.6,10.50910829));
#217238=CARTESIAN_POINT('Ctrl Pts',(3.43491175999994,15.2,10.506644995));
#217239=CARTESIAN_POINT('Ctrl Pts',(3.43491175999994,11.6,10.506644995));
#217240=CARTESIAN_POINT('Ctrl Pts',(3.43293072999994,15.2,10.504184131));
#217241=CARTESIAN_POINT('Ctrl Pts',(3.43293072999994,11.6,10.504184131));
#217242=CARTESIAN_POINT('Ctrl Pts',(3.43095493699995,15.2,10.501725709));
#217243=CARTESIAN_POINT('Ctrl Pts',(3.43095493699995,11.6,10.501725709));
#217244=CARTESIAN_POINT('Ctrl Pts',(3.42898437999994,15.2,10.49926974));
#217245=CARTESIAN_POINT('Ctrl Pts',(3.42898437999994,11.6,10.49926974));
#217246=CARTESIAN_POINT('Ctrl Pts',(3.42701905899994,15.2,10.496816237));
#217247=CARTESIAN_POINT('Ctrl Pts',(3.42701905899994,11.6,10.496816237));
#217248=CARTESIAN_POINT('Ctrl Pts',(3.42505897399994,15.2,10.49436521));
#217249=CARTESIAN_POINT('Ctrl Pts',(3.42505897399994,11.6,10.49436521));
#217250=CARTESIAN_POINT('Ctrl Pts',(3.42310412599995,15.2,10.491916672));
#217251=CARTESIAN_POINT('Ctrl Pts',(3.42310412599995,11.6,10.491916672));
#217252=CARTESIAN_POINT('Ctrl Pts',(3.42115451199994,15.2,10.489470632));
#217253=CARTESIAN_POINT('Ctrl Pts',(3.42115451199994,11.6,10.489470632));
#217254=CARTESIAN_POINT('Ctrl Pts',(3.41921013599995,15.2,10.487027105));
#217255=CARTESIAN_POINT('Ctrl Pts',(3.41921013599995,11.6,10.487027105));
#217256=CARTESIAN_POINT('Ctrl Pts',(3.41727099499994,15.2,10.4845861));
#217257=CARTESIAN_POINT('Ctrl Pts',(3.41727099499994,11.6,10.4845861));
#217258=CARTESIAN_POINT('Ctrl Pts',(3.41533709199994,15.2,10.482147629));
#217259=CARTESIAN_POINT('Ctrl Pts',(3.41533709199994,11.6,10.482147629));
#217260=CARTESIAN_POINT('Ctrl Pts',(3.41340842399994,15.2,10.479711706));
#217261=CARTESIAN_POINT('Ctrl Pts',(3.41340842399994,11.6,10.479711706));
#217262=CARTESIAN_POINT('Ctrl Pts',(3.41148499199994,15.2,10.477278339));
#217263=CARTESIAN_POINT('Ctrl Pts',(3.41148499199994,11.6,10.477278339));
#217264=CARTESIAN_POINT('Ctrl Pts',(3.40956679599994,15.2,10.474847543));
#217265=CARTESIAN_POINT('Ctrl Pts',(3.40956679599994,11.6,10.474847543));
#217266=CARTESIAN_POINT('Ctrl Pts',(3.40765383599994,15.2,10.472419326));
#217267=CARTESIAN_POINT('Ctrl Pts',(3.40765383599994,11.6,10.472419326));
#217268=CARTESIAN_POINT('Ctrl Pts',(3.40574611299994,15.2,10.469993704));
#217269=CARTESIAN_POINT('Ctrl Pts',(3.40574611299994,11.6,10.469993704));
#217270=CARTESIAN_POINT('Ctrl Pts',(3.40384362599994,15.2,10.467570687));
#217271=CARTESIAN_POINT('Ctrl Pts',(3.40384362599994,11.6,10.467570687));
#217272=CARTESIAN_POINT('Ctrl Pts',(3.40194637399994,15.2,10.465150286));
#217273=CARTESIAN_POINT('Ctrl Pts',(3.40194637399994,11.6,10.465150286));
#217274=CARTESIAN_POINT('Ctrl Pts',(3.40005435899994,15.2,10.462732513));
#217275=CARTESIAN_POINT('Ctrl Pts',(3.40005435899994,11.6,10.462732513));
#217276=CARTESIAN_POINT('Ctrl Pts',(3.39816757899994,15.2,10.460317381));
#217277=CARTESIAN_POINT('Ctrl Pts',(3.39816757899994,11.6,10.460317381));
#217278=CARTESIAN_POINT('Ctrl Pts',(3.39628603499994,15.2,10.4579049));
#217279=CARTESIAN_POINT('Ctrl Pts',(3.39628603499994,11.6,10.4579049));
#217280=CARTESIAN_POINT('Ctrl Pts',(3.39440972599995,15.2,10.455495084));
#217281=CARTESIAN_POINT('Ctrl Pts',(3.39440972599995,11.6,10.455495084));
#217282=CARTESIAN_POINT('Ctrl Pts',(3.39253865299994,15.2,10.453087944));
#217283=CARTESIAN_POINT('Ctrl Pts',(3.39253865299994,11.6,10.453087944));
#217284=CARTESIAN_POINT('Ctrl Pts',(3.39067281599994,15.2,10.450683492));
#217285=CARTESIAN_POINT('Ctrl Pts',(3.39067281599994,11.6,10.450683492));
#217286=CARTESIAN_POINT('Ctrl Pts',(3.38881221399994,15.2,10.448281741));
#217287=CARTESIAN_POINT('Ctrl Pts',(3.38881221399994,11.6,10.448281741));
#217288=CARTESIAN_POINT('Ctrl Pts',(3.38695684699994,15.2,10.445882701));
#217289=CARTESIAN_POINT('Ctrl Pts',(3.38695684699994,11.6,10.445882701));
#217290=CARTESIAN_POINT('Ctrl Pts',(3.38510671499994,15.2,10.443486385));
#217291=CARTESIAN_POINT('Ctrl Pts',(3.38510671499994,11.6,10.443486385));
#217292=CARTESIAN_POINT('Ctrl Pts',(3.38326181899995,15.2,10.441092806));
#217293=CARTESIAN_POINT('Ctrl Pts',(3.38326181899995,11.6,10.441092806));
#217294=CARTESIAN_POINT('Ctrl Pts',(3.38142215599994,15.2,10.438701973));
#217295=CARTESIAN_POINT('Ctrl Pts',(3.38142215599994,11.6,10.438701973));
#217296=CARTESIAN_POINT('Ctrl Pts',(3.37958772799994,15.2,10.436313903));
#217297=CARTESIAN_POINT('Ctrl Pts',(3.37958772799994,11.6,10.436313903));
#217298=CARTESIAN_POINT('Ctrl Pts',(3.37775853499994,15.2,10.433928604));
#217299=CARTESIAN_POINT('Ctrl Pts',(3.37775853499994,11.6,10.433928604));
#217300=CARTESIAN_POINT('Ctrl Pts',(3.37593457599994,15.2,10.43154609));
#217301=CARTESIAN_POINT('Ctrl Pts',(3.37593457599994,11.6,10.43154609));
#217302=CARTESIAN_POINT('Ctrl Pts',(3.37411584999994,15.2,10.429166374));
#217303=CARTESIAN_POINT('Ctrl Pts',(3.37411584999994,11.6,10.429166374));
#217304=CARTESIAN_POINT('Ctrl Pts',(3.37230235899994,15.2,10.426789465));
#217305=CARTESIAN_POINT('Ctrl Pts',(3.37230235899994,11.6,10.426789465));
#217306=CARTESIAN_POINT('Ctrl Pts',(3.37049410099994,15.2,10.424415378));
#217307=CARTESIAN_POINT('Ctrl Pts',(3.37049410099994,11.6,10.424415378));
#217308=CARTESIAN_POINT('Ctrl Pts',(3.36869107699994,15.2,10.422044126));
#217309=CARTESIAN_POINT('Ctrl Pts',(3.36869107699994,11.6,10.422044126));
#217310=CARTESIAN_POINT('Ctrl Pts',(3.36689328399994,15.2,10.419675719));
#217311=CARTESIAN_POINT('Ctrl Pts',(3.36689328399994,11.6,10.419675719));
#217312=CARTESIAN_POINT('Ctrl Pts',(3.36510072599994,15.2,10.417310171));
#217313=CARTESIAN_POINT('Ctrl Pts',(3.36510072599994,11.6,10.417310171));
#217314=CARTESIAN_POINT('Ctrl Pts',(3.36331339899994,15.2,10.414947493));
#217315=CARTESIAN_POINT('Ctrl Pts',(3.36331339899994,11.6,10.414947493));
#217316=CARTESIAN_POINT('Ctrl Pts',(3.36153130499994,15.2,10.412587698));
#217317=CARTESIAN_POINT('Ctrl Pts',(3.36153130499994,11.6,10.412587698));
#217318=CARTESIAN_POINT('Ctrl Pts',(3.35975444299994,15.2,10.410230799));
#217319=CARTESIAN_POINT('Ctrl Pts',(3.35975444299994,11.6,10.410230799));
#217320=CARTESIAN_POINT('Ctrl Pts',(3.35798281299994,15.2,10.407876808));
#217321=CARTESIAN_POINT('Ctrl Pts',(3.35798281299994,11.6,10.407876808));
#217322=CARTESIAN_POINT('Ctrl Pts',(3.35621641399994,15.2,10.405525737));
#217323=CARTESIAN_POINT('Ctrl Pts',(3.35621641399994,11.6,10.405525737));
#217324=CARTESIAN_POINT('Ctrl Pts',(3.35445524599994,15.2,10.4031776));
#217325=CARTESIAN_POINT('Ctrl Pts',(3.35445524599994,11.6,10.4031776));
#217326=CARTESIAN_POINT('Ctrl Pts',(3.35269930899994,15.2,10.400832408));
#217327=CARTESIAN_POINT('Ctrl Pts',(3.35269930899994,11.6,10.400832408));
#217328=CARTESIAN_POINT('Ctrl Pts',(3.35094860199994,15.2,10.398490174));
#217329=CARTESIAN_POINT('Ctrl Pts',(3.35094860199994,11.6,10.398490174));
#217330=CARTESIAN_POINT('Ctrl Pts',(3.34920312499994,15.2,10.396150911));
#217331=CARTESIAN_POINT('Ctrl Pts',(3.34920312499994,11.6,10.396150911));
#217332=CARTESIAN_POINT('Ctrl Pts',(3.34746287999995,15.2,10.393814631));
#217333=CARTESIAN_POINT('Ctrl Pts',(3.34746287999995,11.6,10.393814631));
#217334=CARTESIAN_POINT('Ctrl Pts',(3.34572786099995,15.2,10.391481347));
#217335=CARTESIAN_POINT('Ctrl Pts',(3.34572786099995,11.6,10.391481347));
#217336=CARTESIAN_POINT('Ctrl Pts',(3.34399807299994,15.2,10.389151072));
#217337=CARTESIAN_POINT('Ctrl Pts',(3.34399807299994,11.6,10.389151072));
#217338=CARTESIAN_POINT('Ctrl Pts',(3.34227351299994,15.2,10.386823818));
#217339=CARTESIAN_POINT('Ctrl Pts',(3.34227351299994,11.6,10.386823818));
#217340=CARTESIAN_POINT('Ctrl Pts',(3.34055418199994,15.2,10.384499599));
#217341=CARTESIAN_POINT('Ctrl Pts',(3.34055418199994,11.6,10.384499599));
#217342=CARTESIAN_POINT('Ctrl Pts',(3.33884007799994,15.2,10.382178427));
#217343=CARTESIAN_POINT('Ctrl Pts',(3.33884007799994,11.6,10.382178427));
#217344=CARTESIAN_POINT('Ctrl Pts',(3.33713120199994,15.2,10.379860313));
#217345=CARTESIAN_POINT('Ctrl Pts',(3.33713120199994,11.6,10.379860313));
#217346=CARTESIAN_POINT('Ctrl Pts',(3.33542755199994,15.2,10.377545274));
#217347=CARTESIAN_POINT('Ctrl Pts',(3.33542755199994,11.6,10.377545274));
#217348=CARTESIAN_POINT('Ctrl Pts',(3.33372912899994,15.2,10.375233319));
#217349=CARTESIAN_POINT('Ctrl Pts',(3.33372912899994,11.6,10.375233319));
#217350=CARTESIAN_POINT('Ctrl Pts',(3.33203593199995,15.2,10.372924463));
#217351=CARTESIAN_POINT('Ctrl Pts',(3.33203593199995,11.6,10.372924463));
#217352=CARTESIAN_POINT('Ctrl Pts',(3.33034796099994,15.2,10.370618718));
#217353=CARTESIAN_POINT('Ctrl Pts',(3.33034796099994,11.6,10.370618718));
#217354=CARTESIAN_POINT('Ctrl Pts',(3.32866521499994,15.2,10.368316097));
#217355=CARTESIAN_POINT('Ctrl Pts',(3.32866521499994,11.6,10.368316097));
#217356=CARTESIAN_POINT('Ctrl Pts',(3.32698769299994,15.2,10.366016614));
#217357=CARTESIAN_POINT('Ctrl Pts',(3.32698769299994,11.6,10.366016614));
#217358=CARTESIAN_POINT('Ctrl Pts',(3.32531539599994,15.2,10.36372028));
#217359=CARTESIAN_POINT('Ctrl Pts',(3.32531539599994,11.6,10.36372028));
#217360=CARTESIAN_POINT('Ctrl Pts',(3.32364832199994,15.2,10.36142711));
#217361=CARTESIAN_POINT('Ctrl Pts',(3.32364832199994,11.6,10.36142711));
#217362=CARTESIAN_POINT('Ctrl Pts',(3.32198647199994,15.2,10.359137117));
#217363=CARTESIAN_POINT('Ctrl Pts',(3.32198647199994,11.6,10.359137117));
#217364=CARTESIAN_POINT('Ctrl Pts',(3.32032984499994,15.2,10.356850313));
#217365=CARTESIAN_POINT('Ctrl Pts',(3.32032984499994,11.6,10.356850313));
#217366=CARTESIAN_POINT('Ctrl Pts',(3.31867843899994,15.2,10.354566712));
#217367=CARTESIAN_POINT('Ctrl Pts',(3.31867843899994,11.6,10.354566712));
#217368=CARTESIAN_POINT('Ctrl Pts',(3.31703225499994,15.2,10.352286327));
#217369=CARTESIAN_POINT('Ctrl Pts',(3.31703225499994,11.6,10.352286327));
#217370=CARTESIAN_POINT('Ctrl Pts',(3.31539129199995,15.2,10.35000917));
#217371=CARTESIAN_POINT('Ctrl Pts',(3.31539129199995,11.6,10.35000917));
#217372=CARTESIAN_POINT('Ctrl Pts',(3.31375554899994,15.2,10.347735256));
#217373=CARTESIAN_POINT('Ctrl Pts',(3.31375554899994,11.6,10.347735256));
#217374=CARTESIAN_POINT('Ctrl Pts',(3.31212502599994,15.2,10.345464598));
#217375=CARTESIAN_POINT('Ctrl Pts',(3.31212502599994,11.6,10.345464598));
#217376=CARTESIAN_POINT('Ctrl Pts',(3.31049972299994,15.2,10.343197209));
#217377=CARTESIAN_POINT('Ctrl Pts',(3.31049972299994,11.6,10.343197209));
#217378=CARTESIAN_POINT('Ctrl Pts',(3.30887963899994,15.2,10.340933102));
#217379=CARTESIAN_POINT('Ctrl Pts',(3.30887963899994,11.6,10.340933102));
#217380=CARTESIAN_POINT('Ctrl Pts',(3.30726477099994,15.2,10.33867229));
#217381=CARTESIAN_POINT('Ctrl Pts',(3.30726477099994,11.6,10.33867229));
#217382=CARTESIAN_POINT('Ctrl Pts',(3.30565512199994,15.2,10.336414786));
#217383=CARTESIAN_POINT('Ctrl Pts',(3.30565512199994,11.6,10.336414786));
#217384=CARTESIAN_POINT('Ctrl Pts',(3.30405068899994,15.2,10.334160606));
#217385=CARTESIAN_POINT('Ctrl Pts',(3.30405068899994,11.6,10.334160606));
#217386=CARTESIAN_POINT('Ctrl Pts',(3.30245147199994,15.2,10.331909762));
#217387=CARTESIAN_POINT('Ctrl Pts',(3.30245147199994,11.6,10.331909762));
#217388=CARTESIAN_POINT('Ctrl Pts',(3.30085747199994,15.2,10.329662268));
#217389=CARTESIAN_POINT('Ctrl Pts',(3.30085747199994,11.6,10.329662268));
#217390=CARTESIAN_POINT('Ctrl Pts',(3.29926868599994,15.2,10.327418135));
#217391=CARTESIAN_POINT('Ctrl Pts',(3.29926868599994,11.6,10.327418135));
#217392=CARTESIAN_POINT('Ctrl Pts',(3.29768511299994,15.2,10.325177379));
#217393=CARTESIAN_POINT('Ctrl Pts',(3.29768511299994,11.6,10.325177379));
#217394=CARTESIAN_POINT('Ctrl Pts',(3.29610675499994,15.2,10.322940014));
#217395=CARTESIAN_POINT('Ctrl Pts',(3.29610675499994,11.6,10.322940014));
#217396=CARTESIAN_POINT('Ctrl Pts',(3.29453360899994,15.2,10.320706052));
#217397=CARTESIAN_POINT('Ctrl Pts',(3.29453360899994,11.6,10.320706052));
#217398=CARTESIAN_POINT('Ctrl Pts',(3.29296567499994,15.2,10.318475509));
#217399=CARTESIAN_POINT('Ctrl Pts',(3.29296567499994,11.6,10.318475509));
#217400=CARTESIAN_POINT('Ctrl Pts',(3.29140295199994,15.2,10.316248395));
#217401=CARTESIAN_POINT('Ctrl Pts',(3.29140295199994,11.6,10.316248395));
#217402=CARTESIAN_POINT('Ctrl Pts',(3.28984543999994,15.2,10.314024727));
#217403=CARTESIAN_POINT('Ctrl Pts',(3.28984543999994,11.6,10.314024727));
#217404=CARTESIAN_POINT('Ctrl Pts',(3.28829313699994,15.2,10.311804518));
#217405=CARTESIAN_POINT('Ctrl Pts',(3.28829313699994,11.6,10.311804518));
#217406=CARTESIAN_POINT('Ctrl Pts',(3.28674604399994,15.2,10.30958778));
#217407=CARTESIAN_POINT('Ctrl Pts',(3.28674604399994,11.6,10.30958778));
#217408=CARTESIAN_POINT('Ctrl Pts',(3.28520415899995,15.2,10.307374529));
#217409=CARTESIAN_POINT('Ctrl Pts',(3.28520415899995,11.6,10.307374529));
#217410=CARTESIAN_POINT('Ctrl Pts',(3.28366748099994,15.2,10.305164779));
#217411=CARTESIAN_POINT('Ctrl Pts',(3.28366748099994,11.6,10.305164779));
#217412=CARTESIAN_POINT('Ctrl Pts',(3.28213600999995,15.2,10.302958542));
#217413=CARTESIAN_POINT('Ctrl Pts',(3.28213600999995,11.6,10.302958542));
#217414=CARTESIAN_POINT('Ctrl Pts',(3.28060974399994,15.2,10.300755834));
#217415=CARTESIAN_POINT('Ctrl Pts',(3.28060974399994,11.6,10.300755834));
#217416=CARTESIAN_POINT('Ctrl Pts',(3.27908868399994,15.2,10.298556666));
#217417=CARTESIAN_POINT('Ctrl Pts',(3.27908868399994,11.6,10.298556666));
#217418=CARTESIAN_POINT('Ctrl Pts',(3.27757282699995,15.2,10.296361056));
#217419=CARTESIAN_POINT('Ctrl Pts',(3.27757282699995,11.6,10.296361056));
#217420=CARTESIAN_POINT('Ctrl Pts',(3.27606217499994,15.2,10.294169016));
#217421=CARTESIAN_POINT('Ctrl Pts',(3.27606217499994,11.6,10.294169016));
#217422=CARTESIAN_POINT('Ctrl Pts',(3.27455672399994,15.2,10.291980559));
#217423=CARTESIAN_POINT('Ctrl Pts',(3.27455672399994,11.6,10.291980559));
#217424=CARTESIAN_POINT('Ctrl Pts',(3.27305647499994,15.2,10.2897957));
#217425=CARTESIAN_POINT('Ctrl Pts',(3.27305647499994,11.6,10.2897957));
#217426=CARTESIAN_POINT('Ctrl Pts',(3.27156142599994,15.2,10.287614454));
#217427=CARTESIAN_POINT('Ctrl Pts',(3.27156142599994,11.6,10.287614454));
#217428=CARTESIAN_POINT('Ctrl Pts',(3.27007157799994,15.2,10.285436836));
#217429=CARTESIAN_POINT('Ctrl Pts',(3.27007157799994,11.6,10.285436836));
#217430=CARTESIAN_POINT('Ctrl Pts',(3.26858692799994,15.2,10.283262858));
#217431=CARTESIAN_POINT('Ctrl Pts',(3.26858692799994,11.6,10.283262858));
#217432=CARTESIAN_POINT('Ctrl Pts',(3.26710747499994,15.2,10.281092534));
#217433=CARTESIAN_POINT('Ctrl Pts',(3.26710747499994,11.6,10.281092534));
#217434=CARTESIAN_POINT('Ctrl Pts',(3.26563321999994,15.2,10.27892588));
#217435=CARTESIAN_POINT('Ctrl Pts',(3.26563321999994,11.6,10.27892588));
#217436=CARTESIAN_POINT('Ctrl Pts',(3.26416416099994,15.2,10.276762911));
#217437=CARTESIAN_POINT('Ctrl Pts',(3.26416416099994,11.6,10.276762911));
#217438=CARTESIAN_POINT('Ctrl Pts',(3.26270029699995,15.2,10.274603639));
#217439=CARTESIAN_POINT('Ctrl Pts',(3.26270029699995,11.6,10.274603639));
#217440=CARTESIAN_POINT('Ctrl Pts',(3.26124162699994,15.2,10.272448079));
#217441=CARTESIAN_POINT('Ctrl Pts',(3.26124162699994,11.6,10.272448079));
#217442=CARTESIAN_POINT('Ctrl Pts',(3.25978815099994,15.2,10.270296246));
#217443=CARTESIAN_POINT('Ctrl Pts',(3.25978815099994,11.6,10.270296246));
#217444=CARTESIAN_POINT('Ctrl Pts',(3.25833986599994,15.2,10.268148156));
#217445=CARTESIAN_POINT('Ctrl Pts',(3.25833986599994,11.6,10.268148156));
#217446=CARTESIAN_POINT('Ctrl Pts',(3.25689677199994,15.2,10.266003821));
#217447=CARTESIAN_POINT('Ctrl Pts',(3.25689677199994,11.6,10.266003821));
#217448=CARTESIAN_POINT('Ctrl Pts',(3.25545886799994,15.2,10.263863257));
#217449=CARTESIAN_POINT('Ctrl Pts',(3.25545886799994,11.6,10.263863257));
#217450=CARTESIAN_POINT('Ctrl Pts',(3.25402615299994,15.2,10.261726478));
#217451=CARTESIAN_POINT('Ctrl Pts',(3.25402615299994,11.6,10.261726478));
#217452=CARTESIAN_POINT('Ctrl Pts',(3.25259862599995,15.2,10.259593498));
#217453=CARTESIAN_POINT('Ctrl Pts',(3.25259862599995,11.6,10.259593498));
#217454=CARTESIAN_POINT('Ctrl Pts',(3.25117628599994,15.2,10.257464334));
#217455=CARTESIAN_POINT('Ctrl Pts',(3.25117628599994,11.6,10.257464334));
#217456=CARTESIAN_POINT('Ctrl Pts',(3.24975913199995,15.2,10.255338999));
#217457=CARTESIAN_POINT('Ctrl Pts',(3.24975913199995,11.6,10.255338999));
#217458=CARTESIAN_POINT('Ctrl Pts',(3.24834716199994,15.2,10.253217507));
#217459=CARTESIAN_POINT('Ctrl Pts',(3.24834716199994,11.6,10.253217507));
#217460=CARTESIAN_POINT('Ctrl Pts',(3.24694037599994,15.2,10.251099875));
#217461=CARTESIAN_POINT('Ctrl Pts',(3.24694037599994,11.6,10.251099875));
#217462=CARTESIAN_POINT('Ctrl Pts',(3.24553877199994,15.2,10.248986116));
#217463=CARTESIAN_POINT('Ctrl Pts',(3.24553877199994,11.6,10.248986116));
#217464=CARTESIAN_POINT('Ctrl Pts',(3.24414234999994,15.2,10.246876245));
#217465=CARTESIAN_POINT('Ctrl Pts',(3.24414234999994,11.6,10.246876245));
#217466=CARTESIAN_POINT('Ctrl Pts',(3.24275110699995,15.2,10.244770278));
#217467=CARTESIAN_POINT('Ctrl Pts',(3.24275110699995,11.6,10.244770278));
#217468=CARTESIAN_POINT('Ctrl Pts',(3.24136504399994,15.2,10.242668229));
#217469=CARTESIAN_POINT('Ctrl Pts',(3.24136504399994,11.6,10.242668229));
#217470=CARTESIAN_POINT('Ctrl Pts',(3.23998415799994,15.2,10.240570115));
#217471=CARTESIAN_POINT('Ctrl Pts',(3.23998415799994,11.6,10.240570115));
#217472=CARTESIAN_POINT('Ctrl Pts',(3.23860844899994,15.2,10.238475948));
#217473=CARTESIAN_POINT('Ctrl Pts',(3.23860844899994,11.6,10.238475948));
#217474=CARTESIAN_POINT('Ctrl Pts',(3.23723791499994,15.2,10.236385745));
#217475=CARTESIAN_POINT('Ctrl Pts',(3.23723791499994,11.6,10.236385745));
#217476=CARTESIAN_POINT('Ctrl Pts',(3.23587255499994,15.2,10.23429952));
#217477=CARTESIAN_POINT('Ctrl Pts',(3.23587255499994,11.6,10.23429952));
#217478=CARTESIAN_POINT('Ctrl Pts',(3.23451236799994,15.2,10.232217288));
#217479=CARTESIAN_POINT('Ctrl Pts',(3.23451236799994,11.6,10.232217288));
#217480=CARTESIAN_POINT('Ctrl Pts',(3.23315735299994,15.2,10.230139067));
#217481=CARTESIAN_POINT('Ctrl Pts',(3.23315735299994,11.6,10.230139067));
#217482=CARTESIAN_POINT('Ctrl Pts',(3.23180750799994,15.2,10.228064869));
#217483=CARTESIAN_POINT('Ctrl Pts',(3.23180750799994,11.6,10.228064869));
#217484=CARTESIAN_POINT('Ctrl Pts',(3.23046283199994,15.2,10.225994711));
#217485=CARTESIAN_POINT('Ctrl Pts',(3.23046283199994,11.6,10.225994711));
#217486=CARTESIAN_POINT('Ctrl Pts',(3.22912332499994,15.2,10.223928608));
#217487=CARTESIAN_POINT('Ctrl Pts',(3.22912332499994,11.6,10.223928608));
#217488=CARTESIAN_POINT('Ctrl Pts',(3.22778898299994,15.2,10.221866575));
#217489=CARTESIAN_POINT('Ctrl Pts',(3.22778898299994,11.6,10.221866575));
#217490=CARTESIAN_POINT('Ctrl Pts',(3.22645980699994,15.2,10.219808628));
#217491=CARTESIAN_POINT('Ctrl Pts',(3.22645980699994,11.6,10.219808628));
#217492=CARTESIAN_POINT('Ctrl Pts',(3.22513579399994,15.2,10.217754781));
#217493=CARTESIAN_POINT('Ctrl Pts',(3.22513579399994,11.6,10.217754781));
#217494=CARTESIAN_POINT('Ctrl Pts',(3.22381694499994,15.2,10.215705052));
#217495=CARTESIAN_POINT('Ctrl Pts',(3.22381694499994,11.6,10.215705052));
#217496=CARTESIAN_POINT('Ctrl Pts',(3.22250325599994,15.2,10.213659454));
#217497=CARTESIAN_POINT('Ctrl Pts',(3.22250325599994,11.6,10.213659454));
#217498=CARTESIAN_POINT('Ctrl Pts',(3.22119472699995,15.2,10.211618004));
#217499=CARTESIAN_POINT('Ctrl Pts',(3.22119472699995,11.6,10.211618004));
#217500=CARTESIAN_POINT('Ctrl Pts',(3.21989135599994,15.2,10.209580717));
#217501=CARTESIAN_POINT('Ctrl Pts',(3.21989135599994,11.6,10.209580717));
#217502=CARTESIAN_POINT('Ctrl Pts',(3.21859314299994,15.2,10.20754761));
#217503=CARTESIAN_POINT('Ctrl Pts',(3.21859314299994,11.6,10.20754761));
#217504=CARTESIAN_POINT('Ctrl Pts',(3.21730008399994,15.2,10.205518696));
#217505=CARTESIAN_POINT('Ctrl Pts',(3.21730008399994,11.6,10.205518696));
#217506=CARTESIAN_POINT('Ctrl Pts',(3.21601217999994,15.2,10.203493994));
#217507=CARTESIAN_POINT('Ctrl Pts',(3.21601217999994,11.6,10.203493994));
#217508=CARTESIAN_POINT('Ctrl Pts',(3.21472942799994,15.2,10.201473517));
#217509=CARTESIAN_POINT('Ctrl Pts',(3.21472942799994,11.6,10.201473517));
#217510=CARTESIAN_POINT('Ctrl Pts',(3.21345182799994,15.2,10.199457283));
#217511=CARTESIAN_POINT('Ctrl Pts',(3.21345182799994,11.6,10.199457283));
#217512=CARTESIAN_POINT('Ctrl Pts',(3.21217937699994,15.2,10.197445307));
#217513=CARTESIAN_POINT('Ctrl Pts',(3.21217937699994,11.6,10.197445307));
#217514=CARTESIAN_POINT('Ctrl Pts',(3.21091207399995,15.2,10.195437604));
#217515=CARTESIAN_POINT('Ctrl Pts',(3.21091207399995,11.6,10.195437604));
#217516=CARTESIAN_POINT('Ctrl Pts',(3.20964991799995,15.2,10.193434192));
#217517=CARTESIAN_POINT('Ctrl Pts',(3.20964991799995,11.6,10.193434192));
#217518=CARTESIAN_POINT('Ctrl Pts',(3.20839290699994,15.2,10.191435086));
#217519=CARTESIAN_POINT('Ctrl Pts',(3.20839290699994,11.6,10.191435086));
#217520=CARTESIAN_POINT('Ctrl Pts',(3.20714103999994,15.2,10.189440301));
#217521=CARTESIAN_POINT('Ctrl Pts',(3.20714103999994,11.6,10.189440301));
#217522=CARTESIAN_POINT('Ctrl Pts',(3.20589431499994,15.2,10.187449854));
#217523=CARTESIAN_POINT('Ctrl Pts',(3.20589431499994,11.6,10.187449854));
#217524=CARTESIAN_POINT('Ctrl Pts',(3.20465272999995,15.2,10.185463762));
#217525=CARTESIAN_POINT('Ctrl Pts',(3.20465272999995,11.6,10.185463762));
#217526=CARTESIAN_POINT('Ctrl Pts',(3.20341628299994,15.2,10.183482041));
#217527=CARTESIAN_POINT('Ctrl Pts',(3.20341628299994,11.6,10.183482041));
#217528=CARTESIAN_POINT('Ctrl Pts',(3.20218497399994,15.2,10.181504705));
#217529=CARTESIAN_POINT('Ctrl Pts',(3.20218497399994,11.6,10.181504705));
#217530=CARTESIAN_POINT('Ctrl Pts',(3.20095880099994,15.2,10.179531773));
#217531=CARTESIAN_POINT('Ctrl Pts',(3.20095880099994,11.6,10.179531773));
#217532=CARTESIAN_POINT('Ctrl Pts',(3.19973776199994,15.2,10.17756326));
#217533=CARTESIAN_POINT('Ctrl Pts',(3.19973776199994,11.6,10.17756326));
#217534=CARTESIAN_POINT('Ctrl Pts',(3.19852185399994,15.2,10.175599184));
#217535=CARTESIAN_POINT('Ctrl Pts',(3.19852185399994,11.6,10.175599184));
#217536=CARTESIAN_POINT('Ctrl Pts',(3.19731107699994,15.2,10.173639559));
#217537=CARTESIAN_POINT('Ctrl Pts',(3.19731107699994,11.6,10.173639559));
#217538=CARTESIAN_POINT('Ctrl Pts',(3.19610542999994,15.2,10.171684403));
#217539=CARTESIAN_POINT('Ctrl Pts',(3.19610542999994,11.6,10.171684403));
#217540=CARTESIAN_POINT('Ctrl Pts',(3.19490490899994,15.2,10.169733732));
#217541=CARTESIAN_POINT('Ctrl Pts',(3.19490490899994,11.6,10.169733732));
#217542=CARTESIAN_POINT('Ctrl Pts',(3.19370951399994,15.2,10.167787564));
#217543=CARTESIAN_POINT('Ctrl Pts',(3.19370951399994,11.6,10.167787564));
#217544=CARTESIAN_POINT('Ctrl Pts',(3.19251924199994,15.2,10.165845913));
#217545=CARTESIAN_POINT('Ctrl Pts',(3.19251924199994,11.6,10.165845913));
#217546=CARTESIAN_POINT('Ctrl Pts',(3.19133409399994,15.2,10.163908798));
#217547=CARTESIAN_POINT('Ctrl Pts',(3.19133409399994,11.6,10.163908798));
#217548=CARTESIAN_POINT('Ctrl Pts',(3.19015406399994,15.2,10.161976234));
#217549=CARTESIAN_POINT('Ctrl Pts',(3.19015406399994,11.6,10.161976234));
#217550=CARTESIAN_POINT('Ctrl Pts',(3.18897915299994,15.2,10.160048239));
#217551=CARTESIAN_POINT('Ctrl Pts',(3.18897915299994,11.6,10.160048239));
#217552=CARTESIAN_POINT('Ctrl Pts',(3.18780935899994,15.2,10.158124831));
#217553=CARTESIAN_POINT('Ctrl Pts',(3.18780935899994,11.6,10.158124831));
#217554=CARTESIAN_POINT('Ctrl Pts',(3.18664467899994,15.2,10.156206023));
#217555=CARTESIAN_POINT('Ctrl Pts',(3.18664467899994,11.6,10.156206023));
#217556=CARTESIAN_POINT('Ctrl Pts',(3.18548511399994,15.2,10.154291836));
#217557=CARTESIAN_POINT('Ctrl Pts',(3.18548511399994,11.6,10.154291836));
#217558=CARTESIAN_POINT('Ctrl Pts',(3.18433065699995,15.2,10.152382285));
#217559=CARTESIAN_POINT('Ctrl Pts',(3.18433065699995,11.6,10.152382285));
#217560=CARTESIAN_POINT('Ctrl Pts',(3.18318131199995,15.2,10.150477387));
#217561=CARTESIAN_POINT('Ctrl Pts',(3.18318131199995,11.6,10.150477387));
#217562=CARTESIAN_POINT('Ctrl Pts',(3.18203707299994,15.2,10.148577159));
#217563=CARTESIAN_POINT('Ctrl Pts',(3.18203707299994,11.6,10.148577159));
#217564=CARTESIAN_POINT('Ctrl Pts',(3.18089793999994,15.2,10.146681619));
#217565=CARTESIAN_POINT('Ctrl Pts',(3.18089793999994,11.6,10.146681619));
#217566=CARTESIAN_POINT('Ctrl Pts',(3.17976390999994,15.2,10.144790784));
#217567=CARTESIAN_POINT('Ctrl Pts',(3.17976390999994,11.6,10.144790784));
#217568=CARTESIAN_POINT('Ctrl Pts',(3.17863498099995,15.2,10.142904671));
#217569=CARTESIAN_POINT('Ctrl Pts',(3.17863498099995,11.6,10.142904671));
#217570=CARTESIAN_POINT('Ctrl Pts',(3.17751115299994,15.2,10.141023297));
#217571=CARTESIAN_POINT('Ctrl Pts',(3.17751115299994,11.6,10.141023297));
#217572=CARTESIAN_POINT('Ctrl Pts',(3.17639242199995,15.2,10.13914668));
#217573=CARTESIAN_POINT('Ctrl Pts',(3.17639242199995,11.6,10.13914668));
#217574=CARTESIAN_POINT('Ctrl Pts',(3.17527878599994,15.2,10.137274836));
#217575=CARTESIAN_POINT('Ctrl Pts',(3.17527878599994,11.6,10.137274836));
#217576=CARTESIAN_POINT('Ctrl Pts',(3.17417024399994,15.2,10.135407784));
#217577=CARTESIAN_POINT('Ctrl Pts',(3.17417024399994,11.6,10.135407784));
#217578=CARTESIAN_POINT('Ctrl Pts',(3.17306679399994,15.2,10.133545542));
#217579=CARTESIAN_POINT('Ctrl Pts',(3.17306679399994,11.6,10.133545542));
#217580=CARTESIAN_POINT('Ctrl Pts',(3.17196843199994,15.2,10.131688125));
#217581=CARTESIAN_POINT('Ctrl Pts',(3.17196843199994,11.6,10.131688125));
#217582=CARTESIAN_POINT('Ctrl Pts',(3.17087515899994,15.2,10.129835553));
#217583=CARTESIAN_POINT('Ctrl Pts',(3.17087515899994,11.6,10.129835553));
#217584=CARTESIAN_POINT('Ctrl Pts',(3.16978697099994,15.2,10.127987842));
#217585=CARTESIAN_POINT('Ctrl Pts',(3.16978697099994,11.6,10.127987842));
#217586=CARTESIAN_POINT('Ctrl Pts',(3.16870386699994,15.2,10.126145011));
#217587=CARTESIAN_POINT('Ctrl Pts',(3.16870386699994,11.6,10.126145011));
#217588=CARTESIAN_POINT('Ctrl Pts',(3.16762584299994,15.2,10.124307078));
#217589=CARTESIAN_POINT('Ctrl Pts',(3.16762584299994,11.6,10.124307078));
#217590=CARTESIAN_POINT('Ctrl Pts',(3.16655289799994,15.2,10.12247406));
#217591=CARTESIAN_POINT('Ctrl Pts',(3.16655289799994,11.6,10.12247406));
#217592=CARTESIAN_POINT('Ctrl Pts',(3.16548502999995,15.2,10.120645975));
#217593=CARTESIAN_POINT('Ctrl Pts',(3.16548502999995,11.6,10.120645975));
#217594=CARTESIAN_POINT('Ctrl Pts',(3.16442223699994,15.2,10.11882284));
#217595=CARTESIAN_POINT('Ctrl Pts',(3.16442223699994,11.6,10.11882284));
#217596=CARTESIAN_POINT('Ctrl Pts',(3.16336451599994,15.2,10.117004675));
#217597=CARTESIAN_POINT('Ctrl Pts',(3.16336451599994,11.6,10.117004675));
#217598=CARTESIAN_POINT('Ctrl Pts',(3.16231186499994,15.2,10.115191496));
#217599=CARTESIAN_POINT('Ctrl Pts',(3.16231186499994,11.6,10.115191496));
#217600=CARTESIAN_POINT('Ctrl Pts',(3.16126428299994,15.2,10.113383323));
#217601=CARTESIAN_POINT('Ctrl Pts',(3.16126428299994,11.6,10.113383323));
#217602=CARTESIAN_POINT('Ctrl Pts',(3.16022176599994,15.2,10.111580173));
#217603=CARTESIAN_POINT('Ctrl Pts',(3.16022176599994,11.6,10.111580173));
#217604=CARTESIAN_POINT('Ctrl Pts',(3.15918431399994,15.2,10.109782065));
#217605=CARTESIAN_POINT('Ctrl Pts',(3.15918431399994,11.6,10.109782065));
#217606=CARTESIAN_POINT('Ctrl Pts',(3.15815192199994,15.2,10.107989016));
#217607=CARTESIAN_POINT('Ctrl Pts',(3.15815192199994,11.6,10.107989016));
#217608=CARTESIAN_POINT('Ctrl Pts',(3.15712458699994,15.2,10.106201046));
#217609=CARTESIAN_POINT('Ctrl Pts',(3.15712458699994,11.6,10.106201046));
#217610=CARTESIAN_POINT('Ctrl Pts',(3.15610231199994,15.2,10.104418172));
#217611=CARTESIAN_POINT('Ctrl Pts',(3.15610231199994,11.6,10.104418172));
#217612=CARTESIAN_POINT('Ctrl Pts',(3.15508508899994,15.2,10.102640413));
#217613=CARTESIAN_POINT('Ctrl Pts',(3.15508508899994,11.6,10.102640413));
#217614=CARTESIAN_POINT('Ctrl Pts',(3.15407291799994,15.2,10.100867788));
#217615=CARTESIAN_POINT('Ctrl Pts',(3.15407291799994,11.6,10.100867788));
#217616=CARTESIAN_POINT('Ctrl Pts',(3.15306579799994,15.2,10.099100315));
#217617=CARTESIAN_POINT('Ctrl Pts',(3.15306579799994,11.6,10.099100315));
#217618=CARTESIAN_POINT('Ctrl Pts',(3.15206372299994,15.2,10.097338013));
#217619=CARTESIAN_POINT('Ctrl Pts',(3.15206372299994,11.6,10.097338013));
#217620=CARTESIAN_POINT('Ctrl Pts',(3.15106669299994,15.2,10.0955809));
#217621=CARTESIAN_POINT('Ctrl Pts',(3.15106669299994,11.6,10.0955809));
#217622=CARTESIAN_POINT('Ctrl Pts',(3.15007470599994,15.2,10.093828996));
#217623=CARTESIAN_POINT('Ctrl Pts',(3.15007470599994,11.6,10.093828996));
#217624=CARTESIAN_POINT('Ctrl Pts',(3.14908775899994,15.2,10.092082318));
#217625=CARTESIAN_POINT('Ctrl Pts',(3.14908775899994,11.6,10.092082318));
#217626=CARTESIAN_POINT('Ctrl Pts',(3.14810584799994,15.2,10.090340886));
#217627=CARTESIAN_POINT('Ctrl Pts',(3.14810584799994,11.6,10.090340886));
#217628=CARTESIAN_POINT('Ctrl Pts',(3.14712897199994,15.2,10.08860472));
#217629=CARTESIAN_POINT('Ctrl Pts',(3.14712897199994,11.6,10.08860472));
#217630=CARTESIAN_POINT('Ctrl Pts',(3.14615712899994,15.2,10.086873837));
#217631=CARTESIAN_POINT('Ctrl Pts',(3.14615712899994,11.6,10.086873837));
#217632=CARTESIAN_POINT('Ctrl Pts',(3.14519031499994,15.2,10.085148257));
#217633=CARTESIAN_POINT('Ctrl Pts',(3.14519031499994,11.6,10.085148257));
#217634=CARTESIAN_POINT('Ctrl Pts',(3.14422852799995,15.2,10.083427999));
#217635=CARTESIAN_POINT('Ctrl Pts',(3.14422852799995,11.6,10.083427999));
#217636=CARTESIAN_POINT('Ctrl Pts',(3.14327176599994,15.2,10.081713083));
#217637=CARTESIAN_POINT('Ctrl Pts',(3.14327176599994,11.6,10.081713083));
#217638=CARTESIAN_POINT('Ctrl Pts',(3.14232002399994,15.2,10.080003527));
#217639=CARTESIAN_POINT('Ctrl Pts',(3.14232002399994,11.6,10.080003527));
#217640=CARTESIAN_POINT('Ctrl Pts',(3.14137330399994,15.2,10.078299351));
#217641=CARTESIAN_POINT('Ctrl Pts',(3.14137330399994,11.6,10.078299351));
#217642=CARTESIAN_POINT('Ctrl Pts',(3.14043159899994,15.2,10.076600574));
#217643=CARTESIAN_POINT('Ctrl Pts',(3.14043159899994,11.6,10.076600574));
#217644=CARTESIAN_POINT('Ctrl Pts',(3.13949490699994,15.2,10.074907216));
#217645=CARTESIAN_POINT('Ctrl Pts',(3.13949490699994,11.6,10.074907216));
#217646=CARTESIAN_POINT('Ctrl Pts',(3.13856322699994,15.2,10.073219296));
#217647=CARTESIAN_POINT('Ctrl Pts',(3.13856322699994,11.6,10.073219296));
#217648=CARTESIAN_POINT('Ctrl Pts',(3.13763655599994,15.2,10.071536834));
#217649=CARTESIAN_POINT('Ctrl Pts',(3.13763655599994,11.6,10.071536834));
#217650=CARTESIAN_POINT('Ctrl Pts',(3.13671488999994,15.2,10.069859849));
#217651=CARTESIAN_POINT('Ctrl Pts',(3.13671488999994,11.6,10.069859849));
#217652=CARTESIAN_POINT('Ctrl Pts',(3.13579822699994,15.2,10.068188362));
#217653=CARTESIAN_POINT('Ctrl Pts',(3.13579822699994,11.6,10.068188362));
#217654=CARTESIAN_POINT('Ctrl Pts',(3.13488656499994,15.2,10.066522392));
#217655=CARTESIAN_POINT('Ctrl Pts',(3.13488656499994,11.6,10.066522392));
#217656=CARTESIAN_POINT('Ctrl Pts',(3.13397989999994,15.2,10.064861958));
#217657=CARTESIAN_POINT('Ctrl Pts',(3.13397989999994,11.6,10.064861958));
#217658=CARTESIAN_POINT('Ctrl Pts',(3.13307822999994,15.2,10.063207081));
#217659=CARTESIAN_POINT('Ctrl Pts',(3.13307822999994,11.6,10.063207081));
#217660=CARTESIAN_POINT('Ctrl Pts',(3.13218154999995,15.2,10.061557781));
#217661=CARTESIAN_POINT('Ctrl Pts',(3.13218154999995,11.6,10.061557781));
#217662=CARTESIAN_POINT('Ctrl Pts',(3.13128985999994,15.2,10.059914077));
#217663=CARTESIAN_POINT('Ctrl Pts',(3.13128985999994,11.6,10.059914077));
#217664=CARTESIAN_POINT('Ctrl Pts',(3.13040315599994,15.2,10.058275991));
#217665=CARTESIAN_POINT('Ctrl Pts',(3.13040315599994,11.6,10.058275991));
#217666=CARTESIAN_POINT('Ctrl Pts',(3.12952143499994,15.2,10.056643542));
#217667=CARTESIAN_POINT('Ctrl Pts',(3.12952143499994,11.6,10.056643542));
#217668=CARTESIAN_POINT('Ctrl Pts',(3.12864469399994,15.2,10.05501675));
#217669=CARTESIAN_POINT('Ctrl Pts',(3.12864469399994,11.6,10.05501675));
#217670=CARTESIAN_POINT('Ctrl Pts',(3.12777292999994,15.2,10.053395635));
#217671=CARTESIAN_POINT('Ctrl Pts',(3.12777292999994,11.6,10.053395635));
#217672=CARTESIAN_POINT('Ctrl Pts',(3.12690613999994,15.2,10.051780219));
#217673=CARTESIAN_POINT('Ctrl Pts',(3.12690613999994,11.6,10.051780219));
#217674=CARTESIAN_POINT('Ctrl Pts',(3.12604432099994,15.2,10.050170521));
#217675=CARTESIAN_POINT('Ctrl Pts',(3.12604432099994,11.6,10.050170521));
#217676=CARTESIAN_POINT('Ctrl Pts',(3.12518747099995,15.2,10.048566563));
#217677=CARTESIAN_POINT('Ctrl Pts',(3.12518747099995,11.6,10.048566563));
#217678=CARTESIAN_POINT('Ctrl Pts',(3.12433558499994,15.2,10.046968364));
#217679=CARTESIAN_POINT('Ctrl Pts',(3.12433558499994,11.6,10.046968364));
#217680=CARTESIAN_POINT('Ctrl Pts',(3.12348866099994,15.2,10.045375946));
#217681=CARTESIAN_POINT('Ctrl Pts',(3.12348866099994,11.6,10.045375946));
#217682=CARTESIAN_POINT('Ctrl Pts',(3.12264669699994,15.2,10.043789328));
#217683=CARTESIAN_POINT('Ctrl Pts',(3.12264669699994,11.6,10.043789328));
#217684=CARTESIAN_POINT('Ctrl Pts',(3.12180968799994,15.2,10.042208533));
#217685=CARTESIAN_POINT('Ctrl Pts',(3.12180968799994,11.6,10.042208533));
#217686=CARTESIAN_POINT('Ctrl Pts',(3.12097763099994,15.2,10.040633581));
#217687=CARTESIAN_POINT('Ctrl Pts',(3.12097763099994,11.6,10.040633581));
#217688=CARTESIAN_POINT('Ctrl Pts',(3.12015052399994,15.2,10.039064492));
#217689=CARTESIAN_POINT('Ctrl Pts',(3.12015052399994,11.6,10.039064492));
#217690=CARTESIAN_POINT('Ctrl Pts',(3.11932836299994,15.2,10.037501289));
#217691=CARTESIAN_POINT('Ctrl Pts',(3.11932836299994,11.6,10.037501289));
#217692=CARTESIAN_POINT('Ctrl Pts',(3.11851114499994,15.2,10.035943991));
#217693=CARTESIAN_POINT('Ctrl Pts',(3.11851114499994,11.6,10.035943991));
#217694=CARTESIAN_POINT('Ctrl Pts',(3.11769886699994,15.2,10.034392622));
#217695=CARTESIAN_POINT('Ctrl Pts',(3.11769886699994,11.6,10.034392622));
#217696=CARTESIAN_POINT('Ctrl Pts',(3.11689152499994,15.2,10.0328472));
#217697=CARTESIAN_POINT('Ctrl Pts',(3.11689152499994,11.6,10.0328472));
#217698=CARTESIAN_POINT('Ctrl Pts',(3.11608911699994,15.2,10.031307748));
#217699=CARTESIAN_POINT('Ctrl Pts',(3.11608911699994,11.6,10.031307748));
#217700=CARTESIAN_POINT('Ctrl Pts',(3.11529163799994,15.2,10.029774289));
#217701=CARTESIAN_POINT('Ctrl Pts',(3.11529163799994,11.6,10.029774289));
#217702=CARTESIAN_POINT('Ctrl Pts',(3.11449908499994,15.2,10.028246841));
#217703=CARTESIAN_POINT('Ctrl Pts',(3.11449908499994,11.6,10.028246841));
#217704=CARTESIAN_POINT('Ctrl Pts',(3.11371145699994,15.2,10.026725429));
#217705=CARTESIAN_POINT('Ctrl Pts',(3.11371145699994,11.6,10.026725429));
#217706=CARTESIAN_POINT('Ctrl Pts',(3.11292874799994,15.2,10.025210072));
#217707=CARTESIAN_POINT('Ctrl Pts',(3.11292874799994,11.6,10.025210072));
#217708=CARTESIAN_POINT('Ctrl Pts',(3.11215095499994,15.2,10.023700794));
#217709=CARTESIAN_POINT('Ctrl Pts',(3.11215095499994,11.6,10.023700794));
#217710=CARTESIAN_POINT('Ctrl Pts',(3.11137807399994,15.2,10.022197616));
#217711=CARTESIAN_POINT('Ctrl Pts',(3.11137807399994,11.6,10.022197616));
#217712=CARTESIAN_POINT('Ctrl Pts',(3.11061010399994,15.2,10.020700559));
#217713=CARTESIAN_POINT('Ctrl Pts',(3.11061010399994,11.6,10.020700559));
#217714=CARTESIAN_POINT('Ctrl Pts',(3.10984703899994,15.2,10.019209646));
#217715=CARTESIAN_POINT('Ctrl Pts',(3.10984703899994,11.6,10.019209646));
#217716=CARTESIAN_POINT('Ctrl Pts',(3.10908887599994,15.2,10.017724899));
#217717=CARTESIAN_POINT('Ctrl Pts',(3.10908887599994,11.6,10.017724899));
#217718=CARTESIAN_POINT('Ctrl Pts',(3.10833561299994,15.2,10.01624634));
#217719=CARTESIAN_POINT('Ctrl Pts',(3.10833561299994,11.6,10.01624634));
#217720=CARTESIAN_POINT('Ctrl Pts',(3.10758724499994,15.2,10.01477399));
#217721=CARTESIAN_POINT('Ctrl Pts',(3.10758724499994,11.6,10.01477399));
#217722=CARTESIAN_POINT('Ctrl Pts',(3.10684376799994,15.2,10.013307874));
#217723=CARTESIAN_POINT('Ctrl Pts',(3.10684376799994,11.6,10.013307874));
#217724=CARTESIAN_POINT('Ctrl Pts',(3.10610517999995,15.2,10.011848013));
#217725=CARTESIAN_POINT('Ctrl Pts',(3.10610517999995,11.6,10.011848013));
#217726=CARTESIAN_POINT('Ctrl Pts',(3.10537147499995,15.2,10.010394428));
#217727=CARTESIAN_POINT('Ctrl Pts',(3.10537147499995,11.6,10.010394428));
#217728=CARTESIAN_POINT('Ctrl Pts',(3.10464265199994,15.2,10.008947144));
#217729=CARTESIAN_POINT('Ctrl Pts',(3.10464265199994,11.6,10.008947144));
#217730=CARTESIAN_POINT('Ctrl Pts',(3.10391870499994,15.2,10.007506183));
#217731=CARTESIAN_POINT('Ctrl Pts',(3.10391870499994,11.6,10.007506183));
#217732=CARTESIAN_POINT('Ctrl Pts',(3.10319963199994,15.2,10.006071567));
#217733=CARTESIAN_POINT('Ctrl Pts',(3.10319963199994,11.6,10.006071567));
#217734=CARTESIAN_POINT('Ctrl Pts',(3.10248542799994,15.2,10.00464332));
#217735=CARTESIAN_POINT('Ctrl Pts',(3.10248542799994,11.6,10.00464332));
#217736=CARTESIAN_POINT('Ctrl Pts',(3.10177608999994,15.2,10.003221464));
#217737=CARTESIAN_POINT('Ctrl Pts',(3.10177608999994,11.6,10.003221464));
#217738=CARTESIAN_POINT('Ctrl Pts',(3.10107161399995,15.2,10.001806022));
#217739=CARTESIAN_POINT('Ctrl Pts',(3.10107161399995,11.6,10.001806022));
#217740=CARTESIAN_POINT('Ctrl Pts',(3.10037199499994,15.2,10.000397017));
#217741=CARTESIAN_POINT('Ctrl Pts',(3.10037199499994,11.6,10.000397017));
#217742=CARTESIAN_POINT('Ctrl Pts',(3.09967723099994,15.2,9.99899447299999));
#217743=CARTESIAN_POINT('Ctrl Pts',(3.09967723099994,11.6,9.99899447299999));
#217744=CARTESIAN_POINT('Ctrl Pts',(3.09898731599994,15.2,9.99759841199998));
#217745=CARTESIAN_POINT('Ctrl Pts',(3.09898731599994,11.6,9.99759841199998));
#217746=CARTESIAN_POINT('Ctrl Pts',(3.09830224899994,15.2,9.99620885899999));
#217747=CARTESIAN_POINT('Ctrl Pts',(3.09830224899994,11.6,9.99620885899999));
#217748=CARTESIAN_POINT('Ctrl Pts',(3.09762202399994,15.2,9.99482583699999));
#217749=CARTESIAN_POINT('Ctrl Pts',(3.09762202399994,11.6,9.99482583699999));
#217750=CARTESIAN_POINT('Ctrl Pts',(3.09694663699994,15.2,9.99344936799999));
#217751=CARTESIAN_POINT('Ctrl Pts',(3.09694663699994,11.6,9.99344936799999));
#217752=CARTESIAN_POINT('Ctrl Pts',(3.09627608499994,15.2,9.99207947799999));
#217753=CARTESIAN_POINT('Ctrl Pts',(3.09627608499994,11.6,9.99207947799999));
#217754=CARTESIAN_POINT('Ctrl Pts',(3.09561036199994,15.2,9.99071618899999));
#217755=CARTESIAN_POINT('Ctrl Pts',(3.09561036199994,11.6,9.99071618899999));
#217756=CARTESIAN_POINT('Ctrl Pts',(3.09494946499994,15.2,9.98935952599999));
#217757=CARTESIAN_POINT('Ctrl Pts',(3.09494946499994,11.6,9.98935952599999));
#217758=CARTESIAN_POINT('Ctrl Pts',(3.09429339099994,15.2,9.98800951199998));
#217759=CARTESIAN_POINT('Ctrl Pts',(3.09429339099994,11.6,9.98800951199998));
#217760=CARTESIAN_POINT('Ctrl Pts',(3.09364213499994,15.2,9.98666617199999));
#217761=CARTESIAN_POINT('Ctrl Pts',(3.09364213499994,11.6,9.98666617199999));
#217762=CARTESIAN_POINT('Ctrl Pts',(3.09299569299994,15.2,9.98532952799999));
#217763=CARTESIAN_POINT('Ctrl Pts',(3.09299569299994,11.6,9.98532952799999));
#217764=CARTESIAN_POINT('Ctrl Pts',(3.09235405999994,15.2,9.98399960799999));
#217765=CARTESIAN_POINT('Ctrl Pts',(3.09235405999994,11.6,9.98399960799999));
#217766=CARTESIAN_POINT('Ctrl Pts',(3.09171723299994,15.2,9.98267643199998));
#217767=CARTESIAN_POINT('Ctrl Pts',(3.09171723299994,11.6,9.98267643199998));
#217768=CARTESIAN_POINT('Ctrl Pts',(3.09108520699994,15.2,9.98136002699999));
#217769=CARTESIAN_POINT('Ctrl Pts',(3.09108520699994,11.6,9.98136002699999));
#217770=CARTESIAN_POINT('Ctrl Pts',(3.09045797699994,15.2,9.98005041799999));
#217771=CARTESIAN_POINT('Ctrl Pts',(3.09045797699994,11.6,9.98005041799999));
#217772=CARTESIAN_POINT('Ctrl Pts',(3.08983553999994,15.2,9.97874762799999));
#217773=CARTESIAN_POINT('Ctrl Pts',(3.08983553999994,11.6,9.97874762799999));
#217774=CARTESIAN_POINT('Ctrl Pts',(3.08921789099994,15.2,9.97745168099998));
#217775=CARTESIAN_POINT('Ctrl Pts',(3.08921789099994,11.6,9.97745168099998));
#217776=CARTESIAN_POINT('Ctrl Pts',(3.08860502499994,15.2,9.97616260499999));
#217777=CARTESIAN_POINT('Ctrl Pts',(3.08860502499994,11.6,9.97616260499999));
#217778=CARTESIAN_POINT('Ctrl Pts',(3.08799693999994,15.2,9.97488042299998));
#217779=CARTESIAN_POINT('Ctrl Pts',(3.08799693999994,11.6,9.97488042299998));
#217780=CARTESIAN_POINT('Ctrl Pts',(3.08739362899995,15.2,9.97360515799999));
#217781=CARTESIAN_POINT('Ctrl Pts',(3.08739362899995,11.6,9.97360515799999));
#217782=CARTESIAN_POINT('Ctrl Pts',(3.08679508799994,15.2,9.97233683899999));
#217783=CARTESIAN_POINT('Ctrl Pts',(3.08679508799994,11.6,9.97233683899999));
#217784=CARTESIAN_POINT('Ctrl Pts',(3.08620131299994,15.2,9.97107548899999));
#217785=CARTESIAN_POINT('Ctrl Pts',(3.08620131299994,11.6,9.97107548899999));
#217786=CARTESIAN_POINT('Ctrl Pts',(3.08561229999994,15.2,9.96982113299998));
#217787=CARTESIAN_POINT('Ctrl Pts',(3.08561229999994,11.6,9.96982113299998));
#217788=CARTESIAN_POINT('Ctrl Pts',(3.08502804299994,15.2,9.96857379799999));
#217789=CARTESIAN_POINT('Ctrl Pts',(3.08502804299994,11.6,9.96857379799999));
#217790=CARTESIAN_POINT('Ctrl Pts',(3.08444853899994,15.2,9.96733350799998));
#217791=CARTESIAN_POINT('Ctrl Pts',(3.08444853899994,11.6,9.96733350799998));
#217792=CARTESIAN_POINT('Ctrl Pts',(3.08387378199994,15.2,9.96610028999999));
#217793=CARTESIAN_POINT('Ctrl Pts',(3.08387378199994,11.6,9.96610028999999));
#217794=CARTESIAN_POINT('Ctrl Pts',(3.08330376799994,15.2,9.96487416799998));
#217795=CARTESIAN_POINT('Ctrl Pts',(3.08330376799994,11.6,9.96487416799998));
#217796=CARTESIAN_POINT('Ctrl Pts',(3.08273849199994,15.2,9.96365516999998));
#217797=CARTESIAN_POINT('Ctrl Pts',(3.08273849199994,11.6,9.96365516999998));
#217798=CARTESIAN_POINT('Ctrl Pts',(3.08217794999994,15.2,9.96244332099998));
#217799=CARTESIAN_POINT('Ctrl Pts',(3.08217794999994,11.6,9.96244332099998));
#217800=CARTESIAN_POINT('Ctrl Pts',(3.08162213499994,15.2,9.96123864599999));
#217801=CARTESIAN_POINT('Ctrl Pts',(3.08162213499994,11.6,9.96123864599999));
#217802=CARTESIAN_POINT('Ctrl Pts',(3.08107104499994,15.2,9.96004117299999));
#217803=CARTESIAN_POINT('Ctrl Pts',(3.08107104499994,11.6,9.96004117299999));
#217804=CARTESIAN_POINT('Ctrl Pts',(3.08052467399994,15.2,9.95885092599998));
#217805=CARTESIAN_POINT('Ctrl Pts',(3.08052467399994,11.6,9.95885092599998));
#217806=CARTESIAN_POINT('Ctrl Pts',(3.07998301799994,15.2,9.95766793499998));
#217807=CARTESIAN_POINT('Ctrl Pts',(3.07998301799994,11.6,9.95766793499998));
#217808=CARTESIAN_POINT('Ctrl Pts',(3.07944606999994,15.2,9.95649222299999));
#217809=CARTESIAN_POINT('Ctrl Pts',(3.07944606999994,11.6,9.95649222299999));
#217810=CARTESIAN_POINT('Ctrl Pts',(3.07891382499994,15.2,9.95532381799999));
#217811=CARTESIAN_POINT('Ctrl Pts',(3.07891382499994,11.6,9.95532381799999));
#217812=CARTESIAN_POINT('Ctrl Pts',(3.07838628099995,15.2,9.95416274699998));
#217813=CARTESIAN_POINT('Ctrl Pts',(3.07838628099995,11.6,9.95416274699998));
#217814=CARTESIAN_POINT('Ctrl Pts',(3.07786343199994,15.2,9.95300903699999));
#217815=CARTESIAN_POINT('Ctrl Pts',(3.07786343199994,11.6,9.95300903699999));
#217816=CARTESIAN_POINT('Ctrl Pts',(3.07734526999994,15.2,9.95186271399999));
#217817=CARTESIAN_POINT('Ctrl Pts',(3.07734526999994,11.6,9.95186271399999));
#217818=CARTESIAN_POINT('Ctrl Pts',(3.07683179299994,15.2,9.95072380599998));
#217819=CARTESIAN_POINT('Ctrl Pts',(3.07683179299994,11.6,9.95072380599998));
#217820=CARTESIAN_POINT('Ctrl Pts',(3.07632299499994,15.2,9.94959233999998));
#217821=CARTESIAN_POINT('Ctrl Pts',(3.07632299499994,11.6,9.94959233999998));
#217822=CARTESIAN_POINT('Ctrl Pts',(3.07581887099994,15.2,9.94846834399999));
#217823=CARTESIAN_POINT('Ctrl Pts',(3.07581887099994,11.6,9.94846834399999));
#217824=CARTESIAN_POINT('Ctrl Pts',(3.07531941599994,15.2,9.94735184399998));
#217825=CARTESIAN_POINT('Ctrl Pts',(3.07531941599994,11.6,9.94735184399998));
#217826=CARTESIAN_POINT('Ctrl Pts',(3.07482462299994,15.2,9.94624286799999));
#217827=CARTESIAN_POINT('Ctrl Pts',(3.07482462299994,11.6,9.94624286799999));
#217828=CARTESIAN_POINT('Ctrl Pts',(3.07433448899994,15.2,9.94514144399999));
#217829=CARTESIAN_POINT('Ctrl Pts',(3.07433448899994,11.6,9.94514144399999));
#217830=CARTESIAN_POINT('Ctrl Pts',(3.07384900699994,15.2,9.94404759999998));
#217831=CARTESIAN_POINT('Ctrl Pts',(3.07384900699994,11.6,9.94404759999998));
#217832=CARTESIAN_POINT('Ctrl Pts',(3.07336817399994,15.2,9.94296136499998));
#217833=CARTESIAN_POINT('Ctrl Pts',(3.07336817399994,11.6,9.94296136499998));
#217834=CARTESIAN_POINT('Ctrl Pts',(3.07289198199994,15.2,9.94188276499998));
#217835=CARTESIAN_POINT('Ctrl Pts',(3.07289198199994,11.6,9.94188276499998));
#217836=CARTESIAN_POINT('Ctrl Pts',(3.07242042599994,15.2,9.94081182999999));
#217837=CARTESIAN_POINT('Ctrl Pts',(3.07242042599994,11.6,9.94081182999999));
#217838=CARTESIAN_POINT('Ctrl Pts',(3.07195350199994,15.2,9.93974858599999));
#217839=CARTESIAN_POINT('Ctrl Pts',(3.07195350199994,11.6,9.93974858599999));
#217840=CARTESIAN_POINT('Ctrl Pts',(3.07149120299994,15.2,9.93869306299998));
#217841=CARTESIAN_POINT('Ctrl Pts',(3.07149120299994,11.6,9.93869306299998));
#217842=CARTESIAN_POINT('Ctrl Pts',(3.07103352399994,15.2,9.93764528999998));
#217843=CARTESIAN_POINT('Ctrl Pts',(3.07103352399994,11.6,9.93764528999998));
#217844=CARTESIAN_POINT('Ctrl Pts',(3.07058045999994,15.2,9.93660529599998));
#217845=CARTESIAN_POINT('Ctrl Pts',(3.07058045999994,11.6,9.93660529599998));
#217846=CARTESIAN_POINT('Ctrl Pts',(3.07013200399994,15.2,9.93557310899998));
#217847=CARTESIAN_POINT('Ctrl Pts',(3.07013200399994,11.6,9.93557310899998));
#217848=CARTESIAN_POINT('Ctrl Pts',(3.06968815199995,15.2,9.93454875599999));
#217849=CARTESIAN_POINT('Ctrl Pts',(3.06968815199995,11.6,9.93454875599999));
#217850=CARTESIAN_POINT('Ctrl Pts',(3.06924889699994,15.2,9.93353227099998));
#217851=CARTESIAN_POINT('Ctrl Pts',(3.06924889699994,11.6,9.93353227099998));
#217852=CARTESIAN_POINT('Ctrl Pts',(3.06881423399994,15.2,9.93252367899998));
#217853=CARTESIAN_POINT('Ctrl Pts',(3.06881423399994,11.6,9.93252367899998));
#217854=CARTESIAN_POINT('Ctrl Pts',(3.06838415699994,15.2,9.93152301099999));
#217855=CARTESIAN_POINT('Ctrl Pts',(3.06838415699994,11.6,9.93152301099999));
#217856=CARTESIAN_POINT('Ctrl Pts',(3.06795865999994,15.2,9.93053029599999));
#217857=CARTESIAN_POINT('Ctrl Pts',(3.06795865999994,11.6,9.93053029599999));
#217858=CARTESIAN_POINT('Ctrl Pts',(3.06753773799994,15.2,9.92954556499999));
#217859=CARTESIAN_POINT('Ctrl Pts',(3.06753773799994,11.6,9.92954556499999));
#217860=CARTESIAN_POINT('Ctrl Pts',(3.06712138399994,15.2,9.92856884599998));
#217861=CARTESIAN_POINT('Ctrl Pts',(3.06712138399994,11.6,9.92856884599998));
#217862=CARTESIAN_POINT('Ctrl Pts',(3.06670959199994,15.2,9.92760017099998));
#217863=CARTESIAN_POINT('Ctrl Pts',(3.06670959199994,11.6,9.92760017099998));
#217864=CARTESIAN_POINT('Ctrl Pts',(3.06630235599994,15.2,9.92663956799999));
#217865=CARTESIAN_POINT('Ctrl Pts',(3.06630235599994,11.6,9.92663956799999));
#217866=CARTESIAN_POINT('Ctrl Pts',(3.06589967099994,15.2,9.92568706699998));
#217867=CARTESIAN_POINT('Ctrl Pts',(3.06589967099994,11.6,9.92568706699998));
#217868=CARTESIAN_POINT('Ctrl Pts',(3.06550152999994,15.2,9.92474270099999));
#217869=CARTESIAN_POINT('Ctrl Pts',(3.06550152999994,11.6,9.92474270099999));
#217870=CARTESIAN_POINT('Ctrl Pts',(3.06510792699994,15.2,9.92380649899999));
#217871=CARTESIAN_POINT('Ctrl Pts',(3.06510792699994,11.6,9.92380649899999));
#217872=CARTESIAN_POINT('Ctrl Pts',(3.06471885599994,15.2,9.92287849099998));
#217873=CARTESIAN_POINT('Ctrl Pts',(3.06471885599994,11.6,9.92287849099998));
#217874=CARTESIAN_POINT('Ctrl Pts',(3.06433431199994,15.2,9.92195870799998));
#217875=CARTESIAN_POINT('Ctrl Pts',(3.06433431199994,11.6,9.92195870799998));
#217876=CARTESIAN_POINT('Ctrl Pts',(3.06395428599994,15.2,9.92104718299998));
#217877=CARTESIAN_POINT('Ctrl Pts',(3.06395428599994,11.6,9.92104718299998));
#217878=CARTESIAN_POINT('Ctrl Pts',(3.06357877399994,15.2,9.92014394499999));
#217879=CARTESIAN_POINT('Ctrl Pts',(3.06357877399994,11.6,9.92014394499999));
#217880=CARTESIAN_POINT('Ctrl Pts',(3.06320776799994,15.2,9.91924902499999));
#217881=CARTESIAN_POINT('Ctrl Pts',(3.06320776799994,11.6,9.91924902499999));
#217882=CARTESIAN_POINT('Ctrl Pts',(3.06284126399994,15.2,9.91836245599998));
#217883=CARTESIAN_POINT('Ctrl Pts',(3.06284126399994,11.6,9.91836245599998));
#217884=CARTESIAN_POINT('Ctrl Pts',(3.06247925299994,15.2,9.91748426799998));
#217885=CARTESIAN_POINT('Ctrl Pts',(3.06247925299994,11.6,9.91748426799998));
#217886=CARTESIAN_POINT('Ctrl Pts',(3.06212172999994,15.2,9.91661449399999));
#217887=CARTESIAN_POINT('Ctrl Pts',(3.06212172999994,11.6,9.91661449399999));
#217888=CARTESIAN_POINT('Ctrl Pts',(3.06176868699994,15.2,9.91575316599998));
#217889=CARTESIAN_POINT('Ctrl Pts',(3.06176868699994,11.6,9.91575316599998));
#217890=CARTESIAN_POINT('Ctrl Pts',(3.06142212599994,15.2,9.91490522599998));
#217891=CARTESIAN_POINT('Ctrl Pts',(3.06142212599994,11.6,9.91490522599998));
#217892=CARTESIAN_POINT('Ctrl Pts',(3.06114880299994,15.2,9.91423456699999));
#217893=CARTESIAN_POINT('Ctrl Pts',(3.06114880299994,11.6,9.91423456699999));
#217894=CARTESIAN_POINT('Ctrl Pts',(3.06094627499994,15.2,9.91373655899999));
#217895=CARTESIAN_POINT('Ctrl Pts',(3.06094627499994,11.6,9.91373655899999));
#217896=CARTESIAN_POINT('Ctrl Pts',(3.06081277599994,15.2,9.91340782599998));
#217897=CARTESIAN_POINT('Ctrl Pts',(3.06081277599994,11.6,9.91340782599998));
#217898=CARTESIAN_POINT('Ctrl Pts',(3.06074721199994,15.2,9.91324626499999));
#217899=CARTESIAN_POINT('Ctrl Pts',(3.06074721199994,11.6,9.91324626499999));
#217900=CARTESIAN_POINT('',(3.06074721199994,12.2,9.91324626499999));
#217901=CARTESIAN_POINT('',(3.06074721199994,15.2,9.91324626499999));
#217902=CARTESIAN_POINT('',(3.06074721199994,12.2,9.91324626499999));
#217903=CARTESIAN_POINT('Ctrl Pts',(3.76106045499994,12.2,10.867585944));
#217904=CARTESIAN_POINT('Ctrl Pts',(3.76051902299994,12.2,10.867046091));
#217905=CARTESIAN_POINT('Ctrl Pts',(3.75943667399994,12.2,10.865966495));
#217906=CARTESIAN_POINT('Ctrl Pts',(3.75781469799994,12.2,10.864347421));
#217907=CARTESIAN_POINT('Ctrl Pts',(3.75565515599994,12.2,10.862189302));
#217908=CARTESIAN_POINT('Ctrl Pts',(3.75296088399994,12.2,10.85949273));
#217909=CARTESIAN_POINT('Ctrl Pts',(3.75027176799994,12.2,10.856797236));
#217910=CARTESIAN_POINT('Ctrl Pts',(3.74758780799994,12.2,10.854102822));
#217911=CARTESIAN_POINT('Ctrl Pts',(3.74490900499994,12.2,10.85140949));
#217912=CARTESIAN_POINT('Ctrl Pts',(3.74223535999994,12.2,10.84871725));
#217913=CARTESIAN_POINT('Ctrl Pts',(3.73956687399994,12.2,10.846026106));
#217914=CARTESIAN_POINT('Ctrl Pts',(3.73690354699994,12.2,10.843336071));
#217915=CARTESIAN_POINT('Ctrl Pts',(3.73424538199994,12.2,10.840647153));
#217916=CARTESIAN_POINT('Ctrl Pts',(3.73159237799995,12.2,10.837959365));
#217917=CARTESIAN_POINT('Ctrl Pts',(3.72894453699994,12.2,10.835272717));
#217918=CARTESIAN_POINT('Ctrl Pts',(3.72630186199994,12.2,10.832587221));
#217919=CARTESIAN_POINT('Ctrl Pts',(3.72366435199994,12.2,10.829902884));
#217920=CARTESIAN_POINT('Ctrl Pts',(3.72103200699994,12.2,10.827219716));
#217921=CARTESIAN_POINT('Ctrl Pts',(3.71840482999994,12.2,10.824537725));
#217922=CARTESIAN_POINT('Ctrl Pts',(3.71578282099994,12.2,10.821856919));
#217923=CARTESIAN_POINT('Ctrl Pts',(3.71316598199994,12.2,10.819177306));
#217924=CARTESIAN_POINT('Ctrl Pts',(3.71055431199994,12.2,10.816498895));
#217925=CARTESIAN_POINT('Ctrl Pts',(3.70794781299994,12.2,10.813821695));
#217926=CARTESIAN_POINT('Ctrl Pts',(3.70534648499994,12.2,10.811145713));
#217927=CARTESIAN_POINT('Ctrl Pts',(3.70275033099994,12.2,10.808470961));
#217928=CARTESIAN_POINT('Ctrl Pts',(3.70015935099994,12.2,10.805797449));
#217929=CARTESIAN_POINT('Ctrl Pts',(3.69757354499994,12.2,10.803125184));
#217930=CARTESIAN_POINT('Ctrl Pts',(3.69499291499995,12.2,10.800454179));
#217931=CARTESIAN_POINT('Ctrl Pts',(3.69241746099994,12.2,10.797784438));
#217932=CARTESIAN_POINT('Ctrl Pts',(3.68984718499994,12.2,10.795115974));
#217933=CARTESIAN_POINT('Ctrl Pts',(3.68728208699994,12.2,10.792448794));
#217934=CARTESIAN_POINT('Ctrl Pts',(3.68472216799994,12.2,10.789782909));
#217935=CARTESIAN_POINT('Ctrl Pts',(3.68216742899994,12.2,10.787118327));
#217936=CARTESIAN_POINT('Ctrl Pts',(3.67961787099994,12.2,10.784455057));
#217937=CARTESIAN_POINT('Ctrl Pts',(3.67707349599994,12.2,10.781793108));
#217938=CARTESIAN_POINT('Ctrl Pts',(3.67453430199994,12.2,10.77913249));
#217939=CARTESIAN_POINT('Ctrl Pts',(3.67200029299994,12.2,10.776473211));
#217940=CARTESIAN_POINT('Ctrl Pts',(3.66947146699994,12.2,10.773815282));
#217941=CARTESIAN_POINT('Ctrl Pts',(3.66694782699994,12.2,10.771158713));
#217942=CARTESIAN_POINT('Ctrl Pts',(3.66442937399994,12.2,10.768503511));
#217943=CARTESIAN_POINT('Ctrl Pts',(3.66191610699994,12.2,10.765849687));
#217944=CARTESIAN_POINT('Ctrl Pts',(3.65940802899994,12.2,10.76319725));
#217945=CARTESIAN_POINT('Ctrl Pts',(3.65690513699994,12.2,10.760546208));
#217946=CARTESIAN_POINT('Ctrl Pts',(3.65440743699994,12.2,10.757896573));
#217947=CARTESIAN_POINT('Ctrl Pts',(3.65191492599994,12.2,10.755248353));
#217948=CARTESIAN_POINT('Ctrl Pts',(3.64942760599994,12.2,10.752601556));
#217949=CARTESIAN_POINT('Ctrl Pts',(3.64694547899994,12.2,10.749956194));
#217950=CARTESIAN_POINT('Ctrl Pts',(3.64446854399994,12.2,10.747312275));
#217951=CARTESIAN_POINT('Ctrl Pts',(3.64199680199994,12.2,10.744669808));
#217952=CARTESIAN_POINT('Ctrl Pts',(3.63953025499994,12.2,10.742028805));
#217953=CARTESIAN_POINT('Ctrl Pts',(3.63706890199994,12.2,10.739389272));
#217954=CARTESIAN_POINT('Ctrl Pts',(3.63461274499994,12.2,10.736751222));
#217955=CARTESIAN_POINT('Ctrl Pts',(3.63216178499994,12.2,10.734114662));
#217956=CARTESIAN_POINT('Ctrl Pts',(3.62971602199994,12.2,10.731479602));
#217957=CARTESIAN_POINT('Ctrl Pts',(3.62727545699994,12.2,10.728846054));
#217958=CARTESIAN_POINT('Ctrl Pts',(3.62484009099994,12.2,10.726214025));
#217959=CARTESIAN_POINT('Ctrl Pts',(3.62240992399994,12.2,10.723583524));
#217960=CARTESIAN_POINT('Ctrl Pts',(3.61998495799994,12.2,10.720954563));
#217961=CARTESIAN_POINT('Ctrl Pts',(3.61756519199994,12.2,10.718327151));
#217962=CARTESIAN_POINT('Ctrl Pts',(3.61515062899994,12.2,10.715701296));
#217963=CARTESIAN_POINT('Ctrl Pts',(3.61274126699994,12.2,10.71307701));
#217964=CARTESIAN_POINT('Ctrl Pts',(3.61033710899994,12.2,10.710454302));
#217965=CARTESIAN_POINT('Ctrl Pts',(3.60793815399994,12.2,10.707833181));
#217966=CARTESIAN_POINT('Ctrl Pts',(3.60554440399994,12.2,10.705213657));
#217967=CARTESIAN_POINT('Ctrl Pts',(3.60315585899994,12.2,10.702595741));
#217968=CARTESIAN_POINT('Ctrl Pts',(3.60077251999994,12.2,10.699979441));
#217969=CARTESIAN_POINT('Ctrl Pts',(3.59839438799994,12.2,10.697364767));
#217970=CARTESIAN_POINT('Ctrl Pts',(3.59602146199994,12.2,10.694751731));
#217971=CARTESIAN_POINT('Ctrl Pts',(3.59365374499994,12.2,10.692140339));
#217972=CARTESIAN_POINT('Ctrl Pts',(3.59129123599994,12.2,10.689530605));
#217973=CARTESIAN_POINT('Ctrl Pts',(3.58893393499994,12.2,10.686922536));
#217974=CARTESIAN_POINT('Ctrl Pts',(3.58658184499994,12.2,10.684316143));
#217975=CARTESIAN_POINT('Ctrl Pts',(3.58423496399995,12.2,10.681711437));
#217976=CARTESIAN_POINT('Ctrl Pts',(3.58189329599994,12.2,10.679108425));
#217977=CARTESIAN_POINT('Ctrl Pts',(3.57955683799994,12.2,10.67650712));
#217978=CARTESIAN_POINT('Ctrl Pts',(3.57722559299994,12.2,10.673907531));
#217979=CARTESIAN_POINT('Ctrl Pts',(3.57489956099994,12.2,10.671309666));
#217980=CARTESIAN_POINT('Ctrl Pts',(3.57257874199994,12.2,10.668713538));
#217981=CARTESIAN_POINT('Ctrl Pts',(3.57026313699994,12.2,10.666119155));
#217982=CARTESIAN_POINT('Ctrl Pts',(3.56795274699994,12.2,10.663526528));
#217983=CARTESIAN_POINT('Ctrl Pts',(3.56564757099994,12.2,10.660935667));
#217984=CARTESIAN_POINT('Ctrl Pts',(3.56334761099994,12.2,10.658346581));
#217985=CARTESIAN_POINT('Ctrl Pts',(3.56105286799994,12.2,10.655759282));
#217986=CARTESIAN_POINT('Ctrl Pts',(3.55876334099994,12.2,10.653173779));
#217987=CARTESIAN_POINT('Ctrl Pts',(3.55647903199994,12.2,10.650590083));
#217988=CARTESIAN_POINT('Ctrl Pts',(3.55419994099994,12.2,10.648008202));
#217989=CARTESIAN_POINT('Ctrl Pts',(3.55192606799994,12.2,10.645428149));
#217990=CARTESIAN_POINT('Ctrl Pts',(3.54965741499994,12.2,10.642849932));
#217991=CARTESIAN_POINT('Ctrl Pts',(3.54739397999994,12.2,10.640273563));
#217992=CARTESIAN_POINT('Ctrl Pts',(3.54513576499994,12.2,10.637699051));
#217993=CARTESIAN_POINT('Ctrl Pts',(3.54288277099994,12.2,10.635126406));
#217994=CARTESIAN_POINT('Ctrl Pts',(3.54063499799994,12.2,10.632555639));
#217995=CARTESIAN_POINT('Ctrl Pts',(3.53839244699994,12.2,10.62998676));
#217996=CARTESIAN_POINT('Ctrl Pts',(3.53615511699994,12.2,10.62741978));
#217997=CARTESIAN_POINT('Ctrl Pts',(3.53392300999994,12.2,10.624854709));
#217998=CARTESIAN_POINT('Ctrl Pts',(3.53169612599994,12.2,10.622291557));
#217999=CARTESIAN_POINT('Ctrl Pts',(3.52947446499994,12.2,10.619730334));
#218000=CARTESIAN_POINT('Ctrl Pts',(3.52725802799994,12.2,10.617171051));
#218001=CARTESIAN_POINT('Ctrl Pts',(3.52504681399994,12.2,10.61461372));
#218002=CARTESIAN_POINT('Ctrl Pts',(3.52284082599994,12.2,10.612058349));
#218003=CARTESIAN_POINT('Ctrl Pts',(3.52064006199994,12.2,10.609504948));
#218004=CARTESIAN_POINT('Ctrl Pts',(3.51844452399994,12.2,10.606953531));
#218005=CARTESIAN_POINT('Ctrl Pts',(3.51625421199994,12.2,10.604404106));
#218006=CARTESIAN_POINT('Ctrl Pts',(3.51406912699994,12.2,10.601856683));
#218007=CARTESIAN_POINT('Ctrl Pts',(3.51188926799994,12.2,10.599311274));
#218008=CARTESIAN_POINT('Ctrl Pts',(3.50971463599994,12.2,10.596767889));
#218009=CARTESIAN_POINT('Ctrl Pts',(3.50754523199994,12.2,10.594226538));
#218010=CARTESIAN_POINT('Ctrl Pts',(3.50538105499994,12.2,10.591687233));
#218011=CARTESIAN_POINT('Ctrl Pts',(3.50322210699994,12.2,10.589149983));
#218012=CARTESIAN_POINT('Ctrl Pts',(3.50106838699995,12.2,10.5866148));
#218013=CARTESIAN_POINT('Ctrl Pts',(3.49891989599994,12.2,10.584081694));
#218014=CARTESIAN_POINT('Ctrl Pts',(3.49677663399994,12.2,10.581550676));
#218015=CARTESIAN_POINT('Ctrl Pts',(3.49463860199994,12.2,10.579021758));
#218016=CARTESIAN_POINT('Ctrl Pts',(3.49250580099994,12.2,10.576494948));
#218017=CARTESIAN_POINT('Ctrl Pts',(3.49037822899994,12.2,10.573970259));
#218018=CARTESIAN_POINT('Ctrl Pts',(3.48825588699994,12.2,10.571447699));
#218019=CARTESIAN_POINT('Ctrl Pts',(3.48613877699994,12.2,10.568927282));
#218020=CARTESIAN_POINT('Ctrl Pts',(3.48402689799994,12.2,10.566409018));
#218021=CARTESIAN_POINT('Ctrl Pts',(3.48192024899994,12.2,10.563892917));
#218022=CARTESIAN_POINT('Ctrl Pts',(3.47981883399994,12.2,10.561378991));
#218023=CARTESIAN_POINT('Ctrl Pts',(3.47772264999994,12.2,10.558867249));
#218024=CARTESIAN_POINT('Ctrl Pts',(3.47563169699994,12.2,10.556357703));
#218025=CARTESIAN_POINT('Ctrl Pts',(3.47354597799994,12.2,10.553850365));
#218026=CARTESIAN_POINT('Ctrl Pts',(3.47146549099994,12.2,10.551345244));
#218027=CARTESIAN_POINT('Ctrl Pts',(3.46939023699994,12.2,10.548842353));
#218028=CARTESIAN_POINT('Ctrl Pts',(3.46732021699995,12.2,10.546341702));
#218029=CARTESIAN_POINT('Ctrl Pts',(3.46525542999994,12.2,10.543843302));
#218030=CARTESIAN_POINT('Ctrl Pts',(3.46319587599994,12.2,10.541347163));
#218031=CARTESIAN_POINT('Ctrl Pts',(3.46114155699994,12.2,10.538853298));
#218032=CARTESIAN_POINT('Ctrl Pts',(3.45909247099994,12.2,10.536361718));
#218033=CARTESIAN_POINT('Ctrl Pts',(3.45704861999995,12.2,10.533872432));
#218034=CARTESIAN_POINT('Ctrl Pts',(3.45501000299994,12.2,10.531385453));
#218035=CARTESIAN_POINT('Ctrl Pts',(3.45297662099994,12.2,10.528900792));
#218036=CARTESIAN_POINT('Ctrl Pts',(3.45094847299994,12.2,10.526418461));
#218037=CARTESIAN_POINT('Ctrl Pts',(3.44892555999994,12.2,10.523938468));
#218038=CARTESIAN_POINT('Ctrl Pts',(3.44690788299994,12.2,10.521460827));
#218039=CARTESIAN_POINT('Ctrl Pts',(3.44489543999994,12.2,10.51898555));
#218040=CARTESIAN_POINT('Ctrl Pts',(3.44288823299994,12.2,10.516512645));
#218041=CARTESIAN_POINT('Ctrl Pts',(3.44088626199994,12.2,10.514042126));
#218042=CARTESIAN_POINT('Ctrl Pts',(3.43888952499994,12.2,10.511574004));
#218043=CARTESIAN_POINT('Ctrl Pts',(3.43689802499994,12.2,10.50910829));
#218044=CARTESIAN_POINT('Ctrl Pts',(3.43491175999994,12.2,10.506644995));
#218045=CARTESIAN_POINT('Ctrl Pts',(3.43293072999994,12.2,10.504184131));
#218046=CARTESIAN_POINT('Ctrl Pts',(3.43095493699995,12.2,10.501725709));
#218047=CARTESIAN_POINT('Ctrl Pts',(3.42898437999994,12.2,10.49926974));
#218048=CARTESIAN_POINT('Ctrl Pts',(3.42701905899994,12.2,10.496816237));
#218049=CARTESIAN_POINT('Ctrl Pts',(3.42505897399994,12.2,10.49436521));
#218050=CARTESIAN_POINT('Ctrl Pts',(3.42310412599995,12.2,10.491916672));
#218051=CARTESIAN_POINT('Ctrl Pts',(3.42115451199994,12.2,10.489470632));
#218052=CARTESIAN_POINT('Ctrl Pts',(3.41921013599995,12.2,10.487027105));
#218053=CARTESIAN_POINT('Ctrl Pts',(3.41727099499994,12.2,10.4845861));
#218054=CARTESIAN_POINT('Ctrl Pts',(3.41533709199994,12.2,10.482147629));
#218055=CARTESIAN_POINT('Ctrl Pts',(3.41340842399994,12.2,10.479711706));
#218056=CARTESIAN_POINT('Ctrl Pts',(3.41148499199994,12.2,10.477278339));
#218057=CARTESIAN_POINT('Ctrl Pts',(3.40956679599994,12.2,10.474847543));
#218058=CARTESIAN_POINT('Ctrl Pts',(3.40765383599994,12.2,10.472419326));
#218059=CARTESIAN_POINT('Ctrl Pts',(3.40574611299994,12.2,10.469993704));
#218060=CARTESIAN_POINT('Ctrl Pts',(3.40384362599994,12.2,10.467570687));
#218061=CARTESIAN_POINT('Ctrl Pts',(3.40194637399994,12.2,10.465150286));
#218062=CARTESIAN_POINT('Ctrl Pts',(3.40005435899994,12.2,10.462732513));
#218063=CARTESIAN_POINT('Ctrl Pts',(3.39816757899994,12.2,10.460317381));
#218064=CARTESIAN_POINT('Ctrl Pts',(3.39628603499994,12.2,10.4579049));
#218065=CARTESIAN_POINT('Ctrl Pts',(3.39440972599995,12.2,10.455495084));
#218066=CARTESIAN_POINT('Ctrl Pts',(3.39253865299994,12.2,10.453087944));
#218067=CARTESIAN_POINT('Ctrl Pts',(3.39067281599994,12.2,10.450683492));
#218068=CARTESIAN_POINT('Ctrl Pts',(3.38881221399994,12.2,10.448281741));
#218069=CARTESIAN_POINT('Ctrl Pts',(3.38695684699994,12.2,10.445882701));
#218070=CARTESIAN_POINT('Ctrl Pts',(3.38510671499994,12.2,10.443486385));
#218071=CARTESIAN_POINT('Ctrl Pts',(3.38326181899995,12.2,10.441092806));
#218072=CARTESIAN_POINT('Ctrl Pts',(3.38142215599994,12.2,10.438701973));
#218073=CARTESIAN_POINT('Ctrl Pts',(3.37958772799994,12.2,10.436313903));
#218074=CARTESIAN_POINT('Ctrl Pts',(3.37775853499994,12.2,10.433928604));
#218075=CARTESIAN_POINT('Ctrl Pts',(3.37593457599994,12.2,10.43154609));
#218076=CARTESIAN_POINT('Ctrl Pts',(3.37411584999994,12.2,10.429166374));
#218077=CARTESIAN_POINT('Ctrl Pts',(3.37230235899994,12.2,10.426789465));
#218078=CARTESIAN_POINT('Ctrl Pts',(3.37049410099994,12.2,10.424415378));
#218079=CARTESIAN_POINT('Ctrl Pts',(3.36869107699994,12.2,10.422044126));
#218080=CARTESIAN_POINT('Ctrl Pts',(3.36689328399994,12.2,10.419675719));
#218081=CARTESIAN_POINT('Ctrl Pts',(3.36510072599994,12.2,10.417310171));
#218082=CARTESIAN_POINT('Ctrl Pts',(3.36331339899994,12.2,10.414947493));
#218083=CARTESIAN_POINT('Ctrl Pts',(3.36153130499994,12.2,10.412587698));
#218084=CARTESIAN_POINT('Ctrl Pts',(3.35975444299994,12.2,10.410230799));
#218085=CARTESIAN_POINT('Ctrl Pts',(3.35798281299994,12.2,10.407876808));
#218086=CARTESIAN_POINT('Ctrl Pts',(3.35621641399994,12.2,10.405525737));
#218087=CARTESIAN_POINT('Ctrl Pts',(3.35445524599994,12.2,10.4031776));
#218088=CARTESIAN_POINT('Ctrl Pts',(3.35269930899994,12.2,10.400832408));
#218089=CARTESIAN_POINT('Ctrl Pts',(3.35094860199994,12.2,10.398490174));
#218090=CARTESIAN_POINT('Ctrl Pts',(3.34920312499994,12.2,10.396150911));
#218091=CARTESIAN_POINT('Ctrl Pts',(3.34746287999995,12.2,10.393814631));
#218092=CARTESIAN_POINT('Ctrl Pts',(3.34572786099995,12.2,10.391481347));
#218093=CARTESIAN_POINT('Ctrl Pts',(3.34399807299994,12.2,10.389151072));
#218094=CARTESIAN_POINT('Ctrl Pts',(3.34227351299994,12.2,10.386823818));
#218095=CARTESIAN_POINT('Ctrl Pts',(3.34055418199994,12.2,10.384499599));
#218096=CARTESIAN_POINT('Ctrl Pts',(3.33884007799994,12.2,10.382178427));
#218097=CARTESIAN_POINT('Ctrl Pts',(3.33713120199994,12.2,10.379860313));
#218098=CARTESIAN_POINT('Ctrl Pts',(3.33542755199994,12.2,10.377545274));
#218099=CARTESIAN_POINT('Ctrl Pts',(3.33372912899994,12.2,10.375233319));
#218100=CARTESIAN_POINT('Ctrl Pts',(3.33203593199995,12.2,10.372924463));
#218101=CARTESIAN_POINT('Ctrl Pts',(3.33034796099994,12.2,10.370618718));
#218102=CARTESIAN_POINT('Ctrl Pts',(3.32866521499994,12.2,10.368316097));
#218103=CARTESIAN_POINT('Ctrl Pts',(3.32698769299994,12.2,10.366016614));
#218104=CARTESIAN_POINT('Ctrl Pts',(3.32531539599994,12.2,10.36372028));
#218105=CARTESIAN_POINT('Ctrl Pts',(3.32364832199994,12.2,10.36142711));
#218106=CARTESIAN_POINT('Ctrl Pts',(3.32198647199994,12.2,10.359137117));
#218107=CARTESIAN_POINT('Ctrl Pts',(3.32032984499994,12.2,10.356850313));
#218108=CARTESIAN_POINT('Ctrl Pts',(3.31867843899994,12.2,10.354566712));
#218109=CARTESIAN_POINT('Ctrl Pts',(3.31703225499994,12.2,10.352286327));
#218110=CARTESIAN_POINT('Ctrl Pts',(3.31506309947149,12.2,10.3495537386993));
#218111=CARTESIAN_POINT('Ctrl Pts',(3.31310177376417,12.2,10.3468260146503));
#218112=CARTESIAN_POINT('Ctrl Pts',(3.31114827823572,12.2,10.3441031813496));
#218113=CARTESIAN_POINT('Ctrl Pts',(3.30920261270513,12.2,10.3413852645476));
#218114=CARTESIAN_POINT('Ctrl Pts',(3.30726477099994,12.2,10.33867229));
#218115=CARTESIAN_POINT('Ctrl Pts',(3.30565512199994,12.2,10.336414786));
#218116=CARTESIAN_POINT('Ctrl Pts',(3.30405068899994,12.2,10.334160606));
#218117=CARTESIAN_POINT('Ctrl Pts',(3.30245147199994,12.2,10.331909762));
#218118=CARTESIAN_POINT('Ctrl Pts',(3.30085747199994,12.2,10.329662268));
#218119=CARTESIAN_POINT('Ctrl Pts',(3.29926868599994,12.2,10.327418135));
#218120=CARTESIAN_POINT('Ctrl Pts',(3.29768511299994,12.2,10.325177379));
#218121=CARTESIAN_POINT('Ctrl Pts',(3.29610675499994,12.2,10.322940014));
#218122=CARTESIAN_POINT('Ctrl Pts',(3.29453360899994,12.2,10.320706052));
#218123=CARTESIAN_POINT('Ctrl Pts',(3.29296567499994,12.2,10.318475509));
#218124=CARTESIAN_POINT('Ctrl Pts',(3.29140295199994,12.2,10.316248395));
#218125=CARTESIAN_POINT('Ctrl Pts',(3.28984543999994,12.2,10.314024727));
#218126=CARTESIAN_POINT('Ctrl Pts',(3.28829313699994,12.2,10.311804518));
#218127=CARTESIAN_POINT('Ctrl Pts',(3.28674604399994,12.2,10.30958778));
#218128=CARTESIAN_POINT('Ctrl Pts',(3.28520415899995,12.2,10.307374529));
#218129=CARTESIAN_POINT('Ctrl Pts',(3.28366748099994,12.2,10.305164779));
#218130=CARTESIAN_POINT('Ctrl Pts',(3.28213600999995,12.2,10.302958542));
#218131=CARTESIAN_POINT('Ctrl Pts',(3.28060974399994,12.2,10.300755834));
#218132=CARTESIAN_POINT('Ctrl Pts',(3.27908868399994,12.2,10.298556666));
#218133=CARTESIAN_POINT('Ctrl Pts',(3.27757282699995,12.2,10.296361056));
#218134=CARTESIAN_POINT('Ctrl Pts',(3.27606217499994,12.2,10.294169016));
#218135=CARTESIAN_POINT('Ctrl Pts',(3.27455672399994,12.2,10.291980559));
#218136=CARTESIAN_POINT('Ctrl Pts',(3.27305647499994,12.2,10.2897957));
#218137=CARTESIAN_POINT('Ctrl Pts',(3.27156142599994,12.2,10.287614454));
#218138=CARTESIAN_POINT('Ctrl Pts',(3.27007157799994,12.2,10.285436836));
#218139=CARTESIAN_POINT('Ctrl Pts',(3.26858692799994,12.2,10.283262858));
#218140=CARTESIAN_POINT('Ctrl Pts',(3.26710747499994,12.2,10.281092534));
#218141=CARTESIAN_POINT('Ctrl Pts',(3.26563321999994,12.2,10.27892588));
#218142=CARTESIAN_POINT('Ctrl Pts',(3.26416416099994,12.2,10.276762911));
#218143=CARTESIAN_POINT('Ctrl Pts',(3.26270029699995,12.2,10.274603639));
#218144=CARTESIAN_POINT('Ctrl Pts',(3.26124162699994,12.2,10.272448079));
#218145=CARTESIAN_POINT('Ctrl Pts',(3.25978815099994,12.2,10.270296246));
#218146=CARTESIAN_POINT('Ctrl Pts',(3.25833986599994,12.2,10.268148156));
#218147=CARTESIAN_POINT('Ctrl Pts',(3.25689677199994,12.2,10.266003821));
#218148=CARTESIAN_POINT('Ctrl Pts',(3.25545886799994,12.2,10.263863257));
#218149=CARTESIAN_POINT('Ctrl Pts',(3.25402615299994,12.2,10.261726478));
#218150=CARTESIAN_POINT('Ctrl Pts',(3.25259862599995,12.2,10.259593498));
#218151=CARTESIAN_POINT('Ctrl Pts',(3.25117628599994,12.2,10.257464334));
#218152=CARTESIAN_POINT('Ctrl Pts',(3.24975913199995,12.2,10.255338999));
#218153=CARTESIAN_POINT('Ctrl Pts',(3.24834716199994,12.2,10.253217507));
#218154=CARTESIAN_POINT('Ctrl Pts',(3.24694037599994,12.2,10.251099875));
#218155=CARTESIAN_POINT('Ctrl Pts',(3.24553877199994,12.2,10.248986116));
#218156=CARTESIAN_POINT('Ctrl Pts',(3.24414234999994,12.2,10.246876245));
#218157=CARTESIAN_POINT('Ctrl Pts',(3.24275110699995,12.2,10.244770278));
#218158=CARTESIAN_POINT('Ctrl Pts',(3.24136504399994,12.2,10.242668229));
#218159=CARTESIAN_POINT('Ctrl Pts',(3.23998415799994,12.2,10.240570115));
#218160=CARTESIAN_POINT('Ctrl Pts',(3.23860844899994,12.2,10.238475948));
#218161=CARTESIAN_POINT('Ctrl Pts',(3.23723791499994,12.2,10.236385745));
#218162=CARTESIAN_POINT('Ctrl Pts',(3.23587255499994,12.2,10.23429952));
#218163=CARTESIAN_POINT('Ctrl Pts',(3.23451236799994,12.2,10.232217288));
#218164=CARTESIAN_POINT('Ctrl Pts',(3.23315735299994,12.2,10.230139067));
#218165=CARTESIAN_POINT('Ctrl Pts',(3.23180750799994,12.2,10.228064869));
#218166=CARTESIAN_POINT('Ctrl Pts',(3.23046283199994,12.2,10.225994711));
#218167=CARTESIAN_POINT('Ctrl Pts',(3.22912332499994,12.2,10.223928608));
#218168=CARTESIAN_POINT('Ctrl Pts',(3.22778898299994,12.2,10.221866575));
#218169=CARTESIAN_POINT('Ctrl Pts',(3.22645980699994,12.2,10.219808628));
#218170=CARTESIAN_POINT('Ctrl Pts',(3.22513579399994,12.2,10.217754781));
#218171=CARTESIAN_POINT('Ctrl Pts',(3.22381694499994,12.2,10.215705052));
#218172=CARTESIAN_POINT('Ctrl Pts',(3.22250325599994,12.2,10.213659454));
#218173=CARTESIAN_POINT('Ctrl Pts',(3.22119472699995,12.2,10.211618004));
#218174=CARTESIAN_POINT('Ctrl Pts',(3.21989135599994,12.2,10.209580717));
#218175=CARTESIAN_POINT('Ctrl Pts',(3.21859314299994,12.2,10.20754761));
#218176=CARTESIAN_POINT('Ctrl Pts',(3.21730008399994,12.2,10.205518696));
#218177=CARTESIAN_POINT('Ctrl Pts',(3.21601217999994,12.2,10.203493994));
#218178=CARTESIAN_POINT('Ctrl Pts',(3.21472942799994,12.2,10.201473517));
#218179=CARTESIAN_POINT('Ctrl Pts',(3.21345182799994,12.2,10.199457283));
#218180=CARTESIAN_POINT('Ctrl Pts',(3.21217937699994,12.2,10.197445307));
#218181=CARTESIAN_POINT('Ctrl Pts',(3.21091207399995,12.2,10.195437604));
#218182=CARTESIAN_POINT('Ctrl Pts',(3.20964991799995,12.2,10.193434192));
#218183=CARTESIAN_POINT('Ctrl Pts',(3.20839290699994,12.2,10.191435086));
#218184=CARTESIAN_POINT('Ctrl Pts',(3.20714103999994,12.2,10.189440301));
#218185=CARTESIAN_POINT('Ctrl Pts',(3.20589431499994,12.2,10.187449854));
#218186=CARTESIAN_POINT('Ctrl Pts',(3.20465272999995,12.2,10.185463762));
#218187=CARTESIAN_POINT('Ctrl Pts',(3.20341628299994,12.2,10.183482041));
#218188=CARTESIAN_POINT('Ctrl Pts',(3.20218497399994,12.2,10.181504705));
#218189=CARTESIAN_POINT('Ctrl Pts',(3.20095880099994,12.2,10.179531773));
#218190=CARTESIAN_POINT('Ctrl Pts',(3.19973776199994,12.2,10.17756326));
#218191=CARTESIAN_POINT('Ctrl Pts',(3.19852185399994,12.2,10.175599184));
#218192=CARTESIAN_POINT('Ctrl Pts',(3.19731107699994,12.2,10.173639559));
#218193=CARTESIAN_POINT('Ctrl Pts',(3.19610542999994,12.2,10.171684403));
#218194=CARTESIAN_POINT('Ctrl Pts',(3.19490490899994,12.2,10.169733732));
#218195=CARTESIAN_POINT('Ctrl Pts',(3.19370951399994,12.2,10.167787564));
#218196=CARTESIAN_POINT('Ctrl Pts',(3.19251924199994,12.2,10.165845913));
#218197=CARTESIAN_POINT('Ctrl Pts',(3.19133409399994,12.2,10.163908798));
#218198=CARTESIAN_POINT('Ctrl Pts',(3.19015406399994,12.2,10.161976234));
#218199=CARTESIAN_POINT('Ctrl Pts',(3.18897915299994,12.2,10.160048239));
#218200=CARTESIAN_POINT('Ctrl Pts',(3.18780935899994,12.2,10.158124831));
#218201=CARTESIAN_POINT('Ctrl Pts',(3.18664467899994,12.2,10.156206023));
#218202=CARTESIAN_POINT('Ctrl Pts',(3.18548511399994,12.2,10.154291836));
#218203=CARTESIAN_POINT('Ctrl Pts',(3.18433065699995,12.2,10.152382285));
#218204=CARTESIAN_POINT('Ctrl Pts',(3.18318131199995,12.2,10.150477387));
#218205=CARTESIAN_POINT('Ctrl Pts',(3.18203707299994,12.2,10.148577159));
#218206=CARTESIAN_POINT('Ctrl Pts',(3.18089793999994,12.2,10.146681619));
#218207=CARTESIAN_POINT('Ctrl Pts',(3.17976390999994,12.2,10.144790784));
#218208=CARTESIAN_POINT('Ctrl Pts',(3.17863498099995,12.2,10.142904671));
#218209=CARTESIAN_POINT('Ctrl Pts',(3.17751115299994,12.2,10.141023297));
#218210=CARTESIAN_POINT('Ctrl Pts',(3.17639242199995,12.2,10.13914668));
#218211=CARTESIAN_POINT('Ctrl Pts',(3.17527878599994,12.2,10.137274836));
#218212=CARTESIAN_POINT('Ctrl Pts',(3.17417024399994,12.2,10.135407784));
#218213=CARTESIAN_POINT('Ctrl Pts',(3.17306679399994,12.2,10.133545542));
#218214=CARTESIAN_POINT('Ctrl Pts',(3.17196843199994,12.2,10.131688125));
#218215=CARTESIAN_POINT('Ctrl Pts',(3.17087515899994,12.2,10.129835553));
#218216=CARTESIAN_POINT('Ctrl Pts',(3.16978697099994,12.2,10.127987842));
#218217=CARTESIAN_POINT('Ctrl Pts',(3.16870386699994,12.2,10.126145011));
#218218=CARTESIAN_POINT('Ctrl Pts',(3.16762584299994,12.2,10.124307078));
#218219=CARTESIAN_POINT('Ctrl Pts',(3.16655289799994,12.2,10.12247406));
#218220=CARTESIAN_POINT('Ctrl Pts',(3.16548502999995,12.2,10.120645975));
#218221=CARTESIAN_POINT('Ctrl Pts',(3.16442223699994,12.2,10.11882284));
#218222=CARTESIAN_POINT('Ctrl Pts',(3.16336451599994,12.2,10.117004675));
#218223=CARTESIAN_POINT('Ctrl Pts',(3.16231186499994,12.2,10.115191496));
#218224=CARTESIAN_POINT('Ctrl Pts',(3.16126428299994,12.2,10.113383323));
#218225=CARTESIAN_POINT('Ctrl Pts',(3.16022176599994,12.2,10.111580173));
#218226=CARTESIAN_POINT('Ctrl Pts',(3.15918431399994,12.2,10.109782065));
#218227=CARTESIAN_POINT('Ctrl Pts',(3.15815192199994,12.2,10.107989016));
#218228=CARTESIAN_POINT('Ctrl Pts',(3.15712458699994,12.2,10.106201046));
#218229=CARTESIAN_POINT('Ctrl Pts',(3.15610231199994,12.2,10.104418172));
#218230=CARTESIAN_POINT('Ctrl Pts',(3.15508508899994,12.2,10.102640413));
#218231=CARTESIAN_POINT('Ctrl Pts',(3.15407291799994,12.2,10.100867788));
#218232=CARTESIAN_POINT('Ctrl Pts',(3.15306579799994,12.2,10.099100315));
#218233=CARTESIAN_POINT('Ctrl Pts',(3.15206372299994,12.2,10.097338013));
#218234=CARTESIAN_POINT('Ctrl Pts',(3.15106669299994,12.2,10.0955809));
#218235=CARTESIAN_POINT('Ctrl Pts',(3.15007470599994,12.2,10.093828996));
#218236=CARTESIAN_POINT('Ctrl Pts',(3.14908775899994,12.2,10.092082318));
#218237=CARTESIAN_POINT('Ctrl Pts',(3.14810584799994,12.2,10.090340886));
#218238=CARTESIAN_POINT('Ctrl Pts',(3.14712897199994,12.2,10.08860472));
#218239=CARTESIAN_POINT('Ctrl Pts',(3.14615712899994,12.2,10.086873837));
#218240=CARTESIAN_POINT('Ctrl Pts',(3.14519031499994,12.2,10.085148257));
#218241=CARTESIAN_POINT('Ctrl Pts',(3.14422852799995,12.2,10.083427999));
#218242=CARTESIAN_POINT('Ctrl Pts',(3.14327176599994,12.2,10.081713083));
#218243=CARTESIAN_POINT('Ctrl Pts',(3.14232002399994,12.2,10.080003527));
#218244=CARTESIAN_POINT('Ctrl Pts',(3.14137330399994,12.2,10.078299351));
#218245=CARTESIAN_POINT('Ctrl Pts',(3.14043159899994,12.2,10.076600574));
#218246=CARTESIAN_POINT('Ctrl Pts',(3.13949490699994,12.2,10.074907216));
#218247=CARTESIAN_POINT('Ctrl Pts',(3.13856322699994,12.2,10.073219296));
#218248=CARTESIAN_POINT('Ctrl Pts',(3.13763655599994,12.2,10.071536834));
#218249=CARTESIAN_POINT('Ctrl Pts',(3.13671488999994,12.2,10.069859849));
#218250=CARTESIAN_POINT('Ctrl Pts',(3.13579822699994,12.2,10.068188362));
#218251=CARTESIAN_POINT('Ctrl Pts',(3.13488656499994,12.2,10.066522392));
#218252=CARTESIAN_POINT('Ctrl Pts',(3.13397989999994,12.2,10.064861958));
#218253=CARTESIAN_POINT('Ctrl Pts',(3.13307822999994,12.2,10.063207081));
#218254=CARTESIAN_POINT('Ctrl Pts',(3.13218154999995,12.2,10.061557781));
#218255=CARTESIAN_POINT('Ctrl Pts',(3.13128985999994,12.2,10.059914077));
#218256=CARTESIAN_POINT('Ctrl Pts',(3.13040315599994,12.2,10.058275991));
#218257=CARTESIAN_POINT('Ctrl Pts',(3.12952143499994,12.2,10.056643542));
#218258=CARTESIAN_POINT('Ctrl Pts',(3.12864469399994,12.2,10.05501675));
#218259=CARTESIAN_POINT('Ctrl Pts',(3.12777292999994,12.2,10.053395635));
#218260=CARTESIAN_POINT('Ctrl Pts',(3.12690613999994,12.2,10.051780219));
#218261=CARTESIAN_POINT('Ctrl Pts',(3.12604432099994,12.2,10.050170521));
#218262=CARTESIAN_POINT('Ctrl Pts',(3.12518747099995,12.2,10.048566563));
#218263=CARTESIAN_POINT('Ctrl Pts',(3.12433558499994,12.2,10.046968364));
#218264=CARTESIAN_POINT('Ctrl Pts',(3.12348866099994,12.2,10.045375946));
#218265=CARTESIAN_POINT('Ctrl Pts',(3.12264669699994,12.2,10.043789328));
#218266=CARTESIAN_POINT('Ctrl Pts',(3.12180968799994,12.2,10.042208533));
#218267=CARTESIAN_POINT('Ctrl Pts',(3.12097763099994,12.2,10.040633581));
#218268=CARTESIAN_POINT('Ctrl Pts',(3.12015052399994,12.2,10.039064492));
#218269=CARTESIAN_POINT('Ctrl Pts',(3.11932836299994,12.2,10.037501289));
#218270=CARTESIAN_POINT('Ctrl Pts',(3.11851114499994,12.2,10.035943991));
#218271=CARTESIAN_POINT('Ctrl Pts',(3.11769886699994,12.2,10.034392622));
#218272=CARTESIAN_POINT('Ctrl Pts',(3.11689152499994,12.2,10.0328472));
#218273=CARTESIAN_POINT('Ctrl Pts',(3.11608911699994,12.2,10.031307748));
#218274=CARTESIAN_POINT('Ctrl Pts',(3.11529163799994,12.2,10.029774289));
#218275=CARTESIAN_POINT('Ctrl Pts',(3.11449908499994,12.2,10.028246841));
#218276=CARTESIAN_POINT('Ctrl Pts',(3.11371145699994,12.2,10.026725429));
#218277=CARTESIAN_POINT('Ctrl Pts',(3.11292874799994,12.2,10.025210072));
#218278=CARTESIAN_POINT('Ctrl Pts',(3.11215095499994,12.2,10.023700794));
#218279=CARTESIAN_POINT('Ctrl Pts',(3.11137807399994,12.2,10.022197616));
#218280=CARTESIAN_POINT('Ctrl Pts',(3.11061010399994,12.2,10.020700559));
#218281=CARTESIAN_POINT('Ctrl Pts',(3.10984703899994,12.2,10.019209646));
#218282=CARTESIAN_POINT('Ctrl Pts',(3.10908887599994,12.2,10.017724899));
#218283=CARTESIAN_POINT('Ctrl Pts',(3.10833561299994,12.2,10.01624634));
#218284=CARTESIAN_POINT('Ctrl Pts',(3.10758724499994,12.2,10.01477399));
#218285=CARTESIAN_POINT('Ctrl Pts',(3.10684376799994,12.2,10.013307874));
#218286=CARTESIAN_POINT('Ctrl Pts',(3.10610517999995,12.2,10.011848013));
#218287=CARTESIAN_POINT('Ctrl Pts',(3.10537147499995,12.2,10.010394428));
#218288=CARTESIAN_POINT('Ctrl Pts',(3.10464265199994,12.2,10.008947144));
#218289=CARTESIAN_POINT('Ctrl Pts',(3.10391870499994,12.2,10.007506183));
#218290=CARTESIAN_POINT('Ctrl Pts',(3.10319963199994,12.2,10.006071567));
#218291=CARTESIAN_POINT('Ctrl Pts',(3.10248542799994,12.2,10.00464332));
#218292=CARTESIAN_POINT('Ctrl Pts',(3.10177608999994,12.2,10.003221464));
#218293=CARTESIAN_POINT('Ctrl Pts',(3.10107161399995,12.2,10.001806022));
#218294=CARTESIAN_POINT('Ctrl Pts',(3.10037199499994,12.2,10.000397017));
#218295=CARTESIAN_POINT('Ctrl Pts',(3.09967723099994,12.2,9.99899447299999));
#218296=CARTESIAN_POINT('Ctrl Pts',(3.09898731599994,12.2,9.99759841199998));
#218297=CARTESIAN_POINT('Ctrl Pts',(3.09830224899994,12.2,9.99620885899999));
#218298=CARTESIAN_POINT('Ctrl Pts',(3.09762202399994,12.2,9.99482583699999));
#218299=CARTESIAN_POINT('Ctrl Pts',(3.09694663699994,12.2,9.99344936799999));
#218300=CARTESIAN_POINT('Ctrl Pts',(3.09627608499994,12.2,9.99207947799999));
#218301=CARTESIAN_POINT('Ctrl Pts',(3.09561036199994,12.2,9.99071618899999));
#218302=CARTESIAN_POINT('Ctrl Pts',(3.09494946499994,12.2,9.98935952599999));
#218303=CARTESIAN_POINT('Ctrl Pts',(3.09429339099994,12.2,9.98800951199998));
#218304=CARTESIAN_POINT('Ctrl Pts',(3.09364213499994,12.2,9.98666617199999));
#218305=CARTESIAN_POINT('Ctrl Pts',(3.09299569299994,12.2,9.98532952799999));
#218306=CARTESIAN_POINT('Ctrl Pts',(3.09235405999994,12.2,9.98399960799999));
#218307=CARTESIAN_POINT('Ctrl Pts',(3.09171723299994,12.2,9.98267643199998));
#218308=CARTESIAN_POINT('Ctrl Pts',(3.09108520699994,12.2,9.98136002699999));
#218309=CARTESIAN_POINT('Ctrl Pts',(3.09045797699994,12.2,9.98005041799999));
#218310=CARTESIAN_POINT('Ctrl Pts',(3.08983553999994,12.2,9.97874762799999));
#218311=CARTESIAN_POINT('Ctrl Pts',(3.08921789099994,12.2,9.97745168099998));
#218312=CARTESIAN_POINT('Ctrl Pts',(3.08860502499994,12.2,9.97616260499999));
#218313=CARTESIAN_POINT('Ctrl Pts',(3.08799693999994,12.2,9.97488042299998));
#218314=CARTESIAN_POINT('Ctrl Pts',(3.08739362899995,12.2,9.97360515799999));
#218315=CARTESIAN_POINT('Ctrl Pts',(3.08679508799994,12.2,9.97233683899999));
#218316=CARTESIAN_POINT('Ctrl Pts',(3.08620131299994,12.2,9.97107548899999));
#218317=CARTESIAN_POINT('Ctrl Pts',(3.08561229999994,12.2,9.96982113299998));
#218318=CARTESIAN_POINT('Ctrl Pts',(3.08502804299994,12.2,9.96857379799999));
#218319=CARTESIAN_POINT('Ctrl Pts',(3.08444853899994,12.2,9.96733350799998));
#218320=CARTESIAN_POINT('Ctrl Pts',(3.08387378199994,12.2,9.96610028999999));
#218321=CARTESIAN_POINT('Ctrl Pts',(3.08330376799994,12.2,9.96487416799998));
#218322=CARTESIAN_POINT('Ctrl Pts',(3.08273849199994,12.2,9.96365516999998));
#218323=CARTESIAN_POINT('Ctrl Pts',(3.08217794999994,12.2,9.96244332099998));
#218324=CARTESIAN_POINT('Ctrl Pts',(3.08162213499994,12.2,9.96123864599999));
#218325=CARTESIAN_POINT('Ctrl Pts',(3.08107104499994,12.2,9.96004117299999));
#218326=CARTESIAN_POINT('Ctrl Pts',(3.08052467399994,12.2,9.95885092599998));
#218327=CARTESIAN_POINT('Ctrl Pts',(3.07998301799994,12.2,9.95766793499998));
#218328=CARTESIAN_POINT('Ctrl Pts',(3.07944606999994,12.2,9.95649222299999));
#218329=CARTESIAN_POINT('Ctrl Pts',(3.07891382499994,12.2,9.95532381799999));
#218330=CARTESIAN_POINT('Ctrl Pts',(3.07838628099995,12.2,9.95416274699998));
#218331=CARTESIAN_POINT('Ctrl Pts',(3.07786343199994,12.2,9.95300903699999));
#218332=CARTESIAN_POINT('Ctrl Pts',(3.07734526999994,12.2,9.95186271399999));
#218333=CARTESIAN_POINT('Ctrl Pts',(3.07683179299994,12.2,9.95072380599998));
#218334=CARTESIAN_POINT('Ctrl Pts',(3.07632299499994,12.2,9.94959233999998));
#218335=CARTESIAN_POINT('Ctrl Pts',(3.07581887099994,12.2,9.94846834399999));
#218336=CARTESIAN_POINT('Ctrl Pts',(3.07531941599994,12.2,9.94735184399998));
#218337=CARTESIAN_POINT('Ctrl Pts',(3.07482462299994,12.2,9.94624286799999));
#218338=CARTESIAN_POINT('Ctrl Pts',(3.07433448899994,12.2,9.94514144399999));
#218339=CARTESIAN_POINT('Ctrl Pts',(3.07384900699994,12.2,9.94404759999998));
#218340=CARTESIAN_POINT('Ctrl Pts',(3.07336817399994,12.2,9.94296136499998));
#218341=CARTESIAN_POINT('Ctrl Pts',(3.07289198199994,12.2,9.94188276499998));
#218342=CARTESIAN_POINT('Ctrl Pts',(3.07242042599994,12.2,9.94081182999999));
#218343=CARTESIAN_POINT('Ctrl Pts',(3.07195350199994,12.2,9.93974858599999));
#218344=CARTESIAN_POINT('Ctrl Pts',(3.07149120299994,12.2,9.93869306299998));
#218345=CARTESIAN_POINT('Ctrl Pts',(3.07103352399994,12.2,9.93764528999998));
#218346=CARTESIAN_POINT('Ctrl Pts',(3.07058045999994,12.2,9.93660529599998));
#218347=CARTESIAN_POINT('Ctrl Pts',(3.07013200399994,12.2,9.93557310899998));
#218348=CARTESIAN_POINT('Ctrl Pts',(3.06968815199995,12.2,9.93454875599999));
#218349=CARTESIAN_POINT('Ctrl Pts',(3.06924889699994,12.2,9.93353227099998));
#218350=CARTESIAN_POINT('Ctrl Pts',(3.06881423399994,12.2,9.93252367899998));
#218351=CARTESIAN_POINT('Ctrl Pts',(3.06838415699994,12.2,9.93152301099999));
#218352=CARTESIAN_POINT('Ctrl Pts',(3.06795865999994,12.2,9.93053029599999));
#218353=CARTESIAN_POINT('Ctrl Pts',(3.06753773799994,12.2,9.92954556499999));
#218354=CARTESIAN_POINT('Ctrl Pts',(3.06712138399994,12.2,9.92856884599998));
#218355=CARTESIAN_POINT('Ctrl Pts',(3.06670959199994,12.2,9.92760017099998));
#218356=CARTESIAN_POINT('Ctrl Pts',(3.06630235599994,12.2,9.92663956799999));
#218357=CARTESIAN_POINT('Ctrl Pts',(3.06589967099994,12.2,9.92568706699998));
#218358=CARTESIAN_POINT('Ctrl Pts',(3.06550152999994,12.2,9.92474270099999));
#218359=CARTESIAN_POINT('Ctrl Pts',(3.06510792699994,12.2,9.92380649899999));
#218360=CARTESIAN_POINT('Ctrl Pts',(3.06471885599994,12.2,9.92287849099998));
#218361=CARTESIAN_POINT('Ctrl Pts',(3.06433431199994,12.2,9.92195870799998));
#218362=CARTESIAN_POINT('Ctrl Pts',(3.06395428599994,12.2,9.92104718299998));
#218363=CARTESIAN_POINT('Ctrl Pts',(3.06357877399994,12.2,9.92014394499999));
#218364=CARTESIAN_POINT('Ctrl Pts',(3.06320776799994,12.2,9.91924902499999));
#218365=CARTESIAN_POINT('Ctrl Pts',(3.06284126399994,12.2,9.91836245599998));
#218366=CARTESIAN_POINT('Ctrl Pts',(3.06247925299994,12.2,9.91748426799998));
#218367=CARTESIAN_POINT('Ctrl Pts',(3.06212172999994,12.2,9.91661449399999));
#218368=CARTESIAN_POINT('Ctrl Pts',(3.06176868699994,12.2,9.91575316599998));
#218369=CARTESIAN_POINT('Ctrl Pts',(3.06142212599994,12.2,9.91490522599998));
#218370=CARTESIAN_POINT('Ctrl Pts',(3.06114880299994,12.2,9.91423456699999));
#218371=CARTESIAN_POINT('Ctrl Pts',(3.06094627499994,12.2,9.91373655899999));
#218372=CARTESIAN_POINT('Ctrl Pts',(3.06081277599994,12.2,9.91340782599998));
#218373=CARTESIAN_POINT('Ctrl Pts',(3.06074721199994,12.2,9.91324626499999));
#218374=CARTESIAN_POINT('Ctrl Pts',(3.06074721199994,15.2,9.91324626499999));
#218375=CARTESIAN_POINT('Ctrl Pts',(3.06081277599994,15.2,9.91340782599998));
#218376=CARTESIAN_POINT('Ctrl Pts',(3.06094627499994,15.2,9.91373655899999));
#218377=CARTESIAN_POINT('Ctrl Pts',(3.06114880299994,15.2,9.91423456699999));
#218378=CARTESIAN_POINT('Ctrl Pts',(3.06142212599994,15.2,9.91490522599998));
#218379=CARTESIAN_POINT('Ctrl Pts',(3.06176868699994,15.2,9.91575316599998));
#218380=CARTESIAN_POINT('Ctrl Pts',(3.06212172999994,15.2,9.91661449399999));
#218381=CARTESIAN_POINT('Ctrl Pts',(3.06247925299994,15.2,9.91748426799998));
#218382=CARTESIAN_POINT('Ctrl Pts',(3.06284126399994,15.2,9.91836245599998));
#218383=CARTESIAN_POINT('Ctrl Pts',(3.06320776799994,15.2,9.91924902499999));
#218384=CARTESIAN_POINT('Ctrl Pts',(3.06357877399994,15.2,9.92014394499999));
#218385=CARTESIAN_POINT('Ctrl Pts',(3.06395428599994,15.2,9.92104718299998));
#218386=CARTESIAN_POINT('Ctrl Pts',(3.06433431199994,15.2,9.92195870799998));
#218387=CARTESIAN_POINT('Ctrl Pts',(3.06471885599994,15.2,9.92287849099998));
#218388=CARTESIAN_POINT('Ctrl Pts',(3.06510792699994,15.2,9.92380649899999));
#218389=CARTESIAN_POINT('Ctrl Pts',(3.06550152999994,15.2,9.92474270099999));
#218390=CARTESIAN_POINT('Ctrl Pts',(3.06589967099994,15.2,9.92568706699998));
#218391=CARTESIAN_POINT('Ctrl Pts',(3.06630235599994,15.2,9.92663956799999));
#218392=CARTESIAN_POINT('Ctrl Pts',(3.06670959199994,15.2,9.92760017099998));
#218393=CARTESIAN_POINT('Ctrl Pts',(3.06712138399994,15.2,9.92856884599998));
#218394=CARTESIAN_POINT('Ctrl Pts',(3.06753773799994,15.2,9.92954556499999));
#218395=CARTESIAN_POINT('Ctrl Pts',(3.06795865999994,15.2,9.93053029599999));
#218396=CARTESIAN_POINT('Ctrl Pts',(3.06838415699994,15.2,9.93152301099999));
#218397=CARTESIAN_POINT('Ctrl Pts',(3.06881423399994,15.2,9.93252367899998));
#218398=CARTESIAN_POINT('Ctrl Pts',(3.06924889699994,15.2,9.93353227099998));
#218399=CARTESIAN_POINT('Ctrl Pts',(3.06968815199995,15.2,9.93454875599999));
#218400=CARTESIAN_POINT('Ctrl Pts',(3.07013200399994,15.2,9.93557310899998));
#218401=CARTESIAN_POINT('Ctrl Pts',(3.07058045999994,15.2,9.93660529599998));
#218402=CARTESIAN_POINT('Ctrl Pts',(3.07103352399994,15.2,9.93764528999998));
#218403=CARTESIAN_POINT('Ctrl Pts',(3.07149120299994,15.2,9.93869306299998));
#218404=CARTESIAN_POINT('Ctrl Pts',(3.07195350199994,15.2,9.93974858599999));
#218405=CARTESIAN_POINT('Ctrl Pts',(3.07242042599994,15.2,9.94081182999999));
#218406=CARTESIAN_POINT('Ctrl Pts',(3.07289198199994,15.2,9.94188276499998));
#218407=CARTESIAN_POINT('Ctrl Pts',(3.07336817399994,15.2,9.94296136499998));
#218408=CARTESIAN_POINT('Ctrl Pts',(3.07384900699994,15.2,9.94404759999998));
#218409=CARTESIAN_POINT('Ctrl Pts',(3.07433448899994,15.2,9.94514144399999));
#218410=CARTESIAN_POINT('Ctrl Pts',(3.07482462299994,15.2,9.94624286799999));
#218411=CARTESIAN_POINT('Ctrl Pts',(3.07531941599994,15.2,9.94735184399998));
#218412=CARTESIAN_POINT('Ctrl Pts',(3.07581887099994,15.2,9.94846834399999));
#218413=CARTESIAN_POINT('Ctrl Pts',(3.07632299499994,15.2,9.94959233999998));
#218414=CARTESIAN_POINT('Ctrl Pts',(3.07683179299994,15.2,9.95072380599998));
#218415=CARTESIAN_POINT('Ctrl Pts',(3.07734526999994,15.2,9.95186271399999));
#218416=CARTESIAN_POINT('Ctrl Pts',(3.07786343199994,15.2,9.95300903699999));
#218417=CARTESIAN_POINT('Ctrl Pts',(3.07838628099995,15.2,9.95416274699998));
#218418=CARTESIAN_POINT('Ctrl Pts',(3.07891382499994,15.2,9.95532381799999));
#218419=CARTESIAN_POINT('Ctrl Pts',(3.07944606999994,15.2,9.95649222299999));
#218420=CARTESIAN_POINT('Ctrl Pts',(3.07998301799994,15.2,9.95766793499998));
#218421=CARTESIAN_POINT('Ctrl Pts',(3.08052467399994,15.2,9.95885092599998));
#218422=CARTESIAN_POINT('Ctrl Pts',(3.08107104499994,15.2,9.96004117299999));
#218423=CARTESIAN_POINT('Ctrl Pts',(3.08162213499994,15.2,9.96123864599999));
#218424=CARTESIAN_POINT('Ctrl Pts',(3.08217794999994,15.2,9.96244332099998));
#218425=CARTESIAN_POINT('Ctrl Pts',(3.08273849199994,15.2,9.96365516999998));
#218426=CARTESIAN_POINT('Ctrl Pts',(3.08330376799994,15.2,9.96487416799998));
#218427=CARTESIAN_POINT('Ctrl Pts',(3.08387378199994,15.2,9.96610028999999));
#218428=CARTESIAN_POINT('Ctrl Pts',(3.08444853899994,15.2,9.96733350799998));
#218429=CARTESIAN_POINT('Ctrl Pts',(3.08502804299994,15.2,9.96857379799999));
#218430=CARTESIAN_POINT('Ctrl Pts',(3.08561229999994,15.2,9.96982113299998));
#218431=CARTESIAN_POINT('Ctrl Pts',(3.08620131299994,15.2,9.97107548899999));
#218432=CARTESIAN_POINT('Ctrl Pts',(3.08679508799994,15.2,9.97233683899999));
#218433=CARTESIAN_POINT('Ctrl Pts',(3.08739362899995,15.2,9.97360515799999));
#218434=CARTESIAN_POINT('Ctrl Pts',(3.08799693999994,15.2,9.97488042299998));
#218435=CARTESIAN_POINT('Ctrl Pts',(3.08860502499994,15.2,9.97616260499999));
#218436=CARTESIAN_POINT('Ctrl Pts',(3.08921789099994,15.2,9.97745168099998));
#218437=CARTESIAN_POINT('Ctrl Pts',(3.08983553999994,15.2,9.97874762799999));
#218438=CARTESIAN_POINT('Ctrl Pts',(3.09045797699994,15.2,9.98005041799999));
#218439=CARTESIAN_POINT('Ctrl Pts',(3.09108520699994,15.2,9.98136002699999));
#218440=CARTESIAN_POINT('Ctrl Pts',(3.09171723299994,15.2,9.98267643199998));
#218441=CARTESIAN_POINT('Ctrl Pts',(3.09235405999994,15.2,9.98399960799999));
#218442=CARTESIAN_POINT('Ctrl Pts',(3.09299569299994,15.2,9.98532952799999));
#218443=CARTESIAN_POINT('Ctrl Pts',(3.09364213499994,15.2,9.98666617199999));
#218444=CARTESIAN_POINT('Ctrl Pts',(3.09429339099994,15.2,9.98800951199998));
#218445=CARTESIAN_POINT('Ctrl Pts',(3.09494946499994,15.2,9.98935952599999));
#218446=CARTESIAN_POINT('Ctrl Pts',(3.09561036199994,15.2,9.99071618899999));
#218447=CARTESIAN_POINT('Ctrl Pts',(3.09627608499994,15.2,9.99207947799999));
#218448=CARTESIAN_POINT('Ctrl Pts',(3.09694663699994,15.2,9.99344936799999));
#218449=CARTESIAN_POINT('Ctrl Pts',(3.09762202399994,15.2,9.99482583699999));
#218450=CARTESIAN_POINT('Ctrl Pts',(3.09830224899994,15.2,9.99620885899999));
#218451=CARTESIAN_POINT('Ctrl Pts',(3.09898731599994,15.2,9.99759841199998));
#218452=CARTESIAN_POINT('Ctrl Pts',(3.09967723099994,15.2,9.99899447299999));
#218453=CARTESIAN_POINT('Ctrl Pts',(3.10037199499994,15.2,10.000397017));
#218454=CARTESIAN_POINT('Ctrl Pts',(3.10107161399995,15.2,10.001806022));
#218455=CARTESIAN_POINT('Ctrl Pts',(3.10177608999994,15.2,10.003221464));
#218456=CARTESIAN_POINT('Ctrl Pts',(3.10248542799994,15.2,10.00464332));
#218457=CARTESIAN_POINT('Ctrl Pts',(3.10319963199994,15.2,10.006071567));
#218458=CARTESIAN_POINT('Ctrl Pts',(3.10391870499994,15.2,10.007506183));
#218459=CARTESIAN_POINT('Ctrl Pts',(3.10464265199994,15.2,10.008947144));
#218460=CARTESIAN_POINT('Ctrl Pts',(3.10537147499995,15.2,10.010394428));
#218461=CARTESIAN_POINT('Ctrl Pts',(3.10610517999995,15.2,10.011848013));
#218462=CARTESIAN_POINT('Ctrl Pts',(3.10684376799994,15.2,10.013307874));
#218463=CARTESIAN_POINT('Ctrl Pts',(3.10758724499994,15.2,10.01477399));
#218464=CARTESIAN_POINT('Ctrl Pts',(3.10833561299994,15.2,10.01624634));
#218465=CARTESIAN_POINT('Ctrl Pts',(3.10908887599994,15.2,10.017724899));
#218466=CARTESIAN_POINT('Ctrl Pts',(3.10984703899994,15.2,10.019209646));
#218467=CARTESIAN_POINT('Ctrl Pts',(3.11061010399994,15.2,10.020700559));
#218468=CARTESIAN_POINT('Ctrl Pts',(3.11137807399994,15.2,10.022197616));
#218469=CARTESIAN_POINT('Ctrl Pts',(3.11215095499994,15.2,10.023700794));
#218470=CARTESIAN_POINT('Ctrl Pts',(3.11292874799994,15.2,10.025210072));
#218471=CARTESIAN_POINT('Ctrl Pts',(3.11371145699994,15.2,10.026725429));
#218472=CARTESIAN_POINT('Ctrl Pts',(3.11449908499994,15.2,10.028246841));
#218473=CARTESIAN_POINT('Ctrl Pts',(3.11529163799994,15.2,10.029774289));
#218474=CARTESIAN_POINT('Ctrl Pts',(3.11608911699994,15.2,10.031307748));
#218475=CARTESIAN_POINT('Ctrl Pts',(3.11689152499994,15.2,10.0328472));
#218476=CARTESIAN_POINT('Ctrl Pts',(3.11769886699994,15.2,10.034392622));
#218477=CARTESIAN_POINT('Ctrl Pts',(3.11851114499994,15.2,10.035943991));
#218478=CARTESIAN_POINT('Ctrl Pts',(3.11932836299994,15.2,10.037501289));
#218479=CARTESIAN_POINT('Ctrl Pts',(3.12015052399994,15.2,10.039064492));
#218480=CARTESIAN_POINT('Ctrl Pts',(3.12097763099994,15.2,10.040633581));
#218481=CARTESIAN_POINT('Ctrl Pts',(3.12180968799994,15.2,10.042208533));
#218482=CARTESIAN_POINT('Ctrl Pts',(3.12264669699994,15.2,10.043789328));
#218483=CARTESIAN_POINT('Ctrl Pts',(3.12348866099994,15.2,10.045375946));
#218484=CARTESIAN_POINT('Ctrl Pts',(3.12433558499994,15.2,10.046968364));
#218485=CARTESIAN_POINT('Ctrl Pts',(3.12518747099995,15.2,10.048566563));
#218486=CARTESIAN_POINT('Ctrl Pts',(3.12604432099994,15.2,10.050170521));
#218487=CARTESIAN_POINT('Ctrl Pts',(3.12690613999994,15.2,10.051780219));
#218488=CARTESIAN_POINT('Ctrl Pts',(3.12777292999994,15.2,10.053395635));
#218489=CARTESIAN_POINT('Ctrl Pts',(3.12864469399994,15.2,10.05501675));
#218490=CARTESIAN_POINT('Ctrl Pts',(3.12952143499994,15.2,10.056643542));
#218491=CARTESIAN_POINT('Ctrl Pts',(3.13040315599994,15.2,10.058275991));
#218492=CARTESIAN_POINT('Ctrl Pts',(3.13128985999994,15.2,10.059914077));
#218493=CARTESIAN_POINT('Ctrl Pts',(3.13218154999995,15.2,10.061557781));
#218494=CARTESIAN_POINT('Ctrl Pts',(3.13307822999994,15.2,10.063207081));
#218495=CARTESIAN_POINT('Ctrl Pts',(3.13397989999994,15.2,10.064861958));
#218496=CARTESIAN_POINT('Ctrl Pts',(3.13488656499994,15.2,10.066522392));
#218497=CARTESIAN_POINT('Ctrl Pts',(3.13579822699994,15.2,10.068188362));
#218498=CARTESIAN_POINT('Ctrl Pts',(3.13671488999994,15.2,10.069859849));
#218499=CARTESIAN_POINT('Ctrl Pts',(3.13763655599994,15.2,10.071536834));
#218500=CARTESIAN_POINT('Ctrl Pts',(3.13856322699994,15.2,10.073219296));
#218501=CARTESIAN_POINT('Ctrl Pts',(3.13949490699994,15.2,10.074907216));
#218502=CARTESIAN_POINT('Ctrl Pts',(3.14043159899994,15.2,10.076600574));
#218503=CARTESIAN_POINT('Ctrl Pts',(3.14137330399994,15.2,10.078299351));
#218504=CARTESIAN_POINT('Ctrl Pts',(3.14232002399994,15.2,10.080003527));
#218505=CARTESIAN_POINT('Ctrl Pts',(3.14327176599994,15.2,10.081713083));
#218506=CARTESIAN_POINT('Ctrl Pts',(3.14422852799995,15.2,10.083427999));
#218507=CARTESIAN_POINT('Ctrl Pts',(3.14519031499994,15.2,10.085148257));
#218508=CARTESIAN_POINT('Ctrl Pts',(3.14615712899994,15.2,10.086873837));
#218509=CARTESIAN_POINT('Ctrl Pts',(3.14712897199994,15.2,10.08860472));
#218510=CARTESIAN_POINT('Ctrl Pts',(3.14810584799994,15.2,10.090340886));
#218511=CARTESIAN_POINT('Ctrl Pts',(3.14908775899994,15.2,10.092082318));
#218512=CARTESIAN_POINT('Ctrl Pts',(3.15007470599994,15.2,10.093828996));
#218513=CARTESIAN_POINT('Ctrl Pts',(3.15106669299994,15.2,10.0955809));
#218514=CARTESIAN_POINT('Ctrl Pts',(3.15206372299994,15.2,10.097338013));
#218515=CARTESIAN_POINT('Ctrl Pts',(3.15306579799994,15.2,10.099100315));
#218516=CARTESIAN_POINT('Ctrl Pts',(3.15407291799994,15.2,10.100867788));
#218517=CARTESIAN_POINT('Ctrl Pts',(3.15508508899994,15.2,10.102640413));
#218518=CARTESIAN_POINT('Ctrl Pts',(3.15610231199994,15.2,10.104418172));
#218519=CARTESIAN_POINT('Ctrl Pts',(3.15712458699994,15.2,10.106201046));
#218520=CARTESIAN_POINT('Ctrl Pts',(3.15815192199994,15.2,10.107989016));
#218521=CARTESIAN_POINT('Ctrl Pts',(3.15918431399994,15.2,10.109782065));
#218522=CARTESIAN_POINT('Ctrl Pts',(3.16022176599994,15.2,10.111580173));
#218523=CARTESIAN_POINT('Ctrl Pts',(3.16126428299994,15.2,10.113383323));
#218524=CARTESIAN_POINT('Ctrl Pts',(3.16231186499994,15.2,10.115191496));
#218525=CARTESIAN_POINT('Ctrl Pts',(3.16336451599994,15.2,10.117004675));
#218526=CARTESIAN_POINT('Ctrl Pts',(3.16442223699994,15.2,10.11882284));
#218527=CARTESIAN_POINT('Ctrl Pts',(3.16548502999995,15.2,10.120645975));
#218528=CARTESIAN_POINT('Ctrl Pts',(3.16655289799994,15.2,10.12247406));
#218529=CARTESIAN_POINT('Ctrl Pts',(3.16762584299994,15.2,10.124307078));
#218530=CARTESIAN_POINT('Ctrl Pts',(3.16870386699994,15.2,10.126145011));
#218531=CARTESIAN_POINT('Ctrl Pts',(3.16978697099994,15.2,10.127987842));
#218532=CARTESIAN_POINT('Ctrl Pts',(3.17087515899994,15.2,10.129835553));
#218533=CARTESIAN_POINT('Ctrl Pts',(3.17196843199994,15.2,10.131688125));
#218534=CARTESIAN_POINT('Ctrl Pts',(3.17306679399994,15.2,10.133545542));
#218535=CARTESIAN_POINT('Ctrl Pts',(3.17417024399994,15.2,10.135407784));
#218536=CARTESIAN_POINT('Ctrl Pts',(3.17527878599994,15.2,10.137274836));
#218537=CARTESIAN_POINT('Ctrl Pts',(3.17639242199995,15.2,10.13914668));
#218538=CARTESIAN_POINT('Ctrl Pts',(3.17751115299994,15.2,10.141023297));
#218539=CARTESIAN_POINT('Ctrl Pts',(3.17863498099995,15.2,10.142904671));
#218540=CARTESIAN_POINT('Ctrl Pts',(3.17976390999994,15.2,10.144790784));
#218541=CARTESIAN_POINT('Ctrl Pts',(3.18089793999994,15.2,10.146681619));
#218542=CARTESIAN_POINT('Ctrl Pts',(3.18203707299994,15.2,10.148577159));
#218543=CARTESIAN_POINT('Ctrl Pts',(3.18318131199995,15.2,10.150477387));
#218544=CARTESIAN_POINT('Ctrl Pts',(3.18433065699995,15.2,10.152382285));
#218545=CARTESIAN_POINT('Ctrl Pts',(3.18548511399994,15.2,10.154291836));
#218546=CARTESIAN_POINT('Ctrl Pts',(3.18664467899994,15.2,10.156206023));
#218547=CARTESIAN_POINT('Ctrl Pts',(3.18780935899994,15.2,10.158124831));
#218548=CARTESIAN_POINT('Ctrl Pts',(3.18897915299994,15.2,10.160048239));
#218549=CARTESIAN_POINT('Ctrl Pts',(3.19015406399994,15.2,10.161976234));
#218550=CARTESIAN_POINT('Ctrl Pts',(3.19133409399994,15.2,10.163908798));
#218551=CARTESIAN_POINT('Ctrl Pts',(3.19251924199994,15.2,10.165845913));
#218552=CARTESIAN_POINT('Ctrl Pts',(3.19370951399994,15.2,10.167787564));
#218553=CARTESIAN_POINT('Ctrl Pts',(3.19490490899994,15.2,10.169733732));
#218554=CARTESIAN_POINT('Ctrl Pts',(3.19610542999994,15.2,10.171684403));
#218555=CARTESIAN_POINT('Ctrl Pts',(3.19731107699994,15.2,10.173639559));
#218556=CARTESIAN_POINT('Ctrl Pts',(3.19852185399994,15.2,10.175599184));
#218557=CARTESIAN_POINT('Ctrl Pts',(3.19973776199994,15.2,10.17756326));
#218558=CARTESIAN_POINT('Ctrl Pts',(3.20095880099994,15.2,10.179531773));
#218559=CARTESIAN_POINT('Ctrl Pts',(3.20218497399994,15.2,10.181504705));
#218560=CARTESIAN_POINT('Ctrl Pts',(3.20341628299994,15.2,10.183482041));
#218561=CARTESIAN_POINT('Ctrl Pts',(3.20465272999995,15.2,10.185463762));
#218562=CARTESIAN_POINT('Ctrl Pts',(3.20589431499994,15.2,10.187449854));
#218563=CARTESIAN_POINT('Ctrl Pts',(3.20714103999994,15.2,10.189440301));
#218564=CARTESIAN_POINT('Ctrl Pts',(3.20839290699994,15.2,10.191435086));
#218565=CARTESIAN_POINT('Ctrl Pts',(3.20964991799995,15.2,10.193434192));
#218566=CARTESIAN_POINT('Ctrl Pts',(3.21091207399995,15.2,10.195437604));
#218567=CARTESIAN_POINT('Ctrl Pts',(3.21217937699994,15.2,10.197445307));
#218568=CARTESIAN_POINT('Ctrl Pts',(3.21345182799994,15.2,10.199457283));
#218569=CARTESIAN_POINT('Ctrl Pts',(3.21472942799994,15.2,10.201473517));
#218570=CARTESIAN_POINT('Ctrl Pts',(3.21601217999994,15.2,10.203493994));
#218571=CARTESIAN_POINT('Ctrl Pts',(3.21730008399994,15.2,10.205518696));
#218572=CARTESIAN_POINT('Ctrl Pts',(3.21859314299994,15.2,10.20754761));
#218573=CARTESIAN_POINT('Ctrl Pts',(3.21989135599994,15.2,10.209580717));
#218574=CARTESIAN_POINT('Ctrl Pts',(3.22119472699995,15.2,10.211618004));
#218575=CARTESIAN_POINT('Ctrl Pts',(3.22250325599994,15.2,10.213659454));
#218576=CARTESIAN_POINT('Ctrl Pts',(3.22381694499994,15.2,10.215705052));
#218577=CARTESIAN_POINT('Ctrl Pts',(3.22513579399994,15.2,10.217754781));
#218578=CARTESIAN_POINT('Ctrl Pts',(3.22645980699994,15.2,10.219808628));
#218579=CARTESIAN_POINT('Ctrl Pts',(3.22778898299994,15.2,10.221866575));
#218580=CARTESIAN_POINT('Ctrl Pts',(3.22912332499994,15.2,10.223928608));
#218581=CARTESIAN_POINT('Ctrl Pts',(3.23046283199994,15.2,10.225994711));
#218582=CARTESIAN_POINT('Ctrl Pts',(3.23180750799994,15.2,10.228064869));
#218583=CARTESIAN_POINT('Ctrl Pts',(3.23315735299994,15.2,10.230139067));
#218584=CARTESIAN_POINT('Ctrl Pts',(3.23451236799994,15.2,10.232217288));
#218585=CARTESIAN_POINT('Ctrl Pts',(3.23587255499994,15.2,10.23429952));
#218586=CARTESIAN_POINT('Ctrl Pts',(3.23723791499994,15.2,10.236385745));
#218587=CARTESIAN_POINT('Ctrl Pts',(3.23860844899994,15.2,10.238475948));
#218588=CARTESIAN_POINT('Ctrl Pts',(3.23998415799994,15.2,10.240570115));
#218589=CARTESIAN_POINT('Ctrl Pts',(3.24136504399994,15.2,10.242668229));
#218590=CARTESIAN_POINT('Ctrl Pts',(3.24275110699995,15.2,10.244770278));
#218591=CARTESIAN_POINT('Ctrl Pts',(3.24414234999994,15.2,10.246876245));
#218592=CARTESIAN_POINT('Ctrl Pts',(3.24553877199994,15.2,10.248986116));
#218593=CARTESIAN_POINT('Ctrl Pts',(3.24694037599994,15.2,10.251099875));
#218594=CARTESIAN_POINT('Ctrl Pts',(3.24834716199994,15.2,10.253217507));
#218595=CARTESIAN_POINT('Ctrl Pts',(3.24975913199995,15.2,10.255338999));
#218596=CARTESIAN_POINT('Ctrl Pts',(3.25117628599994,15.2,10.257464334));
#218597=CARTESIAN_POINT('Ctrl Pts',(3.25259862599995,15.2,10.259593498));
#218598=CARTESIAN_POINT('Ctrl Pts',(3.25402615299994,15.2,10.261726478));
#218599=CARTESIAN_POINT('Ctrl Pts',(3.25545886799994,15.2,10.263863257));
#218600=CARTESIAN_POINT('Ctrl Pts',(3.25689677199994,15.2,10.266003821));
#218601=CARTESIAN_POINT('Ctrl Pts',(3.25833986599994,15.2,10.268148156));
#218602=CARTESIAN_POINT('Ctrl Pts',(3.25978815099994,15.2,10.270296246));
#218603=CARTESIAN_POINT('Ctrl Pts',(3.26124162699994,15.2,10.272448079));
#218604=CARTESIAN_POINT('Ctrl Pts',(3.26270029699995,15.2,10.274603639));
#218605=CARTESIAN_POINT('Ctrl Pts',(3.26416416099994,15.2,10.276762911));
#218606=CARTESIAN_POINT('Ctrl Pts',(3.26563321999994,15.2,10.27892588));
#218607=CARTESIAN_POINT('Ctrl Pts',(3.26710747499994,15.2,10.281092534));
#218608=CARTESIAN_POINT('Ctrl Pts',(3.26858692799994,15.2,10.283262858));
#218609=CARTESIAN_POINT('Ctrl Pts',(3.27007157799994,15.2,10.285436836));
#218610=CARTESIAN_POINT('Ctrl Pts',(3.27156142599994,15.2,10.287614454));
#218611=CARTESIAN_POINT('Ctrl Pts',(3.27305647499994,15.2,10.2897957));
#218612=CARTESIAN_POINT('Ctrl Pts',(3.27455672399994,15.2,10.291980559));
#218613=CARTESIAN_POINT('Ctrl Pts',(3.27606217499994,15.2,10.294169016));
#218614=CARTESIAN_POINT('Ctrl Pts',(3.27757282699995,15.2,10.296361056));
#218615=CARTESIAN_POINT('Ctrl Pts',(3.27908868399994,15.2,10.298556666));
#218616=CARTESIAN_POINT('Ctrl Pts',(3.28060974399994,15.2,10.300755834));
#218617=CARTESIAN_POINT('Ctrl Pts',(3.28213600999995,15.2,10.302958542));
#218618=CARTESIAN_POINT('Ctrl Pts',(3.28366748099994,15.2,10.305164779));
#218619=CARTESIAN_POINT('Ctrl Pts',(3.28520415899995,15.2,10.307374529));
#218620=CARTESIAN_POINT('Ctrl Pts',(3.28674604399994,15.2,10.30958778));
#218621=CARTESIAN_POINT('Ctrl Pts',(3.28829313699994,15.2,10.311804518));
#218622=CARTESIAN_POINT('Ctrl Pts',(3.28984543999994,15.2,10.314024727));
#218623=CARTESIAN_POINT('Ctrl Pts',(3.29140295199994,15.2,10.316248395));
#218624=CARTESIAN_POINT('Ctrl Pts',(3.29296567499994,15.2,10.318475509));
#218625=CARTESIAN_POINT('Ctrl Pts',(3.29453360899994,15.2,10.320706052));
#218626=CARTESIAN_POINT('Ctrl Pts',(3.29610675499994,15.2,10.322940014));
#218627=CARTESIAN_POINT('Ctrl Pts',(3.29768511299994,15.2,10.325177379));
#218628=CARTESIAN_POINT('Ctrl Pts',(3.29926868599994,15.2,10.327418135));
#218629=CARTESIAN_POINT('Ctrl Pts',(3.30085747199994,15.2,10.329662268));
#218630=CARTESIAN_POINT('Ctrl Pts',(3.30245147199994,15.2,10.331909762));
#218631=CARTESIAN_POINT('Ctrl Pts',(3.30405068899994,15.2,10.334160606));
#218632=CARTESIAN_POINT('Ctrl Pts',(3.30565512199994,15.2,10.336414786));
#218633=CARTESIAN_POINT('Ctrl Pts',(3.30726477099994,15.2,10.33867229));
#218634=CARTESIAN_POINT('Ctrl Pts',(3.30920261270556,15.2,10.3413852645478));
#218635=CARTESIAN_POINT('Ctrl Pts',(3.3111482782355,15.2,10.3441031813495));
#218636=CARTESIAN_POINT('Ctrl Pts',(3.31310177376438,15.2,10.3468260146505));
#218637=CARTESIAN_POINT('Ctrl Pts',(3.31506309947107,15.2,10.349553738699));
#218638=CARTESIAN_POINT('Ctrl Pts',(3.31703225499994,15.2,10.352286327));
#218639=CARTESIAN_POINT('Ctrl Pts',(3.31867843899994,15.2,10.354566712));
#218640=CARTESIAN_POINT('Ctrl Pts',(3.32032984499994,15.2,10.356850313));
#218641=CARTESIAN_POINT('Ctrl Pts',(3.32198647199994,15.2,10.359137117));
#218642=CARTESIAN_POINT('Ctrl Pts',(3.32364832199994,15.2,10.36142711));
#218643=CARTESIAN_POINT('Ctrl Pts',(3.32531539599994,15.2,10.36372028));
#218644=CARTESIAN_POINT('Ctrl Pts',(3.32698769299994,15.2,10.366016614));
#218645=CARTESIAN_POINT('Ctrl Pts',(3.32866521499994,15.2,10.368316097));
#218646=CARTESIAN_POINT('Ctrl Pts',(3.33034796099994,15.2,10.370618718));
#218647=CARTESIAN_POINT('Ctrl Pts',(3.33203593199995,15.2,10.372924463));
#218648=CARTESIAN_POINT('Ctrl Pts',(3.33372912899994,15.2,10.375233319));
#218649=CARTESIAN_POINT('Ctrl Pts',(3.33542755199994,15.2,10.377545274));
#218650=CARTESIAN_POINT('Ctrl Pts',(3.33713120199994,15.2,10.379860313));
#218651=CARTESIAN_POINT('Ctrl Pts',(3.33884007799994,15.2,10.382178427));
#218652=CARTESIAN_POINT('Ctrl Pts',(3.34055418199994,15.2,10.384499599));
#218653=CARTESIAN_POINT('Ctrl Pts',(3.34227351299994,15.2,10.386823818));
#218654=CARTESIAN_POINT('Ctrl Pts',(3.34399807299994,15.2,10.389151072));
#218655=CARTESIAN_POINT('Ctrl Pts',(3.34572786099995,15.2,10.391481347));
#218656=CARTESIAN_POINT('Ctrl Pts',(3.34746287999995,15.2,10.393814631));
#218657=CARTESIAN_POINT('Ctrl Pts',(3.34920312499994,15.2,10.396150911));
#218658=CARTESIAN_POINT('Ctrl Pts',(3.35094860199994,15.2,10.398490174));
#218659=CARTESIAN_POINT('Ctrl Pts',(3.35269930899994,15.2,10.400832408));
#218660=CARTESIAN_POINT('Ctrl Pts',(3.35445524599994,15.2,10.4031776));
#218661=CARTESIAN_POINT('Ctrl Pts',(3.35621641399994,15.2,10.405525737));
#218662=CARTESIAN_POINT('Ctrl Pts',(3.35798281299994,15.2,10.407876808));
#218663=CARTESIAN_POINT('Ctrl Pts',(3.35975444299994,15.2,10.410230799));
#218664=CARTESIAN_POINT('Ctrl Pts',(3.36153130499994,15.2,10.412587698));
#218665=CARTESIAN_POINT('Ctrl Pts',(3.36331339899994,15.2,10.414947493));
#218666=CARTESIAN_POINT('Ctrl Pts',(3.36510072599994,15.2,10.417310171));
#218667=CARTESIAN_POINT('Ctrl Pts',(3.36689328399994,15.2,10.419675719));
#218668=CARTESIAN_POINT('Ctrl Pts',(3.36869107699994,15.2,10.422044126));
#218669=CARTESIAN_POINT('Ctrl Pts',(3.37049410099994,15.2,10.424415378));
#218670=CARTESIAN_POINT('Ctrl Pts',(3.37230235899994,15.2,10.426789465));
#218671=CARTESIAN_POINT('Ctrl Pts',(3.37411584999994,15.2,10.429166374));
#218672=CARTESIAN_POINT('Ctrl Pts',(3.37593457599994,15.2,10.43154609));
#218673=CARTESIAN_POINT('Ctrl Pts',(3.37775853499994,15.2,10.433928604));
#218674=CARTESIAN_POINT('Ctrl Pts',(3.37958772799994,15.2,10.436313903));
#218675=CARTESIAN_POINT('Ctrl Pts',(3.38142215599994,15.2,10.438701973));
#218676=CARTESIAN_POINT('Ctrl Pts',(3.38326181899995,15.2,10.441092806));
#218677=CARTESIAN_POINT('Ctrl Pts',(3.38510671499994,15.2,10.443486385));
#218678=CARTESIAN_POINT('Ctrl Pts',(3.38695684699994,15.2,10.445882701));
#218679=CARTESIAN_POINT('Ctrl Pts',(3.38881221399994,15.2,10.448281741));
#218680=CARTESIAN_POINT('Ctrl Pts',(3.39067281599994,15.2,10.450683492));
#218681=CARTESIAN_POINT('Ctrl Pts',(3.39253865299994,15.2,10.453087944));
#218682=CARTESIAN_POINT('Ctrl Pts',(3.39440972599995,15.2,10.455495084));
#218683=CARTESIAN_POINT('Ctrl Pts',(3.39628603499994,15.2,10.4579049));
#218684=CARTESIAN_POINT('Ctrl Pts',(3.39816757899994,15.2,10.460317381));
#218685=CARTESIAN_POINT('Ctrl Pts',(3.40005435899994,15.2,10.462732513));
#218686=CARTESIAN_POINT('Ctrl Pts',(3.40194637399994,15.2,10.465150286));
#218687=CARTESIAN_POINT('Ctrl Pts',(3.40384362599994,15.2,10.467570687));
#218688=CARTESIAN_POINT('Ctrl Pts',(3.40574611299994,15.2,10.469993704));
#218689=CARTESIAN_POINT('Ctrl Pts',(3.40765383599994,15.2,10.472419326));
#218690=CARTESIAN_POINT('Ctrl Pts',(3.40956679599994,15.2,10.474847543));
#218691=CARTESIAN_POINT('Ctrl Pts',(3.41148499199994,15.2,10.477278339));
#218692=CARTESIAN_POINT('Ctrl Pts',(3.41340842399994,15.2,10.479711706));
#218693=CARTESIAN_POINT('Ctrl Pts',(3.41533709199994,15.2,10.482147629));
#218694=CARTESIAN_POINT('Ctrl Pts',(3.41727099499994,15.2,10.4845861));
#218695=CARTESIAN_POINT('Ctrl Pts',(3.41921013599995,15.2,10.487027105));
#218696=CARTESIAN_POINT('Ctrl Pts',(3.42115451199994,15.2,10.489470632));
#218697=CARTESIAN_POINT('Ctrl Pts',(3.42310412599995,15.2,10.491916672));
#218698=CARTESIAN_POINT('Ctrl Pts',(3.42505897399994,15.2,10.49436521));
#218699=CARTESIAN_POINT('Ctrl Pts',(3.42701905899994,15.2,10.496816237));
#218700=CARTESIAN_POINT('Ctrl Pts',(3.42898437999994,15.2,10.49926974));
#218701=CARTESIAN_POINT('Ctrl Pts',(3.43095493699995,15.2,10.501725709));
#218702=CARTESIAN_POINT('Ctrl Pts',(3.43293072999994,15.2,10.504184131));
#218703=CARTESIAN_POINT('Ctrl Pts',(3.43491175999994,15.2,10.506644995));
#218704=CARTESIAN_POINT('Ctrl Pts',(3.43689802499994,15.2,10.50910829));
#218705=CARTESIAN_POINT('Ctrl Pts',(3.43888952499994,15.2,10.511574004));
#218706=CARTESIAN_POINT('Ctrl Pts',(3.44088626199994,15.2,10.514042126));
#218707=CARTESIAN_POINT('Ctrl Pts',(3.44288823299994,15.2,10.516512645));
#218708=CARTESIAN_POINT('Ctrl Pts',(3.44489543999994,15.2,10.51898555));
#218709=CARTESIAN_POINT('Ctrl Pts',(3.44690788299994,15.2,10.521460827));
#218710=CARTESIAN_POINT('Ctrl Pts',(3.44892555999994,15.2,10.523938468));
#218711=CARTESIAN_POINT('Ctrl Pts',(3.45094847299994,15.2,10.526418461));
#218712=CARTESIAN_POINT('Ctrl Pts',(3.45297662099994,15.2,10.528900792));
#218713=CARTESIAN_POINT('Ctrl Pts',(3.45501000299994,15.2,10.531385453));
#218714=CARTESIAN_POINT('Ctrl Pts',(3.45704861999995,15.2,10.533872432));
#218715=CARTESIAN_POINT('Ctrl Pts',(3.45909247099994,15.2,10.536361718));
#218716=CARTESIAN_POINT('Ctrl Pts',(3.46114155699994,15.2,10.538853298));
#218717=CARTESIAN_POINT('Ctrl Pts',(3.46319587599994,15.2,10.541347163));
#218718=CARTESIAN_POINT('Ctrl Pts',(3.46525542999994,15.2,10.543843302));
#218719=CARTESIAN_POINT('Ctrl Pts',(3.46732021699995,15.2,10.546341702));
#218720=CARTESIAN_POINT('Ctrl Pts',(3.46939023699994,15.2,10.548842353));
#218721=CARTESIAN_POINT('Ctrl Pts',(3.47146549099994,15.2,10.551345244));
#218722=CARTESIAN_POINT('Ctrl Pts',(3.47354597799994,15.2,10.553850365));
#218723=CARTESIAN_POINT('Ctrl Pts',(3.47563169699994,15.2,10.556357703));
#218724=CARTESIAN_POINT('Ctrl Pts',(3.47772264999994,15.2,10.558867249));
#218725=CARTESIAN_POINT('Ctrl Pts',(3.47981883399994,15.2,10.561378991));
#218726=CARTESIAN_POINT('Ctrl Pts',(3.48192024899994,15.2,10.563892917));
#218727=CARTESIAN_POINT('Ctrl Pts',(3.48402689799994,15.2,10.566409018));
#218728=CARTESIAN_POINT('Ctrl Pts',(3.48613877699994,15.2,10.568927282));
#218729=CARTESIAN_POINT('Ctrl Pts',(3.48825588699994,15.2,10.571447699));
#218730=CARTESIAN_POINT('Ctrl Pts',(3.49037822899994,15.2,10.573970259));
#218731=CARTESIAN_POINT('Ctrl Pts',(3.49250580099994,15.2,10.576494948));
#218732=CARTESIAN_POINT('Ctrl Pts',(3.49463860199994,15.2,10.579021758));
#218733=CARTESIAN_POINT('Ctrl Pts',(3.49677663399994,15.2,10.581550676));
#218734=CARTESIAN_POINT('Ctrl Pts',(3.49891989599994,15.2,10.584081694));
#218735=CARTESIAN_POINT('Ctrl Pts',(3.50106838699995,15.2,10.5866148));
#218736=CARTESIAN_POINT('Ctrl Pts',(3.50322210699994,15.2,10.589149983));
#218737=CARTESIAN_POINT('Ctrl Pts',(3.50538105499994,15.2,10.591687233));
#218738=CARTESIAN_POINT('Ctrl Pts',(3.50754523199994,15.2,10.594226538));
#218739=CARTESIAN_POINT('Ctrl Pts',(3.50971463599994,15.2,10.596767889));
#218740=CARTESIAN_POINT('Ctrl Pts',(3.51188926799994,15.2,10.599311274));
#218741=CARTESIAN_POINT('Ctrl Pts',(3.51406912699994,15.2,10.601856683));
#218742=CARTESIAN_POINT('Ctrl Pts',(3.51625421199994,15.2,10.604404106));
#218743=CARTESIAN_POINT('Ctrl Pts',(3.51844452399994,15.2,10.606953531));
#218744=CARTESIAN_POINT('Ctrl Pts',(3.52064006199994,15.2,10.609504948));
#218745=CARTESIAN_POINT('Ctrl Pts',(3.52284082599994,15.2,10.612058349));
#218746=CARTESIAN_POINT('Ctrl Pts',(3.52504681399994,15.2,10.61461372));
#218747=CARTESIAN_POINT('Ctrl Pts',(3.52725802799994,15.2,10.617171051));
#218748=CARTESIAN_POINT('Ctrl Pts',(3.52947446499994,15.2,10.619730334));
#218749=CARTESIAN_POINT('Ctrl Pts',(3.53169612599994,15.2,10.622291557));
#218750=CARTESIAN_POINT('Ctrl Pts',(3.53392300999994,15.2,10.624854709));
#218751=CARTESIAN_POINT('Ctrl Pts',(3.53615511699994,15.2,10.62741978));
#218752=CARTESIAN_POINT('Ctrl Pts',(3.53839244699994,15.2,10.62998676));
#218753=CARTESIAN_POINT('Ctrl Pts',(3.54063499799994,15.2,10.632555639));
#218754=CARTESIAN_POINT('Ctrl Pts',(3.54288277099994,15.2,10.635126406));
#218755=CARTESIAN_POINT('Ctrl Pts',(3.54513576499994,15.2,10.637699051));
#218756=CARTESIAN_POINT('Ctrl Pts',(3.54739397999994,15.2,10.640273563));
#218757=CARTESIAN_POINT('Ctrl Pts',(3.54965741499994,15.2,10.642849932));
#218758=CARTESIAN_POINT('Ctrl Pts',(3.55192606799994,15.2,10.645428149));
#218759=CARTESIAN_POINT('Ctrl Pts',(3.55419994099994,15.2,10.648008202));
#218760=CARTESIAN_POINT('Ctrl Pts',(3.55647903199994,15.2,10.650590083));
#218761=CARTESIAN_POINT('Ctrl Pts',(3.55876334099994,15.2,10.653173779));
#218762=CARTESIAN_POINT('Ctrl Pts',(3.56105286799994,15.2,10.655759282));
#218763=CARTESIAN_POINT('Ctrl Pts',(3.56334761099994,15.2,10.658346581));
#218764=CARTESIAN_POINT('Ctrl Pts',(3.56564757099994,15.2,10.660935667));
#218765=CARTESIAN_POINT('Ctrl Pts',(3.56795274699994,15.2,10.663526528));
#218766=CARTESIAN_POINT('Ctrl Pts',(3.57026313699994,15.2,10.666119155));
#218767=CARTESIAN_POINT('Ctrl Pts',(3.57257874199994,15.2,10.668713538));
#218768=CARTESIAN_POINT('Ctrl Pts',(3.57489956099994,15.2,10.671309666));
#218769=CARTESIAN_POINT('Ctrl Pts',(3.57722559299994,15.2,10.673907531));
#218770=CARTESIAN_POINT('Ctrl Pts',(3.57955683799994,15.2,10.67650712));
#218771=CARTESIAN_POINT('Ctrl Pts',(3.58189329599994,15.2,10.679108425));
#218772=CARTESIAN_POINT('Ctrl Pts',(3.58423496399995,15.2,10.681711437));
#218773=CARTESIAN_POINT('Ctrl Pts',(3.58658184499994,15.2,10.684316143));
#218774=CARTESIAN_POINT('Ctrl Pts',(3.58893393499994,15.2,10.686922536));
#218775=CARTESIAN_POINT('Ctrl Pts',(3.59129123599994,15.2,10.689530605));
#218776=CARTESIAN_POINT('Ctrl Pts',(3.59365374499994,15.2,10.692140339));
#218777=CARTESIAN_POINT('Ctrl Pts',(3.59602146199994,15.2,10.694751731));
#218778=CARTESIAN_POINT('Ctrl Pts',(3.59839438799994,15.2,10.697364767));
#218779=CARTESIAN_POINT('Ctrl Pts',(3.60077251999994,15.2,10.699979441));
#218780=CARTESIAN_POINT('Ctrl Pts',(3.60315585899994,15.2,10.702595741));
#218781=CARTESIAN_POINT('Ctrl Pts',(3.60554440399994,15.2,10.705213657));
#218782=CARTESIAN_POINT('Ctrl Pts',(3.60793815399994,15.2,10.707833181));
#218783=CARTESIAN_POINT('Ctrl Pts',(3.61033710899994,15.2,10.710454302));
#218784=CARTESIAN_POINT('Ctrl Pts',(3.61274126699994,15.2,10.71307701));
#218785=CARTESIAN_POINT('Ctrl Pts',(3.61515062899994,15.2,10.715701296));
#218786=CARTESIAN_POINT('Ctrl Pts',(3.61756519199994,15.2,10.718327151));
#218787=CARTESIAN_POINT('Ctrl Pts',(3.61998495799994,15.2,10.720954563));
#218788=CARTESIAN_POINT('Ctrl Pts',(3.62240992399994,15.2,10.723583524));
#218789=CARTESIAN_POINT('Ctrl Pts',(3.62484009099994,15.2,10.726214025));
#218790=CARTESIAN_POINT('Ctrl Pts',(3.62727545699994,15.2,10.728846054));
#218791=CARTESIAN_POINT('Ctrl Pts',(3.62971602199994,15.2,10.731479602));
#218792=CARTESIAN_POINT('Ctrl Pts',(3.63216178499994,15.2,10.734114662));
#218793=CARTESIAN_POINT('Ctrl Pts',(3.63461274499994,15.2,10.736751222));
#218794=CARTESIAN_POINT('Ctrl Pts',(3.63706890199994,15.2,10.739389272));
#218795=CARTESIAN_POINT('Ctrl Pts',(3.63953025499994,15.2,10.742028805));
#218796=CARTESIAN_POINT('Ctrl Pts',(3.64199680199994,15.2,10.744669808));
#218797=CARTESIAN_POINT('Ctrl Pts',(3.64446854399994,15.2,10.747312275));
#218798=CARTESIAN_POINT('Ctrl Pts',(3.64694547899994,15.2,10.749956194));
#218799=CARTESIAN_POINT('Ctrl Pts',(3.64942760599994,15.2,10.752601556));
#218800=CARTESIAN_POINT('Ctrl Pts',(3.65191492599994,15.2,10.755248353));
#218801=CARTESIAN_POINT('Ctrl Pts',(3.65440743699994,15.2,10.757896573));
#218802=CARTESIAN_POINT('Ctrl Pts',(3.65690513699994,15.2,10.760546208));
#218803=CARTESIAN_POINT('Ctrl Pts',(3.65940802899994,15.2,10.76319725));
#218804=CARTESIAN_POINT('Ctrl Pts',(3.66191610699994,15.2,10.765849687));
#218805=CARTESIAN_POINT('Ctrl Pts',(3.66442937399994,15.2,10.768503511));
#218806=CARTESIAN_POINT('Ctrl Pts',(3.66694782699994,15.2,10.771158713));
#218807=CARTESIAN_POINT('Ctrl Pts',(3.66947146699994,15.2,10.773815282));
#218808=CARTESIAN_POINT('Ctrl Pts',(3.67200029299994,15.2,10.776473211));
#218809=CARTESIAN_POINT('Ctrl Pts',(3.67453430199994,15.2,10.77913249));
#218810=CARTESIAN_POINT('Ctrl Pts',(3.67707349599994,15.2,10.781793108));
#218811=CARTESIAN_POINT('Ctrl Pts',(3.67961787099994,15.2,10.784455057));
#218812=CARTESIAN_POINT('Ctrl Pts',(3.68216742899994,15.2,10.787118327));
#218813=CARTESIAN_POINT('Ctrl Pts',(3.68472216799994,15.2,10.789782909));
#218814=CARTESIAN_POINT('Ctrl Pts',(3.68728208699994,15.2,10.792448794));
#218815=CARTESIAN_POINT('Ctrl Pts',(3.68984718499994,15.2,10.795115974));
#218816=CARTESIAN_POINT('Ctrl Pts',(3.69241746099994,15.2,10.797784438));
#218817=CARTESIAN_POINT('Ctrl Pts',(3.69499291499995,15.2,10.800454179));
#218818=CARTESIAN_POINT('Ctrl Pts',(3.69757354499994,15.2,10.803125184));
#218819=CARTESIAN_POINT('Ctrl Pts',(3.70015935099994,15.2,10.805797449));
#218820=CARTESIAN_POINT('Ctrl Pts',(3.70275033099994,15.2,10.808470961));
#218821=CARTESIAN_POINT('Ctrl Pts',(3.70534648499994,15.2,10.811145713));
#218822=CARTESIAN_POINT('Ctrl Pts',(3.70794781299994,15.2,10.813821695));
#218823=CARTESIAN_POINT('Ctrl Pts',(3.71055431199994,15.2,10.816498895));
#218824=CARTESIAN_POINT('Ctrl Pts',(3.71316598199994,15.2,10.819177306));
#218825=CARTESIAN_POINT('Ctrl Pts',(3.71578282099994,15.2,10.821856919));
#218826=CARTESIAN_POINT('Ctrl Pts',(3.71840482999994,15.2,10.824537725));
#218827=CARTESIAN_POINT('Ctrl Pts',(3.72103200699994,15.2,10.827219716));
#218828=CARTESIAN_POINT('Ctrl Pts',(3.72366435199994,15.2,10.829902884));
#218829=CARTESIAN_POINT('Ctrl Pts',(3.72630186199994,15.2,10.832587221));
#218830=CARTESIAN_POINT('Ctrl Pts',(3.72894453699994,15.2,10.835272717));
#218831=CARTESIAN_POINT('Ctrl Pts',(3.73159237799995,15.2,10.837959365));
#218832=CARTESIAN_POINT('Ctrl Pts',(3.73424538199994,15.2,10.840647153));
#218833=CARTESIAN_POINT('Ctrl Pts',(3.73690354699994,15.2,10.843336071));
#218834=CARTESIAN_POINT('Ctrl Pts',(3.73956687399994,15.2,10.846026106));
#218835=CARTESIAN_POINT('Ctrl Pts',(3.74223535999994,15.2,10.84871725));
#218836=CARTESIAN_POINT('Ctrl Pts',(3.74490900499994,15.2,10.85140949));
#218837=CARTESIAN_POINT('Ctrl Pts',(3.74758780799994,15.2,10.854102822));
#218838=CARTESIAN_POINT('Ctrl Pts',(3.75027176799994,15.2,10.856797236));
#218839=CARTESIAN_POINT('Ctrl Pts',(3.75296088399994,15.2,10.85949273));
#218840=CARTESIAN_POINT('Ctrl Pts',(3.75565515599994,15.2,10.862189302));
#218841=CARTESIAN_POINT('Ctrl Pts',(3.75781469799994,15.2,10.864347421));
#218842=CARTESIAN_POINT('Ctrl Pts',(3.75943667399994,15.2,10.865966495));
#218843=CARTESIAN_POINT('Ctrl Pts',(3.76051902299994,15.2,10.867046091));
#218844=CARTESIAN_POINT('Ctrl Pts',(3.76106045499994,15.2,10.867585944));
#218845=CARTESIAN_POINT('Ctrl Pts',(4.04260911699994,15.2,9.55499537099998));
#218846=CARTESIAN_POINT('Ctrl Pts',(4.04260911699994,11.6,9.55499537099998));
#218847=CARTESIAN_POINT('Ctrl Pts',(4.04266300399994,15.2,9.55516119299999));
#218848=CARTESIAN_POINT('Ctrl Pts',(4.04266300399994,11.6,9.55516119299999));
#218849=CARTESIAN_POINT('Ctrl Pts',(4.04277257899994,15.2,9.55549865399998));
#218850=CARTESIAN_POINT('Ctrl Pts',(4.04277257899994,11.6,9.55549865399998));
#218851=CARTESIAN_POINT('Ctrl Pts',(4.04293835799994,15.2,9.55601007199999));
#218852=CARTESIAN_POINT('Ctrl Pts',(4.04293835799994,11.6,9.55601007199999));
#218853=CARTESIAN_POINT('Ctrl Pts',(4.04316116499994,15.2,9.55669916199999));
#218854=CARTESIAN_POINT('Ctrl Pts',(4.04316116499994,11.6,9.55669916199999));
#218855=CARTESIAN_POINT('Ctrl Pts',(4.04344211299995,15.2,9.55757104199999));
#218856=CARTESIAN_POINT('Ctrl Pts',(4.04344211299995,11.6,9.55757104199999));
#218857=CARTESIAN_POINT('Ctrl Pts',(4.04372672499994,15.2,9.55845733799999));
#218858=CARTESIAN_POINT('Ctrl Pts',(4.04372672499994,11.6,9.55845733799999));
#218859=CARTESIAN_POINT('Ctrl Pts',(4.04401334799994,15.2,9.55935298199999));
#218860=CARTESIAN_POINT('Ctrl Pts',(4.04401334799994,11.6,9.55935298199999));
#218861=CARTESIAN_POINT('Ctrl Pts',(4.04430195599994,15.2,9.56025795199999));
#218862=CARTESIAN_POINT('Ctrl Pts',(4.04430195599994,11.6,9.56025795199999));
#218863=CARTESIAN_POINT('Ctrl Pts',(4.04459252299994,15.2,9.56117222799998));
#218864=CARTESIAN_POINT('Ctrl Pts',(4.04459252299994,11.6,9.56117222799998));
#218865=CARTESIAN_POINT('Ctrl Pts',(4.04488502599994,15.2,9.56209579099998));
#218866=CARTESIAN_POINT('Ctrl Pts',(4.04488502599994,11.6,9.56209579099998));
#218867=CARTESIAN_POINT('Ctrl Pts',(4.04517943799994,15.2,9.56302861999998));
#218868=CARTESIAN_POINT('Ctrl Pts',(4.04517943799994,11.6,9.56302861999998));
#218869=CARTESIAN_POINT('Ctrl Pts',(4.04547573399994,15.2,9.56397069599999));
#218870=CARTESIAN_POINT('Ctrl Pts',(4.04547573399994,11.6,9.56397069599999));
#218871=CARTESIAN_POINT('Ctrl Pts',(4.04577388999994,15.2,9.56492199899999));
#218872=CARTESIAN_POINT('Ctrl Pts',(4.04577388999994,11.6,9.56492199899999));
#218873=CARTESIAN_POINT('Ctrl Pts',(4.04607388099994,15.2,9.56588250899999));
#218874=CARTESIAN_POINT('Ctrl Pts',(4.04607388099994,11.6,9.56588250899999));
#218875=CARTESIAN_POINT('Ctrl Pts',(4.04637568199994,15.2,9.56685220699999));
#218876=CARTESIAN_POINT('Ctrl Pts',(4.04637568199994,11.6,9.56685220699999));
#218877=CARTESIAN_POINT('Ctrl Pts',(4.04667926799995,15.2,9.56783107399998));
#218878=CARTESIAN_POINT('Ctrl Pts',(4.04667926799995,11.6,9.56783107399998));
#218879=CARTESIAN_POINT('Ctrl Pts',(4.04698461699994,15.2,9.56881908899998));
#218880=CARTESIAN_POINT('Ctrl Pts',(4.04698461699994,11.6,9.56881908899998));
#218881=CARTESIAN_POINT('Ctrl Pts',(4.04729170299994,15.2,9.56981623299999));
#218882=CARTESIAN_POINT('Ctrl Pts',(4.04729170299994,11.6,9.56981623299999));
#218883=CARTESIAN_POINT('Ctrl Pts',(4.04760050099994,15.2,9.57082248799999));
#218884=CARTESIAN_POINT('Ctrl Pts',(4.04760050099994,11.6,9.57082248799999));
#218885=CARTESIAN_POINT('Ctrl Pts',(4.04791098999994,15.2,9.57183783399999));
#218886=CARTESIAN_POINT('Ctrl Pts',(4.04791098999994,11.6,9.57183783399999));
#218887=CARTESIAN_POINT('Ctrl Pts',(4.04822314399994,15.2,9.57286225199999));
#218888=CARTESIAN_POINT('Ctrl Pts',(4.04822314399994,11.6,9.57286225199999));
#218889=CARTESIAN_POINT('Ctrl Pts',(4.04853693799994,15.2,9.57389572199999));
#218890=CARTESIAN_POINT('Ctrl Pts',(4.04853693799994,11.6,9.57389572199999));
#218891=CARTESIAN_POINT('Ctrl Pts',(4.04885235199994,15.2,9.57493822799999));
#218892=CARTESIAN_POINT('Ctrl Pts',(4.04885235199994,11.6,9.57493822799999));
#218893=CARTESIAN_POINT('Ctrl Pts',(4.04916935999994,15.2,9.57598974799998));
#218894=CARTESIAN_POINT('Ctrl Pts',(4.04916935999994,11.6,9.57598974799998));
#218895=CARTESIAN_POINT('Ctrl Pts',(4.04948793899994,15.2,9.57705026599999));
#218896=CARTESIAN_POINT('Ctrl Pts',(4.04948793899994,11.6,9.57705026599999));
#218897=CARTESIAN_POINT('Ctrl Pts',(4.04980806699994,15.2,9.57811975999999));
#218898=CARTESIAN_POINT('Ctrl Pts',(4.04980806699994,11.6,9.57811975999999));
#218899=CARTESIAN_POINT('Ctrl Pts',(4.05012971799994,15.2,9.57919821499999));
#218900=CARTESIAN_POINT('Ctrl Pts',(4.05012971799994,11.6,9.57919821499999));
#218901=CARTESIAN_POINT('Ctrl Pts',(4.05045287199994,15.2,9.58028560899999));
#218902=CARTESIAN_POINT('Ctrl Pts',(4.05045287199994,11.6,9.58028560899999));
#218903=CARTESIAN_POINT('Ctrl Pts',(4.05077750499994,15.2,9.58138192699998));
#218904=CARTESIAN_POINT('Ctrl Pts',(4.05077750499994,11.6,9.58138192699998));
#218905=CARTESIAN_POINT('Ctrl Pts',(4.05110359499994,15.2,9.58248714699998));
#218906=CARTESIAN_POINT('Ctrl Pts',(4.05110359499994,11.6,9.58248714699998));
#218907=CARTESIAN_POINT('Ctrl Pts',(4.05143111699994,15.2,9.58360125399999));
#218908=CARTESIAN_POINT('Ctrl Pts',(4.05143111699994,11.6,9.58360125399999));
#218909=CARTESIAN_POINT('Ctrl Pts',(4.05176005199994,15.2,9.58472422799998));
#218910=CARTESIAN_POINT('Ctrl Pts',(4.05176005199994,11.6,9.58472422799998));
#218911=CARTESIAN_POINT('Ctrl Pts',(4.05209037399994,15.2,9.58585605099999));
#218912=CARTESIAN_POINT('Ctrl Pts',(4.05209037399994,11.6,9.58585605099999));
#218913=CARTESIAN_POINT('Ctrl Pts',(4.05242206299994,15.2,9.58699670499998));
#218914=CARTESIAN_POINT('Ctrl Pts',(4.05242206299994,11.6,9.58699670499998));
#218915=CARTESIAN_POINT('Ctrl Pts',(4.05275509599995,15.2,9.58814617299998));
#218916=CARTESIAN_POINT('Ctrl Pts',(4.05275509599995,11.6,9.58814617299998));
#218917=CARTESIAN_POINT('Ctrl Pts',(4.05308945099994,15.2,9.58930443499998));
#218918=CARTESIAN_POINT('Ctrl Pts',(4.05308945099994,11.6,9.58930443499998));
#218919=CARTESIAN_POINT('Ctrl Pts',(4.05342510599994,15.2,9.59047147499999));
#218920=CARTESIAN_POINT('Ctrl Pts',(4.05342510599994,11.6,9.59047147499999));
#218921=CARTESIAN_POINT('Ctrl Pts',(4.05376203899994,15.2,9.59164727399998));
#218922=CARTESIAN_POINT('Ctrl Pts',(4.05376203899994,11.6,9.59164727399998));
#218923=CARTESIAN_POINT('Ctrl Pts',(4.05410022799995,15.2,9.59283181599999));
#218924=CARTESIAN_POINT('Ctrl Pts',(4.05410022799995,11.6,9.59283181599999));
#218925=CARTESIAN_POINT('Ctrl Pts',(4.05443965299995,15.2,9.59402508099998));
#218926=CARTESIAN_POINT('Ctrl Pts',(4.05443965299995,11.6,9.59402508099998));
#218927=CARTESIAN_POINT('Ctrl Pts',(4.05478029099995,15.2,9.59522705199999));
#218928=CARTESIAN_POINT('Ctrl Pts',(4.05478029099995,11.6,9.59522705199999));
#218929=CARTESIAN_POINT('Ctrl Pts',(4.05512211899994,15.2,9.59643771299999));
#218930=CARTESIAN_POINT('Ctrl Pts',(4.05512211899994,11.6,9.59643771299999));
#218931=CARTESIAN_POINT('Ctrl Pts',(4.05546511799994,15.2,9.59765704599998));
#218932=CARTESIAN_POINT('Ctrl Pts',(4.05546511799994,11.6,9.59765704599998));
#218933=CARTESIAN_POINT('Ctrl Pts',(4.05580926699994,15.2,9.59888503199998));
#218934=CARTESIAN_POINT('Ctrl Pts',(4.05580926699994,11.6,9.59888503199998));
#218935=CARTESIAN_POINT('Ctrl Pts',(4.05615454399994,15.2,9.60012165499998));
#218936=CARTESIAN_POINT('Ctrl Pts',(4.05615454399994,11.6,9.60012165499998));
#218937=CARTESIAN_POINT('Ctrl Pts',(4.05650092699995,15.2,9.60136689799998));
#218938=CARTESIAN_POINT('Ctrl Pts',(4.05650092699995,11.6,9.60136689799998));
#218939=CARTESIAN_POINT('Ctrl Pts',(4.05684839499994,15.2,9.60262074399999));
#218940=CARTESIAN_POINT('Ctrl Pts',(4.05684839499994,11.6,9.60262074399999));
#218941=CARTESIAN_POINT('Ctrl Pts',(4.05719692999994,15.2,9.60388317399998));
#218942=CARTESIAN_POINT('Ctrl Pts',(4.05719692999994,11.6,9.60388317399998));
#218943=CARTESIAN_POINT('Ctrl Pts',(4.05754650899994,15.2,9.60515417299998));
#218944=CARTESIAN_POINT('Ctrl Pts',(4.05754650899994,11.6,9.60515417299998));
#218945=CARTESIAN_POINT('Ctrl Pts',(4.05789711099994,15.2,9.60643372199998));
#218946=CARTESIAN_POINT('Ctrl Pts',(4.05789711099994,11.6,9.60643372199998));
#218947=CARTESIAN_POINT('Ctrl Pts',(4.05824871699994,15.2,9.60772180699998));
#218948=CARTESIAN_POINT('Ctrl Pts',(4.05824871699994,11.6,9.60772180699998));
#218949=CARTESIAN_POINT('Ctrl Pts',(4.05860130599994,15.2,9.60901840899999));
#218950=CARTESIAN_POINT('Ctrl Pts',(4.05860130599994,11.6,9.60901840899999));
#218951=CARTESIAN_POINT('Ctrl Pts',(4.05895485599994,15.2,9.61032350999999));
#218952=CARTESIAN_POINT('Ctrl Pts',(4.05895485599994,11.6,9.61032350999999));
#218953=CARTESIAN_POINT('Ctrl Pts',(4.05930934899995,15.2,9.61163709599998));
#218954=CARTESIAN_POINT('Ctrl Pts',(4.05930934899995,11.6,9.61163709599998));
#218955=CARTESIAN_POINT('Ctrl Pts',(4.05966476299994,15.2,9.61295914899999));
#218956=CARTESIAN_POINT('Ctrl Pts',(4.05966476299994,11.6,9.61295914899999));
#218957=CARTESIAN_POINT('Ctrl Pts',(4.06002107999995,15.2,9.61428965199998));
#218958=CARTESIAN_POINT('Ctrl Pts',(4.06002107999995,11.6,9.61428965199998));
#218959=CARTESIAN_POINT('Ctrl Pts',(4.06037827899994,15.2,9.61562858999999));
#218960=CARTESIAN_POINT('Ctrl Pts',(4.06037827899994,11.6,9.61562858999999));
#218961=CARTESIAN_POINT('Ctrl Pts',(4.06073633899994,15.2,9.61697594399999));
#218962=CARTESIAN_POINT('Ctrl Pts',(4.06073633899994,11.6,9.61697594399999));
#218963=CARTESIAN_POINT('Ctrl Pts',(4.06109524299994,15.2,9.61833170099998));
#218964=CARTESIAN_POINT('Ctrl Pts',(4.06109524299994,11.6,9.61833170099998));
#218965=CARTESIAN_POINT('Ctrl Pts',(4.06145496899994,15.2,9.61969584099998));
#218966=CARTESIAN_POINT('Ctrl Pts',(4.06145496899994,11.6,9.61969584099998));
#218967=CARTESIAN_POINT('Ctrl Pts',(4.06181549599994,15.2,9.62106834999998));
#218968=CARTESIAN_POINT('Ctrl Pts',(4.06181549599994,11.6,9.62106834999998));
#218969=CARTESIAN_POINT('Ctrl Pts',(4.06217680899995,15.2,9.62244920999998));
#218970=CARTESIAN_POINT('Ctrl Pts',(4.06217680899995,11.6,9.62244920999998));
#218971=CARTESIAN_POINT('Ctrl Pts',(4.06253888499994,15.2,9.62383840699999));
#218972=CARTESIAN_POINT('Ctrl Pts',(4.06253888499994,11.6,9.62383840699999));
#218973=CARTESIAN_POINT('Ctrl Pts',(4.06290170499994,15.2,9.62523592299998));
#218974=CARTESIAN_POINT('Ctrl Pts',(4.06290170499994,11.6,9.62523592299998));
#218975=CARTESIAN_POINT('Ctrl Pts',(4.06326525199994,15.2,9.62664174299999));
#218976=CARTESIAN_POINT('Ctrl Pts',(4.06326525199994,11.6,9.62664174299999));
#218977=CARTESIAN_POINT('Ctrl Pts',(4.06362950399994,15.2,9.62805584999998));
#218978=CARTESIAN_POINT('Ctrl Pts',(4.06362950399994,11.6,9.62805584999998));
#218979=CARTESIAN_POINT('Ctrl Pts',(4.06399444399994,15.2,9.62947822899999));
#218980=CARTESIAN_POINT('Ctrl Pts',(4.06399444399994,11.6,9.62947822899999));
#218981=CARTESIAN_POINT('Ctrl Pts',(4.06436005099994,15.2,9.63090886299998));
#218982=CARTESIAN_POINT('Ctrl Pts',(4.06436005099994,11.6,9.63090886299998));
#218983=CARTESIAN_POINT('Ctrl Pts',(4.06472630999995,15.2,9.63234773599999));
#218984=CARTESIAN_POINT('Ctrl Pts',(4.06472630999995,11.6,9.63234773599999));
#218985=CARTESIAN_POINT('Ctrl Pts',(4.06509319699994,15.2,9.63379483399999));
#218986=CARTESIAN_POINT('Ctrl Pts',(4.06509319699994,11.6,9.63379483399999));
#218987=CARTESIAN_POINT('Ctrl Pts',(4.06546069699994,15.2,9.63525013999998));
#218988=CARTESIAN_POINT('Ctrl Pts',(4.06546069699994,11.6,9.63525013999998));
#218989=CARTESIAN_POINT('Ctrl Pts',(4.06582878999994,15.2,9.63671363799998));
#218990=CARTESIAN_POINT('Ctrl Pts',(4.06582878999994,11.6,9.63671363799998));
#218991=CARTESIAN_POINT('Ctrl Pts',(4.06619745799994,15.2,9.63818531199998));
#218992=CARTESIAN_POINT('Ctrl Pts',(4.06619745799994,11.6,9.63818531199998));
#218993=CARTESIAN_POINT('Ctrl Pts',(4.06656668099994,15.2,9.63966514799999));
#218994=CARTESIAN_POINT('Ctrl Pts',(4.06656668099994,11.6,9.63966514799999));
#218995=CARTESIAN_POINT('Ctrl Pts',(4.06693644299994,15.2,9.64115312899999));
#218996=CARTESIAN_POINT('Ctrl Pts',(4.06693644299994,11.6,9.64115312899999));
#218997=CARTESIAN_POINT('Ctrl Pts',(4.06730672399994,15.2,9.64264924199998));
#218998=CARTESIAN_POINT('Ctrl Pts',(4.06730672399994,11.6,9.64264924199998));
#218999=CARTESIAN_POINT('Ctrl Pts',(4.06767750699994,15.2,9.64415346799999));
#219000=CARTESIAN_POINT('Ctrl Pts',(4.06767750699994,11.6,9.64415346799999));
#219001=CARTESIAN_POINT('Ctrl Pts',(4.06804877199994,15.2,9.64566579199998));
#219002=CARTESIAN_POINT('Ctrl Pts',(4.06804877199994,11.6,9.64566579199998));
#219003=CARTESIAN_POINT('Ctrl Pts',(4.06842050299994,15.2,9.64718620099998));
#219004=CARTESIAN_POINT('Ctrl Pts',(4.06842050299994,11.6,9.64718620099998));
#219005=CARTESIAN_POINT('Ctrl Pts',(4.06879268099994,15.2,9.64871467899999));
#219006=CARTESIAN_POINT('Ctrl Pts',(4.06879268099994,11.6,9.64871467899999));
#219007=CARTESIAN_POINT('Ctrl Pts',(4.06916528699994,15.2,9.65025120999999));
#219008=CARTESIAN_POINT('Ctrl Pts',(4.06916528699994,11.6,9.65025120999999));
#219009=CARTESIAN_POINT('Ctrl Pts',(4.06953830599995,15.2,9.65179577899999));
#219010=CARTESIAN_POINT('Ctrl Pts',(4.06953830599995,11.6,9.65179577899999));
#219011=CARTESIAN_POINT('Ctrl Pts',(4.06991171799994,15.2,9.65334837099999));
#219012=CARTESIAN_POINT('Ctrl Pts',(4.06991171799994,11.6,9.65334837099999));
#219013=CARTESIAN_POINT('Ctrl Pts',(4.07028550499995,15.2,9.65490897099999));
#219014=CARTESIAN_POINT('Ctrl Pts',(4.07028550499995,11.6,9.65490897099999));
#219015=CARTESIAN_POINT('Ctrl Pts',(4.07065965199994,15.2,9.65647756299998));
#219016=CARTESIAN_POINT('Ctrl Pts',(4.07065965199994,11.6,9.65647756299998));
#219017=CARTESIAN_POINT('Ctrl Pts',(4.07103413799994,15.2,9.65805413399998));
#219018=CARTESIAN_POINT('Ctrl Pts',(4.07103413799994,11.6,9.65805413399998));
#219019=CARTESIAN_POINT('Ctrl Pts',(4.07140894899995,15.2,9.65963866699998));
#219020=CARTESIAN_POINT('Ctrl Pts',(4.07140894899995,11.6,9.65963866699998));
#219021=CARTESIAN_POINT('Ctrl Pts',(4.07178406499995,15.2,9.66123114899998));
#219022=CARTESIAN_POINT('Ctrl Pts',(4.07178406499995,11.6,9.66123114899998));
#219023=CARTESIAN_POINT('Ctrl Pts',(4.07215946999994,15.2,9.66283156199999));
#219024=CARTESIAN_POINT('Ctrl Pts',(4.07215946999994,11.6,9.66283156199999));
#219025=CARTESIAN_POINT('Ctrl Pts',(4.07253514699994,15.2,9.66443989599998));
#219026=CARTESIAN_POINT('Ctrl Pts',(4.07253514699994,11.6,9.66443989599998));
#219027=CARTESIAN_POINT('Ctrl Pts',(4.07291107799994,15.2,9.66605613199999));
#219028=CARTESIAN_POINT('Ctrl Pts',(4.07291107799994,11.6,9.66605613199999));
#219029=CARTESIAN_POINT('Ctrl Pts',(4.07328724699994,15.2,9.66768025699999));
#219030=CARTESIAN_POINT('Ctrl Pts',(4.07328724699994,11.6,9.66768025699999));
#219031=CARTESIAN_POINT('Ctrl Pts',(4.07366363499994,15.2,9.66931225599998));
#219032=CARTESIAN_POINT('Ctrl Pts',(4.07366363499994,11.6,9.66931225599998));
#219033=CARTESIAN_POINT('Ctrl Pts',(4.07404022799995,15.2,9.67095211499998));
#219034=CARTESIAN_POINT('Ctrl Pts',(4.07404022799995,11.6,9.67095211499998));
#219035=CARTESIAN_POINT('Ctrl Pts',(4.07441700599994,15.2,9.67259981799998));
#219036=CARTESIAN_POINT('Ctrl Pts',(4.07441700599994,11.6,9.67259981799998));
#219037=CARTESIAN_POINT('Ctrl Pts',(4.07479395499994,15.2,9.67425535199999));
#219038=CARTESIAN_POINT('Ctrl Pts',(4.07479395499994,11.6,9.67425535199999));
#219039=CARTESIAN_POINT('Ctrl Pts',(4.07517105699994,15.2,9.67591870199998));
#219040=CARTESIAN_POINT('Ctrl Pts',(4.07517105699994,11.6,9.67591870199998));
#219041=CARTESIAN_POINT('Ctrl Pts',(4.07554829499994,15.2,9.67758985299999));
#219042=CARTESIAN_POINT('Ctrl Pts',(4.07554829499994,11.6,9.67758985299999));
#219043=CARTESIAN_POINT('Ctrl Pts',(4.07592565399994,15.2,9.67926879099998));
#219044=CARTESIAN_POINT('Ctrl Pts',(4.07592565399994,11.6,9.67926879099998));
#219045=CARTESIAN_POINT('Ctrl Pts',(4.07630311499994,15.2,9.68095550299999));
#219046=CARTESIAN_POINT('Ctrl Pts',(4.07630311499994,11.6,9.68095550299999));
#219047=CARTESIAN_POINT('Ctrl Pts',(4.07668066299994,15.2,9.68264997199999));
#219048=CARTESIAN_POINT('Ctrl Pts',(4.07668066299994,11.6,9.68264997199999));
#219049=CARTESIAN_POINT('Ctrl Pts',(4.07705828299994,15.2,9.68435218599998));
#219050=CARTESIAN_POINT('Ctrl Pts',(4.07705828299994,11.6,9.68435218599998));
#219051=CARTESIAN_POINT('Ctrl Pts',(4.07743595699994,15.2,9.68606212899999));
#219052=CARTESIAN_POINT('Ctrl Pts',(4.07743595699994,11.6,9.68606212899999));
#219053=CARTESIAN_POINT('Ctrl Pts',(4.07781366899994,15.2,9.68777978899999));
#219054=CARTESIAN_POINT('Ctrl Pts',(4.07781366899994,11.6,9.68777978899999));
#219055=CARTESIAN_POINT('Ctrl Pts',(4.07819140299994,15.2,9.68950514999998));
#219056=CARTESIAN_POINT('Ctrl Pts',(4.07819140299994,11.6,9.68950514999998));
#219057=CARTESIAN_POINT('Ctrl Pts',(4.07856914299995,15.2,9.69123819799999));
#219058=CARTESIAN_POINT('Ctrl Pts',(4.07856914299995,11.6,9.69123819799999));
#219059=CARTESIAN_POINT('Ctrl Pts',(4.07894687299994,15.2,9.69297891999998));
#219060=CARTESIAN_POINT('Ctrl Pts',(4.07894687299994,11.6,9.69297891999998));
#219061=CARTESIAN_POINT('Ctrl Pts',(4.07932457699994,15.2,9.69472730199998));
#219062=CARTESIAN_POINT('Ctrl Pts',(4.07932457699994,11.6,9.69472730199998));
#219063=CARTESIAN_POINT('Ctrl Pts',(4.07970223899994,15.2,9.69648332799999));
#219064=CARTESIAN_POINT('Ctrl Pts',(4.07970223899994,11.6,9.69648332799999));
#219065=CARTESIAN_POINT('Ctrl Pts',(4.08007984399995,15.2,9.69824698699998));
#219066=CARTESIAN_POINT('Ctrl Pts',(4.08007984399995,11.6,9.69824698699998));
#219067=CARTESIAN_POINT('Ctrl Pts',(4.08045737499994,15.2,9.70001826299999));
#219068=CARTESIAN_POINT('Ctrl Pts',(4.08045737499994,11.6,9.70001826299999));
#219069=CARTESIAN_POINT('Ctrl Pts',(4.08083481699994,15.2,9.70179714299999));
#219070=CARTESIAN_POINT('Ctrl Pts',(4.08083481699994,11.6,9.70179714299999));
#219071=CARTESIAN_POINT('Ctrl Pts',(4.08121215399994,15.2,9.70358361299999));
#219072=CARTESIAN_POINT('Ctrl Pts',(4.08121215399994,11.6,9.70358361299999));
#219073=CARTESIAN_POINT('Ctrl Pts',(4.08158937099994,15.2,9.70537765899999));
#219074=CARTESIAN_POINT('Ctrl Pts',(4.08158937099994,11.6,9.70537765899999));
#219075=CARTESIAN_POINT('Ctrl Pts',(4.08196645199994,15.2,9.70717926799999));
#219076=CARTESIAN_POINT('Ctrl Pts',(4.08196645199994,11.6,9.70717926799999));
#219077=CARTESIAN_POINT('Ctrl Pts',(4.08234338299994,15.2,9.70898842499999));
#219078=CARTESIAN_POINT('Ctrl Pts',(4.08234338299994,11.6,9.70898842499999));
#219079=CARTESIAN_POINT('Ctrl Pts',(4.08272014699994,15.2,9.71080511799999));
#219080=CARTESIAN_POINT('Ctrl Pts',(4.08272014699994,11.6,9.71080511799999));
#219081=CARTESIAN_POINT('Ctrl Pts',(4.08309672799995,15.2,9.71262933199998));
#219082=CARTESIAN_POINT('Ctrl Pts',(4.08309672799995,11.6,9.71262933199998));
#219083=CARTESIAN_POINT('Ctrl Pts',(4.08347311299995,15.2,9.71446105499999));
#219084=CARTESIAN_POINT('Ctrl Pts',(4.08347311299995,11.6,9.71446105499999));
#219085=CARTESIAN_POINT('Ctrl Pts',(4.08384928499994,15.2,9.71630027099998));
#219086=CARTESIAN_POINT('Ctrl Pts',(4.08384928499994,11.6,9.71630027099998));
#219087=CARTESIAN_POINT('Ctrl Pts',(4.08422522999994,15.2,9.71814696999999));
#219088=CARTESIAN_POINT('Ctrl Pts',(4.08422522999994,11.6,9.71814696999999));
#219089=CARTESIAN_POINT('Ctrl Pts',(4.08460093299994,15.2,9.72000113399999));
#219090=CARTESIAN_POINT('Ctrl Pts',(4.08460093299994,11.6,9.72000113399999));
#219091=CARTESIAN_POINT('Ctrl Pts',(4.08497637899994,15.2,9.72186275399999));
#219092=CARTESIAN_POINT('Ctrl Pts',(4.08497637899994,11.6,9.72186275399999));
#219093=CARTESIAN_POINT('Ctrl Pts',(4.08535155199994,15.2,9.72373181399998));
#219094=CARTESIAN_POINT('Ctrl Pts',(4.08535155199994,11.6,9.72373181399998));
#219095=CARTESIAN_POINT('Ctrl Pts',(4.08572643699994,15.2,9.72560830099999));
#219096=CARTESIAN_POINT('Ctrl Pts',(4.08572643699994,11.6,9.72560830099999));
#219097=CARTESIAN_POINT('Ctrl Pts',(4.08610102099995,15.2,9.72749220299999));
#219098=CARTESIAN_POINT('Ctrl Pts',(4.08610102099995,11.6,9.72749220299999));
#219099=CARTESIAN_POINT('Ctrl Pts',(4.08647528899994,15.2,9.72938350599998));
#219100=CARTESIAN_POINT('Ctrl Pts',(4.08647528899994,11.6,9.72938350599998));
#219101=CARTESIAN_POINT('Ctrl Pts',(4.08684922499994,15.2,9.73128219599998));
#219102=CARTESIAN_POINT('Ctrl Pts',(4.08684922499994,11.6,9.73128219599998));
#219103=CARTESIAN_POINT('Ctrl Pts',(4.08722281399994,15.2,9.73318826099998));
#219104=CARTESIAN_POINT('Ctrl Pts',(4.08722281399994,11.6,9.73318826099998));
#219105=CARTESIAN_POINT('Ctrl Pts',(4.08759604299994,15.2,9.73510168599999));
#219106=CARTESIAN_POINT('Ctrl Pts',(4.08759604299994,11.6,9.73510168599999));
#219107=CARTESIAN_POINT('Ctrl Pts',(4.08796889599994,15.2,9.73702245899998));
#219108=CARTESIAN_POINT('Ctrl Pts',(4.08796889599994,11.6,9.73702245899998));
#219109=CARTESIAN_POINT('Ctrl Pts',(4.08834136099994,15.2,9.73895056799999));
#219110=CARTESIAN_POINT('Ctrl Pts',(4.08834136099994,11.6,9.73895056799999));
#219111=CARTESIAN_POINT('Ctrl Pts',(4.08871342099994,15.2,9.74088599899999));
#219112=CARTESIAN_POINT('Ctrl Pts',(4.08871342099994,11.6,9.74088599899999));
#219113=CARTESIAN_POINT('Ctrl Pts',(4.08908506299994,15.2,9.74282873799999));
#219114=CARTESIAN_POINT('Ctrl Pts',(4.08908506299994,11.6,9.74282873799999));
#219115=CARTESIAN_POINT('Ctrl Pts',(4.08945627199994,15.2,9.74477877499999));
#219116=CARTESIAN_POINT('Ctrl Pts',(4.08945627199994,11.6,9.74477877499999));
#219117=CARTESIAN_POINT('Ctrl Pts',(4.08982703399994,15.2,9.74673609299998));
#219118=CARTESIAN_POINT('Ctrl Pts',(4.08982703399994,11.6,9.74673609299998));
#219119=CARTESIAN_POINT('Ctrl Pts',(4.09019733499994,15.2,9.74870068099998));
#219120=CARTESIAN_POINT('Ctrl Pts',(4.09019733499994,11.6,9.74870068099998));
#219121=CARTESIAN_POINT('Ctrl Pts',(4.09056716099994,15.2,9.75067252799998));
#219122=CARTESIAN_POINT('Ctrl Pts',(4.09056716099994,11.6,9.75067252799998));
#219123=CARTESIAN_POINT('Ctrl Pts',(4.09093649799994,15.2,9.75265161799998));
#219124=CARTESIAN_POINT('Ctrl Pts',(4.09093649799994,11.6,9.75265161799998));
#219125=CARTESIAN_POINT('Ctrl Pts',(4.09130533199995,15.2,9.75463793999998));
#219126=CARTESIAN_POINT('Ctrl Pts',(4.09130533199995,11.6,9.75463793999998));
#219127=CARTESIAN_POINT('Ctrl Pts',(4.09167364799994,15.2,9.75663148099999));
#219128=CARTESIAN_POINT('Ctrl Pts',(4.09167364799994,11.6,9.75663148099999));
#219129=CARTESIAN_POINT('Ctrl Pts',(4.09204143299995,15.2,9.75863222699999));
#219130=CARTESIAN_POINT('Ctrl Pts',(4.09204143299995,11.6,9.75863222699999));
#219131=CARTESIAN_POINT('Ctrl Pts',(4.09240867299994,15.2,9.76064016799998));
#219132=CARTESIAN_POINT('Ctrl Pts',(4.09240867299994,11.6,9.76064016799998));
#219133=CARTESIAN_POINT('Ctrl Pts',(4.09277535499994,15.2,9.76265528899999));
#219134=CARTESIAN_POINT('Ctrl Pts',(4.09277535499994,11.6,9.76265528899999));
#219135=CARTESIAN_POINT('Ctrl Pts',(4.09314146399994,15.2,9.76467757799998));
#219136=CARTESIAN_POINT('Ctrl Pts',(4.09314146399994,11.6,9.76467757799998));
#219137=CARTESIAN_POINT('Ctrl Pts',(4.09350698699994,15.2,9.76670702199998));
#219138=CARTESIAN_POINT('Ctrl Pts',(4.09350698699994,11.6,9.76670702199998));
#219139=CARTESIAN_POINT('Ctrl Pts',(4.09387190999994,15.2,9.76874360899998));
#219140=CARTESIAN_POINT('Ctrl Pts',(4.09387190999994,11.6,9.76874360899998));
#219141=CARTESIAN_POINT('Ctrl Pts',(4.09423621899994,15.2,9.77078732699999));
#219142=CARTESIAN_POINT('Ctrl Pts',(4.09423621899994,11.6,9.77078732699999));
#219143=CARTESIAN_POINT('Ctrl Pts',(4.09459990199994,15.2,9.77283816299998));
#219144=CARTESIAN_POINT('Ctrl Pts',(4.09459990199994,11.6,9.77283816299998));
#219145=CARTESIAN_POINT('Ctrl Pts',(4.09496294399994,15.2,9.77489610299998));
#219146=CARTESIAN_POINT('Ctrl Pts',(4.09496294399994,11.6,9.77489610299998));
#219147=CARTESIAN_POINT('Ctrl Pts',(4.09532533299994,15.2,9.77696113599999));
#219148=CARTESIAN_POINT('Ctrl Pts',(4.09532533299994,11.6,9.77696113599999));
#219149=CARTESIAN_POINT('Ctrl Pts',(4.09568705399994,15.2,9.77903324999998));
#219150=CARTESIAN_POINT('Ctrl Pts',(4.09568705399994,11.6,9.77903324999998));
#219151=CARTESIAN_POINT('Ctrl Pts',(4.09604809499994,15.2,9.78111243199999));
#219152=CARTESIAN_POINT('Ctrl Pts',(4.09604809499994,11.6,9.78111243199999));
#219153=CARTESIAN_POINT('Ctrl Pts',(4.09640844199994,15.2,9.78319866999998));
#219154=CARTESIAN_POINT('Ctrl Pts',(4.09640844199994,11.6,9.78319866999998));
#219155=CARTESIAN_POINT('Ctrl Pts',(4.09676808199994,15.2,9.78529195099998));
#219156=CARTESIAN_POINT('Ctrl Pts',(4.09676808199994,11.6,9.78529195099998));
#219157=CARTESIAN_POINT('Ctrl Pts',(4.09712700199994,15.2,9.78739226399998));
#219158=CARTESIAN_POINT('Ctrl Pts',(4.09712700199994,11.6,9.78739226399998));
#219159=CARTESIAN_POINT('Ctrl Pts',(4.09748518799994,15.2,9.78949959399999));
#219160=CARTESIAN_POINT('Ctrl Pts',(4.09748518799994,11.6,9.78949959399999));
#219161=CARTESIAN_POINT('Ctrl Pts',(4.09784262799994,15.2,9.79161393199998));
#219162=CARTESIAN_POINT('Ctrl Pts',(4.09784262799994,11.6,9.79161393199998));
#219163=CARTESIAN_POINT('Ctrl Pts',(4.09819930899994,15.2,9.79373526399998));
#219164=CARTESIAN_POINT('Ctrl Pts',(4.09819930899994,11.6,9.79373526399998));
#219165=CARTESIAN_POINT('Ctrl Pts',(4.09855521699994,15.2,9.79586357899999));
#219166=CARTESIAN_POINT('Ctrl Pts',(4.09855521699994,11.6,9.79586357899999));
#219167=CARTESIAN_POINT('Ctrl Pts',(4.09891033999994,15.2,9.79799886199999));
#219168=CARTESIAN_POINT('Ctrl Pts',(4.09891033999994,11.6,9.79799886199999));
#219169=CARTESIAN_POINT('Ctrl Pts',(4.09926466499994,15.2,9.80014110499998));
#219170=CARTESIAN_POINT('Ctrl Pts',(4.09926466499994,11.6,9.80014110499998));
#219171=CARTESIAN_POINT('Ctrl Pts',(4.09961817899995,15.2,9.80229029299998));
#219172=CARTESIAN_POINT('Ctrl Pts',(4.09961817899995,11.6,9.80229029299998));
#219173=CARTESIAN_POINT('Ctrl Pts',(4.09997086899994,15.2,9.80444641499999));
#219174=CARTESIAN_POINT('Ctrl Pts',(4.09997086899994,11.6,9.80444641499999));
#219175=CARTESIAN_POINT('Ctrl Pts',(4.10032272299994,15.2,9.80660945799999));
#219176=CARTESIAN_POINT('Ctrl Pts',(4.10032272299994,11.6,9.80660945799999));
#219177=CARTESIAN_POINT('Ctrl Pts',(4.10067372699995,15.2,9.80877941199999));
#219178=CARTESIAN_POINT('Ctrl Pts',(4.10067372699995,11.6,9.80877941199999));
#219179=CARTESIAN_POINT('Ctrl Pts',(4.10102386899994,15.2,9.81095626399998));
#219180=CARTESIAN_POINT('Ctrl Pts',(4.10102386899994,11.6,9.81095626399998));
#219181=CARTESIAN_POINT('Ctrl Pts',(4.10137313699994,15.2,9.81314000099999));
#219182=CARTESIAN_POINT('Ctrl Pts',(4.10137313699994,11.6,9.81314000099999));
#219183=CARTESIAN_POINT('Ctrl Pts',(4.10172151799994,15.2,9.81533061199999));
#219184=CARTESIAN_POINT('Ctrl Pts',(4.10172151799994,11.6,9.81533061199999));
#219185=CARTESIAN_POINT('Ctrl Pts',(4.10206899999995,15.2,9.81752808499999));
#219186=CARTESIAN_POINT('Ctrl Pts',(4.10206899999995,11.6,9.81752808499999));
#219187=CARTESIAN_POINT('Ctrl Pts',(4.10241556999994,15.2,9.81973240899999));
#219188=CARTESIAN_POINT('Ctrl Pts',(4.10241556999994,11.6,9.81973240899999));
#219189=CARTESIAN_POINT('Ctrl Pts',(4.10276121599995,15.2,9.82194357099999));
#219190=CARTESIAN_POINT('Ctrl Pts',(4.10276121599995,11.6,9.82194357099999));
#219191=CARTESIAN_POINT('Ctrl Pts',(4.10310592399994,15.2,9.82416155899998));
#219192=CARTESIAN_POINT('Ctrl Pts',(4.10310592399994,11.6,9.82416155899998));
#219193=CARTESIAN_POINT('Ctrl Pts',(4.10344968399994,15.2,9.82638636299999));
#219194=CARTESIAN_POINT('Ctrl Pts',(4.10344968399994,11.6,9.82638636299999));
#219195=CARTESIAN_POINT('Ctrl Pts',(4.10379248299995,15.2,9.82861796999998));
#219196=CARTESIAN_POINT('Ctrl Pts',(4.10379248299995,11.6,9.82861796999998));
#219197=CARTESIAN_POINT('Ctrl Pts',(4.10413430799994,15.2,9.83085636799998));
#219198=CARTESIAN_POINT('Ctrl Pts',(4.10413430799994,11.6,9.83085636799998));
#219199=CARTESIAN_POINT('Ctrl Pts',(4.10447514699994,15.2,9.83310154499998));
#219200=CARTESIAN_POINT('Ctrl Pts',(4.10447514699994,11.6,9.83310154499998));
#219201=CARTESIAN_POINT('Ctrl Pts',(4.10481498799994,15.2,9.83535349199999));
#219202=CARTESIAN_POINT('Ctrl Pts',(4.10481498799994,11.6,9.83535349199999));
#219203=CARTESIAN_POINT('Ctrl Pts',(4.10515382099994,15.2,9.83761219399998));
#219204=CARTESIAN_POINT('Ctrl Pts',(4.10515382099994,11.6,9.83761219399998));
#219205=CARTESIAN_POINT('Ctrl Pts',(4.10549163099994,15.2,9.83987764099999));
#219206=CARTESIAN_POINT('Ctrl Pts',(4.10549163099994,11.6,9.83987764099999));
#219207=CARTESIAN_POINT('Ctrl Pts',(4.10582840599994,15.2,9.84214982099999));
#219208=CARTESIAN_POINT('Ctrl Pts',(4.10582840599994,11.6,9.84214982099999));
#219209=CARTESIAN_POINT('Ctrl Pts',(4.10616413599994,15.2,9.84442872299999));
#219210=CARTESIAN_POINT('Ctrl Pts',(4.10616413599994,11.6,9.84442872299999));
#219211=CARTESIAN_POINT('Ctrl Pts',(4.10649880899994,15.2,9.84671433499998));
#219212=CARTESIAN_POINT('Ctrl Pts',(4.10649880899994,11.6,9.84671433499998));
#219213=CARTESIAN_POINT('Ctrl Pts',(4.10683241099994,15.2,9.84900664599999));
#219214=CARTESIAN_POINT('Ctrl Pts',(4.10683241099994,11.6,9.84900664599999));
#219215=CARTESIAN_POINT('Ctrl Pts',(4.10716493199994,15.2,9.85130564399999));
#219216=CARTESIAN_POINT('Ctrl Pts',(4.10716493199994,11.6,9.85130564399999));
#219217=CARTESIAN_POINT('Ctrl Pts',(4.10749635899994,15.2,9.85361131699998));
#219218=CARTESIAN_POINT('Ctrl Pts',(4.10749635899994,11.6,9.85361131699998));
#219219=CARTESIAN_POINT('Ctrl Pts',(4.10782668199994,15.2,9.85592365499999));
#219220=CARTESIAN_POINT('Ctrl Pts',(4.10782668199994,11.6,9.85592365499999));
#219221=CARTESIAN_POINT('Ctrl Pts',(4.10815588799994,15.2,9.85824264699998));
#219222=CARTESIAN_POINT('Ctrl Pts',(4.10815588799994,11.6,9.85824264699998));
#219223=CARTESIAN_POINT('Ctrl Pts',(4.10848396599994,15.2,9.86056827999998));
#219224=CARTESIAN_POINT('Ctrl Pts',(4.10848396599994,11.6,9.86056827999998));
#219225=CARTESIAN_POINT('Ctrl Pts',(4.10881090399995,15.2,9.86290054199999));
#219226=CARTESIAN_POINT('Ctrl Pts',(4.10881090399995,11.6,9.86290054199999));
#219227=CARTESIAN_POINT('Ctrl Pts',(4.10913668999994,15.2,9.86523942399998));
#219228=CARTESIAN_POINT('Ctrl Pts',(4.10913668999994,11.6,9.86523942399998));
#219229=CARTESIAN_POINT('Ctrl Pts',(4.10946131299994,15.2,9.86758491299998));
#219230=CARTESIAN_POINT('Ctrl Pts',(4.10946131299994,11.6,9.86758491299998));
#219231=CARTESIAN_POINT('Ctrl Pts',(4.10978476099995,15.2,9.86993699799999));
#219232=CARTESIAN_POINT('Ctrl Pts',(4.10978476099995,11.6,9.86993699799999));
#219233=CARTESIAN_POINT('Ctrl Pts',(4.11010702299994,15.2,9.87229566899998));
#219234=CARTESIAN_POINT('Ctrl Pts',(4.11010702299994,11.6,9.87229566899998));
#219235=CARTESIAN_POINT('Ctrl Pts',(4.11042808799994,15.2,9.87466091399998));
#219236=CARTESIAN_POINT('Ctrl Pts',(4.11042808799994,11.6,9.87466091399998));
#219237=CARTESIAN_POINT('Ctrl Pts',(4.11074794399994,15.2,9.87703271999998));
#219238=CARTESIAN_POINT('Ctrl Pts',(4.11074794399994,11.6,9.87703271999998));
#219239=CARTESIAN_POINT('Ctrl Pts',(4.11106657999994,15.2,9.87941107899999));
#219240=CARTESIAN_POINT('Ctrl Pts',(4.11106657999994,11.6,9.87941107899999));
#219241=CARTESIAN_POINT('Ctrl Pts',(4.11138398399994,15.2,9.88179597699999));
#219242=CARTESIAN_POINT('Ctrl Pts',(4.11138398399994,11.6,9.88179597699999));
#219243=CARTESIAN_POINT('Ctrl Pts',(4.11170014699994,15.2,9.88418740499998));
#219244=CARTESIAN_POINT('Ctrl Pts',(4.11170014699994,11.6,9.88418740499998));
#219245=CARTESIAN_POINT('Ctrl Pts',(4.11201505399994,15.2,9.88658535199999));
#219246=CARTESIAN_POINT('Ctrl Pts',(4.11201505399994,11.6,9.88658535199999));
#219247=CARTESIAN_POINT('Ctrl Pts',(4.11232869799994,15.2,9.88898980399998));
#219248=CARTESIAN_POINT('Ctrl Pts',(4.11232869799994,11.6,9.88898980399998));
#219249=CARTESIAN_POINT('Ctrl Pts',(4.11264106399994,15.2,9.89140075399998));
#219250=CARTESIAN_POINT('Ctrl Pts',(4.11264106399994,11.6,9.89140075399998));
#219251=CARTESIAN_POINT('Ctrl Pts',(4.11295214299995,15.2,9.89381818699999));
#219252=CARTESIAN_POINT('Ctrl Pts',(4.11295214299995,11.6,9.89381818699999));
#219253=CARTESIAN_POINT('Ctrl Pts',(4.11326192499994,15.2,9.89624209499999));
#219254=CARTESIAN_POINT('Ctrl Pts',(4.11326192499994,11.6,9.89624209499999));
#219255=CARTESIAN_POINT('Ctrl Pts',(4.11357039599995,15.2,9.89867246599999));
#219256=CARTESIAN_POINT('Ctrl Pts',(4.11357039599995,11.6,9.89867246599999));
#219257=CARTESIAN_POINT('Ctrl Pts',(4.11387754699994,15.2,9.90110928899998));
#219258=CARTESIAN_POINT('Ctrl Pts',(4.11387754699994,11.6,9.90110928899998));
#219259=CARTESIAN_POINT('Ctrl Pts',(4.11418336699994,15.2,9.90355255299999));
#219260=CARTESIAN_POINT('Ctrl Pts',(4.11418336699994,11.6,9.90355255299999));
#219261=CARTESIAN_POINT('Ctrl Pts',(4.11448784499994,15.2,9.90600224699998));
#219262=CARTESIAN_POINT('Ctrl Pts',(4.11448784499994,11.6,9.90600224699998));
#219263=CARTESIAN_POINT('Ctrl Pts',(4.11479096999994,15.2,9.90845835999998));
#219264=CARTESIAN_POINT('Ctrl Pts',(4.11479096999994,11.6,9.90845835999998));
#219265=CARTESIAN_POINT('Ctrl Pts',(4.11509273099994,15.2,9.91092088199998));
#219266=CARTESIAN_POINT('Ctrl Pts',(4.11509273099994,11.6,9.91092088199998));
#219267=CARTESIAN_POINT('Ctrl Pts',(4.11539311699994,15.2,9.91338979999998));
#219268=CARTESIAN_POINT('Ctrl Pts',(4.11539311699994,11.6,9.91338979999998));
#219269=CARTESIAN_POINT('Ctrl Pts',(4.11569211799994,15.2,9.91586510699998));
#219270=CARTESIAN_POINT('Ctrl Pts',(4.11569211799994,11.6,9.91586510699998));
#219271=CARTESIAN_POINT('Ctrl Pts',(4.11598972299995,15.2,9.91834678799999));
#219272=CARTESIAN_POINT('Ctrl Pts',(4.11598972299995,11.6,9.91834678799999));
#219273=CARTESIAN_POINT('Ctrl Pts',(4.11628592199994,15.2,9.92083483499999));
#219274=CARTESIAN_POINT('Ctrl Pts',(4.11628592199994,11.6,9.92083483499999));
#219275=CARTESIAN_POINT('Ctrl Pts',(4.11658070199994,15.2,9.92332923599999));
#219276=CARTESIAN_POINT('Ctrl Pts',(4.11658070199994,11.6,9.92332923599999));
#219277=CARTESIAN_POINT('Ctrl Pts',(4.11687405499995,15.2,9.92582998099999));
#219278=CARTESIAN_POINT('Ctrl Pts',(4.11687405499995,11.6,9.92582998099999));
#219279=CARTESIAN_POINT('Ctrl Pts',(4.11716596799994,15.2,9.92833705899999));
#219280=CARTESIAN_POINT('Ctrl Pts',(4.11716596799994,11.6,9.92833705899999));
#219281=CARTESIAN_POINT('Ctrl Pts',(4.11745643399995,15.2,9.93085045899999));
#219282=CARTESIAN_POINT('Ctrl Pts',(4.11745643399995,11.6,9.93085045899999));
#219283=CARTESIAN_POINT('Ctrl Pts',(4.11774543899995,15.2,9.93337017099999));
#219284=CARTESIAN_POINT('Ctrl Pts',(4.11774543899995,11.6,9.93337017099999));
#219285=CARTESIAN_POINT('Ctrl Pts',(4.11803297499994,15.2,9.93589618299998));
#219286=CARTESIAN_POINT('Ctrl Pts',(4.11803297499994,11.6,9.93589618299998));
#219287=CARTESIAN_POINT('Ctrl Pts',(4.11831903099994,15.2,9.93842848499998));
#219288=CARTESIAN_POINT('Ctrl Pts',(4.11831903099994,11.6,9.93842848499998));
#219289=CARTESIAN_POINT('Ctrl Pts',(4.11860359399994,15.2,9.94096706799999));
#219290=CARTESIAN_POINT('Ctrl Pts',(4.11860359399994,11.6,9.94096706799999));
#219291=CARTESIAN_POINT('Ctrl Pts',(4.11888665799994,15.2,9.94351191999998));
#219292=CARTESIAN_POINT('Ctrl Pts',(4.11888665799994,11.6,9.94351191999998));
#219293=CARTESIAN_POINT('Ctrl Pts',(4.11916820899994,15.2,9.94606302999999));
#219294=CARTESIAN_POINT('Ctrl Pts',(4.11916820899994,11.6,9.94606302999999));
#219295=CARTESIAN_POINT('Ctrl Pts',(4.11944823799994,15.2,9.94862038699999));
#219296=CARTESIAN_POINT('Ctrl Pts',(4.11944823799994,11.6,9.94862038699999));
#219297=CARTESIAN_POINT('Ctrl Pts',(4.11972673699994,15.2,9.95118398199999));
#219298=CARTESIAN_POINT('Ctrl Pts',(4.11972673699994,11.6,9.95118398199999));
#219299=CARTESIAN_POINT('Ctrl Pts',(4.12000369199994,15.2,9.95375380499999));
#219300=CARTESIAN_POINT('Ctrl Pts',(4.12000369199994,11.6,9.95375380499999));
#219301=CARTESIAN_POINT('Ctrl Pts',(4.12027909599994,15.2,9.95632984399998));
#219302=CARTESIAN_POINT('Ctrl Pts',(4.12027909599994,11.6,9.95632984399998));
#219303=CARTESIAN_POINT('Ctrl Pts',(4.12055293699995,15.2,9.95891208799998));
#219304=CARTESIAN_POINT('Ctrl Pts',(4.12055293699995,11.6,9.95891208799998));
#219305=CARTESIAN_POINT('Ctrl Pts',(4.12082520399994,15.2,9.96150052899999));
#219306=CARTESIAN_POINT('Ctrl Pts',(4.12082520399994,11.6,9.96150052899999));
#219307=CARTESIAN_POINT('Ctrl Pts',(4.12109588999995,15.2,9.96409515399998));
#219308=CARTESIAN_POINT('Ctrl Pts',(4.12109588999995,11.6,9.96409515399998));
#219309=CARTESIAN_POINT('Ctrl Pts',(4.12136498299995,15.2,9.96669595499998));
#219310=CARTESIAN_POINT('Ctrl Pts',(4.12136498299995,11.6,9.96669595499998));
#219311=CARTESIAN_POINT('Ctrl Pts',(4.12163247299994,15.2,9.96930291999998));
#219312=CARTESIAN_POINT('Ctrl Pts',(4.12163247299994,11.6,9.96930291999998));
#219313=CARTESIAN_POINT('Ctrl Pts',(4.12189834999994,15.2,9.97191603899999));
#219314=CARTESIAN_POINT('Ctrl Pts',(4.12189834999994,11.6,9.97191603899999));
#219315=CARTESIAN_POINT('Ctrl Pts',(4.12216260499994,15.2,9.97453530099998));
#219316=CARTESIAN_POINT('Ctrl Pts',(4.12216260499994,11.6,9.97453530099998));
#219317=CARTESIAN_POINT('Ctrl Pts',(4.12242522799994,15.2,9.97716069699998));
#219318=CARTESIAN_POINT('Ctrl Pts',(4.12242522799994,11.6,9.97716069699998));
#219319=CARTESIAN_POINT('Ctrl Pts',(4.12268620699995,15.2,9.97979221699998));
#219320=CARTESIAN_POINT('Ctrl Pts',(4.12268620699995,11.6,9.97979221699998));
#219321=CARTESIAN_POINT('Ctrl Pts',(4.12294553499994,15.2,9.98242984899999));
#219322=CARTESIAN_POINT('Ctrl Pts',(4.12294553499994,11.6,9.98242984899999));
#219323=CARTESIAN_POINT('Ctrl Pts',(4.12320319999994,15.2,9.98507358299998));
#219324=CARTESIAN_POINT('Ctrl Pts',(4.12320319999994,11.6,9.98507358299998));
#219325=CARTESIAN_POINT('Ctrl Pts',(4.12345919399994,15.2,9.98772340999999));
#219326=CARTESIAN_POINT('Ctrl Pts',(4.12345919399994,11.6,9.98772340999999));
#219327=CARTESIAN_POINT('Ctrl Pts',(4.12371350699994,15.2,9.99037931899998));
#219328=CARTESIAN_POINT('Ctrl Pts',(4.12371350699994,11.6,9.99037931899998));
#219329=CARTESIAN_POINT('Ctrl Pts',(4.12396612799994,15.2,9.99304129999998));
#219330=CARTESIAN_POINT('Ctrl Pts',(4.12396612799994,11.6,9.99304129999998));
#219331=CARTESIAN_POINT('Ctrl Pts',(4.12421704799994,15.2,9.99570934199999));
#219332=CARTESIAN_POINT('Ctrl Pts',(4.12421704799994,11.6,9.99570934199999));
#219333=CARTESIAN_POINT('Ctrl Pts',(4.12446625799994,15.2,9.99838343599999));
#219334=CARTESIAN_POINT('Ctrl Pts',(4.12446625799994,11.6,9.99838343599999));
#219335=CARTESIAN_POINT('Ctrl Pts',(4.12471374799994,15.2,10.001063571));
#219336=CARTESIAN_POINT('Ctrl Pts',(4.12471374799994,11.6,10.001063571));
#219337=CARTESIAN_POINT('Ctrl Pts',(4.12495950799994,15.2,10.003749739));
#219338=CARTESIAN_POINT('Ctrl Pts',(4.12495950799994,11.6,10.003749739));
#219339=CARTESIAN_POINT('Ctrl Pts',(4.12520352799994,15.2,10.006441926));
#219340=CARTESIAN_POINT('Ctrl Pts',(4.12520352799994,11.6,10.006441926));
#219341=CARTESIAN_POINT('Ctrl Pts',(4.12544579999994,15.2,10.009140125));
#219342=CARTESIAN_POINT('Ctrl Pts',(4.12544579999994,11.6,10.009140125));
#219343=CARTESIAN_POINT('Ctrl Pts',(4.12568631399994,15.2,10.011844325));
#219344=CARTESIAN_POINT('Ctrl Pts',(4.12568631399994,11.6,10.011844325));
#219345=CARTESIAN_POINT('Ctrl Pts',(4.12592505999995,15.2,10.014554516));
#219346=CARTESIAN_POINT('Ctrl Pts',(4.12592505999995,11.6,10.014554516));
#219347=CARTESIAN_POINT('Ctrl Pts',(4.12616202899994,15.2,10.017270688));
#219348=CARTESIAN_POINT('Ctrl Pts',(4.12616202899994,11.6,10.017270688));
#219349=CARTESIAN_POINT('Ctrl Pts',(4.12639721099994,15.2,10.01999283));
#219350=CARTESIAN_POINT('Ctrl Pts',(4.12639721099994,11.6,10.01999283));
#219351=CARTESIAN_POINT('Ctrl Pts',(4.12663059799994,15.2,10.022720935));
#219352=CARTESIAN_POINT('Ctrl Pts',(4.12663059799994,11.6,10.022720935));
#219353=CARTESIAN_POINT('Ctrl Pts',(4.12686217999994,15.2,10.02545499));
#219354=CARTESIAN_POINT('Ctrl Pts',(4.12686217999994,11.6,10.02545499));
#219355=CARTESIAN_POINT('Ctrl Pts',(4.12709194699994,15.2,10.028194985));
#219356=CARTESIAN_POINT('Ctrl Pts',(4.12709194699994,11.6,10.028194985));
#219357=CARTESIAN_POINT('Ctrl Pts',(4.12731988999994,15.2,10.030940912));
#219358=CARTESIAN_POINT('Ctrl Pts',(4.12731988999994,11.6,10.030940912));
#219359=CARTESIAN_POINT('Ctrl Pts',(4.12754600099994,15.2,10.03369276));
#219360=CARTESIAN_POINT('Ctrl Pts',(4.12754600099994,11.6,10.03369276));
#219361=CARTESIAN_POINT('Ctrl Pts',(4.12777026999995,15.2,10.03645052));
#219362=CARTESIAN_POINT('Ctrl Pts',(4.12777026999995,11.6,10.03645052));
#219363=CARTESIAN_POINT('Ctrl Pts',(4.12799268599994,15.2,10.03921418));
#219364=CARTESIAN_POINT('Ctrl Pts',(4.12799268599994,11.6,10.03921418));
#219365=CARTESIAN_POINT('Ctrl Pts',(4.12821324299994,15.2,10.041983733));
#219366=CARTESIAN_POINT('Ctrl Pts',(4.12821324299994,11.6,10.041983733));
#219367=CARTESIAN_POINT('Ctrl Pts',(4.12843192999994,15.2,10.044759166));
#219368=CARTESIAN_POINT('Ctrl Pts',(4.12843192999994,11.6,10.044759166));
#219369=CARTESIAN_POINT('Ctrl Pts',(4.12864873899994,15.2,10.047540472));
#219370=CARTESIAN_POINT('Ctrl Pts',(4.12864873899994,11.6,10.047540472));
#219371=CARTESIAN_POINT('Ctrl Pts',(4.12886365999994,15.2,10.050327639));
#219372=CARTESIAN_POINT('Ctrl Pts',(4.12886365999994,11.6,10.050327639));
#219373=CARTESIAN_POINT('Ctrl Pts',(4.12907668299995,15.2,10.053120659));
#219374=CARTESIAN_POINT('Ctrl Pts',(4.12907668299995,11.6,10.053120659));
#219375=CARTESIAN_POINT('Ctrl Pts',(4.12928780099994,15.2,10.055919521));
#219376=CARTESIAN_POINT('Ctrl Pts',(4.12928780099994,11.6,10.055919521));
#219377=CARTESIAN_POINT('Ctrl Pts',(4.12949700599994,15.2,10.058724216));
#219378=CARTESIAN_POINT('Ctrl Pts',(4.12949700599994,11.6,10.058724216));
#219379=CARTESIAN_POINT('Ctrl Pts',(4.12970428599994,15.2,10.061534734));
#219380=CARTESIAN_POINT('Ctrl Pts',(4.12970428599994,11.6,10.061534734));
#219381=CARTESIAN_POINT('Ctrl Pts',(4.12990963199994,15.2,10.064351065));
#219382=CARTESIAN_POINT('Ctrl Pts',(4.12990963199994,11.6,10.064351065));
#219383=CARTESIAN_POINT('Ctrl Pts',(4.13011303899994,15.2,10.067173199));
#219384=CARTESIAN_POINT('Ctrl Pts',(4.13011303899994,11.6,10.067173199));
#219385=CARTESIAN_POINT('Ctrl Pts',(4.13031449499994,15.2,10.070001128));
#219386=CARTESIAN_POINT('Ctrl Pts',(4.13031449499994,11.6,10.070001128));
#219387=CARTESIAN_POINT('Ctrl Pts',(4.13051399199994,15.2,10.072834839));
#219388=CARTESIAN_POINT('Ctrl Pts',(4.13051399199994,11.6,10.072834839));
#219389=CARTESIAN_POINT('Ctrl Pts',(4.13071152099994,15.2,10.075674326));
#219390=CARTESIAN_POINT('Ctrl Pts',(4.13071152099994,11.6,10.075674326));
#219391=CARTESIAN_POINT('Ctrl Pts',(4.13090707399994,15.2,10.078519578));
#219392=CARTESIAN_POINT('Ctrl Pts',(4.13090707399994,11.6,10.078519578));
#219393=CARTESIAN_POINT('Ctrl Pts',(4.13110064099994,15.2,10.081370584));
#219394=CARTESIAN_POINT('Ctrl Pts',(4.13110064099994,11.6,10.081370584));
#219395=CARTESIAN_POINT('Ctrl Pts',(4.13129221399995,15.2,10.084227337));
#219396=CARTESIAN_POINT('Ctrl Pts',(4.13129221399995,11.6,10.084227337));
#219397=CARTESIAN_POINT('Ctrl Pts',(4.13148178399994,15.2,10.087089825));
#219398=CARTESIAN_POINT('Ctrl Pts',(4.13148178399994,11.6,10.087089825));
#219399=CARTESIAN_POINT('Ctrl Pts',(4.13166934299994,15.2,10.089958039));
#219400=CARTESIAN_POINT('Ctrl Pts',(4.13166934299994,11.6,10.089958039));
#219401=CARTESIAN_POINT('Ctrl Pts',(4.13185488199994,15.2,10.09283197));
#219402=CARTESIAN_POINT('Ctrl Pts',(4.13185488199994,11.6,10.09283197));
#219403=CARTESIAN_POINT('Ctrl Pts',(4.13203839299995,15.2,10.095711608));
#219404=CARTESIAN_POINT('Ctrl Pts',(4.13203839299995,11.6,10.095711608));
#219405=CARTESIAN_POINT('Ctrl Pts',(4.13221986599994,15.2,10.098596945));
#219406=CARTESIAN_POINT('Ctrl Pts',(4.13221986599994,11.6,10.098596945));
#219407=CARTESIAN_POINT('Ctrl Pts',(4.13239929399994,15.2,10.101487969));
#219408=CARTESIAN_POINT('Ctrl Pts',(4.13239929399994,11.6,10.101487969));
#219409=CARTESIAN_POINT('Ctrl Pts',(4.13257666799994,15.2,10.104384672));
#219410=CARTESIAN_POINT('Ctrl Pts',(4.13257666799994,11.6,10.104384672));
#219411=CARTESIAN_POINT('Ctrl Pts',(4.13275197799994,15.2,10.107287045));
#219412=CARTESIAN_POINT('Ctrl Pts',(4.13275197799994,11.6,10.107287045));
#219413=CARTESIAN_POINT('Ctrl Pts',(4.13292521699994,15.2,10.110195076));
#219414=CARTESIAN_POINT('Ctrl Pts',(4.13292521699994,11.6,10.110195076));
#219415=CARTESIAN_POINT('Ctrl Pts',(4.13309637699994,15.2,10.113108759));
#219416=CARTESIAN_POINT('Ctrl Pts',(4.13309637699994,11.6,10.113108759));
#219417=CARTESIAN_POINT('Ctrl Pts',(4.13326544899994,15.2,10.116028082));
#219418=CARTESIAN_POINT('Ctrl Pts',(4.13326544899994,11.6,10.116028082));
#219419=CARTESIAN_POINT('Ctrl Pts',(4.13343242499994,15.2,10.118953037));
#219420=CARTESIAN_POINT('Ctrl Pts',(4.13343242499994,11.6,10.118953037));
#219421=CARTESIAN_POINT('Ctrl Pts',(4.13359729599994,15.2,10.121883614));
#219422=CARTESIAN_POINT('Ctrl Pts',(4.13359729599994,11.6,10.121883614));
#219423=CARTESIAN_POINT('Ctrl Pts',(4.13376005399994,15.2,10.124819803));
#219424=CARTESIAN_POINT('Ctrl Pts',(4.13376005399994,11.6,10.124819803));
#219425=CARTESIAN_POINT('Ctrl Pts',(4.13392068999994,15.2,10.127761596));
#219426=CARTESIAN_POINT('Ctrl Pts',(4.13392068999994,11.6,10.127761596));
#219427=CARTESIAN_POINT('Ctrl Pts',(4.13407919799995,15.2,10.130708982));
#219428=CARTESIAN_POINT('Ctrl Pts',(4.13407919799995,11.6,10.130708982));
#219429=CARTESIAN_POINT('Ctrl Pts',(4.13423556699995,15.2,10.133661953));
#219430=CARTESIAN_POINT('Ctrl Pts',(4.13423556699995,11.6,10.133661953));
#219431=CARTESIAN_POINT('Ctrl Pts',(4.13438978999995,15.2,10.136620499));
#219432=CARTESIAN_POINT('Ctrl Pts',(4.13438978999995,11.6,10.136620499));
#219433=CARTESIAN_POINT('Ctrl Pts',(4.13454185899994,15.2,10.139584612));
#219434=CARTESIAN_POINT('Ctrl Pts',(4.13454185899994,11.6,10.139584612));
#219435=CARTESIAN_POINT('Ctrl Pts',(4.13469176399994,15.2,10.142554281));
#219436=CARTESIAN_POINT('Ctrl Pts',(4.13469176399994,11.6,10.142554281));
#219437=CARTESIAN_POINT('Ctrl Pts',(4.13483949999994,15.2,10.145529497));
#219438=CARTESIAN_POINT('Ctrl Pts',(4.13483949999994,11.6,10.145529497));
#219439=CARTESIAN_POINT('Ctrl Pts',(4.13498505699994,15.2,10.148510252));
#219440=CARTESIAN_POINT('Ctrl Pts',(4.13498505699994,11.6,10.148510252));
#219441=CARTESIAN_POINT('Ctrl Pts',(4.13512842699994,15.2,10.151496535));
#219442=CARTESIAN_POINT('Ctrl Pts',(4.13512842699994,11.6,10.151496535));
#219443=CARTESIAN_POINT('Ctrl Pts',(4.13526960299994,15.2,10.154488338));
#219444=CARTESIAN_POINT('Ctrl Pts',(4.13526960299994,11.6,10.154488338));
#219445=CARTESIAN_POINT('Ctrl Pts',(4.13540857599994,15.2,10.157485651));
#219446=CARTESIAN_POINT('Ctrl Pts',(4.13540857599994,11.6,10.157485651));
#219447=CARTESIAN_POINT('Ctrl Pts',(4.13554533699994,15.2,10.160488465));
#219448=CARTESIAN_POINT('Ctrl Pts',(4.13554533699994,11.6,10.160488465));
#219449=CARTESIAN_POINT('Ctrl Pts',(4.13567987999994,15.2,10.163496772));
#219450=CARTESIAN_POINT('Ctrl Pts',(4.13567987999994,11.6,10.163496772));
#219451=CARTESIAN_POINT('Ctrl Pts',(4.13581219499994,15.2,10.166510561));
#219452=CARTESIAN_POINT('Ctrl Pts',(4.13581219499994,11.6,10.166510561));
#219453=CARTESIAN_POINT('Ctrl Pts',(4.13594227699994,15.2,10.169529823));
#219454=CARTESIAN_POINT('Ctrl Pts',(4.13594227699994,11.6,10.169529823));
#219455=CARTESIAN_POINT('Ctrl Pts',(4.13607011399994,15.2,10.172554551));
#219456=CARTESIAN_POINT('Ctrl Pts',(4.13607011399994,11.6,10.172554551));
#219457=CARTESIAN_POINT('Ctrl Pts',(4.13619570299994,15.2,10.175584734));
#219458=CARTESIAN_POINT('Ctrl Pts',(4.13619570299994,11.6,10.175584734));
#219459=CARTESIAN_POINT('Ctrl Pts',(4.13631903099995,15.2,10.178620362));
#219460=CARTESIAN_POINT('Ctrl Pts',(4.13631903099995,11.6,10.178620362));
#219461=CARTESIAN_POINT('Ctrl Pts',(4.13644009399994,15.2,10.181661428));
#219462=CARTESIAN_POINT('Ctrl Pts',(4.13644009399994,11.6,10.181661428));
#219463=CARTESIAN_POINT('Ctrl Pts',(4.13655888299994,15.2,10.184707922));
#219464=CARTESIAN_POINT('Ctrl Pts',(4.13655888299994,11.6,10.184707922));
#219465=CARTESIAN_POINT('Ctrl Pts',(4.13667538999994,15.2,10.187759835));
#219466=CARTESIAN_POINT('Ctrl Pts',(4.13667538999994,11.6,10.187759835));
#219467=CARTESIAN_POINT('Ctrl Pts',(4.13678960699994,15.2,10.190817157));
#219468=CARTESIAN_POINT('Ctrl Pts',(4.13678960699994,11.6,10.190817157));
#219469=CARTESIAN_POINT('Ctrl Pts',(4.13690152699994,15.2,10.193879881));
#219470=CARTESIAN_POINT('Ctrl Pts',(4.13690152699994,11.6,10.193879881));
#219471=CARTESIAN_POINT('Ctrl Pts',(4.13701114099995,15.2,10.196947997));
#219472=CARTESIAN_POINT('Ctrl Pts',(4.13701114099995,11.6,10.196947997));
#219473=CARTESIAN_POINT('Ctrl Pts',(4.13711844299994,15.2,10.200021495));
#219474=CARTESIAN_POINT('Ctrl Pts',(4.13711844299994,11.6,10.200021495));
#219475=CARTESIAN_POINT('Ctrl Pts',(4.13722342399994,15.2,10.203100367));
#219476=CARTESIAN_POINT('Ctrl Pts',(4.13722342399994,11.6,10.203100367));
#219477=CARTESIAN_POINT('Ctrl Pts',(4.13732607699994,15.2,10.206184603));
#219478=CARTESIAN_POINT('Ctrl Pts',(4.13732607699994,11.6,10.206184603));
#219479=CARTESIAN_POINT('Ctrl Pts',(4.13742639399994,15.2,10.209274196));
#219480=CARTESIAN_POINT('Ctrl Pts',(4.13742639399994,11.6,10.209274196));
#219481=CARTESIAN_POINT('Ctrl Pts',(4.13752436799994,15.2,10.212369135));
#219482=CARTESIAN_POINT('Ctrl Pts',(4.13752436799994,11.6,10.212369135));
#219483=CARTESIAN_POINT('Ctrl Pts',(4.13761998999994,15.2,10.215469412));
#219484=CARTESIAN_POINT('Ctrl Pts',(4.13761998999994,11.6,10.215469412));
#219485=CARTESIAN_POINT('Ctrl Pts',(4.13771325399995,15.2,10.218575018));
#219486=CARTESIAN_POINT('Ctrl Pts',(4.13771325399995,11.6,10.218575018));
#219487=CARTESIAN_POINT('Ctrl Pts',(4.13780415199995,15.2,10.221685944));
#219488=CARTESIAN_POINT('Ctrl Pts',(4.13780415199995,11.6,10.221685944));
#219489=CARTESIAN_POINT('Ctrl Pts',(4.13789267699994,15.2,10.224802182));
#219490=CARTESIAN_POINT('Ctrl Pts',(4.13789267699994,11.6,10.224802182));
#219491=CARTESIAN_POINT('Ctrl Pts',(4.13797881999994,15.2,10.22792372));
#219492=CARTESIAN_POINT('Ctrl Pts',(4.13797881999994,11.6,10.22792372));
#219493=CARTESIAN_POINT('Ctrl Pts',(4.13806257499994,15.2,10.231050553));
#219494=CARTESIAN_POINT('Ctrl Pts',(4.13806257499994,11.6,10.231050553));
#219495=CARTESIAN_POINT('Ctrl Pts',(4.13814393399994,15.2,10.23418267));
#219496=CARTESIAN_POINT('Ctrl Pts',(4.13814393399994,11.6,10.23418267));
#219497=CARTESIAN_POINT('Ctrl Pts',(4.13822288999994,15.2,10.237320063));
#219498=CARTESIAN_POINT('Ctrl Pts',(4.13822288999994,11.6,10.237320063));
#219499=CARTESIAN_POINT('Ctrl Pts',(4.13829943399994,15.2,10.240462722));
#219500=CARTESIAN_POINT('Ctrl Pts',(4.13829943399994,11.6,10.240462722));
#219501=CARTESIAN_POINT('Ctrl Pts',(4.13837356099994,15.2,10.243610638));
#219502=CARTESIAN_POINT('Ctrl Pts',(4.13837356099994,11.6,10.243610638));
#219503=CARTESIAN_POINT('Ctrl Pts',(4.13844526199994,15.2,10.246763804));
#219504=CARTESIAN_POINT('Ctrl Pts',(4.13844526199994,11.6,10.246763804));
#219505=CARTESIAN_POINT('Ctrl Pts',(4.13851452999995,15.2,10.249922211));
#219506=CARTESIAN_POINT('Ctrl Pts',(4.13851452999995,11.6,10.249922211));
#219507=CARTESIAN_POINT('Ctrl Pts',(4.13858135799994,15.2,10.253085849));
#219508=CARTESIAN_POINT('Ctrl Pts',(4.13858135799994,11.6,10.253085849));
#219509=CARTESIAN_POINT('Ctrl Pts',(4.13864573899995,15.2,10.256254709));
#219510=CARTESIAN_POINT('Ctrl Pts',(4.13864573899995,11.6,10.256254709));
#219511=CARTESIAN_POINT('Ctrl Pts',(4.13870766499994,15.2,10.259428783));
#219512=CARTESIAN_POINT('Ctrl Pts',(4.13870766499994,11.6,10.259428783));
#219513=CARTESIAN_POINT('Ctrl Pts',(4.13876712899994,15.2,10.262608063));
#219514=CARTESIAN_POINT('Ctrl Pts',(4.13876712899994,11.6,10.262608063));
#219515=CARTESIAN_POINT('Ctrl Pts',(4.13882412399994,15.2,10.265792539));
#219516=CARTESIAN_POINT('Ctrl Pts',(4.13882412399994,11.6,10.265792539));
#219517=CARTESIAN_POINT('Ctrl Pts',(4.13887864299994,15.2,10.268982203));
#219518=CARTESIAN_POINT('Ctrl Pts',(4.13887864299994,11.6,10.268982203));
#219519=CARTESIAN_POINT('Ctrl Pts',(4.13893067799994,15.2,10.272177045));
#219520=CARTESIAN_POINT('Ctrl Pts',(4.13893067799994,11.6,10.272177045));
#219521=CARTESIAN_POINT('Ctrl Pts',(4.13898022299994,15.2,10.275377058));
#219522=CARTESIAN_POINT('Ctrl Pts',(4.13898022299994,11.6,10.275377058));
#219523=CARTESIAN_POINT('Ctrl Pts',(4.13902726899994,15.2,10.278582233));
#219524=CARTESIAN_POINT('Ctrl Pts',(4.13902726899994,11.6,10.278582233));
#219525=CARTESIAN_POINT('Ctrl Pts',(4.13907180999994,15.2,10.281792559));
#219526=CARTESIAN_POINT('Ctrl Pts',(4.13907180999994,11.6,10.281792559));
#219527=CARTESIAN_POINT('Ctrl Pts',(4.13911384099994,15.2,10.285008031));
#219528=CARTESIAN_POINT('Ctrl Pts',(4.13911384099994,11.6,10.285008031));
#219529=CARTESIAN_POINT('Ctrl Pts',(4.13915335099994,15.2,10.288228638));
#219530=CARTESIAN_POINT('Ctrl Pts',(4.13915335099994,11.6,10.288228638));
#219531=CARTESIAN_POINT('Ctrl Pts',(4.13919033599994,15.2,10.291454371));
#219532=CARTESIAN_POINT('Ctrl Pts',(4.13919033599994,11.6,10.291454371));
#219533=CARTESIAN_POINT('Ctrl Pts',(4.13922478799994,15.2,10.294685223));
#219534=CARTESIAN_POINT('Ctrl Pts',(4.13922478799994,11.6,10.294685223));
#219535=CARTESIAN_POINT('Ctrl Pts',(4.13925669999994,15.2,10.297921185));
#219536=CARTESIAN_POINT('Ctrl Pts',(4.13925669999994,11.6,10.297921185));
#219537=CARTESIAN_POINT('Ctrl Pts',(4.13928606399994,15.2,10.301162247));
#219538=CARTESIAN_POINT('Ctrl Pts',(4.13928606399994,11.6,10.301162247));
#219539=CARTESIAN_POINT('Ctrl Pts',(4.13931287499994,15.2,10.304408403));
#219540=CARTESIAN_POINT('Ctrl Pts',(4.13931287499994,11.6,10.304408403));
#219541=CARTESIAN_POINT('Ctrl Pts',(4.13933712499994,15.2,10.307659642));
#219542=CARTESIAN_POINT('Ctrl Pts',(4.13933712499994,11.6,10.307659642));
#219543=CARTESIAN_POINT('Ctrl Pts',(4.13935880599994,15.2,10.310915956));
#219544=CARTESIAN_POINT('Ctrl Pts',(4.13935880599994,11.6,10.310915956));
#219545=CARTESIAN_POINT('Ctrl Pts',(4.13937791299994,15.2,10.314177338));
#219546=CARTESIAN_POINT('Ctrl Pts',(4.13937791299994,11.6,10.314177338));
#219547=CARTESIAN_POINT('Ctrl Pts',(4.13939443899995,15.2,10.317443777));
#219548=CARTESIAN_POINT('Ctrl Pts',(4.13939443899995,11.6,10.317443777));
#219549=CARTESIAN_POINT('Ctrl Pts',(4.13940837499994,15.2,10.320715266));
#219550=CARTESIAN_POINT('Ctrl Pts',(4.13940837499994,11.6,10.320715266));
#219551=CARTESIAN_POINT('Ctrl Pts',(4.13941971699994,15.2,10.323991796));
#219552=CARTESIAN_POINT('Ctrl Pts',(4.13941971699994,11.6,10.323991796));
#219553=CARTESIAN_POINT('Ctrl Pts',(4.13942845599994,15.2,10.327273358));
#219554=CARTESIAN_POINT('Ctrl Pts',(4.13942845599994,11.6,10.327273358));
#219555=CARTESIAN_POINT('Ctrl Pts',(4.13943458699995,15.2,10.330559945));
#219556=CARTESIAN_POINT('Ctrl Pts',(4.13943458699995,11.6,10.330559945));
#219557=CARTESIAN_POINT('Ctrl Pts',(4.13943810199994,15.2,10.333851547));
#219558=CARTESIAN_POINT('Ctrl Pts',(4.13943810199994,11.6,10.333851547));
#219559=CARTESIAN_POINT('Ctrl Pts',(4.13943899399994,15.2,10.337148157));
#219560=CARTESIAN_POINT('Ctrl Pts',(4.13943899399994,11.6,10.337148157));
#219561=CARTESIAN_POINT('Ctrl Pts',(4.13943725799994,15.2,10.340449765));
#219562=CARTESIAN_POINT('Ctrl Pts',(4.13943725799994,11.6,10.340449765));
#219563=CARTESIAN_POINT('Ctrl Pts',(4.13943288499994,15.2,10.343756363));
#219564=CARTESIAN_POINT('Ctrl Pts',(4.13943288499994,11.6,10.343756363));
#219565=CARTESIAN_POINT('Ctrl Pts',(4.13942586899995,15.2,10.347067944));
#219566=CARTESIAN_POINT('Ctrl Pts',(4.13942586899995,11.6,10.347067944));
#219567=CARTESIAN_POINT('Ctrl Pts',(4.13941620499994,15.2,10.350384497));
#219568=CARTESIAN_POINT('Ctrl Pts',(4.13941620499994,11.6,10.350384497));
#219569=CARTESIAN_POINT('Ctrl Pts',(4.13940388399994,15.2,10.353706016));
#219570=CARTESIAN_POINT('Ctrl Pts',(4.13940388399994,11.6,10.353706016));
#219571=CARTESIAN_POINT('Ctrl Pts',(4.13938890099994,15.2,10.357032491));
#219572=CARTESIAN_POINT('Ctrl Pts',(4.13938890099994,11.6,10.357032491));
#219573=CARTESIAN_POINT('Ctrl Pts',(4.13937124999994,15.2,10.360363915));
#219574=CARTESIAN_POINT('Ctrl Pts',(4.13937124999994,11.6,10.360363915));
#219575=CARTESIAN_POINT('Ctrl Pts',(4.13935092099995,15.2,10.363700278));
#219576=CARTESIAN_POINT('Ctrl Pts',(4.13935092099995,11.6,10.363700278));
#219577=CARTESIAN_POINT('Ctrl Pts',(4.13932791199994,15.2,10.367041572));
#219578=CARTESIAN_POINT('Ctrl Pts',(4.13932791199994,11.6,10.367041572));
#219579=CARTESIAN_POINT('Ctrl Pts',(4.13930221199994,15.2,10.370387789));
#219580=CARTESIAN_POINT('Ctrl Pts',(4.13930221199994,11.6,10.370387789));
#219581=CARTESIAN_POINT('Ctrl Pts',(4.13927381799994,15.2,10.373738921));
#219582=CARTESIAN_POINT('Ctrl Pts',(4.13927381799994,11.6,10.373738921));
#219583=CARTESIAN_POINT('Ctrl Pts',(4.13924272199994,15.2,10.37709496));
#219584=CARTESIAN_POINT('Ctrl Pts',(4.13924272199994,11.6,10.37709496));
#219585=CARTESIAN_POINT('Ctrl Pts',(4.13920891699994,15.2,10.380455897));
#219586=CARTESIAN_POINT('Ctrl Pts',(4.13920891699994,11.6,10.380455897));
#219587=CARTESIAN_POINT('Ctrl Pts',(4.13917239799994,15.2,10.383821722));
#219588=CARTESIAN_POINT('Ctrl Pts',(4.13917239799994,11.6,10.383821722));
#219589=CARTESIAN_POINT('Ctrl Pts',(4.13913315699994,15.2,10.38719243));
#219590=CARTESIAN_POINT('Ctrl Pts',(4.13913315699994,11.6,10.38719243));
#219591=CARTESIAN_POINT('Ctrl Pts',(4.13909118899995,15.2,10.39056801));
#219592=CARTESIAN_POINT('Ctrl Pts',(4.13909118899995,11.6,10.39056801));
#219593=CARTESIAN_POINT('Ctrl Pts',(4.13904648599994,15.2,10.393948456));
#219594=CARTESIAN_POINT('Ctrl Pts',(4.13904648599994,11.6,10.393948456));
#219595=CARTESIAN_POINT('Ctrl Pts',(4.13899904399995,15.2,10.397333758));
#219596=CARTESIAN_POINT('Ctrl Pts',(4.13899904399995,11.6,10.397333758));
#219597=CARTESIAN_POINT('Ctrl Pts',(4.13894885299994,15.2,10.400723909));
#219598=CARTESIAN_POINT('Ctrl Pts',(4.13894885299994,11.6,10.400723909));
#219599=CARTESIAN_POINT('Ctrl Pts',(4.13889590999994,15.2,10.4041189));
#219600=CARTESIAN_POINT('Ctrl Pts',(4.13889590999994,11.6,10.4041189));
#219601=CARTESIAN_POINT('Ctrl Pts',(4.13884020599994,15.2,10.407518721));
#219602=CARTESIAN_POINT('Ctrl Pts',(4.13884020599994,11.6,10.407518721));
#219603=CARTESIAN_POINT('Ctrl Pts',(4.13878173799994,15.2,10.410923367));
#219604=CARTESIAN_POINT('Ctrl Pts',(4.13878173799994,11.6,10.410923367));
#219605=CARTESIAN_POINT('Ctrl Pts',(4.13872049699994,15.2,10.414332828));
#219606=CARTESIAN_POINT('Ctrl Pts',(4.13872049699994,11.6,10.414332828));
#219607=CARTESIAN_POINT('Ctrl Pts',(4.13865647599994,15.2,10.417747096));
#219608=CARTESIAN_POINT('Ctrl Pts',(4.13865647599994,11.6,10.417747096));
#219609=CARTESIAN_POINT('Ctrl Pts',(4.13858967199995,15.2,10.421166163));
#219610=CARTESIAN_POINT('Ctrl Pts',(4.13858967199995,11.6,10.421166163));
#219611=CARTESIAN_POINT('Ctrl Pts',(4.13852007699994,15.2,10.424590021));
#219612=CARTESIAN_POINT('Ctrl Pts',(4.13852007699994,11.6,10.424590021));
#219613=CARTESIAN_POINT('Ctrl Pts',(4.13844768399994,15.2,10.428018661));
#219614=CARTESIAN_POINT('Ctrl Pts',(4.13844768399994,11.6,10.428018661));
#219615=CARTESIAN_POINT('Ctrl Pts',(4.13837248699994,15.2,10.431452077));
#219616=CARTESIAN_POINT('Ctrl Pts',(4.13837248699994,11.6,10.431452077));
#219617=CARTESIAN_POINT('Ctrl Pts',(4.13829448099994,15.2,10.434890258));
#219618=CARTESIAN_POINT('Ctrl Pts',(4.13829448099994,11.6,10.434890258));
#219619=CARTESIAN_POINT('Ctrl Pts',(4.13821365899994,15.2,10.438333197));
#219620=CARTESIAN_POINT('Ctrl Pts',(4.13821365899994,11.6,10.438333197));
#219621=CARTESIAN_POINT('Ctrl Pts',(4.13813001599994,15.2,10.441780886));
#219622=CARTESIAN_POINT('Ctrl Pts',(4.13813001599994,11.6,10.441780886));
#219623=CARTESIAN_POINT('Ctrl Pts',(4.13804354399994,15.2,10.445233317));
#219624=CARTESIAN_POINT('Ctrl Pts',(4.13804354399994,11.6,10.445233317));
#219625=CARTESIAN_POINT('Ctrl Pts',(4.13795423699994,15.2,10.448690482));
#219626=CARTESIAN_POINT('Ctrl Pts',(4.13795423699994,11.6,10.448690482));
#219627=CARTESIAN_POINT('Ctrl Pts',(4.13786209099994,15.2,10.452152373));
#219628=CARTESIAN_POINT('Ctrl Pts',(4.13786209099994,11.6,10.452152373));
#219629=CARTESIAN_POINT('Ctrl Pts',(4.13776709699994,15.2,10.45561898));
#219630=CARTESIAN_POINT('Ctrl Pts',(4.13776709699994,11.6,10.45561898));
#219631=CARTESIAN_POINT('Ctrl Pts',(4.13766925199995,15.2,10.459090298));
#219632=CARTESIAN_POINT('Ctrl Pts',(4.13766925199995,11.6,10.459090298));
#219633=CARTESIAN_POINT('Ctrl Pts',(4.13756854799994,15.2,10.462566317));
#219634=CARTESIAN_POINT('Ctrl Pts',(4.13756854799994,11.6,10.462566317));
#219635=CARTESIAN_POINT('Ctrl Pts',(4.13746497999994,15.2,10.466047029));
#219636=CARTESIAN_POINT('Ctrl Pts',(4.13746497999994,11.6,10.466047029));
#219637=CARTESIAN_POINT('Ctrl Pts',(4.13735853899994,15.2,10.469532426));
#219638=CARTESIAN_POINT('Ctrl Pts',(4.13735853899994,11.6,10.469532426));
#219639=CARTESIAN_POINT('Ctrl Pts',(4.13724922399994,15.2,10.473022501));
#219640=CARTESIAN_POINT('Ctrl Pts',(4.13724922399994,11.6,10.473022501));
#219641=CARTESIAN_POINT('Ctrl Pts',(4.13713702599994,15.2,10.476517245));
#219642=CARTESIAN_POINT('Ctrl Pts',(4.13713702599994,11.6,10.476517245));
#219643=CARTESIAN_POINT('Ctrl Pts',(4.13702193799994,15.2,10.48001665));
#219644=CARTESIAN_POINT('Ctrl Pts',(4.13702193799994,11.6,10.48001665));
#219645=CARTESIAN_POINT('Ctrl Pts',(4.13690395699994,15.2,10.483520709));
#219646=CARTESIAN_POINT('Ctrl Pts',(4.13690395699994,11.6,10.483520709));
#219647=CARTESIAN_POINT('Ctrl Pts',(4.13678307499994,15.2,10.487029411));
#219648=CARTESIAN_POINT('Ctrl Pts',(4.13678307499994,11.6,10.487029411));
#219649=CARTESIAN_POINT('Ctrl Pts',(4.13665928599994,15.2,10.490542752));
#219650=CARTESIAN_POINT('Ctrl Pts',(4.13665928599994,11.6,10.490542752));
#219651=CARTESIAN_POINT('Ctrl Pts',(4.13653258699994,15.2,10.494060722));
#219652=CARTESIAN_POINT('Ctrl Pts',(4.13653258699994,11.6,10.494060722));
#219653=CARTESIAN_POINT('Ctrl Pts',(4.13640296799994,15.2,10.497583313));
#219654=CARTESIAN_POINT('Ctrl Pts',(4.13640296799994,11.6,10.497583313));
#219655=CARTESIAN_POINT('Ctrl Pts',(4.13627042599995,15.2,10.501110517));
#219656=CARTESIAN_POINT('Ctrl Pts',(4.13627042599995,11.6,10.501110517));
#219657=CARTESIAN_POINT('Ctrl Pts',(4.13613495399995,15.2,10.504642327));
#219658=CARTESIAN_POINT('Ctrl Pts',(4.13613495399995,11.6,10.504642327));
#219659=CARTESIAN_POINT('Ctrl Pts',(4.13599654599994,15.2,10.508178734));
#219660=CARTESIAN_POINT('Ctrl Pts',(4.13599654599994,11.6,10.508178734));
#219661=CARTESIAN_POINT('Ctrl Pts',(4.13585519699994,15.2,10.51171973));
#219662=CARTESIAN_POINT('Ctrl Pts',(4.13585519699994,11.6,10.51171973));
#219663=CARTESIAN_POINT('Ctrl Pts',(4.13571090199994,15.2,10.515265308));
#219664=CARTESIAN_POINT('Ctrl Pts',(4.13571090199994,11.6,10.515265308));
#219665=CARTESIAN_POINT('Ctrl Pts',(4.13556365199994,15.2,10.518815459));
#219666=CARTESIAN_POINT('Ctrl Pts',(4.13556365199994,11.6,10.518815459));
#219667=CARTESIAN_POINT('Ctrl Pts',(4.13541344499994,15.2,10.522370177));
#219668=CARTESIAN_POINT('Ctrl Pts',(4.13541344499994,11.6,10.522370177));
#219669=CARTESIAN_POINT('Ctrl Pts',(4.13526027299994,15.2,10.525929452));
#219670=CARTESIAN_POINT('Ctrl Pts',(4.13526027299994,11.6,10.525929452));
#219671=CARTESIAN_POINT('Ctrl Pts',(4.13510412999995,15.2,10.529493277));
#219672=CARTESIAN_POINT('Ctrl Pts',(4.13510412999995,11.6,10.529493277));
#219673=CARTESIAN_POINT('Ctrl Pts',(4.13494501199995,15.2,10.533061644));
#219674=CARTESIAN_POINT('Ctrl Pts',(4.13494501199995,11.6,10.533061644));
#219675=CARTESIAN_POINT('Ctrl Pts',(4.13478291299994,15.2,10.536634545));
#219676=CARTESIAN_POINT('Ctrl Pts',(4.13478291299994,11.6,10.536634545));
#219677=CARTESIAN_POINT('Ctrl Pts',(4.13461782599994,15.2,10.540211972));
#219678=CARTESIAN_POINT('Ctrl Pts',(4.13461782599994,11.6,10.540211972));
#219679=CARTESIAN_POINT('Ctrl Pts',(4.13444974499994,15.2,10.543793918));
#219680=CARTESIAN_POINT('Ctrl Pts',(4.13444974499994,11.6,10.543793918));
#219681=CARTESIAN_POINT('Ctrl Pts',(4.13427866799995,15.2,10.547380374));
#219682=CARTESIAN_POINT('Ctrl Pts',(4.13427866799995,11.6,10.547380374));
#219683=CARTESIAN_POINT('Ctrl Pts',(4.13410458499994,15.2,10.550971333));
#219684=CARTESIAN_POINT('Ctrl Pts',(4.13410458499994,11.6,10.550971333));
#219685=CARTESIAN_POINT('Ctrl Pts',(4.13392749299994,15.2,10.554566788));
#219686=CARTESIAN_POINT('Ctrl Pts',(4.13392749299994,11.6,10.554566788));
#219687=CARTESIAN_POINT('Ctrl Pts',(4.13374738599994,15.2,10.55816673));
#219688=CARTESIAN_POINT('Ctrl Pts',(4.13374738599994,11.6,10.55816673));
#219689=CARTESIAN_POINT('Ctrl Pts',(4.13356425899994,15.2,10.561771151));
#219690=CARTESIAN_POINT('Ctrl Pts',(4.13356425899994,11.6,10.561771151));
#219691=CARTESIAN_POINT('Ctrl Pts',(4.13337810299994,15.2,10.565380043));
#219692=CARTESIAN_POINT('Ctrl Pts',(4.13337810299994,11.6,10.565380043));
#219693=CARTESIAN_POINT('Ctrl Pts',(4.13318891699994,15.2,10.568993399));
#219694=CARTESIAN_POINT('Ctrl Pts',(4.13318891699994,11.6,10.568993399));
#219695=CARTESIAN_POINT('Ctrl Pts',(4.13299669299994,15.2,10.572611211));
#219696=CARTESIAN_POINT('Ctrl Pts',(4.13299669299994,11.6,10.572611211));
#219697=CARTESIAN_POINT('Ctrl Pts',(4.13280142599994,15.2,10.576233472));
#219698=CARTESIAN_POINT('Ctrl Pts',(4.13280142599994,11.6,10.576233472));
#219699=CARTESIAN_POINT('Ctrl Pts',(4.13260311099994,15.2,10.579860173));
#219700=CARTESIAN_POINT('Ctrl Pts',(4.13260311099994,11.6,10.579860173));
#219701=CARTESIAN_POINT('Ctrl Pts',(4.13240174099994,15.2,10.583491307));
#219702=CARTESIAN_POINT('Ctrl Pts',(4.13240174099994,11.6,10.583491307));
#219703=CARTESIAN_POINT('Ctrl Pts',(4.13219731199994,15.2,10.587126865));
#219704=CARTESIAN_POINT('Ctrl Pts',(4.13219731199994,11.6,10.587126865));
#219705=CARTESIAN_POINT('Ctrl Pts',(4.13198981899995,15.2,10.590766842));
#219706=CARTESIAN_POINT('Ctrl Pts',(4.13198981899995,11.6,10.590766842));
#219707=CARTESIAN_POINT('Ctrl Pts',(4.13177925499994,15.2,10.594411227));
#219708=CARTESIAN_POINT('Ctrl Pts',(4.13177925499994,11.6,10.594411227));
#219709=CARTESIAN_POINT('Ctrl Pts',(4.13156561499994,15.2,10.598060015));
#219710=CARTESIAN_POINT('Ctrl Pts',(4.13156561499994,11.6,10.598060015));
#219711=CARTESIAN_POINT('Ctrl Pts',(4.13134889399995,15.2,10.601713197));
#219712=CARTESIAN_POINT('Ctrl Pts',(4.13134889399995,11.6,10.601713197));
#219713=CARTESIAN_POINT('Ctrl Pts',(4.13112908699994,15.2,10.605370765));
#219714=CARTESIAN_POINT('Ctrl Pts',(4.13112908699994,11.6,10.605370765));
#219715=CARTESIAN_POINT('Ctrl Pts',(4.13090618799994,15.2,10.609032712));
#219716=CARTESIAN_POINT('Ctrl Pts',(4.13090618799994,11.6,10.609032712));
#219717=CARTESIAN_POINT('Ctrl Pts',(4.13068019199994,15.2,10.612699031));
#219718=CARTESIAN_POINT('Ctrl Pts',(4.13068019199994,11.6,10.612699031));
#219719=CARTESIAN_POINT('Ctrl Pts',(4.13045109399994,15.2,10.616369713));
#219720=CARTESIAN_POINT('Ctrl Pts',(4.13045109399994,11.6,10.616369713));
#219721=CARTESIAN_POINT('Ctrl Pts',(4.13021888699994,15.2,10.62004475));
#219722=CARTESIAN_POINT('Ctrl Pts',(4.13021888699994,11.6,10.62004475));
#219723=CARTESIAN_POINT('Ctrl Pts',(4.12998356799995,15.2,10.623724135));
#219724=CARTESIAN_POINT('Ctrl Pts',(4.12998356799995,11.6,10.623724135));
#219725=CARTESIAN_POINT('Ctrl Pts',(4.12974512999994,15.2,10.627407862));
#219726=CARTESIAN_POINT('Ctrl Pts',(4.12974512999994,11.6,10.627407862));
#219727=CARTESIAN_POINT('Ctrl Pts',(4.12950356699994,15.2,10.63109592));
#219728=CARTESIAN_POINT('Ctrl Pts',(4.12950356699994,11.6,10.63109592));
#219729=CARTESIAN_POINT('Ctrl Pts',(4.12925887599994,15.2,10.634788304));
#219730=CARTESIAN_POINT('Ctrl Pts',(4.12925887599994,11.6,10.634788304));
#219731=CARTESIAN_POINT('Ctrl Pts',(4.12901105099994,15.2,10.638485005));
#219732=CARTESIAN_POINT('Ctrl Pts',(4.12901105099994,11.6,10.638485005));
#219733=CARTESIAN_POINT('Ctrl Pts',(4.12876008699994,15.2,10.642186018));
#219734=CARTESIAN_POINT('Ctrl Pts',(4.12876008699994,11.6,10.642186018));
#219735=CARTESIAN_POINT('Ctrl Pts',(4.12850597799994,15.2,10.645891332));
#219736=CARTESIAN_POINT('Ctrl Pts',(4.12850597799994,11.6,10.645891332));
#219737=CARTESIAN_POINT('Ctrl Pts',(4.12824871999994,15.2,10.649600943));
#219738=CARTESIAN_POINT('Ctrl Pts',(4.12824871999994,11.6,10.649600943));
#219739=CARTESIAN_POINT('Ctrl Pts',(4.12798830699994,15.2,10.65331484));
#219740=CARTESIAN_POINT('Ctrl Pts',(4.12798830699994,11.6,10.65331484));
#219741=CARTESIAN_POINT('Ctrl Pts',(4.12772473399994,15.2,10.657033018));
#219742=CARTESIAN_POINT('Ctrl Pts',(4.12772473399994,11.6,10.657033018));
#219743=CARTESIAN_POINT('Ctrl Pts',(4.12745799499994,15.2,10.660755467));
#219744=CARTESIAN_POINT('Ctrl Pts',(4.12745799499994,11.6,10.660755467));
#219745=CARTESIAN_POINT('Ctrl Pts',(4.12718808399995,15.2,10.66448218));
#219746=CARTESIAN_POINT('Ctrl Pts',(4.12718808399995,11.6,10.66448218));
#219747=CARTESIAN_POINT('Ctrl Pts',(4.12691499899995,15.2,10.668213149));
#219748=CARTESIAN_POINT('Ctrl Pts',(4.12691499899995,11.6,10.668213149));
#219749=CARTESIAN_POINT('Ctrl Pts',(4.12663873099994,15.2,10.671948366));
#219750=CARTESIAN_POINT('Ctrl Pts',(4.12663873099994,11.6,10.671948366));
#219751=CARTESIAN_POINT('Ctrl Pts',(4.12635927699994,15.2,10.675687826));
#219752=CARTESIAN_POINT('Ctrl Pts',(4.12635927699994,11.6,10.675687826));
#219753=CARTESIAN_POINT('Ctrl Pts',(4.12607663299995,15.2,10.679431519));
#219754=CARTESIAN_POINT('Ctrl Pts',(4.12607663299995,11.6,10.679431519));
#219755=CARTESIAN_POINT('Ctrl Pts',(4.12579079399995,15.2,10.683179442));
#219756=CARTESIAN_POINT('Ctrl Pts',(4.12579079399995,11.6,10.683179442));
#219757=CARTESIAN_POINT('Ctrl Pts',(4.12550175599994,15.2,10.686931586));
#219758=CARTESIAN_POINT('Ctrl Pts',(4.12550175599994,11.6,10.686931586));
#219759=CARTESIAN_POINT('Ctrl Pts',(4.12520951199994,15.2,10.690687944));
#219760=CARTESIAN_POINT('Ctrl Pts',(4.12520951199994,11.6,10.690687944));
#219761=CARTESIAN_POINT('Ctrl Pts',(4.12491405899994,15.2,10.694448508));
#219762=CARTESIAN_POINT('Ctrl Pts',(4.12491405899994,11.6,10.694448508));
#219763=CARTESIAN_POINT('Ctrl Pts',(4.12461539099994,15.2,10.698213269));
#219764=CARTESIAN_POINT('Ctrl Pts',(4.12461539099994,11.6,10.698213269));
#219765=CARTESIAN_POINT('Ctrl Pts',(4.12431349899994,15.2,10.70198222));
#219766=CARTESIAN_POINT('Ctrl Pts',(4.12431349899994,11.6,10.70198222));
#219767=CARTESIAN_POINT('Ctrl Pts',(4.12400838099995,15.2,10.705755348));
#219768=CARTESIAN_POINT('Ctrl Pts',(4.12400838099995,11.6,10.705755348));
#219769=CARTESIAN_POINT('Ctrl Pts',(4.12370002799994,15.2,10.709532648));
#219770=CARTESIAN_POINT('Ctrl Pts',(4.12370002799994,11.6,10.709532648));
#219771=CARTESIAN_POINT('Ctrl Pts',(4.12338843599994,15.2,10.713314109));
#219772=CARTESIAN_POINT('Ctrl Pts',(4.12338843599994,11.6,10.713314109));
#219773=CARTESIAN_POINT('Ctrl Pts',(4.12307359999994,15.2,10.717099726));
#219774=CARTESIAN_POINT('Ctrl Pts',(4.12307359999994,11.6,10.717099726));
#219775=CARTESIAN_POINT('Ctrl Pts',(4.12275551699994,15.2,10.720889492));
#219776=CARTESIAN_POINT('Ctrl Pts',(4.12275551699994,11.6,10.720889492));
#219777=CARTESIAN_POINT('Ctrl Pts',(4.12243418399994,15.2,10.724683406));
#219778=CARTESIAN_POINT('Ctrl Pts',(4.12243418399994,11.6,10.724683406));
#219779=CARTESIAN_POINT('Ctrl Pts',(4.12210959999994,15.2,10.728481465));
#219780=CARTESIAN_POINT('Ctrl Pts',(4.12210959999994,11.6,10.728481465));
#219781=CARTESIAN_POINT('Ctrl Pts',(4.12184733299994,15.2,10.731523226));
#219782=CARTESIAN_POINT('Ctrl Pts',(4.12184733299994,11.6,10.731523226));
#219783=CARTESIAN_POINT('Ctrl Pts',(4.12164916999994,15.2,10.733806412));
#219784=CARTESIAN_POINT('Ctrl Pts',(4.12164916999994,11.6,10.733806412));
#219785=CARTESIAN_POINT('Ctrl Pts',(4.12151640999994,15.2,10.735329364));
#219786=CARTESIAN_POINT('Ctrl Pts',(4.12151640999994,11.6,10.735329364));
#219787=CARTESIAN_POINT('Ctrl Pts',(4.12144986799994,15.2,10.736091048));
#219788=CARTESIAN_POINT('Ctrl Pts',(4.12144986799994,11.6,10.736091048));
#219789=CARTESIAN_POINT('Ctrl Pts',(4.04260911699994,15.2,9.55499537099998));
#219790=CARTESIAN_POINT('Ctrl Pts',(4.0431612978139,15.2,9.55669455126485));
#219791=CARTESIAN_POINT('Ctrl Pts',(4.04372605441455,15.2,9.55844976666689));
#219792=CARTESIAN_POINT('Ctrl Pts',(4.0443024457118,15.2,9.56026027830994));
#219793=CARTESIAN_POINT('Ctrl Pts',(4.04488161665923,15.2,9.56207952115529));
#219794=CARTESIAN_POINT('Ctrl Pts',(4.04547254566134,15.2,9.5639546011486));
#219795=CARTESIAN_POINT('Ctrl Pts',(4.04607433355817,15.2,9.56588480618675));
#219796=CARTESIAN_POINT('Ctrl Pts',(4.04667612140033,15.2,9.56781501104957));
#219797=CARTESIAN_POINT('Ctrl Pts',(4.0472887675309,15.2,9.56980034131573));
#219798=CARTESIAN_POINT('Ctrl Pts',(4.04791140625826,15.2,9.57184010199156));
#219799=CARTESIAN_POINT('Ctrl Pts',(4.04853404498562,15.2,9.57387986266738));
#219800=CARTESIAN_POINT('Ctrl Pts',(4.04916667256298,15.2,9.57597405404105));
#219801=CARTESIAN_POINT('Ctrl Pts',(4.04980844773787,15.2,9.5781219999839));
#219802=CARTESIAN_POINT('Ctrl Pts',(4.05045022297105,15.2,9.58026994612186));
#219803=CARTESIAN_POINT('Ctrl Pts',(4.05110114566863,15.2,9.58247164636916));
#219804=CARTESIAN_POINT('Ctrl Pts',(4.05176039887179,15.2,9.58472644049568));
#219805=CARTESIAN_POINT('Ctrl Pts',(4.05241965201507,15.2,9.58698123441737));
#219806=CARTESIAN_POINT('Ctrl Pts',(4.05308723453836,15.2,9.58928912179259));
#219807=CARTESIAN_POINT('Ctrl Pts',(4.05376235301691,15.2,9.59164945971764));
#219808=CARTESIAN_POINT('Ctrl Pts',(4.05443747149546,15.2,9.59400979764269));
#219809=CARTESIAN_POINT('Ctrl Pts',(4.05512012665439,15.2,9.59642258494925));
#219810=CARTESIAN_POINT('Ctrl Pts',(4.05580954896239,15.2,9.59888719110747));
#219811=CARTESIAN_POINT('Ctrl Pts',(4.05649897133301,15.2,9.60135179748954));
#219812=CARTESIAN_POINT('Ctrl Pts',(4.05719515735446,15.2,9.60386822484468));
#219813=CARTESIAN_POINT('Ctrl Pts',(4.05789736205981,15.2,9.60643585623811));
#219814=CARTESIAN_POINT('Ctrl Pts',(4.05859956670138,15.2,9.60900348739833));
#219815=CARTESIAN_POINT('Ctrl Pts',(4.05930778806454,15.2,9.6116223227904));
#219816=CARTESIAN_POINT('Ctrl Pts',(4.06002130053884,15.2,9.61429176086226));
#219817=CARTESIAN_POINT('Ctrl Pts',(4.06073481301314,15.2,9.61696119893412));
#219818=CARTESIAN_POINT('Ctrl Pts',(4.06145361427035,15.2,9.6196812398353));
#219819=CARTESIAN_POINT('Ctrl Pts',(4.06217699974386,15.2,9.62245129406581));
#219820=CARTESIAN_POINT('Ctrl Pts',(4.06290038521737,15.2,9.6252213482963));
#219821=CARTESIAN_POINT('Ctrl Pts',(4.06362835112202,15.2,9.62804141806142));
#219822=CARTESIAN_POINT('Ctrl Pts',(4.06436021384517,15.2,9.6309109224538));
#219823=CARTESIAN_POINT('Ctrl Pts',(4.06509207663479,15.2,9.63378042710684));
#219824=CARTESIAN_POINT('Ctrl Pts',(4.06582783371649,15.2,9.63669936978133));
#219825=CARTESIAN_POINT('Ctrl Pts',(4.06656681575689,15.2,9.63966718444519));
#219826=CARTESIAN_POINT('Ctrl Pts',(4.06730579773018,15.2,9.64263499883946));
#219827=CARTESIAN_POINT('Ctrl Pts',(4.06804800688995,15.2,9.64565168593773));
#219828=CARTESIAN_POINT('Ctrl Pts',(4.06879278803294,15.2,9.64871669225685));
#219829=CARTESIAN_POINT('Ctrl Pts',(4.06953756917591,15.2,9.65178169857597));
#219830=CARTESIAN_POINT('Ctrl Pts',(4.07028492497895,15.2,9.65489502280677));
#219831=CARTESIAN_POINT('Ctrl Pts',(4.07103421911827,15.2,9.65805612418869));
#219832=CARTESIAN_POINT('Ctrl Pts',(4.07178351332565,15.2,9.66121722585776));
#219833=CARTESIAN_POINT('Ctrl Pts',(4.07253474754156,15.2,9.66442610392306));
#219834=CARTESIAN_POINT('Ctrl Pts',(4.07328730183263,15.2,9.6676822256859));
#219835=CARTESIAN_POINT('Ctrl Pts',(4.07403985605534,15.2,9.67093834715298));
#219836=CARTESIAN_POINT('Ctrl Pts',(4.07479373107359,15.2,9.67424171311334));
#219837=CARTESIAN_POINT('Ctrl Pts',(4.07554832521627,15.2,9.67759179975672));
#219838=CARTESIAN_POINT('Ctrl Pts',(4.07630291935894,15.2,9.68094188640011));
#219839=CARTESIAN_POINT('Ctrl Pts',(4.07705823111172,15.2,9.68433869551952));
#219840=CARTESIAN_POINT('Ctrl Pts',(4.0778136744176,15.2,9.6877817138913));
#219841=CARTESIAN_POINT('Ctrl Pts',(4.07869502498687,15.2,9.69179856886687));
#219842=CARTESIAN_POINT('Ctrl Pts',(4.0795765539041,15.2,9.69587831786509));
#219843=CARTESIAN_POINT('Ctrl Pts',(4.08045735274127,15.2,9.70002016398996));
#219844=CARTESIAN_POINT('Ctrl Pts',(4.08121232313394,15.2,9.70357031762702));
#219845=CARTESIAN_POINT('Ctrl Pts',(4.0819667586368,15.2,9.70716609326345));
#219846=CARTESIAN_POINT('Ctrl Pts',(4.08272010119283,15.2,9.71080699787805));
#219847=CARTESIAN_POINT('Ctrl Pts',(4.08347344381729,15.2,9.71444790282339));
#219848=CARTESIAN_POINT('Ctrl Pts',(4.08422569433591,15.2,9.71813393641028));
#219849=CARTESIAN_POINT('Ctrl Pts',(4.08497631083089,15.2,9.72186461438592));
#219850=CARTESIAN_POINT('Ctrl Pts',(4.0857269272577,15.2,9.72559529202268));
#219851=CARTESIAN_POINT('Ctrl Pts',(4.08647590841874,15.2,9.72937061341363));
#219852=CARTESIAN_POINT('Ctrl Pts',(4.08722272397495,15.2,9.7331901010249));
#219853=CARTESIAN_POINT('Ctrl Pts',(4.08796953953115,15.2,9.73700958863618));
#219854=CARTESIAN_POINT('Ctrl Pts',(4.08871419150124,15.2,9.74087324220468));
#219855=CARTESIAN_POINT('Ctrl Pts',(4.08945616017817,15.2,9.74478059492203));
#219856=CARTESIAN_POINT('Ctrl Pts',(4.09007446743141,15.2,9.74803672230481));
#219857=CARTESIAN_POINT('Ctrl Pts',(4.09069091275409,15.2,9.75132319390142));
#219858=CARTESIAN_POINT('Ctrl Pts',(4.09130520247643,15.2,9.75463974452485));
#219859=CARTESIAN_POINT('Ctrl Pts',(4.09191949219876,15.2,9.75795629514829));
#219860=CARTESIAN_POINT('Ctrl Pts',(4.09253162599326,15.2,9.76130292410859));
#219861=CARTESIAN_POINT('Ctrl Pts',(4.09314131745173,15.2,9.76467936653761));
#219862=CARTESIAN_POINT('Ctrl Pts',(4.0938729471753,15.2,9.7687310973052));
#219863=CARTESIAN_POINT('Ctrl Pts',(4.09460105822206,15.2,9.77282576102715));
#219864=CARTESIAN_POINT('Ctrl Pts',(4.09532516594602,15.2,9.77696290579064));
#219865=CARTESIAN_POINT('Ctrl Pts',(4.09592858907126,15.2,9.78041052655215));
#219866=CARTESIAN_POINT('Ctrl Pts',(4.09652923191043,15.2,9.7838876503437));
#219867=CARTESIAN_POINT('Ctrl Pts',(4.09712681843845,15.2,9.78739401784129));
#219868=CARTESIAN_POINT('Ctrl Pts',(4.09784392231117,15.2,9.79160165906773));
#219869=CARTESIAN_POINT('Ctrl Pts',(4.09855662541143,15.2,9.79585141241445));
#219870=CARTESIAN_POINT('Ctrl Pts',(4.09926446231842,15.2,9.80014284169849));
#219871=CARTESIAN_POINT('Ctrl Pts',(4.09985432637543,15.2,9.80371903257362));
#219872=CARTESIAN_POINT('Ctrl Pts',(4.1004408106376,15.2,9.80732416323955));
#219873=CARTESIAN_POINT('Ctrl Pts',(4.10102365056785,15.2,9.81095798574189));
#219874=CARTESIAN_POINT('Ctrl Pts',(4.10160649049811,15.2,9.81459180824422));
#219875=CARTESIAN_POINT('Ctrl Pts',(4.10218568827552,15.2,9.81825432119145));
#219876=CARTESIAN_POINT('Ctrl Pts',(4.10276098160853,15.2,9.82194527799936));
#219877=CARTESIAN_POINT('Ctrl Pts',(4.10333627487884,15.2,9.82563623440494));
#219878=CARTESIAN_POINT('Ctrl Pts',(4.10390766569836,15.2,9.82935563570384));
#219879=CARTESIAN_POINT('Ctrl Pts',(4.10447489744243,15.2,9.83310323695974));
#219880=CARTESIAN_POINT('Ctrl Pts',(4.10504212924833,15.2,9.83685083862413));
#219881=CARTESIAN_POINT('Ctrl Pts',(4.10560520429875,15.2,9.8406266399436));
#219882=CARTESIAN_POINT('Ctrl Pts',(4.10616387166021,15.2,9.84443040001072));
#219883=CARTESIAN_POINT('Ctrl Pts',(4.1068342725305,15.2,9.84899491234003));
#219884=CARTESIAN_POINT('Ctrl Pts',(4.10749832390359,15.2,9.85359968430348));
#219885=CARTESIAN_POINT('Ctrl Pts',(4.10815560605519,15.2,9.85824430770765));
#219886=CARTESIAN_POINT('Ctrl Pts',(4.10903198219763,15.2,9.86443713849133));
#219887=CARTESIAN_POINT('Ctrl Pts',(4.1098963189273,15.2,9.87070080765411));
#219888=CARTESIAN_POINT('Ctrl Pts',(4.11074763902639,15.2,9.87703435845896));
#219889=CARTESIAN_POINT('Ctrl Pts',(4.11149254413484,15.2,9.88257621557503));
#219890=CARTESIAN_POINT('Ctrl Pts',(4.11222748327364,15.2,9.88817157693104));
#219891=CARTESIAN_POINT('Ctrl Pts',(4.1129518187843,15.2,9.8938198062443));
#219892=CARTESIAN_POINT('Ctrl Pts',(4.11346920122746,15.2,9.89785425525118));
#219893=CARTESIAN_POINT('Ctrl Pts',(4.1139811724329,15.2,9.90191568062968));
#219894=CARTESIAN_POINT('Ctrl Pts',(4.11448750668373,15.2,9.90600385122352));
#219895=CARTESIAN_POINT('Ctrl Pts',(4.11499384098974,15.2,9.91009202226297));
#219896=CARTESIAN_POINT('Ctrl Pts',(4.11549453634031,15.2,9.91420694031595));
#219897=CARTESIAN_POINT('Ctrl Pts',(4.11598937141023,15.2,9.9183483789249));
#219898=CARTESIAN_POINT('Ctrl Pts',(4.11648420648016,15.2,9.92248981753384));
#219899=CARTESIAN_POINT('Ctrl Pts',(4.11697317774711,15.2,9.92665777781657));
#219900=CARTESIAN_POINT('Ctrl Pts',(4.11745606874388,15.2,9.93085203649644));
#219901=CARTESIAN_POINT('Ctrl Pts',(4.11793895974064,15.2,9.93504629517632));
#219902=CARTESIAN_POINT('Ctrl Pts',(4.11841576885771,15.2,9.93926685075148));
#219903=CARTESIAN_POINT('Ctrl Pts',(4.11888627976082,15.2,9.94351348422233));
#219904=CARTESIAN_POINT('Ctrl Pts',(4.11926268850381,15.2,9.94691079118418));
#219905=CARTESIAN_POINT('Ctrl Pts',(4.11963506594078,15.2,9.95032478571192));
#219906=CARTESIAN_POINT('Ctrl Pts',(4.12000330423836,15.2,9.95375535928887));
#219907=CARTESIAN_POINT('Ctrl Pts',(4.12046360208525,15.2,9.95804357602636));
#219908=CARTESIAN_POINT('Ctrl Pts',(4.12091743116886,15.2,9.96235769282965));
#219909=CARTESIAN_POINT('Ctrl Pts',(4.12136458230185,15.2,9.96669749652046));
#219910=CARTESIAN_POINT('Ctrl Pts',(4.12172230317899,15.2,9.97016933918929));
#219911=CARTESIAN_POINT('Ctrl Pts',(4.12207575009686,15.2,9.97365761854002));
#219912=CARTESIAN_POINT('Ctrl Pts',(4.12242481701305,15.2,9.9771622276969));
#219913=CARTESIAN_POINT('Ctrl Pts',(4.12286115069396,15.2,9.98154298950111));
#219914=CARTESIAN_POINT('Ctrl Pts',(4.12329064037748,15.2,9.98594926316156));
#219915=CARTESIAN_POINT('Ctrl Pts',(4.12371308398896,15.2,9.99038083670192));
#219916=CARTESIAN_POINT('Ctrl Pts',(4.12413552760045,15.2,9.99481241024228));
#219917=CARTESIAN_POINT('Ctrl Pts',(4.12455092426453,15.2,9.99926928274387));
#219918=CARTESIAN_POINT('Ctrl Pts',(4.12495907301641,15.2,10.0037512438058));
#219919=CARTESIAN_POINT('Ctrl Pts',(4.1252855920357,15.2,10.0073368128508));
#219920=CARTESIAN_POINT('Ctrl Pts',(4.1256074734989,15.2,10.0109384374676));
#219921=CARTESIAN_POINT('Ctrl Pts',(4.12592461579348,15.2,10.0145560118331));
#219922=CARTESIAN_POINT('Ctrl Pts',(4.12624175804484,15.2,10.0181735857056));
#219923=CARTESIAN_POINT('Ctrl Pts',(4.12655416131349,15.2,10.0218071093511));
#219924=CARTESIAN_POINT('Ctrl Pts',(4.12686172623311,15.2,10.0254564747184));
#219925=CARTESIAN_POINT('Ctrl Pts',(4.12724618241406,15.2,10.0300181818004));
#219926=CARTESIAN_POINT('Ctrl Pts',(4.12762307822029,15.2,10.034604643732));
#219927=CARTESIAN_POINT('Ctrl Pts',(4.1279922212081,15.2,10.0392156531974));
#219928=CARTESIAN_POINT('Ctrl Pts',(4.12828753561444,15.2,10.0429044609708));
#219929=CARTESIAN_POINT('Ctrl Pts',(4.12857789050102,15.2,10.0466089790177));
#219930=CARTESIAN_POINT('Ctrl Pts',(4.12886318557161,15.2,10.0503291028332));
#219931=CARTESIAN_POINT('Ctrl Pts',(4.12914848060332,15.2,10.0540492261418));
#219932=CARTESIAN_POINT('Ctrl Pts',(4.12942871931069,15.2,10.0577849556955));
#219933=CARTESIAN_POINT('Ctrl Pts',(4.12970380251076,15.2,10.0615361869434));
#219934=CARTESIAN_POINT('Ctrl Pts',(4.13004765653896,15.2,10.0662252263866));
#219935=CARTESIAN_POINT('Ctrl Pts',(4.13038345989827,15.2,10.0709384862537));
#219936=CARTESIAN_POINT('Ctrl Pts',(4.13071102698312,15.2,10.0756757672474));
#219937=CARTESIAN_POINT('Ctrl Pts',(4.13103859406796,15.2,10.080413048241));
#219938=CARTESIAN_POINT('Ctrl Pts',(4.13135792418885,15.2,10.0851743487277));
#219939=CARTESIAN_POINT('Ctrl Pts',(4.1316688380083,15.2,10.0899594682416));
#219940=CARTESIAN_POINT('Ctrl Pts',(4.13191756907742,15.2,10.0937875640614));
#219941=CARTESIAN_POINT('Ctrl Pts',(4.13216091357368,15.2,10.0976309054384));
#219942=CARTESIAN_POINT('Ctrl Pts',(4.13239878053052,15.2,10.1014893893725));
#219943=CARTESIAN_POINT('Ctrl Pts',(4.13281504765639,15.2,10.1082417354685));
#219944=CARTESIAN_POINT('Ctrl Pts',(4.13321453556633,15.2,10.1150404585417));
#219945=CARTESIAN_POINT('Ctrl Pts',(4.13359676772372,15.2,10.121885016697));
#219946=CARTESIAN_POINT('Ctrl Pts',(4.13392439532547,15.2,10.1277517815153));
#219947=CARTESIAN_POINT('Ctrl Pts',(4.13423934530897,15.2,10.1336522210044));
#219948=CARTESIAN_POINT('Ctrl Pts',(4.13454131807455,15.2,10.1395860016634));
#219949=CARTESIAN_POINT('Ctrl Pts',(4.13474263322417,15.2,10.1435418548971));
#219950=CARTESIAN_POINT('Ctrl Pts',(4.13493818205335,15.2,10.1475125256216));
#219951=CARTESIAN_POINT('Ctrl Pts',(4.13512787848317,15.2,10.1514979149806));
#219952=CARTESIAN_POINT('Ctrl Pts',(4.13531757493884,15.2,10.1554833048825));
#219953=CARTESIAN_POINT('Ctrl Pts',(4.13550141856163,15.2,10.1594834133972));
#219954=CARTESIAN_POINT('Ctrl Pts',(4.13567932307072,15.2,10.163498143173));
#219955=CARTESIAN_POINT('Ctrl Pts',(4.13585722755556,15.2,10.1675128724018));
#219956=CARTESIAN_POINT('Ctrl Pts',(4.13602919410229,15.2,10.1715422222205));
#219957=CARTESIAN_POINT('Ctrl Pts',(4.13619513781135,15.2,10.1755860949445));
#219958=CARTESIAN_POINT('Ctrl Pts',(4.13640256746461,15.2,10.1806409362627));
#219959=CARTESIAN_POINT('Ctrl Pts',(4.13660058633153,15.2,10.1857184699899));
#219960=CARTESIAN_POINT('Ctrl Pts',(4.13678903272092,15.2,10.1908185071415));
#219961=CARTESIAN_POINT('Ctrl Pts',(4.13693978984065,15.2,10.1948985370852));
#219962=CARTESIAN_POINT('Ctrl Pts',(4.13708442016443,15.2,10.1989929704685));
#219963=CARTESIAN_POINT('Ctrl Pts',(4.13722284201169,15.2,10.2031017086212));
#219964=CARTESIAN_POINT('Ctrl Pts',(4.13739586931133,15.2,10.2082376310322));
#219965=CARTESIAN_POINT('Ctrl Pts',(4.13755919523751,15.2,10.2133959065313));
#219966=CARTESIAN_POINT('Ctrl Pts',(4.13771266252837,15.2,10.2185763486859));
#219967=CARTESIAN_POINT('Ctrl Pts',(4.13783543635102,15.2,10.2227207020708));
#219968=CARTESIAN_POINT('Ctrl Pts',(4.13795190084116,15.2,10.2268792417482));
#219969=CARTESIAN_POINT('Ctrl Pts',(4.13806197599924,15.2,10.2310518736839));
#219970=CARTESIAN_POINT('Ctrl Pts',(4.13817205117233,15.2,10.2352245061882));
#219971=CARTESIAN_POINT('Ctrl Pts',(4.13827573674334,15.2,10.2394112302085));
#219972=CARTESIAN_POINT('Ctrl Pts',(4.13837295453071,15.2,10.2436119510929));
#219973=CARTESIAN_POINT('Ctrl Pts',(4.13847017230483,15.2,10.247812671405));
#219974=CARTESIAN_POINT('Ctrl Pts',(4.13856092142448,15.2,10.2520273907232));
#219975=CARTESIAN_POINT('Ctrl Pts',(4.13864512525136,15.2,10.2562560121544));
#219976=CARTESIAN_POINT('Ctrl Pts',(4.13875038004356,15.2,10.2615417893755));
#219977=CARTESIAN_POINT('Ctrl Pts',(4.13884540651049,15.2,10.2668492926638));
#219978=CARTESIAN_POINT('Ctrl Pts',(4.13893005546937,15.2,10.2721783373849));
#219979=CARTESIAN_POINT('Ctrl Pts',(4.13904856401364,15.2,10.2796390001105));
#219980=CARTESIAN_POINT('Ctrl Pts',(4.13914672978642,15.2,10.287141886239));
#219981=CARTESIAN_POINT('Ctrl Pts',(4.13922415299519,15.2,10.2946865008442));
#219982=CARTESIAN_POINT('Ctrl Pts',(4.1392794552863,15.2,10.3000755111925));
#219983=CARTESIAN_POINT('Ctrl Pts',(4.13932417331936,15.2,10.3054858112375));
#219984=CARTESIAN_POINT('Ctrl Pts',(4.13935816248546,15.2,10.3109172233219));
#219985=CARTESIAN_POINT('Ctrl Pts',(4.13940574731505,15.2,10.3185211997665));
#219986=CARTESIAN_POINT('Ctrl Pts',(4.13943230593189,15.2,10.3261665530574));
#219987=CARTESIAN_POINT('Ctrl Pts',(4.13943744626615,15.2,10.3338527982568));
#219988=CARTESIAN_POINT('Ctrl Pts',(4.13944038360036,15.2,10.3382449388837));
#219989=CARTESIAN_POINT('Ctrl Pts',(4.13943632774502,15.2,10.3426504317452));
#219990=CARTESIAN_POINT('Ctrl Pts',(4.13942520696664,15.2,10.3470691870416));
#219991=CARTESIAN_POINT('Ctrl Pts',(4.13941408618825,15.2,10.351487942338));
#219992=CARTESIAN_POINT('Ctrl Pts',(4.13939590123127,15.2,10.3559199599165));
#219993=CARTESIAN_POINT('Ctrl Pts',(4.1393705805625,15.2,10.3603651504934));
#219994=CARTESIAN_POINT('Ctrl Pts',(4.13935159006264,15.2,10.3636990431232));
#219995=CARTESIAN_POINT('Ctrl Pts',(4.1393285859122,15.2,10.3670403445181));
#219996=CARTESIAN_POINT('Ctrl Pts',(4.13930153845303,15.2,10.3703890183979));
#219997=CARTESIAN_POINT('Ctrl Pts',(4.13927449099386,15.2,10.3737376922777));
#219998=CARTESIAN_POINT('Ctrl Pts',(4.13924340101181,15.2,10.3770937391549));
#219999=CARTESIAN_POINT('Ctrl Pts',(4.13920823847107,15.2,10.3804571194083));
#220000=CARTESIAN_POINT('Ctrl Pts',(4.13917307593033,15.2,10.3838204996618));
#220001=CARTESIAN_POINT('Ctrl Pts',(4.13913384128174,15.2,10.387191214256));
#220002=CARTESIAN_POINT('Ctrl Pts',(4.13909050528331,15.2,10.3905692264666));
#220003=CARTESIAN_POINT('Ctrl Pts',(4.13903272394683,15.2,10.3950732431565));
#220004=CARTESIAN_POINT('Ctrl Pts',(4.13896765179283,15.2,10.3995902342007));
#220005=CARTESIAN_POINT('Ctrl Pts',(4.13889521978813,15.2,10.4041201082823));
#220006=CARTESIAN_POINT('Ctrl Pts',(4.13884089578953,15.2,10.4075175135348));
#220007=CARTESIAN_POINT('Ctrl Pts',(4.13878243343915,15.2,10.4109221665295));
#220008=CARTESIAN_POINT('Ctrl Pts',(4.13871980202115,15.2,10.4143340304101));
#220009=CARTESIAN_POINT('Ctrl Pts',(4.1386362934676,15.2,10.4188831820444));
#220010=CARTESIAN_POINT('Ctrl Pts',(4.13854537695219,15.2,10.4234451519036));
#220011=CARTESIAN_POINT('Ctrl Pts',(4.13844698301628,15.2,10.4280198545844));
#220012=CARTESIAN_POINT('Ctrl Pts',(4.138373187561,15.2,10.4314508817508));
#220013=CARTESIAN_POINT('Ctrl Pts',(4.138295186781,15.2,10.4348890705417));
#220014=CARTESIAN_POINT('Ctrl Pts',(4.1382129537429,15.2,10.4383343837489));
#220015=CARTESIAN_POINT('Ctrl Pts',(4.13813072068985,15.2,10.4417796975819));
#220016=CARTESIAN_POINT('Ctrl Pts',(4.13804425424396,15.2,10.4452321364837));
#220017=CARTESIAN_POINT('Ctrl Pts',(4.13795352718853,15.2,10.4486916642374));
#220018=CARTESIAN_POINT('Ctrl Pts',(4.13783255780875,15.2,10.4533043668616));
#220019=CARTESIAN_POINT('Ctrl Pts',(4.13770401406731,15.2,10.4579296708271));
#220020=CARTESIAN_POINT('Ctrl Pts',(4.13756783196673,15.2,10.4625674902468));
#220021=CARTESIAN_POINT('Ctrl Pts',(4.13746569538666,15.2,10.4660458549695));
#220022=CARTESIAN_POINT('Ctrl Pts',(4.13735926044091,15.2,10.4695312592136));
#220023=CARTESIAN_POINT('Ctrl Pts',(4.13724850327864,15.2,10.4730236678777));
#220024=CARTESIAN_POINT('Ctrl Pts',(4.13713774611637,15.2,10.4765160765419));
#220025=CARTESIAN_POINT('Ctrl Pts',(4.13702266387107,15.2,10.4800154892972));
#220026=CARTESIAN_POINT('Ctrl Pts',(4.13690323179267,15.2,10.4835218690439));
#220027=CARTESIAN_POINT('Ctrl Pts',(4.13678379969258,15.2,10.4870282494276));
#220028=CARTESIAN_POINT('Ctrl Pts',(4.13666001659125,15.2,10.4905415976715));
#220029=CARTESIAN_POINT('Ctrl Pts',(4.13653185703036,15.2,10.4940618780174));
#220030=CARTESIAN_POINT('Ctrl Pts',(4.13640369749276,15.2,10.4975821577237));
#220031=CARTESIAN_POINT('Ctrl Pts',(4.13627116044248,15.2,10.5011093691015));
#220032=CARTESIAN_POINT('Ctrl Pts',(4.13613421998177,15.2,10.5046434769421));
#220033=CARTESIAN_POINT('Ctrl Pts',(4.13599727952106,15.2,10.5081775847827));
#220034=CARTESIAN_POINT('Ctrl Pts',(4.13585593624577,15.2,10.511718587915));
#220035=CARTESIAN_POINT('Ctrl Pts',(4.13571016329234,15.2,10.5152664516618));
#220036=CARTESIAN_POINT('Ctrl Pts',(4.13556439033892,15.2,10.5188143154085));
#220037=CARTESIAN_POINT('Ctrl Pts',(4.13541418817769,15.2,10.522369040246));
#220038=CARTESIAN_POINT('Ctrl Pts',(4.13525953026665,15.2,10.5259305894916));
#220039=CARTESIAN_POINT('Ctrl Pts',(4.1351048723556,15.2,10.5294921387373));
#220040=CARTESIAN_POINT('Ctrl Pts',(4.1349457595614,15.2,10.5330605128742));
#220041=CARTESIAN_POINT('Ctrl Pts',(4.13478216602607,15.2,10.5366356761187));
#220042=CARTESIAN_POINT('Ctrl Pts',(4.13461857249073,15.2,10.5402108393632));
#220043=CARTESIAN_POINT('Ctrl Pts',(4.13445049713071,15.2,10.5437927921822));
#220044=CARTESIAN_POINT('Ctrl Pts',(4.13427791659593,15.2,10.5473814989676));
#220045=CARTESIAN_POINT('Ctrl Pts',(4.13410533602979,15.2,10.5509702064049));
#220046=CARTESIAN_POINT('Ctrl Pts',(4.13392824853739,15.2,10.5545656691775));
#220047=CARTESIAN_POINT('Ctrl Pts',(4.13374663092704,15.2,10.5581678505352));
#220048=CARTESIAN_POINT('Ctrl Pts',(4.13356501334969,15.2,10.5617700312386));
#220049=CARTESIAN_POINT('Ctrl Pts',(4.13337886303283,15.2,10.5653789302828));
#220050=CARTESIAN_POINT('Ctrl Pts',(4.13318815748803,15.2,10.5689945137079));
#220051=CARTESIAN_POINT('Ctrl Pts',(4.13293388343986,15.2,10.573815291389));
#220052=CARTESIAN_POINT('Ctrl Pts',(4.1326715094077,15.2,10.5786479524786));
#220053=CARTESIAN_POINT('Ctrl Pts',(4.13240097626368,15.2,10.5834924126374));
#220054=CARTESIAN_POINT('Ctrl Pts',(4.13219807639645,15.2,10.5871257579214));
#220055=CARTESIAN_POINT('Ctrl Pts',(4.13199058845455,15.2,10.5907657411383));
#220056=CARTESIAN_POINT('Ctrl Pts',(4.13177848604621,15.2,10.5944123269217));
#220057=CARTESIAN_POINT('Ctrl Pts',(4.13156638359935,15.2,10.5980589133674));
#220058=CARTESIAN_POINT('Ctrl Pts',(4.13134966745119,15.2,10.6017121030983));
#220059=CARTESIAN_POINT('Ctrl Pts',(4.13112831396005,15.2,10.6053718605478));
#220060=CARTESIAN_POINT('Ctrl Pts',(4.13090696050913,15.2,10.6090316173324));
#220061=CARTESIAN_POINT('Ctrl Pts',(4.13068096965899,15.2,10.6126979435431));
#220062=CARTESIAN_POINT('Ctrl Pts',(4.13045031673864,15.2,10.6163708024689));
#220063=CARTESIAN_POINT('Ctrl Pts',(4.13006589519075,15.2,10.6224922342344));
#220064=CARTESIAN_POINT('Ctrl Pts',(4.12966852321958,15.2,10.6286318142261));
#220065=CARTESIAN_POINT('Ctrl Pts',(4.12925809245462,15.2,10.6347893840887));
#220066=CARTESIAN_POINT('Ctrl Pts',(4.12901183400459,15.2,10.638483925872));
#220067=CARTESIAN_POINT('Ctrl Pts',(4.12876087461315,15.2,10.642184944855));
#220068=CARTESIAN_POINT('Ctrl Pts',(4.12850519070536,15.2,10.6458924065958));
#220069=CARTESIAN_POINT('Ctrl Pts',(4.12824950679757,15.2,10.6495998683367));
#220070=CARTESIAN_POINT('Ctrl Pts',(4.12798909899133,15.2,10.6533137731049));
#220071=CARTESIAN_POINT('Ctrl Pts',(4.12772394249973,15.2,10.6570340857783));
#220072=CARTESIAN_POINT('Ctrl Pts',(4.12745878600814,15.2,10.6607543984518));
#220073=CARTESIAN_POINT('Ctrl Pts',(4.12718888029147,15.2,10.6644811186819));
#220074=CARTESIAN_POINT('Ctrl Pts',(4.12691420330023,15.2,10.6682142110215));
#220075=CARTESIAN_POINT('Ctrl Pts',(4.12663952630898,15.2,10.6719473033612));
#220076=CARTESIAN_POINT('Ctrl Pts',(4.12636007615346,15.2,10.6756867686784));
#220077=CARTESIAN_POINT('Ctrl Pts',(4.12607583428921,15.2,10.6794325760418));
#220078=CARTESIAN_POINT('Ctrl Pts',(4.12569684510245,15.2,10.6844269863132));
#220079=CARTESIAN_POINT('Ctrl Pts',(4.12530933671467,15.2,10.6894326749582));
#220080=CARTESIAN_POINT('Ctrl Pts',(4.12491325519252,15.2,10.6944495576769));
#220081=CARTESIAN_POINT('Ctrl Pts',(4.12461619407789,15.2,10.698212219374));
#220082=CARTESIAN_POINT('Ctrl Pts',(4.1243143083233,15.2,10.7019811777401));
#220083=CARTESIAN_POINT('Ctrl Pts',(4.12400757229137,15.2,10.7057563909534));
#220084=CARTESIAN_POINT('Ctrl Pts',(4.1234963455529,15.2,10.7120484132042));
#220085=CARTESIAN_POINT('Ctrl Pts',(4.12297163538237,15.2,10.7183577989103));
#220086=CARTESIAN_POINT('Ctrl Pts',(4.12243337123359,15.2,10.7246844426642));
#220087=CARTESIAN_POINT('Ctrl Pts',(4.12211041275606,15.2,10.7284804287786));
#220088=CARTESIAN_POINT('Ctrl Pts',(4.12178257806039,15.2,10.7322826273081));
#220089=CARTESIAN_POINT('Ctrl Pts',(4.12144986799994,15.2,10.736091048));
#220090=CARTESIAN_POINT('Ctrl Pts',(4.04260911699994,12.2,9.55499537099998));
#220091=CARTESIAN_POINT('Ctrl Pts',(4.0431612978139,12.2,9.55669455126485));
#220092=CARTESIAN_POINT('Ctrl Pts',(4.04372605441455,12.2,9.55844976666689));
#220093=CARTESIAN_POINT('Ctrl Pts',(4.0443024457118,12.2,9.56026027830994));
#220094=CARTESIAN_POINT('Ctrl Pts',(4.04488161665923,12.2,9.56207952115529));
#220095=CARTESIAN_POINT('Ctrl Pts',(4.04547254566134,12.2,9.5639546011486));
#220096=CARTESIAN_POINT('Ctrl Pts',(4.04607433355817,12.2,9.56588480618675));
#220097=CARTESIAN_POINT('Ctrl Pts',(4.04667612140033,12.2,9.56781501104957));
#220098=CARTESIAN_POINT('Ctrl Pts',(4.0472887675309,12.2,9.56980034131573));
#220099=CARTESIAN_POINT('Ctrl Pts',(4.04791140625826,12.2,9.57184010199156));
#220100=CARTESIAN_POINT('Ctrl Pts',(4.04853404498562,12.2,9.57387986266738));
#220101=CARTESIAN_POINT('Ctrl Pts',(4.04916667256298,12.2,9.57597405404106));
#220102=CARTESIAN_POINT('Ctrl Pts',(4.04980844773787,12.2,9.5781219999839));
#220103=CARTESIAN_POINT('Ctrl Pts',(4.05045022297105,12.2,9.58026994612186));
#220104=CARTESIAN_POINT('Ctrl Pts',(4.05110114566863,12.2,9.58247164636916));
#220105=CARTESIAN_POINT('Ctrl Pts',(4.05176039887179,12.2,9.58472644049568));
#220106=CARTESIAN_POINT('Ctrl Pts',(4.05241965201507,12.2,9.58698123441737));
#220107=CARTESIAN_POINT('Ctrl Pts',(4.05308723453836,12.2,9.58928912179259));
#220108=CARTESIAN_POINT('Ctrl Pts',(4.05376235301691,12.2,9.59164945971764));
#220109=CARTESIAN_POINT('Ctrl Pts',(4.05443747149546,12.2,9.59400979764269));
#220110=CARTESIAN_POINT('Ctrl Pts',(4.05512012665439,12.2,9.59642258494925));
#220111=CARTESIAN_POINT('Ctrl Pts',(4.05580954896239,12.2,9.59888719110747));
#220112=CARTESIAN_POINT('Ctrl Pts',(4.05649897133301,12.2,9.60135179748954));
#220113=CARTESIAN_POINT('Ctrl Pts',(4.05719515735446,12.2,9.60386822484468));
#220114=CARTESIAN_POINT('Ctrl Pts',(4.05789736205981,12.2,9.60643585623811));
#220115=CARTESIAN_POINT('Ctrl Pts',(4.05859956670138,12.2,9.60900348739833));
#220116=CARTESIAN_POINT('Ctrl Pts',(4.05930778806454,12.2,9.6116223227904));
#220117=CARTESIAN_POINT('Ctrl Pts',(4.06002130053884,12.2,9.61429176086226));
#220118=CARTESIAN_POINT('Ctrl Pts',(4.06073481301314,12.2,9.61696119893412));
#220119=CARTESIAN_POINT('Ctrl Pts',(4.06145361427035,12.2,9.6196812398353));
#220120=CARTESIAN_POINT('Ctrl Pts',(4.06217699974386,12.2,9.62245129406581));
#220121=CARTESIAN_POINT('Ctrl Pts',(4.06290038521737,12.2,9.6252213482963));
#220122=CARTESIAN_POINT('Ctrl Pts',(4.06362835112202,12.2,9.62804141806142));
#220123=CARTESIAN_POINT('Ctrl Pts',(4.06436021384517,12.2,9.6309109224538));
#220124=CARTESIAN_POINT('Ctrl Pts',(4.06509207663479,12.2,9.63378042710684));
#220125=CARTESIAN_POINT('Ctrl Pts',(4.06582783371649,12.2,9.63669936978133));
#220126=CARTESIAN_POINT('Ctrl Pts',(4.06656681575689,12.2,9.63966718444519));
#220127=CARTESIAN_POINT('Ctrl Pts',(4.06730579773018,12.2,9.64263499883946));
#220128=CARTESIAN_POINT('Ctrl Pts',(4.06804800688995,12.2,9.64565168593774));
#220129=CARTESIAN_POINT('Ctrl Pts',(4.06879278803294,12.2,9.64871669225687));
#220130=CARTESIAN_POINT('Ctrl Pts',(4.06953756917592,12.2,9.65178169857599));
#220131=CARTESIAN_POINT('Ctrl Pts',(4.07028492497895,12.2,9.65489502280677));
#220132=CARTESIAN_POINT('Ctrl Pts',(4.07103421911827,12.2,9.65805612418869));
#220133=CARTESIAN_POINT('Ctrl Pts',(4.07178351332565,12.2,9.66121722585776));
#220134=CARTESIAN_POINT('Ctrl Pts',(4.07253474754156,12.2,9.66442610392306));
#220135=CARTESIAN_POINT('Ctrl Pts',(4.07328730183263,12.2,9.6676822256859));
#220136=CARTESIAN_POINT('Ctrl Pts',(4.07403985605534,12.2,9.67093834715298));
#220137=CARTESIAN_POINT('Ctrl Pts',(4.07479373107359,12.2,9.67424171311334));
#220138=CARTESIAN_POINT('Ctrl Pts',(4.07554832521627,12.2,9.67759179975672));
#220139=CARTESIAN_POINT('Ctrl Pts',(4.07630291935894,12.2,9.68094188640011));
#220140=CARTESIAN_POINT('Ctrl Pts',(4.07705823111172,12.2,9.68433869551952));
#220141=CARTESIAN_POINT('Ctrl Pts',(4.0778136744176,12.2,9.6877817138913));
#220142=CARTESIAN_POINT('Ctrl Pts',(4.0785691177921,12.2,9.69122473257582));
#220143=CARTESIAN_POINT('Ctrl Pts',(4.07932469217746,12.2,9.6947139586617));
#220144=CARTESIAN_POINT('Ctrl Pts',(4.08007982558966,12.2,9.69824889161697));
#220145=CARTESIAN_POINT('Ctrl Pts',(4.08083495893326,12.2,9.70178382425116));
#220146=CARTESIAN_POINT('Ctrl Pts',(4.08158964903567,12.2,9.70536446135665));
#220147=CARTESIAN_POINT('Ctrl Pts',(4.08234334125828,12.2,9.70899030897491));
#220148=CARTESIAN_POINT('Ctrl Pts',(4.0830970334809,12.2,9.71261615659317));
#220149=CARTESIAN_POINT('Ctrl Pts',(4.08384972224196,12.2,9.71628721561753));
#220150=CARTESIAN_POINT('Ctrl Pts',(4.08460086866894,12.2,9.72000299758223));
#220151=CARTESIAN_POINT('Ctrl Pts',(4.08535201516417,12.2,9.72371877988444));
#220152=CARTESIAN_POINT('Ctrl Pts',(4.08610161564083,12.2,9.72747928717927));
#220153=CARTESIAN_POINT('Ctrl Pts',(4.08684913834809,12.2,9.73128404013963));
#220154=CARTESIAN_POINT('Ctrl Pts',(4.08759666098745,12.2,9.73508879275439));
#220155=CARTESIAN_POINT('Ctrl Pts',(4.08834210619891,12.2,9.738937788817));
#220156=CARTESIAN_POINT('Ctrl Pts',(4.08908495475862,12.2,9.74283056244335));
#220157=CARTESIAN_POINT('Ctrl Pts',(4.08982780331833,12.2,9.74672333606969));
#220158=CARTESIAN_POINT('Ctrl Pts',(4.09056805483641,12.2,9.75065988392134));
#220159=CARTESIAN_POINT('Ctrl Pts',(4.09130520247643,12.2,9.75463974452485));
#220160=CARTESIAN_POINT('Ctrl Pts',(4.09191949219876,12.2,9.75795629514829));
#220161=CARTESIAN_POINT('Ctrl Pts',(4.09253162599326,12.2,9.76130292410859));
#220162=CARTESIAN_POINT('Ctrl Pts',(4.09314131745173,12.2,9.76467936653761));
#220163=CARTESIAN_POINT('Ctrl Pts',(4.0938729471753,12.2,9.7687310973052));
#220164=CARTESIAN_POINT('Ctrl Pts',(4.09460105822206,12.2,9.77282576102715));
#220165=CARTESIAN_POINT('Ctrl Pts',(4.09532516594602,12.2,9.77696290579064));
#220166=CARTESIAN_POINT('Ctrl Pts',(4.09592858907126,12.2,9.78041052655215));
#220167=CARTESIAN_POINT('Ctrl Pts',(4.09652923191043,12.2,9.7838876503437));
#220168=CARTESIAN_POINT('Ctrl Pts',(4.09712681843845,12.2,9.78739401784129));
#220169=CARTESIAN_POINT('Ctrl Pts',(4.09772440496648,12.2,9.79090038533889));
#220170=CARTESIAN_POINT('Ctrl Pts',(4.09831893554042,12.2,9.794435997949));
#220171=CARTESIAN_POINT('Ctrl Pts',(4.09891014043131,12.2,9.79800060152789));
#220172=CARTESIAN_POINT('Ctrl Pts',(4.09950134532219,12.2,9.80156520510676));
#220173=CARTESIAN_POINT('Ctrl Pts',(4.10008922479487,12.2,9.80515879973693));
#220174=CARTESIAN_POINT('Ctrl Pts',(4.10067351146172,12.2,9.80878113626318));
#220175=CARTESIAN_POINT('Ctrl Pts',(4.10125779812857,12.2,9.81240347278944));
#220176=CARTESIAN_POINT('Ctrl Pts',(4.10183849408423,12.2,9.81605454833873));
#220177=CARTESIAN_POINT('Ctrl Pts',(4.10241533894554,12.2,9.81973411826777));
#220178=CARTESIAN_POINT('Ctrl Pts',(4.10299218380685,12.2,9.82341368819682));
#220179=CARTESIAN_POINT('Ctrl Pts',(4.10356517649705,12.2,9.82712175171432));
#220180=CARTESIAN_POINT('Ctrl Pts',(4.10413406149964,12.2,9.83085806277287));
#220181=CARTESIAN_POINT('Ctrl Pts',(4.10470294650224,12.2,9.83459437383143));
#220182=CARTESIAN_POINT('Ctrl Pts',(4.10526772542774,12.2,9.83835893475549));
#220183=CARTESIAN_POINT('Ctrl Pts',(4.10582814473329,12.2,9.84215150149158));
#220184=CARTESIAN_POINT('Ctrl Pts',(4.10638856403884,12.2,9.84594406822768));
#220185=CARTESIAN_POINT('Ctrl Pts',(4.10694462623665,12.2,9.84976464218446));
#220186=CARTESIAN_POINT('Ctrl Pts',(4.10749608297526,12.2,9.85361298324368));
#220187=CARTESIAN_POINT('Ctrl Pts',(4.10804753971386,12.2,9.8574613243029));
#220188=CARTESIAN_POINT('Ctrl Pts',(4.10859439337452,12.2,9.86133743518729));
#220189=CARTESIAN_POINT('Ctrl Pts',(4.10913639927704,12.2,9.86524107602204));
#220190=CARTESIAN_POINT('Ctrl Pts',(4.10967840517957,12.2,9.86914471685678));
#220191=CARTESIAN_POINT('Ctrl Pts',(4.11021556395721,12.2,9.87307588915198));
#220192=CARTESIAN_POINT('Ctrl Pts',(4.11074763902639,12.2,9.87703435845895));
#220193=CARTESIAN_POINT('Ctrl Pts',(4.1113861290862,12.2,9.88178452145474));
#220194=CARTESIAN_POINT('Ctrl Pts',(4.11201729881327,12.2,9.88657399363908));
#220195=CARTESIAN_POINT('Ctrl Pts',(4.11264074220761,12.2,9.89140237454526));
#220196=CARTESIAN_POINT('Ctrl Pts',(4.11316027838845,12.2,9.89542602544662));
#220197=CARTESIAN_POINT('Ctrl Pts',(4.11367445135847,12.2,9.89947669700703));
#220198=CARTESIAN_POINT('Ctrl Pts',(4.11418303149968,12.2,9.9035541604977));
#220199=CARTESIAN_POINT('Ctrl Pts',(4.1146916116409,12.2,9.90763162398837));
#220200=CARTESIAN_POINT('Ctrl Pts',(4.11519459879996,12.2,9.9117358788221));
#220201=CARTESIAN_POINT('Ctrl Pts',(4.1156917690083,12.2,9.91586670055825));
#220202=CARTESIAN_POINT('Ctrl Pts',(4.11608950519664,12.2,9.91917135812728));
#220203=CARTESIAN_POINT('Ctrl Pts',(4.11648351887066,12.2,9.92249301716767));
#220204=CARTESIAN_POINT('Ctrl Pts',(4.11687369511375,12.2,9.92583156479579));
#220205=CARTESIAN_POINT('Ctrl Pts',(4.11726387130368,12.2,9.92917011196903));
#220206=CARTESIAN_POINT('Ctrl Pts',(4.11765021167921,12.2,9.93252554748861));
#220207=CARTESIAN_POINT('Ctrl Pts',(4.11803260498303,12.2,9.93589775550596));
#220208=CARTESIAN_POINT('Ctrl Pts',(4.11841499833896,12.2,9.93926996398276));
#220209=CARTESIAN_POINT('Ctrl Pts',(4.11879344282729,12.2,9.94265894858054));
#220210=CARTESIAN_POINT('Ctrl Pts',(4.1191678285695,12.2,9.94606459232342));
#220211=CARTESIAN_POINT('Ctrl Pts',(4.11954221426071,12.2,9.94947023560229));
#220212=CARTESIAN_POINT('Ctrl Pts',(4.11991254320243,12.2,9.95289254099839));
#220213=CARTESIAN_POINT('Ctrl Pts',(4.12027870522832,12.2,9.95633139499395));
#220214=CARTESIAN_POINT('Ctrl Pts',(4.1206448673041,12.2,9.95977024945805));
#220215=CARTESIAN_POINT('Ctrl Pts',(4.12100686137596,12.2,9.9632256533786));
#220216=CARTESIAN_POINT('Ctrl Pts',(4.12136458230185,12.2,9.96669749652046));
#220217=CARTESIAN_POINT('Ctrl Pts',(4.12172230317899,12.2,9.97016933918929));
#220218=CARTESIAN_POINT('Ctrl Pts',(4.12207575009686,12.2,9.97365761854002));
#220219=CARTESIAN_POINT('Ctrl Pts',(4.12242481701305,12.2,9.9771622276969));
#220220=CARTESIAN_POINT('Ctrl Pts',(4.12286115069396,12.2,9.98154298950111));
#220221=CARTESIAN_POINT('Ctrl Pts',(4.12329064037748,12.2,9.98594926316156));
#220222=CARTESIAN_POINT('Ctrl Pts',(4.12371308398896,12.2,9.99038083670192));
#220223=CARTESIAN_POINT('Ctrl Pts',(4.12405103889657,12.2,9.99392609572743));
#220224=CARTESIAN_POINT('Ctrl Pts',(4.12438448329148,12.2,9.99748754523291));
#220225=CARTESIAN_POINT('Ctrl Pts',(4.12471331554765,12.2,10.0010650797191));
#220226=CARTESIAN_POINT('Ctrl Pts',(4.12504214775902,12.2,10.0046426137179));
#220227=CARTESIAN_POINT('Ctrl Pts',(4.12536636639683,12.2,10.0082362298622));
#220228=CARTESIAN_POINT('Ctrl Pts',(4.12568587198213,12.2,10.011845822455));
#220229=CARTESIAN_POINT('Ctrl Pts',(4.12600537761096,12.2,10.0154554155395));
#220230=CARTESIAN_POINT('Ctrl Pts',(4.12632016853646,12.2,10.019080983901));
#220231=CARTESIAN_POINT('Ctrl Pts',(4.12663014677526,12.2,10.0227224228228));
#220232=CARTESIAN_POINT('Ctrl Pts',(4.12694012497183,12.2,10.0263638612484));
#220233=CARTESIAN_POINT('Ctrl Pts',(4.12724528829049,12.2,10.0300211667268));
#220234=CARTESIAN_POINT('Ctrl Pts',(4.12754554044803,12.2,10.033694237442));
#220235=CARTESIAN_POINT('Ctrl Pts',(4.12784579264649,12.2,10.0373673086577));
#220236=CARTESIAN_POINT('Ctrl Pts',(4.12814113082482,12.2,10.0410561426972));
#220237=CARTESIAN_POINT('Ctrl Pts',(4.12843146050698,12.2,10.0447606345112));
#220238=CARTESIAN_POINT('Ctrl Pts',(4.12872179014959,12.2,10.0484651258205));
#220239=CARTESIAN_POINT('Ctrl Pts',(4.12900710847098,12.2,10.0521852753267));
#220240=CARTESIAN_POINT('Ctrl Pts',(4.12928732267081,12.2,10.0559209786308));
#220241=CARTESIAN_POINT('Ctrl Pts',(4.12956753690882,12.2,10.0596566824439));
#220242=CARTESIAN_POINT('Ctrl Pts',(4.12984264371201,12.2,10.0634079399884));
#220243=CARTESIAN_POINT('Ctrl Pts',(4.13011255128348,12.2,10.0671746477108));
#220244=CARTESIAN_POINT('Ctrl Pts',(4.13038245881818,12.2,10.0709413549201));
#220245=CARTESIAN_POINT('Ctrl Pts',(4.13064716516154,12.2,10.074723511891));
#220246=CARTESIAN_POINT('Ctrl Pts',(4.13090657747422,12.2,10.0785210159124));
#220247=CARTESIAN_POINT('Ctrl Pts',(4.13116598982223,12.2,10.0823185204511));
#220248=CARTESIAN_POINT('Ctrl Pts',(4.13142010693919,12.2,10.0861313724218));
#220249=CARTESIAN_POINT('Ctrl Pts',(4.1316688380083,12.2,10.0899594682416));
#220250=CARTESIAN_POINT('Ctrl Pts',(4.13191756907742,12.2,10.0937875640614));
#220251=CARTESIAN_POINT('Ctrl Pts',(4.13216091357368,12.2,10.0976309054384));
#220252=CARTESIAN_POINT('Ctrl Pts',(4.13239878053052,12.2,10.1014893893725));
#220253=CARTESIAN_POINT('Ctrl Pts',(4.13263664745496,12.2,10.1053478727808));
#220254=CARTESIAN_POINT('Ctrl Pts',(4.13286903463675,12.2,10.1092214997754));
#220255=CARTESIAN_POINT('Ctrl Pts',(4.13309585500814,12.2,10.1131101690306));
#220256=CARTESIAN_POINT('Ctrl Pts',(4.13332267541044,12.2,10.1169988388157));
#220257=CARTESIAN_POINT('Ctrl Pts',(4.13354392838237,12.2,10.1209025507894));
#220258=CARTESIAN_POINT('Ctrl Pts',(4.13375952356021,12.2,10.1248212046156));
#220259=CARTESIAN_POINT('Ctrl Pts',(4.13397511870868,12.2,10.1287398579079));
#220260=CARTESIAN_POINT('Ctrl Pts',(4.1341850578162,12.2,10.1326734524482));
#220261=CARTESIAN_POINT('Ctrl Pts',(4.13438925146655,12.2,10.1366218904023));
#220262=CARTESIAN_POINT('Ctrl Pts',(4.13459344514473,12.2,10.1405703288943));
#220263=CARTESIAN_POINT('Ctrl Pts',(4.13479189309994,12.2,10.1445336099077));
#220264=CARTESIAN_POINT('Ctrl Pts',(4.13498451028622,12.2,10.1485116346023));
#220265=CARTESIAN_POINT('Ctrl Pts',(4.13517712744625,12.2,10.1524896587548));
#220266=CARTESIAN_POINT('Ctrl Pts',(4.13536391402175,12.2,10.1564824252816));
#220267=CARTESIAN_POINT('Ctrl Pts',(4.13554478245179,12.2,10.1604898378975));
#220268=CARTESIAN_POINT('Ctrl Pts',(4.13577086800783,12.2,10.1654991040767));
#220269=CARTESIAN_POINT('Ctrl Pts',(4.13598770815807,12.2,10.1705312536262));
#220270=CARTESIAN_POINT('Ctrl Pts',(4.13619513781135,12.2,10.1755860949445));
#220271=CARTESIAN_POINT('Ctrl Pts',(4.13640256746461,12.2,10.1806409362627));
#220272=CARTESIAN_POINT('Ctrl Pts',(4.13660058633153,12.2,10.1857184699899));
#220273=CARTESIAN_POINT('Ctrl Pts',(4.13678903272092,12.2,10.1908185071415));
#220274=CARTESIAN_POINT('Ctrl Pts',(4.13693978984065,12.2,10.1948985370852));
#220275=CARTESIAN_POINT('Ctrl Pts',(4.13708442016443,12.2,10.1989929704685));
#220276=CARTESIAN_POINT('Ctrl Pts',(4.13722284201169,12.2,10.2031017086212));
#220277=CARTESIAN_POINT('Ctrl Pts',(4.13736126384008,12.2,10.2072104462141));
#220278=CARTESIAN_POINT('Ctrl Pts',(4.13749347726061,12.2,10.2113334899177));
#220279=CARTESIAN_POINT('Ctrl Pts',(4.13761940047295,12.2,10.2154707439118));
#220280=CARTESIAN_POINT('Ctrl Pts',(4.13777680450124,12.2,10.2206423118273));
#220281=CARTESIAN_POINT('Ctrl Pts',(4.13792438204039,12.2,10.2258360833379));
#220282=CARTESIAN_POINT('Ctrl Pts',(4.13806197599924,12.2,10.2310518736839));
#220283=CARTESIAN_POINT('Ctrl Pts',(4.13817205117233,12.2,10.2352245061882));
#220284=CARTESIAN_POINT('Ctrl Pts',(4.13827573674334,12.2,10.2394112302085));
#220285=CARTESIAN_POINT('Ctrl Pts',(4.13837295453071,12.2,10.2436119510929));
#220286=CARTESIAN_POINT('Ctrl Pts',(4.13847017230483,12.2,10.247812671405));
#220287=CARTESIAN_POINT('Ctrl Pts',(4.13856092142448,12.2,10.2520273907232));
#220288=CARTESIAN_POINT('Ctrl Pts',(4.13864512525136,12.2,10.2562560121544));
#220289=CARTESIAN_POINT('Ctrl Pts',(4.13872932908971,12.2,10.2604846341617));
#220290=CARTESIAN_POINT('Ctrl Pts',(4.13880698679672,12.2,10.2647271612513));
#220291=CARTESIAN_POINT('Ctrl Pts',(4.13887802202238,12.2,10.268983497873));
#220292=CARTESIAN_POINT('Ctrl Pts',(4.13894905723836,12.2,10.2732398339148));
#220293=CARTESIAN_POINT('Ctrl Pts',(4.13901346866503,12.2,10.2775099805213));
#220294=CARTESIAN_POINT('Ctrl Pts',(4.13907118244156,12.2,10.2817938448284));
#220295=CARTESIAN_POINT('Ctrl Pts',(4.13912889622595,12.2,10.2860777097191));
#220296=CARTESIAN_POINT('Ctrl Pts',(4.13917991115988,12.2,10.2903752923306));
#220297=CARTESIAN_POINT('Ctrl Pts',(4.13922415299519,12.2,10.2946865008442));
#220298=CARTESIAN_POINT('Ctrl Pts',(4.13926839482446,12.2,10.2989977087704));
#220299=CARTESIAN_POINT('Ctrl Pts',(4.13930586282732,12.2,10.3033225425717));
#220300=CARTESIAN_POINT('Ctrl Pts',(4.13933648276996,12.2,10.3076609100489));
#220301=CARTESIAN_POINT('Ctrl Pts',(4.13936710271677,12.2,10.3119992781173));
#220302=CARTESIAN_POINT('Ctrl Pts',(4.13939087517956,12.2,10.3163511809951));
#220303=CARTESIAN_POINT('Ctrl Pts',(4.13940772645831,12.2,10.3207165262529));
#220304=CARTESIAN_POINT('Ctrl Pts',(4.13942457773477,12.2,10.3250818709159));
#220305=CARTESIAN_POINT('Ctrl Pts',(4.13943450893234,12.2,10.3294606582283));
#220306=CARTESIAN_POINT('Ctrl Pts',(4.13943744626615,12.2,10.3338527982568));
#220307=CARTESIAN_POINT('Ctrl Pts',(4.13944038360036,12.2,10.3382449388837));
#220308=CARTESIAN_POINT('Ctrl Pts',(4.13943632774502,12.2,10.3426504317452));
#220309=CARTESIAN_POINT('Ctrl Pts',(4.13942520696664,12.2,10.3470691870416));
#220310=CARTESIAN_POINT('Ctrl Pts',(4.13941130599442,12.2,10.3525926308611));
#220311=CARTESIAN_POINT('Ctrl Pts',(4.13938636682792,12.2,10.3581367976721));
#220312=CARTESIAN_POINT('Ctrl Pts',(4.13935025092495,12.2,10.363701510753));
#220313=CARTESIAN_POINT('Ctrl Pts',(4.13932135820494,12.2,10.3681532808538));
#220314=CARTESIAN_POINT('Ctrl Pts',(4.13928531276943,12.2,10.3726182011825));
#220315=CARTESIAN_POINT('Ctrl Pts',(4.13924204477371,12.2,10.3770961837595));
#220316=CARTESIAN_POINT('Ctrl Pts',(4.13920959376955,12.2,10.3804546714548));
#220317=CARTESIAN_POINT('Ctrl Pts',(4.13917308026424,12.2,10.383820504994));
#220318=CARTESIAN_POINT('Ctrl Pts',(4.13913247521612,12.2,10.387193648777));
#220319=CARTESIAN_POINT('Ctrl Pts',(4.13909187017537,12.2,10.3905667919471));
#220320=CARTESIAN_POINT('Ctrl Pts',(4.13904717384317,12.2,10.3939472448917));
#220321=CARTESIAN_POINT('Ctrl Pts',(4.13899835680292,12.2,10.3973349706027));
#220322=CARTESIAN_POINT('Ctrl Pts',(4.13893326741887,12.2,10.4018519380121));
#220323=CARTESIAN_POINT('Ctrl Pts',(4.13886085166389,12.2,10.4063818332531));
#220324=CARTESIAN_POINT('Ctrl Pts',(4.13878104477818,12.2,10.4109245701075));
#220325=CARTESIAN_POINT('Ctrl Pts',(4.1387012378816,12.2,10.4154673075809));
#220326=CARTESIAN_POINT('Ctrl Pts',(4.13861403689503,12.2,10.4200228854821));
#220327=CARTESIAN_POINT('Ctrl Pts',(4.1385193775005,12.2,10.4245912168985));
#220328=CARTESIAN_POINT('Ctrl Pts',(4.13844838296104,12.2,10.4280174651496));
#220329=CARTESIAN_POINT('Ctrl Pts',(4.13837319151376,12.2,10.4314508882416));
#220330=CARTESIAN_POINT('Ctrl Pts',(4.13829377701664,12.2,10.4348914474916));
#220331=CARTESIAN_POINT('Ctrl Pts',(4.13821436251953,12.2,10.4383320067416));
#220332=CARTESIAN_POINT('Ctrl Pts',(4.13813072518925,12.2,10.4417797029163));
#220333=CARTESIAN_POINT('Ctrl Pts',(4.13804283527615,12.2,10.4452345001235));
#220334=CARTESIAN_POINT('Ctrl Pts',(4.13795494536304,12.2,10.4486892973307));
#220335=CARTESIAN_POINT('Ctrl Pts',(4.13786280418607,12.2,10.4521511951157));
#220336=CARTESIAN_POINT('Ctrl Pts',(4.13776638422692,12.2,10.4556201570372));
#220337=CARTESIAN_POINT('Ctrl Pts',(4.13766996426777,12.2,10.4590891189587));
#220338=CARTESIAN_POINT('Ctrl Pts',(4.13756926675179,12.2,10.4625651457515));
#220339=CARTESIAN_POINT('Ctrl Pts',(4.13746426183953,12.2,10.466048199499));
#220340=CARTESIAN_POINT('Ctrl Pts',(4.13735925690819,12.2,10.4695312538792));
#220341=CARTESIAN_POINT('Ctrl Pts',(4.1372499469423,12.2,10.4730213366364));
#220342=CARTESIAN_POINT('Ctrl Pts',(4.13713630350853,12.2,10.4765184110206));
#220343=CARTESIAN_POINT('Ctrl Pts',(4.1370226600954,12.2,10.4800154847696));
#220344=CARTESIAN_POINT('Ctrl Pts',(4.1369046841325,12.2,10.4835195502931));
#220345=CARTESIAN_POINT('Ctrl Pts',(4.13678234826157,12.2,10.4870305710828));
#220346=CARTESIAN_POINT('Ctrl Pts',(4.13666001239063,12.2,10.4905415918725));
#220347=CARTESIAN_POINT('Ctrl Pts',(4.13653331812904,12.2,10.4940595694985));
#220348=CARTESIAN_POINT('Ctrl Pts',(4.13640223721652,12.2,10.4975844662615));
#220349=CARTESIAN_POINT('Ctrl Pts',(4.13622746267443,12.2,10.5022843283986));
#220350=CARTESIAN_POINT('Ctrl Pts',(4.13604489059251,12.2,10.5069964933205));
#220351=CARTESIAN_POINT('Ctrl Pts',(4.13585446049777,12.2,10.5117208747108));
#220352=CARTESIAN_POINT('Ctrl Pts',(4.13571163789428,12.2,10.5152641615582));
#220353=CARTESIAN_POINT('Ctrl Pts',(4.13556439383956,12.2,10.5188143207408));
#220354=CARTESIAN_POINT('Ctrl Pts',(4.13541270373357,12.2,10.5223713170504));
#220355=CARTESIAN_POINT('Ctrl Pts',(4.13521045030485,12.2,10.5271139777195));
#220356=CARTESIAN_POINT('Ctrl Pts',(4.13500029072993,12.2,10.5318687920092));
#220357=CARTESIAN_POINT('Ctrl Pts',(4.13478216602607,12.2,10.5366356761187));
#220358=CARTESIAN_POINT('Ctrl Pts',(4.13461857249073,12.2,10.5402108393632));
#220359=CARTESIAN_POINT('Ctrl Pts',(4.13445049713071,12.2,10.5437927921822));
#220360=CARTESIAN_POINT('Ctrl Pts',(4.13427791659593,12.2,10.5473814989676));
#220361=CARTESIAN_POINT('Ctrl Pts',(4.13410533602979,12.2,10.5509702064049));
#220362=CARTESIAN_POINT('Ctrl Pts',(4.13392824853739,12.2,10.5545656691775));
#220363=CARTESIAN_POINT('Ctrl Pts',(4.13374663092704,12.2,10.5581678505352));
#220364=CARTESIAN_POINT('Ctrl Pts',(4.13356501334969,12.2,10.5617700312386));
#220365=CARTESIAN_POINT('Ctrl Pts',(4.13337886303283,12.2,10.5653789302828));
#220366=CARTESIAN_POINT('Ctrl Pts',(4.13318815748803,12.2,10.5689945137079));
#220367=CARTESIAN_POINT('Ctrl Pts',(4.13293388343986,12.2,10.573815291389));
#220368=CARTESIAN_POINT('Ctrl Pts',(4.1326715094077,12.2,10.5786479524786));
#220369=CARTESIAN_POINT('Ctrl Pts',(4.13240097626368,12.2,10.5834924126374));
#220370=CARTESIAN_POINT('Ctrl Pts',(4.13219807639645,12.2,10.5871257579214));
#220371=CARTESIAN_POINT('Ctrl Pts',(4.13199058845455,12.2,10.5907657411383));
#220372=CARTESIAN_POINT('Ctrl Pts',(4.13177848604621,12.2,10.5944123269217));
#220373=CARTESIAN_POINT('Ctrl Pts',(4.13149568280942,12.2,10.599274441741));
#220374=CARTESIAN_POINT('Ctrl Pts',(4.13120467765636,12.2,10.6041482949203));
#220375=CARTESIAN_POINT('Ctrl Pts',(4.13090541374977,12.2,10.6090338049866));
#220376=CARTESIAN_POINT('Ctrl Pts',(4.13068096584022,12.2,10.6126979372035));
#220377=CARTESIAN_POINT('Ctrl Pts',(4.13045187237607,12.2,10.6163686266635));
#220378=CARTESIAN_POINT('Ctrl Pts',(4.13021810896685,12.2,10.6200458370049));
#220379=CARTESIAN_POINT('Ctrl Pts',(4.12998434555764,12.2,10.6237230473463));
#220380=CARTESIAN_POINT('Ctrl Pts',(4.12974591236715,12.2,10.6274067807825));
#220381=CARTESIAN_POINT('Ctrl Pts',(4.1295027850014,12.2,10.6310970010645));
#220382=CARTESIAN_POINT('Ctrl Pts',(4.12925965763564,12.2,10.6347872213465));
#220383=CARTESIAN_POINT('Ctrl Pts',(4.12901183772854,12.2,10.6384839297615));
#220384=CARTESIAN_POINT('Ctrl Pts',(4.12875930082169,12.2,10.642187092501));
#220385=CARTESIAN_POINT('Ctrl Pts',(4.12842258491532,12.2,10.6471246432688));
#220386=CARTESIAN_POINT('Ctrl Pts',(4.12807748452064,12.2,10.6520736684298));
#220387=CARTESIAN_POINT('Ctrl Pts',(4.12772394249973,12.2,10.6570340857783));
#220388=CARTESIAN_POINT('Ctrl Pts',(4.127370400527,12.2,10.661994502451));
#220389=CARTESIAN_POINT('Ctrl Pts',(4.12700841624328,12.2,10.6669663091354));
#220390=CARTESIAN_POINT('Ctrl Pts',(4.12663793455221,12.2,10.6719494258935));
#220391=CARTESIAN_POINT('Ctrl Pts',(4.12636007322082,12.2,10.6756867643108));
#220392=CARTESIAN_POINT('Ctrl Pts',(4.12607743316307,12.2,10.6794304647049));
#220393=CARTESIAN_POINT('Ctrl Pts',(4.12578999416231,12.2,10.6831804980841));
#220394=CARTESIAN_POINT('Ctrl Pts',(4.12550255521377,12.2,10.686930530782));
#220395=CARTESIAN_POINT('Ctrl Pts',(4.12521031630714,12.2,10.6906868959797));
#220396=CARTESIAN_POINT('Ctrl Pts',(4.12491325519252,12.2,10.6944495576769));
#220397=CARTESIAN_POINT('Ctrl Pts',(4.12451717372434,12.2,10.6994664397119));
#220398=CARTESIAN_POINT('Ctrl Pts',(4.12411251545434,12.2,10.7044945146189));
#220399=CARTESIAN_POINT('Ctrl Pts',(4.12369921830157,12.2,10.7095336875688));
#220400=CARTESIAN_POINT('Ctrl Pts',(4.12328592109248,12.2,10.7145728612053));
#220401=CARTESIAN_POINT('Ctrl Pts',(4.12286398257608,12.2,10.7196231273852));
#220402=CARTESIAN_POINT('Ctrl Pts',(4.12243337123359,12.2,10.7246844426642));
#220403=CARTESIAN_POINT('Ctrl Pts',(4.12211041275606,12.2,10.7284804287786));
#220404=CARTESIAN_POINT('Ctrl Pts',(4.12178257806039,12.2,10.7322826273081));
#220405=CARTESIAN_POINT('Ctrl Pts',(4.12144986799994,12.2,10.736091048));
#220406=CARTESIAN_POINT('Origin',(-5.66257110645729E-14,15.2,-1.77635683940025E-14));
#220407=CARTESIAN_POINT('',(2.64164356330595,15.2,10.0330625578962));
#220408=CARTESIAN_POINT('',(2.64164356330595,12.2,10.0330625578962));
#220409=CARTESIAN_POINT('',(2.64164356299994,15.2,10.033062558));
#220410=CARTESIAN_POINT('Origin',(-5.66257110645729E-14,12.2,-1.77635683940025E-14));
#220411=CARTESIAN_POINT('Origin',(-5.66257110645729E-14,15.2,-1.77635683940025E-14));
#220412=CARTESIAN_POINT('Origin',(-5.66257110645729E-14,15.2,-1.77635683940025E-14));
#220413=CARTESIAN_POINT('',(2.55159438999994,15.2,11.213356593));
#220414=CARTESIAN_POINT('',(2.17615954695741,15.2,11.2922242994459));
#220415=CARTESIAN_POINT('Origin',(-5.66257110645729E-14,15.2,-1.77635683940025E-14));
#220416=CARTESIAN_POINT('',(2.17615954695741,12.2,11.2922242994459));
#220417=CARTESIAN_POINT('',(2.17615954699994,15.2,11.2922243));
#220418=CARTESIAN_POINT('',(2.55159438999994,12.2,11.213356593));
#220419=CARTESIAN_POINT('Origin',(-5.66257110645729E-14,12.2,-1.77635683940025E-14));
#220420=CARTESIAN_POINT('',(2.55159438999994,15.2,11.213356593));
#220421=CARTESIAN_POINT('Ctrl Pts',(2.64164356399994,15.2,10.033062558));
#220422=CARTESIAN_POINT('Ctrl Pts',(2.64164356399994,11.6,10.033062558));
#220423=CARTESIAN_POINT('Ctrl Pts',(2.64167330399995,15.2,10.033234361));
#220424=CARTESIAN_POINT('Ctrl Pts',(2.64167330399995,11.6,10.033234361));
#220425=CARTESIAN_POINT('Ctrl Pts',(2.64173373799995,15.2,10.033583982));
#220426=CARTESIAN_POINT('Ctrl Pts',(2.64173373799995,11.6,10.033583982));
#220427=CARTESIAN_POINT('Ctrl Pts',(2.64182504799995,15.2,10.034113786));
#220428=CARTESIAN_POINT('Ctrl Pts',(2.64182504799995,11.6,10.034113786));
#220429=CARTESIAN_POINT('Ctrl Pts',(2.64194751799995,15.2,10.034827572));
#220430=CARTESIAN_POINT('Ctrl Pts',(2.64194751799995,11.6,10.034827572));
#220431=CARTESIAN_POINT('Ctrl Pts',(2.64210152599994,15.2,10.03573056));
#220432=CARTESIAN_POINT('Ctrl Pts',(2.64210152599994,11.6,10.03573056));
#220433=CARTESIAN_POINT('Ctrl Pts',(2.64225710799994,15.2,10.03664834));
#220434=CARTESIAN_POINT('Ctrl Pts',(2.64225710799994,11.6,10.03664834));
#220435=CARTESIAN_POINT('Ctrl Pts',(2.64241334999994,15.2,10.037575658));
#220436=CARTESIAN_POINT('Ctrl Pts',(2.64241334999994,11.6,10.037575658));
#220437=CARTESIAN_POINT('Ctrl Pts',(2.64257022899994,15.2,10.03851249));
#220438=CARTESIAN_POINT('Ctrl Pts',(2.64257022899994,11.6,10.03851249));
#220439=CARTESIAN_POINT('Ctrl Pts',(2.64272772399994,15.2,10.039458812));
#220440=CARTESIAN_POINT('Ctrl Pts',(2.64272772399994,11.6,10.039458812));
#220441=CARTESIAN_POINT('Ctrl Pts',(2.64288581299994,15.2,10.040414602));
#220442=CARTESIAN_POINT('Ctrl Pts',(2.64288581299994,11.6,10.040414602));
#220443=CARTESIAN_POINT('Ctrl Pts',(2.64304447199994,15.2,10.041379835));
#220444=CARTESIAN_POINT('Ctrl Pts',(2.64304447199994,11.6,10.041379835));
#220445=CARTESIAN_POINT('Ctrl Pts',(2.64320368099995,15.2,10.04235449));
#220446=CARTESIAN_POINT('Ctrl Pts',(2.64320368099995,11.6,10.04235449));
#220447=CARTESIAN_POINT('Ctrl Pts',(2.64336341799994,15.2,10.043338541));
#220448=CARTESIAN_POINT('Ctrl Pts',(2.64336341799994,11.6,10.043338541));
#220449=CARTESIAN_POINT('Ctrl Pts',(2.64352365999994,15.2,10.044331969));
#220450=CARTESIAN_POINT('Ctrl Pts',(2.64352365999994,11.6,10.044331969));
#220451=CARTESIAN_POINT('Ctrl Pts',(2.64368438699994,15.2,10.045334747));
#220452=CARTESIAN_POINT('Ctrl Pts',(2.64368438699994,11.6,10.045334747));
#220453=CARTESIAN_POINT('Ctrl Pts',(2.64384557599994,15.2,10.046346855));
#220454=CARTESIAN_POINT('Ctrl Pts',(2.64384557599994,11.6,10.046346855));
#220455=CARTESIAN_POINT('Ctrl Pts',(2.64400720799994,15.2,10.047368269));
#220456=CARTESIAN_POINT('Ctrl Pts',(2.64400720799994,11.6,10.047368269));
#220457=CARTESIAN_POINT('Ctrl Pts',(2.64416925899994,15.2,10.048398967));
#220458=CARTESIAN_POINT('Ctrl Pts',(2.64416925899994,11.6,10.048398967));
#220459=CARTESIAN_POINT('Ctrl Pts',(2.64433170999995,15.2,10.049438926));
#220460=CARTESIAN_POINT('Ctrl Pts',(2.64433170999995,11.6,10.049438926));
#220461=CARTESIAN_POINT('Ctrl Pts',(2.64449453899994,15.2,10.050488124));
#220462=CARTESIAN_POINT('Ctrl Pts',(2.64449453899994,11.6,10.050488124));
#220463=CARTESIAN_POINT('Ctrl Pts',(2.64465772599995,15.2,10.051546539));
#220464=CARTESIAN_POINT('Ctrl Pts',(2.64465772599995,11.6,10.051546539));
#220465=CARTESIAN_POINT('Ctrl Pts',(2.64482124899994,15.2,10.052614149));
#220466=CARTESIAN_POINT('Ctrl Pts',(2.64482124899994,11.6,10.052614149));
#220467=CARTESIAN_POINT('Ctrl Pts',(2.64498508799994,15.2,10.053690931));
#220468=CARTESIAN_POINT('Ctrl Pts',(2.64498508799994,11.6,10.053690931));
#220469=CARTESIAN_POINT('Ctrl Pts',(2.64514922199994,15.2,10.054776862));
#220470=CARTESIAN_POINT('Ctrl Pts',(2.64514922199994,11.6,10.054776862));
#220471=CARTESIAN_POINT('Ctrl Pts',(2.64531363099994,15.2,10.055871924));
#220472=CARTESIAN_POINT('Ctrl Pts',(2.64531363099994,11.6,10.055871924));
#220473=CARTESIAN_POINT('Ctrl Pts',(2.64547829399994,15.2,10.056976092));
#220474=CARTESIAN_POINT('Ctrl Pts',(2.64547829399994,11.6,10.056976092));
#220475=CARTESIAN_POINT('Ctrl Pts',(2.64564319299994,15.2,10.058089345));
#220476=CARTESIAN_POINT('Ctrl Pts',(2.64564319299994,11.6,10.058089345));
#220477=CARTESIAN_POINT('Ctrl Pts',(2.64580830599995,15.2,10.059211661));
#220478=CARTESIAN_POINT('Ctrl Pts',(2.64580830599995,11.6,10.059211661));
#220479=CARTESIAN_POINT('Ctrl Pts',(2.64597361199994,15.2,10.060343019));
#220480=CARTESIAN_POINT('Ctrl Pts',(2.64597361199994,11.6,10.060343019));
#220481=CARTESIAN_POINT('Ctrl Pts',(2.64613909299994,15.2,10.061483398));
#220482=CARTESIAN_POINT('Ctrl Pts',(2.64613909299994,11.6,10.061483398));
#220483=CARTESIAN_POINT('Ctrl Pts',(2.64630472899994,15.2,10.062632776));
#220484=CARTESIAN_POINT('Ctrl Pts',(2.64630472899994,11.6,10.062632776));
#220485=CARTESIAN_POINT('Ctrl Pts',(2.64647049899994,15.2,10.063791132));
#220486=CARTESIAN_POINT('Ctrl Pts',(2.64647049899994,11.6,10.063791132));
#220487=CARTESIAN_POINT('Ctrl Pts',(2.64663638299994,15.2,10.064958444));
#220488=CARTESIAN_POINT('Ctrl Pts',(2.64663638299994,11.6,10.064958444));
#220489=CARTESIAN_POINT('Ctrl Pts',(2.64680236499995,15.2,10.066134693));
#220490=CARTESIAN_POINT('Ctrl Pts',(2.64680236499995,11.6,10.066134693));
#220491=CARTESIAN_POINT('Ctrl Pts',(2.64696842099994,15.2,10.067319856));
#220492=CARTESIAN_POINT('Ctrl Pts',(2.64696842099994,11.6,10.067319856));
#220493=CARTESIAN_POINT('Ctrl Pts',(2.64713453499994,15.2,10.068513912));
#220494=CARTESIAN_POINT('Ctrl Pts',(2.64713453499994,11.6,10.068513912));
#220495=CARTESIAN_POINT('Ctrl Pts',(2.64730068699994,15.2,10.069716842));
#220496=CARTESIAN_POINT('Ctrl Pts',(2.64730068699994,11.6,10.069716842));
#220497=CARTESIAN_POINT('Ctrl Pts',(2.64746685599994,15.2,10.070928625));
#220498=CARTESIAN_POINT('Ctrl Pts',(2.64746685599994,11.6,10.070928625));
#220499=CARTESIAN_POINT('Ctrl Pts',(2.64763302599994,15.2,10.072149238));
#220500=CARTESIAN_POINT('Ctrl Pts',(2.64763302599994,11.6,10.072149238));
#220501=CARTESIAN_POINT('Ctrl Pts',(2.64779917599994,15.2,10.073378662));
#220502=CARTESIAN_POINT('Ctrl Pts',(2.64779917599994,11.6,10.073378662));
#220503=CARTESIAN_POINT('Ctrl Pts',(2.64796528699994,15.2,10.074616878));
#220504=CARTESIAN_POINT('Ctrl Pts',(2.64796528699994,11.6,10.074616878));
#220505=CARTESIAN_POINT('Ctrl Pts',(2.64813134299994,15.2,10.075863863));
#220506=CARTESIAN_POINT('Ctrl Pts',(2.64813134299994,11.6,10.075863863));
#220507=CARTESIAN_POINT('Ctrl Pts',(2.64829732199995,15.2,10.077119598));
#220508=CARTESIAN_POINT('Ctrl Pts',(2.64829732199995,11.6,10.077119598));
#220509=CARTESIAN_POINT('Ctrl Pts',(2.64846320599994,15.2,10.078384063));
#220510=CARTESIAN_POINT('Ctrl Pts',(2.64846320599994,11.6,10.078384063));
#220511=CARTESIAN_POINT('Ctrl Pts',(2.64862897799994,15.2,10.079657238));
#220512=CARTESIAN_POINT('Ctrl Pts',(2.64862897799994,11.6,10.079657238));
#220513=CARTESIAN_POINT('Ctrl Pts',(2.64879461899994,15.2,10.080939101));
#220514=CARTESIAN_POINT('Ctrl Pts',(2.64879461899994,11.6,10.080939101));
#220515=CARTESIAN_POINT('Ctrl Pts',(2.64896010999994,15.2,10.082229634));
#220516=CARTESIAN_POINT('Ctrl Pts',(2.64896010999994,11.6,10.082229634));
#220517=CARTESIAN_POINT('Ctrl Pts',(2.64912543499995,15.2,10.083528816));
#220518=CARTESIAN_POINT('Ctrl Pts',(2.64912543499995,11.6,10.083528816));
#220519=CARTESIAN_POINT('Ctrl Pts',(2.64929057299994,15.2,10.084836628));
#220520=CARTESIAN_POINT('Ctrl Pts',(2.64929057299994,11.6,10.084836628));
#220521=CARTESIAN_POINT('Ctrl Pts',(2.64945550799994,15.2,10.08615305));
#220522=CARTESIAN_POINT('Ctrl Pts',(2.64945550799994,11.6,10.08615305));
#220523=CARTESIAN_POINT('Ctrl Pts',(2.64962022199994,15.2,10.087478062));
#220524=CARTESIAN_POINT('Ctrl Pts',(2.64962022199994,11.6,10.087478062));
#220525=CARTESIAN_POINT('Ctrl Pts',(2.64978469499995,15.2,10.088811644));
#220526=CARTESIAN_POINT('Ctrl Pts',(2.64978469499995,11.6,10.088811644));
#220527=CARTESIAN_POINT('Ctrl Pts',(2.64994891199994,15.2,10.090153777));
#220528=CARTESIAN_POINT('Ctrl Pts',(2.64994891199994,11.6,10.090153777));
#220529=CARTESIAN_POINT('Ctrl Pts',(2.65011285399994,15.2,10.091504443));
#220530=CARTESIAN_POINT('Ctrl Pts',(2.65011285399994,11.6,10.091504443));
#220531=CARTESIAN_POINT('Ctrl Pts',(2.65027650299994,15.2,10.09286362));
#220532=CARTESIAN_POINT('Ctrl Pts',(2.65027650299994,11.6,10.09286362));
#220533=CARTESIAN_POINT('Ctrl Pts',(2.65043984299994,15.2,10.09423129));
#220534=CARTESIAN_POINT('Ctrl Pts',(2.65043984299994,11.6,10.09423129));
#220535=CARTESIAN_POINT('Ctrl Pts',(2.65060285499994,15.2,10.095607434));
#220536=CARTESIAN_POINT('Ctrl Pts',(2.65060285499994,11.6,10.095607434));
#220537=CARTESIAN_POINT('Ctrl Pts',(2.65076552299994,15.2,10.096992032));
#220538=CARTESIAN_POINT('Ctrl Pts',(2.65076552299994,11.6,10.096992032));
#220539=CARTESIAN_POINT('Ctrl Pts',(2.65092782799994,15.2,10.098385066));
#220540=CARTESIAN_POINT('Ctrl Pts',(2.65092782799994,11.6,10.098385066));
#220541=CARTESIAN_POINT('Ctrl Pts',(2.65108975499994,15.2,10.099786515));
#220542=CARTESIAN_POINT('Ctrl Pts',(2.65108975499994,11.6,10.099786515));
#220543=CARTESIAN_POINT('Ctrl Pts',(2.65125128499994,15.2,10.101196362));
#220544=CARTESIAN_POINT('Ctrl Pts',(2.65125128499994,11.6,10.101196362));
#220545=CARTESIAN_POINT('Ctrl Pts',(2.65141240299994,15.2,10.102614588));
#220546=CARTESIAN_POINT('Ctrl Pts',(2.65141240299994,11.6,10.102614588));
#220547=CARTESIAN_POINT('Ctrl Pts',(2.65157308999994,15.2,10.104041173));
#220548=CARTESIAN_POINT('Ctrl Pts',(2.65157308999994,11.6,10.104041173));
#220549=CARTESIAN_POINT('Ctrl Pts',(2.65173333099994,15.2,10.1054761));
#220550=CARTESIAN_POINT('Ctrl Pts',(2.65173333099994,11.6,10.1054761));
#220551=CARTESIAN_POINT('Ctrl Pts',(2.65189310699995,15.2,10.106919348));
#220552=CARTESIAN_POINT('Ctrl Pts',(2.65189310699995,11.6,10.106919348));
#220553=CARTESIAN_POINT('Ctrl Pts',(2.65205240399994,15.2,10.1083709));
#220554=CARTESIAN_POINT('Ctrl Pts',(2.65205240399994,11.6,10.1083709));
#220555=CARTESIAN_POINT('Ctrl Pts',(2.65221120299994,15.2,10.109830736));
#220556=CARTESIAN_POINT('Ctrl Pts',(2.65221120299994,11.6,10.109830736));
#220557=CARTESIAN_POINT('Ctrl Pts',(2.65236948999994,15.2,10.11129884));
#220558=CARTESIAN_POINT('Ctrl Pts',(2.65236948999994,11.6,10.11129884));
#220559=CARTESIAN_POINT('Ctrl Pts',(2.65252724599994,15.2,10.112775193));
#220560=CARTESIAN_POINT('Ctrl Pts',(2.65252724599994,11.6,10.112775193));
#220561=CARTESIAN_POINT('Ctrl Pts',(2.65268445599995,15.2,10.114259774));
#220562=CARTESIAN_POINT('Ctrl Pts',(2.65268445599995,11.6,10.114259774));
#220563=CARTESIAN_POINT('Ctrl Pts',(2.65284110299994,15.2,10.115752568));
#220564=CARTESIAN_POINT('Ctrl Pts',(2.65284110299994,11.6,10.115752568));
#220565=CARTESIAN_POINT('Ctrl Pts',(2.65299717299994,15.2,10.117253554));
#220566=CARTESIAN_POINT('Ctrl Pts',(2.65299717299994,11.6,10.117253554));
#220567=CARTESIAN_POINT('Ctrl Pts',(2.65315264599994,15.2,10.118762716));
#220568=CARTESIAN_POINT('Ctrl Pts',(2.65315264599994,11.6,10.118762716));
#220569=CARTESIAN_POINT('Ctrl Pts',(2.65330750999994,15.2,10.120280036));
#220570=CARTESIAN_POINT('Ctrl Pts',(2.65330750999994,11.6,10.120280036));
#220571=CARTESIAN_POINT('Ctrl Pts',(2.65346174599994,15.2,10.121805494));
#220572=CARTESIAN_POINT('Ctrl Pts',(2.65346174599994,11.6,10.121805494));
#220573=CARTESIAN_POINT('Ctrl Pts',(2.65361533899994,15.2,10.123339075));
#220574=CARTESIAN_POINT('Ctrl Pts',(2.65361533899994,11.6,10.123339075));
#220575=CARTESIAN_POINT('Ctrl Pts',(2.65376827399994,15.2,10.124880757));
#220576=CARTESIAN_POINT('Ctrl Pts',(2.65376827399994,11.6,10.124880757));
#220577=CARTESIAN_POINT('Ctrl Pts',(2.65392053399994,15.2,10.126430526));
#220578=CARTESIAN_POINT('Ctrl Pts',(2.65392053399994,11.6,10.126430526));
#220579=CARTESIAN_POINT('Ctrl Pts',(2.65407210499994,15.2,10.127988362));
#220580=CARTESIAN_POINT('Ctrl Pts',(2.65407210499994,11.6,10.127988362));
#220581=CARTESIAN_POINT('Ctrl Pts',(2.65422296899994,15.2,10.129554248));
#220582=CARTESIAN_POINT('Ctrl Pts',(2.65422296899994,11.6,10.129554248));
#220583=CARTESIAN_POINT('Ctrl Pts',(2.65437311199994,15.2,10.131128167));
#220584=CARTESIAN_POINT('Ctrl Pts',(2.65437311199994,11.6,10.131128167));
#220585=CARTESIAN_POINT('Ctrl Pts',(2.65452251799994,15.2,10.132710101));
#220586=CARTESIAN_POINT('Ctrl Pts',(2.65452251799994,11.6,10.132710101));
#220587=CARTESIAN_POINT('Ctrl Pts',(2.65467117299994,15.2,10.134300032));
#220588=CARTESIAN_POINT('Ctrl Pts',(2.65467117299994,11.6,10.134300032));
#220589=CARTESIAN_POINT('Ctrl Pts',(2.65481905899994,15.2,10.135897942));
#220590=CARTESIAN_POINT('Ctrl Pts',(2.65481905899994,11.6,10.135897942));
#220591=CARTESIAN_POINT('Ctrl Pts',(2.65496616299994,15.2,10.137503816));
#220592=CARTESIAN_POINT('Ctrl Pts',(2.65496616299994,11.6,10.137503816));
#220593=CARTESIAN_POINT('Ctrl Pts',(2.65511246899994,15.2,10.139117634));
#220594=CARTESIAN_POINT('Ctrl Pts',(2.65511246899994,11.6,10.139117634));
#220595=CARTESIAN_POINT('Ctrl Pts',(2.65525796099995,15.2,10.14073938));
#220596=CARTESIAN_POINT('Ctrl Pts',(2.65525796099995,11.6,10.14073938));
#220597=CARTESIAN_POINT('Ctrl Pts',(2.65540262499994,15.2,10.142369037));
#220598=CARTESIAN_POINT('Ctrl Pts',(2.65540262499994,11.6,10.142369037));
#220599=CARTESIAN_POINT('Ctrl Pts',(2.65554644699994,15.2,10.144006587));
#220600=CARTESIAN_POINT('Ctrl Pts',(2.65554644699994,11.6,10.144006587));
#220601=CARTESIAN_POINT('Ctrl Pts',(2.65568941099994,15.2,10.145652013));
#220602=CARTESIAN_POINT('Ctrl Pts',(2.65568941099994,11.6,10.145652013));
#220603=CARTESIAN_POINT('Ctrl Pts',(2.65583150099994,15.2,10.147305299));
#220604=CARTESIAN_POINT('Ctrl Pts',(2.65583150099994,11.6,10.147305299));
#220605=CARTESIAN_POINT('Ctrl Pts',(2.65597270299994,15.2,10.148966427));
#220606=CARTESIAN_POINT('Ctrl Pts',(2.65597270299994,11.6,10.148966427));
#220607=CARTESIAN_POINT('Ctrl Pts',(2.65611300299994,15.2,10.150635381));
#220608=CARTESIAN_POINT('Ctrl Pts',(2.65611300299994,11.6,10.150635381));
#220609=CARTESIAN_POINT('Ctrl Pts',(2.65625238599994,15.2,10.152312142));
#220610=CARTESIAN_POINT('Ctrl Pts',(2.65625238599994,11.6,10.152312142));
#220611=CARTESIAN_POINT('Ctrl Pts',(2.65639083699994,15.2,10.153996696));
#220612=CARTESIAN_POINT('Ctrl Pts',(2.65639083699994,11.6,10.153996696));
#220613=CARTESIAN_POINT('Ctrl Pts',(2.65652834299994,15.2,10.155689024));
#220614=CARTESIAN_POINT('Ctrl Pts',(2.65652834299994,11.6,10.155689024));
#220615=CARTESIAN_POINT('Ctrl Pts',(2.65666488599994,15.2,10.157389111));
#220616=CARTESIAN_POINT('Ctrl Pts',(2.65666488599994,11.6,10.157389111));
#220617=CARTESIAN_POINT('Ctrl Pts',(2.65680045599994,15.2,10.159096939));
#220618=CARTESIAN_POINT('Ctrl Pts',(2.65680045599994,11.6,10.159096939));
#220619=CARTESIAN_POINT('Ctrl Pts',(2.65693503499994,15.2,10.160812492));
#220620=CARTESIAN_POINT('Ctrl Pts',(2.65693503499994,11.6,10.160812492));
#220621=CARTESIAN_POINT('Ctrl Pts',(2.65706860999994,15.2,10.162535753));
#220622=CARTESIAN_POINT('Ctrl Pts',(2.65706860999994,11.6,10.162535753));
#220623=CARTESIAN_POINT('Ctrl Pts',(2.65720116799995,15.2,10.164266705));
#220624=CARTESIAN_POINT('Ctrl Pts',(2.65720116799995,11.6,10.164266705));
#220625=CARTESIAN_POINT('Ctrl Pts',(2.65733269399994,15.2,10.166005334));
#220626=CARTESIAN_POINT('Ctrl Pts',(2.65733269399994,11.6,10.166005334));
#220627=CARTESIAN_POINT('Ctrl Pts',(2.65746317299994,15.2,10.167751622));
#220628=CARTESIAN_POINT('Ctrl Pts',(2.65746317299994,11.6,10.167751622));
#220629=CARTESIAN_POINT('Ctrl Pts',(2.65759259199994,15.2,10.169505552));
#220630=CARTESIAN_POINT('Ctrl Pts',(2.65759259199994,11.6,10.169505552));
#220631=CARTESIAN_POINT('Ctrl Pts',(2.65772093699994,15.2,10.171267109));
#220632=CARTESIAN_POINT('Ctrl Pts',(2.65772093699994,11.6,10.171267109));
#220633=CARTESIAN_POINT('Ctrl Pts',(2.65784819299994,15.2,10.173036275));
#220634=CARTESIAN_POINT('Ctrl Pts',(2.65784819299994,11.6,10.173036275));
#220635=CARTESIAN_POINT('Ctrl Pts',(2.65797434799994,15.2,10.174813035));
#220636=CARTESIAN_POINT('Ctrl Pts',(2.65797434799994,11.6,10.174813035));
#220637=CARTESIAN_POINT('Ctrl Pts',(2.65809938699994,15.2,10.176597374));
#220638=CARTESIAN_POINT('Ctrl Pts',(2.65809938699994,11.6,10.176597374));
#220639=CARTESIAN_POINT('Ctrl Pts',(2.65822329599994,15.2,10.178389274));
#220640=CARTESIAN_POINT('Ctrl Pts',(2.65822329599994,11.6,10.178389274));
#220641=CARTESIAN_POINT('Ctrl Pts',(2.65834606299994,15.2,10.18018872));
#220642=CARTESIAN_POINT('Ctrl Pts',(2.65834606299994,11.6,10.18018872));
#220643=CARTESIAN_POINT('Ctrl Pts',(2.65846767199994,15.2,10.181995695));
#220644=CARTESIAN_POINT('Ctrl Pts',(2.65846767199994,11.6,10.181995695));
#220645=CARTESIAN_POINT('Ctrl Pts',(2.65858811199994,15.2,10.183810184));
#220646=CARTESIAN_POINT('Ctrl Pts',(2.65858811199994,11.6,10.183810184));
#220647=CARTESIAN_POINT('Ctrl Pts',(2.65870736599994,15.2,10.185632171));
#220648=CARTESIAN_POINT('Ctrl Pts',(2.65870736599994,11.6,10.185632171));
#220649=CARTESIAN_POINT('Ctrl Pts',(2.65882542499994,15.2,10.18746164));
#220650=CARTESIAN_POINT('Ctrl Pts',(2.65882542499994,11.6,10.18746164));
#220651=CARTESIAN_POINT('Ctrl Pts',(2.65894227299994,15.2,10.189298575));
#220652=CARTESIAN_POINT('Ctrl Pts',(2.65894227299994,11.6,10.189298575));
#220653=CARTESIAN_POINT('Ctrl Pts',(2.65905789599994,15.2,10.19114296));
#220654=CARTESIAN_POINT('Ctrl Pts',(2.65905789599994,11.6,10.19114296));
#220655=CARTESIAN_POINT('Ctrl Pts',(2.65917228199994,15.2,10.192994781));
#220656=CARTESIAN_POINT('Ctrl Pts',(2.65917228199994,11.6,10.192994781));
#220657=CARTESIAN_POINT('Ctrl Pts',(2.65928541899994,15.2,10.194854021));
#220658=CARTESIAN_POINT('Ctrl Pts',(2.65928541899994,11.6,10.194854021));
#220659=CARTESIAN_POINT('Ctrl Pts',(2.65939729099995,15.2,10.196720664));
#220660=CARTESIAN_POINT('Ctrl Pts',(2.65939729099995,11.6,10.196720664));
#220661=CARTESIAN_POINT('Ctrl Pts',(2.65950788599994,15.2,10.198594695));
#220662=CARTESIAN_POINT('Ctrl Pts',(2.65950788599994,11.6,10.198594695));
#220663=CARTESIAN_POINT('Ctrl Pts',(2.65961719199994,15.2,10.200476099));
#220664=CARTESIAN_POINT('Ctrl Pts',(2.65961719199994,11.6,10.200476099));
#220665=CARTESIAN_POINT('Ctrl Pts',(2.65972519499994,15.2,10.202364859));
#220666=CARTESIAN_POINT('Ctrl Pts',(2.65972519499994,11.6,10.202364859));
#220667=CARTESIAN_POINT('Ctrl Pts',(2.65983188299994,15.2,10.204260962));
#220668=CARTESIAN_POINT('Ctrl Pts',(2.65983188299994,11.6,10.204260962));
#220669=CARTESIAN_POINT('Ctrl Pts',(2.65993724399994,15.2,10.20616439));
#220670=CARTESIAN_POINT('Ctrl Pts',(2.65993724399994,11.6,10.20616439));
#220671=CARTESIAN_POINT('Ctrl Pts',(2.66004126099994,15.2,10.20807513));
#220672=CARTESIAN_POINT('Ctrl Pts',(2.66004126099994,11.6,10.20807513));
#220673=CARTESIAN_POINT('Ctrl Pts',(2.66014392499994,15.2,10.209993164));
#220674=CARTESIAN_POINT('Ctrl Pts',(2.66014392499994,11.6,10.209993164));
#220675=CARTESIAN_POINT('Ctrl Pts',(2.66024522199994,15.2,10.21191848));
#220676=CARTESIAN_POINT('Ctrl Pts',(2.66024522199994,11.6,10.21191848));
#220677=CARTESIAN_POINT('Ctrl Pts',(2.66034513999994,15.2,10.213851061));
#220678=CARTESIAN_POINT('Ctrl Pts',(2.66034513999994,11.6,10.213851061));
#220679=CARTESIAN_POINT('Ctrl Pts',(2.66044366599994,15.2,10.215790892));
#220680=CARTESIAN_POINT('Ctrl Pts',(2.66044366599994,11.6,10.215790892));
#220681=CARTESIAN_POINT('Ctrl Pts',(2.66054078599995,15.2,10.217737957));
#220682=CARTESIAN_POINT('Ctrl Pts',(2.66054078599995,11.6,10.217737957));
#220683=CARTESIAN_POINT('Ctrl Pts',(2.66063649099994,15.2,10.219692243));
#220684=CARTESIAN_POINT('Ctrl Pts',(2.66063649099994,11.6,10.219692243));
#220685=CARTESIAN_POINT('Ctrl Pts',(2.66073076499994,15.2,10.221653733));
#220686=CARTESIAN_POINT('Ctrl Pts',(2.66073076499994,11.6,10.221653733));
#220687=CARTESIAN_POINT('Ctrl Pts',(2.66082359799994,15.2,10.223622414));
#220688=CARTESIAN_POINT('Ctrl Pts',(2.66082359799994,11.6,10.223622414));
#220689=CARTESIAN_POINT('Ctrl Pts',(2.66091497699994,15.2,10.22559827));
#220690=CARTESIAN_POINT('Ctrl Pts',(2.66091497699994,11.6,10.22559827));
#220691=CARTESIAN_POINT('Ctrl Pts',(2.66100488899994,15.2,10.227581285));
#220692=CARTESIAN_POINT('Ctrl Pts',(2.66100488899994,11.6,10.227581285));
#220693=CARTESIAN_POINT('Ctrl Pts',(2.66109332099994,15.2,10.229571446));
#220694=CARTESIAN_POINT('Ctrl Pts',(2.66109332099994,11.6,10.229571446));
#220695=CARTESIAN_POINT('Ctrl Pts',(2.66118026299994,15.2,10.231568737));
#220696=CARTESIAN_POINT('Ctrl Pts',(2.66118026299994,11.6,10.231568737));
#220697=CARTESIAN_POINT('Ctrl Pts',(2.66126570199994,15.2,10.233573145));
#220698=CARTESIAN_POINT('Ctrl Pts',(2.66126570199994,11.6,10.233573145));
#220699=CARTESIAN_POINT('Ctrl Pts',(2.66134962599994,15.2,10.235584653));
#220700=CARTESIAN_POINT('Ctrl Pts',(2.66134962599994,11.6,10.235584653));
#220701=CARTESIAN_POINT('Ctrl Pts',(2.66143202199994,15.2,10.237603247));
#220702=CARTESIAN_POINT('Ctrl Pts',(2.66143202199994,11.6,10.237603247));
#220703=CARTESIAN_POINT('Ctrl Pts',(2.66151287899994,15.2,10.239628914));
#220704=CARTESIAN_POINT('Ctrl Pts',(2.66151287899994,11.6,10.239628914));
#220705=CARTESIAN_POINT('Ctrl Pts',(2.66159218399994,15.2,10.241661637));
#220706=CARTESIAN_POINT('Ctrl Pts',(2.66159218399994,11.6,10.241661637));
#220707=CARTESIAN_POINT('Ctrl Pts',(2.66166992699994,15.2,10.243701404));
#220708=CARTESIAN_POINT('Ctrl Pts',(2.66166992699994,11.6,10.243701404));
#220709=CARTESIAN_POINT('Ctrl Pts',(2.66174609499994,15.2,10.245748197));
#220710=CARTESIAN_POINT('Ctrl Pts',(2.66174609499994,11.6,10.245748197));
#220711=CARTESIAN_POINT('Ctrl Pts',(2.66182067499994,15.2,10.247802005));
#220712=CARTESIAN_POINT('Ctrl Pts',(2.66182067499994,11.6,10.247802005));
#220713=CARTESIAN_POINT('Ctrl Pts',(2.66189365799995,15.2,10.249862812));
#220714=CARTESIAN_POINT('Ctrl Pts',(2.66189365799995,11.6,10.249862812));
#220715=CARTESIAN_POINT('Ctrl Pts',(2.66196502999994,15.2,10.251930604));
#220716=CARTESIAN_POINT('Ctrl Pts',(2.66196502999994,11.6,10.251930604));
#220717=CARTESIAN_POINT('Ctrl Pts',(2.66203477999994,15.2,10.254005366));
#220718=CARTESIAN_POINT('Ctrl Pts',(2.66203477999994,11.6,10.254005366));
#220719=CARTESIAN_POINT('Ctrl Pts',(2.66210289699994,15.2,10.256087084));
#220720=CARTESIAN_POINT('Ctrl Pts',(2.66210289699994,11.6,10.256087084));
#220721=CARTESIAN_POINT('Ctrl Pts',(2.66216936799994,15.2,10.258175744));
#220722=CARTESIAN_POINT('Ctrl Pts',(2.66216936799994,11.6,10.258175744));
#220723=CARTESIAN_POINT('Ctrl Pts',(2.66223418299994,15.2,10.260271332));
#220724=CARTESIAN_POINT('Ctrl Pts',(2.66223418299994,11.6,10.260271332));
#220725=CARTESIAN_POINT('Ctrl Pts',(2.66229732999994,15.2,10.262373833));
#220726=CARTESIAN_POINT('Ctrl Pts',(2.66229732999994,11.6,10.262373833));
#220727=CARTESIAN_POINT('Ctrl Pts',(2.66235879699994,15.2,10.264483234));
#220728=CARTESIAN_POINT('Ctrl Pts',(2.66235879699994,11.6,10.264483234));
#220729=CARTESIAN_POINT('Ctrl Pts',(2.66241857399995,15.2,10.266599519));
#220730=CARTESIAN_POINT('Ctrl Pts',(2.66241857399995,11.6,10.266599519));
#220731=CARTESIAN_POINT('Ctrl Pts',(2.66247664799995,15.2,10.268722676));
#220732=CARTESIAN_POINT('Ctrl Pts',(2.66247664799995,11.6,10.268722676));
#220733=CARTESIAN_POINT('Ctrl Pts',(2.66253300899994,15.2,10.270852689));
#220734=CARTESIAN_POINT('Ctrl Pts',(2.66253300899994,11.6,10.270852689));
#220735=CARTESIAN_POINT('Ctrl Pts',(2.66258764499995,15.2,10.272989546));
#220736=CARTESIAN_POINT('Ctrl Pts',(2.66258764499995,11.6,10.272989546));
#220737=CARTESIAN_POINT('Ctrl Pts',(2.66264054499994,15.2,10.275133232));
#220738=CARTESIAN_POINT('Ctrl Pts',(2.66264054499994,11.6,10.275133232));
#220739=CARTESIAN_POINT('Ctrl Pts',(2.66269169899994,15.2,10.277283732));
#220740=CARTESIAN_POINT('Ctrl Pts',(2.66269169899994,11.6,10.277283732));
#220741=CARTESIAN_POINT('Ctrl Pts',(2.66274109399995,15.2,10.279441035));
#220742=CARTESIAN_POINT('Ctrl Pts',(2.66274109399995,11.6,10.279441035));
#220743=CARTESIAN_POINT('Ctrl Pts',(2.66278871999994,15.2,10.281605124));
#220744=CARTESIAN_POINT('Ctrl Pts',(2.66278871999994,11.6,10.281605124));
#220745=CARTESIAN_POINT('Ctrl Pts',(2.66283456499994,15.2,10.283775987));
#220746=CARTESIAN_POINT('Ctrl Pts',(2.66283456499994,11.6,10.283775987));
#220747=CARTESIAN_POINT('Ctrl Pts',(2.66287861899994,15.2,10.285953609));
#220748=CARTESIAN_POINT('Ctrl Pts',(2.66287861899994,11.6,10.285953609));
#220749=CARTESIAN_POINT('Ctrl Pts',(2.66292087099994,15.2,10.288137978));
#220750=CARTESIAN_POINT('Ctrl Pts',(2.66292087099994,11.6,10.288137978));
#220751=CARTESIAN_POINT('Ctrl Pts',(2.66296130999994,15.2,10.290329079));
#220752=CARTESIAN_POINT('Ctrl Pts',(2.66296130999994,11.6,10.290329079));
#220753=CARTESIAN_POINT('Ctrl Pts',(2.66299992499994,15.2,10.292526899));
#220754=CARTESIAN_POINT('Ctrl Pts',(2.66299992499994,11.6,10.292526899));
#220755=CARTESIAN_POINT('Ctrl Pts',(2.66303670499994,15.2,10.294731424));
#220756=CARTESIAN_POINT('Ctrl Pts',(2.66303670499994,11.6,10.294731424));
#220757=CARTESIAN_POINT('Ctrl Pts',(2.66307164099994,15.2,10.29694264));
#220758=CARTESIAN_POINT('Ctrl Pts',(2.66307164099994,11.6,10.29694264));
#220759=CARTESIAN_POINT('Ctrl Pts',(2.66310471899994,15.2,10.299160533));
#220760=CARTESIAN_POINT('Ctrl Pts',(2.66310471899994,11.6,10.299160533));
#220761=CARTESIAN_POINT('Ctrl Pts',(2.66313593099994,15.2,10.301385091));
#220762=CARTESIAN_POINT('Ctrl Pts',(2.66313593099994,11.6,10.301385091));
#220763=CARTESIAN_POINT('Ctrl Pts',(2.66316526499994,15.2,10.3036163));
#220764=CARTESIAN_POINT('Ctrl Pts',(2.66316526499994,11.6,10.3036163));
#220765=CARTESIAN_POINT('Ctrl Pts',(2.66319271099994,15.2,10.305854146));
#220766=CARTESIAN_POINT('Ctrl Pts',(2.66319271099994,11.6,10.305854146));
#220767=CARTESIAN_POINT('Ctrl Pts',(2.66321825799994,15.2,10.308098616));
#220768=CARTESIAN_POINT('Ctrl Pts',(2.66321825799994,11.6,10.308098616));
#220769=CARTESIAN_POINT('Ctrl Pts',(2.66324189699994,15.2,10.310349697));
#220770=CARTESIAN_POINT('Ctrl Pts',(2.66324189699994,11.6,10.310349697));
#220771=CARTESIAN_POINT('Ctrl Pts',(2.66326361499994,15.2,10.312607375));
#220772=CARTESIAN_POINT('Ctrl Pts',(2.66326361499994,11.6,10.312607375));
#220773=CARTESIAN_POINT('Ctrl Pts',(2.66328340399994,15.2,10.314871635));
#220774=CARTESIAN_POINT('Ctrl Pts',(2.66328340399994,11.6,10.314871635));
#220775=CARTESIAN_POINT('Ctrl Pts',(2.66330125199994,15.2,10.317142467));
#220776=CARTESIAN_POINT('Ctrl Pts',(2.66330125199994,11.6,10.317142467));
#220777=CARTESIAN_POINT('Ctrl Pts',(2.66331714899994,15.2,10.319419856));
#220778=CARTESIAN_POINT('Ctrl Pts',(2.66331714899994,11.6,10.319419856));
#220779=CARTESIAN_POINT('Ctrl Pts',(2.66333108599994,15.2,10.321703789));
#220780=CARTESIAN_POINT('Ctrl Pts',(2.66333108599994,11.6,10.321703789));
#220781=CARTESIAN_POINT('Ctrl Pts',(2.66334304999994,15.2,10.323994251));
#220782=CARTESIAN_POINT('Ctrl Pts',(2.66334304999994,11.6,10.323994251));
#220783=CARTESIAN_POINT('Ctrl Pts',(2.66335303299994,15.2,10.326291233));
#220784=CARTESIAN_POINT('Ctrl Pts',(2.66335303299994,11.6,10.326291233));
#220785=CARTESIAN_POINT('Ctrl Pts',(2.66336102399995,15.2,10.328594718));
#220786=CARTESIAN_POINT('Ctrl Pts',(2.66336102399995,11.6,10.328594718));
#220787=CARTESIAN_POINT('Ctrl Pts',(2.66336701299994,15.2,10.330904695));
#220788=CARTESIAN_POINT('Ctrl Pts',(2.66336701299994,11.6,10.330904695));
#220789=CARTESIAN_POINT('Ctrl Pts',(2.66337099099994,15.2,10.33322115));
#220790=CARTESIAN_POINT('Ctrl Pts',(2.66337099099994,11.6,10.33322115));
#220791=CARTESIAN_POINT('Ctrl Pts',(2.66337294499994,15.2,10.33554407));
#220792=CARTESIAN_POINT('Ctrl Pts',(2.66337294499994,11.6,10.33554407));
#220793=CARTESIAN_POINT('Ctrl Pts',(2.66337286799994,15.2,10.337873442));
#220794=CARTESIAN_POINT('Ctrl Pts',(2.66337286799994,11.6,10.337873442));
#220795=CARTESIAN_POINT('Ctrl Pts',(2.66337074899994,15.2,10.340209254));
#220796=CARTESIAN_POINT('Ctrl Pts',(2.66337074899994,11.6,10.340209254));
#220797=CARTESIAN_POINT('Ctrl Pts',(2.66336657799994,15.2,10.342551492));
#220798=CARTESIAN_POINT('Ctrl Pts',(2.66336657799994,11.6,10.342551492));
#220799=CARTESIAN_POINT('Ctrl Pts',(2.66336034299994,15.2,10.344900144));
#220800=CARTESIAN_POINT('Ctrl Pts',(2.66336034299994,11.6,10.344900144));
#220801=CARTESIAN_POINT('Ctrl Pts',(2.66335203699994,15.2,10.347255195));
#220802=CARTESIAN_POINT('Ctrl Pts',(2.66335203699994,11.6,10.347255195));
#220803=CARTESIAN_POINT('Ctrl Pts',(2.66334164999994,15.2,10.349616634));
#220804=CARTESIAN_POINT('Ctrl Pts',(2.66334164999994,11.6,10.349616634));
#220805=CARTESIAN_POINT('Ctrl Pts',(2.66332917099994,15.2,10.351984449));
#220806=CARTESIAN_POINT('Ctrl Pts',(2.66332917099994,11.6,10.351984449));
#220807=CARTESIAN_POINT('Ctrl Pts',(2.66331458999994,15.2,10.354358624));
#220808=CARTESIAN_POINT('Ctrl Pts',(2.66331458999994,11.6,10.354358624));
#220809=CARTESIAN_POINT('Ctrl Pts',(2.66329789899994,15.2,10.35673915));
#220810=CARTESIAN_POINT('Ctrl Pts',(2.66329789899994,11.6,10.35673915));
#220811=CARTESIAN_POINT('Ctrl Pts',(2.66327908599994,15.2,10.359126012));
#220812=CARTESIAN_POINT('Ctrl Pts',(2.66327908599994,11.6,10.359126012));
#220813=CARTESIAN_POINT('Ctrl Pts',(2.66325814399994,15.2,10.361519198));
#220814=CARTESIAN_POINT('Ctrl Pts',(2.66325814399994,11.6,10.361519198));
#220815=CARTESIAN_POINT('Ctrl Pts',(2.66323505999994,15.2,10.363918694));
#220816=CARTESIAN_POINT('Ctrl Pts',(2.66323505999994,11.6,10.363918694));
#220817=CARTESIAN_POINT('Ctrl Pts',(2.66320982799995,15.2,10.36632449));
#220818=CARTESIAN_POINT('Ctrl Pts',(2.66320982799995,11.6,10.36632449));
#220819=CARTESIAN_POINT('Ctrl Pts',(2.66318243599994,15.2,10.368736571));
#220820=CARTESIAN_POINT('Ctrl Pts',(2.66318243599994,11.6,10.368736571));
#220821=CARTESIAN_POINT('Ctrl Pts',(2.66315287499994,15.2,10.371154926));
#220822=CARTESIAN_POINT('Ctrl Pts',(2.66315287499994,11.6,10.371154926));
#220823=CARTESIAN_POINT('Ctrl Pts',(2.66312113599994,15.2,10.37357954));
#220824=CARTESIAN_POINT('Ctrl Pts',(2.66312113599994,11.6,10.37357954));
#220825=CARTESIAN_POINT('Ctrl Pts',(2.66308720999994,15.2,10.376010404));
#220826=CARTESIAN_POINT('Ctrl Pts',(2.66308720999994,11.6,10.376010404));
#220827=CARTESIAN_POINT('Ctrl Pts',(2.66305108599994,15.2,10.378447504));
#220828=CARTESIAN_POINT('Ctrl Pts',(2.66305108599994,11.6,10.378447504));
#220829=CARTESIAN_POINT('Ctrl Pts',(2.66301275499994,15.2,10.380890825));
#220830=CARTESIAN_POINT('Ctrl Pts',(2.66301275499994,11.6,10.380890825));
#220831=CARTESIAN_POINT('Ctrl Pts',(2.66297220899995,15.2,10.383340359));
#220832=CARTESIAN_POINT('Ctrl Pts',(2.66297220899995,11.6,10.383340359));
#220833=CARTESIAN_POINT('Ctrl Pts',(2.66292943799994,15.2,10.385796091));
#220834=CARTESIAN_POINT('Ctrl Pts',(2.66292943799994,11.6,10.385796091));
#220835=CARTESIAN_POINT('Ctrl Pts',(2.66288443199994,15.2,10.388258008));
#220836=CARTESIAN_POINT('Ctrl Pts',(2.66288443199994,11.6,10.388258008));
#220837=CARTESIAN_POINT('Ctrl Pts',(2.66283718399994,15.2,10.3907261));
#220838=CARTESIAN_POINT('Ctrl Pts',(2.66283718399994,11.6,10.3907261));
#220839=CARTESIAN_POINT('Ctrl Pts',(2.66278768199995,15.2,10.393200352));
#220840=CARTESIAN_POINT('Ctrl Pts',(2.66278768199995,11.6,10.393200352));
#220841=CARTESIAN_POINT('Ctrl Pts',(2.66273591799994,15.2,10.395680754));
#220842=CARTESIAN_POINT('Ctrl Pts',(2.66273591799994,11.6,10.395680754));
#220843=CARTESIAN_POINT('Ctrl Pts',(2.66268188299994,15.2,10.398167293));
#220844=CARTESIAN_POINT('Ctrl Pts',(2.66268188299994,11.6,10.398167293));
#220845=CARTESIAN_POINT('Ctrl Pts',(2.66262556799994,15.2,10.400659956));
#220846=CARTESIAN_POINT('Ctrl Pts',(2.66262556799994,11.6,10.400659956));
#220847=CARTESIAN_POINT('Ctrl Pts',(2.66256696299994,15.2,10.40315873));
#220848=CARTESIAN_POINT('Ctrl Pts',(2.66256696299994,11.6,10.40315873));
#220849=CARTESIAN_POINT('Ctrl Pts',(2.66250606099995,15.2,10.405663606));
#220850=CARTESIAN_POINT('Ctrl Pts',(2.66250606099995,11.6,10.405663606));
#220851=CARTESIAN_POINT('Ctrl Pts',(2.66244285099994,15.2,10.408174569));
#220852=CARTESIAN_POINT('Ctrl Pts',(2.66244285099994,11.6,10.408174569));
#220853=CARTESIAN_POINT('Ctrl Pts',(2.66237732499994,15.2,10.410691609));
#220854=CARTESIAN_POINT('Ctrl Pts',(2.66237732499994,11.6,10.410691609));
#220855=CARTESIAN_POINT('Ctrl Pts',(2.66230947199994,15.2,10.413214712));
#220856=CARTESIAN_POINT('Ctrl Pts',(2.66230947199994,11.6,10.413214712));
#220857=CARTESIAN_POINT('Ctrl Pts',(2.66223928699994,15.2,10.415743866));
#220858=CARTESIAN_POINT('Ctrl Pts',(2.66223928699994,11.6,10.415743866));
#220859=CARTESIAN_POINT('Ctrl Pts',(2.66216675899994,15.2,10.418279061));
#220860=CARTESIAN_POINT('Ctrl Pts',(2.66216675899994,11.6,10.418279061));
#220861=CARTESIAN_POINT('Ctrl Pts',(2.66209187899995,15.2,10.420820283));
#220862=CARTESIAN_POINT('Ctrl Pts',(2.66209187899995,11.6,10.420820283));
#220863=CARTESIAN_POINT('Ctrl Pts',(2.66201463799994,15.2,10.42336752));
#220864=CARTESIAN_POINT('Ctrl Pts',(2.66201463799994,11.6,10.42336752));
#220865=CARTESIAN_POINT('Ctrl Pts',(2.66193502799994,15.2,10.425920761));
#220866=CARTESIAN_POINT('Ctrl Pts',(2.66193502799994,11.6,10.425920761));
#220867=CARTESIAN_POINT('Ctrl Pts',(2.66185303999994,15.2,10.428479993));
#220868=CARTESIAN_POINT('Ctrl Pts',(2.66185303999994,11.6,10.428479993));
#220869=CARTESIAN_POINT('Ctrl Pts',(2.66176866499995,15.2,10.431045206));
#220870=CARTESIAN_POINT('Ctrl Pts',(2.66176866499995,11.6,10.431045206));
#220871=CARTESIAN_POINT('Ctrl Pts',(2.66168189399994,15.2,10.433616386));
#220872=CARTESIAN_POINT('Ctrl Pts',(2.66168189399994,11.6,10.433616386));
#220873=CARTESIAN_POINT('Ctrl Pts',(2.66159271899994,15.2,10.436193522));
#220874=CARTESIAN_POINT('Ctrl Pts',(2.66159271899994,11.6,10.436193522));
#220875=CARTESIAN_POINT('Ctrl Pts',(2.66150113199994,15.2,10.438776602));
#220876=CARTESIAN_POINT('Ctrl Pts',(2.66150113199994,11.6,10.438776602));
#220877=CARTESIAN_POINT('Ctrl Pts',(2.66140712299994,15.2,10.441365615));
#220878=CARTESIAN_POINT('Ctrl Pts',(2.66140712299994,11.6,10.441365615));
#220879=CARTESIAN_POINT('Ctrl Pts',(2.66131068499994,15.2,10.443960548));
#220880=CARTESIAN_POINT('Ctrl Pts',(2.66131068499994,11.6,10.443960548));
#220881=CARTESIAN_POINT('Ctrl Pts',(2.66121180899995,15.2,10.44656139));
#220882=CARTESIAN_POINT('Ctrl Pts',(2.66121180899995,11.6,10.44656139));
#220883=CARTESIAN_POINT('Ctrl Pts',(2.66111048499994,15.2,10.449168128));
#220884=CARTESIAN_POINT('Ctrl Pts',(2.66111048499994,11.6,10.449168128));
#220885=CARTESIAN_POINT('Ctrl Pts',(2.66100670699994,15.2,10.451780752));
#220886=CARTESIAN_POINT('Ctrl Pts',(2.66100670699994,11.6,10.451780752));
#220887=CARTESIAN_POINT('Ctrl Pts',(2.66090046499994,15.2,10.45439925));
#220888=CARTESIAN_POINT('Ctrl Pts',(2.66090046499994,11.6,10.45439925));
#220889=CARTESIAN_POINT('Ctrl Pts',(2.66079174899994,15.2,10.457023609));
#220890=CARTESIAN_POINT('Ctrl Pts',(2.66079174899994,11.6,10.457023609));
#220891=CARTESIAN_POINT('Ctrl Pts',(2.66068055499994,15.2,10.459653818));
#220892=CARTESIAN_POINT('Ctrl Pts',(2.66068055499994,11.6,10.459653818));
#220893=CARTESIAN_POINT('Ctrl Pts',(2.66056687099995,15.2,10.462289868));
#220894=CARTESIAN_POINT('Ctrl Pts',(2.66056687099995,11.6,10.462289868));
#220895=CARTESIAN_POINT('Ctrl Pts',(2.66045068999994,15.2,10.464931742));
#220896=CARTESIAN_POINT('Ctrl Pts',(2.66045068999994,11.6,10.464931742));
#220897=CARTESIAN_POINT('Ctrl Pts',(2.66033200499994,15.2,10.467579433));
#220898=CARTESIAN_POINT('Ctrl Pts',(2.66033200499994,11.6,10.467579433));
#220899=CARTESIAN_POINT('Ctrl Pts',(2.66021080499995,15.2,10.470232928));
#220900=CARTESIAN_POINT('Ctrl Pts',(2.66021080499995,11.6,10.470232928));
#220901=CARTESIAN_POINT('Ctrl Pts',(2.66008708299994,15.2,10.472892215));
#220902=CARTESIAN_POINT('Ctrl Pts',(2.66008708299994,11.6,10.472892215));
#220903=CARTESIAN_POINT('Ctrl Pts',(2.65996083199994,15.2,10.475557283));
#220904=CARTESIAN_POINT('Ctrl Pts',(2.65996083199994,11.6,10.475557283));
#220905=CARTESIAN_POINT('Ctrl Pts',(2.65983204199994,15.2,10.47822812));
#220906=CARTESIAN_POINT('Ctrl Pts',(2.65983204199994,11.6,10.47822812));
#220907=CARTESIAN_POINT('Ctrl Pts',(2.65970070699994,15.2,10.480904716));
#220908=CARTESIAN_POINT('Ctrl Pts',(2.65970070699994,11.6,10.480904716));
#220909=CARTESIAN_POINT('Ctrl Pts',(2.65956681699994,15.2,10.483587057));
#220910=CARTESIAN_POINT('Ctrl Pts',(2.65956681699994,11.6,10.483587057));
#220911=CARTESIAN_POINT('Ctrl Pts',(2.65943036399995,15.2,10.486275135));
#220912=CARTESIAN_POINT('Ctrl Pts',(2.65943036399995,11.6,10.486275135));
#220913=CARTESIAN_POINT('Ctrl Pts',(2.65929134199994,15.2,10.488968935));
#220914=CARTESIAN_POINT('Ctrl Pts',(2.65929134199994,11.6,10.488968935));
#220915=CARTESIAN_POINT('Ctrl Pts',(2.65914973999994,15.2,10.491668448));
#220916=CARTESIAN_POINT('Ctrl Pts',(2.65914973999994,11.6,10.491668448));
#220917=CARTESIAN_POINT('Ctrl Pts',(2.65900555199994,15.2,10.494373663));
#220918=CARTESIAN_POINT('Ctrl Pts',(2.65900555199994,11.6,10.494373663));
#220919=CARTESIAN_POINT('Ctrl Pts',(2.65885876999994,15.2,10.497084567));
#220920=CARTESIAN_POINT('Ctrl Pts',(2.65885876999994,11.6,10.497084567));
#220921=CARTESIAN_POINT('Ctrl Pts',(2.65870938599994,15.2,10.499801148));
#220922=CARTESIAN_POINT('Ctrl Pts',(2.65870938599994,11.6,10.499801148));
#220923=CARTESIAN_POINT('Ctrl Pts',(2.65855739099994,15.2,10.502523398));
#220924=CARTESIAN_POINT('Ctrl Pts',(2.65855739099994,11.6,10.502523398));
#220925=CARTESIAN_POINT('Ctrl Pts',(2.65840277899994,15.2,10.505251304));
#220926=CARTESIAN_POINT('Ctrl Pts',(2.65840277899994,11.6,10.505251304));
#220927=CARTESIAN_POINT('Ctrl Pts',(2.65824553999995,15.2,10.507984853));
#220928=CARTESIAN_POINT('Ctrl Pts',(2.65824553999995,11.6,10.507984853));
#220929=CARTESIAN_POINT('Ctrl Pts',(2.65808566799994,15.2,10.510724037));
#220930=CARTESIAN_POINT('Ctrl Pts',(2.65808566799994,11.6,10.510724037));
#220931=CARTESIAN_POINT('Ctrl Pts',(2.65792315399994,15.2,10.513468843));
#220932=CARTESIAN_POINT('Ctrl Pts',(2.65792315399994,11.6,10.513468843));
#220933=CARTESIAN_POINT('Ctrl Pts',(2.65775799099994,15.2,10.51621926));
#220934=CARTESIAN_POINT('Ctrl Pts',(2.65775799099994,11.6,10.51621926));
#220935=CARTESIAN_POINT('Ctrl Pts',(2.65759017099994,15.2,10.518975277));
#220936=CARTESIAN_POINT('Ctrl Pts',(2.65759017099994,11.6,10.518975277));
#220937=CARTESIAN_POINT('Ctrl Pts',(2.65741968699994,15.2,10.521736883));
#220938=CARTESIAN_POINT('Ctrl Pts',(2.65741968699994,11.6,10.521736883));
#220939=CARTESIAN_POINT('Ctrl Pts',(2.65724653099995,15.2,10.524504067));
#220940=CARTESIAN_POINT('Ctrl Pts',(2.65724653099995,11.6,10.524504067));
#220941=CARTESIAN_POINT('Ctrl Pts',(2.65707069399994,15.2,10.527276817));
#220942=CARTESIAN_POINT('Ctrl Pts',(2.65707069399994,11.6,10.527276817));
#220943=CARTESIAN_POINT('Ctrl Pts',(2.65689216999994,15.2,10.530055124));
#220944=CARTESIAN_POINT('Ctrl Pts',(2.65689216999994,11.6,10.530055124));
#220945=CARTESIAN_POINT('Ctrl Pts',(2.65671094999994,15.2,10.532838975));
#220946=CARTESIAN_POINT('Ctrl Pts',(2.65671094999994,11.6,10.532838975));
#220947=CARTESIAN_POINT('Ctrl Pts',(2.65652702799994,15.2,10.535628359));
#220948=CARTESIAN_POINT('Ctrl Pts',(2.65652702799994,11.6,10.535628359));
#220949=CARTESIAN_POINT('Ctrl Pts',(2.65634039499994,15.2,10.538423266));
#220950=CARTESIAN_POINT('Ctrl Pts',(2.65634039499994,11.6,10.538423266));
#220951=CARTESIAN_POINT('Ctrl Pts',(2.65615104499994,15.2,10.541223686));
#220952=CARTESIAN_POINT('Ctrl Pts',(2.65615104499994,11.6,10.541223686));
#220953=CARTESIAN_POINT('Ctrl Pts',(2.65595896999994,15.2,10.544029606));
#220954=CARTESIAN_POINT('Ctrl Pts',(2.65595896999994,11.6,10.544029606));
#220955=CARTESIAN_POINT('Ctrl Pts',(2.65576416199994,15.2,10.546841015));
#220956=CARTESIAN_POINT('Ctrl Pts',(2.65576416199994,11.6,10.546841015));
#220957=CARTESIAN_POINT('Ctrl Pts',(2.65556661299994,15.2,10.549657904));
#220958=CARTESIAN_POINT('Ctrl Pts',(2.65556661299994,11.6,10.549657904));
#220959=CARTESIAN_POINT('Ctrl Pts',(2.65536631799994,15.2,10.552480261));
#220960=CARTESIAN_POINT('Ctrl Pts',(2.65536631799994,11.6,10.552480261));
#220961=CARTESIAN_POINT('Ctrl Pts',(2.65516326699994,15.2,10.555308075));
#220962=CARTESIAN_POINT('Ctrl Pts',(2.65516326699994,11.6,10.555308075));
#220963=CARTESIAN_POINT('Ctrl Pts',(2.65495745399994,15.2,10.558141336));
#220964=CARTESIAN_POINT('Ctrl Pts',(2.65495745399994,11.6,10.558141336));
#220965=CARTESIAN_POINT('Ctrl Pts',(2.65474887199994,15.2,10.560980032));
#220966=CARTESIAN_POINT('Ctrl Pts',(2.65474887199994,11.6,10.560980032));
#220967=CARTESIAN_POINT('Ctrl Pts',(2.65453751199995,15.2,10.563824153));
#220968=CARTESIAN_POINT('Ctrl Pts',(2.65453751199995,11.6,10.563824153));
#220969=CARTESIAN_POINT('Ctrl Pts',(2.65432336899994,15.2,10.566673688));
#220970=CARTESIAN_POINT('Ctrl Pts',(2.65432336899994,11.6,10.566673688));
#220971=CARTESIAN_POINT('Ctrl Pts',(2.65410643399994,15.2,10.569528625));
#220972=CARTESIAN_POINT('Ctrl Pts',(2.65410643399994,11.6,10.569528625));
#220973=CARTESIAN_POINT('Ctrl Pts',(2.65388669999994,15.2,10.572388957));
#220974=CARTESIAN_POINT('Ctrl Pts',(2.65388669999994,11.6,10.572388957));
#220975=CARTESIAN_POINT('Ctrl Pts',(2.65366415999994,15.2,10.575254668));
#220976=CARTESIAN_POINT('Ctrl Pts',(2.65366415999994,11.6,10.575254668));
#220977=CARTESIAN_POINT('Ctrl Pts',(2.65343880799994,15.2,10.578125753));
#220978=CARTESIAN_POINT('Ctrl Pts',(2.65343880799994,11.6,10.578125753));
#220979=CARTESIAN_POINT('Ctrl Pts',(2.65321063499994,15.2,10.581002197));
#220980=CARTESIAN_POINT('Ctrl Pts',(2.65321063499994,11.6,10.581002197));
#220981=CARTESIAN_POINT('Ctrl Pts',(2.65297963499994,15.2,10.583883991));
#220982=CARTESIAN_POINT('Ctrl Pts',(2.65297963499994,11.6,10.583883991));
#220983=CARTESIAN_POINT('Ctrl Pts',(2.65274580099994,15.2,10.586771124));
#220984=CARTESIAN_POINT('Ctrl Pts',(2.65274580099994,11.6,10.586771124));
#220985=CARTESIAN_POINT('Ctrl Pts',(2.65250912499994,15.2,10.589663585));
#220986=CARTESIAN_POINT('Ctrl Pts',(2.65250912499994,11.6,10.589663585));
#220987=CARTESIAN_POINT('Ctrl Pts',(2.65226959999994,15.2,10.592561365));
#220988=CARTESIAN_POINT('Ctrl Pts',(2.65226959999994,11.6,10.592561365));
#220989=CARTESIAN_POINT('Ctrl Pts',(2.65202722099994,15.2,10.595464452));
#220990=CARTESIAN_POINT('Ctrl Pts',(2.65202722099994,11.6,10.595464452));
#220991=CARTESIAN_POINT('Ctrl Pts',(2.65178197899994,15.2,10.598372837));
#220992=CARTESIAN_POINT('Ctrl Pts',(2.65178197899994,11.6,10.598372837));
#220993=CARTESIAN_POINT('Ctrl Pts',(2.65153386699994,15.2,10.601286506));
#220994=CARTESIAN_POINT('Ctrl Pts',(2.65153386699994,11.6,10.601286506));
#220995=CARTESIAN_POINT('Ctrl Pts',(2.65128287799994,15.2,10.604205452));
#220996=CARTESIAN_POINT('Ctrl Pts',(2.65128287799994,11.6,10.604205452));
#220997=CARTESIAN_POINT('Ctrl Pts',(2.65102900699994,15.2,10.607129663));
#220998=CARTESIAN_POINT('Ctrl Pts',(2.65102900699994,11.6,10.607129663));
#220999=CARTESIAN_POINT('Ctrl Pts',(2.65077224499994,15.2,10.61005913));
#221000=CARTESIAN_POINT('Ctrl Pts',(2.65077224499994,11.6,10.61005913));
#221001=CARTESIAN_POINT('Ctrl Pts',(2.65051258499994,15.2,10.61299384));
#221002=CARTESIAN_POINT('Ctrl Pts',(2.65051258499994,11.6,10.61299384));
#221003=CARTESIAN_POINT('Ctrl Pts',(2.65025002199994,15.2,10.615933784));
#221004=CARTESIAN_POINT('Ctrl Pts',(2.65025002199994,11.6,10.615933784));
#221005=CARTESIAN_POINT('Ctrl Pts',(2.64998454799994,15.2,10.618878952));
#221006=CARTESIAN_POINT('Ctrl Pts',(2.64998454799994,11.6,10.618878952));
#221007=CARTESIAN_POINT('Ctrl Pts',(2.64971615599995,15.2,10.621829333));
#221008=CARTESIAN_POINT('Ctrl Pts',(2.64971615599995,11.6,10.621829333));
#221009=CARTESIAN_POINT('Ctrl Pts',(2.64944483999995,15.2,10.624784916));
#221010=CARTESIAN_POINT('Ctrl Pts',(2.64944483999995,11.6,10.624784916));
#221011=CARTESIAN_POINT('Ctrl Pts',(2.64917059199994,15.2,10.627745693));
#221012=CARTESIAN_POINT('Ctrl Pts',(2.64917059199994,11.6,10.627745693));
#221013=CARTESIAN_POINT('Ctrl Pts',(2.64889340699995,15.2,10.63071165));
#221014=CARTESIAN_POINT('Ctrl Pts',(2.64889340699995,11.6,10.63071165));
#221015=CARTESIAN_POINT('Ctrl Pts',(2.64861327699994,15.2,10.63368278));
#221016=CARTESIAN_POINT('Ctrl Pts',(2.64861327699994,11.6,10.63368278));
#221017=CARTESIAN_POINT('Ctrl Pts',(2.64833019499994,15.2,10.636659071));
#221018=CARTESIAN_POINT('Ctrl Pts',(2.64833019499994,11.6,10.636659071));
#221019=CARTESIAN_POINT('Ctrl Pts',(2.64804415599994,15.2,10.639640513));
#221020=CARTESIAN_POINT('Ctrl Pts',(2.64804415599994,11.6,10.639640513));
#221021=CARTESIAN_POINT('Ctrl Pts',(2.64775515099994,15.2,10.642627096));
#221022=CARTESIAN_POINT('Ctrl Pts',(2.64775515099994,11.6,10.642627096));
#221023=CARTESIAN_POINT('Ctrl Pts',(2.64746317599994,15.2,10.645618809));
#221024=CARTESIAN_POINT('Ctrl Pts',(2.64746317599994,11.6,10.645618809));
#221025=CARTESIAN_POINT('Ctrl Pts',(2.64716822299994,15.2,10.648615642));
#221026=CARTESIAN_POINT('Ctrl Pts',(2.64716822299994,11.6,10.648615642));
#221027=CARTESIAN_POINT('Ctrl Pts',(2.64687028499994,15.2,10.651617586));
#221028=CARTESIAN_POINT('Ctrl Pts',(2.64687028499994,11.6,10.651617586));
#221029=CARTESIAN_POINT('Ctrl Pts',(2.64656935599994,15.2,10.65462463));
#221030=CARTESIAN_POINT('Ctrl Pts',(2.64656935599994,11.6,10.65462463));
#221031=CARTESIAN_POINT('Ctrl Pts',(2.64626542899994,15.2,10.657636762));
#221032=CARTESIAN_POINT('Ctrl Pts',(2.64626542899994,11.6,10.657636762));
#221033=CARTESIAN_POINT('Ctrl Pts',(2.64595849899994,15.2,10.660653975));
#221034=CARTESIAN_POINT('Ctrl Pts',(2.64595849899994,11.6,10.660653975));
#221035=CARTESIAN_POINT('Ctrl Pts',(2.64564855699994,15.2,10.663676257));
#221036=CARTESIAN_POINT('Ctrl Pts',(2.64564855699994,11.6,10.663676257));
#221037=CARTESIAN_POINT('Ctrl Pts',(2.64533559999995,15.2,10.666703598));
#221038=CARTESIAN_POINT('Ctrl Pts',(2.64533559999995,11.6,10.666703598));
#221039=CARTESIAN_POINT('Ctrl Pts',(2.64501961799994,15.2,10.669735989));
#221040=CARTESIAN_POINT('Ctrl Pts',(2.64501961799994,11.6,10.669735989));
#221041=CARTESIAN_POINT('Ctrl Pts',(2.64470060599994,15.2,10.672773419));
#221042=CARTESIAN_POINT('Ctrl Pts',(2.64470060599994,11.6,10.672773419));
#221043=CARTESIAN_POINT('Ctrl Pts',(2.64437855799994,15.2,10.675815876));
#221044=CARTESIAN_POINT('Ctrl Pts',(2.64437855799994,11.6,10.675815876));
#221045=CARTESIAN_POINT('Ctrl Pts',(2.64405346699994,15.2,10.678863354));
#221046=CARTESIAN_POINT('Ctrl Pts',(2.64405346699994,11.6,10.678863354));
#221047=CARTESIAN_POINT('Ctrl Pts',(2.64372532799994,15.2,10.68191584));
#221048=CARTESIAN_POINT('Ctrl Pts',(2.64372532799994,11.6,10.68191584));
#221049=CARTESIAN_POINT('Ctrl Pts',(2.64339413299994,15.2,10.684973325));
#221050=CARTESIAN_POINT('Ctrl Pts',(2.64339413299994,11.6,10.684973325));
#221051=CARTESIAN_POINT('Ctrl Pts',(2.64305987599994,15.2,10.688035799));
#221052=CARTESIAN_POINT('Ctrl Pts',(2.64305987599994,11.6,10.688035799));
#221053=CARTESIAN_POINT('Ctrl Pts',(2.64272255199994,15.2,10.691103251));
#221054=CARTESIAN_POINT('Ctrl Pts',(2.64272255199994,11.6,10.691103251));
#221055=CARTESIAN_POINT('Ctrl Pts',(2.64238215299994,15.2,10.694175673));
#221056=CARTESIAN_POINT('Ctrl Pts',(2.64238215299994,11.6,10.694175673));
#221057=CARTESIAN_POINT('Ctrl Pts',(2.64203867399994,15.2,10.697253054));
#221058=CARTESIAN_POINT('Ctrl Pts',(2.64203867399994,11.6,10.697253054));
#221059=CARTESIAN_POINT('Ctrl Pts',(2.64169210799994,15.2,10.700335382));
#221060=CARTESIAN_POINT('Ctrl Pts',(2.64169210799994,11.6,10.700335382));
#221061=CARTESIAN_POINT('Ctrl Pts',(2.64134244799994,15.2,10.703422651));
#221062=CARTESIAN_POINT('Ctrl Pts',(2.64134244799994,11.6,10.703422651));
#221063=CARTESIAN_POINT('Ctrl Pts',(2.64098969099994,15.2,10.706514848));
#221064=CARTESIAN_POINT('Ctrl Pts',(2.64098969099994,11.6,10.706514848));
#221065=CARTESIAN_POINT('Ctrl Pts',(2.64063382699995,15.2,10.709611966));
#221066=CARTESIAN_POINT('Ctrl Pts',(2.64063382699995,11.6,10.709611966));
#221067=CARTESIAN_POINT('Ctrl Pts',(2.64027485199994,15.2,10.712713991));
#221068=CARTESIAN_POINT('Ctrl Pts',(2.64027485199994,11.6,10.712713991));
#221069=CARTESIAN_POINT('Ctrl Pts',(2.63991275999994,15.2,10.715820917));
#221070=CARTESIAN_POINT('Ctrl Pts',(2.63991275999994,11.6,10.715820917));
#221071=CARTESIAN_POINT('Ctrl Pts',(2.63954754299994,15.2,10.718932732));
#221072=CARTESIAN_POINT('Ctrl Pts',(2.63954754299994,11.6,10.718932732));
#221073=CARTESIAN_POINT('Ctrl Pts',(2.63917919799994,15.2,10.722049427));
#221074=CARTESIAN_POINT('Ctrl Pts',(2.63917919799994,11.6,10.722049427));
#221075=CARTESIAN_POINT('Ctrl Pts',(2.63880771699994,15.2,10.725170991));
#221076=CARTESIAN_POINT('Ctrl Pts',(2.63880771699994,11.6,10.725170991));
#221077=CARTESIAN_POINT('Ctrl Pts',(2.63843309399994,15.2,10.728297417));
#221078=CARTESIAN_POINT('Ctrl Pts',(2.63843309399994,11.6,10.728297417));
#221079=CARTESIAN_POINT('Ctrl Pts',(2.63805532199994,15.2,10.731428692));
#221080=CARTESIAN_POINT('Ctrl Pts',(2.63805532199994,11.6,10.731428692));
#221081=CARTESIAN_POINT('Ctrl Pts',(2.63767439799994,15.2,10.734564809));
#221082=CARTESIAN_POINT('Ctrl Pts',(2.63767439799994,11.6,10.734564809));
#221083=CARTESIAN_POINT('Ctrl Pts',(2.63729031299994,15.2,10.737705755));
#221084=CARTESIAN_POINT('Ctrl Pts',(2.63729031299994,11.6,10.737705755));
#221085=CARTESIAN_POINT('Ctrl Pts',(2.63690306199994,15.2,10.740851524));
#221086=CARTESIAN_POINT('Ctrl Pts',(2.63690306199994,11.6,10.740851524));
#221087=CARTESIAN_POINT('Ctrl Pts',(2.63651263999995,15.2,10.744002104));
#221088=CARTESIAN_POINT('Ctrl Pts',(2.63651263999995,11.6,10.744002104));
#221089=CARTESIAN_POINT('Ctrl Pts',(2.63611903999994,15.2,10.747157485));
#221090=CARTESIAN_POINT('Ctrl Pts',(2.63611903999994,11.6,10.747157485));
#221091=CARTESIAN_POINT('Ctrl Pts',(2.63572225699995,15.2,10.750317659));
#221092=CARTESIAN_POINT('Ctrl Pts',(2.63572225699995,11.6,10.750317659));
#221093=CARTESIAN_POINT('Ctrl Pts',(2.63532228399994,15.2,10.753482615));
#221094=CARTESIAN_POINT('Ctrl Pts',(2.63532228399994,11.6,10.753482615));
#221095=CARTESIAN_POINT('Ctrl Pts',(2.63491911699994,15.2,10.756652344));
#221096=CARTESIAN_POINT('Ctrl Pts',(2.63491911699994,11.6,10.756652344));
#221097=CARTESIAN_POINT('Ctrl Pts',(2.63451274799994,15.2,10.759826836));
#221098=CARTESIAN_POINT('Ctrl Pts',(2.63451274799994,11.6,10.759826836));
#221099=CARTESIAN_POINT('Ctrl Pts',(2.63410317099994,15.2,10.763006082));
#221100=CARTESIAN_POINT('Ctrl Pts',(2.63410317099994,11.6,10.763006082));
#221101=CARTESIAN_POINT('Ctrl Pts',(2.63369038199994,15.2,10.766190072));
#221102=CARTESIAN_POINT('Ctrl Pts',(2.63369038199994,11.6,10.766190072));
#221103=CARTESIAN_POINT('Ctrl Pts',(2.63327437499994,15.2,10.769378796));
#221104=CARTESIAN_POINT('Ctrl Pts',(2.63327437499994,11.6,10.769378796));
#221105=CARTESIAN_POINT('Ctrl Pts',(2.63285514299994,15.2,10.772572244));
#221106=CARTESIAN_POINT('Ctrl Pts',(2.63285514299994,11.6,10.772572244));
#221107=CARTESIAN_POINT('Ctrl Pts',(2.63243268299994,15.2,10.775770408));
#221108=CARTESIAN_POINT('Ctrl Pts',(2.63243268299994,11.6,10.775770408));
#221109=CARTESIAN_POINT('Ctrl Pts',(2.63200698499995,15.2,10.778973278));
#221110=CARTESIAN_POINT('Ctrl Pts',(2.63200698499995,11.6,10.778973278));
#221111=CARTESIAN_POINT('Ctrl Pts',(2.63157804599994,15.2,10.782180844));
#221112=CARTESIAN_POINT('Ctrl Pts',(2.63157804599994,11.6,10.782180844));
#221113=CARTESIAN_POINT('Ctrl Pts',(2.63114586099995,15.2,10.785393097));
#221114=CARTESIAN_POINT('Ctrl Pts',(2.63114586099995,11.6,10.785393097));
#221115=CARTESIAN_POINT('Ctrl Pts',(2.63071042299994,15.2,10.788610025));
#221116=CARTESIAN_POINT('Ctrl Pts',(2.63071042299994,11.6,10.788610025));
#221117=CARTESIAN_POINT('Ctrl Pts',(2.63027172599994,15.2,10.791831623));
#221118=CARTESIAN_POINT('Ctrl Pts',(2.63027172599994,11.6,10.791831623));
#221119=CARTESIAN_POINT('Ctrl Pts',(2.62982976499994,15.2,10.795057878));
#221120=CARTESIAN_POINT('Ctrl Pts',(2.62982976499994,11.6,10.795057878));
#221121=CARTESIAN_POINT('Ctrl Pts',(2.62938453499994,15.2,10.798288782));
#221122=CARTESIAN_POINT('Ctrl Pts',(2.62938453499994,11.6,10.798288782));
#221123=CARTESIAN_POINT('Ctrl Pts',(2.62893602899994,15.2,10.801524325));
#221124=CARTESIAN_POINT('Ctrl Pts',(2.62893602899994,11.6,10.801524325));
#221125=CARTESIAN_POINT('Ctrl Pts',(2.62848424199994,15.2,10.804764499));
#221126=CARTESIAN_POINT('Ctrl Pts',(2.62848424199994,11.6,10.804764499));
#221127=CARTESIAN_POINT('Ctrl Pts',(2.62802916999994,15.2,10.808009293));
#221128=CARTESIAN_POINT('Ctrl Pts',(2.62802916999994,11.6,10.808009293));
#221129=CARTESIAN_POINT('Ctrl Pts',(2.62757080599994,15.2,10.811258697));
#221130=CARTESIAN_POINT('Ctrl Pts',(2.62757080599994,11.6,10.811258697));
#221131=CARTESIAN_POINT('Ctrl Pts',(2.62710914299995,15.2,10.814512704));
#221132=CARTESIAN_POINT('Ctrl Pts',(2.62710914299995,11.6,10.814512704));
#221133=CARTESIAN_POINT('Ctrl Pts',(2.62664417899994,15.2,10.817771303));
#221134=CARTESIAN_POINT('Ctrl Pts',(2.62664417899994,11.6,10.817771303));
#221135=CARTESIAN_POINT('Ctrl Pts',(2.62617590599994,15.2,10.821034484));
#221136=CARTESIAN_POINT('Ctrl Pts',(2.62617590599994,11.6,10.821034484));
#221137=CARTESIAN_POINT('Ctrl Pts',(2.62570431899994,15.2,10.82430224));
#221138=CARTESIAN_POINT('Ctrl Pts',(2.62570431899994,11.6,10.82430224));
#221139=CARTESIAN_POINT('Ctrl Pts',(2.62522941199994,15.2,10.82757456));
#221140=CARTESIAN_POINT('Ctrl Pts',(2.62522941199994,11.6,10.82757456));
#221141=CARTESIAN_POINT('Ctrl Pts',(2.62475118199994,15.2,10.830851435));
#221142=CARTESIAN_POINT('Ctrl Pts',(2.62475118199994,11.6,10.830851435));
#221143=CARTESIAN_POINT('Ctrl Pts',(2.62426961999994,15.2,10.834132855));
#221144=CARTESIAN_POINT('Ctrl Pts',(2.62426961999994,11.6,10.834132855));
#221145=CARTESIAN_POINT('Ctrl Pts',(2.62378472399994,15.2,10.837418812));
#221146=CARTESIAN_POINT('Ctrl Pts',(2.62378472399994,11.6,10.837418812));
#221147=CARTESIAN_POINT('Ctrl Pts',(2.62329648699994,15.2,10.840709296));
#221148=CARTESIAN_POINT('Ctrl Pts',(2.62329648699994,11.6,10.840709296));
#221149=CARTESIAN_POINT('Ctrl Pts',(2.62280490399994,15.2,10.844004298));
#221150=CARTESIAN_POINT('Ctrl Pts',(2.62280490399994,11.6,10.844004298));
#221151=CARTESIAN_POINT('Ctrl Pts',(2.62230996799994,15.2,10.847303809));
#221152=CARTESIAN_POINT('Ctrl Pts',(2.62230996799994,11.6,10.847303809));
#221153=CARTESIAN_POINT('Ctrl Pts',(2.62181167599994,15.2,10.850607819));
#221154=CARTESIAN_POINT('Ctrl Pts',(2.62181167599994,11.6,10.850607819));
#221155=CARTESIAN_POINT('Ctrl Pts',(2.62131002299994,15.2,10.85391632));
#221156=CARTESIAN_POINT('Ctrl Pts',(2.62131002299994,11.6,10.85391632));
#221157=CARTESIAN_POINT('Ctrl Pts',(2.62080500299994,15.2,10.857229301));
#221158=CARTESIAN_POINT('Ctrl Pts',(2.62080500299994,11.6,10.857229301));
#221159=CARTESIAN_POINT('Ctrl Pts',(2.62029660899994,15.2,10.860546755));
#221160=CARTESIAN_POINT('Ctrl Pts',(2.62029660899994,11.6,10.860546755));
#221161=CARTESIAN_POINT('Ctrl Pts',(2.61978483699994,15.2,10.86386867));
#221162=CARTESIAN_POINT('Ctrl Pts',(2.61978483699994,11.6,10.86386867));
#221163=CARTESIAN_POINT('Ctrl Pts',(2.61926968199994,15.2,10.86719504));
#221164=CARTESIAN_POINT('Ctrl Pts',(2.61926968199994,11.6,10.86719504));
#221165=CARTESIAN_POINT('Ctrl Pts',(2.61875113899994,15.2,10.870525854));
#221166=CARTESIAN_POINT('Ctrl Pts',(2.61875113899994,11.6,10.870525854));
#221167=CARTESIAN_POINT('Ctrl Pts',(2.61822920199994,15.2,10.873861104));
#221168=CARTESIAN_POINT('Ctrl Pts',(2.61822920199994,11.6,10.873861104));
#221169=CARTESIAN_POINT('Ctrl Pts',(2.61770386699994,15.2,10.877200779));
#221170=CARTESIAN_POINT('Ctrl Pts',(2.61770386699994,11.6,10.877200779));
#221171=CARTESIAN_POINT('Ctrl Pts',(2.61717512799994,15.2,10.880544872));
#221172=CARTESIAN_POINT('Ctrl Pts',(2.61717512799994,11.6,10.880544872));
#221173=CARTESIAN_POINT('Ctrl Pts',(2.61664297999994,15.2,10.883893373));
#221174=CARTESIAN_POINT('Ctrl Pts',(2.61664297999994,11.6,10.883893373));
#221175=CARTESIAN_POINT('Ctrl Pts',(2.61610741899994,15.2,10.887246272));
#221176=CARTESIAN_POINT('Ctrl Pts',(2.61610741899994,11.6,10.887246272));
#221177=CARTESIAN_POINT('Ctrl Pts',(2.61556843699994,15.2,10.890603562));
#221178=CARTESIAN_POINT('Ctrl Pts',(2.61556843699994,11.6,10.890603562));
#221179=CARTESIAN_POINT('Ctrl Pts',(2.61502603099995,15.2,10.893965232));
#221180=CARTESIAN_POINT('Ctrl Pts',(2.61502603099995,11.6,10.893965232));
#221181=CARTESIAN_POINT('Ctrl Pts',(2.61448019699994,15.2,10.897331274));
#221182=CARTESIAN_POINT('Ctrl Pts',(2.61448019699994,11.6,10.897331274));
#221183=CARTESIAN_POINT('Ctrl Pts',(2.61393092799994,15.2,10.900701679));
#221184=CARTESIAN_POINT('Ctrl Pts',(2.61393092799994,11.6,10.900701679));
#221185=CARTESIAN_POINT('Ctrl Pts',(2.61337821899994,15.2,10.904076437));
#221186=CARTESIAN_POINT('Ctrl Pts',(2.61337821899994,11.6,10.904076437));
#221187=CARTESIAN_POINT('Ctrl Pts',(2.61282206599994,15.2,10.907455542));
#221188=CARTESIAN_POINT('Ctrl Pts',(2.61282206599994,11.6,10.907455542));
#221189=CARTESIAN_POINT('Ctrl Pts',(2.61226246399994,15.2,10.910838981));
#221190=CARTESIAN_POINT('Ctrl Pts',(2.61226246399994,11.6,10.910838981));
#221191=CARTESIAN_POINT('Ctrl Pts',(2.61169940699994,15.2,10.914226746));
#221192=CARTESIAN_POINT('Ctrl Pts',(2.61169940699994,11.6,10.914226746));
#221193=CARTESIAN_POINT('Ctrl Pts',(2.61113289099994,15.2,10.917618831));
#221194=CARTESIAN_POINT('Ctrl Pts',(2.61113289099994,11.6,10.917618831));
#221195=CARTESIAN_POINT('Ctrl Pts',(2.61056290999994,15.2,10.921015224));
#221196=CARTESIAN_POINT('Ctrl Pts',(2.61056290999994,11.6,10.921015224));
#221197=CARTESIAN_POINT('Ctrl Pts',(2.60998946099994,15.2,10.924415916));
#221198=CARTESIAN_POINT('Ctrl Pts',(2.60998946099994,11.6,10.924415916));
#221199=CARTESIAN_POINT('Ctrl Pts',(2.60941253699994,15.2,10.9278209));
#221200=CARTESIAN_POINT('Ctrl Pts',(2.60941253699994,11.6,10.9278209));
#221201=CARTESIAN_POINT('Ctrl Pts',(2.60883213299994,15.2,10.931230167));
#221202=CARTESIAN_POINT('Ctrl Pts',(2.60883213299994,11.6,10.931230167));
#221203=CARTESIAN_POINT('Ctrl Pts',(2.60824824599994,15.2,10.934643706));
#221204=CARTESIAN_POINT('Ctrl Pts',(2.60824824599994,11.6,10.934643706));
#221205=CARTESIAN_POINT('Ctrl Pts',(2.60766086999995,15.2,10.93806151));
#221206=CARTESIAN_POINT('Ctrl Pts',(2.60766086999995,11.6,10.93806151));
#221207=CARTESIAN_POINT('Ctrl Pts',(2.60706999999994,15.2,10.941483569));
#221208=CARTESIAN_POINT('Ctrl Pts',(2.60706999999994,11.6,10.941483569));
#221209=CARTESIAN_POINT('Ctrl Pts',(2.60647563299994,15.2,10.944909876));
#221210=CARTESIAN_POINT('Ctrl Pts',(2.60647563299994,11.6,10.944909876));
#221211=CARTESIAN_POINT('Ctrl Pts',(2.60587776199994,15.2,10.94834042));
#221212=CARTESIAN_POINT('Ctrl Pts',(2.60587776199994,11.6,10.94834042));
#221213=CARTESIAN_POINT('Ctrl Pts',(2.60527638099994,15.2,10.951775193));
#221214=CARTESIAN_POINT('Ctrl Pts',(2.60527638099994,11.6,10.951775193));
#221215=CARTESIAN_POINT('Ctrl Pts',(2.60467148899994,15.2,10.955214187));
#221216=CARTESIAN_POINT('Ctrl Pts',(2.60467148899994,11.6,10.955214187));
#221217=CARTESIAN_POINT('Ctrl Pts',(2.60406307899995,15.2,10.958657392));
#221218=CARTESIAN_POINT('Ctrl Pts',(2.60406307899995,11.6,10.958657392));
#221219=CARTESIAN_POINT('Ctrl Pts',(2.60345114599994,15.2,10.9621048));
#221220=CARTESIAN_POINT('Ctrl Pts',(2.60345114599994,11.6,10.9621048));
#221221=CARTESIAN_POINT('Ctrl Pts',(2.60283568599994,15.2,10.965556401));
#221222=CARTESIAN_POINT('Ctrl Pts',(2.60283568599994,11.6,10.965556401));
#221223=CARTESIAN_POINT('Ctrl Pts',(2.60221669299994,15.2,10.969012187));
#221224=CARTESIAN_POINT('Ctrl Pts',(2.60221669299994,11.6,10.969012187));
#221225=CARTESIAN_POINT('Ctrl Pts',(2.60159416499994,15.2,10.972472151));
#221226=CARTESIAN_POINT('Ctrl Pts',(2.60159416499994,11.6,10.972472151));
#221227=CARTESIAN_POINT('Ctrl Pts',(2.60096809499994,15.2,10.975936282));
#221228=CARTESIAN_POINT('Ctrl Pts',(2.60096809499994,11.6,10.975936282));
#221229=CARTESIAN_POINT('Ctrl Pts',(2.60033847899994,15.2,10.979404571));
#221230=CARTESIAN_POINT('Ctrl Pts',(2.60033847899994,11.6,10.979404571));
#221231=CARTESIAN_POINT('Ctrl Pts',(2.59970531199994,15.2,10.982877011));
#221232=CARTESIAN_POINT('Ctrl Pts',(2.59970531199994,11.6,10.982877011));
#221233=CARTESIAN_POINT('Ctrl Pts',(2.59906858999994,15.2,10.986353591));
#221234=CARTESIAN_POINT('Ctrl Pts',(2.59906858999994,11.6,10.986353591));
#221235=CARTESIAN_POINT('Ctrl Pts',(2.59842830799994,15.2,10.989834306));
#221236=CARTESIAN_POINT('Ctrl Pts',(2.59842830799994,11.6,10.989834306));
#221237=CARTESIAN_POINT('Ctrl Pts',(2.59778446099994,15.2,10.993319144));
#221238=CARTESIAN_POINT('Ctrl Pts',(2.59778446099994,11.6,10.993319144));
#221239=CARTESIAN_POINT('Ctrl Pts',(2.59713704599994,15.2,10.996808097));
#221240=CARTESIAN_POINT('Ctrl Pts',(2.59713704599994,11.6,10.996808097));
#221241=CARTESIAN_POINT('Ctrl Pts',(2.59648605699994,15.2,11.000301157));
#221242=CARTESIAN_POINT('Ctrl Pts',(2.59648605699994,11.6,11.000301157));
#221243=CARTESIAN_POINT('Ctrl Pts',(2.59583148899994,15.2,11.003798316));
#221244=CARTESIAN_POINT('Ctrl Pts',(2.59583148899994,11.6,11.003798316));
#221245=CARTESIAN_POINT('Ctrl Pts',(2.59517333799994,15.2,11.007299564));
#221246=CARTESIAN_POINT('Ctrl Pts',(2.59517333799994,11.6,11.007299564));
#221247=CARTESIAN_POINT('Ctrl Pts',(2.59451159899994,15.2,11.010804893));
#221248=CARTESIAN_POINT('Ctrl Pts',(2.59451159899994,11.6,11.010804893));
#221249=CARTESIAN_POINT('Ctrl Pts',(2.59384626999994,15.2,11.014314294));
#221250=CARTESIAN_POINT('Ctrl Pts',(2.59384626999994,11.6,11.014314294));
#221251=CARTESIAN_POINT('Ctrl Pts',(2.59317734299994,15.2,11.017827759));
#221252=CARTESIAN_POINT('Ctrl Pts',(2.59317734299994,11.6,11.017827759));
#221253=CARTESIAN_POINT('Ctrl Pts',(2.59250481599994,15.2,11.021345279));
#221254=CARTESIAN_POINT('Ctrl Pts',(2.59250481599994,11.6,11.021345279));
#221255=CARTESIAN_POINT('Ctrl Pts',(2.59182868199994,15.2,11.024866846));
#221256=CARTESIAN_POINT('Ctrl Pts',(2.59182868199994,11.6,11.024866846));
#221257=CARTESIAN_POINT('Ctrl Pts',(2.59114893999994,15.2,11.02839245));
#221258=CARTESIAN_POINT('Ctrl Pts',(2.59114893999994,11.6,11.02839245));
#221259=CARTESIAN_POINT('Ctrl Pts',(2.59046558299994,15.2,11.031922084));
#221260=CARTESIAN_POINT('Ctrl Pts',(2.59046558299994,11.6,11.031922084));
#221261=CARTESIAN_POINT('Ctrl Pts',(2.58977860699994,15.2,11.035455739));
#221262=CARTESIAN_POINT('Ctrl Pts',(2.58977860699994,11.6,11.035455739));
#221263=CARTESIAN_POINT('Ctrl Pts',(2.58908800699994,15.2,11.038993406));
#221264=CARTESIAN_POINT('Ctrl Pts',(2.58908800699994,11.6,11.038993406));
#221265=CARTESIAN_POINT('Ctrl Pts',(2.58839378099994,15.2,11.042535078));
#221266=CARTESIAN_POINT('Ctrl Pts',(2.58839378099994,11.6,11.042535078));
#221267=CARTESIAN_POINT('Ctrl Pts',(2.58769592199994,15.2,11.046080744));
#221268=CARTESIAN_POINT('Ctrl Pts',(2.58769592199994,11.6,11.046080744));
#221269=CARTESIAN_POINT('Ctrl Pts',(2.58699442799994,15.2,11.049630398));
#221270=CARTESIAN_POINT('Ctrl Pts',(2.58699442799994,11.6,11.049630398));
#221271=CARTESIAN_POINT('Ctrl Pts',(2.58628929199994,15.2,11.05318403));
#221272=CARTESIAN_POINT('Ctrl Pts',(2.58628929199994,11.6,11.05318403));
#221273=CARTESIAN_POINT('Ctrl Pts',(2.58558051099994,15.2,11.056741632));
#221274=CARTESIAN_POINT('Ctrl Pts',(2.58558051099994,11.6,11.056741632));
#221275=CARTESIAN_POINT('Ctrl Pts',(2.58486808099994,15.2,11.060303195));
#221276=CARTESIAN_POINT('Ctrl Pts',(2.58486808099994,11.6,11.060303195));
#221277=CARTESIAN_POINT('Ctrl Pts',(2.58415199599995,15.2,11.06386871));
#221278=CARTESIAN_POINT('Ctrl Pts',(2.58415199599995,11.6,11.06386871));
#221279=CARTESIAN_POINT('Ctrl Pts',(2.58343225499994,15.2,11.067438172));
#221280=CARTESIAN_POINT('Ctrl Pts',(2.58343225499994,11.6,11.067438172));
#221281=CARTESIAN_POINT('Ctrl Pts',(2.58270885099994,15.2,11.071011569));
#221282=CARTESIAN_POINT('Ctrl Pts',(2.58270885099994,11.6,11.071011569));
#221283=CARTESIAN_POINT('Ctrl Pts',(2.58198177999994,15.2,11.074588894));
#221284=CARTESIAN_POINT('Ctrl Pts',(2.58198177999994,11.6,11.074588894));
#221285=CARTESIAN_POINT('Ctrl Pts',(2.58125103799994,15.2,11.078170138));
#221286=CARTESIAN_POINT('Ctrl Pts',(2.58125103799994,11.6,11.078170138));
#221287=CARTESIAN_POINT('Ctrl Pts',(2.58051662099994,15.2,11.081755293));
#221288=CARTESIAN_POINT('Ctrl Pts',(2.58051662099994,11.6,11.081755293));
#221289=CARTESIAN_POINT('Ctrl Pts',(2.57977852499994,15.2,11.085344351));
#221290=CARTESIAN_POINT('Ctrl Pts',(2.57977852499994,11.6,11.085344351));
#221291=CARTESIAN_POINT('Ctrl Pts',(2.57903674499994,15.2,11.088937303));
#221292=CARTESIAN_POINT('Ctrl Pts',(2.57903674499994,11.6,11.088937303));
#221293=CARTESIAN_POINT('Ctrl Pts',(2.57829127799994,15.2,11.092534141));
#221294=CARTESIAN_POINT('Ctrl Pts',(2.57829127799994,11.6,11.092534141));
#221295=CARTESIAN_POINT('Ctrl Pts',(2.57754211899994,15.2,11.096134856));
#221296=CARTESIAN_POINT('Ctrl Pts',(2.57754211899994,11.6,11.096134856));
#221297=CARTESIAN_POINT('Ctrl Pts',(2.57678926299994,15.2,11.09973944));
#221298=CARTESIAN_POINT('Ctrl Pts',(2.57678926299994,11.6,11.09973944));
#221299=CARTESIAN_POINT('Ctrl Pts',(2.57603270799994,15.2,11.103347886));
#221300=CARTESIAN_POINT('Ctrl Pts',(2.57603270799994,11.6,11.103347886));
#221301=CARTESIAN_POINT('Ctrl Pts',(2.57527244699994,15.2,11.106960183));
#221302=CARTESIAN_POINT('Ctrl Pts',(2.57527244699994,11.6,11.106960183));
#221303=CARTESIAN_POINT('Ctrl Pts',(2.57450847899994,15.2,11.110576325));
#221304=CARTESIAN_POINT('Ctrl Pts',(2.57450847899994,11.6,11.110576325));
#221305=CARTESIAN_POINT('Ctrl Pts',(2.57374079699995,15.2,11.114196302));
#221306=CARTESIAN_POINT('Ctrl Pts',(2.57374079699995,11.6,11.114196302));
#221307=CARTESIAN_POINT('Ctrl Pts',(2.57296939999994,15.2,11.117820108));
#221308=CARTESIAN_POINT('Ctrl Pts',(2.57296939999994,11.6,11.117820108));
#221309=CARTESIAN_POINT('Ctrl Pts',(2.57219427999994,15.2,11.121447733));
#221310=CARTESIAN_POINT('Ctrl Pts',(2.57219427999994,11.6,11.121447733));
#221311=CARTESIAN_POINT('Ctrl Pts',(2.57141543699994,15.2,11.125079169));
#221312=CARTESIAN_POINT('Ctrl Pts',(2.57141543699994,11.6,11.125079169));
#221313=CARTESIAN_POINT('Ctrl Pts',(2.57063286499994,15.2,11.128714409));
#221314=CARTESIAN_POINT('Ctrl Pts',(2.57063286499994,11.6,11.128714409));
#221315=CARTESIAN_POINT('Ctrl Pts',(2.56984655899994,15.2,11.132353445));
#221316=CARTESIAN_POINT('Ctrl Pts',(2.56984655899994,11.6,11.132353445));
#221317=CARTESIAN_POINT('Ctrl Pts',(2.56905651699994,15.2,11.135996265));
#221318=CARTESIAN_POINT('Ctrl Pts',(2.56905651699994,11.6,11.135996265));
#221319=CARTESIAN_POINT('Ctrl Pts',(2.56826273399994,15.2,11.139642864));
#221320=CARTESIAN_POINT('Ctrl Pts',(2.56826273399994,11.6,11.139642864));
#221321=CARTESIAN_POINT('Ctrl Pts',(2.56746520399994,15.2,11.143293232));
#221322=CARTESIAN_POINT('Ctrl Pts',(2.56746520399994,11.6,11.143293232));
#221323=CARTESIAN_POINT('Ctrl Pts',(2.56666392499994,15.2,11.146947362));
#221324=CARTESIAN_POINT('Ctrl Pts',(2.56666392499994,11.6,11.146947362));
#221325=CARTESIAN_POINT('Ctrl Pts',(2.56585889299994,15.2,11.150605243));
#221326=CARTESIAN_POINT('Ctrl Pts',(2.56585889299994,11.6,11.150605243));
#221327=CARTESIAN_POINT('Ctrl Pts',(2.56505010399994,15.2,11.15426687));
#221328=CARTESIAN_POINT('Ctrl Pts',(2.56505010399994,11.6,11.15426687));
#221329=CARTESIAN_POINT('Ctrl Pts',(2.56423755299994,15.2,11.157932235));
#221330=CARTESIAN_POINT('Ctrl Pts',(2.56423755299994,11.6,11.157932235));
#221331=CARTESIAN_POINT('Ctrl Pts',(2.56342123799994,15.2,11.161601329));
#221332=CARTESIAN_POINT('Ctrl Pts',(2.56342123799994,11.6,11.161601329));
#221333=CARTESIAN_POINT('Ctrl Pts',(2.56260115599994,15.2,11.165274147));
#221334=CARTESIAN_POINT('Ctrl Pts',(2.56260115599994,11.6,11.165274147));
#221335=CARTESIAN_POINT('Ctrl Pts',(2.56177730199994,15.2,11.168950679));
#221336=CARTESIAN_POINT('Ctrl Pts',(2.56177730199994,11.6,11.168950679));
#221337=CARTESIAN_POINT('Ctrl Pts',(2.56094967199994,15.2,11.172630919));
#221338=CARTESIAN_POINT('Ctrl Pts',(2.56094967199994,11.6,11.172630919));
#221339=CARTESIAN_POINT('Ctrl Pts',(2.56011826199994,15.2,11.176314857));
#221340=CARTESIAN_POINT('Ctrl Pts',(2.56011826199994,11.6,11.176314857));
#221341=CARTESIAN_POINT('Ctrl Pts',(2.55928306599994,15.2,11.18000248));
#221342=CARTESIAN_POINT('Ctrl Pts',(2.55928306599994,11.6,11.18000248));
#221343=CARTESIAN_POINT('Ctrl Pts',(2.55844408099994,15.2,11.183693782));
#221344=CARTESIAN_POINT('Ctrl Pts',(2.55844408099994,11.6,11.183693782));
#221345=CARTESIAN_POINT('Ctrl Pts',(2.55760130099994,15.2,11.18738875));
#221346=CARTESIAN_POINT('Ctrl Pts',(2.55760130099994,11.6,11.18738875));
#221347=CARTESIAN_POINT('Ctrl Pts',(2.55675472199994,15.2,11.191087377));
#221348=CARTESIAN_POINT('Ctrl Pts',(2.55675472199994,11.6,11.191087377));
#221349=CARTESIAN_POINT('Ctrl Pts',(2.55590434099994,15.2,11.194789655));
#221350=CARTESIAN_POINT('Ctrl Pts',(2.55590434099994,11.6,11.194789655));
#221351=CARTESIAN_POINT('Ctrl Pts',(2.55505015499994,15.2,11.19849558));
#221352=CARTESIAN_POINT('Ctrl Pts',(2.55505015499994,11.6,11.19849558));
#221353=CARTESIAN_POINT('Ctrl Pts',(2.55419216299994,15.2,11.202205147));
#221354=CARTESIAN_POINT('Ctrl Pts',(2.55419216299994,11.6,11.202205147));
#221355=CARTESIAN_POINT('Ctrl Pts',(2.55333036399994,15.2,11.205918353));
#221356=CARTESIAN_POINT('Ctrl Pts',(2.55333036399994,11.6,11.205918353));
#221357=CARTESIAN_POINT('Ctrl Pts',(2.55263787799994,15.2,11.20889183));
#221358=CARTESIAN_POINT('Ctrl Pts',(2.55263787799994,11.6,11.20889183));
#221359=CARTESIAN_POINT('Ctrl Pts',(2.55211680099994,15.2,11.211123574));
#221360=CARTESIAN_POINT('Ctrl Pts',(2.55211680099994,11.6,11.211123574));
#221361=CARTESIAN_POINT('Ctrl Pts',(2.55176865299994,15.2,11.212612132));
#221362=CARTESIAN_POINT('Ctrl Pts',(2.55176865299994,11.6,11.212612132));
#221363=CARTESIAN_POINT('Ctrl Pts',(2.55159438999994,15.2,11.213356593));
#221364=CARTESIAN_POINT('Ctrl Pts',(2.55159438999994,11.6,11.213356593));
#221365=CARTESIAN_POINT('Ctrl Pts',(2.64164356399994,15.2,10.033062558));
#221366=CARTESIAN_POINT('Ctrl Pts',(2.64194831228518,15.2,10.0348230378133));
#221367=CARTESIAN_POINT('Ctrl Pts',(2.64225752130084,15.2,10.0366407499629));
#221368=CARTESIAN_POINT('Ctrl Pts',(2.64257038295734,15.2,10.0385148623113));
#221369=CARTESIAN_POINT('Ctrl Pts',(2.6428847533909,15.2,10.0403980125768));
#221370=CARTESIAN_POINT('Ctrl Pts',(2.64320281580563,15.2,10.0423381044564));
#221371=CARTESIAN_POINT('Ctrl Pts',(2.643523781256,15.2,10.0443343067515));
#221372=CARTESIAN_POINT('Ctrl Pts',(2.6438447466772,15.2,10.0463305088653));
#221373=CARTESIAN_POINT('Ctrl Pts',(2.64416861599511,15.2,10.0483828189931));
#221374=CARTESIAN_POINT('Ctrl Pts',(2.64449462848328,15.2,10.0504904282499));
#221375=CARTESIAN_POINT('Ctrl Pts',(2.64482064097144,15.2,10.0525980375067));
#221376=CARTESIAN_POINT('Ctrl Pts',(2.64514879426365,15.2,10.0547609455835));
#221377=CARTESIAN_POINT('Ctrl Pts',(2.64547835293473,15.2,10.0569783630272));
#221378=CARTESIAN_POINT('Ctrl Pts',(2.64580791163574,15.2,10.0591957806723));
#221379=CARTESIAN_POINT('Ctrl Pts',(2.6461388765513,15.2,10.0614677065646));
#221380=CARTESIAN_POINT('Ctrl Pts',(2.64647052756943,15.2,10.0637933712784));
#221381=CARTESIAN_POINT('Ctrl Pts',(2.64680217855742,15.2,10.0661190357809));
#221382=CARTESIAN_POINT('Ctrl Pts',(2.64713452030233,15.2,10.0684984401115));
#221383=CARTESIAN_POINT('Ctrl Pts',(2.64746685620843,15.2,10.0709308325343));
#221384=CARTESIAN_POINT('Ctrl Pts',(2.64779919211453,15.2,10.0733632249571));
#221385=CARTESIAN_POINT('Ctrl Pts',(2.64813152497723,15.2,10.0758486039396));
#221386=CARTESIAN_POINT('Ctrl Pts',(2.6484631779652,15.2,10.0783862403452));
#221387=CARTESIAN_POINT('Ctrl Pts',(2.6487948309833,15.2,10.0809238769812));
#221388=CARTESIAN_POINT('Ctrl Pts',(2.64912580691801,15.2,10.0835137669737));
#221389=CARTESIAN_POINT('Ctrl Pts',(2.64945545276921,15.2,10.0861551977878));
#221390=CARTESIAN_POINT('Ctrl Pts',(2.64978509859048,15.2,10.088796628362));
#221391=CARTESIAN_POINT('Ctrl Pts',(2.65011341197134,15.2,10.0914895979888));
#221392=CARTESIAN_POINT('Ctrl Pts',(2.65043976104272,15.2,10.0942334086413));
#221393=CARTESIAN_POINT('Ctrl Pts',(2.65076611011411,15.2,10.0969772192938));
#221394=CARTESIAN_POINT('Ctrl Pts',(2.65109049311065,15.2,10.0997718698089));
#221395=CARTESIAN_POINT('Ctrl Pts',(2.65141229526573,15.2,10.1026166776201));
#221396=CARTESIAN_POINT('Ctrl Pts',(2.65173409742082,15.2,10.1054614854312));
#221397=CARTESIAN_POINT('Ctrl Pts',(2.65205331709344,15.2,10.108356448356));
#221398=CARTESIAN_POINT('Ctrl Pts',(2.65236935724883,15.2,10.1113009019123));
#221399=CARTESIAN_POINT('Ctrl Pts',(2.65268539743294,15.2,10.1142453557361));
#221400=CARTESIAN_POINT('Ctrl Pts',(2.65299825586676,15.2,10.1172392954563));
#221401=CARTESIAN_POINT('Ctrl Pts',(2.65330735305012,15.2,10.1202820707076));
#221402=CARTESIAN_POINT('Ctrl Pts',(2.65366796638857,15.2,10.1238319747529));
#221403=CARTESIAN_POINT('Ctrl Pts',(2.65402345683872,15.2,10.1274483456391));
#221404=CARTESIAN_POINT('Ctrl Pts',(2.65437292773397,15.2,10.1311301704059));
#221405=CARTESIAN_POINT('Ctrl Pts',(2.65472239865642,15.2,10.1348119954594));
#221406=CARTESIAN_POINT('Ctrl Pts',(2.65506585037871,15.2,10.1385592719262));
#221407=CARTESIAN_POINT('Ctrl Pts',(2.65540241446754,15.2,10.1423710100804));
#221408=CARTESIAN_POINT('Ctrl Pts',(2.65569089798348,15.2,10.1456382143397));
#221409=CARTESIAN_POINT('Ctrl Pts',(2.65597432136547,15.2,10.1489527781383));
#221410=CARTESIAN_POINT('Ctrl Pts',(2.6562521530469,15.2,10.1523140905746));
#221411=CARTESIAN_POINT('Ctrl Pts',(2.6565299847031,15.2,10.1556754027057));
#221412=CARTESIAN_POINT('Ctrl Pts',(2.65680222509103,15.2,10.1590834656702));
#221413=CARTESIAN_POINT('Ctrl Pts',(2.65706835574777,15.2,10.1625376759633));
#221414=CARTESIAN_POINT('Ctrl Pts',(2.6573344864045,15.2,10.1659918862565));
#221415=CARTESIAN_POINT('Ctrl Pts',(2.65759450897003,15.2,10.1694922499377));
#221416=CARTESIAN_POINT('Ctrl Pts',(2.65784791771112,15.2,10.1730381733068));
#221417=CARTESIAN_POINT('Ctrl Pts',(2.6581013264522,15.2,10.176584096676));
#221418=CARTESIAN_POINT('Ctrl Pts',(2.65834812371539,15.2,10.1801755849054));
#221419=CARTESIAN_POINT('Ctrl Pts',(2.65858781554049,15.2,10.1838120581035));
#221420=CARTESIAN_POINT('Ctrl Pts',(2.65886745601764,15.2,10.1880546103882));
#221421=CARTESIAN_POINT('Ctrl Pts',(2.65913742923337,15.2,10.1923583939805));
#221422=CARTESIAN_POINT('Ctrl Pts',(2.6593969717378,15.2,10.1967225107962));
#221423=CARTESIAN_POINT('Ctrl Pts',(2.65961943673005,15.2,10.2004631821584));
#221424=CARTESIAN_POINT('Ctrl Pts',(2.65983424360939,15.2,10.2042481817746));
#221425=CARTESIAN_POINT('Ctrl Pts',(2.66004092268576,15.2,10.2080769531326));
#221426=CARTESIAN_POINT('Ctrl Pts',(2.66024760178091,15.2,10.2119057248383));
#221427=CARTESIAN_POINT('Ctrl Pts',(2.66044615646696,15.2,10.2157782705315));
#221428=CARTESIAN_POINT('Ctrl Pts',(2.66063613331028,15.2,10.2196940442468));
#221429=CARTESIAN_POINT('Ctrl Pts',(2.66085777293492,15.2,10.2242624463811));
#221430=CARTESIAN_POINT('Ctrl Pts',(2.66106773549864,15.2,10.2288896875629));
#221431=CARTESIAN_POINT('Ctrl Pts',(2.66126532322316,15.2,10.2335749195872));
#221432=CARTESIAN_POINT('Ctrl Pts',(2.6614064573209,15.2,10.2369215140987));
#221433=CARTESIAN_POINT('Ctrl Pts',(2.66154127587154,15.2,10.2402976954625));
#221434=CARTESIAN_POINT('Ctrl Pts',(2.66166953323318,15.2,10.2437031601128));
#221435=CARTESIAN_POINT('Ctrl Pts',(2.66182344207555,15.2,10.247789717916));
#221436=CARTESIAN_POINT('Ctrl Pts',(2.66196789944114,15.2,10.2519184437987));
#221437=CARTESIAN_POINT('Ctrl Pts',(2.66210248553796,15.2,10.2560888199035));
#221438=CARTESIAN_POINT('Ctrl Pts',(2.66221464061253,15.2,10.2595641331347));
#221439=CARTESIAN_POINT('Ctrl Pts',(2.66231994071894,15.2,10.2630683710375));
#221440=CARTESIAN_POINT('Ctrl Pts',(2.66241814828781,15.2,10.2666012374287));
#221441=CARTESIAN_POINT('Ctrl Pts',(2.66251635585667,15.2,10.2701341038199));
#221442=CARTESIAN_POINT('Ctrl Pts',(2.66260747005041,15.2,10.2736955992783));
#221443=CARTESIAN_POINT('Ctrl Pts',(2.66269125928592,15.2,10.2772854331695));
#221444=CARTESIAN_POINT('Ctrl Pts',(2.6627750485123,15.2,10.2808752666694));
#221445=CARTESIAN_POINT('Ctrl Pts',(2.66285151010895,15.2,10.2844934378839));
#221446=CARTESIAN_POINT('Ctrl Pts',(2.66292041774095,15.2,10.2881396605397));
#221447=CARTESIAN_POINT('Ctrl Pts',(2.66298932538046,15.2,10.2917858835929));
#221448=CARTESIAN_POINT('Ctrl Pts',(2.66305067884788,15.2,10.2954601580569));
#221449=CARTESIAN_POINT('Ctrl Pts',(2.66310425245962,15.2,10.299162198749));
#221450=CARTESIAN_POINT('Ctrl Pts',(2.66315782607137,15.2,10.3028642394412));
#221451=CARTESIAN_POINT('Ctrl Pts',(2.6632036207431,15.2,10.306594048467));
#221452=CARTESIAN_POINT('Ctrl Pts',(2.66324141678721,15.2,10.3103513458055));
#221453=CARTESIAN_POINT('Ctrl Pts',(2.66328677204262,15.2,10.3148601028575));
#221454=CARTESIAN_POINT('Ctrl Pts',(2.6633206093103,15.2,10.3194084393473));
#221455=CARTESIAN_POINT('Ctrl Pts',(2.66334255472735,15.2,10.3239958814333));
#221456=CARTESIAN_POINT('Ctrl Pts',(2.6633608425739,15.2,10.32781874963));
#221457=CARTESIAN_POINT('Ctrl Pts',(2.66337087430086,15.2,10.3316687752493));
#221458=CARTESIAN_POINT('Ctrl Pts',(2.66337243721683,15.2,10.3355456835154));
#221459=CARTESIAN_POINT('Ctrl Pts',(2.66337400013264,15.2,10.3394225913589));
#221460=CARTESIAN_POINT('Ctrl Pts',(2.66336709569959,15.2,10.3433263851719));
#221461=CARTESIAN_POINT('Ctrl Pts',(2.66335151674367,15.2,10.3472567914775));
#221462=CARTESIAN_POINT('Ctrl Pts',(2.66333593778604,15.2,10.3511871982115));
#221463=CARTESIAN_POINT('Ctrl Pts',(2.66331168425913,15.2,10.3551442209366));
#221464=CARTESIAN_POINT('Ctrl Pts',(2.6632785537043,15.2,10.3591275924622));
#221465=CARTESIAN_POINT('Ctrl Pts',(2.66323879703633,15.2,10.3639076385535));
#221466=CARTESIAN_POINT('Ctrl Pts',(2.66318625590048,15.2,10.3687256263734));
#221467=CARTESIAN_POINT('Ctrl Pts',(2.66312058922967,15.2,10.373581102723));
#221468=CARTESIAN_POINT('Ctrl Pts',(2.66305492256482,15.2,10.3784365786316));
#221469=CARTESIAN_POINT('Ctrl Pts',(2.66297612703871,15.2,10.3833295449462));
#221470=CARTESIAN_POINT('Ctrl Pts',(2.66288387145834,15.2,10.388259551706));
#221471=CARTESIAN_POINT('Ctrl Pts',(2.66279161587797,15.2,10.3931895584659));
#221472=CARTESIAN_POINT('Ctrl Pts',(2.66268589722438,15.2,10.3981566070889));
#221473=CARTESIAN_POINT('Ctrl Pts',(2.66256638872966,15.2,10.4031602549045));
#221474=CARTESIAN_POINT('Ctrl Pts',(2.66248671639261,15.2,10.406496020418));
#221475=CARTESIAN_POINT('Ctrl Pts',(2.66240091517758,15.2,10.4098480544589));
#221476=CARTESIAN_POINT('Ctrl Pts',(2.6623088889499,15.2,10.4132162247689));
#221477=CARTESIAN_POINT('Ctrl Pts',(2.66214784305774,15.2,10.4191105225819));
#221478=CARTESIAN_POINT('Ctrl Pts',(2.66196773798001,15.2,10.4250542421692));
#221479=CARTESIAN_POINT('Ctrl Pts',(2.66176806598964,15.2,10.4310466983348));
#221480=CARTESIAN_POINT('Ctrl Pts',(2.66159691857822,15.2,10.4361830890673));
#221481=CARTESIAN_POINT('Ctrl Pts',(2.66141139836021,15.2,10.4413552861094));
#221482=CARTESIAN_POINT('Ctrl Pts',(2.66121119703321,15.2,10.4465628640273));
#221483=CARTESIAN_POINT('Ctrl Pts',(2.66101099570621,15.2,10.4517704419452));
#221484=CARTESIAN_POINT('Ctrl Pts',(2.6607961129201,15.2,10.4570134019889));
#221485=CARTESIAN_POINT('Ctrl Pts',(2.66056624676244,15.2,10.4622913237957));
#221486=CARTESIAN_POINT('Ctrl Pts',(2.66037469162409,15.2,10.4666895921279));
#221487=CARTESIAN_POINT('Ctrl Pts',(2.66017273257437,15.2,10.4711121390049));
#221488=CARTESIAN_POINT('Ctrl Pts',(2.65996019729714,15.2,10.4755587249759));
#221489=CARTESIAN_POINT('Ctrl Pts',(2.6597901690661,15.2,10.4791159939466));
#221490=CARTESIAN_POINT('Ctrl Pts',(2.65961337264584,15.2,10.4826886483612));
#221491=CARTESIAN_POINT('Ctrl Pts',(2.65942972168162,15.2,10.4862765660707));
#221492=CARTESIAN_POINT('Ctrl Pts',(2.65920015798885,15.2,10.490761462963));
#221493=CARTESIAN_POINT('Ctrl Pts',(2.65895988345134,15.2,10.4952702080909));
#221494=CARTESIAN_POINT('Ctrl Pts',(2.65870873324212,15.2,10.4998025658011));
#221495=CARTESIAN_POINT('Ctrl Pts',(2.65850781309116,15.2,10.5034284516729));
#221496=CARTESIAN_POINT('Ctrl Pts',(2.658299932405,15.2,10.5070694505177));
#221497=CARTESIAN_POINT('Ctrl Pts',(2.65808500753414,15.2,10.5107254422179));
#221498=CARTESIAN_POINT('Ctrl Pts',(2.65787008263399,15.2,10.5143814344162));
#221499=CARTESIAN_POINT('Ctrl Pts',(2.65764811326068,15.2,10.518052418918));
#221500=CARTESIAN_POINT('Ctrl Pts',(2.65741901895836,15.2,10.5217382780265));
#221501=CARTESIAN_POINT('Ctrl Pts',(2.65713265109606,15.2,10.5263456016611));
#221502=CARTESIAN_POINT('Ctrl Pts',(2.6568351471105,15.2,10.5309761659123));
#221503=CARTESIAN_POINT('Ctrl Pts',(2.65652635023458,15.2,10.5356297403586));
#221504=CARTESIAN_POINT('Ctrl Pts',(2.65627931275404,15.2,10.5393525996113));
#221505=CARTESIAN_POINT('Ctrl Pts',(2.65602504882998,15.2,10.543090187476));
#221506=CARTESIAN_POINT('Ctrl Pts',(2.65576347679629,15.2,10.5468423846683));
#221507=CARTESIAN_POINT('Ctrl Pts',(2.65550190472695,15.2,10.5505945823719));
#221508=CARTESIAN_POINT('Ctrl Pts',(2.6552330259449,15.2,10.5543613914746));
#221509=CARTESIAN_POINT('Ctrl Pts',(2.65495676169318,15.2,10.5581426953154));
#221510=CARTESIAN_POINT('Ctrl Pts',(2.65468049747909,15.2,10.5619239986409));
#221511=CARTESIAN_POINT('Ctrl Pts',(2.65439684769386,15.2,10.5657197956204));
#221512=CARTESIAN_POINT('Ctrl Pts',(2.6541057342737,15.2,10.5695299733636));
#221513=CARTESIAN_POINT('Ctrl Pts',(2.65374184246875,15.2,10.5742926959319));
#221514=CARTESIAN_POINT('Ctrl Pts',(2.65336628922462,15.2,10.5790778877979));
#221515=CARTESIAN_POINT('Ctrl Pts',(2.6529789265169,15.2,10.5838853254357));
#221516=CARTESIAN_POINT('Ctrl Pts',(2.65266903633384,15.2,10.5877312757555));
#221517=CARTESIAN_POINT('Ctrl Pts',(2.6523515868096,15.2,10.5915914632257));
#221518=CARTESIAN_POINT('Ctrl Pts',(2.65202650521943,15.2,10.5954657770205));
#221519=CARTESIAN_POINT('Ctrl Pts',(2.65162015325385,15.2,10.6003086690001));
#221520=CARTESIAN_POINT('Ctrl Pts',(2.65120187296133,15.2,10.6051736287818));
#221521=CARTESIAN_POINT('Ctrl Pts',(2.65077152046035,15.2,10.6100604414225));
#221522=CARTESIAN_POINT('Ctrl Pts',(2.6504272384877,15.2,10.6139698912154));
#221523=CARTESIAN_POINT('Ctrl Pts',(2.65007523109384,15.2,10.6178933252482));
#221524=CARTESIAN_POINT('Ctrl Pts',(2.64971542501265,15.2,10.6218306332032));
#221525=CARTESIAN_POINT('Ctrl Pts',(2.64935561888244,15.2,10.6257679416947));
#221526=CARTESIAN_POINT('Ctrl Pts',(2.64898801433535,15.2,10.6297191243156));
#221527=CARTESIAN_POINT('Ctrl Pts',(2.64861253896211,15.2,10.633684070842));
#221528=CARTESIAN_POINT('Ctrl Pts',(2.64823706364004,15.2,10.6376490168282));
#221529=CARTESIAN_POINT('Ctrl Pts',(2.64785371767437,15.2,10.6416277260649));
#221530=CARTESIAN_POINT('Ctrl Pts',(2.64746243154022,15.2,10.645620088682));
#221531=CARTESIAN_POINT('Ctrl Pts',(2.64707114535275,15.2,10.6496124518431));
#221532=CARTESIAN_POINT('Ctrl Pts',(2.64667191698377,15.2,10.6536184700392));
#221533=CARTESIAN_POINT('Ctrl Pts',(2.64626467818327,15.2,10.657638032537));
#221534=CARTESIAN_POINT('Ctrl Pts',(2.64585743943827,15.2,10.6616575944871));
#221535=CARTESIAN_POINT('Ctrl Pts',(2.64544219046987,15.2,10.6656907023566));
#221536=CARTESIAN_POINT('Ctrl Pts',(2.64501886056085,15.2,10.66973724808));
#221537=CARTESIAN_POINT('Ctrl Pts',(2.64448969813133,15.2,10.6747954306477));
#221538=CARTESIAN_POINT('Ctrl Pts',(2.64394791169668,15.2,10.6798746070213));
#221539=CARTESIAN_POINT('Ctrl Pts',(2.64339336757264,15.2,10.6849745716497));
#221540=CARTESIAN_POINT('Ctrl Pts',(2.64294973224923,15.2,10.6890545435747));
#221541=CARTESIAN_POINT('Ctrl Pts',(2.64249793301568,15.2,10.6931478192444));
#221542=CARTESIAN_POINT('Ctrl Pts',(2.64203790221229,15.2,10.6972542911358));
#221543=CARTESIAN_POINT('Ctrl Pts',(2.64157787147158,15.2,10.7013607624676));
#221544=CARTESIAN_POINT('Ctrl Pts',(2.6411096091603,15.2,10.7054804315912));
#221545=CARTESIAN_POINT('Ctrl Pts',(2.64063304931123,15.2,10.7096131921409));
#221546=CARTESIAN_POINT('Ctrl Pts',(2.63979906949417,15.2,10.7168455238067));
#221547=CARTESIAN_POINT('Ctrl Pts',(2.63893968046807,15.2,10.7241179469112));
#221548=CARTESIAN_POINT('Ctrl Pts',(2.63805453395032,15.2,10.7314299024471));
#221549=CARTESIAN_POINT('Ctrl Pts',(2.63716938743256,15.2,10.738741857983));
#221550=CARTESIAN_POINT('Ctrl Pts',(2.63625848327169,15.2,10.7460933444843));
#221551=CARTESIAN_POINT('Ctrl Pts',(2.63532148542279,15.2,10.753483808587));
#221552=CARTESIAN_POINT('Ctrl Pts',(2.63438448764684,15.2,10.7608742721142));
#221553=CARTESIAN_POINT('Ctrl Pts',(2.63342139251814,15.2,10.7683037132141));
#221554=CARTESIAN_POINT('Ctrl Pts',(2.63243187365076,15.2,10.7757715838022));
#221555=CARTESIAN_POINT('Ctrl Pts',(2.63144235470634,15.2,10.7832394549718));
#221556=CARTESIAN_POINT('Ctrl Pts',(2.63042640924717,15.2,10.7907457548816));
#221557=CARTESIAN_POINT('Ctrl Pts',(2.62938371606527,15.2,10.7982899414143));
#221558=CARTESIAN_POINT('Ctrl Pts',(2.6284899790986,15.2,10.8047563866781));
#221559=CARTESIAN_POINT('Ctrl Pts',(2.62757658992477,15.2,10.8112506694695));
#221560=CARTESIAN_POINT('Ctrl Pts',(2.6266433518767,15.2,10.8177724478141));
#221561=CARTESIAN_POINT('Ctrl Pts',(2.62571011374384,15.2,10.824294226751));
#221562=CARTESIAN_POINT('Ctrl Pts',(2.62475702276745,15.2,10.8308435043405));
#221563=CARTESIAN_POINT('Ctrl Pts',(2.62378388871353,15.2,10.8374199441168));
#221564=CARTESIAN_POINT('Ctrl Pts',(2.62313513276597,15.2,10.8418042367037));
#221565=CARTESIAN_POINT('Ctrl Pts',(2.62247746642747,15.2,10.8462006016154));
#221566=CARTESIAN_POINT('Ctrl Pts',(2.62181083583833,15.2,10.8506089410853));
#221567=CARTESIAN_POINT('Ctrl Pts',(2.62131086287377,15.2,10.8539151958379));
#221568=CARTESIAN_POINT('Ctrl Pts',(2.62080584795862,15.2,10.8572281859478));
#221569=CARTESIAN_POINT('Ctrl Pts',(2.62029576460284,15.2,10.8605478695762));
#221570=CARTESIAN_POINT('Ctrl Pts',(2.6197856811544,15.2,10.8638675538078));
#221571=CARTESIAN_POINT('Ctrl Pts',(2.6192705308962,15.2,10.8671939320079));
#221572=CARTESIAN_POINT('Ctrl Pts',(2.61875029040323,15.2,10.8705269637016));
#221573=CARTESIAN_POINT('Ctrl Pts',(2.61788322304095,15.2,10.876082015717));
#221574=CARTESIAN_POINT('Ctrl Pts',(2.61700201693956,15.2,10.8816555475299));
#221575=CARTESIAN_POINT('Ctrl Pts',(2.61610656367452,15.2,10.887247370448));
#221576=CARTESIAN_POINT('Ctrl Pts',(2.61556929173501,15.2,10.890602464077));
#221577=CARTESIAN_POINT('Ctrl Pts',(2.61502689016871,15.2,10.8939641426383));
#221578=CARTESIAN_POINT('Ctrl Pts',(2.61447933816066,15.2,10.8973323653933));
#221579=CARTESIAN_POINT('Ctrl Pts',(2.6139317861526,15.2,10.9007005881484));
#221580=CARTESIAN_POINT('Ctrl Pts',(2.61337908161927,15.2,10.9040753549076));
#221581=CARTESIAN_POINT('Ctrl Pts',(2.61282120368075,15.2,10.9074566259103));
#221582=CARTESIAN_POINT('Ctrl Pts',(2.61226332574224,15.2,10.910837896913));
#221583=CARTESIAN_POINT('Ctrl Pts',(2.61170027362933,15.2,10.9142256700233));
#221584=CARTESIAN_POINT('Ctrl Pts',(2.61113202477498,15.2,10.9176199080249));
#221585=CARTESIAN_POINT('Ctrl Pts',(2.61037435956703,15.2,10.9221455591049));
#221586=CARTESIAN_POINT('Ctrl Pts',(2.60960745664132,15.2,10.9266826991946));
#221587=CARTESIAN_POINT('Ctrl Pts',(2.60883126209807,15.2,10.931231235777));
#221588=CARTESIAN_POINT('Ctrl Pts',(2.6082491162435,15.2,10.9346426379039));
#221589=CARTESIAN_POINT('Ctrl Pts',(2.60766174452729,15.2,10.9380604493318));
#221590=CARTESIAN_POINT('Ctrl Pts',(2.60706912560194,15.2,10.9414846316292));
#221591=CARTESIAN_POINT('Ctrl Pts',(2.60647650667659,15.2,10.9449088139266));
#221592=CARTESIAN_POINT('Ctrl Pts',(2.60587863994603,15.2,10.9483393659823));
#221593=CARTESIAN_POINT('Ctrl Pts',(2.60527550313415,15.2,10.951776248608));
#221594=CARTESIAN_POINT('Ctrl Pts',(2.60447132075484,15.2,10.9563587585675));
#221595=CARTESIAN_POINT('Ctrl Pts',(2.60365777196074,15.2,10.9609525230496));
#221596=CARTESIAN_POINT('Ctrl Pts',(2.60283480291787,15.2,10.9655574465054));
#221597=CARTESIAN_POINT('Ctrl Pts',(2.60221757599555,15.2,10.9690111398815));
#221598=CARTESIAN_POINT('Ctrl Pts',(2.60159505182174,15.2,10.9724711124344));
#221599=CARTESIAN_POINT('Ctrl Pts',(2.60096720835477,15.2,10.9759373222722));
#221600=CARTESIAN_POINT('Ctrl Pts',(2.60033936500187,15.2,10.9794035314804));
#221601=CARTESIAN_POINT('Ctrl Pts',(2.59970620230238,15.2,10.9828759785249));
#221602=CARTESIAN_POINT('Ctrl Pts',(2.59906769987639,15.2,10.9863546253647));
#221603=CARTESIAN_POINT('Ctrl Pts',(2.5984291974504,15.2,10.9898332722045));
#221604=CARTESIAN_POINT('Ctrl Pts',(2.59778535487268,15.2,10.9933181184235));
#221605=CARTESIAN_POINT('Ctrl Pts',(2.59713615243746,15.2,10.9968091241306));
#221606=CARTESIAN_POINT('Ctrl Pts',(2.59627054922982,15.2,11.0014637981952));
#221607=CARTESIAN_POINT('Ctrl Pts',(2.59539541407688,15.2,11.0061294249049));
#221608=CARTESIAN_POINT('Ctrl Pts',(2.59451070159463,15.2,11.0108059102437));
#221609=CARTESIAN_POINT('Ctrl Pts',(2.59362598899183,15.2,11.0154823962197));
#221610=CARTESIAN_POINT('Ctrl Pts',(2.59273169777704,15.2,11.0201697419633));
#221611=CARTESIAN_POINT('Ctrl Pts',(2.59182777994998,15.2,11.024867855275));
#221612=CARTESIAN_POINT('Ctrl Pts',(2.59114984164126,15.2,11.0283914399387));
#221613=CARTESIAN_POINT('Ctrl Pts',(2.59046648936613,15.2,11.031921081427));
#221614=CARTESIAN_POINT('Ctrl Pts',(2.58977770109997,15.2,11.0354567416313));
#221615=CARTESIAN_POINT('Ctrl Pts',(2.58885931666166,15.2,11.0401709556653));
#221616=CARTESIAN_POINT('Ctrl Pts',(2.58793127138487,15.2,11.0448958697083));
#221617=CARTESIAN_POINT('Ctrl Pts',(2.58699351739719,15.2,11.0496313932038));
#221618=CARTESIAN_POINT('Ctrl Pts',(2.58629020197032,15.2,11.0531830355029));
#221619=CARTESIAN_POINT('Ctrl Pts',(2.5855814249799,15.2,11.0567406451341));
#221620=CARTESIAN_POINT('Ctrl Pts',(2.5848671672137,15.2,11.0603041834218));
#221621=CARTESIAN_POINT('Ctrl Pts',(2.58415290944751,15.2,11.0638677217095));
#221622=CARTESIAN_POINT('Ctrl Pts',(2.58343317205698,15.2,11.0674371907798));
#221623=CARTESIAN_POINT('Ctrl Pts',(2.58270793424998,15.2,11.0710125509833));
#221624=CARTESIAN_POINT('Ctrl Pts',(2.58198269644299,15.2,11.0745879111868));
#221625=CARTESIAN_POINT('Ctrl Pts',(2.58125195816958,15.2,11.0781691626899));
#221626=CARTESIAN_POINT('Ctrl Pts',(2.58051570132181,15.2,11.0817562683507));
#221627=CARTESIAN_POINT('Ctrl Pts',(2.57977944447404,15.2,11.0853433740115));
#221628=CARTESIAN_POINT('Ctrl Pts',(2.57903766857072,15.2,11.088936333722));
#221629=CARTESIAN_POINT('Ctrl Pts',(2.57829035514452,15.2,11.0925351095621));
#221630=CARTESIAN_POINT('Ctrl Pts',(2.5772939371524,15.2,11.0973334777846));
#221631=CARTESIAN_POINT('Ctrl Pts',(2.57628767328396,15.2,11.1021421859029));
#221632=CARTESIAN_POINT('Ctrl Pts',(2.57527152011682,15.2,11.1069611446107));
#221633=CARTESIAN_POINT('Ctrl Pts',(2.57450940531068,15.2,11.1105753633132));
#221634=CARTESIAN_POINT('Ctrl Pts',(2.57374172812189,15.2,11.1141953481483));
#221635=CARTESIAN_POINT('Ctrl Pts',(2.57296846931665,15.2,11.1178210627666));
#221636=CARTESIAN_POINT('Ctrl Pts',(2.57167970459443,15.2,11.1238639206833));
#221637=CARTESIAN_POINT('Ctrl Pts',(2.57037543667752,15.2,11.1299226948923));
#221638=CARTESIAN_POINT('Ctrl Pts',(2.56905558174093,15.2,11.1359972097116));
#221639=CARTESIAN_POINT('Ctrl Pts',(2.56826366880775,15.2,11.1396419184707));
#221640=CARTESIAN_POINT('Ctrl Pts',(2.56746614255848,15.2,11.1432922950796));
#221641=CARTESIAN_POINT('Ctrl Pts',(2.56666298675071,15.2,11.1469482997966));
#221642=CARTESIAN_POINT('Ctrl Pts',(2.56585983094294,15.2,11.1506043045137));
#221643=CARTESIAN_POINT('Ctrl Pts',(2.56505104525857,15.2,11.1542659381007));
#221644=CARTESIAN_POINT('Ctrl Pts',(2.56423661208033,15.2,11.1579331668836));
#221645=CARTESIAN_POINT('Ctrl Pts',(2.56315070107737,15.2,11.162822805705));
#221646=CARTESIAN_POINT('Ctrl Pts',(2.56205475417597,15.2,11.1677223928859));
#221647=CARTESIAN_POINT('Ctrl Pts',(2.56094872689281,15.2,11.1726318438764));
#221648=CARTESIAN_POINT('Ctrl Pts',(2.56011920650578,15.2,11.1763139317848));
#221649=CARTESIAN_POINT('Ctrl Pts',(2.55928401515584,15.2,11.180001564504));
#221650=CARTESIAN_POINT('Ctrl Pts',(2.55844313226588,15.2,11.1836946985533));
#221651=CARTESIAN_POINT('Ctrl Pts',(2.55760224937592,15.2,11.1873878326026));
#221652=CARTESIAN_POINT('Ctrl Pts',(2.55675567340697,15.2,11.1910864657311));
#221653=CARTESIAN_POINT('Ctrl Pts',(2.55590338976742,15.2,11.1947905667382));
#221654=CARTESIAN_POINT('Ctrl Pts',(2.55448291698325,15.2,11.2009640686412));
#221655=CARTESIAN_POINT('Ctrl Pts',(2.55304658198318,15.2,11.2071527499809));
#221656=CARTESIAN_POINT('Ctrl Pts',(2.55159438999994,15.2,11.213356593));
#221657=CARTESIAN_POINT('Ctrl Pts',(2.64164356399994,12.2,10.033062558));
#221658=CARTESIAN_POINT('Ctrl Pts',(2.64194831228518,12.2,10.0348230378133));
#221659=CARTESIAN_POINT('Ctrl Pts',(2.64225752130084,12.2,10.0366407499629));
#221660=CARTESIAN_POINT('Ctrl Pts',(2.64257038295734,12.2,10.0385148623113));
#221661=CARTESIAN_POINT('Ctrl Pts',(2.6428847533909,12.2,10.0403980125768));
#221662=CARTESIAN_POINT('Ctrl Pts',(2.64320281580563,12.2,10.0423381044564));
#221663=CARTESIAN_POINT('Ctrl Pts',(2.643523781256,12.2,10.0443343067515));
#221664=CARTESIAN_POINT('Ctrl Pts',(2.6438447466772,12.2,10.0463305088653));
#221665=CARTESIAN_POINT('Ctrl Pts',(2.64416861599511,12.2,10.0483828189931));
#221666=CARTESIAN_POINT('Ctrl Pts',(2.64449462848328,12.2,10.0504904282499));
#221667=CARTESIAN_POINT('Ctrl Pts',(2.64482064097144,12.2,10.0525980375067));
#221668=CARTESIAN_POINT('Ctrl Pts',(2.64514879426365,12.2,10.0547609455835));
#221669=CARTESIAN_POINT('Ctrl Pts',(2.64547835293473,12.2,10.0569783630272));
#221670=CARTESIAN_POINT('Ctrl Pts',(2.64580791163574,12.2,10.0591957806723));
#221671=CARTESIAN_POINT('Ctrl Pts',(2.6461388765513,12.2,10.0614677065646));
#221672=CARTESIAN_POINT('Ctrl Pts',(2.64647052756943,12.2,10.0637933712784));
#221673=CARTESIAN_POINT('Ctrl Pts',(2.64680217855742,12.2,10.0661190357809));
#221674=CARTESIAN_POINT('Ctrl Pts',(2.64713452030233,12.2,10.0684984401115));
#221675=CARTESIAN_POINT('Ctrl Pts',(2.64746685620843,12.2,10.0709308325343));
#221676=CARTESIAN_POINT('Ctrl Pts',(2.64779919211453,12.2,10.0733632249571));
#221677=CARTESIAN_POINT('Ctrl Pts',(2.64813152497723,12.2,10.0758486039396));
#221678=CARTESIAN_POINT('Ctrl Pts',(2.6484631779652,12.2,10.0783862403452));
#221679=CARTESIAN_POINT('Ctrl Pts',(2.6487948309833,12.2,10.0809238769812));
#221680=CARTESIAN_POINT('Ctrl Pts',(2.64912580691801,12.2,10.0835137669737));
#221681=CARTESIAN_POINT('Ctrl Pts',(2.64945545276921,12.2,10.0861551977878));
#221682=CARTESIAN_POINT('Ctrl Pts',(2.64978509859048,12.2,10.088796628362));
#221683=CARTESIAN_POINT('Ctrl Pts',(2.65011341197134,12.2,10.0914895979888));
#221684=CARTESIAN_POINT('Ctrl Pts',(2.65043976104272,12.2,10.0942334086413));
#221685=CARTESIAN_POINT('Ctrl Pts',(2.65076611011411,12.2,10.0969772192938));
#221686=CARTESIAN_POINT('Ctrl Pts',(2.65109049311065,12.2,10.0997718698089));
#221687=CARTESIAN_POINT('Ctrl Pts',(2.65141229526573,12.2,10.1026166776201));
#221688=CARTESIAN_POINT('Ctrl Pts',(2.65173409742082,12.2,10.1054614854312));
#221689=CARTESIAN_POINT('Ctrl Pts',(2.65205331709344,12.2,10.108356448356));
#221690=CARTESIAN_POINT('Ctrl Pts',(2.65236935724883,12.2,10.1113009019123));
#221691=CARTESIAN_POINT('Ctrl Pts',(2.65268539743294,12.2,10.1142453557361));
#221692=CARTESIAN_POINT('Ctrl Pts',(2.65299825586676,12.2,10.1172392954563));
#221693=CARTESIAN_POINT('Ctrl Pts',(2.65330735305012,12.2,10.1202820707076));
#221694=CARTESIAN_POINT('Ctrl Pts',(2.65366796638857,12.2,10.1238319747529));
#221695=CARTESIAN_POINT('Ctrl Pts',(2.65402345683872,12.2,10.1274483456391));
#221696=CARTESIAN_POINT('Ctrl Pts',(2.65437292773397,12.2,10.1311301704059));
#221697=CARTESIAN_POINT('Ctrl Pts',(2.65472239865642,12.2,10.1348119954594));
#221698=CARTESIAN_POINT('Ctrl Pts',(2.65506585037871,12.2,10.1385592719262));
#221699=CARTESIAN_POINT('Ctrl Pts',(2.65540241446754,12.2,10.1423710100804));
#221700=CARTESIAN_POINT('Ctrl Pts',(2.65569089798348,12.2,10.1456382143397));
#221701=CARTESIAN_POINT('Ctrl Pts',(2.65597432136547,12.2,10.1489527781383));
#221702=CARTESIAN_POINT('Ctrl Pts',(2.6562521530469,12.2,10.1523140905746));
#221703=CARTESIAN_POINT('Ctrl Pts',(2.65652998470309,12.2,10.1556754027057));
#221704=CARTESIAN_POINT('Ctrl Pts',(2.65680222509103,12.2,10.1590834656702));
#221705=CARTESIAN_POINT('Ctrl Pts',(2.65706835574777,12.2,10.1625376759633));
#221706=CARTESIAN_POINT('Ctrl Pts',(2.6573344864045,12.2,10.1659918862565));
#221707=CARTESIAN_POINT('Ctrl Pts',(2.65759450897003,12.2,10.1694922499377));
#221708=CARTESIAN_POINT('Ctrl Pts',(2.65784791771112,12.2,10.1730381733068));
#221709=CARTESIAN_POINT('Ctrl Pts',(2.6581013264522,12.2,10.176584096676));
#221710=CARTESIAN_POINT('Ctrl Pts',(2.65834812371539,12.2,10.1801755849054));
#221711=CARTESIAN_POINT('Ctrl Pts',(2.6585878155405,12.2,10.1838120581035));
#221712=CARTESIAN_POINT('Ctrl Pts',(2.65882750738738,12.2,10.187448531632));
#221713=CARTESIAN_POINT('Ctrl Pts',(2.65906009611692,12.2,10.1911299913398));
#221714=CARTESIAN_POINT('Ctrl Pts',(2.65928510279552,12.2,10.1948558719615));
#221715=CARTESIAN_POINT('Ctrl Pts',(2.65951010945368,12.2,10.1985817522447));
#221716=CARTESIAN_POINT('Ctrl Pts',(2.65972753223983,12.2,10.2023520526612));
#221717=CARTESIAN_POINT('Ctrl Pts',(2.65993690806653,12.2,10.2061662179565));
#221718=CARTESIAN_POINT('Ctrl Pts',(2.66014628389323,12.2,10.2099803832518));
#221719=CARTESIAN_POINT('Ctrl Pts',(2.66034760926037,12.2,10.213838413436));
#221720=CARTESIAN_POINT('Ctrl Pts',(2.66054043217061,12.2,10.2177397617913));
#221721=CARTESIAN_POINT('Ctrl Pts',(2.66073325509836,12.2,10.221641110501));
#221722=CARTESIAN_POINT('Ctrl Pts',(2.66091757639077,12.2,10.2255857789084));
#221723=CARTESIAN_POINT('Ctrl Pts',(2.6610929484919,12.2,10.2295732289107));
#221724=CARTESIAN_POINT('Ctrl Pts',(2.66123909190155,12.2,10.2328961037316));
#221725=CARTESIAN_POINT('Ctrl Pts',(2.66137902430683,12.2,10.2362486888288));
#221726=CARTESIAN_POINT('Ctrl Pts',(2.66151249104242,12.2,10.239630678484));
#221727=CARTESIAN_POINT('Ctrl Pts',(2.66164595777799,12.2,10.2430126681391));
#221728=CARTESIAN_POINT('Ctrl Pts',(2.66177296119402,12.2,10.2464240615365));
#221729=CARTESIAN_POINT('Ctrl Pts',(2.66189325529069,12.2,10.2498645586916));
#221730=CARTESIAN_POINT('Ctrl Pts',(2.66203760820146,12.2,10.2539931551278));
#221731=CARTESIAN_POINT('Ctrl Pts',(2.66217229786168,12.2,10.2581636587725));
#221732=CARTESIAN_POINT('Ctrl Pts',(2.66229691002338,12.2,10.2623755582046));
#221733=CARTESIAN_POINT('Ctrl Pts',(2.66240075349523,12.2,10.2658854745256));
#221734=CARTESIAN_POINT('Ctrl Pts',(2.66249759913949,12.2,10.2694241363985));
#221735=CARTESIAN_POINT('Ctrl Pts',(2.66258721101411,12.2,10.2729912534834));
#221736=CARTESIAN_POINT('Ctrl Pts',(2.66267682288873,12.2,10.2765583705682));
#221737=CARTESIAN_POINT('Ctrl Pts',(2.66275920287207,12.2,10.2801539413877));
#221738=CARTESIAN_POINT('Ctrl Pts',(2.6628341172503,12.2,10.2837776771957));
#221739=CARTESIAN_POINT('Ctrl Pts',(2.66290903162853,12.2,10.2874014130037));
#221740=CARTESIAN_POINT('Ctrl Pts',(2.66297648223063,12.2,10.2910533150067));
#221741=CARTESIAN_POINT('Ctrl Pts',(2.66303624396611,12.2,10.2947330972312));
#221742=CARTESIAN_POINT('Ctrl Pts',(2.66310795804609,12.2,10.2991488357403));
#221743=CARTESIAN_POINT('Ctrl Pts',(2.66316859680157,12.2,10.3036047201364));
#221744=CARTESIAN_POINT('Ctrl Pts',(2.66321778096665,12.2,10.3081002687436));
#221745=CARTESIAN_POINT('Ctrl Pts',(2.66325876777237,12.2,10.3118465593857));
#221746=CARTESIAN_POINT('Ctrl Pts',(2.66329179882974,12.2,10.3156203925083));
#221747=CARTESIAN_POINT('Ctrl Pts',(2.66331665896821,12.2,10.319421492232));
#221748=CARTESIAN_POINT('Ctrl Pts',(2.66334151910667,12.2,10.3232225919557));
#221749=CARTESIAN_POINT('Ctrl Pts',(2.66335820591201,12.2,10.3270509566341));
#221750=CARTESIAN_POINT('Ctrl Pts',(2.66336651021712,12.2,10.3309063147606));
#221751=CARTESIAN_POINT('Ctrl Pts',(2.66337813624356,12.2,10.3363038158013));
#221752=CARTESIAN_POINT('Ctrl Pts',(2.66337332728298,12.2,10.3417542223926));
#221753=CARTESIAN_POINT('Ctrl Pts',(2.66335151674367,12.2,10.3472567914775));
#221754=CARTESIAN_POINT('Ctrl Pts',(2.66333593778604,12.2,10.3511871982115));
#221755=CARTESIAN_POINT('Ctrl Pts',(2.66331168425913,12.2,10.3551442209366));
#221756=CARTESIAN_POINT('Ctrl Pts',(2.6632785537043,12.2,10.3591275924622));
#221757=CARTESIAN_POINT('Ctrl Pts',(2.66323879703633,12.2,10.3639076385535));
#221758=CARTESIAN_POINT('Ctrl Pts',(2.66318625590048,12.2,10.3687256263734));
#221759=CARTESIAN_POINT('Ctrl Pts',(2.66312058922967,12.2,10.373581102723));
#221760=CARTESIAN_POINT('Ctrl Pts',(2.66305492256482,12.2,10.3784365786316));
#221761=CARTESIAN_POINT('Ctrl Pts',(2.66297612703871,12.2,10.3833295449462));
#221762=CARTESIAN_POINT('Ctrl Pts',(2.66288387145834,12.2,10.388259551706));
#221763=CARTESIAN_POINT('Ctrl Pts',(2.66280699180524,12.2,10.3923678908218));
#221764=CARTESIAN_POINT('Ctrl Pts',(2.66272076337219,12.2,10.3965019544776));
#221765=CARTESIAN_POINT('Ctrl Pts',(2.66262499552497,12.2,10.4006614837833));
#221766=CARTESIAN_POINT('Ctrl Pts',(2.66254838124302,12.2,10.4039891074091));
#221767=CARTESIAN_POINT('Ctrl Pts',(2.66246566351313,12.2,10.4073330312423));
#221768=CARTESIAN_POINT('Ctrl Pts',(2.66237674328543,12.2,10.410693125316));
#221769=CARTESIAN_POINT('Ctrl Pts',(2.66228782306984,12.2,10.4140532189319));
#221770=CARTESIAN_POINT('Ctrl Pts',(2.66219270369496,12.2,10.4174294822957));
#221771=CARTESIAN_POINT('Ctrl Pts',(2.66209128875837,12.2,10.4208217867559));
#221772=CARTESIAN_POINT('Ctrl Pts',(2.66198987380796,12.2,10.4242140916783));
#221773=CARTESIAN_POINT('Ctrl Pts',(2.66188216427429,12.2,10.4276224375355));
#221774=CARTESIAN_POINT('Ctrl Pts',(2.66176806598964,12.2,10.4310466983348));
#221775=CARTESIAN_POINT('Ctrl Pts',(2.66165396772054,12.2,10.4344709586676));
#221776=CARTESIAN_POINT('Ctrl Pts',(2.66153348128837,12.2,10.4379111323511));
#221777=CARTESIAN_POINT('Ctrl Pts',(2.66140651574362,12.2,10.4413670947342));
#221778=CARTESIAN_POINT('Ctrl Pts',(2.66124780879971,12.2,10.4456870480662));
#221779=CARTESIAN_POINT('Ctrl Pts',(2.66107897918974,12.2,10.450031669411));
#221780=CARTESIAN_POINT('Ctrl Pts',(2.66089984655007,12.2,10.4544007152642));
#221781=CARTESIAN_POINT('Ctrl Pts',(2.66075654043052,12.2,10.4578959521373));
#221782=CARTESIAN_POINT('Ctrl Pts',(2.66060664228359,12.2,10.4614068210272));
#221783=CARTESIAN_POINT('Ctrl Pts',(2.66045006394103,12.2,10.4649331967765));
#221784=CARTESIAN_POINT('Ctrl Pts',(2.66029348561982,12.2,10.4684595720453));
#221785=CARTESIAN_POINT('Ctrl Pts',(2.66013022550502,12.2,10.4720014564899));
#221786=CARTESIAN_POINT('Ctrl Pts',(2.65996019729714,12.2,10.4755587249759));
#221787=CARTESIAN_POINT('Ctrl Pts',(2.65979016906609,12.2,10.4791159939466));
#221788=CARTESIAN_POINT('Ctrl Pts',(2.65961337264584,12.2,10.4826886483612));
#221789=CARTESIAN_POINT('Ctrl Pts',(2.65942972168162,12.2,10.4862765660706));
#221790=CARTESIAN_POINT('Ctrl Pts',(2.65924607074242,12.2,10.4898644832912));
#221791=CARTESIAN_POINT('Ctrl Pts',(2.65905556443556,12.2,10.4934676640622));
#221792=CARTESIAN_POINT('Ctrl Pts',(2.65885811950771,12.2,10.4970859859876));
#221793=CARTESIAN_POINT('Ctrl Pts',(2.65866067455296,12.2,10.500704308406));
#221794=CARTESIAN_POINT('Ctrl Pts',(2.65845628988627,12.2,10.5043377743068));
#221795=CARTESIAN_POINT('Ctrl Pts',(2.65824488170762,12.2,10.5079862620067));
#221796=CARTESIAN_POINT('Ctrl Pts',(2.65803347355778,12.2,10.5116347492095));
#221797=CARTESIAN_POINT('Ctrl Pts',(2.65781504184987,12.2,10.5152982597234));
#221798=CARTESIAN_POINT('Ctrl Pts',(2.65758950502433,12.2,10.5189766737163));
#221799=CARTESIAN_POINT('Ctrl Pts',(2.65736396816805,12.2,10.5226550882103));
#221800=CARTESIAN_POINT('Ctrl Pts',(2.65713132618551,12.2,10.5263484061167));
#221801=CARTESIAN_POINT('Ctrl Pts',(2.6568914960053,12.2,10.5300565103199));
#221802=CARTESIAN_POINT('Ctrl Pts',(2.65665166585776,12.2,10.5337646140178));
#221803=CARTESIAN_POINT('Ctrl Pts',(2.65640464799223,12.2,10.5374875020459));
#221804=CARTESIAN_POINT('Ctrl Pts',(2.65615036379154,12.2,10.5412250604055));
#221805=CARTESIAN_POINT('Ctrl Pts',(2.65589607955621,12.2,10.5449626192743));
#221806=CARTESIAN_POINT('Ctrl Pts',(2.65563452727124,12.2,10.5487148455384));
#221807=CARTESIAN_POINT('Ctrl Pts',(2.65536562903312,12.2,10.5524816252608));
#221808=CARTESIAN_POINT('Ctrl Pts',(2.65509673083164,12.2,10.55624840447));
#221809=CARTESIAN_POINT('Ctrl Pts',(2.65482048568351,12.2,10.5600297367939));
#221810=CARTESIAN_POINT('Ctrl Pts',(2.65453681626302,12.2,10.563825505871));
#221811=CARTESIAN_POINT('Ctrl Pts',(2.65425314680387,12.2,10.5676212754653));
#221812=CARTESIAN_POINT('Ctrl Pts',(2.65396205249125,12.2,10.5714314816526));
#221813=CARTESIAN_POINT('Ctrl Pts',(2.65366345697498,12.2,10.5752560114166));
#221814=CARTESIAN_POINT('Ctrl Pts',(2.6533648614587,12.2,10.5790805411806));
#221815=CARTESIAN_POINT('Ctrl Pts',(2.65305876464155,12.2,10.5829193948796));
#221816=CARTESIAN_POINT('Ctrl Pts',(2.65274509045702,12.2,10.5867724566466));
#221817=CARTESIAN_POINT('Ctrl Pts',(2.65235299779045,12.2,10.5915887830678));
#221818=CARTESIAN_POINT('Ctrl Pts',(2.65194906610805,12.2,10.5964273139236));
#221819=CARTESIAN_POINT('Ctrl Pts',(2.65153314782104,12.2,10.6012878245725));
#221820=CARTESIAN_POINT('Ctrl Pts',(2.65120041313703,12.2,10.6051762337274));
#221821=CARTESIAN_POINT('Ctrl Pts',(2.65086000863283,12.2,10.6090787133337));
#221822=CARTESIAN_POINT('Ctrl Pts',(2.65051185922498,12.2,10.6129951484916));
#221823=CARTESIAN_POINT('Ctrl Pts',(2.65016370981712,12.2,10.6169115836495));
#221824=CARTESIAN_POINT('Ctrl Pts',(2.64980781704169,12.2,10.6208419761006));
#221825=CARTESIAN_POINT('Ctrl Pts',(2.6494441069655,12.2,10.6247862150948));
#221826=CARTESIAN_POINT('Ctrl Pts',(2.64908039693888,12.2,10.6287304535517));
#221827=CARTESIAN_POINT('Ctrl Pts',(2.64870887046536,12.2,10.632688538165));
#221828=CARTESIAN_POINT('Ctrl Pts',(2.6483294557169,12.2,10.6366603587472));
#221829=CARTESIAN_POINT('Ctrl Pts',(2.64795004091675,12.2,10.6406321798705));
#221830=CARTESIAN_POINT('Ctrl Pts',(2.64756273810492,12.2,10.6446177366123));
#221831=CARTESIAN_POINT('Ctrl Pts',(2.64716747669368,12.2,10.6486169203871));
#221832=CARTESIAN_POINT('Ctrl Pts',(2.64677221533629,12.2,10.6526161036171));
#221833=CARTESIAN_POINT('Ctrl Pts',(2.64636899471604,12.2,10.6566289134899));
#221834=CARTESIAN_POINT('Ctrl Pts',(2.64595774608352,12.2,10.6606552419376));
#221835=CARTESIAN_POINT('Ctrl Pts',(2.64554649739497,12.2,10.6646815709339));
#221836=CARTESIAN_POINT('Ctrl Pts',(2.64512722103601,12.2,10.6687214189096));
#221837=CARTESIAN_POINT('Ctrl Pts',(2.64469984695663,12.2,10.6727746761314));
#221838=CARTESIAN_POINT('Ctrl Pts',(2.64427247293547,12.2,10.676827932801));
#221839=CARTESIAN_POINT('Ctrl Pts',(2.64383700283561,12.2,10.6808946002805));
#221840=CARTESIAN_POINT('Ctrl Pts',(2.64339336757264,12.2,10.6849745716497));
#221841=CARTESIAN_POINT('Ctrl Pts',(2.64294973224923,12.2,10.6890545435747));
#221842=CARTESIAN_POINT('Ctrl Pts',(2.64249793301568,12.2,10.6931478192444));
#221843=CARTESIAN_POINT('Ctrl Pts',(2.64203790221229,12.2,10.6972542911358));
#221844=CARTESIAN_POINT('Ctrl Pts',(2.64157787147158,12.2,10.7013607624676));
#221845=CARTESIAN_POINT('Ctrl Pts',(2.6411096091603,12.2,10.7054804315912));
#221846=CARTESIAN_POINT('Ctrl Pts',(2.64063304931123,12.2,10.7096131921409));
#221847=CARTESIAN_POINT('Ctrl Pts',(2.64015648939721,12.2,10.7137459532536));
#221848=CARTESIAN_POINT('Ctrl Pts',(2.63967163215657,12.2,10.7178918057072));
#221849=CARTESIAN_POINT('Ctrl Pts',(2.63917841401631,12.2,10.7220506442861));
#221850=CARTESIAN_POINT('Ctrl Pts',(2.63868519594325,12.2,10.7262094822984));
#221851=CARTESIAN_POINT('Ctrl Pts',(2.63818361460192,12.2,10.7303813083564));
#221852=CARTESIAN_POINT('Ctrl Pts',(2.63767360786669,12.2,10.7345660156241));
#221853=CARTESIAN_POINT('Ctrl Pts',(2.63716360106198,12.2,10.7387507234619));
#221854=CARTESIAN_POINT('Ctrl Pts',(2.6366451669287,12.2,10.742948314051));
#221855=CARTESIAN_POINT('Ctrl Pts',(2.63611824423331,12.2,10.7471586832249));
#221856=CARTESIAN_POINT('Ctrl Pts',(2.63559132153793,12.2,10.7513690523989));
#221857=CARTESIAN_POINT('Ctrl Pts',(2.63505591051378,12.2,10.7555922006743));
#221858=CARTESIAN_POINT('Ctrl Pts',(2.6345119459277,12.2,10.7598280251842));
#221859=CARTESIAN_POINT('Ctrl Pts',(2.63383199030629,12.2,10.7651228049559));
#221860=CARTESIAN_POINT('Ctrl Pts',(2.63313867280872,12.2,10.7704373907742));
#221861=CARTESIAN_POINT('Ctrl Pts',(2.63243187365076,12.2,10.7757715838022));
#221862=CARTESIAN_POINT('Ctrl Pts',(2.63186643423193,12.2,10.7800389389224));
#221863=CARTESIAN_POINT('Ctrl Pts',(2.63129236556785,12.2,10.7843188425327));
#221864=CARTESIAN_POINT('Ctrl Pts',(2.63070960825831,12.2,10.7886111924333));
#221865=CARTESIAN_POINT('Ctrl Pts',(2.63012685094879,12.2,10.7929035423338));
#221866=CARTESIAN_POINT('Ctrl Pts',(2.62953540452712,12.2,10.7972083395831));
#221867=CARTESIAN_POINT('Ctrl Pts',(2.62893520866017,12.2,10.8015254834308));
#221868=CARTESIAN_POINT('Ctrl Pts',(2.628335012875,12.2,10.8058426266903));
#221869=CARTESIAN_POINT('Ctrl Pts',(2.62772606954156,12.2,10.8101721161739));
#221870=CARTESIAN_POINT('Ctrl Pts',(2.6271083177004,12.2,10.8145138520053));
#221871=CARTESIAN_POINT('Ctrl Pts',(2.62649056577506,12.2,10.8188555884283));
#221872=CARTESIAN_POINT('Ctrl Pts',(2.62586400646495,12.2,10.8232095702718));
#221873=CARTESIAN_POINT('Ctrl Pts',(2.62522858109608,12.2,10.8275756994555));
#221874=CARTESIAN_POINT('Ctrl Pts',(2.62459315581379,12.2,10.8319418280442));
#221875=CARTESIAN_POINT('Ctrl Pts',(2.62394886448265,12.2,10.8363201025008));
#221876=CARTESIAN_POINT('Ctrl Pts',(2.62329565053663,12.2,10.8407104251411));
#221877=CARTESIAN_POINT('Ctrl Pts',(2.62280574005486,12.2,10.8440031672709));
#221878=CARTESIAN_POINT('Ctrl Pts',(2.62231080880289,12.2,10.8473026863327));
#221879=CARTESIAN_POINT('Ctrl Pts',(2.62181083583833,12.2,10.8506089410853));
#221880=CARTESIAN_POINT('Ctrl Pts',(2.62131086287377,12.2,10.8539151958379));
#221881=CARTESIAN_POINT('Ctrl Pts',(2.62080584795862,12.2,10.8572281859478));
#221882=CARTESIAN_POINT('Ctrl Pts',(2.62029576460284,12.2,10.8605478695762));
#221883=CARTESIAN_POINT('Ctrl Pts',(2.6197856811544,12.2,10.8638675538078));
#221884=CARTESIAN_POINT('Ctrl Pts',(2.6192705308962,12.2,10.8671939320079));
#221885=CARTESIAN_POINT('Ctrl Pts',(2.61875029040323,12.2,10.8705269637016));
#221886=CARTESIAN_POINT('Ctrl Pts',(2.61823005000476,12.2,10.8738599947897));
#221887=CARTESIAN_POINT('Ctrl Pts',(2.61770471955658,12.2,10.8771996783191));
#221888=CARTESIAN_POINT('Ctrl Pts',(2.61717427570041,12.2,10.8805459743648));
#221889=CARTESIAN_POINT('Ctrl Pts',(2.61664383184423,12.2,10.8838922704105));
#221890=CARTESIAN_POINT('Ctrl Pts',(2.61610827526565,12.2,10.8872451779264));
#221891=CARTESIAN_POINT('Ctrl Pts',(2.61556758099115,12.2,10.890604657028));
#221892=CARTESIAN_POINT('Ctrl Pts',(2.61484665532456,12.2,10.8950839622933));
#221893=CARTESIAN_POINT('Ctrl Pts',(2.61411659988447,12.2,10.8995749490469));
#221894=CARTESIAN_POINT('Ctrl Pts',(2.61337735811251,12.2,10.9040775229554));
#221895=CARTESIAN_POINT('Ctrl Pts',(2.61282292665763,12.2,10.9074544541537));
#221896=CARTESIAN_POINT('Ctrl Pts',(2.61226332910964,12.2,10.9108379019454));
#221897=CARTESIAN_POINT('Ctrl Pts',(2.61169854211018,12.2,10.914227826689));
#221898=CARTESIAN_POINT('Ctrl Pts',(2.61094549294858,12.2,10.9187477253207));
#221899=CARTESIAN_POINT('Ctrl Pts',(2.6101832194604,12.2,10.9232791378452));
#221900=CARTESIAN_POINT('Ctrl Pts',(2.60941166707963,12.2,10.927821970362));
#221901=CARTESIAN_POINT('Ctrl Pts',(2.60883300276778,12.2,10.9312290949044));
#221902=CARTESIAN_POINT('Ctrl Pts',(2.60824911997133,12.2,10.9346426422758));
#221903=CARTESIAN_POINT('Ctrl Pts',(2.60765999663058,12.2,10.9380625731133));
#221904=CARTESIAN_POINT('Ctrl Pts',(2.60707087328983,12.2,10.9414825039508));
#221905=CARTESIAN_POINT('Ctrl Pts',(2.60647651094153,12.2,10.9449088187939));
#221906=CARTESIAN_POINT('Ctrl Pts',(2.60587688467236,12.2,10.9483414765016));
#221907=CARTESIAN_POINT('Ctrl Pts',(2.60527725829426,12.2,10.951774134833));
#221908=CARTESIAN_POINT('Ctrl Pts',(2.60467237008969,12.2,10.9552131372328));
#221909=CARTESIAN_POINT('Ctrl Pts',(2.60406219812529,12.2,10.9586584434844));
#221910=CARTESIAN_POINT('Ctrl Pts',(2.60345202627174,12.2,10.96210374911));
#221911=CARTESIAN_POINT('Ctrl Pts',(2.60283656999347,12.2,10.9655553577187));
#221912=CARTESIAN_POINT('Ctrl Pts',(2.60221580914056,12.2,10.9690132318436));
#221913=CARTESIAN_POINT('Ctrl Pts',(2.60138812804095,12.2,10.9736237304674));
#221914=CARTESIAN_POINT('Ctrl Pts',(2.60055101650336,12.2,10.9782453664149));
#221915=CARTESIAN_POINT('Ctrl Pts',(2.59970442336445,12.2,10.9828780453778));
#221916=CARTESIAN_POINT('Ctrl Pts',(2.59906947848142,12.2,10.9863525547577));
#221917=CARTESIAN_POINT('Ctrl Pts',(2.59842920046654,12.2,10.989833277284));
#221918=CARTESIAN_POINT('Ctrl Pts',(2.59778356911573,12.2,10.9933201719898));
#221919=CARTESIAN_POINT('Ctrl Pts',(2.59713793764762,12.2,10.9968070673291));
#221920=CARTESIAN_POINT('Ctrl Pts',(2.59648695306968,12.2,11.0003001357701));
#221921=CARTESIAN_POINT('Ctrl Pts',(2.59583059309856,12.2,11.0037993390295));
#221922=CARTESIAN_POINT('Ctrl Pts',(2.59495544666912,12.2,11.0084649423158));
#221923=CARTESIAN_POINT('Ctrl Pts',(2.59407074612426,12.2,11.0131414503702));
#221924=CARTESIAN_POINT('Ctrl Pts',(2.59317644303133,12.2,11.0178287723752));
#221925=CARTESIAN_POINT('Ctrl Pts',(2.59250571568118,12.2,11.0213442640386));
#221926=CARTESIAN_POINT('Ctrl Pts',(2.59182958635638,12.2,11.0248658385099));
#221927=CARTESIAN_POINT('Ctrl Pts',(2.59114803642356,12.2,11.0283934567143));
#221928=CARTESIAN_POINT('Ctrl Pts',(2.59046648636691,12.2,11.0319210755594));
#221929=CARTESIAN_POINT('Ctrl Pts',(2.58977951378373,12.2,11.035454738723));
#221930=CARTESIAN_POINT('Ctrl Pts',(2.58908710030737,12.2,11.0389944079883));
#221931=CARTESIAN_POINT('Ctrl Pts',(2.58839468695679,12.2,11.0425340766104));
#221932=CARTESIAN_POINT('Ctrl Pts',(2.58769683282407,12.2,11.0460797509048));
#221933=CARTESIAN_POINT('Ctrl Pts',(2.58699351739719,12.2,11.0496313932038));
#221934=CARTESIAN_POINT('Ctrl Pts',(2.58605576353728,12.2,11.0543669160541));
#221935=CARTESIAN_POINT('Ctrl Pts',(2.58510829972704,12.2,11.0591130463035));
#221936=CARTESIAN_POINT('Ctrl Pts',(2.58415108202815,12.2,11.0638696963028));
#221937=CARTESIAN_POINT('Ctrl Pts',(2.58343316872137,12.2,11.0674371839644));
#221938=CARTESIAN_POINT('Ctrl Pts',(2.58270976921498,12.2,11.0710105893172));
#221939=CARTESIAN_POINT('Ctrl Pts',(2.58198086240888,12.2,11.074589872978));
#221940=CARTESIAN_POINT('Ctrl Pts',(2.58125195547036,12.2,11.078169157289));
#221941=CARTESIAN_POINT('Ctrl Pts',(2.58051754229697,12.2,11.0817543204768));
#221942=CARTESIAN_POINT('Ctrl Pts',(2.57977760385534,12.2,11.0853453252911));
#221943=CARTESIAN_POINT('Ctrl Pts',(2.57879101949055,12.2,11.090133330623));
#221944=CARTESIAN_POINT('Ctrl Pts',(2.57779461263128,12.2,11.094931720168));
#221945=CARTESIAN_POINT('Ctrl Pts',(2.576788338209,12.2,11.0997404054634));
#221946=CARTESIAN_POINT('Ctrl Pts',(2.57603363235801,12.2,11.1033469195987));
#221947=CARTESIAN_POINT('Ctrl Pts',(2.57527337593838,12.2,11.1069592246876));
#221948=CARTESIAN_POINT('Ctrl Pts',(2.57450755063337,12.2,11.110577283389));
#221949=CARTESIAN_POINT('Ctrl Pts',(2.57374172532834,12.2,11.1141953420904));
#221950=CARTESIAN_POINT('Ctrl Pts',(2.57297033109037,12.2,11.1178191552247));
#221951=CARTESIAN_POINT('Ctrl Pts',(2.57219334936936,12.2,11.121448684967));
#221952=CARTESIAN_POINT('Ctrl Pts',(2.57115737364725,12.2,11.1262880583964));
#221953=CARTESIAN_POINT('Ctrl Pts',(2.57011146574774,12.2,11.1311375975913));
#221954=CARTESIAN_POINT('Ctrl Pts',(2.56905558174093,12.2,11.1359972097116));
#221955=CARTESIAN_POINT('Ctrl Pts',(2.56826366880775,12.2,11.1396419184707));
#221956=CARTESIAN_POINT('Ctrl Pts',(2.56746614255848,12.2,11.1432922950796));
#221957=CARTESIAN_POINT('Ctrl Pts',(2.56666298675071,12.2,11.1469482997966));
#221958=CARTESIAN_POINT('Ctrl Pts',(2.56585983094294,12.2,11.1506043045137));
#221959=CARTESIAN_POINT('Ctrl Pts',(2.56505104525857,12.2,11.1542659381007));
#221960=CARTESIAN_POINT('Ctrl Pts',(2.56423661208033,12.2,11.1579331668836));
#221961=CARTESIAN_POINT('Ctrl Pts',(2.56342217890209,12.2,11.1616003956665));
#221962=CARTESIAN_POINT('Ctrl Pts',(2.56260210048255,12.2,11.1652732199658));
#221963=CARTESIAN_POINT('Ctrl Pts',(2.56177635817999,12.2,11.1689516051647));
#221964=CARTESIAN_POINT('Ctrl Pts',(2.56095061572743,12.2,11.1726299910319));
#221965=CARTESIAN_POINT('Ctrl Pts',(2.56011920953992,12.2,11.1763139382507));
#221966=CARTESIAN_POINT('Ctrl Pts',(2.55928211854249,12.2,11.1800034004959));
#221967=CARTESIAN_POINT('Ctrl Pts',(2.55844502769714,12.2,11.183692862071));
#221968=CARTESIAN_POINT('Ctrl Pts',(2.55760225159798,12.2,11.1873878384482));
#221969=CARTESIAN_POINT('Ctrl Pts',(2.55675377133577,12.2,11.1910882904993));
#221970=CARTESIAN_POINT('Ctrl Pts',(2.55590529107355,12.2,11.1947887425503));
#221971=CARTESIAN_POINT('Ctrl Pts',(2.55505110672384,12.2,11.198494670904));
#221972=CARTESIAN_POINT('Ctrl Pts',(2.55419121115239,12.2,11.2022060571883));
#221973=CARTESIAN_POINT('Ctrl Pts',(2.55333131558093,12.2,11.2059174434726));
#221974=CARTESIAN_POINT('Ctrl Pts',(2.55246570515823,12.2,11.2096342873238));
#221975=CARTESIAN_POINT('Ctrl Pts',(2.55159438999994,12.2,11.213356593));
#221976=CARTESIAN_POINT('Ctrl Pts',(2.17615954699994,15.2,11.292224299));
#221977=CARTESIAN_POINT('Ctrl Pts',(2.17615954699994,11.6,11.292224299));
#221978=CARTESIAN_POINT('Ctrl Pts',(2.17570045499994,15.2,11.291612888));
#221979=CARTESIAN_POINT('Ctrl Pts',(2.17570045499994,11.6,11.291612888));
#221980=CARTESIAN_POINT('Ctrl Pts',(2.17478276499994,15.2,11.290390245));
#221981=CARTESIAN_POINT('Ctrl Pts',(2.17478276499994,11.6,11.290390245));
#221982=CARTESIAN_POINT('Ctrl Pts',(2.17340771699994,15.2,11.28855682));
#221983=CARTESIAN_POINT('Ctrl Pts',(2.17340771699994,11.6,11.28855682));
#221984=CARTESIAN_POINT('Ctrl Pts',(2.17157728799994,15.2,11.286113333));
#221985=CARTESIAN_POINT('Ctrl Pts',(2.17157728799994,11.6,11.286113333));
#221986=CARTESIAN_POINT('Ctrl Pts',(2.16929420199994,15.2,11.283060774));
#221987=CARTESIAN_POINT('Ctrl Pts',(2.16929420199994,11.6,11.283060774));
#221988=CARTESIAN_POINT('Ctrl Pts',(2.16701606599994,15.2,11.280010014));
#221989=CARTESIAN_POINT('Ctrl Pts',(2.16701606599994,11.6,11.280010014));
#221990=CARTESIAN_POINT('Ctrl Pts',(2.16474288099994,15.2,11.276961058));
#221991=CARTESIAN_POINT('Ctrl Pts',(2.16474288099994,11.6,11.276961058));
#221992=CARTESIAN_POINT('Ctrl Pts',(2.16247464499994,15.2,11.273913908));
#221993=CARTESIAN_POINT('Ctrl Pts',(2.16247464499994,11.6,11.273913908));
#221994=CARTESIAN_POINT('Ctrl Pts',(2.16021135899994,15.2,11.270868571));
#221995=CARTESIAN_POINT('Ctrl Pts',(2.16021135899994,11.6,11.270868571));
#221996=CARTESIAN_POINT('Ctrl Pts',(2.15795302399994,15.2,11.267825055));
#221997=CARTESIAN_POINT('Ctrl Pts',(2.15795302399994,11.6,11.267825055));
#221998=CARTESIAN_POINT('Ctrl Pts',(2.15569963799994,15.2,11.264783368));
#221999=CARTESIAN_POINT('Ctrl Pts',(2.15569963799994,11.6,11.264783368));
#222000=CARTESIAN_POINT('Ctrl Pts',(2.15345120199994,15.2,11.261743524));
#222001=CARTESIAN_POINT('Ctrl Pts',(2.15345120199994,11.6,11.261743524));
#222002=CARTESIAN_POINT('Ctrl Pts',(2.15120771399994,15.2,11.258705532));
#222003=CARTESIAN_POINT('Ctrl Pts',(2.15120771399994,11.6,11.258705532));
#222004=CARTESIAN_POINT('Ctrl Pts',(2.14896917399995,15.2,11.255669403));
#222005=CARTESIAN_POINT('Ctrl Pts',(2.14896917399995,11.6,11.255669403));
#222006=CARTESIAN_POINT('Ctrl Pts',(2.14673558299994,15.2,11.252635149));
#222007=CARTESIAN_POINT('Ctrl Pts',(2.14673558299994,11.6,11.252635149));
#222008=CARTESIAN_POINT('Ctrl Pts',(2.14450693999995,15.2,11.249602778));
#222009=CARTESIAN_POINT('Ctrl Pts',(2.14450693999995,11.6,11.249602778));
#222010=CARTESIAN_POINT('Ctrl Pts',(2.14228324299994,15.2,11.246572299));
#222011=CARTESIAN_POINT('Ctrl Pts',(2.14228324299994,11.6,11.246572299));
#222012=CARTESIAN_POINT('Ctrl Pts',(2.14006449499994,15.2,11.243543721));
#222013=CARTESIAN_POINT('Ctrl Pts',(2.14006449499994,11.6,11.243543721));
#222014=CARTESIAN_POINT('Ctrl Pts',(2.13785069299994,15.2,11.24051705));
#222015=CARTESIAN_POINT('Ctrl Pts',(2.13785069299994,11.6,11.24051705));
#222016=CARTESIAN_POINT('Ctrl Pts',(2.13564183699994,15.2,11.237492297));
#222017=CARTESIAN_POINT('Ctrl Pts',(2.13564183699994,11.6,11.237492297));
#222018=CARTESIAN_POINT('Ctrl Pts',(2.13343792799995,15.2,11.234469469));
#222019=CARTESIAN_POINT('Ctrl Pts',(2.13343792799995,11.6,11.234469469));
#222020=CARTESIAN_POINT('Ctrl Pts',(2.13123896499994,15.2,11.231448575));
#222021=CARTESIAN_POINT('Ctrl Pts',(2.13123896499994,11.6,11.231448575));
#222022=CARTESIAN_POINT('Ctrl Pts',(2.12904494799994,15.2,11.228429624));
#222023=CARTESIAN_POINT('Ctrl Pts',(2.12904494799994,11.6,11.228429624));
#222024=CARTESIAN_POINT('Ctrl Pts',(2.12685587499994,15.2,11.225412627));
#222025=CARTESIAN_POINT('Ctrl Pts',(2.12685587499994,11.6,11.225412627));
#222026=CARTESIAN_POINT('Ctrl Pts',(2.12467174699994,15.2,11.222397591));
#222027=CARTESIAN_POINT('Ctrl Pts',(2.12467174699994,11.6,11.222397591));
#222028=CARTESIAN_POINT('Ctrl Pts',(2.12249256499994,15.2,11.219384528));
#222029=CARTESIAN_POINT('Ctrl Pts',(2.12249256499994,11.6,11.219384528));
#222030=CARTESIAN_POINT('Ctrl Pts',(2.12031832399994,15.2,11.216373447));
#222031=CARTESIAN_POINT('Ctrl Pts',(2.12031832399994,11.6,11.216373447));
#222032=CARTESIAN_POINT('Ctrl Pts',(2.11814902899994,15.2,11.213364355));
#222033=CARTESIAN_POINT('Ctrl Pts',(2.11814902899994,11.6,11.213364355));
#222034=CARTESIAN_POINT('Ctrl Pts',(2.11598467599994,15.2,11.210357263));
#222035=CARTESIAN_POINT('Ctrl Pts',(2.11598467599994,11.6,11.210357263));
#222036=CARTESIAN_POINT('Ctrl Pts',(2.11382526699994,15.2,11.207352181));
#222037=CARTESIAN_POINT('Ctrl Pts',(2.11382526699994,11.6,11.207352181));
#222038=CARTESIAN_POINT('Ctrl Pts',(2.11167079899994,15.2,11.204349116));
#222039=CARTESIAN_POINT('Ctrl Pts',(2.11167079899994,11.6,11.204349116));
#222040=CARTESIAN_POINT('Ctrl Pts',(2.10952127399994,15.2,11.201348078));
#222041=CARTESIAN_POINT('Ctrl Pts',(2.10952127399994,11.6,11.201348078));
#222042=CARTESIAN_POINT('Ctrl Pts',(2.10737668999994,15.2,11.198349076));
#222043=CARTESIAN_POINT('Ctrl Pts',(2.10737668999994,11.6,11.198349076));
#222044=CARTESIAN_POINT('Ctrl Pts',(2.10523704699995,15.2,11.19535212));
#222045=CARTESIAN_POINT('Ctrl Pts',(2.10523704699995,11.6,11.19535212));
#222046=CARTESIAN_POINT('Ctrl Pts',(2.10310234499994,15.2,11.192357218));
#222047=CARTESIAN_POINT('Ctrl Pts',(2.10310234499994,11.6,11.192357218));
#222048=CARTESIAN_POINT('Ctrl Pts',(2.10097258199994,15.2,11.189364381));
#222049=CARTESIAN_POINT('Ctrl Pts',(2.10097258199994,11.6,11.189364381));
#222050=CARTESIAN_POINT('Ctrl Pts',(2.09884775899994,15.2,11.186373617));
#222051=CARTESIAN_POINT('Ctrl Pts',(2.09884775899994,11.6,11.186373617));
#222052=CARTESIAN_POINT('Ctrl Pts',(2.09672787599994,15.2,11.183384935));
#222053=CARTESIAN_POINT('Ctrl Pts',(2.09672787599994,11.6,11.183384935));
#222054=CARTESIAN_POINT('Ctrl Pts',(2.09461293099994,15.2,11.180398346));
#222055=CARTESIAN_POINT('Ctrl Pts',(2.09461293099994,11.6,11.180398346));
#222056=CARTESIAN_POINT('Ctrl Pts',(2.09250292399994,15.2,11.177413859));
#222057=CARTESIAN_POINT('Ctrl Pts',(2.09250292399994,11.6,11.177413859));
#222058=CARTESIAN_POINT('Ctrl Pts',(2.09039785499994,15.2,11.174431483));
#222059=CARTESIAN_POINT('Ctrl Pts',(2.09039785499994,11.6,11.174431483));
#222060=CARTESIAN_POINT('Ctrl Pts',(2.08829772299994,15.2,11.171451227));
#222061=CARTESIAN_POINT('Ctrl Pts',(2.08829772299994,11.6,11.171451227));
#222062=CARTESIAN_POINT('Ctrl Pts',(2.08620252699994,15.2,11.168473101));
#222063=CARTESIAN_POINT('Ctrl Pts',(2.08620252699994,11.6,11.168473101));
#222064=CARTESIAN_POINT('Ctrl Pts',(2.08411226699994,15.2,11.165497114));
#222065=CARTESIAN_POINT('Ctrl Pts',(2.08411226699994,11.6,11.165497114));
#222066=CARTESIAN_POINT('Ctrl Pts',(2.08202694399994,15.2,11.162523276));
#222067=CARTESIAN_POINT('Ctrl Pts',(2.08202694399994,11.6,11.162523276));
#222068=CARTESIAN_POINT('Ctrl Pts',(2.07994655499994,15.2,11.159551596));
#222069=CARTESIAN_POINT('Ctrl Pts',(2.07994655499994,11.6,11.159551596));
#222070=CARTESIAN_POINT('Ctrl Pts',(2.07787109999995,15.2,11.156582083));
#222071=CARTESIAN_POINT('Ctrl Pts',(2.07787109999995,11.6,11.156582083));
#222072=CARTESIAN_POINT('Ctrl Pts',(2.07580057999994,15.2,11.153614749));
#222073=CARTESIAN_POINT('Ctrl Pts',(2.07580057999994,11.6,11.153614749));
#222074=CARTESIAN_POINT('Ctrl Pts',(2.07373499199994,15.2,11.1506496));
#222075=CARTESIAN_POINT('Ctrl Pts',(2.07373499199994,11.6,11.1506496));
#222076=CARTESIAN_POINT('Ctrl Pts',(2.07167433699994,15.2,11.147686647));
#222077=CARTESIAN_POINT('Ctrl Pts',(2.07167433699994,11.6,11.147686647));
#222078=CARTESIAN_POINT('Ctrl Pts',(2.06961861499994,15.2,11.144725901));
#222079=CARTESIAN_POINT('Ctrl Pts',(2.06961861499994,11.6,11.144725901));
#222080=CARTESIAN_POINT('Ctrl Pts',(2.06756782299994,15.2,11.14176737));
#222081=CARTESIAN_POINT('Ctrl Pts',(2.06756782299994,11.6,11.14176737));
#222082=CARTESIAN_POINT('Ctrl Pts',(2.06552196199994,15.2,11.138811063));
#222083=CARTESIAN_POINT('Ctrl Pts',(2.06552196199994,11.6,11.138811063));
#222084=CARTESIAN_POINT('Ctrl Pts',(2.06348103199994,15.2,11.13585699));
#222085=CARTESIAN_POINT('Ctrl Pts',(2.06348103199994,11.6,11.13585699));
#222086=CARTESIAN_POINT('Ctrl Pts',(2.06144503099994,15.2,11.132905163));
#222087=CARTESIAN_POINT('Ctrl Pts',(2.06144503099994,11.6,11.132905163));
#222088=CARTESIAN_POINT('Ctrl Pts',(2.05941395899994,15.2,11.129955588));
#222089=CARTESIAN_POINT('Ctrl Pts',(2.05941395899994,11.6,11.129955588));
#222090=CARTESIAN_POINT('Ctrl Pts',(2.05738781599994,15.2,11.127008278));
#222091=CARTESIAN_POINT('Ctrl Pts',(2.05738781599994,11.6,11.127008278));
#222092=CARTESIAN_POINT('Ctrl Pts',(2.05536659999995,15.2,11.12406324));
#222093=CARTESIAN_POINT('Ctrl Pts',(2.05536659999995,11.6,11.12406324));
#222094=CARTESIAN_POINT('Ctrl Pts',(2.05335030999994,15.2,11.121120485));
#222095=CARTESIAN_POINT('Ctrl Pts',(2.05335030999994,11.6,11.121120485));
#222096=CARTESIAN_POINT('Ctrl Pts',(2.05133894799994,15.2,11.118180022));
#222097=CARTESIAN_POINT('Ctrl Pts',(2.05133894799994,11.6,11.118180022));
#222098=CARTESIAN_POINT('Ctrl Pts',(2.04933251099995,15.2,11.115241863));
#222099=CARTESIAN_POINT('Ctrl Pts',(2.04933251099995,11.6,11.115241863));
#222100=CARTESIAN_POINT('Ctrl Pts',(2.04733099799994,15.2,11.112306014));
#222101=CARTESIAN_POINT('Ctrl Pts',(2.04733099799994,11.6,11.112306014));
#222102=CARTESIAN_POINT('Ctrl Pts',(2.04533441099994,15.2,11.109372487));
#222103=CARTESIAN_POINT('Ctrl Pts',(2.04533441099994,11.6,11.109372487));
#222104=CARTESIAN_POINT('Ctrl Pts',(2.04334274699994,15.2,11.106441291));
#222105=CARTESIAN_POINT('Ctrl Pts',(2.04334274699994,11.6,11.106441291));
#222106=CARTESIAN_POINT('Ctrl Pts',(2.04135600499994,15.2,11.103512437));
#222107=CARTESIAN_POINT('Ctrl Pts',(2.04135600499994,11.6,11.103512437));
#222108=CARTESIAN_POINT('Ctrl Pts',(2.03937418399994,15.2,11.100585934));
#222109=CARTESIAN_POINT('Ctrl Pts',(2.03937418399994,11.6,11.100585934));
#222110=CARTESIAN_POINT('Ctrl Pts',(2.03739728499994,15.2,11.097661791));
#222111=CARTESIAN_POINT('Ctrl Pts',(2.03739728499994,11.6,11.097661791));
#222112=CARTESIAN_POINT('Ctrl Pts',(2.03542530699994,15.2,11.094740019));
#222113=CARTESIAN_POINT('Ctrl Pts',(2.03542530699994,11.6,11.094740019));
#222114=CARTESIAN_POINT('Ctrl Pts',(2.03345824999994,15.2,11.091820628));
#222115=CARTESIAN_POINT('Ctrl Pts',(2.03345824999994,11.6,11.091820628));
#222116=CARTESIAN_POINT('Ctrl Pts',(2.03149610999994,15.2,11.088903627));
#222117=CARTESIAN_POINT('Ctrl Pts',(2.03149610999994,11.6,11.088903627));
#222118=CARTESIAN_POINT('Ctrl Pts',(2.02953888899994,15.2,11.085989026));
#222119=CARTESIAN_POINT('Ctrl Pts',(2.02953888899994,11.6,11.085989026));
#222120=CARTESIAN_POINT('Ctrl Pts',(2.02758658499994,15.2,11.083076836));
#222121=CARTESIAN_POINT('Ctrl Pts',(2.02758658499994,11.6,11.083076836));
#222122=CARTESIAN_POINT('Ctrl Pts',(2.02563919799994,15.2,11.080167065));
#222123=CARTESIAN_POINT('Ctrl Pts',(2.02563919799994,11.6,11.080167065));
#222124=CARTESIAN_POINT('Ctrl Pts',(2.02369672699994,15.2,11.077259725));
#222125=CARTESIAN_POINT('Ctrl Pts',(2.02369672699994,11.6,11.077259725));
#222126=CARTESIAN_POINT('Ctrl Pts',(2.02175917099995,15.2,11.074354824));
#222127=CARTESIAN_POINT('Ctrl Pts',(2.02175917099995,11.6,11.074354824));
#222128=CARTESIAN_POINT('Ctrl Pts',(2.01982652899994,15.2,11.071452374));
#222129=CARTESIAN_POINT('Ctrl Pts',(2.01982652899994,11.6,11.071452374));
#222130=CARTESIAN_POINT('Ctrl Pts',(2.01789879999994,15.2,11.068552383));
#222131=CARTESIAN_POINT('Ctrl Pts',(2.01789879999994,11.6,11.068552383));
#222132=CARTESIAN_POINT('Ctrl Pts',(2.01597598299994,15.2,11.065654862));
#222133=CARTESIAN_POINT('Ctrl Pts',(2.01597598299994,11.6,11.065654862));
#222134=CARTESIAN_POINT('Ctrl Pts',(2.01405807799994,15.2,11.062759822));
#222135=CARTESIAN_POINT('Ctrl Pts',(2.01405807799994,11.6,11.062759822));
#222136=CARTESIAN_POINT('Ctrl Pts',(2.01214508399994,15.2,11.059867271));
#222137=CARTESIAN_POINT('Ctrl Pts',(2.01214508399994,11.6,11.059867271));
#222138=CARTESIAN_POINT('Ctrl Pts',(2.01023699999994,15.2,11.056977221));
#222139=CARTESIAN_POINT('Ctrl Pts',(2.01023699999994,11.6,11.056977221));
#222140=CARTESIAN_POINT('Ctrl Pts',(2.00833382599995,15.2,11.054089681));
#222141=CARTESIAN_POINT('Ctrl Pts',(2.00833382599995,11.6,11.054089681));
#222142=CARTESIAN_POINT('Ctrl Pts',(2.00643555799994,15.2,11.051204661));
#222143=CARTESIAN_POINT('Ctrl Pts',(2.00643555799994,11.6,11.051204661));
#222144=CARTESIAN_POINT('Ctrl Pts',(2.00454219899994,15.2,11.048322171));
#222145=CARTESIAN_POINT('Ctrl Pts',(2.00454219899994,11.6,11.048322171));
#222146=CARTESIAN_POINT('Ctrl Pts',(2.00265374499994,15.2,11.045442222));
#222147=CARTESIAN_POINT('Ctrl Pts',(2.00265374499994,11.6,11.045442222));
#222148=CARTESIAN_POINT('Ctrl Pts',(2.00077019699994,15.2,11.042564824));
#222149=CARTESIAN_POINT('Ctrl Pts',(2.00077019699994,11.6,11.042564824));
#222150=CARTESIAN_POINT('Ctrl Pts',(1.99889155299994,15.2,11.039689986));
#222151=CARTESIAN_POINT('Ctrl Pts',(1.99889155299994,11.6,11.039689986));
#222152=CARTESIAN_POINT('Ctrl Pts',(1.99701781299994,15.2,11.036817721));
#222153=CARTESIAN_POINT('Ctrl Pts',(1.99701781299994,11.6,11.036817721));
#222154=CARTESIAN_POINT('Ctrl Pts',(1.99514897499994,15.2,11.033948035));
#222155=CARTESIAN_POINT('Ctrl Pts',(1.99514897499994,11.6,11.033948035));
#222156=CARTESIAN_POINT('Ctrl Pts',(1.99328503899994,15.2,11.031080942));
#222157=CARTESIAN_POINT('Ctrl Pts',(1.99328503899994,11.6,11.031080942));
#222158=CARTESIAN_POINT('Ctrl Pts',(1.99142600299994,15.2,11.02821645));
#222159=CARTESIAN_POINT('Ctrl Pts',(1.99142600299994,11.6,11.02821645));
#222160=CARTESIAN_POINT('Ctrl Pts',(1.98957186799994,15.2,11.025354571));
#222161=CARTESIAN_POINT('Ctrl Pts',(1.98957186799994,11.6,11.025354571));
#222162=CARTESIAN_POINT('Ctrl Pts',(1.98772262899995,15.2,11.022495314));
#222163=CARTESIAN_POINT('Ctrl Pts',(1.98772262899995,11.6,11.022495314));
#222164=CARTESIAN_POINT('Ctrl Pts',(1.98587828999994,15.2,11.019638689));
#222165=CARTESIAN_POINT('Ctrl Pts',(1.98587828999994,11.6,11.019638689));
#222166=CARTESIAN_POINT('Ctrl Pts',(1.98403884699994,15.2,11.016784707));
#222167=CARTESIAN_POINT('Ctrl Pts',(1.98403884699994,11.6,11.016784707));
#222168=CARTESIAN_POINT('Ctrl Pts',(1.98220429799994,15.2,11.01393338));
#222169=CARTESIAN_POINT('Ctrl Pts',(1.98220429799994,11.6,11.01393338));
#222170=CARTESIAN_POINT('Ctrl Pts',(1.98037464499994,15.2,11.011084715));
#222171=CARTESIAN_POINT('Ctrl Pts',(1.98037464499994,11.6,11.011084715));
#222172=CARTESIAN_POINT('Ctrl Pts',(1.97854988599994,15.2,11.008238724));
#222173=CARTESIAN_POINT('Ctrl Pts',(1.97854988599994,11.6,11.008238724));
#222174=CARTESIAN_POINT('Ctrl Pts',(1.97673001799994,15.2,11.005395419));
#222175=CARTESIAN_POINT('Ctrl Pts',(1.97673001799994,11.6,11.005395419));
#222176=CARTESIAN_POINT('Ctrl Pts',(1.97491504199994,15.2,11.002554807));
#222177=CARTESIAN_POINT('Ctrl Pts',(1.97491504199994,11.6,11.002554807));
#222178=CARTESIAN_POINT('Ctrl Pts',(1.97310495599994,15.2,10.999716902));
#222179=CARTESIAN_POINT('Ctrl Pts',(1.97310495599994,11.6,10.999716902));
#222180=CARTESIAN_POINT('Ctrl Pts',(1.97129975999994,15.2,10.996881711));
#222181=CARTESIAN_POINT('Ctrl Pts',(1.97129975999994,11.6,10.996881711));
#222182=CARTESIAN_POINT('Ctrl Pts',(1.96949945099994,15.2,10.994049248));
#222183=CARTESIAN_POINT('Ctrl Pts',(1.96949945099994,11.6,10.994049248));
#222184=CARTESIAN_POINT('Ctrl Pts',(1.96770402899994,15.2,10.991219521));
#222185=CARTESIAN_POINT('Ctrl Pts',(1.96770402899994,11.6,10.991219521));
#222186=CARTESIAN_POINT('Ctrl Pts',(1.96591349399994,15.2,10.988392541));
#222187=CARTESIAN_POINT('Ctrl Pts',(1.96591349399994,11.6,10.988392541));
#222188=CARTESIAN_POINT('Ctrl Pts',(1.96412784199994,15.2,10.98556832));
#222189=CARTESIAN_POINT('Ctrl Pts',(1.96412784199994,11.6,10.98556832));
#222190=CARTESIAN_POINT('Ctrl Pts',(1.96234707499994,15.2,10.982746866));
#222191=CARTESIAN_POINT('Ctrl Pts',(1.96234707499994,11.6,10.982746866));
#222192=CARTESIAN_POINT('Ctrl Pts',(1.96057118999994,15.2,10.979928192));
#222193=CARTESIAN_POINT('Ctrl Pts',(1.96057118999994,11.6,10.979928192));
#222194=CARTESIAN_POINT('Ctrl Pts',(1.95880018599994,15.2,10.977112307));
#222195=CARTESIAN_POINT('Ctrl Pts',(1.95880018599994,11.6,10.977112307));
#222196=CARTESIAN_POINT('Ctrl Pts',(1.95703406199994,15.2,10.974299224));
#222197=CARTESIAN_POINT('Ctrl Pts',(1.95703406199994,11.6,10.974299224));
#222198=CARTESIAN_POINT('Ctrl Pts',(1.95527281699994,15.2,10.971488949));
#222199=CARTESIAN_POINT('Ctrl Pts',(1.95527281699994,11.6,10.971488949));
#222200=CARTESIAN_POINT('Ctrl Pts',(1.95351644999994,15.2,10.968681497));
#222201=CARTESIAN_POINT('Ctrl Pts',(1.95351644999994,11.6,10.968681497));
#222202=CARTESIAN_POINT('Ctrl Pts',(1.95176495899994,15.2,10.965876878));
#222203=CARTESIAN_POINT('Ctrl Pts',(1.95176495899994,11.6,10.965876878));
#222204=CARTESIAN_POINT('Ctrl Pts',(1.95001834399994,15.2,10.9630751));
#222205=CARTESIAN_POINT('Ctrl Pts',(1.95001834399994,11.6,10.9630751));
#222206=CARTESIAN_POINT('Ctrl Pts',(1.94827660299994,15.2,10.960276177));
#222207=CARTESIAN_POINT('Ctrl Pts',(1.94827660299994,11.6,10.960276177));
#222208=CARTESIAN_POINT('Ctrl Pts',(1.94653973299994,15.2,10.957480118));
#222209=CARTESIAN_POINT('Ctrl Pts',(1.94653973299994,11.6,10.957480118));
#222210=CARTESIAN_POINT('Ctrl Pts',(1.94480773699994,15.2,10.954686935));
#222211=CARTESIAN_POINT('Ctrl Pts',(1.94480773699994,11.6,10.954686935));
#222212=CARTESIAN_POINT('Ctrl Pts',(1.94308060999994,15.2,10.951896637));
#222213=CARTESIAN_POINT('Ctrl Pts',(1.94308060999994,11.6,10.951896637));
#222214=CARTESIAN_POINT('Ctrl Pts',(1.94135835199994,15.2,10.949109235));
#222215=CARTESIAN_POINT('Ctrl Pts',(1.94135835199994,11.6,10.949109235));
#222216=CARTESIAN_POINT('Ctrl Pts',(1.93964096199994,15.2,10.946324741));
#222217=CARTESIAN_POINT('Ctrl Pts',(1.93964096199994,11.6,10.946324741));
#222218=CARTESIAN_POINT('Ctrl Pts',(1.93792843899994,15.2,10.943543166));
#222219=CARTESIAN_POINT('Ctrl Pts',(1.93792843899994,11.6,10.943543166));
#222220=CARTESIAN_POINT('Ctrl Pts',(1.93622078099994,15.2,10.94076452));
#222221=CARTESIAN_POINT('Ctrl Pts',(1.93622078099994,11.6,10.94076452));
#222222=CARTESIAN_POINT('Ctrl Pts',(1.93451798599994,15.2,10.937988814));
#222223=CARTESIAN_POINT('Ctrl Pts',(1.93451798599994,11.6,10.937988814));
#222224=CARTESIAN_POINT('Ctrl Pts',(1.93282005399994,15.2,10.935216059));
#222225=CARTESIAN_POINT('Ctrl Pts',(1.93282005399994,11.6,10.935216059));
#222226=CARTESIAN_POINT('Ctrl Pts',(1.93112698299994,15.2,10.932446265));
#222227=CARTESIAN_POINT('Ctrl Pts',(1.93112698299994,11.6,10.932446265));
#222228=CARTESIAN_POINT('Ctrl Pts',(1.92943877199994,15.2,10.929679446));
#222229=CARTESIAN_POINT('Ctrl Pts',(1.92943877199994,11.6,10.929679446));
#222230=CARTESIAN_POINT('Ctrl Pts',(1.92775541899994,15.2,10.92691561));
#222231=CARTESIAN_POINT('Ctrl Pts',(1.92775541899994,11.6,10.92691561));
#222232=CARTESIAN_POINT('Ctrl Pts',(1.92607692399994,15.2,10.924154768));
#222233=CARTESIAN_POINT('Ctrl Pts',(1.92607692399994,11.6,10.924154768));
#222234=CARTESIAN_POINT('Ctrl Pts',(1.92440328299994,15.2,10.921396933));
#222235=CARTESIAN_POINT('Ctrl Pts',(1.92440328299994,11.6,10.921396933));
#222236=CARTESIAN_POINT('Ctrl Pts',(1.92273449799994,15.2,10.918642115));
#222237=CARTESIAN_POINT('Ctrl Pts',(1.92273449799994,11.6,10.918642115));
#222238=CARTESIAN_POINT('Ctrl Pts',(1.92107056499994,15.2,10.915890325));
#222239=CARTESIAN_POINT('Ctrl Pts',(1.92107056499994,11.6,10.915890325));
#222240=CARTESIAN_POINT('Ctrl Pts',(1.91941148399994,15.2,10.913141574));
#222241=CARTESIAN_POINT('Ctrl Pts',(1.91941148399994,11.6,10.913141574));
#222242=CARTESIAN_POINT('Ctrl Pts',(1.91775725299994,15.2,10.910395872));
#222243=CARTESIAN_POINT('Ctrl Pts',(1.91775725299994,11.6,10.910395872));
#222244=CARTESIAN_POINT('Ctrl Pts',(1.91610786999994,15.2,10.907653233));
#222245=CARTESIAN_POINT('Ctrl Pts',(1.91610786999994,11.6,10.907653233));
#222246=CARTESIAN_POINT('Ctrl Pts',(1.91446333499994,15.2,10.904913665));
#222247=CARTESIAN_POINT('Ctrl Pts',(1.91446333499994,11.6,10.904913665));
#222248=CARTESIAN_POINT('Ctrl Pts',(1.91282364499994,15.2,10.902177181));
#222249=CARTESIAN_POINT('Ctrl Pts',(1.91282364499994,11.6,10.902177181));
#222250=CARTESIAN_POINT('Ctrl Pts',(1.91118879899994,15.2,10.899443792));
#222251=CARTESIAN_POINT('Ctrl Pts',(1.91118879899994,11.6,10.899443792));
#222252=CARTESIAN_POINT('Ctrl Pts',(1.90955879599994,15.2,10.896713509));
#222253=CARTESIAN_POINT('Ctrl Pts',(1.90955879599994,11.6,10.896713509));
#222254=CARTESIAN_POINT('Ctrl Pts',(1.90793363299994,15.2,10.893986344));
#222255=CARTESIAN_POINT('Ctrl Pts',(1.90793363299994,11.6,10.893986344));
#222256=CARTESIAN_POINT('Ctrl Pts',(1.90631331099994,15.2,10.891262308));
#222257=CARTESIAN_POINT('Ctrl Pts',(1.90631331099994,11.6,10.891262308));
#222258=CARTESIAN_POINT('Ctrl Pts',(1.90469782699994,15.2,10.88854141));
#222259=CARTESIAN_POINT('Ctrl Pts',(1.90469782699994,11.6,10.88854141));
#222260=CARTESIAN_POINT('Ctrl Pts',(1.90308717899994,15.2,10.885823664));
#222261=CARTESIAN_POINT('Ctrl Pts',(1.90308717899994,11.6,10.885823664));
#222262=CARTESIAN_POINT('Ctrl Pts',(1.90148136699994,15.2,10.883109081));
#222263=CARTESIAN_POINT('Ctrl Pts',(1.90148136699994,11.6,10.883109081));
#222264=CARTESIAN_POINT('Ctrl Pts',(1.89988038799994,15.2,10.88039767));
#222265=CARTESIAN_POINT('Ctrl Pts',(1.89988038799994,11.6,10.88039767));
#222266=CARTESIAN_POINT('Ctrl Pts',(1.89828424099994,15.2,10.877689446));
#222267=CARTESIAN_POINT('Ctrl Pts',(1.89828424099994,11.6,10.877689446));
#222268=CARTESIAN_POINT('Ctrl Pts',(1.89669292499994,15.2,10.874984418));
#222269=CARTESIAN_POINT('Ctrl Pts',(1.89669292499994,11.6,10.874984418));
#222270=CARTESIAN_POINT('Ctrl Pts',(1.89510643699994,15.2,10.872282598));
#222271=CARTESIAN_POINT('Ctrl Pts',(1.89510643699994,11.6,10.872282598));
#222272=CARTESIAN_POINT('Ctrl Pts',(1.89352477599994,15.2,10.869583997));
#222273=CARTESIAN_POINT('Ctrl Pts',(1.89352477599994,11.6,10.869583997));
#222274=CARTESIAN_POINT('Ctrl Pts',(1.89194794099994,15.2,10.866888628));
#222275=CARTESIAN_POINT('Ctrl Pts',(1.89194794099994,11.6,10.866888628));
#222276=CARTESIAN_POINT('Ctrl Pts',(1.89037592899994,15.2,10.8641965));
#222277=CARTESIAN_POINT('Ctrl Pts',(1.89037592899994,11.6,10.8641965));
#222278=CARTESIAN_POINT('Ctrl Pts',(1.88880873999994,15.2,10.861507627));
#222279=CARTESIAN_POINT('Ctrl Pts',(1.88880873999994,11.6,10.861507627));
#222280=CARTESIAN_POINT('Ctrl Pts',(1.88724637099994,15.2,10.858822018));
#222281=CARTESIAN_POINT('Ctrl Pts',(1.88724637099994,11.6,10.858822018));
#222282=CARTESIAN_POINT('Ctrl Pts',(1.88568882099994,15.2,10.856139687));
#222283=CARTESIAN_POINT('Ctrl Pts',(1.88568882099994,11.6,10.856139687));
#222284=CARTESIAN_POINT('Ctrl Pts',(1.88413608799994,15.2,10.853460645));
#222285=CARTESIAN_POINT('Ctrl Pts',(1.88413608799994,11.6,10.853460645));
#222286=CARTESIAN_POINT('Ctrl Pts',(1.88258817099994,15.2,10.850784902));
#222287=CARTESIAN_POINT('Ctrl Pts',(1.88258817099994,11.6,10.850784902));
#222288=CARTESIAN_POINT('Ctrl Pts',(1.88104506799994,15.2,10.848112472));
#222289=CARTESIAN_POINT('Ctrl Pts',(1.88104506799994,11.6,10.848112472));
#222290=CARTESIAN_POINT('Ctrl Pts',(1.87950677599994,15.2,10.845443365));
#222291=CARTESIAN_POINT('Ctrl Pts',(1.87950677599994,11.6,10.845443365));
#222292=CARTESIAN_POINT('Ctrl Pts',(1.87797329499995,15.2,10.842777593));
#222293=CARTESIAN_POINT('Ctrl Pts',(1.87797329499995,11.6,10.842777593));
#222294=CARTESIAN_POINT('Ctrl Pts',(1.87644462199994,15.2,10.840115168));
#222295=CARTESIAN_POINT('Ctrl Pts',(1.87644462199994,11.6,10.840115168));
#222296=CARTESIAN_POINT('Ctrl Pts',(1.87492075599994,15.2,10.837456102));
#222297=CARTESIAN_POINT('Ctrl Pts',(1.87492075599994,11.6,10.837456102));
#222298=CARTESIAN_POINT('Ctrl Pts',(1.87340169499994,15.2,10.834800405));
#222299=CARTESIAN_POINT('Ctrl Pts',(1.87340169499994,11.6,10.834800405));
#222300=CARTESIAN_POINT('Ctrl Pts',(1.87188743799994,15.2,10.832148092));
#222301=CARTESIAN_POINT('Ctrl Pts',(1.87188743799994,11.6,10.832148092));
#222302=CARTESIAN_POINT('Ctrl Pts',(1.87037798199994,15.2,10.829499171));
#222303=CARTESIAN_POINT('Ctrl Pts',(1.87037798199994,11.6,10.829499171));
#222304=CARTESIAN_POINT('Ctrl Pts',(1.86887332499994,15.2,10.826853657));
#222305=CARTESIAN_POINT('Ctrl Pts',(1.86887332499994,11.6,10.826853657));
#222306=CARTESIAN_POINT('Ctrl Pts',(1.86737346599994,15.2,10.82421156));
#222307=CARTESIAN_POINT('Ctrl Pts',(1.86737346599994,11.6,10.82421156));
#222308=CARTESIAN_POINT('Ctrl Pts',(1.86587840299994,15.2,10.821572892));
#222309=CARTESIAN_POINT('Ctrl Pts',(1.86587840299994,11.6,10.821572892));
#222310=CARTESIAN_POINT('Ctrl Pts',(1.86438813399994,15.2,10.818937667));
#222311=CARTESIAN_POINT('Ctrl Pts',(1.86438813399994,11.6,10.818937667));
#222312=CARTESIAN_POINT('Ctrl Pts',(1.86290265699994,15.2,10.816305893));
#222313=CARTESIAN_POINT('Ctrl Pts',(1.86290265699994,11.6,10.816305893));
#222314=CARTESIAN_POINT('Ctrl Pts',(1.86142197099994,15.2,10.813677587));
#222315=CARTESIAN_POINT('Ctrl Pts',(1.86142197099994,11.6,10.813677587));
#222316=CARTESIAN_POINT('Ctrl Pts',(1.85994607299994,15.2,10.811052756));
#222317=CARTESIAN_POINT('Ctrl Pts',(1.85994607299994,11.6,10.811052756));
#222318=CARTESIAN_POINT('Ctrl Pts',(1.85847496099994,15.2,10.808431415));
#222319=CARTESIAN_POINT('Ctrl Pts',(1.85847496099994,11.6,10.808431415));
#222320=CARTESIAN_POINT('Ctrl Pts',(1.85700863399994,15.2,10.805813575));
#222321=CARTESIAN_POINT('Ctrl Pts',(1.85700863399994,11.6,10.805813575));
#222322=CARTESIAN_POINT('Ctrl Pts',(1.85554708999994,15.2,10.803199249));
#222323=CARTESIAN_POINT('Ctrl Pts',(1.85554708999994,11.6,10.803199249));
#222324=CARTESIAN_POINT('Ctrl Pts',(1.85409032699994,15.2,10.800588447));
#222325=CARTESIAN_POINT('Ctrl Pts',(1.85409032699994,11.6,10.800588447));
#222326=CARTESIAN_POINT('Ctrl Pts',(1.85263834199994,15.2,10.797981184));
#222327=CARTESIAN_POINT('Ctrl Pts',(1.85263834199994,11.6,10.797981184));
#222328=CARTESIAN_POINT('Ctrl Pts',(1.85119113399994,15.2,10.79537747));
#222329=CARTESIAN_POINT('Ctrl Pts',(1.85119113399994,11.6,10.79537747));
#222330=CARTESIAN_POINT('Ctrl Pts',(1.84974869999994,15.2,10.792777317));
#222331=CARTESIAN_POINT('Ctrl Pts',(1.84974869999994,11.6,10.792777317));
#222332=CARTESIAN_POINT('Ctrl Pts',(1.84831103999994,15.2,10.790180739));
#222333=CARTESIAN_POINT('Ctrl Pts',(1.84831103999994,11.6,10.790180739));
#222334=CARTESIAN_POINT('Ctrl Pts',(1.84687814999994,15.2,10.787587747));
#222335=CARTESIAN_POINT('Ctrl Pts',(1.84687814999994,11.6,10.787587747));
#222336=CARTESIAN_POINT('Ctrl Pts',(1.84545002899994,15.2,10.784998353));
#222337=CARTESIAN_POINT('Ctrl Pts',(1.84545002899994,11.6,10.784998353));
#222338=CARTESIAN_POINT('Ctrl Pts',(1.84402667499994,15.2,10.78241257));
#222339=CARTESIAN_POINT('Ctrl Pts',(1.84402667499994,11.6,10.78241257));
#222340=CARTESIAN_POINT('Ctrl Pts',(1.84260808499994,15.2,10.77983041));
#222341=CARTESIAN_POINT('Ctrl Pts',(1.84260808499994,11.6,10.77983041));
#222342=CARTESIAN_POINT('Ctrl Pts',(1.84119425799994,15.2,10.777251886));
#222343=CARTESIAN_POINT('Ctrl Pts',(1.84119425799994,11.6,10.777251886));
#222344=CARTESIAN_POINT('Ctrl Pts',(1.83978518999994,15.2,10.774677008));
#222345=CARTESIAN_POINT('Ctrl Pts',(1.83978518999994,11.6,10.774677008));
#222346=CARTESIAN_POINT('Ctrl Pts',(1.83838088199994,15.2,10.772105791));
#222347=CARTESIAN_POINT('Ctrl Pts',(1.83838088199994,11.6,10.772105791));
#222348=CARTESIAN_POINT('Ctrl Pts',(1.83698132999994,15.2,10.769538246));
#222349=CARTESIAN_POINT('Ctrl Pts',(1.83698132999994,11.6,10.769538246));
#222350=CARTESIAN_POINT('Ctrl Pts',(1.83558653199994,15.2,10.766974385));
#222351=CARTESIAN_POINT('Ctrl Pts',(1.83558653199994,11.6,10.766974385));
#222352=CARTESIAN_POINT('Ctrl Pts',(1.83419648599994,15.2,10.764414223));
#222353=CARTESIAN_POINT('Ctrl Pts',(1.83419648599994,11.6,10.764414223));
#222354=CARTESIAN_POINT('Ctrl Pts',(1.83281118899994,15.2,10.761857769));
#222355=CARTESIAN_POINT('Ctrl Pts',(1.83281118899994,11.6,10.761857769));
#222356=CARTESIAN_POINT('Ctrl Pts',(1.83143063899994,15.2,10.759305039));
#222357=CARTESIAN_POINT('Ctrl Pts',(1.83143063899994,11.6,10.759305039));
#222358=CARTESIAN_POINT('Ctrl Pts',(1.83005483599994,15.2,10.756756044));
#222359=CARTESIAN_POINT('Ctrl Pts',(1.83005483599994,11.6,10.756756044));
#222360=CARTESIAN_POINT('Ctrl Pts',(1.82868377599994,15.2,10.754210794));
#222361=CARTESIAN_POINT('Ctrl Pts',(1.82868377599994,11.6,10.754210794));
#222362=CARTESIAN_POINT('Ctrl Pts',(1.82731745699994,15.2,10.751669306));
#222363=CARTESIAN_POINT('Ctrl Pts',(1.82731745699994,11.6,10.751669306));
#222364=CARTESIAN_POINT('Ctrl Pts',(1.82595587499994,15.2,10.74913159));
#222365=CARTESIAN_POINT('Ctrl Pts',(1.82595587499994,11.6,10.74913159));
#222366=CARTESIAN_POINT('Ctrl Pts',(1.82459903099994,15.2,10.746597659));
#222367=CARTESIAN_POINT('Ctrl Pts',(1.82459903099994,11.6,10.746597659));
#222368=CARTESIAN_POINT('Ctrl Pts',(1.82324692099994,15.2,10.744067525));
#222369=CARTESIAN_POINT('Ctrl Pts',(1.82324692099994,11.6,10.744067525));
#222370=CARTESIAN_POINT('Ctrl Pts',(1.82189954399994,15.2,10.741541203));
#222371=CARTESIAN_POINT('Ctrl Pts',(1.82189954399994,11.6,10.741541203));
#222372=CARTESIAN_POINT('Ctrl Pts',(1.82055689499994,15.2,10.739018704));
#222373=CARTESIAN_POINT('Ctrl Pts',(1.82055689499994,11.6,10.739018704));
#222374=CARTESIAN_POINT('Ctrl Pts',(1.81921897399994,15.2,10.736500041));
#222375=CARTESIAN_POINT('Ctrl Pts',(1.81921897399994,11.6,10.736500041));
#222376=CARTESIAN_POINT('Ctrl Pts',(1.81788577799994,15.2,10.733985226));
#222377=CARTESIAN_POINT('Ctrl Pts',(1.81788577799994,11.6,10.733985226));
#222378=CARTESIAN_POINT('Ctrl Pts',(1.81655730499994,15.2,10.731474274));
#222379=CARTESIAN_POINT('Ctrl Pts',(1.81655730499994,11.6,10.731474274));
#222380=CARTESIAN_POINT('Ctrl Pts',(1.81523355199994,15.2,10.728967196));
#222381=CARTESIAN_POINT('Ctrl Pts',(1.81523355199994,11.6,10.728967196));
#222382=CARTESIAN_POINT('Ctrl Pts',(1.81391451699994,15.2,10.726464006));
#222383=CARTESIAN_POINT('Ctrl Pts',(1.81391451699994,11.6,10.726464006));
#222384=CARTESIAN_POINT('Ctrl Pts',(1.81260019699994,15.2,10.723964716));
#222385=CARTESIAN_POINT('Ctrl Pts',(1.81260019699994,11.6,10.723964716));
#222386=CARTESIAN_POINT('Ctrl Pts',(1.81129059099994,15.2,10.721469338));
#222387=CARTESIAN_POINT('Ctrl Pts',(1.81129059099994,11.6,10.721469338));
#222388=CARTESIAN_POINT('Ctrl Pts',(1.80998569499994,15.2,10.718977888));
#222389=CARTESIAN_POINT('Ctrl Pts',(1.80998569499994,11.6,10.718977888));
#222390=CARTESIAN_POINT('Ctrl Pts',(1.80868550699994,15.2,10.716490376));
#222391=CARTESIAN_POINT('Ctrl Pts',(1.80868550699994,11.6,10.716490376));
#222392=CARTESIAN_POINT('Ctrl Pts',(1.80739002699994,15.2,10.714006816));
#222393=CARTESIAN_POINT('Ctrl Pts',(1.80739002699994,11.6,10.714006816));
#222394=CARTESIAN_POINT('Ctrl Pts',(1.80609924799994,15.2,10.711527222));
#222395=CARTESIAN_POINT('Ctrl Pts',(1.80609924799994,11.6,10.711527222));
#222396=CARTESIAN_POINT('Ctrl Pts',(1.80481317199994,15.2,10.709051607));
#222397=CARTESIAN_POINT('Ctrl Pts',(1.80481317199994,11.6,10.709051607));
#222398=CARTESIAN_POINT('Ctrl Pts',(1.80353179199994,15.2,10.706579983));
#222399=CARTESIAN_POINT('Ctrl Pts',(1.80353179199994,11.6,10.706579983));
#222400=CARTESIAN_POINT('Ctrl Pts',(1.80225510999994,15.2,10.704112364));
#222401=CARTESIAN_POINT('Ctrl Pts',(1.80225510999994,11.6,10.704112364));
#222402=CARTESIAN_POINT('Ctrl Pts',(1.80098311999994,15.2,10.701648763));
#222403=CARTESIAN_POINT('Ctrl Pts',(1.80098311999994,11.6,10.701648763));
#222404=CARTESIAN_POINT('Ctrl Pts',(1.79971582199994,15.2,10.699189192));
#222405=CARTESIAN_POINT('Ctrl Pts',(1.79971582199994,11.6,10.699189192));
#222406=CARTESIAN_POINT('Ctrl Pts',(1.79845321199994,15.2,10.696733665));
#222407=CARTESIAN_POINT('Ctrl Pts',(1.79845321199994,11.6,10.696733665));
#222408=CARTESIAN_POINT('Ctrl Pts',(1.79719528699994,15.2,10.694282197));
#222409=CARTESIAN_POINT('Ctrl Pts',(1.79719528699994,11.6,10.694282197));
#222410=CARTESIAN_POINT('Ctrl Pts',(1.79594204599994,15.2,10.691834799));
#222411=CARTESIAN_POINT('Ctrl Pts',(1.79594204599994,11.6,10.691834799));
#222412=CARTESIAN_POINT('Ctrl Pts',(1.79469348599994,15.2,10.689391486));
#222413=CARTESIAN_POINT('Ctrl Pts',(1.79469348599994,11.6,10.689391486));
#222414=CARTESIAN_POINT('Ctrl Pts',(1.79344960199994,15.2,10.68695227));
#222415=CARTESIAN_POINT('Ctrl Pts',(1.79344960199994,11.6,10.68695227));
#222416=CARTESIAN_POINT('Ctrl Pts',(1.79221039399994,15.2,10.684517164));
#222417=CARTESIAN_POINT('Ctrl Pts',(1.79221039399994,11.6,10.684517164));
#222418=CARTESIAN_POINT('Ctrl Pts',(1.79097585899994,15.2,10.682086184));
#222419=CARTESIAN_POINT('Ctrl Pts',(1.79097585899994,11.6,10.682086184));
#222420=CARTESIAN_POINT('Ctrl Pts',(1.78974599399994,15.2,10.679659341));
#222421=CARTESIAN_POINT('Ctrl Pts',(1.78974599399994,11.6,10.679659341));
#222422=CARTESIAN_POINT('Ctrl Pts',(1.78852079599994,15.2,10.677236649));
#222423=CARTESIAN_POINT('Ctrl Pts',(1.78852079599994,11.6,10.677236649));
#222424=CARTESIAN_POINT('Ctrl Pts',(1.78730026299994,15.2,10.674818122));
#222425=CARTESIAN_POINT('Ctrl Pts',(1.78730026299994,11.6,10.674818122));
#222426=CARTESIAN_POINT('Ctrl Pts',(1.78608439099994,15.2,10.672403774));
#222427=CARTESIAN_POINT('Ctrl Pts',(1.78608439099994,11.6,10.672403774));
#222428=CARTESIAN_POINT('Ctrl Pts',(1.78487317799994,15.2,10.669993618));
#222429=CARTESIAN_POINT('Ctrl Pts',(1.78487317799994,11.6,10.669993618));
#222430=CARTESIAN_POINT('Ctrl Pts',(1.78366662199994,15.2,10.667587667));
#222431=CARTESIAN_POINT('Ctrl Pts',(1.78366662199994,11.6,10.667587667));
#222432=CARTESIAN_POINT('Ctrl Pts',(1.78246471799994,15.2,10.665185936));
#222433=CARTESIAN_POINT('Ctrl Pts',(1.78246471799994,11.6,10.665185936));
#222434=CARTESIAN_POINT('Ctrl Pts',(1.78126746699994,15.2,10.662788437));
#222435=CARTESIAN_POINT('Ctrl Pts',(1.78126746699994,11.6,10.662788437));
#222436=CARTESIAN_POINT('Ctrl Pts',(1.78007486299994,15.2,10.660395185));
#222437=CARTESIAN_POINT('Ctrl Pts',(1.78007486299994,11.6,10.660395185));
#222438=CARTESIAN_POINT('Ctrl Pts',(1.77888690299994,15.2,10.658006193));
#222439=CARTESIAN_POINT('Ctrl Pts',(1.77888690299994,11.6,10.658006193));
#222440=CARTESIAN_POINT('Ctrl Pts',(1.77770358699994,15.2,10.655621476));
#222441=CARTESIAN_POINT('Ctrl Pts',(1.77770358699994,11.6,10.655621476));
#222442=CARTESIAN_POINT('Ctrl Pts',(1.77652490899994,15.2,10.653241047));
#222443=CARTESIAN_POINT('Ctrl Pts',(1.77652490899994,11.6,10.653241047));
#222444=CARTESIAN_POINT('Ctrl Pts',(1.77535086799994,15.2,10.650864921));
#222445=CARTESIAN_POINT('Ctrl Pts',(1.77535086799994,11.6,10.650864921));
#222446=CARTESIAN_POINT('Ctrl Pts',(1.77418146099994,15.2,10.648493109));
#222447=CARTESIAN_POINT('Ctrl Pts',(1.77418146099994,11.6,10.648493109));
#222448=CARTESIAN_POINT('Ctrl Pts',(1.77301668399994,15.2,10.646125627));
#222449=CARTESIAN_POINT('Ctrl Pts',(1.77301668399994,11.6,10.646125627));
#222450=CARTESIAN_POINT('Ctrl Pts',(1.77185653499994,15.2,10.643762489));
#222451=CARTESIAN_POINT('Ctrl Pts',(1.77185653499994,11.6,10.643762489));
#222452=CARTESIAN_POINT('Ctrl Pts',(1.77070101099994,15.2,10.641403709));
#222453=CARTESIAN_POINT('Ctrl Pts',(1.77070101099994,11.6,10.641403709));
#222454=CARTESIAN_POINT('Ctrl Pts',(1.76955010899994,15.2,10.6390493));
#222455=CARTESIAN_POINT('Ctrl Pts',(1.76955010899994,11.6,10.6390493));
#222456=CARTESIAN_POINT('Ctrl Pts',(1.76840382499994,15.2,10.636699276));
#222457=CARTESIAN_POINT('Ctrl Pts',(1.76840382499994,11.6,10.636699276));
#222458=CARTESIAN_POINT('Ctrl Pts',(1.76726215699994,15.2,10.634353653));
#222459=CARTESIAN_POINT('Ctrl Pts',(1.76726215699994,11.6,10.634353653));
#222460=CARTESIAN_POINT('Ctrl Pts',(1.76612510299994,15.2,10.632012444));
#222461=CARTESIAN_POINT('Ctrl Pts',(1.76612510299994,11.6,10.632012444));
#222462=CARTESIAN_POINT('Ctrl Pts',(1.76499265799994,15.2,10.629675662));
#222463=CARTESIAN_POINT('Ctrl Pts',(1.76499265799994,11.6,10.629675662));
#222464=CARTESIAN_POINT('Ctrl Pts',(1.76386481999994,15.2,10.627343324));
#222465=CARTESIAN_POINT('Ctrl Pts',(1.76386481999994,11.6,10.627343324));
#222466=CARTESIAN_POINT('Ctrl Pts',(1.76274158499994,15.2,10.625015441));
#222467=CARTESIAN_POINT('Ctrl Pts',(1.76274158499994,11.6,10.625015441));
#222468=CARTESIAN_POINT('Ctrl Pts',(1.76162295199994,15.2,10.62269203));
#222469=CARTESIAN_POINT('Ctrl Pts',(1.76162295199994,11.6,10.62269203));
#222470=CARTESIAN_POINT('Ctrl Pts',(1.76050891399994,15.2,10.620373104));
#222471=CARTESIAN_POINT('Ctrl Pts',(1.76050891399994,11.6,10.620373104));
#222472=CARTESIAN_POINT('Ctrl Pts',(1.75939947199994,15.2,10.618058677));
#222473=CARTESIAN_POINT('Ctrl Pts',(1.75939947199994,11.6,10.618058677));
#222474=CARTESIAN_POINT('Ctrl Pts',(1.75829462199994,15.2,10.615748764));
#222475=CARTESIAN_POINT('Ctrl Pts',(1.75829462199994,11.6,10.615748764));
#222476=CARTESIAN_POINT('Ctrl Pts',(1.75719435899994,15.2,10.61344338));
#222477=CARTESIAN_POINT('Ctrl Pts',(1.75719435899994,11.6,10.61344338));
#222478=CARTESIAN_POINT('Ctrl Pts',(1.75609867999994,15.2,10.611142538));
#222479=CARTESIAN_POINT('Ctrl Pts',(1.75609867999994,11.6,10.611142538));
#222480=CARTESIAN_POINT('Ctrl Pts',(1.75500758399994,15.2,10.608846253));
#222481=CARTESIAN_POINT('Ctrl Pts',(1.75500758399994,11.6,10.608846253));
#222482=CARTESIAN_POINT('Ctrl Pts',(1.75392106599994,15.2,10.606554541));
#222483=CARTESIAN_POINT('Ctrl Pts',(1.75392106599994,11.6,10.606554541));
#222484=CARTESIAN_POINT('Ctrl Pts',(1.75283912199994,15.2,10.604267413));
#222485=CARTESIAN_POINT('Ctrl Pts',(1.75283912199994,11.6,10.604267413));
#222486=CARTESIAN_POINT('Ctrl Pts',(1.75176175099994,15.2,10.601984888));
#222487=CARTESIAN_POINT('Ctrl Pts',(1.75176175099994,11.6,10.601984888));
#222488=CARTESIAN_POINT('Ctrl Pts',(1.75068894799994,15.2,10.599706978));
#222489=CARTESIAN_POINT('Ctrl Pts',(1.75068894799994,11.6,10.599706978));
#222490=CARTESIAN_POINT('Ctrl Pts',(1.74962071199994,15.2,10.597433698));
#222491=CARTESIAN_POINT('Ctrl Pts',(1.74962071199994,11.6,10.597433698));
#222492=CARTESIAN_POINT('Ctrl Pts',(1.74855703599994,15.2,10.595165063));
#222493=CARTESIAN_POINT('Ctrl Pts',(1.74855703599994,11.6,10.595165063));
#222494=CARTESIAN_POINT('Ctrl Pts',(1.74749791799994,15.2,10.592901088));
#222495=CARTESIAN_POINT('Ctrl Pts',(1.74749791799994,11.6,10.592901088));
#222496=CARTESIAN_POINT('Ctrl Pts',(1.74644335699994,15.2,10.590641787));
#222497=CARTESIAN_POINT('Ctrl Pts',(1.74644335699994,11.6,10.590641787));
#222498=CARTESIAN_POINT('Ctrl Pts',(1.74539334699994,15.2,10.588387175));
#222499=CARTESIAN_POINT('Ctrl Pts',(1.74539334699994,11.6,10.588387175));
#222500=CARTESIAN_POINT('Ctrl Pts',(1.74434788599994,15.2,10.586137268));
#222501=CARTESIAN_POINT('Ctrl Pts',(1.74434788599994,11.6,10.586137268));
#222502=CARTESIAN_POINT('Ctrl Pts',(1.74330696999994,15.2,10.583892079));
#222503=CARTESIAN_POINT('Ctrl Pts',(1.74330696999994,11.6,10.583892079));
#222504=CARTESIAN_POINT('Ctrl Pts',(1.74227059499994,15.2,10.581651625));
#222505=CARTESIAN_POINT('Ctrl Pts',(1.74227059499994,11.6,10.581651625));
#222506=CARTESIAN_POINT('Ctrl Pts',(1.74123875899994,15.2,10.57941592));
#222507=CARTESIAN_POINT('Ctrl Pts',(1.74123875899994,11.6,10.57941592));
#222508=CARTESIAN_POINT('Ctrl Pts',(1.74021145699994,15.2,10.577184979));
#222509=CARTESIAN_POINT('Ctrl Pts',(1.74021145699994,11.6,10.577184979));
#222510=CARTESIAN_POINT('Ctrl Pts',(1.73918868599995,15.2,10.574958817));
#222511=CARTESIAN_POINT('Ctrl Pts',(1.73918868599995,11.6,10.574958817));
#222512=CARTESIAN_POINT('Ctrl Pts',(1.73817044299994,15.2,10.572737449));
#222513=CARTESIAN_POINT('Ctrl Pts',(1.73817044299994,11.6,10.572737449));
#222514=CARTESIAN_POINT('Ctrl Pts',(1.73715672399994,15.2,10.570520891));
#222515=CARTESIAN_POINT('Ctrl Pts',(1.73715672399994,11.6,10.570520891));
#222516=CARTESIAN_POINT('Ctrl Pts',(1.73614752599994,15.2,10.568309157));
#222517=CARTESIAN_POINT('Ctrl Pts',(1.73614752599994,11.6,10.568309157));
#222518=CARTESIAN_POINT('Ctrl Pts',(1.73514284399995,15.2,10.566102263));
#222519=CARTESIAN_POINT('Ctrl Pts',(1.73514284399995,11.6,10.566102263));
#222520=CARTESIAN_POINT('Ctrl Pts',(1.73414267599994,15.2,10.563900224));
#222521=CARTESIAN_POINT('Ctrl Pts',(1.73414267599994,11.6,10.563900224));
#222522=CARTESIAN_POINT('Ctrl Pts',(1.73314701799994,15.2,10.561703055));
#222523=CARTESIAN_POINT('Ctrl Pts',(1.73314701799994,11.6,10.561703055));
#222524=CARTESIAN_POINT('Ctrl Pts',(1.73215586599994,15.2,10.559510772));
#222525=CARTESIAN_POINT('Ctrl Pts',(1.73215586599994,11.6,10.559510772));
#222526=CARTESIAN_POINT('Ctrl Pts',(1.73116921499994,15.2,10.557323391));
#222527=CARTESIAN_POINT('Ctrl Pts',(1.73116921499994,11.6,10.557323391));
#222528=CARTESIAN_POINT('Ctrl Pts',(1.73018706399994,15.2,10.555140925));
#222529=CARTESIAN_POINT('Ctrl Pts',(1.73018706399994,11.6,10.555140925));
#222530=CARTESIAN_POINT('Ctrl Pts',(1.72920940799994,15.2,10.552963392));
#222531=CARTESIAN_POINT('Ctrl Pts',(1.72920940799994,11.6,10.552963392));
#222532=CARTESIAN_POINT('Ctrl Pts',(1.72823624299994,15.2,10.550790806));
#222533=CARTESIAN_POINT('Ctrl Pts',(1.72823624299994,11.6,10.550790806));
#222534=CARTESIAN_POINT('Ctrl Pts',(1.72726756499994,15.2,10.548623183));
#222535=CARTESIAN_POINT('Ctrl Pts',(1.72726756499994,11.6,10.548623183));
#222536=CARTESIAN_POINT('Ctrl Pts',(1.72630337199994,15.2,10.546460539));
#222537=CARTESIAN_POINT('Ctrl Pts',(1.72630337199994,11.6,10.546460539));
#222538=CARTESIAN_POINT('Ctrl Pts',(1.72534365799994,15.2,10.544302888));
#222539=CARTESIAN_POINT('Ctrl Pts',(1.72534365799994,11.6,10.544302888));
#222540=CARTESIAN_POINT('Ctrl Pts',(1.72438841999994,15.2,10.542150249));
#222541=CARTESIAN_POINT('Ctrl Pts',(1.72438841999994,11.6,10.542150249));
#222542=CARTESIAN_POINT('Ctrl Pts',(1.72343765399994,15.2,10.540002635));
#222543=CARTESIAN_POINT('Ctrl Pts',(1.72343765399994,11.6,10.540002635));
#222544=CARTESIAN_POINT('Ctrl Pts',(1.72249135799994,15.2,10.537860062));
#222545=CARTESIAN_POINT('Ctrl Pts',(1.72249135799994,11.6,10.537860062));
#222546=CARTESIAN_POINT('Ctrl Pts',(1.72154952499994,15.2,10.535722546));
#222547=CARTESIAN_POINT('Ctrl Pts',(1.72154952499994,11.6,10.535722546));
#222548=CARTESIAN_POINT('Ctrl Pts',(1.72061215299994,15.2,10.533590105));
#222549=CARTESIAN_POINT('Ctrl Pts',(1.72061215299994,11.6,10.533590105));
#222550=CARTESIAN_POINT('Ctrl Pts',(1.71967923699994,15.2,10.531462751));
#222551=CARTESIAN_POINT('Ctrl Pts',(1.71967923699994,11.6,10.531462751));
#222552=CARTESIAN_POINT('Ctrl Pts',(1.71875077499994,15.2,10.529340503));
#222553=CARTESIAN_POINT('Ctrl Pts',(1.71875077499994,11.6,10.529340503));
#222554=CARTESIAN_POINT('Ctrl Pts',(1.71782676099994,15.2,10.527223377));
#222555=CARTESIAN_POINT('Ctrl Pts',(1.71782676099994,11.6,10.527223377));
#222556=CARTESIAN_POINT('Ctrl Pts',(1.71690719199994,15.2,10.525111386));
#222557=CARTESIAN_POINT('Ctrl Pts',(1.71690719199994,11.6,10.525111386));
#222558=CARTESIAN_POINT('Ctrl Pts',(1.71599206399994,15.2,10.52300455));
#222559=CARTESIAN_POINT('Ctrl Pts',(1.71599206399994,11.6,10.52300455));
#222560=CARTESIAN_POINT('Ctrl Pts',(1.71508137199994,15.2,10.520902882));
#222561=CARTESIAN_POINT('Ctrl Pts',(1.71508137199994,11.6,10.520902882));
#222562=CARTESIAN_POINT('Ctrl Pts',(1.71417511299994,15.2,10.5188064));
#222563=CARTESIAN_POINT('Ctrl Pts',(1.71417511299994,11.6,10.5188064));
#222564=CARTESIAN_POINT('Ctrl Pts',(1.71327328299994,15.2,10.516715119));
#222565=CARTESIAN_POINT('Ctrl Pts',(1.71327328299994,11.6,10.516715119));
#222566=CARTESIAN_POINT('Ctrl Pts',(1.71237587599994,15.2,10.514629057));
#222567=CARTESIAN_POINT('Ctrl Pts',(1.71237587599994,11.6,10.514629057));
#222568=CARTESIAN_POINT('Ctrl Pts',(1.71148289099994,15.2,10.512548229));
#222569=CARTESIAN_POINT('Ctrl Pts',(1.71148289099994,11.6,10.512548229));
#222570=CARTESIAN_POINT('Ctrl Pts',(1.71059432099994,15.2,10.51047265));
#222571=CARTESIAN_POINT('Ctrl Pts',(1.71059432099994,11.6,10.51047265));
#222572=CARTESIAN_POINT('Ctrl Pts',(1.70971016399994,15.2,10.50840234));
#222573=CARTESIAN_POINT('Ctrl Pts',(1.70971016399994,11.6,10.50840234));
#222574=CARTESIAN_POINT('Ctrl Pts',(1.70883041399994,15.2,10.506337312));
#222575=CARTESIAN_POINT('Ctrl Pts',(1.70883041399994,11.6,10.506337312));
#222576=CARTESIAN_POINT('Ctrl Pts',(1.70795506799994,15.2,10.504277585));
#222577=CARTESIAN_POINT('Ctrl Pts',(1.70795506799994,11.6,10.504277585));
#222578=CARTESIAN_POINT('Ctrl Pts',(1.70708411999994,15.2,10.502223173));
#222579=CARTESIAN_POINT('Ctrl Pts',(1.70708411999994,11.6,10.502223173));
#222580=CARTESIAN_POINT('Ctrl Pts',(1.70621756899994,15.2,10.500174096));
#222581=CARTESIAN_POINT('Ctrl Pts',(1.70621756899994,11.6,10.500174096));
#222582=CARTESIAN_POINT('Ctrl Pts',(1.70535540699994,15.2,10.498130368));
#222583=CARTESIAN_POINT('Ctrl Pts',(1.70535540699994,11.6,10.498130368));
#222584=CARTESIAN_POINT('Ctrl Pts',(1.70449763199994,15.2,10.496092007));
#222585=CARTESIAN_POINT('Ctrl Pts',(1.70449763199994,11.6,10.496092007));
#222586=CARTESIAN_POINT('Ctrl Pts',(1.70364423799994,15.2,10.494059028));
#222587=CARTESIAN_POINT('Ctrl Pts',(1.70364423799994,11.6,10.494059028));
#222588=CARTESIAN_POINT('Ctrl Pts',(1.70279522299994,15.2,10.492031449));
#222589=CARTESIAN_POINT('Ctrl Pts',(1.70279522299994,11.6,10.492031449));
#222590=CARTESIAN_POINT('Ctrl Pts',(1.70195057999994,15.2,10.490009287));
#222591=CARTESIAN_POINT('Ctrl Pts',(1.70195057999994,11.6,10.490009287));
#222592=CARTESIAN_POINT('Ctrl Pts',(1.70111030699994,15.2,10.487992559));
#222593=CARTESIAN_POINT('Ctrl Pts',(1.70111030699994,11.6,10.487992559));
#222594=CARTESIAN_POINT('Ctrl Pts',(1.70027439799994,15.2,10.485981282));
#222595=CARTESIAN_POINT('Ctrl Pts',(1.70027439799994,11.6,10.485981282));
#222596=CARTESIAN_POINT('Ctrl Pts',(1.69944284799994,15.2,10.483975472));
#222597=CARTESIAN_POINT('Ctrl Pts',(1.69944284799994,11.6,10.483975472));
#222598=CARTESIAN_POINT('Ctrl Pts',(1.69861565399994,15.2,10.481975147));
#222599=CARTESIAN_POINT('Ctrl Pts',(1.69861565399994,11.6,10.481975147));
#222600=CARTESIAN_POINT('Ctrl Pts',(1.69779281099994,15.2,10.479980323));
#222601=CARTESIAN_POINT('Ctrl Pts',(1.69779281099994,11.6,10.479980323));
#222602=CARTESIAN_POINT('Ctrl Pts',(1.69697431399994,15.2,10.477991018));
#222603=CARTESIAN_POINT('Ctrl Pts',(1.69697431399994,11.6,10.477991018));
#222604=CARTESIAN_POINT('Ctrl Pts',(1.69616015899994,15.2,10.47600725));
#222605=CARTESIAN_POINT('Ctrl Pts',(1.69616015899994,11.6,10.47600725));
#222606=CARTESIAN_POINT('Ctrl Pts',(1.69535033999994,15.2,10.474029035));
#222607=CARTESIAN_POINT('Ctrl Pts',(1.69535033999994,11.6,10.474029035));
#222608=CARTESIAN_POINT('Ctrl Pts',(1.69454485499994,15.2,10.472056389));
#222609=CARTESIAN_POINT('Ctrl Pts',(1.69454485499994,11.6,10.472056389));
#222610=CARTESIAN_POINT('Ctrl Pts',(1.69374369599994,15.2,10.470089333));
#222611=CARTESIAN_POINT('Ctrl Pts',(1.69374369599994,11.6,10.470089333));
#222612=CARTESIAN_POINT('Ctrl Pts',(1.69294686199994,15.2,10.468127882));
#222613=CARTESIAN_POINT('Ctrl Pts',(1.69294686199994,11.6,10.468127882));
#222614=CARTESIAN_POINT('Ctrl Pts',(1.69215434499994,15.2,10.466172053));
#222615=CARTESIAN_POINT('Ctrl Pts',(1.69215434499994,11.6,10.466172053));
#222616=CARTESIAN_POINT('Ctrl Pts',(1.69136614299994,15.2,10.464221864));
#222617=CARTESIAN_POINT('Ctrl Pts',(1.69136614299994,11.6,10.464221864));
#222618=CARTESIAN_POINT('Ctrl Pts',(1.69058224899994,15.2,10.462277333));
#222619=CARTESIAN_POINT('Ctrl Pts',(1.69058224899994,11.6,10.462277333));
#222620=CARTESIAN_POINT('Ctrl Pts',(1.68980265899994,15.2,10.460338478));
#222621=CARTESIAN_POINT('Ctrl Pts',(1.68980265899994,11.6,10.460338478));
#222622=CARTESIAN_POINT('Ctrl Pts',(1.68902736899994,15.2,10.458405317));
#222623=CARTESIAN_POINT('Ctrl Pts',(1.68902736899994,11.6,10.458405317));
#222624=CARTESIAN_POINT('Ctrl Pts',(1.68825637199994,15.2,10.456477865));
#222625=CARTESIAN_POINT('Ctrl Pts',(1.68825637199994,11.6,10.456477865));
#222626=CARTESIAN_POINT('Ctrl Pts',(1.68748966599994,15.2,10.454556143));
#222627=CARTESIAN_POINT('Ctrl Pts',(1.68748966599994,11.6,10.454556143));
#222628=CARTESIAN_POINT('Ctrl Pts',(1.68672724499994,15.2,10.452640167));
#222629=CARTESIAN_POINT('Ctrl Pts',(1.68672724499994,11.6,10.452640167));
#222630=CARTESIAN_POINT('Ctrl Pts',(1.68596910199994,15.2,10.450729955));
#222631=CARTESIAN_POINT('Ctrl Pts',(1.68596910199994,11.6,10.450729955));
#222632=CARTESIAN_POINT('Ctrl Pts',(1.68521523599995,15.2,10.448825525));
#222633=CARTESIAN_POINT('Ctrl Pts',(1.68521523599995,11.6,10.448825525));
#222634=CARTESIAN_POINT('Ctrl Pts',(1.68446563799994,15.2,10.446926895));
#222635=CARTESIAN_POINT('Ctrl Pts',(1.68446563799994,11.6,10.446926895));
#222636=CARTESIAN_POINT('Ctrl Pts',(1.68372030499994,15.2,10.445034085));
#222637=CARTESIAN_POINT('Ctrl Pts',(1.68372030499994,11.6,10.445034085));
#222638=CARTESIAN_POINT('Ctrl Pts',(1.68297923299994,15.2,10.44314711));
#222639=CARTESIAN_POINT('Ctrl Pts',(1.68297923299994,11.6,10.44314711));
#222640=CARTESIAN_POINT('Ctrl Pts',(1.68224241499994,15.2,10.44126599));
#222641=CARTESIAN_POINT('Ctrl Pts',(1.68224241499994,11.6,10.44126599));
#222642=CARTESIAN_POINT('Ctrl Pts',(1.68150984699994,15.2,10.439390743));
#222643=CARTESIAN_POINT('Ctrl Pts',(1.68150984699994,11.6,10.439390743));
#222644=CARTESIAN_POINT('Ctrl Pts',(1.68078152299994,15.2,10.437521387));
#222645=CARTESIAN_POINT('Ctrl Pts',(1.68078152299994,11.6,10.437521387));
#222646=CARTESIAN_POINT('Ctrl Pts',(1.68005743899994,15.2,10.43565794));
#222647=CARTESIAN_POINT('Ctrl Pts',(1.68005743899994,11.6,10.43565794));
#222648=CARTESIAN_POINT('Ctrl Pts',(1.67933758799994,15.2,10.433800421));
#222649=CARTESIAN_POINT('Ctrl Pts',(1.67933758799994,11.6,10.433800421));
#222650=CARTESIAN_POINT('Ctrl Pts',(1.67862196699994,15.2,10.431948848));
#222651=CARTESIAN_POINT('Ctrl Pts',(1.67862196699994,11.6,10.431948848));
#222652=CARTESIAN_POINT('Ctrl Pts',(1.67791056899994,15.2,10.43010324));
#222653=CARTESIAN_POINT('Ctrl Pts',(1.67791056899994,11.6,10.43010324));
#222654=CARTESIAN_POINT('Ctrl Pts',(1.67720338999994,15.2,10.428263616));
#222655=CARTESIAN_POINT('Ctrl Pts',(1.67720338999994,11.6,10.428263616));
#222656=CARTESIAN_POINT('Ctrl Pts',(1.67650042399994,15.2,10.426429993));
#222657=CARTESIAN_POINT('Ctrl Pts',(1.67650042399994,11.6,10.426429993));
#222658=CARTESIAN_POINT('Ctrl Pts',(1.67580166599994,15.2,10.424602391));
#222659=CARTESIAN_POINT('Ctrl Pts',(1.67580166599994,11.6,10.424602391));
#222660=CARTESIAN_POINT('Ctrl Pts',(1.67510710999994,15.2,10.422780829));
#222661=CARTESIAN_POINT('Ctrl Pts',(1.67510710999994,11.6,10.422780829));
#222662=CARTESIAN_POINT('Ctrl Pts',(1.67441675199994,15.2,10.420965325));
#222663=CARTESIAN_POINT('Ctrl Pts',(1.67441675199994,11.6,10.420965325));
#222664=CARTESIAN_POINT('Ctrl Pts',(1.67373058499994,15.2,10.419155898));
#222665=CARTESIAN_POINT('Ctrl Pts',(1.67373058499994,11.6,10.419155898));
#222666=CARTESIAN_POINT('Ctrl Pts',(1.67304860399994,15.2,10.417352566));
#222667=CARTESIAN_POINT('Ctrl Pts',(1.67304860399994,11.6,10.417352566));
#222668=CARTESIAN_POINT('Ctrl Pts',(1.67237080499994,15.2,10.41555535));
#222669=CARTESIAN_POINT('Ctrl Pts',(1.67237080499994,11.6,10.41555535));
#222670=CARTESIAN_POINT('Ctrl Pts',(1.67169717899994,15.2,10.413764268));
#222671=CARTESIAN_POINT('Ctrl Pts',(1.67169717899994,11.6,10.413764268));
#222672=CARTESIAN_POINT('Ctrl Pts',(1.67102772499994,15.2,10.41197934));
#222673=CARTESIAN_POINT('Ctrl Pts',(1.67102772499994,11.6,10.41197934));
#222674=CARTESIAN_POINT('Ctrl Pts',(1.67036243399994,15.2,10.410200583));
#222675=CARTESIAN_POINT('Ctrl Pts',(1.67036243399994,11.6,10.410200583));
#222676=CARTESIAN_POINT('Ctrl Pts',(1.66970130199994,15.2,10.408428019));
#222677=CARTESIAN_POINT('Ctrl Pts',(1.66970130199994,11.6,10.408428019));
#222678=CARTESIAN_POINT('Ctrl Pts',(1.66904432199994,15.2,10.406661665));
#222679=CARTESIAN_POINT('Ctrl Pts',(1.66904432199994,11.6,10.406661665));
#222680=CARTESIAN_POINT('Ctrl Pts',(1.66839148999994,15.2,10.404901541));
#222681=CARTESIAN_POINT('Ctrl Pts',(1.66839148999994,11.6,10.404901541));
#222682=CARTESIAN_POINT('Ctrl Pts',(1.66774279899994,15.2,10.403147668));
#222683=CARTESIAN_POINT('Ctrl Pts',(1.66774279899994,11.6,10.403147668));
#222684=CARTESIAN_POINT('Ctrl Pts',(1.66709824499994,15.2,10.401400063));
#222685=CARTESIAN_POINT('Ctrl Pts',(1.66709824499994,11.6,10.401400063));
#222686=CARTESIAN_POINT('Ctrl Pts',(1.66645781999994,15.2,10.399658748));
#222687=CARTESIAN_POINT('Ctrl Pts',(1.66645781999994,11.6,10.399658748));
#222688=CARTESIAN_POINT('Ctrl Pts',(1.66582151999994,15.2,10.397923741));
#222689=CARTESIAN_POINT('Ctrl Pts',(1.66582151999994,11.6,10.397923741));
#222690=CARTESIAN_POINT('Ctrl Pts',(1.66518933799994,15.2,10.396195062));
#222691=CARTESIAN_POINT('Ctrl Pts',(1.66518933799994,11.6,10.396195062));
#222692=CARTESIAN_POINT('Ctrl Pts',(1.66456126799994,15.2,10.394472732));
#222693=CARTESIAN_POINT('Ctrl Pts',(1.66456126799994,11.6,10.394472732));
#222694=CARTESIAN_POINT('Ctrl Pts',(1.66393730499994,15.2,10.392756769));
#222695=CARTESIAN_POINT('Ctrl Pts',(1.66393730499994,11.6,10.392756769));
#222696=CARTESIAN_POINT('Ctrl Pts',(1.66331744299994,15.2,10.391047193));
#222697=CARTESIAN_POINT('Ctrl Pts',(1.66331744299994,11.6,10.391047193));
#222698=CARTESIAN_POINT('Ctrl Pts',(1.66270167599994,15.2,10.389344026));
#222699=CARTESIAN_POINT('Ctrl Pts',(1.66270167599994,11.6,10.389344026));
#222700=CARTESIAN_POINT('Ctrl Pts',(1.66208999699994,15.2,10.387647286));
#222701=CARTESIAN_POINT('Ctrl Pts',(1.66208999699994,11.6,10.387647286));
#222702=CARTESIAN_POINT('Ctrl Pts',(1.66148240099994,15.2,10.385956994));
#222703=CARTESIAN_POINT('Ctrl Pts',(1.66148240099994,11.6,10.385956994));
#222704=CARTESIAN_POINT('Ctrl Pts',(1.66087888199994,15.2,10.384273171));
#222705=CARTESIAN_POINT('Ctrl Pts',(1.66087888199994,11.6,10.384273171));
#222706=CARTESIAN_POINT('Ctrl Pts',(1.66027943499994,15.2,10.382595835));
#222707=CARTESIAN_POINT('Ctrl Pts',(1.66027943499994,11.6,10.382595835));
#222708=CARTESIAN_POINT('Ctrl Pts',(1.65968404999994,15.2,10.380925008));
#222709=CARTESIAN_POINT('Ctrl Pts',(1.65968404999994,11.6,10.380925008));
#222710=CARTESIAN_POINT('Ctrl Pts',(1.65909272599994,15.2,10.37926071));
#222711=CARTESIAN_POINT('Ctrl Pts',(1.65909272599994,11.6,10.37926071));
#222712=CARTESIAN_POINT('Ctrl Pts',(1.65850545199994,15.2,10.377602961));
#222713=CARTESIAN_POINT('Ctrl Pts',(1.65850545199994,11.6,10.377602961));
#222714=CARTESIAN_POINT('Ctrl Pts',(1.65792222399994,15.2,10.375951783));
#222715=CARTESIAN_POINT('Ctrl Pts',(1.65792222399994,11.6,10.375951783));
#222716=CARTESIAN_POINT('Ctrl Pts',(1.65734303699994,15.2,10.374307195));
#222717=CARTESIAN_POINT('Ctrl Pts',(1.65734303699994,11.6,10.374307195));
#222718=CARTESIAN_POINT('Ctrl Pts',(1.65676788199994,15.2,10.372669218));
#222719=CARTESIAN_POINT('Ctrl Pts',(1.65676788199994,11.6,10.372669218));
#222720=CARTESIAN_POINT('Ctrl Pts',(1.65619675499994,15.2,10.371037874));
#222721=CARTESIAN_POINT('Ctrl Pts',(1.65619675499994,11.6,10.371037874));
#222722=CARTESIAN_POINT('Ctrl Pts',(1.65562964799994,15.2,10.369413182));
#222723=CARTESIAN_POINT('Ctrl Pts',(1.65562964799994,11.6,10.369413182));
#222724=CARTESIAN_POINT('Ctrl Pts',(1.65506655599994,15.2,10.367795164));
#222725=CARTESIAN_POINT('Ctrl Pts',(1.65506655599994,11.6,10.367795164));
#222726=CARTESIAN_POINT('Ctrl Pts',(1.65450747099994,15.2,10.366183841));
#222727=CARTESIAN_POINT('Ctrl Pts',(1.65450747099994,11.6,10.366183841));
#222728=CARTESIAN_POINT('Ctrl Pts',(1.65395238799994,15.2,10.364579233));
#222729=CARTESIAN_POINT('Ctrl Pts',(1.65395238799994,11.6,10.364579233));
#222730=CARTESIAN_POINT('Ctrl Pts',(1.65340129899994,15.2,10.362981363));
#222731=CARTESIAN_POINT('Ctrl Pts',(1.65340129899994,11.6,10.362981363));
#222732=CARTESIAN_POINT('Ctrl Pts',(1.65285419799994,15.2,10.36139025));
#222733=CARTESIAN_POINT('Ctrl Pts',(1.65285419799994,11.6,10.36139025));
#222734=CARTESIAN_POINT('Ctrl Pts',(1.65231107899994,15.2,10.359805917));
#222735=CARTESIAN_POINT('Ctrl Pts',(1.65231107899994,11.6,10.359805917));
#222736=CARTESIAN_POINT('Ctrl Pts',(1.65177193599994,15.2,10.358228384));
#222737=CARTESIAN_POINT('Ctrl Pts',(1.65177193599994,11.6,10.358228384));
#222738=CARTESIAN_POINT('Ctrl Pts',(1.65123676099994,15.2,10.356657674));
#222739=CARTESIAN_POINT('Ctrl Pts',(1.65123676099994,11.6,10.356657674));
#222740=CARTESIAN_POINT('Ctrl Pts',(1.65070554599994,15.2,10.355093807));
#222741=CARTESIAN_POINT('Ctrl Pts',(1.65070554599994,11.6,10.355093807));
#222742=CARTESIAN_POINT('Ctrl Pts',(1.65017828699994,15.2,10.353536806));
#222743=CARTESIAN_POINT('Ctrl Pts',(1.65017828699994,11.6,10.353536806));
#222744=CARTESIAN_POINT('Ctrl Pts',(1.64965497699994,15.2,10.351986692));
#222745=CARTESIAN_POINT('Ctrl Pts',(1.64965497699994,11.6,10.351986692));
#222746=CARTESIAN_POINT('Ctrl Pts',(1.64913560699994,15.2,10.350443486));
#222747=CARTESIAN_POINT('Ctrl Pts',(1.64913560699994,11.6,10.350443486));
#222748=CARTESIAN_POINT('Ctrl Pts',(1.64862017199994,15.2,10.348907211));
#222749=CARTESIAN_POINT('Ctrl Pts',(1.64862017199994,11.6,10.348907211));
#222750=CARTESIAN_POINT('Ctrl Pts',(1.64810866499994,15.2,10.347377888));
#222751=CARTESIAN_POINT('Ctrl Pts',(1.64810866499994,11.6,10.347377888));
#222752=CARTESIAN_POINT('Ctrl Pts',(1.64760107699994,15.2,10.34585554));
#222753=CARTESIAN_POINT('Ctrl Pts',(1.64760107699994,11.6,10.34585554));
#222754=CARTESIAN_POINT('Ctrl Pts',(1.64709740399994,15.2,10.344340188));
#222755=CARTESIAN_POINT('Ctrl Pts',(1.64709740399994,11.6,10.344340188));
#222756=CARTESIAN_POINT('Ctrl Pts',(1.64659763699994,15.2,10.342831855));
#222757=CARTESIAN_POINT('Ctrl Pts',(1.64659763699994,11.6,10.342831855));
#222758=CARTESIAN_POINT('Ctrl Pts',(1.64610176899994,15.2,10.341330562));
#222759=CARTESIAN_POINT('Ctrl Pts',(1.64610176899994,11.6,10.341330562));
#222760=CARTESIAN_POINT('Ctrl Pts',(1.64560979399994,15.2,10.339836333));
#222761=CARTESIAN_POINT('Ctrl Pts',(1.64560979399994,11.6,10.339836333));
#222762=CARTESIAN_POINT('Ctrl Pts',(1.64512170499994,15.2,10.33834919));
#222763=CARTESIAN_POINT('Ctrl Pts',(1.64512170499994,11.6,10.33834919));
#222764=CARTESIAN_POINT('Ctrl Pts',(1.64463749299994,15.2,10.336869155));
#222765=CARTESIAN_POINT('Ctrl Pts',(1.64463749299994,11.6,10.336869155));
#222766=CARTESIAN_POINT('Ctrl Pts',(1.64415715199994,15.2,10.335396249));
#222767=CARTESIAN_POINT('Ctrl Pts',(1.64415715199994,11.6,10.335396249));
#222768=CARTESIAN_POINT('Ctrl Pts',(1.64368067599994,15.2,10.333930498));
#222769=CARTESIAN_POINT('Ctrl Pts',(1.64368067599994,11.6,10.333930498));
#222770=CARTESIAN_POINT('Ctrl Pts',(1.64320805499994,15.2,10.332471923));
#222771=CARTESIAN_POINT('Ctrl Pts',(1.64320805499994,11.6,10.332471923));
#222772=CARTESIAN_POINT('Ctrl Pts',(1.64273928299994,15.2,10.331020546));
#222773=CARTESIAN_POINT('Ctrl Pts',(1.64273928299994,11.6,10.331020546));
#222774=CARTESIAN_POINT('Ctrl Pts',(1.64227435299994,15.2,10.329576392));
#222775=CARTESIAN_POINT('Ctrl Pts',(1.64227435299994,11.6,10.329576392));
#222776=CARTESIAN_POINT('Ctrl Pts',(1.64181325799994,15.2,10.328139482));
#222777=CARTESIAN_POINT('Ctrl Pts',(1.64181325799994,11.6,10.328139482));
#222778=CARTESIAN_POINT('Ctrl Pts',(1.64135598799994,15.2,10.32670984));
#222779=CARTESIAN_POINT('Ctrl Pts',(1.64135598799994,11.6,10.32670984));
#222780=CARTESIAN_POINT('Ctrl Pts',(1.64090253799994,15.2,10.32528749));
#222781=CARTESIAN_POINT('Ctrl Pts',(1.64090253799994,11.6,10.32528749));
#222782=CARTESIAN_POINT('Ctrl Pts',(1.64045289999994,15.2,10.323872453));
#222783=CARTESIAN_POINT('Ctrl Pts',(1.64045289999994,11.6,10.323872453));
#222784=CARTESIAN_POINT('Ctrl Pts',(1.64000706499994,15.2,10.322464755));
#222785=CARTESIAN_POINT('Ctrl Pts',(1.64000706499994,11.6,10.322464755));
#222786=CARTESIAN_POINT('Ctrl Pts',(1.63956502699994,15.2,10.321064418));
#222787=CARTESIAN_POINT('Ctrl Pts',(1.63956502699994,11.6,10.321064418));
#222788=CARTESIAN_POINT('Ctrl Pts',(1.63912677699994,15.2,10.319671465));
#222789=CARTESIAN_POINT('Ctrl Pts',(1.63912677699994,11.6,10.319671465));
#222790=CARTESIAN_POINT('Ctrl Pts',(1.63869230999994,15.2,10.318285922));
#222791=CARTESIAN_POINT('Ctrl Pts',(1.63869230999994,11.6,10.318285922));
#222792=CARTESIAN_POINT('Ctrl Pts',(1.63826161399994,15.2,10.31690781));
#222793=CARTESIAN_POINT('Ctrl Pts',(1.63826161399994,11.6,10.31690781));
#222794=CARTESIAN_POINT('Ctrl Pts',(1.63783468399994,15.2,10.315537154));
#222795=CARTESIAN_POINT('Ctrl Pts',(1.63783468399994,11.6,10.315537154));
#222796=CARTESIAN_POINT('Ctrl Pts',(1.63741151199994,15.2,10.314173979));
#222797=CARTESIAN_POINT('Ctrl Pts',(1.63741151199994,11.6,10.314173979));
#222798=CARTESIAN_POINT('Ctrl Pts',(1.63699208899994,15.2,10.312818307));
#222799=CARTESIAN_POINT('Ctrl Pts',(1.63699208899994,11.6,10.312818307));
#222800=CARTESIAN_POINT('Ctrl Pts',(1.63657640799994,15.2,10.311470163));
#222801=CARTESIAN_POINT('Ctrl Pts',(1.63657640799994,11.6,10.311470163));
#222802=CARTESIAN_POINT('Ctrl Pts',(1.63616445999994,15.2,10.310129573));
#222803=CARTESIAN_POINT('Ctrl Pts',(1.63616445999994,11.6,10.310129573));
#222804=CARTESIAN_POINT('Ctrl Pts',(1.63575623799994,15.2,10.308796559));
#222805=CARTESIAN_POINT('Ctrl Pts',(1.63575623799994,11.6,10.308796559));
#222806=CARTESIAN_POINT('Ctrl Pts',(1.63535173399994,15.2,10.307471145));
#222807=CARTESIAN_POINT('Ctrl Pts',(1.63535173399994,11.6,10.307471145));
#222808=CARTESIAN_POINT('Ctrl Pts',(1.63495093799994,15.2,10.306153357));
#222809=CARTESIAN_POINT('Ctrl Pts',(1.63495093799994,11.6,10.306153357));
#222810=CARTESIAN_POINT('Ctrl Pts',(1.63455384399994,15.2,10.30484322));
#222811=CARTESIAN_POINT('Ctrl Pts',(1.63455384399994,11.6,10.30484322));
#222812=CARTESIAN_POINT('Ctrl Pts',(1.63416044299994,15.2,10.303540758));
#222813=CARTESIAN_POINT('Ctrl Pts',(1.63416044299994,11.6,10.303540758));
#222814=CARTESIAN_POINT('Ctrl Pts',(1.63377072599994,15.2,10.302245995));
#222815=CARTESIAN_POINT('Ctrl Pts',(1.63377072599994,11.6,10.302245995));
#222816=CARTESIAN_POINT('Ctrl Pts',(1.63338468399994,15.2,10.300958957));
#222817=CARTESIAN_POINT('Ctrl Pts',(1.63338468399994,11.6,10.300958957));
#222818=CARTESIAN_POINT('Ctrl Pts',(1.63300231199994,15.2,10.299679669));
#222819=CARTESIAN_POINT('Ctrl Pts',(1.63300231199994,11.6,10.299679669));
#222820=CARTESIAN_POINT('Ctrl Pts',(1.63262359899994,15.2,10.298408156));
#222821=CARTESIAN_POINT('Ctrl Pts',(1.63262359899994,11.6,10.298408156));
#222822=CARTESIAN_POINT('Ctrl Pts',(1.63224853599994,15.2,10.297144443));
#222823=CARTESIAN_POINT('Ctrl Pts',(1.63224853599994,11.6,10.297144443));
#222824=CARTESIAN_POINT('Ctrl Pts',(1.63187711599994,15.2,10.295888555));
#222825=CARTESIAN_POINT('Ctrl Pts',(1.63187711599994,11.6,10.295888555));
#222826=CARTESIAN_POINT('Ctrl Pts',(1.63150932899994,15.2,10.294640518));
#222827=CARTESIAN_POINT('Ctrl Pts',(1.63150932899994,11.6,10.294640518));
#222828=CARTESIAN_POINT('Ctrl Pts',(1.63114516899994,15.2,10.293400358));
#222829=CARTESIAN_POINT('Ctrl Pts',(1.63114516899994,11.6,10.293400358));
#222830=CARTESIAN_POINT('Ctrl Pts',(1.63078462299994,15.2,10.292168099));
#222831=CARTESIAN_POINT('Ctrl Pts',(1.63078462299994,11.6,10.292168099));
#222832=CARTESIAN_POINT('Ctrl Pts',(1.63042768599994,15.2,10.290943769));
#222833=CARTESIAN_POINT('Ctrl Pts',(1.63042768599994,11.6,10.290943769));
#222834=CARTESIAN_POINT('Ctrl Pts',(1.63007434799994,15.2,10.289727393));
#222835=CARTESIAN_POINT('Ctrl Pts',(1.63007434799994,11.6,10.289727393));
#222836=CARTESIAN_POINT('Ctrl Pts',(1.62972459999994,15.2,10.288518995));
#222837=CARTESIAN_POINT('Ctrl Pts',(1.62972459999994,11.6,10.288518995));
#222838=CARTESIAN_POINT('Ctrl Pts',(1.62937843299995,15.2,10.287318605));
#222839=CARTESIAN_POINT('Ctrl Pts',(1.62937843299995,11.6,10.287318605));
#222840=CARTESIAN_POINT('Ctrl Pts',(1.62903583799994,15.2,10.286126245));
#222841=CARTESIAN_POINT('Ctrl Pts',(1.62903583799994,11.6,10.286126245));
#222842=CARTESIAN_POINT('Ctrl Pts',(1.62869680599994,15.2,10.284941946));
#222843=CARTESIAN_POINT('Ctrl Pts',(1.62869680599994,11.6,10.284941946));
#222844=CARTESIAN_POINT('Ctrl Pts',(1.62836132899994,15.2,10.28376573));
#222845=CARTESIAN_POINT('Ctrl Pts',(1.62836132899994,11.6,10.28376573));
#222846=CARTESIAN_POINT('Ctrl Pts',(1.62802939799994,15.2,10.282597626));
#222847=CARTESIAN_POINT('Ctrl Pts',(1.62802939799994,11.6,10.282597626));
#222848=CARTESIAN_POINT('Ctrl Pts',(1.62770099999994,15.2,10.28143766));
#222849=CARTESIAN_POINT('Ctrl Pts',(1.62770099999994,11.6,10.28143766));
#222850=CARTESIAN_POINT('Ctrl Pts',(1.62737613099994,15.2,10.280285859));
#222851=CARTESIAN_POINT('Ctrl Pts',(1.62737613099994,11.6,10.280285859));
#222852=CARTESIAN_POINT('Ctrl Pts',(1.62705477799994,15.2,10.279142249));
#222853=CARTESIAN_POINT('Ctrl Pts',(1.62705477799994,11.6,10.279142249));
#222854=CARTESIAN_POINT('Ctrl Pts',(1.62673693399994,15.2,10.278006859));
#222855=CARTESIAN_POINT('Ctrl Pts',(1.62673693399994,11.6,10.278006859));
#222856=CARTESIAN_POINT('Ctrl Pts',(1.62642258799994,15.2,10.276879714));
#222857=CARTESIAN_POINT('Ctrl Pts',(1.62642258799994,11.6,10.276879714));
#222858=CARTESIAN_POINT('Ctrl Pts',(1.62611173199994,15.2,10.275760843));
#222859=CARTESIAN_POINT('Ctrl Pts',(1.62611173199994,11.6,10.275760843));
#222860=CARTESIAN_POINT('Ctrl Pts',(1.62580435499994,15.2,10.274650272));
#222861=CARTESIAN_POINT('Ctrl Pts',(1.62580435499994,11.6,10.274650272));
#222862=CARTESIAN_POINT('Ctrl Pts',(1.62550044799994,15.2,10.27354803));
#222863=CARTESIAN_POINT('Ctrl Pts',(1.62550044799994,11.6,10.27354803));
#222864=CARTESIAN_POINT('Ctrl Pts',(1.62520000299994,15.2,10.272454143));
#222865=CARTESIAN_POINT('Ctrl Pts',(1.62520000299994,11.6,10.272454143));
#222866=CARTESIAN_POINT('Ctrl Pts',(1.62490300799994,15.2,10.27136864));
#222867=CARTESIAN_POINT('Ctrl Pts',(1.62490300799994,11.6,10.27136864));
#222868=CARTESIAN_POINT('Ctrl Pts',(1.62460945299994,15.2,10.270291547));
#222869=CARTESIAN_POINT('Ctrl Pts',(1.62460945299994,11.6,10.270291547));
#222870=CARTESIAN_POINT('Ctrl Pts',(1.62431932999994,15.2,10.269222896));
#222871=CARTESIAN_POINT('Ctrl Pts',(1.62431932999994,11.6,10.269222896));
#222872=CARTESIAN_POINT('Ctrl Pts',(1.62403262999994,15.2,10.268162711));
#222873=CARTESIAN_POINT('Ctrl Pts',(1.62403262999994,11.6,10.268162711));
#222874=CARTESIAN_POINT('Ctrl Pts',(1.62374933999994,15.2,10.267111022));
#222875=CARTESIAN_POINT('Ctrl Pts',(1.62374933999994,11.6,10.267111022));
#222876=CARTESIAN_POINT('Ctrl Pts',(1.62346945199994,15.2,10.266067857));
#222877=CARTESIAN_POINT('Ctrl Pts',(1.62346945199994,11.6,10.266067857));
#222878=CARTESIAN_POINT('Ctrl Pts',(1.62319295499994,15.2,10.265033245));
#222879=CARTESIAN_POINT('Ctrl Pts',(1.62319295499994,11.6,10.265033245));
#222880=CARTESIAN_POINT('Ctrl Pts',(1.62291983999994,15.2,10.264007215));
#222881=CARTESIAN_POINT('Ctrl Pts',(1.62291983999994,11.6,10.264007215));
#222882=CARTESIAN_POINT('Ctrl Pts',(1.62265009699994,15.2,10.262989795));
#222883=CARTESIAN_POINT('Ctrl Pts',(1.62265009699994,11.6,10.262989795));
#222884=CARTESIAN_POINT('Ctrl Pts',(1.62238371499994,15.2,10.261981014));
#222885=CARTESIAN_POINT('Ctrl Pts',(1.62238371499994,11.6,10.261981014));
#222886=CARTESIAN_POINT('Ctrl Pts',(1.62212068299994,15.2,10.2609809));
#222887=CARTESIAN_POINT('Ctrl Pts',(1.62212068299994,11.6,10.2609809));
#222888=CARTESIAN_POINT('Ctrl Pts',(1.62186099299995,15.2,10.259989485));
#222889=CARTESIAN_POINT('Ctrl Pts',(1.62186099299995,11.6,10.259989485));
#222890=CARTESIAN_POINT('Ctrl Pts',(1.62160463199994,15.2,10.259006796));
#222891=CARTESIAN_POINT('Ctrl Pts',(1.62160463199994,11.6,10.259006796));
#222892=CARTESIAN_POINT('Ctrl Pts',(1.62135158999994,15.2,10.258032864));
#222893=CARTESIAN_POINT('Ctrl Pts',(1.62135158999994,11.6,10.258032864));
#222894=CARTESIAN_POINT('Ctrl Pts',(1.62110185799994,15.2,10.257067718));
#222895=CARTESIAN_POINT('Ctrl Pts',(1.62110185799994,11.6,10.257067718));
#222896=CARTESIAN_POINT('Ctrl Pts',(1.62085542399994,15.2,10.256111387));
#222897=CARTESIAN_POINT('Ctrl Pts',(1.62085542399994,11.6,10.256111387));
#222898=CARTESIAN_POINT('Ctrl Pts',(1.62061227799994,15.2,10.2551639));
#222899=CARTESIAN_POINT('Ctrl Pts',(1.62061227799994,11.6,10.2551639));
#222900=CARTESIAN_POINT('Ctrl Pts',(1.62037240999994,15.2,10.25422529));
#222901=CARTESIAN_POINT('Ctrl Pts',(1.62037240999994,11.6,10.25422529));
#222902=CARTESIAN_POINT('Ctrl Pts',(1.62013580699994,15.2,10.253295587));
#222903=CARTESIAN_POINT('Ctrl Pts',(1.62013580699994,11.6,10.253295587));
#222904=CARTESIAN_POINT('Ctrl Pts',(1.61990245999994,15.2,10.252374818));
#222905=CARTESIAN_POINT('Ctrl Pts',(1.61990245999994,11.6,10.252374818));
#222906=CARTESIAN_POINT('Ctrl Pts',(1.61967235799994,15.2,10.251463016));
#222907=CARTESIAN_POINT('Ctrl Pts',(1.61967235799994,11.6,10.251463016));
#222908=CARTESIAN_POINT('Ctrl Pts',(1.61944548799994,15.2,10.250560211));
#222909=CARTESIAN_POINT('Ctrl Pts',(1.61944548799994,11.6,10.250560211));
#222910=CARTESIAN_POINT('Ctrl Pts',(1.61922312999994,15.2,10.249671582));
#222911=CARTESIAN_POINT('Ctrl Pts',(1.61922312999994,11.6,10.249671582));
#222912=CARTESIAN_POINT('Ctrl Pts',(1.61904803299994,15.2,10.248968852));
#222913=CARTESIAN_POINT('Ctrl Pts',(1.61904803299994,11.6,10.248968852));
#222914=CARTESIAN_POINT('Ctrl Pts',(1.61891843999994,15.2,10.248447089));
#222915=CARTESIAN_POINT('Ctrl Pts',(1.61891843999994,11.6,10.248447089));
#222916=CARTESIAN_POINT('Ctrl Pts',(1.61883308399994,15.2,10.248102704));
#222917=CARTESIAN_POINT('Ctrl Pts',(1.61883308399994,11.6,10.248102704));
#222918=CARTESIAN_POINT('Ctrl Pts',(1.61879117999994,15.2,10.247933457));
#222919=CARTESIAN_POINT('Ctrl Pts',(1.61879117999994,11.6,10.247933457));
#222920=CARTESIAN_POINT('',(1.61879117999994,12.2,10.247933456));
#222921=CARTESIAN_POINT('',(1.61879117999994,15.2,10.247933456));
#222922=CARTESIAN_POINT('',(1.61879117999994,12.2,10.247933456));
#222923=CARTESIAN_POINT('Ctrl Pts',(2.17615954699994,12.2,11.292224299));
#222924=CARTESIAN_POINT('Ctrl Pts',(2.17309893155329,12.2,11.2881482228521));
#222925=CARTESIAN_POINT('Ctrl Pts',(2.17005151744838,12.2,11.2840769414757));
#222926=CARTESIAN_POINT('Ctrl Pts',(2.1670173032288,12.2,11.2800104643101));
#222927=CARTESIAN_POINT('Ctrl Pts',(2.16474164277082,12.2,11.2769606067129));
#222928=CARTESIAN_POINT('Ctrl Pts',(2.16247340685917,12.2,11.2739134515355));
#222929=CARTESIAN_POINT('Ctrl Pts',(2.16021259628755,12.2,11.270869025661));
#222930=CARTESIAN_POINT('Ctrl Pts',(2.15795178571594,12.2,11.2678245997865));
#222931=CARTESIAN_POINT('Ctrl Pts',(2.15569840077296,12.2,11.2647829037414));
#222932=CARTESIAN_POINT('Ctrl Pts',(2.15345243877187,12.2,11.2617439866854));
#222933=CARTESIAN_POINT('Ctrl Pts',(2.15120647677078,12.2,11.2587050696294));
#222934=CARTESIAN_POINT('Ctrl Pts',(2.14896793703549,12.2,11.2556689314398));
#222935=CARTESIAN_POINT('Ctrl Pts',(2.14673681999156,12.2,11.2526356197583));
#222936=CARTESIAN_POINT('Ctrl Pts',(2.14450570294763,12.2,11.2496023080769));
#222937=CARTESIAN_POINT('Ctrl Pts',(2.14228200681172,12.2,11.2465718218036));
#222938=CARTESIAN_POINT('Ctrl Pts',(2.14006573176659,12.2,11.2435441981217));
#222939=CARTESIAN_POINT('Ctrl Pts',(2.13784945672146,12.2,11.2405165744398));
#222940=CARTESIAN_POINT('Ctrl Pts',(2.13564060100672,12.2,11.2374918133761));
#222941=CARTESIAN_POINT('Ctrl Pts',(2.13343916493422,12.2,11.2344699530847));
#222942=CARTESIAN_POINT('Ctrl Pts',(2.13123772886173,12.2,11.2314480927932));
#222943=CARTESIAN_POINT('Ctrl Pts',(2.12904371206482,12.2,11.2284291335483));
#222944=CARTESIAN_POINT('Ctrl Pts',(2.12685711172657,12.2,11.2254131179491));
#222945=CARTESIAN_POINT('Ctrl Pts',(2.12467051099109,12.2,11.222397101802));
#222946=CARTESIAN_POINT('Ctrl Pts',(2.12249132822439,12.2,11.2193840298141));
#222947=CARTESIAN_POINT('Ctrl Pts',(2.12031955995146,12.2,11.2163739436271));
#222948=CARTESIAN_POINT('Ctrl Pts',(2.11814779207307,12.2,11.2133638579869));
#222949=CARTESIAN_POINT('Ctrl Pts',(2.11598344051922,12.2,11.2103567576298));
#222950=CARTESIAN_POINT('Ctrl Pts',(2.11382650205658,12.2,11.2073526849476));
#222951=CARTESIAN_POINT('Ctrl Pts',(2.11166956359395,12.2,11.2043486122654));
#222952=CARTESIAN_POINT('Ctrl Pts',(2.10952003867981,12.2,11.2013475656353));
#222953=CARTESIAN_POINT('Ctrl Pts',(2.10737792524795,12.2,11.1983495874806));
#222954=CARTESIAN_POINT('Ctrl Pts',(2.10523581181609,12.2,11.1953516093259));
#222955=CARTESIAN_POINT('Ctrl Pts',(2.10310110988422,12.2,11.1923566989576));
#222956=CARTESIAN_POINT('Ctrl Pts',(2.1009738169935,12.2,11.189364899261));
#222957=CARTESIAN_POINT('Ctrl Pts',(2.09884652410277,12.2,11.1863730995645));
#222958=CARTESIAN_POINT('Ctrl Pts',(2.09672664165414,12.2,11.1833844089672));
#222959=CARTESIAN_POINT('Ctrl Pts',(2.09461416573028,12.2,11.1803988718254));
#222960=CARTESIAN_POINT('Ctrl Pts',(2.09250168980641,12.2,11.1774133346837));
#222961=CARTESIAN_POINT('Ctrl Pts',(2.090396621432,12.2,11.1744309502416));
#222962=CARTESIAN_POINT('Ctrl Pts',(2.08829895746552,12.2,11.1714517601411));
#222963=CARTESIAN_POINT('Ctrl Pts',(2.08620129311796,12.2,11.1684725694993));
#222964=CARTESIAN_POINT('Ctrl Pts',(2.08411103349752,12.2,11.1654965735335));
#222965=CARTESIAN_POINT('Ctrl Pts',(2.08202817707084,12.2,11.1625238148519));
#222966=CARTESIAN_POINT('Ctrl Pts',(2.07994532102253,12.2,11.1595510567104));
#222967=CARTESIAN_POINT('Ctrl Pts',(2.07786986674384,12.2,11.1565815355495));
#222968=CARTESIAN_POINT('Ctrl Pts',(2.07580181263318,12.2,11.1536152947178));
#222969=CARTESIAN_POINT('Ctrl Pts',(2.07373375852252,12.2,11.1506490538861));
#222970=CARTESIAN_POINT('Ctrl Pts',(2.07167310431762,12.2,11.1476860921196));
#222971=CARTESIAN_POINT('Ctrl Pts',(2.06961984730955,12.2,11.1447264544358));
#222972=CARTESIAN_POINT('Ctrl Pts',(2.06756659030147,12.2,11.1417668167519));
#222973=CARTESIAN_POINT('Ctrl Pts',(2.06552072977582,12.2,11.1388105005927));
#222974=CARTESIAN_POINT('Ctrl Pts',(2.06348226426655,12.2,11.13585755145));
#222975=CARTESIAN_POINT('Ctrl Pts',(2.06144379875728,12.2,11.1329046023072));
#222976=CARTESIAN_POINT('Ctrl Pts',(2.05941272753107,12.2,11.1299550194978));
#222977=CARTESIAN_POINT('Ctrl Pts',(2.05738904797893,12.2,11.1270088463545));
#222978=CARTESIAN_POINT('Ctrl Pts',(2.05536536842678,12.2,11.1240626732112));
#222979=CARTESIAN_POINT('Ctrl Pts',(2.05334907929919,12.2,11.1211199087344));
#222980=CARTESIAN_POINT('Ctrl Pts',(2.05134017970451,12.2,11.1181805985907));
#222981=CARTESIAN_POINT('Ctrl Pts',(2.04933127974487,12.2,11.1152412879131));
#222982=CARTESIAN_POINT('Ctrl Pts',(2.04732976728732,12.2,11.1123054302197));
#222983=CARTESIAN_POINT('Ctrl Pts',(2.04533564133185,12.2,11.1093730691274));
#222984=CARTESIAN_POINT('Ctrl Pts',(2.04334151573865,12.2,11.1064407085677));
#222985=CARTESIAN_POINT('Ctrl Pts',(2.04135477412644,12.2,11.1035118456568));
#222986=CARTESIAN_POINT('Ctrl Pts',(2.03937541410034,12.2,11.1005865234507));
#222987=CARTESIAN_POINT('Ctrl Pts',(2.03739605407425,12.2,11.0976612012446));
#222988=CARTESIAN_POINT('Ctrl Pts',(2.03542407759717,12.2,11.0947394202922));
#222989=CARTESIAN_POINT('Ctrl Pts',(2.03345947908588,12.2,11.0918212251903));
#222990=CARTESIAN_POINT('Ctrl Pts',(2.03149488057459,12.2,11.0889030300883));
#222991=CARTESIAN_POINT('Ctrl Pts',(2.02953765971237,12.2,11.0859884203442));
#222992=CARTESIAN_POINT('Ctrl Pts',(2.02758781424156,12.2,11.0830774407833));
#222993=CARTESIAN_POINT('Ctrl Pts',(2.02563796877075,12.2,11.0801664612224));
#222994=CARTESIAN_POINT('Ctrl Pts',(2.02369549872463,12.2,11.0772591115947));
#222995=CARTESIAN_POINT('Ctrl Pts',(2.02176039971094,12.2,11.0743554370332));
#222996=CARTESIAN_POINT('Ctrl Pts',(2.01982530069725,12.2,11.0714517624717));
#222997=CARTESIAN_POINT('Ctrl Pts',(2.01789757243184,12.2,11.0685517625335));
#222998=CARTESIAN_POINT('Ctrl Pts',(2.01597721136318,12.2,11.0656554827854));
#222999=CARTESIAN_POINT('Ctrl Pts',(2.01405685029451,12.2,11.0627592030372));
#223000=CARTESIAN_POINT('Ctrl Pts',(2.01214385698044,12.2,11.059866643242));
#223001=CARTESIAN_POINT('Ctrl Pts',(2.01023822788199,12.2,11.0569778491381));
#223002=CARTESIAN_POINT('Ctrl Pts',(2.00833259843735,12.2,11.0540890545093));
#223003=CARTESIAN_POINT('Ctrl Pts',(2.00643433177815,12.2,11.0512040246567));
#223004=CARTESIAN_POINT('Ctrl Pts',(2.00454342487935,12.2,11.0483228056135));
#223005=CARTESIAN_POINT('Ctrl Pts',(2.00202221625347,12.2,11.044481181095));
#223006=CARTESIAN_POINT('Ctrl Pts',(1.99951409062867,12.2,11.0406463320394));
#223007=CARTESIAN_POINT('Ctrl Pts',(1.99701903872065,12.2,11.0368183661296));
#223008=CARTESIAN_POINT('Ctrl Pts',(1.99514774970465,12.2,11.0339473915669));
#223009=CARTESIAN_POINT('Ctrl Pts',(1.99328381425198,12.2,11.0310802884434));
#223010=CARTESIAN_POINT('Ctrl Pts',(1.99142722855917,12.2,11.0282171037789));
#223011=CARTESIAN_POINT('Ctrl Pts',(1.98957064286635,12.2,11.0253539191145));
#223012=CARTESIAN_POINT('Ctrl Pts',(1.98772140560218,12.2,11.0224946528192));
#223013=CARTESIAN_POINT('Ctrl Pts',(1.9858795144181,12.2,11.0196393503808));
#223014=CARTESIAN_POINT('Ctrl Pts',(1.98403762289942,12.2,11.0167840474236));
#223015=CARTESIAN_POINT('Ctrl Pts',(1.98220307456614,12.2,11.0139327102925));
#223016=CARTESIAN_POINT('Ctrl Pts',(1.98037586809323,12.2,11.0110853828792));
#223017=CARTESIAN_POINT('Ctrl Pts',(1.97793959334926,12.2,11.0072889471903));
#223018=CARTESIAN_POINT('Ctrl Pts',(1.97551636664254,12.2,11.0034996433922));
#223019=CARTESIAN_POINT('Ctrl Pts',(1.97310617867204,12.2,10.9997175808675));
#223020=CARTESIAN_POINT('Ctrl Pts',(1.97129853761207,12.2,10.9968810338452));
#223021=CARTESIAN_POINT('Ctrl Pts',(1.96949822975547,12.2,10.9940485608862));
#223022=CARTESIAN_POINT('Ctrl Pts',(1.96770525106353,12.2,10.9912202083055));
#223023=CARTESIAN_POINT('Ctrl Pts',(1.96591227237159,12.2,10.9883918557249));
#223024=CARTESIAN_POINT('Ctrl Pts',(1.96412662200731,12.2,10.9855676245629));
#223025=CARTESIAN_POINT('Ctrl Pts',(1.96234829590424,12.2,10.9827475615814));
#223026=CARTESIAN_POINT('Ctrl Pts',(1.95997719421811,12.2,10.9789874772646));
#223027=CARTESIAN_POINT('Ctrl Pts',(1.95761911145266,12.2,10.9752348048568));
#223028=CARTESIAN_POINT('Ctrl Pts',(1.95527403649156,12.2,10.9714896547083));
#223029=CARTESIAN_POINT('Ctrl Pts',(1.95292896153046,12.2,10.9677445045598));
#223030=CARTESIAN_POINT('Ctrl Pts',(1.95059689454579,12.2,10.9640068794509));
#223031=CARTESIAN_POINT('Ctrl Pts',(1.94827782042073,12.2,10.9602768924151));
#223032=CARTESIAN_POINT('Ctrl Pts',(1.94479920954912,12.2,10.9546819123696));
#223033=CARTESIAN_POINT('Ctrl Pts',(1.9413498362714,12.2,10.9491041170025));
#223034=CARTESIAN_POINT('Ctrl Pts',(1.93792965506362,12.2,10.9435438979553));
#223035=CARTESIAN_POINT('Ctrl Pts',(1.93564953436199,12.2,10.9398370854256));
#223036=CARTESIAN_POINT('Ctrl Pts',(1.93338238634383,12.2,10.9361380831136));
#223037=CARTESIAN_POINT('Ctrl Pts',(1.93112819836012,12.2,10.9324470093034));
#223038=CARTESIAN_POINT('Ctrl Pts',(1.92887401006929,12.2,10.9287559349904));
#223039=CARTESIAN_POINT('Ctrl Pts',(1.92663278119101,12.2,10.9250727883061));
#223040=CARTESIAN_POINT('Ctrl Pts',(1.92440449694838,12.2,10.9213976872558));
#223041=CARTESIAN_POINT('Ctrl Pts',(1.92217621300935,12.2,10.9177225867062));
#223042=CARTESIAN_POINT('Ctrl Pts',(1.9199608746424,12.2,10.9140555307777));
#223043=CARTESIAN_POINT('Ctrl Pts',(1.91775846537666,12.2,10.9103966382982));
#223044=CARTESIAN_POINT('Ctrl Pts',(1.91555605581084,12.2,10.9067377453201));
#223045=CARTESIAN_POINT('Ctrl Pts',(1.91336657607407,12.2,10.903087015429));
#223046=CARTESIAN_POINT('Ctrl Pts',(1.91119000973322,12.2,10.8994445685083));
#223047=CARTESIAN_POINT('Ctrl Pts',(1.90901344339237,12.2,10.8958021215875));
#223048=CARTESIAN_POINT('Ctrl Pts',(1.9068497905586,12.2,10.8921679588567));
#223049=CARTESIAN_POINT('Ctrl Pts',(1.90469903566491,12.2,10.8885421973821));
#223050=CARTESIAN_POINT('Ctrl Pts',(1.90254828106427,12.2,10.8849164364016));
#223051=CARTESIAN_POINT('Ctrl Pts',(1.9004104241262,12.2,10.8812990782488));
#223052=CARTESIAN_POINT('Ctrl Pts',(1.89828544873468,12.2,10.8776902450274));
#223053=CARTESIAN_POINT('Ctrl Pts',(1.89616047305363,12.2,10.8740814113143));
#223054=CARTESIAN_POINT('Ctrl Pts',(1.89404837804477,12.2,10.8704811012881));
#223055=CARTESIAN_POINT('Ctrl Pts',(1.89194914643168,12.2,10.8668894377044));
#223056=CARTESIAN_POINT('Ctrl Pts',(1.88984991510461,12.2,10.86329777461));
#223057=CARTESIAN_POINT('Ctrl Pts',(1.88776354742586,12.2,10.8597147567423));
#223058=CARTESIAN_POINT('Ctrl Pts',(1.88569002542786,12.2,10.8561405095339));
#223059=CARTESIAN_POINT('Ctrl Pts',(1.88361650314734,12.2,10.8525662618385));
#223060=CARTESIAN_POINT('Ctrl Pts',(1.88155582747394,12.2,10.8490007832713));
#223061=CARTESIAN_POINT('Ctrl Pts',(1.87950797842781,12.2,10.8454441982339));
#223062=CARTESIAN_POINT('Ctrl Pts',(1.8774601296607,12.2,10.8418876136811));
#223063=CARTESIAN_POINT('Ctrl Pts',(1.87542510820642,12.2,10.8383399229979));
#223064=CARTESIAN_POINT('Ctrl Pts',(1.87340289614866,12.2,10.834801251231));
#223065=CARTESIAN_POINT('Ctrl Pts',(1.87138068381538,12.2,10.8312625789819));
#223066=CARTESIAN_POINT('Ctrl Pts',(1.86937127983366,12.2,10.8277329257257));
#223067=CARTESIAN_POINT('Ctrl Pts',(1.8673746648368,12.2,10.8242124169789));
#223068=CARTESIAN_POINT('Ctrl Pts',(1.86537805011197,12.2,10.8206919087118));
#223069=CARTESIAN_POINT('Ctrl Pts',(1.86339422444842,12.2,10.8171805462149));
#223070=CARTESIAN_POINT('Ctrl Pts',(1.8614231683305,12.2,10.8136784563892));
#223071=CARTESIAN_POINT('Ctrl Pts',(1.85945211194402,12.2,10.8101763660863));
#223072=CARTESIAN_POINT('Ctrl Pts',(1.85749382363286,12.2,10.8066835475227));
#223073=CARTESIAN_POINT('Ctrl Pts',(1.85554828524024,12.2,10.8032001300392));
#223074=CARTESIAN_POINT('Ctrl Pts',(1.85360274711269,12.2,10.7997167130304));
#223075=CARTESIAN_POINT('Ctrl Pts',(1.85166995651375,12.2,10.7962426969536));
#223076=CARTESIAN_POINT('Ctrl Pts',(1.8497498937805,12.2,10.7927782112914));
#223077=CARTESIAN_POINT('Ctrl Pts',(1.84782983078564,12.2,10.7893137251571));
#223078=CARTESIAN_POINT('Ctrl Pts',(1.84592249567537,12.2,10.7858587698905));
#223079=CARTESIAN_POINT('Ctrl Pts',(1.84402786601656,12.2,10.7824134757583));
#223080=CARTESIAN_POINT('Ctrl Pts',(1.84213323635775,12.2,10.7789681816261));
#223081=CARTESIAN_POINT('Ctrl Pts',(1.84025131114487,12.2,10.7755325486895));
#223082=CARTESIAN_POINT('Ctrl Pts',(1.83838207071094,12.2,10.7721067084482));
#223083=CARTESIAN_POINT('Ctrl Pts',(1.8365128305317,12.2,10.7686808686736));
#223084=CARTESIAN_POINT('Ctrl Pts',(1.83465627373659,12.2,10.7652648208643));
#223085=CARTESIAN_POINT('Ctrl Pts',(1.83281237576783,12.2,10.7618586999606));
#223086=CARTESIAN_POINT('Ctrl Pts',(1.83096847754783,12.2,10.7584525785929));
#223087=CARTESIAN_POINT('Ctrl Pts',(1.82913724192538,12.2,10.7550563833771));
#223088=CARTESIAN_POINT('Ctrl Pts',(1.82731864099423,12.2,10.7516702484713));
#223089=CARTESIAN_POINT('Ctrl Pts',(1.82550004031086,12.2,10.7482841140269));
#223090=CARTESIAN_POINT('Ctrl Pts',(1.82369407698697,12.2,10.7449080381008));
#223091=CARTESIAN_POINT('Ctrl Pts',(1.82190072618828,12.2,10.7415421590419));
#223092=CARTESIAN_POINT('Ctrl Pts',(1.82010737514524,12.2,10.7381762795244));
#223093=CARTESIAN_POINT('Ctrl Pts',(1.81832663587978,12.2,10.7348205943326));
#223094=CARTESIAN_POINT('Ctrl Pts',(1.81655848475172,12.2,10.7314752420396));
#223095=CARTESIAN_POINT('Ctrl Pts',(1.81479033386458,12.2,10.7281298902024));
#223096=CARTESIAN_POINT('Ctrl Pts',(1.81303477018419,12.2,10.7247948705063));
#223097=CARTESIAN_POINT('Ctrl Pts',(1.81129176865916,12.2,10.7214703202218));
#223098=CARTESIAN_POINT('Ctrl Pts',(1.80954876689666,12.2,10.7181457694843));
#223099=CARTESIAN_POINT('Ctrl Pts',(1.80781832723848,12.2,10.7148316879288));
#223100=CARTESIAN_POINT('Ctrl Pts',(1.80610042353458,12.2,10.7115282164717));
#223101=CARTESIAN_POINT('Ctrl Pts',(1.80438252006474,12.2,10.7082247454647));
#223102=CARTESIAN_POINT('Ctrl Pts',(1.80267715204844,12.2,10.7049318841117));
#223103=CARTESIAN_POINT('Ctrl Pts',(1.80098429321228,12.2,10.7016497709929));
#223104=CARTESIAN_POINT('Ctrl Pts',(1.79929143414546,12.2,10.6983676574269));
#223105=CARTESIAN_POINT('Ctrl Pts',(1.79761108396485,12.2,10.6950962926355));
#223106=CARTESIAN_POINT('Ctrl Pts',(1.795943216097,12.2,10.6918358199585));
#223107=CARTESIAN_POINT('Ctrl Pts',(1.7942753484564,12.2,10.6885753477258));
#223108=CARTESIAN_POINT('Ctrl Pts',(1.79261996030214,12.2,10.6853257658186));
#223109=CARTESIAN_POINT('Ctrl Pts',(1.79097702676852,12.2,10.6820872188045));
#223110=CARTESIAN_POINT('Ctrl Pts',(1.78933409301105,12.2,10.6788486713491));
#223111=CARTESIAN_POINT('Ctrl Pts',(1.78770361273316,12.2,10.6756211567431));
#223112=CARTESIAN_POINT('Ctrl Pts',(1.7860855557488,12.2,10.6724048219978));
#223113=CARTESIAN_POINT('Ctrl Pts',(1.7844674989849,12.2,10.6691884876906));
#223114=CARTESIAN_POINT('Ctrl Pts',(1.78286186607308,12.2,10.66598333144));
#223115=CARTESIAN_POINT('Ctrl Pts',(1.7812686290354,12.2,10.6627894992555));
#223116=CARTESIAN_POINT('Ctrl Pts',(1.77967539178064,12.2,10.6595956666358));
#223117=CARTESIAN_POINT('Ctrl Pts',(1.77809454787428,12.2,10.6564131581117));
#223118=CARTESIAN_POINT('Ctrl Pts',(1.77652606823323,12.2,10.6532421227166));
#223119=CARTESIAN_POINT('Ctrl Pts',(1.77495758859218,12.2,10.6500710873215));
#223120=CARTESIAN_POINT('Ctrl Pts',(1.77340147341368,12.2,10.6469115219806));
#223121=CARTESIAN_POINT('Ctrl Pts',(1.7718576909975,12.2,10.6437635779769));
#223122=CARTESIAN_POINT('Ctrl Pts',(1.77031390879166,12.2,10.6406156344022));
#223123=CARTESIAN_POINT('Ctrl Pts',(1.76878245874758,12.2,10.6374793094831));
#223124=CARTESIAN_POINT('Ctrl Pts',(1.76726331047594,12.2,10.6343547565021));
#223125=CARTESIAN_POINT('Ctrl Pts',(1.76574416199731,12.2,10.6312302030953));
#223126=CARTESIAN_POINT('Ctrl Pts',(1.76423731439687,12.2,10.6281174196274));
#223127=CARTESIAN_POINT('Ctrl Pts',(1.76274273520554,12.2,10.6250165584596));
#223128=CARTESIAN_POINT('Ctrl Pts',(1.76124815621784,12.2,10.6219156977143));
#223129=CARTESIAN_POINT('Ctrl Pts',(1.75976584454525,12.2,10.6188267593453));
#223130=CARTESIAN_POINT('Ctrl Pts',(1.75829576888686,12.2,10.6157498964849));
#223131=CARTESIAN_POINT('Ctrl Pts',(1.75682569302816,12.2,10.6126730332053));
#223132=CARTESIAN_POINT('Ctrl Pts',(1.75536785107626,12.2,10.6096082452749));
#223133=CARTESIAN_POINT('Ctrl Pts',(1.75392220931519,12.2,10.6065556866237));
#223134=CARTESIAN_POINT('Ctrl Pts',(1.7524765677511,12.2,10.6035031283885));
#223135=CARTESIAN_POINT('Ctrl Pts',(1.75104312720914,12.2,10.6004628009175));
#223136=CARTESIAN_POINT('Ctrl Pts',(1.74962185215787,12.2,10.5974348594976));
#223137=CARTESIAN_POINT('Ctrl Pts',(1.74784525819854,12.2,10.5936499324133));
#223138=CARTESIAN_POINT('Ctrl Pts',(1.74608767042026,12.2,10.5898843590294));
#223139=CARTESIAN_POINT('Ctrl Pts',(1.74434902236372,12.2,10.5861384477784));
#223140=CARTESIAN_POINT('Ctrl Pts',(1.74261037430718,12.2,10.5823925365274));
#223141=CARTESIAN_POINT('Ctrl Pts',(1.74089066348638,12.2,10.5786662883744));
#223142=CARTESIAN_POINT('Ctrl Pts',(1.73918981799249,12.2,10.5749600155103));
#223143=CARTESIAN_POINT('Ctrl Pts',(1.73748897249861,12.2,10.5712537426462));
#223144=CARTESIAN_POINT('Ctrl Pts',(1.73580699238881,12.2,10.5675674460222));
#223145=CARTESIAN_POINT('Ctrl Pts',(1.73414380349989,12.2,10.5639014415083));
#223146=CARTESIAN_POINT('Ctrl Pts',(1.73248061461097,12.2,10.5602354369943));
#223147=CARTESIAN_POINT('Ctrl Pts',(1.73083621547212,12.2,10.5565897258499));
#223148=CARTESIAN_POINT('Ctrl Pts',(1.7292105307499,12.2,10.5529646287666));
#223149=CARTESIAN_POINT('Ctrl Pts',(1.72758484602768,12.2,10.5493395316833));
#223150=CARTESIAN_POINT('Ctrl Pts',(1.7259778751062,12.2,10.545735047442));
#223151=CARTESIAN_POINT('Ctrl Pts',(1.7243895380157,12.2,10.542151505273));
#223152=CARTESIAN_POINT('Ctrl Pts',(1.7228012009252,12.2,10.538567963104));
#223153=CARTESIAN_POINT('Ctrl Pts',(1.72123149925315,12.2,10.5350053598118));
#223154=CARTESIAN_POINT('Ctrl Pts',(1.71968035036523,12.2,10.5314640272435));
#223155=CARTESIAN_POINT('Ctrl Pts',(1.71812920147731,12.2,10.5279226946751));
#223156=CARTESIAN_POINT('Ctrl Pts',(1.71659660646114,12.2,10.5244026342868));
#223157=CARTESIAN_POINT('Ctrl Pts',(1.71508248014265,12.2,10.5209041782463));
#223158=CARTESIAN_POINT('Ctrl Pts',(1.71356835382416,12.2,10.5174057222057));
#223159=CARTESIAN_POINT('Ctrl Pts',(1.71207269717323,12.2,10.51392887217));
#223160=CARTESIAN_POINT('Ctrl Pts',(1.71059542404514,12.2,10.5104739667906));
#223161=CARTESIAN_POINT('Ctrl Pts',(1.70911815091704,12.2,10.5070190614112));
#223162=CARTESIAN_POINT('Ctrl Pts',(1.70765926097109,12.2,10.5035861014465));
#223163=CARTESIAN_POINT('Ctrl Pts',(1.70621866611147,12.2,10.5001754328372));
#223164=CARTESIAN_POINT('Ctrl Pts',(1.70477807125186,12.2,10.4967647642279));
#223165=CARTESIAN_POINT('Ctrl Pts',(1.70335576950365,12.2,10.4933763843634));
#223166=CARTESIAN_POINT('Ctrl Pts',(1.70195167228292,12.2,10.4900106450597));
#223167=CARTESIAN_POINT('Ctrl Pts',(1.70054757521522,12.2,10.4866449061229));
#223168=CARTESIAN_POINT('Ctrl Pts',(1.69916168149787,12.2,10.4833018078242));
#223169=CARTESIAN_POINT('Ctrl Pts',(1.69779389768714,12.2,10.4799817031842));
#223170=CARTESIAN_POINT('Ctrl Pts',(1.69642611372733,12.2,10.4766615981823));
#223171=CARTESIAN_POINT('Ctrl Pts',(1.69507643882556,12.2,10.4733644883078));
#223172=CARTESIAN_POINT('Ctrl Pts',(1.69374477736575,12.2,10.4700907346948));
#223173=CARTESIAN_POINT('Ctrl Pts',(1.69241311590595,12.2,10.4668169810818));
#223174=CARTESIAN_POINT('Ctrl Pts',(1.69109946828857,12.2,10.4635665797207));
#223175=CARTESIAN_POINT('Ctrl Pts',(1.68980373412538,12.2,10.4603399018496));
#223176=CARTESIAN_POINT('Ctrl Pts',(1.6885079999622,12.2,10.4571132239785));
#223177=CARTESIAN_POINT('Ctrl Pts',(1.68723017946111,12.2,10.4539102665425));
#223178=CARTESIAN_POINT('Ctrl Pts',(1.68597017126575,12.2,10.450731400708));
#223179=CARTESIAN_POINT('Ctrl Pts',(1.68471016307039,12.2,10.4475525348734));
#223180=CARTESIAN_POINT('Ctrl Pts',(1.68346796659213,12.2,10.4443977617894));
#223181=CARTESIAN_POINT('Ctrl Pts',(1.68224347756342,12.2,10.4412674584548));
#223182=CARTESIAN_POINT('Ctrl Pts',(1.68077409078236,12.2,10.4375110945897));
#223183=CARTESIAN_POINT('Ctrl Pts',(1.67933020167139,12.2,10.4337899652535));
#223184=CARTESIAN_POINT('Ctrl Pts',(1.67791162388786,12.2,10.430104736385));
#223185=CARTESIAN_POINT('Ctrl Pts',(1.67649304597548,12.2,10.4264195071816));
#223186=CARTESIAN_POINT('Ctrl Pts',(1.67509978025723,12.2,10.4227701775234));
#223187=CARTESIAN_POINT('Ctrl Pts',(1.67373163143378,12.2,10.4191574215782));
#223188=CARTESIAN_POINT('Ctrl Pts',(1.6723634827346,12.2,10.4155446659611));
#223189=CARTESIAN_POINT('Ctrl Pts',(1.67102045290033,12.2,10.4119684863308));
#223190=CARTESIAN_POINT('Ctrl Pts',(1.66970234002549,12.2,10.4084295715265));
#223191=CARTESIAN_POINT('Ctrl Pts',(1.66838422715066,12.2,10.4048906567222));
#223192=CARTESIAN_POINT('Ctrl Pts',(1.66709103268544,12.2,10.4013890058459));
#223193=CARTESIAN_POINT('Ctrl Pts',(1.6658225496465,12.2,10.3979253233858));
#223194=CARTESIAN_POINT('Ctrl Pts',(1.66455406649235,12.2,10.3944616406111));
#223195=CARTESIAN_POINT('Ctrl Pts',(1.66331029366625,12.2,10.3910359265238));
#223196=CARTESIAN_POINT('Ctrl Pts',(1.66209101762368,12.2,10.3876488976724));
#223197=CARTESIAN_POINT('Ctrl Pts',(1.66087174169186,12.2,10.3842618691286));
#223198=CARTESIAN_POINT('Ctrl Pts',(1.65967696619903,12.2,10.380913527188));
#223199=CARTESIAN_POINT('Ctrl Pts',(1.65850646349157,12.2,10.3776046037249));
#223200=CARTESIAN_POINT('Ctrl Pts',(1.65733596078412,12.2,10.3742956802619));
#223201=CARTESIAN_POINT('Ctrl Pts',(1.65618973598353,12.2,10.3710261756837));
#223202=CARTESIAN_POINT('Ctrl Pts',(1.65506755788352,12.2,10.3677968380541));
#223203=CARTESIAN_POINT('Ctrl Pts',(1.65394537968158,12.2,10.3645675001311));
#223204=CARTESIAN_POINT('Ctrl Pts',(1.65284724727307,12.2,10.3613783289672));
#223205=CARTESIAN_POINT('Ctrl Pts',(1.65177292788281,12.2,10.3582300893818));
#223206=CARTESIAN_POINT('Ctrl Pts',(1.65069860859013,12.2,10.3550818500823));
#223207=CARTESIAN_POINT('Ctrl Pts',(1.64964809727928,12.2,10.3519745432386));
#223208=CARTESIAN_POINT('Ctrl Pts',(1.64862115398323,12.2,10.3489089490166));
#223209=CARTESIAN_POINT('Ctrl Pts',(1.64759421068719,12.2,10.3458433547945));
#223210=CARTESIAN_POINT('Ctrl Pts',(1.64659083092614,12.2,10.3428194731649));
#223211=CARTESIAN_POINT('Ctrl Pts',(1.6456107655781,12.2,10.3398381047884));
#223212=CARTESIAN_POINT('Ctrl Pts',(1.64463070014104,12.2,10.3368567361412));
#223213=CARTESIAN_POINT('Ctrl Pts',(1.64367394661412,12.2,10.3339178787225));
#223214=CARTESIAN_POINT('Ctrl Pts',(1.64274024339814,12.2,10.331022351401));
#223215=CARTESIAN_POINT('Ctrl Pts',(1.64180654026696,12.2,10.3281268243424));
#223216=CARTESIAN_POINT('Ctrl Pts',(1.64089588844622,12.2,10.3252746264176));
#223217=CARTESIAN_POINT('Ctrl Pts',(1.6400080142245,12.2,10.322466595257));
#223218=CARTESIAN_POINT('Ctrl Pts',(1.63912014000279,12.2,10.3196585640964));
#223219=CARTESIAN_POINT('Ctrl Pts',(1.63825504561629,12.2,10.3168946979098));
#223220=CARTESIAN_POINT('Ctrl Pts',(1.63741244931259,12.2,10.3141758549233));
#223221=CARTESIAN_POINT('Ctrl Pts',(1.63656985293235,12.2,10.3114570116898));
#223222=CARTESIAN_POINT('Ctrl Pts',(1.6357497546799,12.2,10.3087831905119));
#223223=CARTESIAN_POINT('Ctrl Pts',(1.63495186338794,12.2,10.3061552694551));
#223224=CARTESIAN_POINT('Ctrl Pts',(1.63415397216845,12.2,10.3035273486371));
#223225=CARTESIAN_POINT('Ctrl Pts',(1.63337828878057,12.2,10.3009453276011));
#223226=CARTESIAN_POINT('Ctrl Pts',(1.63262451147558,12.2,10.2984101058619));
#223227=CARTESIAN_POINT('Ctrl Pts',(1.6318707341706,12.2,10.2958748841228));
#223228=CARTESIAN_POINT('Ctrl Pts',(1.63113886235551,12.2,10.2933864594548));
#223229=CARTESIAN_POINT('Ctrl Pts',(1.63042858579704,12.2,10.2909457576248));
#223230=CARTESIAN_POINT('Ctrl Pts',(1.62971830923857,12.2,10.2885050557947));
#223231=CARTESIAN_POINT('Ctrl Pts',(1.62902962534985,12.2,10.2861120735653));
#223232=CARTESIAN_POINT('Ctrl Pts',(1.62836221553933,12.2,10.2837677582304));
#223233=CARTESIAN_POINT('Ctrl Pts',(1.62769480566818,12.2,10.2814234426827));
#223234=CARTESIAN_POINT('Ctrl Pts',(1.62704866405742,12.2,10.2791277938896));
#223235=CARTESIAN_POINT('Ctrl Pts',(1.62642346044092,12.2,10.2768817823527));
#223236=CARTESIAN_POINT('Ctrl Pts',(1.62569405630686,12.2,10.2742614358656));
#223237=CARTESIAN_POINT('Ctrl Pts',(1.62499314804473,12.2,10.2717086493813));
#223238=CARTESIAN_POINT('Ctrl Pts',(1.62432018577945,12.2,10.2692250127819));
#223239=CARTESIAN_POINT('Ctrl Pts',(1.62374336091328,12.2,10.2670961811625));
#223240=CARTESIAN_POINT('Ctrl Pts',(1.62318706408245,12.2,10.2650181509895));
#223241=CARTESIAN_POINT('Ctrl Pts',(1.62265093722078,12.2,10.2629919546313));
#223242=CARTESIAN_POINT('Ctrl Pts',(1.6221148104078,12.2,10.2609657584572));
#223243=CARTESIAN_POINT('Ctrl Pts',(1.62159885033441,12.2,10.2589913938565));
#223244=CARTESIAN_POINT('Ctrl Pts',(1.6211026825168,12.2,10.2570699217508));
#223245=CARTESIAN_POINT('Ctrl Pts',(1.62027811736746,12.2,10.2538766897886));
#223246=CARTESIAN_POINT('Ctrl Pts',(1.61950821818824,12.2,10.2508295185277));
#223247=CARTESIAN_POINT('Ctrl Pts',(1.61879117999994,12.2,10.247933457));
#223248=CARTESIAN_POINT('Ctrl Pts',(1.61879117999994,15.2,10.247933457));
#223249=CARTESIAN_POINT('Ctrl Pts',(1.61922057460978,15.2,10.2496677484646));
#223250=CARTESIAN_POINT('Ctrl Pts',(1.61966892470867,15.2,10.2514562343097));
#223251=CARTESIAN_POINT('Ctrl Pts',(1.62013662093202,15.2,10.2532978203482));
#223252=CARTESIAN_POINT('Ctrl Pts',(1.62060657262298,15.2,10.2551482874454));
#223253=CARTESIAN_POINT('Ctrl Pts',(1.62109605716988,15.2,10.2570523692153));
#223254=CARTESIAN_POINT('Ctrl Pts',(1.62160546180757,15.2,10.2590089854226));
#223255=CARTESIAN_POINT('Ctrl Pts',(1.62211486639899,15.2,10.2609656014523));
#223256=CARTESIAN_POINT('Ctrl Pts',(1.62264418692822,15.2,10.2629747533165));
#223257=CARTESIAN_POINT('Ctrl Pts',(1.62319380049157,15.2,10.2650353904916));
#223258=CARTESIAN_POINT('Ctrl Pts',(1.62374341405492,15.2,10.2670960276667));
#223259=CARTESIAN_POINT('Ctrl Pts',(1.62431331645265,15.2,10.2692081511476));
#223260=CARTESIAN_POINT('Ctrl Pts',(1.6249038679595,15.2,10.2713707423408));
#223261=CARTESIAN_POINT('Ctrl Pts',(1.62549441951999,15.2,10.2735333337305));
#223262=CARTESIAN_POINT('Ctrl Pts',(1.62610561697461,15.2,10.2757463899032));
#223263=CARTESIAN_POINT('Ctrl Pts',(1.62673780859382,15.2,10.2780089205299));
#223264=CARTESIAN_POINT('Ctrl Pts',(1.62737000015561,15.2,10.280271450951));
#223265=CARTESIAN_POINT('Ctrl Pts',(1.62802318434661,15.2,10.2825834561342));
#223266=CARTESIAN_POINT('Ctrl Pts',(1.62869769474188,15.2,10.2849439668093));
#223267=CARTESIAN_POINT('Ctrl Pts',(1.62937220513716,15.2,10.2873044774844));
#223268=CARTESIAN_POINT('Ctrl Pts',(1.63006804094624,15.2,10.2897134965992));
#223269=CARTESIAN_POINT('Ctrl Pts',(1.63078552516923,15.2,10.2921700810912));
#223270=CARTESIAN_POINT('Ctrl Pts',(1.63150300945739,15.2,10.2946266658064));
#223271=CARTESIAN_POINT('Ctrl Pts',(1.63224214013989,15.2,10.2971308160524));
#223272=CARTESIAN_POINT('Ctrl Pts',(1.63300322684954,15.2,10.299681613028));
#223273=CARTESIAN_POINT('Ctrl Pts',(1.63376431349005,15.2,10.3022324097718));
#223274=CARTESIAN_POINT('Ctrl Pts',(1.63454735977218,15.2,10.3048298539799));
#223275=CARTESIAN_POINT('Ctrl Pts',(1.63535266107722,15.2,10.3074730516358));
#223276=CARTESIAN_POINT('Ctrl Pts',(1.63629217931521,15.2,10.3105567823945));
#223277=CARTESIAN_POINT('Ctrl Pts',(1.63726199062046,15.2,10.3137027831072));
#223278=CARTESIAN_POINT('Ctrl Pts',(1.63826255556839,15.2,10.3169096742995));
#223279=CARTESIAN_POINT('Ctrl Pts',(1.6391201826221,15.2,10.319658438036));
#223280=CARTESIAN_POINT('Ctrl Pts',(1.64000040165602,15.2,10.3224519354642));
#223281=CARTESIAN_POINT('Ctrl Pts',(1.64090349104089,15.2,10.3252893184464));
#223282=CARTESIAN_POINT('Ctrl Pts',(1.64210761024805,15.2,10.3290724958419));
#223283=CARTESIAN_POINT('Ctrl Pts',(1.64335238876196,15.2,10.3329336878841));
#223284=CARTESIAN_POINT('Ctrl Pts',(1.64463846075034,15.2,10.3368709372929));
#223285=CARTESIAN_POINT('Ctrl Pts',(1.64560301471972,15.2,10.3398238742825));
#223286=CARTESIAN_POINT('Ctrl Pts',(1.64659079360766,15.2,10.3428195926301));
#223287=CARTESIAN_POINT('Ctrl Pts',(1.64760205565322,15.2,10.3458572888512));
#223288=CARTESIAN_POINT('Ctrl Pts',(1.64861331779063,15.2,10.3488949853482));
#223289=CARTESIAN_POINT('Ctrl Pts',(1.64964806011433,15.2,10.3519746593173));
#223290=CARTESIAN_POINT('Ctrl Pts',(1.65070653509028,15.2,10.3550955238234));
#223291=CARTESIAN_POINT('Ctrl Pts',(1.65176500997008,15.2,10.3582163880461));
#223292=CARTESIAN_POINT('Ctrl Pts',(1.65284721338551,15.2,10.3613784430697));
#223293=CARTESIAN_POINT('Ctrl Pts',(1.65395338651708,15.2,10.364580917468));
#223294=CARTESIAN_POINT('Ctrl Pts',(1.65524392190422,15.2,10.3683171377934));
#223295=CARTESIAN_POINT('Ctrl Pts',(1.65656708212579,15.2,10.3721083743684));
#223296=CARTESIAN_POINT('Ctrl Pts',(1.65792323434328,15.2,10.3759534308758));
#223297=CARTESIAN_POINT('Ctrl Pts',(1.65908565046937,15.2,10.3792491934255));
#223298=CARTESIAN_POINT('Ctrl Pts',(1.66027230438057,15.2,10.3825844995836));
#223299=CARTESIAN_POINT('Ctrl Pts',(1.66148342025879,15.2,10.3859586112265));
#223300=CARTESIAN_POINT('Ctrl Pts',(1.66269453613701,15.2,10.3893327228693));
#223301=CARTESIAN_POINT('Ctrl Pts',(1.66393011306989,15.2,10.3927456434142));
#223302=CARTESIAN_POINT('Ctrl Pts',(1.66519036593965,15.2,10.396196649037));
#223303=CARTESIAN_POINT('Ctrl Pts',(1.66645061892389,15.2,10.3996476549733));
#223304=CARTESIAN_POINT('Ctrl Pts',(1.66773554612792,15.2,10.4031367481145));
#223305=CARTESIAN_POINT('Ctrl Pts',(1.66904535911768,15.2,10.4066632228927));
#223306=CARTESIAN_POINT('Ctrl Pts',(1.67035517198846,15.2,10.4101896973504));
#223307=CARTESIAN_POINT('Ctrl Pts',(1.67168986849743,15.2,10.4137535505506));
#223308=CARTESIAN_POINT('Ctrl Pts',(1.67304964953245,15.2,10.4173540951713));
#223309=CARTESIAN_POINT('Ctrl Pts',(1.67440943056746,15.2,10.420954639792));
#223310=CARTESIAN_POINT('Ctrl Pts',(1.67579429731715,15.2,10.4245918722932));
#223311=CARTESIAN_POINT('Ctrl Pts',(1.67720444318149,15.2,10.4282651160749));
#223312=CARTESIAN_POINT('Ctrl Pts',(1.67861458904582,15.2,10.4319383598565));
#223313=CARTESIAN_POINT('Ctrl Pts',(1.68005001507881,15.2,10.4356476154802));
#223314=CARTESIAN_POINT('Ctrl Pts',(1.68151090785734,15.2,10.4393922153418));
#223315=CARTESIAN_POINT('Ctrl Pts',(1.68272831855034,15.2,10.4425127153398));
#223316=CARTESIAN_POINT('Ctrl Pts',(1.68396341538748,15.2,10.4456577605763));
#223317=CARTESIAN_POINT('Ctrl Pts',(1.68521630288603,15.2,10.4488269746021));
#223318=CARTESIAN_POINT('Ctrl Pts',(1.68646919038459,15.2,10.4519961886279));
#223319=CARTESIAN_POINT('Ctrl Pts',(1.6877398689539,15.2,10.4551895687675));
#223320=CARTESIAN_POINT('Ctrl Pts',(1.68902844214205,15.2,10.4584067439265));
#223321=CARTESIAN_POINT('Ctrl Pts',(1.69031701533019,15.2,10.4616239190857));
#223322=CARTESIAN_POINT('Ctrl Pts',(1.69162348135319,15.2,10.4648648897266));
#223323=CARTESIAN_POINT('Ctrl Pts',(1.69294794121339,15.2,10.4681292872949));
#223324=CARTESIAN_POINT('Ctrl Pts',(1.69427240107359,15.2,10.4713936848632));
#223325=CARTESIAN_POINT('Ctrl Pts',(1.69561485536754,15.2,10.4746815102126));
#223326=CARTESIAN_POINT('Ctrl Pts',(1.69697539939436,15.2,10.4779924020169));
#223327=CARTESIAN_POINT('Ctrl Pts',(1.69860805216722,15.2,10.4819654720377));
#223328=CARTESIAN_POINT('Ctrl Pts',(1.70026675567926,15.2,10.485971758042));
#223329=CARTESIAN_POINT('Ctrl Pts',(1.70195167228292,15.2,10.4900106450597));
#223330=CARTESIAN_POINT('Ctrl Pts',(1.70335576950365,15.2,10.4933763843634));
#223331=CARTESIAN_POINT('Ctrl Pts',(1.70477807125186,15.2,10.4967647642279));
#223332=CARTESIAN_POINT('Ctrl Pts',(1.70621866611148,15.2,10.5001754328372));
#223333=CARTESIAN_POINT('Ctrl Pts',(1.70765926097109,15.2,10.5035861014465));
#223334=CARTESIAN_POINT('Ctrl Pts',(1.70911815091707,15.2,10.5070190614112));
#223335=CARTESIAN_POINT('Ctrl Pts',(1.71059542404514,15.2,10.5104739667906));
#223336=CARTESIAN_POINT('Ctrl Pts',(1.71207269717321,15.2,10.51392887217));
#223337=CARTESIAN_POINT('Ctrl Pts',(1.71356835382412,15.2,10.5174057222056));
#223338=CARTESIAN_POINT('Ctrl Pts',(1.71508248014265,15.2,10.5209041782463));
#223339=CARTESIAN_POINT('Ctrl Pts',(1.71659660646118,15.2,10.5244026342869));
#223340=CARTESIAN_POINT('Ctrl Pts',(1.71812920147731,15.2,10.5279226946751));
#223341=CARTESIAN_POINT('Ctrl Pts',(1.71968035036523,15.2,10.5314640272435));
#223342=CARTESIAN_POINT('Ctrl Pts',(1.7215417289631,15.2,10.535713626171));
#223343=CARTESIAN_POINT('Ctrl Pts',(1.7234298242709,15.2,10.5399938533054));
#223344=CARTESIAN_POINT('Ctrl Pts',(1.72534477678284,15.2,10.5443041404801));
#223345=CARTESIAN_POINT('Ctrl Pts',(1.72694057060076,15.2,10.5478960465895));
#223346=CARTESIAN_POINT('Ctrl Pts',(1.72855501442117,15.2,10.5515088274653));
#223347=CARTESIAN_POINT('Ctrl Pts',(1.73018818754462,15.2,10.5551421577414));
#223348=CARTESIAN_POINT('Ctrl Pts',(1.73182136066807,15.2,10.5587754880174));
#223349=CARTESIAN_POINT('Ctrl Pts',(1.73347326351627,15.2,10.5624293675211));
#223350=CARTESIAN_POINT('Ctrl Pts',(1.7351439722647,15.2,10.5661034762694));
#223351=CARTESIAN_POINT('Ctrl Pts',(1.73681468101314,15.2,10.5697775850177));
#223352=CARTESIAN_POINT('Ctrl Pts',(1.73850419488427,15.2,10.573471922718));
#223353=CARTESIAN_POINT('Ctrl Pts',(1.74021258955164,15.2,10.5771861733188));
#223354=CARTESIAN_POINT('Ctrl Pts',(1.7422626632642,15.2,10.5816432742827));
#223355=CARTESIAN_POINT('Ctrl Pts',(1.74433992322938,15.2,10.5861290490857));
#223356=CARTESIAN_POINT('Ctrl Pts',(1.74644449501264,15.2,10.5906429597503));
#223357=CARTESIAN_POINT('Ctrl Pts',(1.74784754267698,15.2,10.5936522331167));
#223358=CARTESIAN_POINT('Ctrl Pts',(1.74926272992304,15.2,10.5966740105009));
#223359=CARTESIAN_POINT('Ctrl Pts',(1.75069008958332,15.2,10.599708135252));
#223360=CARTESIAN_POINT('Ctrl Pts',(1.75211744943807,15.2,10.6027422604165));
#223361=CARTESIAN_POINT('Ctrl Pts',(1.75355698539958,15.2,10.605788733165));
#223362=CARTESIAN_POINT('Ctrl Pts',(1.75500872871896,15.2,10.6088473966522));
#223363=CARTESIAN_POINT('Ctrl Pts',(1.75646047184052,15.2,10.6119060597227));
#223364=CARTESIAN_POINT('Ctrl Pts',(1.7579244248258,15.2,10.6149769138342));
#223365=CARTESIAN_POINT('Ctrl Pts',(1.75940061987099,15.2,10.618059805248));
#223366=CARTESIAN_POINT('Ctrl Pts',(1.76087681511732,15.2,10.6211426970819));
#223367=CARTESIAN_POINT('Ctrl Pts',(1.76236525520398,15.2,10.6242376254395));
#223368=CARTESIAN_POINT('Ctrl Pts',(1.7638659708977,15.2,10.627344438054));
#223369=CARTESIAN_POINT('Ctrl Pts',(1.7657418654126,15.2,10.6312279536106));
#223370=CARTESIAN_POINT('Ctrl Pts',(1.76763694155852,15.2,10.6351300377746));
#223371=CARTESIAN_POINT('Ctrl Pts',(1.76955126373886,15.2,10.6390503967218));
#223372=CARTESIAN_POINT('Ctrl Pts',(1.77108272135793,15.2,10.6421866836231));
#223373=CARTESIAN_POINT('Ctrl Pts',(1.77262649551749,15.2,10.6453346638175));
#223374=CARTESIAN_POINT('Ctrl Pts',(1.77418261838946,15.2,10.6484941912251));
#223375=CARTESIAN_POINT('Ctrl Pts',(1.77573874147345,15.2,10.6516537190632));
#223376=CARTESIAN_POINT('Ctrl Pts',(1.77730721299229,15.2,10.6548247907083));
#223377=CARTESIAN_POINT('Ctrl Pts',(1.77888806407925,15.2,10.6580072619936));
#223378=CARTESIAN_POINT('Ctrl Pts',(1.78086412783026,15.2,10.6619853508834));
#223379=CARTESIAN_POINT('Ctrl Pts',(1.78285953437075,15.2,10.6659812489754));
#223380=CARTESIAN_POINT('Ctrl Pts',(1.78487434245885,15.2,10.6699946697326));
#223381=CARTESIAN_POINT('Ctrl Pts',(1.78648618879755,15.2,10.6732054060759));
#223382=CARTESIAN_POINT('Ctrl Pts',(1.78811045181469,15.2,10.6764273569729));
#223383=CARTESIAN_POINT('Ctrl Pts',(1.78974716062455,15.2,10.6796603784858));
#223384=CARTESIAN_POINT('Ctrl Pts',(1.79138386965741,15.2,10.6828934004391));
#223385=CARTESIAN_POINT('Ctrl Pts',(1.79303302547503,15.2,10.6861374924019));
#223386=CARTESIAN_POINT('Ctrl Pts',(1.79469465517752,15.2,10.6893925105245));
#223387=CARTESIAN_POINT('Ctrl Pts',(1.79760250681729,15.2,10.6950887915737));
#223388=CARTESIAN_POINT('Ctrl Pts',(1.80054856028695,15.2,10.7008185365223));
#223389=CARTESIAN_POINT('Ctrl Pts',(1.80353296615441,15.2,10.7065809837032));
#223390=CARTESIAN_POINT('Ctrl Pts',(1.80566468476394,15.2,10.7106970176603));
#223391=CARTESIAN_POINT('Ctrl Pts',(1.80781596826203,15.2,10.7148297386586));
#223392=CARTESIAN_POINT('Ctrl Pts',(1.80998687173261,15.2,10.7189788719906));
#223393=CARTESIAN_POINT('Ctrl Pts',(1.81172359460372,15.2,10.722298178837));
#223394=CARTESIAN_POINT('Ctrl Pts',(1.81347287244424,15.2,10.7256279905661));
#223395=CARTESIAN_POINT('Ctrl Pts',(1.81523473149277,15.2,10.7289681679856));
#223396=CARTESIAN_POINT('Ctrl Pts',(1.81699659030124,15.2,10.7323083449499));
#223397=CARTESIAN_POINT('Ctrl Pts',(1.81877102999677,15.2,10.7356588894401));
#223398=CARTESIAN_POINT('Ctrl Pts',(1.82055807668272,15.2,10.7390196624421));
#223399=CARTESIAN_POINT('Ctrl Pts',(1.82279188522277,15.2,10.743220629038));
#223400=CARTESIAN_POINT('Ctrl Pts',(1.82504538995417,15.2,10.7474375800698));
#223401=CARTESIAN_POINT('Ctrl Pts',(1.82731864099423,15.2,10.7516702484713));
#223402=CARTESIAN_POINT('Ctrl Pts',(1.82959189203429,15.2,10.7559029168728));
#223403=CARTESIAN_POINT('Ctrl Pts',(1.83188488669511,15.2,10.7601513044209));
#223404=CARTESIAN_POINT('Ctrl Pts',(1.83419767298982,15.2,10.7644151495634));
#223405=CARTESIAN_POINT('Ctrl Pts',(1.83651045928452,15.2,10.7686789947058));
#223406=CARTESIAN_POINT('Ctrl Pts',(1.83884303493055,15.2,10.7729582973311));
#223407=CARTESIAN_POINT('Ctrl Pts',(1.84119544763783,15.2,10.7772527972608));
#223408=CARTESIAN_POINT('Ctrl Pts',(1.84354786034511,15.2,10.7815472971906));
#223409=CARTESIAN_POINT('Ctrl Pts',(1.84592010702239,15.2,10.7858569951569));
#223410=CARTESIAN_POINT('Ctrl Pts',(1.84831223236857,15.2,10.7901816352255));
#223411=CARTESIAN_POINT('Ctrl Pts',(1.85022593274982,15.2,10.793641347469));
#223412=CARTESIAN_POINT('Ctrl Pts',(1.85215235603877,15.2,10.7971106232378));
#223413=CARTESIAN_POINT('Ctrl Pts',(1.85409152179802,15.2,10.8005893322131));
#223414=CARTESIAN_POINT('Ctrl Pts',(1.85603068729305,15.2,10.8040680407145));
#223415=CARTESIAN_POINT('Ctrl Pts',(1.85798259600919,15.2,10.8075561819118));
#223416=CARTESIAN_POINT('Ctrl Pts',(1.85994726934773,15.2,10.8110536281808));
#223417=CARTESIAN_POINT('Ctrl Pts',(1.86289427975707,15.2,10.8162997982991));
#223418=CARTESIAN_POINT('Ctrl Pts',(1.86587000840336,15.2,10.8215669023867));
#223419=CARTESIAN_POINT('Ctrl Pts',(1.86887452481906,15.2,10.826854511843));
#223420=CARTESIAN_POINT('Ctrl Pts',(1.87087753548994,15.2,10.8303795843335));
#223421=CARTESIAN_POINT('Ctrl Pts',(1.87289333909252,15.2,10.8339137703478));
#223422=CARTESIAN_POINT('Ctrl Pts',(1.8749219570925,15.2,10.837456944002));
#223423=CARTESIAN_POINT('Ctrl Pts',(1.87745772979979,15.2,10.8418859114318));
#223424=CARTESIAN_POINT('Ctrl Pts',(1.88001352413129,15.2,10.8463289210273));
#223425=CARTESIAN_POINT('Ctrl Pts',(1.88258937449016,15.2,10.8507857302142));
#223426=CARTESIAN_POINT('Ctrl Pts',(1.88465005488956,15.2,10.854351177758));
#223427=CARTESIAN_POINT('Ctrl Pts',(1.88672357302046,15.2,10.8579254567091));
#223428=CARTESIAN_POINT('Ctrl Pts',(1.88880994535769,15.2,10.8615084436274));
#223429=CARTESIAN_POINT('Ctrl Pts',(1.89141791063708,15.2,10.8659871770313));
#223430=CARTESIAN_POINT('Ctrl Pts',(1.89404596208352,15.2,10.8704795155104));
#223431=CARTESIAN_POINT('Ctrl Pts',(1.89669413236295,15.2,10.874985220581));
#223432=CARTESIAN_POINT('Ctrl Pts',(1.8988126684133,15.2,10.8785897843427));
#223433=CARTESIAN_POINT('Ctrl Pts',(1.90094408130573,15.2,10.8822029034549));
#223434=CARTESIAN_POINT('Ctrl Pts',(1.90308838797343,15.2,10.8858244547308));
#223435=CARTESIAN_POINT('Ctrl Pts',(1.9052326949333,15.2,10.8894460065001));
#223436=CARTESIAN_POINT('Ctrl Pts',(1.9073898954907,15.2,10.8930759914985));
#223437=CARTESIAN_POINT('Ctrl Pts',(1.90956000638805,15.2,10.8967142890865));
#223438=CARTESIAN_POINT('Ctrl Pts',(1.91173011698973,15.2,10.9003525861788));
#223439=CARTESIAN_POINT('Ctrl Pts',(1.91391313647585,15.2,10.9039991972922));
#223440=CARTESIAN_POINT('Ctrl Pts',(1.9161090817955,15.2,10.9076540004929));
#223441=CARTESIAN_POINT('Ctrl Pts',(1.91885401366945,15.2,10.9122225048673));
#223442=CARTESIAN_POINT('Ctrl Pts',(1.92161914179689,15.2,10.9168038111933));
#223443=CARTESIAN_POINT('Ctrl Pts',(1.92440449694837,15.2,10.9213976872558));
#223444=CARTESIAN_POINT('Ctrl Pts',(1.92718985209986,15.2,10.9259915633183));
#223445=CARTESIAN_POINT('Ctrl Pts',(1.92999543321655,15.2,10.9305980101166));
#223446=CARTESIAN_POINT('Ctrl Pts',(1.93282126925822,15.2,10.9352167992833));
#223447=CARTESIAN_POINT('Ctrl Pts',(1.93621227238501,15.2,10.9407593460819));
#223448=CARTESIAN_POINT('Ctrl Pts',(1.9396324417793,15.2,10.9463196623104));
#223449=CARTESIAN_POINT('Ctrl Pts',(1.94308182690795,15.2,10.9518973604688));
#223450=CARTESIAN_POINT('Ctrl Pts',(1.94538141720259,15.2,10.9556158262454));
#223451=CARTESIAN_POINT('Ctrl Pts',(1.94769399160979,15.2,10.9593420144208));
#223452=CARTESIAN_POINT('Ctrl Pts',(1.9500195626818,15.2,10.9630758140136));
#223453=CARTESIAN_POINT('Ctrl Pts',(1.95292652636337,15.2,10.9677430632503));
#223454=CARTESIAN_POINT('Ctrl Pts',(1.95585379938614,15.2,10.9724222024006));
#223455=CARTESIAN_POINT('Ctrl Pts',(1.95880140619279,15.2,10.9771130077485));
#223456=CARTESIAN_POINT('Ctrl Pts',(1.96115949144534,15.2,10.98086565172));
#223457=CARTESIAN_POINT('Ctrl Pts',(1.96353058975313,15.2,10.9846257640681));
#223458=CARTESIAN_POINT('Ctrl Pts',(1.96591471445402,15.2,10.98839323017));
#223459=CARTESIAN_POINT('Ctrl Pts',(1.96770280806089,15.2,10.9912188298747));
#223460=CARTESIAN_POINT('Ctrl Pts',(1.9694982288234,15.2,10.9940485663524));
#223461=CARTESIAN_POINT('Ctrl Pts',(1.97130098138189,15.2,10.9968823923322));
#223462=CARTESIAN_POINT('Ctrl Pts',(1.9737046516782,15.2,11.0006608273151));
#223463=CARTESIAN_POINT('Ctrl Pts',(1.97612135720634,15.2,11.0044465323071));
#223464=CARTESIAN_POINT('Ctrl Pts',(1.97855110878322,15.2,11.0082393954583));
#223465=CARTESIAN_POINT('Ctrl Pts',(1.98037342230036,15.2,11.0110840425633));
#223466=CARTESIAN_POINT('Ctrl Pts',(1.98220307440052,15.2,11.0139327167931));
#223467=CARTESIAN_POINT('Ctrl Pts',(1.98404007033311,15.2,11.0167853703974));
#223468=CARTESIAN_POINT('Ctrl Pts',(1.98587706626569,15.2,11.0196380240017));
#223469=CARTESIAN_POINT('Ctrl Pts',(1.98772140465066,15.2,11.022494658708));
#223470=CARTESIAN_POINT('Ctrl Pts',(1.98957309171671,15.2,11.0253552259549));
#223471=CARTESIAN_POINT('Ctrl Pts',(1.99142477878276,15.2,11.0282157932017));
#223472=CARTESIAN_POINT('Ctrl Pts',(1.99328381306184,15.2,11.0310802940961));
#223473=CARTESIAN_POINT('Ctrl Pts',(1.99515020007635,15.2,11.0339486825746));
#223474=CARTESIAN_POINT('Ctrl Pts',(1.99763871632174,15.2,11.0377732008935));
#223475=CARTESIAN_POINT('Ctrl Pts',(2.00014030328227,15.2,11.0416046292546));
#223476=CARTESIAN_POINT('Ctrl Pts',(2.00265497147489,15.2,11.0454428597416));
#223477=CARTESIAN_POINT('Ctrl Pts',(2.00454097244804,15.2,11.0483215323454));
#223478=CARTESIAN_POINT('Ctrl Pts',(2.00643433137921,15.2,11.051204031624));
#223479=CARTESIAN_POINT('Ctrl Pts',(2.00833505235117,15.2,11.0540903106854));
#223480=CARTESIAN_POINT('Ctrl Pts',(2.01023577332312,15.2,11.0569765897469));
#223481=CARTESIAN_POINT('Ctrl Pts',(2.01214385577079,15.2,11.0598666490178));
#223482=CARTESIAN_POINT('Ctrl Pts',(2.01405930537938,15.2,11.0627604437235));
#223483=CARTESIAN_POINT('Ctrl Pts',(2.01597475498796,15.2,11.0656542384291));
#223484=CARTESIAN_POINT('Ctrl Pts',(2.01789757131692,15.2,11.0685517685401));
#223485=CARTESIAN_POINT('Ctrl Pts',(2.01982775682912,15.2,11.0714529881425));
#223486=CARTESIAN_POINT('Ctrl Pts',(2.02175794269196,15.2,11.074354208272));
#223487=CARTESIAN_POINT('Ctrl Pts',(2.02369549805691,15.2,11.0772591182608));
#223488=CARTESIAN_POINT('Ctrl Pts',(2.0256404274239,15.2,11.0801676733507));
#223489=CARTESIAN_POINT('Ctrl Pts',(2.02758535643756,15.2,11.0830762279122));
#223490=CARTESIAN_POINT('Ctrl Pts',(2.02953765950087,15.2,11.0859884273068));
#223491=CARTESIAN_POINT('Ctrl Pts',(2.03149733993029,15.2,11.0889042273262));
#223492=CARTESIAN_POINT('Ctrl Pts',(2.03345702035971,15.2,11.0918200273455));
#223493=CARTESIAN_POINT('Ctrl Pts',(2.03542407678109,15.2,11.0947394272122));
#223494=CARTESIAN_POINT('Ctrl Pts',(2.03739851526002,15.2,11.0976623837443));
#223495=CARTESIAN_POINT('Ctrl Pts',(2.04003109977905,15.2,11.1015596589434));
#223496=CARTESIAN_POINT('Ctrl Pts',(2.04267680732835,15.2,11.1054632552255));
#223497=CARTESIAN_POINT('Ctrl Pts',(2.04533564133184,15.2,11.1093730691274));
#223498=CARTESIAN_POINT('Ctrl Pts',(2.0473297672873,15.2,11.1123054302197));
#223499=CARTESIAN_POINT('Ctrl Pts',(2.04933127974491,15.2,11.1152412879131));
#223500=CARTESIAN_POINT('Ctrl Pts',(2.05134017970451,15.2,11.1181805985907));
#223501=CARTESIAN_POINT('Ctrl Pts',(2.05468834581724,15.2,11.1230794490081));
#223502=CARTESIAN_POINT('Ctrl Pts',(2.05805703619151,15.2,11.1279878930202));
#223503=CARTESIAN_POINT('Ctrl Pts',(2.06144626369321,15.2,11.1329057267015));
#223504=CARTESIAN_POINT('Ctrl Pts',(2.06347980012034,15.2,11.1358564268031));
#223505=CARTESIAN_POINT('Ctrl Pts',(2.06552072958039,15.2,11.1388105082295));
#223506=CARTESIAN_POINT('Ctrl Pts',(2.06756905596495,15.2,11.1417679263307));
#223507=CARTESIAN_POINT('Ctrl Pts',(2.06961738234951,15.2,11.1447253444319));
#223508=CARTESIAN_POINT('Ctrl Pts',(2.07167310385066,15.2,11.1476860990135));
#223509=CARTESIAN_POINT('Ctrl Pts',(2.07373622524344,15.2,11.1506501490027));
#223510=CARTESIAN_POINT('Ctrl Pts',(2.07648705364221,15.2,11.1546022154753));
#223511=CARTESIAN_POINT('Ctrl Pts',(2.07925103579924,15.2,11.1585601375099));
#223512=CARTESIAN_POINT('Ctrl Pts',(2.08202817707083,15.2,11.1625238148519));
#223513=CARTESIAN_POINT('Ctrl Pts',(2.08480531872081,15.2,11.1664874927339));
#223514=CARTESIAN_POINT('Ctrl Pts',(2.08759562165266,15.2,11.1704569258472));
#223515=CARTESIAN_POINT('Ctrl Pts',(2.09039908924989,15.2,11.1744320130083));
#223516=CARTESIAN_POINT('Ctrl Pts',(2.09250168975683,15.2,11.1774133281083));
#223517=CARTESIAN_POINT('Ctrl Pts',(2.09461169628014,15.2,11.1803978233499));
#223518=CARTESIAN_POINT('Ctrl Pts',(2.09672911028588,15.2,11.1833854579077));
#223519=CARTESIAN_POINT('Ctrl Pts',(2.09955232921665,15.2,11.1873689710133));
#223520=CARTESIAN_POINT('Ctrl Pts',(2.10238871890352,15.2,11.1913580627424));
#223521=CARTESIAN_POINT('Ctrl Pts',(2.1052382826468,15.2,11.1953526341046));
#223522=CARTESIAN_POINT('Ctrl Pts',(2.10880023713176,15.2,11.2003458480353));
#223523=CARTESIAN_POINT('Ctrl Pts',(2.11238277735841,15.2,11.2053476223102));
#223524=CARTESIAN_POINT('Ctrl Pts',(2.11598591242953,15.2,11.2103577661303));
#223525=CARTESIAN_POINT('Ctrl Pts',(2.11814779339365,15.2,11.2133638523132));
#223526=CARTESIAN_POINT('Ctrl Pts',(2.12031708914906,15.2,11.2163729525875));
#223527=CARTESIAN_POINT('Ctrl Pts',(2.12249380057062,15.2,11.2193850238117));
#223528=CARTESIAN_POINT('Ctrl Pts',(2.12467051199217,15.2,11.2223970950358));
#223529=CARTESIAN_POINT('Ctrl Pts',(2.12685463905486,15.2,11.2254121393153));
#223530=CARTESIAN_POINT('Ctrl Pts',(2.12904618402689,15.2,11.2284301124694));
#223531=CARTESIAN_POINT('Ctrl Pts',(2.13196824385688,15.2,11.232454076492));
#223532=CARTESIAN_POINT('Ctrl Pts',(2.13490349065741,15.2,11.2364832474706));
#223533=CARTESIAN_POINT('Ctrl Pts',(2.13785192902616,15.2,11.240517528807));
#223534=CARTESIAN_POINT('Ctrl Pts',(2.14006325830488,15.2,11.2435432404964));
#223535=CARTESIAN_POINT('Ctrl Pts',(2.14228200674397,15.2,11.2465718269698));
#223536=CARTESIAN_POINT('Ctrl Pts',(2.14450817702687,15.2,11.2496032516608));
#223537=CARTESIAN_POINT('Ctrl Pts',(2.14673434690535,15.2,11.2526346758011));
#223538=CARTESIAN_POINT('Ctrl Pts',(2.14896793737503,15.2,11.2556689386578));
#223539=CARTESIAN_POINT('Ctrl Pts',(2.15120895125263,15.2,11.2587059980894));
#223540=CARTESIAN_POINT('Ctrl Pts',(2.15344996513022,15.2,11.261743057521));
#223541=CARTESIAN_POINT('Ctrl Pts',(2.15569840080699,15.2,11.2647829118161));
#223542=CARTESIAN_POINT('Ctrl Pts',(2.15795426127694,15.2,11.2678255123027));
#223543=CARTESIAN_POINT('Ctrl Pts',(2.16021012174689,15.2,11.2708681127893));
#223544=CARTESIAN_POINT('Ctrl Pts',(2.16247340780339,15.2,11.2739134570108));
#223545=CARTESIAN_POINT('Ctrl Pts',(2.16474411827283,15.2,11.2769615095389));
#223546=CARTESIAN_POINT('Ctrl Pts',(2.16852863585938,15.2,11.2820415972702));
#223547=CARTESIAN_POINT('Ctrl Pts',(2.17233377790013,15.2,11.2871292040928));
#223548=CARTESIAN_POINT('Ctrl Pts',(2.17615954699994,15.2,11.292224299));
#223549=CARTESIAN_POINT('Origin',(-5.66257110645729E-14,15.2,-1.77635683940025E-14));
#223550=CARTESIAN_POINT('',(1.18690176598713,15.2,10.306885524222));
#223551=CARTESIAN_POINT('',(1.18690176598713,12.2,10.306885524222));
#223552=CARTESIAN_POINT('',(1.18690176599994,15.2,10.306885524));
#223553=CARTESIAN_POINT('Origin',(-5.66257110645729E-14,12.2,-1.77635683940025E-14));
#223554=CARTESIAN_POINT('Origin',(-5.66257110645729E-14,15.2,-1.77635683940025E-14));
#223555=CARTESIAN_POINT('Origin',(-5.66257110645729E-14,15.2,-1.77635683940025E-14));
#223556=CARTESIAN_POINT('',(0.929795807999944,15.2,11.462350534));
#223557=CARTESIAN_POINT('',(0.546958305999944,15.2,11.486985532));
#223558=CARTESIAN_POINT('Origin',(-5.66257110645729E-14,15.2,-1.77635683940025E-14));
#223559=CARTESIAN_POINT('',(0.546958305999944,12.2,11.486985532));
#223560=CARTESIAN_POINT('',(0.546958305999944,15.2,11.486985532));
#223561=CARTESIAN_POINT('',(0.929795807999944,12.2,11.462350534));
#223562=CARTESIAN_POINT('Origin',(-5.66257110645729E-14,12.2,-1.77635683940025E-14));
#223563=CARTESIAN_POINT('',(0.929795807999944,15.2,11.462350534));
#223564=CARTESIAN_POINT('Ctrl Pts',(0.546958305999944,15.2,11.486985532));
#223565=CARTESIAN_POINT('Ctrl Pts',(0.546958305999944,11.6,11.486985532));
#223566=CARTESIAN_POINT('Ctrl Pts',(0.546590898999945,15.2,11.486315008));
#223567=CARTESIAN_POINT('Ctrl Pts',(0.546590898999945,11.6,11.486315008));
#223568=CARTESIAN_POINT('Ctrl Pts',(0.545856550999945,15.2,11.484974209));
#223569=CARTESIAN_POINT('Ctrl Pts',(0.545856550999945,11.6,11.484974209));
#223570=CARTESIAN_POINT('Ctrl Pts',(0.544756420999944,15.2,11.482963756));
#223571=CARTESIAN_POINT('Ctrl Pts',(0.544756420999944,11.6,11.482963756));
#223572=CARTESIAN_POINT('Ctrl Pts',(0.543292368999944,15.2,11.480284644));
#223573=CARTESIAN_POINT('Ctrl Pts',(0.543292368999944,11.6,11.480284644));
#223574=CARTESIAN_POINT('Ctrl Pts',(0.541466945999944,15.2,11.476938237));
#223575=CARTESIAN_POINT('Ctrl Pts',(0.541466945999944,11.6,11.476938237));
#223576=CARTESIAN_POINT('Ctrl Pts',(0.539646165999944,15.2,11.473594318));
#223577=CARTESIAN_POINT('Ctrl Pts',(0.539646165999944,11.6,11.473594318));
#223578=CARTESIAN_POINT('Ctrl Pts',(0.537830029999945,15.2,11.470252887));
#223579=CARTESIAN_POINT('Ctrl Pts',(0.537830029999945,11.6,11.470252887));
#223580=CARTESIAN_POINT('Ctrl Pts',(0.536018536999944,15.2,11.466913949));
#223581=CARTESIAN_POINT('Ctrl Pts',(0.536018536999944,11.6,11.466913949));
#223582=CARTESIAN_POINT('Ctrl Pts',(0.534211683999944,15.2,11.46357751));
#223583=CARTESIAN_POINT('Ctrl Pts',(0.534211683999944,11.6,11.46357751));
#223584=CARTESIAN_POINT('Ctrl Pts',(0.532409473999944,15.2,11.460243578));
#223585=CARTESIAN_POINT('Ctrl Pts',(0.532409473999944,11.6,11.460243578));
#223586=CARTESIAN_POINT('Ctrl Pts',(0.530611901999943,15.2,11.456912161));
#223587=CARTESIAN_POINT('Ctrl Pts',(0.530611901999943,11.6,11.456912161));
#223588=CARTESIAN_POINT('Ctrl Pts',(0.528818964999944,15.2,11.453583273));
#223589=CARTESIAN_POINT('Ctrl Pts',(0.528818964999944,11.6,11.453583273));
#223590=CARTESIAN_POINT('Ctrl Pts',(0.527030663999944,15.2,11.450256921));
#223591=CARTESIAN_POINT('Ctrl Pts',(0.527030663999944,11.6,11.450256921));
#223592=CARTESIAN_POINT('Ctrl Pts',(0.525246995999944,15.2,11.446933119));
#223593=CARTESIAN_POINT('Ctrl Pts',(0.525246995999944,11.6,11.446933119));
#223594=CARTESIAN_POINT('Ctrl Pts',(0.523467958999944,15.2,11.443611876));
#223595=CARTESIAN_POINT('Ctrl Pts',(0.523467958999944,11.6,11.443611876));
#223596=CARTESIAN_POINT('Ctrl Pts',(0.521693550999944,15.2,11.440293201));
#223597=CARTESIAN_POINT('Ctrl Pts',(0.521693550999944,11.6,11.440293201));
#223598=CARTESIAN_POINT('Ctrl Pts',(0.519923770999945,15.2,11.436977102));
#223599=CARTESIAN_POINT('Ctrl Pts',(0.519923770999945,11.6,11.436977102));
#223600=CARTESIAN_POINT('Ctrl Pts',(0.518158616999944,15.2,11.43366359));
#223601=CARTESIAN_POINT('Ctrl Pts',(0.518158616999944,11.6,11.43366359));
#223602=CARTESIAN_POINT('Ctrl Pts',(0.516398088999944,15.2,11.43035267));
#223603=CARTESIAN_POINT('Ctrl Pts',(0.516398088999944,11.6,11.43035267));
#223604=CARTESIAN_POINT('Ctrl Pts',(0.514642183999944,15.2,11.427044351));
#223605=CARTESIAN_POINT('Ctrl Pts',(0.514642183999944,11.6,11.427044351));
#223606=CARTESIAN_POINT('Ctrl Pts',(0.512890899999944,15.2,11.423738642));
#223607=CARTESIAN_POINT('Ctrl Pts',(0.512890899999944,11.6,11.423738642));
#223608=CARTESIAN_POINT('Ctrl Pts',(0.511144237999944,15.2,11.420435552));
#223609=CARTESIAN_POINT('Ctrl Pts',(0.511144237999944,11.6,11.420435552));
#223610=CARTESIAN_POINT('Ctrl Pts',(0.509402193999944,15.2,11.417135088));
#223611=CARTESIAN_POINT('Ctrl Pts',(0.509402193999944,11.6,11.417135088));
#223612=CARTESIAN_POINT('Ctrl Pts',(0.507664765999943,15.2,11.413837262));
#223613=CARTESIAN_POINT('Ctrl Pts',(0.507664765999943,11.6,11.413837262));
#223614=CARTESIAN_POINT('Ctrl Pts',(0.505931953999944,15.2,11.410542081));
#223615=CARTESIAN_POINT('Ctrl Pts',(0.505931953999944,11.6,11.410542081));
#223616=CARTESIAN_POINT('Ctrl Pts',(0.504203755999945,15.2,11.407249557));
#223617=CARTESIAN_POINT('Ctrl Pts',(0.504203755999945,11.6,11.407249557));
#223618=CARTESIAN_POINT('Ctrl Pts',(0.502480167999945,15.2,11.403959697));
#223619=CARTESIAN_POINT('Ctrl Pts',(0.502480167999945,11.6,11.403959697));
#223620=CARTESIAN_POINT('Ctrl Pts',(0.500761191999944,15.2,11.400672511));
#223621=CARTESIAN_POINT('Ctrl Pts',(0.500761191999944,11.6,11.400672511));
#223622=CARTESIAN_POINT('Ctrl Pts',(0.499046822999943,15.2,11.397388008));
#223623=CARTESIAN_POINT('Ctrl Pts',(0.499046822999943,11.6,11.397388008));
#223624=CARTESIAN_POINT('Ctrl Pts',(0.497337059999945,15.2,11.394106196));
#223625=CARTESIAN_POINT('Ctrl Pts',(0.497337059999945,11.6,11.394106196));
#223626=CARTESIAN_POINT('Ctrl Pts',(0.495631902999945,15.2,11.390827085));
#223627=CARTESIAN_POINT('Ctrl Pts',(0.495631902999945,11.6,11.390827085));
#223628=CARTESIAN_POINT('Ctrl Pts',(0.493931348999944,15.2,11.387550685));
#223629=CARTESIAN_POINT('Ctrl Pts',(0.493931348999944,11.6,11.387550685));
#223630=CARTESIAN_POINT('Ctrl Pts',(0.492235395999945,15.2,11.384277002));
#223631=CARTESIAN_POINT('Ctrl Pts',(0.492235395999945,11.6,11.384277002));
#223632=CARTESIAN_POINT('Ctrl Pts',(0.490544042999945,15.2,11.381006048));
#223633=CARTESIAN_POINT('Ctrl Pts',(0.490544042999945,11.6,11.381006048));
#223634=CARTESIAN_POINT('Ctrl Pts',(0.488857286999943,15.2,11.37773783));
#223635=CARTESIAN_POINT('Ctrl Pts',(0.488857286999943,11.6,11.37773783));
#223636=CARTESIAN_POINT('Ctrl Pts',(0.487175127999944,15.2,11.374472358));
#223637=CARTESIAN_POINT('Ctrl Pts',(0.487175127999944,11.6,11.374472358));
#223638=CARTESIAN_POINT('Ctrl Pts',(0.485497562999945,15.2,11.371209642));
#223639=CARTESIAN_POINT('Ctrl Pts',(0.485497562999945,11.6,11.371209642));
#223640=CARTESIAN_POINT('Ctrl Pts',(0.483824590999945,15.2,11.36794969));
#223641=CARTESIAN_POINT('Ctrl Pts',(0.483824590999945,11.6,11.36794969));
#223642=CARTESIAN_POINT('Ctrl Pts',(0.482156208999944,15.2,11.364692512));
#223643=CARTESIAN_POINT('Ctrl Pts',(0.482156208999944,11.6,11.364692512));
#223644=CARTESIAN_POINT('Ctrl Pts',(0.480492415999944,15.2,11.361438117));
#223645=CARTESIAN_POINT('Ctrl Pts',(0.480492415999944,11.6,11.361438117));
#223646=CARTESIAN_POINT('Ctrl Pts',(0.478833209999945,15.2,11.358186515));
#223647=CARTESIAN_POINT('Ctrl Pts',(0.478833209999945,11.6,11.358186515));
#223648=CARTESIAN_POINT('Ctrl Pts',(0.477178588999945,15.2,11.354937714));
#223649=CARTESIAN_POINT('Ctrl Pts',(0.477178588999945,11.6,11.354937714));
#223650=CARTESIAN_POINT('Ctrl Pts',(0.475528549999943,15.2,11.351691724));
#223651=CARTESIAN_POINT('Ctrl Pts',(0.475528549999943,11.6,11.351691724));
#223652=CARTESIAN_POINT('Ctrl Pts',(0.473883093999945,15.2,11.348448553));
#223653=CARTESIAN_POINT('Ctrl Pts',(0.473883093999945,11.6,11.348448553));
#223654=CARTESIAN_POINT('Ctrl Pts',(0.472242216999945,15.2,11.345208212));
#223655=CARTESIAN_POINT('Ctrl Pts',(0.472242216999945,11.6,11.345208212));
#223656=CARTESIAN_POINT('Ctrl Pts',(0.470605917999943,15.2,11.34197071));
#223657=CARTESIAN_POINT('Ctrl Pts',(0.470605917999943,11.6,11.34197071));
#223658=CARTESIAN_POINT('Ctrl Pts',(0.468974193999945,15.2,11.338736055));
#223659=CARTESIAN_POINT('Ctrl Pts',(0.468974193999945,11.6,11.338736055));
#223660=CARTESIAN_POINT('Ctrl Pts',(0.467347043999944,15.2,11.335504256));
#223661=CARTESIAN_POINT('Ctrl Pts',(0.467347043999944,11.6,11.335504256));
#223662=CARTESIAN_POINT('Ctrl Pts',(0.465724464999945,15.2,11.332275324));
#223663=CARTESIAN_POINT('Ctrl Pts',(0.465724464999945,11.6,11.332275324));
#223664=CARTESIAN_POINT('Ctrl Pts',(0.464106456999945,15.2,11.329049269));
#223665=CARTESIAN_POINT('Ctrl Pts',(0.464106456999945,11.6,11.329049269));
#223666=CARTESIAN_POINT('Ctrl Pts',(0.462493016999945,15.2,11.325826099));
#223667=CARTESIAN_POINT('Ctrl Pts',(0.462493016999945,11.6,11.325826099));
#223668=CARTESIAN_POINT('Ctrl Pts',(0.460884141999944,15.2,11.322605823));
#223669=CARTESIAN_POINT('Ctrl Pts',(0.460884141999944,11.6,11.322605823));
#223670=CARTESIAN_POINT('Ctrl Pts',(0.459279831999944,15.2,11.319388451));
#223671=CARTESIAN_POINT('Ctrl Pts',(0.459279831999944,11.6,11.319388451));
#223672=CARTESIAN_POINT('Ctrl Pts',(0.457680083999945,15.2,11.316173992));
#223673=CARTESIAN_POINT('Ctrl Pts',(0.457680083999945,11.6,11.316173992));
#223674=CARTESIAN_POINT('Ctrl Pts',(0.456084895999943,15.2,11.312962457));
#223675=CARTESIAN_POINT('Ctrl Pts',(0.456084895999943,11.6,11.312962457));
#223676=CARTESIAN_POINT('Ctrl Pts',(0.454494264999944,15.2,11.309753854));
#223677=CARTESIAN_POINT('Ctrl Pts',(0.454494264999944,11.6,11.309753854));
#223678=CARTESIAN_POINT('Ctrl Pts',(0.452908190999944,15.2,11.306548191));
#223679=CARTESIAN_POINT('Ctrl Pts',(0.452908190999944,11.6,11.306548191));
#223680=CARTESIAN_POINT('Ctrl Pts',(0.451326669999944,15.2,11.303345481));
#223681=CARTESIAN_POINT('Ctrl Pts',(0.451326669999944,11.6,11.303345481));
#223682=CARTESIAN_POINT('Ctrl Pts',(0.449749701999943,15.2,11.300145732));
#223683=CARTESIAN_POINT('Ctrl Pts',(0.449749701999943,11.6,11.300145732));
#223684=CARTESIAN_POINT('Ctrl Pts',(0.448177283999945,15.2,11.296948952));
#223685=CARTESIAN_POINT('Ctrl Pts',(0.448177283999945,11.6,11.296948952));
#223686=CARTESIAN_POINT('Ctrl Pts',(0.446609412999944,15.2,11.293755151));
#223687=CARTESIAN_POINT('Ctrl Pts',(0.446609412999944,11.6,11.293755151));
#223688=CARTESIAN_POINT('Ctrl Pts',(0.445046087999945,15.2,11.290564341));
#223689=CARTESIAN_POINT('Ctrl Pts',(0.445046087999945,11.6,11.290564341));
#223690=CARTESIAN_POINT('Ctrl Pts',(0.443487306999945,15.2,11.287376529));
#223691=CARTESIAN_POINT('Ctrl Pts',(0.443487306999945,11.6,11.287376529));
#223692=CARTESIAN_POINT('Ctrl Pts',(0.441933066999944,15.2,11.284191726));
#223693=CARTESIAN_POINT('Ctrl Pts',(0.441933066999944,11.6,11.284191726));
#223694=CARTESIAN_POINT('Ctrl Pts',(0.440383366999945,15.2,11.28100994));
#223695=CARTESIAN_POINT('Ctrl Pts',(0.440383366999945,11.6,11.28100994));
#223696=CARTESIAN_POINT('Ctrl Pts',(0.438838203999945,15.2,11.277831182));
#223697=CARTESIAN_POINT('Ctrl Pts',(0.438838203999945,11.6,11.277831182));
#223698=CARTESIAN_POINT('Ctrl Pts',(0.437297575999944,15.2,11.27465546));
#223699=CARTESIAN_POINT('Ctrl Pts',(0.437297575999944,11.6,11.27465546));
#223700=CARTESIAN_POINT('Ctrl Pts',(0.435761481999943,15.2,11.271482787));
#223701=CARTESIAN_POINT('Ctrl Pts',(0.435761481999943,11.6,11.271482787));
#223702=CARTESIAN_POINT('Ctrl Pts',(0.434229916999945,15.2,11.268313168));
#223703=CARTESIAN_POINT('Ctrl Pts',(0.434229916999945,11.6,11.268313168));
#223704=CARTESIAN_POINT('Ctrl Pts',(0.432702881999945,15.2,11.265146617));
#223705=CARTESIAN_POINT('Ctrl Pts',(0.432702881999945,11.6,11.265146617));
#223706=CARTESIAN_POINT('Ctrl Pts',(0.431180373999943,15.2,11.261983142));
#223707=CARTESIAN_POINT('Ctrl Pts',(0.431180373999943,11.6,11.261983142));
#223708=CARTESIAN_POINT('Ctrl Pts',(0.429662389999944,15.2,11.258822751));
#223709=CARTESIAN_POINT('Ctrl Pts',(0.429662389999944,11.6,11.258822751));
#223710=CARTESIAN_POINT('Ctrl Pts',(0.428148927999944,15.2,11.255665455));
#223711=CARTESIAN_POINT('Ctrl Pts',(0.428148927999944,11.6,11.255665455));
#223712=CARTESIAN_POINT('Ctrl Pts',(0.426639985999945,15.2,11.252511265));
#223713=CARTESIAN_POINT('Ctrl Pts',(0.426639985999945,11.6,11.252511265));
#223714=CARTESIAN_POINT('Ctrl Pts',(0.425135560999944,15.2,11.249360189));
#223715=CARTESIAN_POINT('Ctrl Pts',(0.425135560999944,11.6,11.249360189));
#223716=CARTESIAN_POINT('Ctrl Pts',(0.423635651999945,15.2,11.246212238));
#223717=CARTESIAN_POINT('Ctrl Pts',(0.423635651999945,11.6,11.246212238));
#223718=CARTESIAN_POINT('Ctrl Pts',(0.422140256999944,15.2,11.24306742));
#223719=CARTESIAN_POINT('Ctrl Pts',(0.422140256999944,11.6,11.24306742));
#223720=CARTESIAN_POINT('Ctrl Pts',(0.420649371999945,15.2,11.239925747));
#223721=CARTESIAN_POINT('Ctrl Pts',(0.420649371999945,11.6,11.239925747));
#223722=CARTESIAN_POINT('Ctrl Pts',(0.419162995999944,15.2,11.236787228));
#223723=CARTESIAN_POINT('Ctrl Pts',(0.419162995999944,11.6,11.236787228));
#223724=CARTESIAN_POINT('Ctrl Pts',(0.417681126999945,15.2,11.233651872));
#223725=CARTESIAN_POINT('Ctrl Pts',(0.417681126999945,11.6,11.233651872));
#223726=CARTESIAN_POINT('Ctrl Pts',(0.416203760999944,15.2,11.230519689));
#223727=CARTESIAN_POINT('Ctrl Pts',(0.416203760999944,11.6,11.230519689));
#223728=CARTESIAN_POINT('Ctrl Pts',(0.414730897999943,15.2,11.227390689));
#223729=CARTESIAN_POINT('Ctrl Pts',(0.414730897999943,11.6,11.227390689));
#223730=CARTESIAN_POINT('Ctrl Pts',(0.413262533999944,15.2,11.224264884));
#223731=CARTESIAN_POINT('Ctrl Pts',(0.413262533999944,11.6,11.224264884));
#223732=CARTESIAN_POINT('Ctrl Pts',(0.411798665999944,15.2,11.22114228));
#223733=CARTESIAN_POINT('Ctrl Pts',(0.411798665999944,11.6,11.22114228));
#223734=CARTESIAN_POINT('Ctrl Pts',(0.410339294999943,15.2,11.21802289));
#223735=CARTESIAN_POINT('Ctrl Pts',(0.410339294999943,11.6,11.21802289));
#223736=CARTESIAN_POINT('Ctrl Pts',(0.408884414999945,15.2,11.214906723));
#223737=CARTESIAN_POINT('Ctrl Pts',(0.408884414999945,11.6,11.214906723));
#223738=CARTESIAN_POINT('Ctrl Pts',(0.407434024999944,15.2,11.211793789));
#223739=CARTESIAN_POINT('Ctrl Pts',(0.407434024999944,11.6,11.211793789));
#223740=CARTESIAN_POINT('Ctrl Pts',(0.405988121999944,15.2,11.208684097));
#223741=CARTESIAN_POINT('Ctrl Pts',(0.405988121999944,11.6,11.208684097));
#223742=CARTESIAN_POINT('Ctrl Pts',(0.404546704999945,15.2,11.205577658));
#223743=CARTESIAN_POINT('Ctrl Pts',(0.404546704999945,11.6,11.205577658));
#223744=CARTESIAN_POINT('Ctrl Pts',(0.403109770999944,15.2,11.202474482));
#223745=CARTESIAN_POINT('Ctrl Pts',(0.403109770999944,11.6,11.202474482));
#223746=CARTESIAN_POINT('Ctrl Pts',(0.401677316999944,15.2,11.199374578));
#223747=CARTESIAN_POINT('Ctrl Pts',(0.401677316999944,11.6,11.199374578));
#223748=CARTESIAN_POINT('Ctrl Pts',(0.400249340999944,15.2,11.196277957));
#223749=CARTESIAN_POINT('Ctrl Pts',(0.400249340999944,11.6,11.196277957));
#223750=CARTESIAN_POINT('Ctrl Pts',(0.398825840999945,15.2,11.193184629));
#223751=CARTESIAN_POINT('Ctrl Pts',(0.398825840999945,11.6,11.193184629));
#223752=CARTESIAN_POINT('Ctrl Pts',(0.397406813999943,15.2,11.190094604));
#223753=CARTESIAN_POINT('Ctrl Pts',(0.397406813999943,11.6,11.190094604));
#223754=CARTESIAN_POINT('Ctrl Pts',(0.395992257999945,15.2,11.187007891));
#223755=CARTESIAN_POINT('Ctrl Pts',(0.395992257999945,11.6,11.187007891));
#223756=CARTESIAN_POINT('Ctrl Pts',(0.394582168999945,15.2,11.183924503));
#223757=CARTESIAN_POINT('Ctrl Pts',(0.394582168999945,11.6,11.183924503));
#223758=CARTESIAN_POINT('Ctrl Pts',(0.393176546999945,15.2,11.180844446));
#223759=CARTESIAN_POINT('Ctrl Pts',(0.393176546999945,11.6,11.180844446));
#223760=CARTESIAN_POINT('Ctrl Pts',(0.391775385999944,15.2,11.177767734));
#223761=CARTESIAN_POINT('Ctrl Pts',(0.391775385999944,11.6,11.177767734));
#223762=CARTESIAN_POINT('Ctrl Pts',(0.390378687999944,15.2,11.174694374));
#223763=CARTESIAN_POINT('Ctrl Pts',(0.390378687999944,11.6,11.174694374));
#223764=CARTESIAN_POINT('Ctrl Pts',(0.388986445999944,15.2,11.171624378));
#223765=CARTESIAN_POINT('Ctrl Pts',(0.388986445999944,11.6,11.171624378));
#223766=CARTESIAN_POINT('Ctrl Pts',(0.387598660999944,15.2,11.168557757));
#223767=CARTESIAN_POINT('Ctrl Pts',(0.387598660999944,11.6,11.168557757));
#223768=CARTESIAN_POINT('Ctrl Pts',(0.386215327999944,15.2,11.165494518));
#223769=CARTESIAN_POINT('Ctrl Pts',(0.386215327999944,11.6,11.165494518));
#223770=CARTESIAN_POINT('Ctrl Pts',(0.384836444999944,15.2,11.162434674));
#223771=CARTESIAN_POINT('Ctrl Pts',(0.384836444999944,11.6,11.162434674));
#223772=CARTESIAN_POINT('Ctrl Pts',(0.383462009999944,15.2,11.159378235));
#223773=CARTESIAN_POINT('Ctrl Pts',(0.383462009999944,11.6,11.159378235));
#223774=CARTESIAN_POINT('Ctrl Pts',(0.382092020999943,15.2,11.15632521));
#223775=CARTESIAN_POINT('Ctrl Pts',(0.382092020999943,11.6,11.15632521));
#223776=CARTESIAN_POINT('Ctrl Pts',(0.380726473999945,15.2,11.15327561));
#223777=CARTESIAN_POINT('Ctrl Pts',(0.380726473999945,11.6,11.15327561));
#223778=CARTESIAN_POINT('Ctrl Pts',(0.379365366999943,15.2,11.150229446));
#223779=CARTESIAN_POINT('Ctrl Pts',(0.379365366999943,11.6,11.150229446));
#223780=CARTESIAN_POINT('Ctrl Pts',(0.378008696999944,15.2,11.147186727));
#223781=CARTESIAN_POINT('Ctrl Pts',(0.378008696999944,11.6,11.147186727));
#223782=CARTESIAN_POINT('Ctrl Pts',(0.376656460999945,15.2,11.144147463));
#223783=CARTESIAN_POINT('Ctrl Pts',(0.376656460999945,11.6,11.144147463));
#223784=CARTESIAN_POINT('Ctrl Pts',(0.375308657999945,15.2,11.141111667));
#223785=CARTESIAN_POINT('Ctrl Pts',(0.375308657999945,11.6,11.141111667));
#223786=CARTESIAN_POINT('Ctrl Pts',(0.373965283999944,15.2,11.138079346));
#223787=CARTESIAN_POINT('Ctrl Pts',(0.373965283999944,11.6,11.138079346));
#223788=CARTESIAN_POINT('Ctrl Pts',(0.372626335999945,15.2,11.135050513));
#223789=CARTESIAN_POINT('Ctrl Pts',(0.372626335999945,11.6,11.135050513));
#223790=CARTESIAN_POINT('Ctrl Pts',(0.371291811999944,15.2,11.132025177));
#223791=CARTESIAN_POINT('Ctrl Pts',(0.371291811999944,11.6,11.132025177));
#223792=CARTESIAN_POINT('Ctrl Pts',(0.369961708999943,15.2,11.129003348));
#223793=CARTESIAN_POINT('Ctrl Pts',(0.369961708999943,11.6,11.129003348));
#223794=CARTESIAN_POINT('Ctrl Pts',(0.368636023999944,15.2,11.125985039));
#223795=CARTESIAN_POINT('Ctrl Pts',(0.368636023999944,11.6,11.125985039));
#223796=CARTESIAN_POINT('Ctrl Pts',(0.367314755999945,15.2,11.122970257));
#223797=CARTESIAN_POINT('Ctrl Pts',(0.367314755999945,11.6,11.122970257));
#223798=CARTESIAN_POINT('Ctrl Pts',(0.365997898999944,15.2,11.119959015));
#223799=CARTESIAN_POINT('Ctrl Pts',(0.365997898999944,11.6,11.119959015));
#223800=CARTESIAN_POINT('Ctrl Pts',(0.364685451999945,15.2,11.116951322));
#223801=CARTESIAN_POINT('Ctrl Pts',(0.364685451999945,11.6,11.116951322));
#223802=CARTESIAN_POINT('Ctrl Pts',(0.363377412999943,15.2,11.11394719));
#223803=CARTESIAN_POINT('Ctrl Pts',(0.363377412999943,11.6,11.11394719));
#223804=CARTESIAN_POINT('Ctrl Pts',(0.362073778999944,15.2,11.110946629));
#223805=CARTESIAN_POINT('Ctrl Pts',(0.362073778999944,11.6,11.110946629));
#223806=CARTESIAN_POINT('Ctrl Pts',(0.360774545999943,15.2,11.107949648));
#223807=CARTESIAN_POINT('Ctrl Pts',(0.360774545999943,11.6,11.107949648));
#223808=CARTESIAN_POINT('Ctrl Pts',(0.359479711999944,15.2,11.104956259));
#223809=CARTESIAN_POINT('Ctrl Pts',(0.359479711999944,11.6,11.104956259));
#223810=CARTESIAN_POINT('Ctrl Pts',(0.358189272999944,15.2,11.101966473));
#223811=CARTESIAN_POINT('Ctrl Pts',(0.358189272999944,11.6,11.101966473));
#223812=CARTESIAN_POINT('Ctrl Pts',(0.356903226999944,15.2,11.0989803));
#223813=CARTESIAN_POINT('Ctrl Pts',(0.356903226999944,11.6,11.0989803));
#223814=CARTESIAN_POINT('Ctrl Pts',(0.355621571999943,15.2,11.095997751));
#223815=CARTESIAN_POINT('Ctrl Pts',(0.355621571999943,11.6,11.095997751));
#223816=CARTESIAN_POINT('Ctrl Pts',(0.354344304999945,15.2,11.093018835));
#223817=CARTESIAN_POINT('Ctrl Pts',(0.354344304999945,11.6,11.093018835));
#223818=CARTESIAN_POINT('Ctrl Pts',(0.353071419999944,15.2,11.090043565));
#223819=CARTESIAN_POINT('Ctrl Pts',(0.353071419999944,11.6,11.090043565));
#223820=CARTESIAN_POINT('Ctrl Pts',(0.351802917999944,15.2,11.087071951));
#223821=CARTESIAN_POINT('Ctrl Pts',(0.351802917999944,11.6,11.087071951));
#223822=CARTESIAN_POINT('Ctrl Pts',(0.350538794999944,15.2,11.084104002));
#223823=CARTESIAN_POINT('Ctrl Pts',(0.350538794999944,11.6,11.084104002));
#223824=CARTESIAN_POINT('Ctrl Pts',(0.349279045999945,15.2,11.081139731));
#223825=CARTESIAN_POINT('Ctrl Pts',(0.349279045999945,11.6,11.081139731));
#223826=CARTESIAN_POINT('Ctrl Pts',(0.348023670999943,15.2,11.078179147));
#223827=CARTESIAN_POINT('Ctrl Pts',(0.348023670999943,11.6,11.078179147));
#223828=CARTESIAN_POINT('Ctrl Pts',(0.346772663999945,15.2,11.075222263));
#223829=CARTESIAN_POINT('Ctrl Pts',(0.346772663999945,11.6,11.075222263));
#223830=CARTESIAN_POINT('Ctrl Pts',(0.345526024999945,15.2,11.072269087));
#223831=CARTESIAN_POINT('Ctrl Pts',(0.345526024999945,11.6,11.072269087));
#223832=CARTESIAN_POINT('Ctrl Pts',(0.344283748999944,15.2,11.069319631));
#223833=CARTESIAN_POINT('Ctrl Pts',(0.344283748999944,11.6,11.069319631));
#223834=CARTESIAN_POINT('Ctrl Pts',(0.343045832999945,15.2,11.066373907));
#223835=CARTESIAN_POINT('Ctrl Pts',(0.343045832999945,11.6,11.066373907));
#223836=CARTESIAN_POINT('Ctrl Pts',(0.341812274999944,15.2,11.063431924));
#223837=CARTESIAN_POINT('Ctrl Pts',(0.341812274999944,11.6,11.063431924));
#223838=CARTESIAN_POINT('Ctrl Pts',(0.340583071999945,15.2,11.060493695));
#223839=CARTESIAN_POINT('Ctrl Pts',(0.340583071999945,11.6,11.060493695));
#223840=CARTESIAN_POINT('Ctrl Pts',(0.339358218999944,15.2,11.057559229));
#223841=CARTESIAN_POINT('Ctrl Pts',(0.339358218999944,11.6,11.057559229));
#223842=CARTESIAN_POINT('Ctrl Pts',(0.338137715999943,15.2,11.054628538));
#223843=CARTESIAN_POINT('Ctrl Pts',(0.338137715999943,11.6,11.054628538));
#223844=CARTESIAN_POINT('Ctrl Pts',(0.336921556999944,15.2,11.051701632));
#223845=CARTESIAN_POINT('Ctrl Pts',(0.336921556999944,11.6,11.051701632));
#223846=CARTESIAN_POINT('Ctrl Pts',(0.335709739999944,15.2,11.048778522));
#223847=CARTESIAN_POINT('Ctrl Pts',(0.335709739999944,11.6,11.048778522));
#223848=CARTESIAN_POINT('Ctrl Pts',(0.334502261999944,15.2,11.04585922));
#223849=CARTESIAN_POINT('Ctrl Pts',(0.334502261999944,11.6,11.04585922));
#223850=CARTESIAN_POINT('Ctrl Pts',(0.333299119999945,15.2,11.042943736));
#223851=CARTESIAN_POINT('Ctrl Pts',(0.333299119999945,11.6,11.042943736));
#223852=CARTESIAN_POINT('Ctrl Pts',(0.332100310999944,15.2,11.040032081));
#223853=CARTESIAN_POINT('Ctrl Pts',(0.332100310999944,11.6,11.040032081));
#223854=CARTESIAN_POINT('Ctrl Pts',(0.330905830999945,15.2,11.037124267));
#223855=CARTESIAN_POINT('Ctrl Pts',(0.330905830999945,11.6,11.037124267));
#223856=CARTESIAN_POINT('Ctrl Pts',(0.329715676999944,15.2,11.034220304));
#223857=CARTESIAN_POINT('Ctrl Pts',(0.329715676999944,11.6,11.034220304));
#223858=CARTESIAN_POINT('Ctrl Pts',(0.328529845999944,15.2,11.031320203));
#223859=CARTESIAN_POINT('Ctrl Pts',(0.328529845999944,11.6,11.031320203));
#223860=CARTESIAN_POINT('Ctrl Pts',(0.327348334999943,15.2,11.028423977));
#223861=CARTESIAN_POINT('Ctrl Pts',(0.327348334999943,11.6,11.028423977));
#223862=CARTESIAN_POINT('Ctrl Pts',(0.326171140999945,15.2,11.025531635));
#223863=CARTESIAN_POINT('Ctrl Pts',(0.326171140999945,11.6,11.025531635));
#223864=CARTESIAN_POINT('Ctrl Pts',(0.324998259999945,15.2,11.02264319));
#223865=CARTESIAN_POINT('Ctrl Pts',(0.324998259999945,11.6,11.02264319));
#223866=CARTESIAN_POINT('Ctrl Pts',(0.323829688999944,15.2,11.01975865));
#223867=CARTESIAN_POINT('Ctrl Pts',(0.323829688999944,11.6,11.01975865));
#223868=CARTESIAN_POINT('Ctrl Pts',(0.322665423999944,15.2,11.016878029));
#223869=CARTESIAN_POINT('Ctrl Pts',(0.322665423999944,11.6,11.016878029));
#223870=CARTESIAN_POINT('Ctrl Pts',(0.321505462999945,15.2,11.014001339));
#223871=CARTESIAN_POINT('Ctrl Pts',(0.321505462999945,11.6,11.014001339));
#223872=CARTESIAN_POINT('Ctrl Pts',(0.320349802999944,15.2,11.011128587));
#223873=CARTESIAN_POINT('Ctrl Pts',(0.320349802999944,11.6,11.011128587));
#223874=CARTESIAN_POINT('Ctrl Pts',(0.319198438999945,15.2,11.008259789));
#223875=CARTESIAN_POINT('Ctrl Pts',(0.319198438999945,11.6,11.008259789));
#223876=CARTESIAN_POINT('Ctrl Pts',(0.318051368999944,15.2,11.005394953));
#223877=CARTESIAN_POINT('Ctrl Pts',(0.318051368999944,11.6,11.005394953));
#223878=CARTESIAN_POINT('Ctrl Pts',(0.316908587999943,15.2,11.002534092));
#223879=CARTESIAN_POINT('Ctrl Pts',(0.316908587999943,11.6,11.002534092));
#223880=CARTESIAN_POINT('Ctrl Pts',(0.315770094999944,15.2,10.999677217));
#223881=CARTESIAN_POINT('Ctrl Pts',(0.315770094999944,11.6,10.999677217));
#223882=CARTESIAN_POINT('Ctrl Pts',(0.314635883999944,15.2,10.996824338));
#223883=CARTESIAN_POINT('Ctrl Pts',(0.314635883999944,11.6,10.996824338));
#223884=CARTESIAN_POINT('Ctrl Pts',(0.313505953999943,15.2,10.993975469));
#223885=CARTESIAN_POINT('Ctrl Pts',(0.313505953999943,11.6,10.993975469));
#223886=CARTESIAN_POINT('Ctrl Pts',(0.312380299999945,15.2,10.991130619));
#223887=CARTESIAN_POINT('Ctrl Pts',(0.312380299999945,11.6,10.991130619));
#223888=CARTESIAN_POINT('Ctrl Pts',(0.311258918999944,15.2,10.988289801));
#223889=CARTESIAN_POINT('Ctrl Pts',(0.311258918999944,11.6,10.988289801));
#223890=CARTESIAN_POINT('Ctrl Pts',(0.310141807999944,15.2,10.985453024));
#223891=CARTESIAN_POINT('Ctrl Pts',(0.310141807999944,11.6,10.985453024));
#223892=CARTESIAN_POINT('Ctrl Pts',(0.309028961999944,15.2,10.982620303));
#223893=CARTESIAN_POINT('Ctrl Pts',(0.309028961999944,11.6,10.982620303));
#223894=CARTESIAN_POINT('Ctrl Pts',(0.307920378999944,15.2,10.979791646));
#223895=CARTESIAN_POINT('Ctrl Pts',(0.307920378999944,11.6,10.979791646));
#223896=CARTESIAN_POINT('Ctrl Pts',(0.306816055999944,15.2,10.976967067));
#223897=CARTESIAN_POINT('Ctrl Pts',(0.306816055999944,11.6,10.976967067));
#223898=CARTESIAN_POINT('Ctrl Pts',(0.305715986999945,15.2,10.974146576));
#223899=CARTESIAN_POINT('Ctrl Pts',(0.305715986999945,11.6,10.974146576));
#223900=CARTESIAN_POINT('Ctrl Pts',(0.304620169999945,15.2,10.971330186));
#223901=CARTESIAN_POINT('Ctrl Pts',(0.304620169999945,11.6,10.971330186));
#223902=CARTESIAN_POINT('Ctrl Pts',(0.303528602999944,15.2,10.968517908));
#223903=CARTESIAN_POINT('Ctrl Pts',(0.303528602999944,11.6,10.968517908));
#223904=CARTESIAN_POINT('Ctrl Pts',(0.302441278999943,15.2,10.965709751));
#223905=CARTESIAN_POINT('Ctrl Pts',(0.302441278999943,11.6,10.965709751));
#223906=CARTESIAN_POINT('Ctrl Pts',(0.301358196999945,15.2,10.962905732));
#223907=CARTESIAN_POINT('Ctrl Pts',(0.301358196999945,11.6,10.962905732));
#223908=CARTESIAN_POINT('Ctrl Pts',(0.300279352999944,15.2,10.960105857));
#223909=CARTESIAN_POINT('Ctrl Pts',(0.300279352999944,11.6,10.960105857));
#223910=CARTESIAN_POINT('Ctrl Pts',(0.299204742999944,15.2,10.957310141));
#223911=CARTESIAN_POINT('Ctrl Pts',(0.299204742999944,11.6,10.957310141));
#223912=CARTESIAN_POINT('Ctrl Pts',(0.298134362999944,15.2,10.954518595));
#223913=CARTESIAN_POINT('Ctrl Pts',(0.298134362999944,11.6,10.954518595));
#223914=CARTESIAN_POINT('Ctrl Pts',(0.297068208999944,15.2,10.951731231));
#223915=CARTESIAN_POINT('Ctrl Pts',(0.297068208999944,11.6,10.951731231));
#223916=CARTESIAN_POINT('Ctrl Pts',(0.296006278999944,15.2,10.94894806));
#223917=CARTESIAN_POINT('Ctrl Pts',(0.296006278999944,11.6,10.94894806));
#223918=CARTESIAN_POINT('Ctrl Pts',(0.294948567999944,15.2,10.946169093));
#223919=CARTESIAN_POINT('Ctrl Pts',(0.294948567999944,11.6,10.946169093));
#223920=CARTESIAN_POINT('Ctrl Pts',(0.293895072999945,15.2,10.943394344));
#223921=CARTESIAN_POINT('Ctrl Pts',(0.293895072999945,11.6,10.943394344));
#223922=CARTESIAN_POINT('Ctrl Pts',(0.292845787999945,15.2,10.940623824));
#223923=CARTESIAN_POINT('Ctrl Pts',(0.292845787999945,11.6,10.940623824));
#223924=CARTESIAN_POINT('Ctrl Pts',(0.291800711999944,15.2,10.937857544));
#223925=CARTESIAN_POINT('Ctrl Pts',(0.291800711999944,11.6,10.937857544));
#223926=CARTESIAN_POINT('Ctrl Pts',(0.290759841999944,15.2,10.935095515));
#223927=CARTESIAN_POINT('Ctrl Pts',(0.290759841999944,11.6,10.935095515));
#223928=CARTESIAN_POINT('Ctrl Pts',(0.289723169999944,15.2,10.932337751));
#223929=CARTESIAN_POINT('Ctrl Pts',(0.289723169999944,11.6,10.932337751));
#223930=CARTESIAN_POINT('Ctrl Pts',(0.288690695999945,15.2,10.929584263));
#223931=CARTESIAN_POINT('Ctrl Pts',(0.288690695999945,11.6,10.929584263));
#223932=CARTESIAN_POINT('Ctrl Pts',(0.287662414999945,15.2,10.926835064));
#223933=CARTESIAN_POINT('Ctrl Pts',(0.287662414999945,11.6,10.926835064));
#223934=CARTESIAN_POINT('Ctrl Pts',(0.286638321999944,15.2,10.924090164));
#223935=CARTESIAN_POINT('Ctrl Pts',(0.286638321999944,11.6,10.924090164));
#223936=CARTESIAN_POINT('Ctrl Pts',(0.285618414999943,15.2,10.921349576));
#223937=CARTESIAN_POINT('Ctrl Pts',(0.285618414999943,11.6,10.921349576));
#223938=CARTESIAN_POINT('Ctrl Pts',(0.284602689999945,15.2,10.918613312));
#223939=CARTESIAN_POINT('Ctrl Pts',(0.284602689999945,11.6,10.918613312));
#223940=CARTESIAN_POINT('Ctrl Pts',(0.283591139999944,15.2,10.915881383));
#223941=CARTESIAN_POINT('Ctrl Pts',(0.283591139999944,11.6,10.915881383));
#223942=CARTESIAN_POINT('Ctrl Pts',(0.282583764999943,15.2,10.913153803));
#223943=CARTESIAN_POINT('Ctrl Pts',(0.282583764999943,11.6,10.913153803));
#223944=CARTESIAN_POINT('Ctrl Pts',(0.281580559999943,15.2,10.910430582));
#223945=CARTESIAN_POINT('Ctrl Pts',(0.281580559999943,11.6,10.910430582));
#223946=CARTESIAN_POINT('Ctrl Pts',(0.280581519999944,15.2,10.907711735));
#223947=CARTESIAN_POINT('Ctrl Pts',(0.280581519999944,11.6,10.907711735));
#223948=CARTESIAN_POINT('Ctrl Pts',(0.279586641999944,15.2,10.904997271));
#223949=CARTESIAN_POINT('Ctrl Pts',(0.279586641999944,11.6,10.904997271));
#223950=CARTESIAN_POINT('Ctrl Pts',(0.278595920999944,15.2,10.902287203));
#223951=CARTESIAN_POINT('Ctrl Pts',(0.278595920999944,11.6,10.902287203));
#223952=CARTESIAN_POINT('Ctrl Pts',(0.277609353999945,15.2,10.899581544));
#223953=CARTESIAN_POINT('Ctrl Pts',(0.277609353999945,11.6,10.899581544));
#223954=CARTESIAN_POINT('Ctrl Pts',(0.276626936999945,15.2,10.896880306));
#223955=CARTESIAN_POINT('Ctrl Pts',(0.276626936999945,11.6,10.896880306));
#223956=CARTESIAN_POINT('Ctrl Pts',(0.275648663999943,15.2,10.894183501));
#223957=CARTESIAN_POINT('Ctrl Pts',(0.275648663999943,11.6,10.894183501));
#223958=CARTESIAN_POINT('Ctrl Pts',(0.274674533999945,15.2,10.89149114));
#223959=CARTESIAN_POINT('Ctrl Pts',(0.274674533999945,11.6,10.89149114));
#223960=CARTESIAN_POINT('Ctrl Pts',(0.273704539999944,15.2,10.888803238));
#223961=CARTESIAN_POINT('Ctrl Pts',(0.273704539999944,11.6,10.888803238));
#223962=CARTESIAN_POINT('Ctrl Pts',(0.272738680999945,15.2,10.886119805));
#223963=CARTESIAN_POINT('Ctrl Pts',(0.272738680999945,11.6,10.886119805));
#223964=CARTESIAN_POINT('Ctrl Pts',(0.271776950999945,15.2,10.883440855));
#223965=CARTESIAN_POINT('Ctrl Pts',(0.271776950999945,11.6,10.883440855));
#223966=CARTESIAN_POINT('Ctrl Pts',(0.270819344999945,15.2,10.880766399));
#223967=CARTESIAN_POINT('Ctrl Pts',(0.270819344999945,11.6,10.880766399));
#223968=CARTESIAN_POINT('Ctrl Pts',(0.269865859999945,15.2,10.878096449));
#223969=CARTESIAN_POINT('Ctrl Pts',(0.269865859999945,11.6,10.878096449));
#223970=CARTESIAN_POINT('Ctrl Pts',(0.268916491999944,15.2,10.875431019));
#223971=CARTESIAN_POINT('Ctrl Pts',(0.268916491999944,11.6,10.875431019));
#223972=CARTESIAN_POINT('Ctrl Pts',(0.267971236999944,15.2,10.872770121));
#223973=CARTESIAN_POINT('Ctrl Pts',(0.267971236999944,11.6,10.872770121));
#223974=CARTESIAN_POINT('Ctrl Pts',(0.267030088999943,15.2,10.870113767));
#223975=CARTESIAN_POINT('Ctrl Pts',(0.267030088999943,11.6,10.870113767));
#223976=CARTESIAN_POINT('Ctrl Pts',(0.266093045999943,15.2,10.867461969));
#223977=CARTESIAN_POINT('Ctrl Pts',(0.266093045999943,11.6,10.867461969));
#223978=CARTESIAN_POINT('Ctrl Pts',(0.265160102999945,15.2,10.864814741));
#223979=CARTESIAN_POINT('Ctrl Pts',(0.265160102999945,11.6,10.864814741));
#223980=CARTESIAN_POINT('Ctrl Pts',(0.264231254999944,15.2,10.862172095));
#223981=CARTESIAN_POINT('Ctrl Pts',(0.264231254999944,11.6,10.862172095));
#223982=CARTESIAN_POINT('Ctrl Pts',(0.263306497999943,15.2,10.859534043));
#223983=CARTESIAN_POINT('Ctrl Pts',(0.263306497999943,11.6,10.859534043));
#223984=CARTESIAN_POINT('Ctrl Pts',(0.262385827999945,15.2,10.856900597));
#223985=CARTESIAN_POINT('Ctrl Pts',(0.262385827999945,11.6,10.856900597));
#223986=CARTESIAN_POINT('Ctrl Pts',(0.261469239999944,15.2,10.854271772));
#223987=CARTESIAN_POINT('Ctrl Pts',(0.261469239999944,11.6,10.854271772));
#223988=CARTESIAN_POINT('Ctrl Pts',(0.260556730999945,15.2,10.851647579));
#223989=CARTESIAN_POINT('Ctrl Pts',(0.260556730999945,11.6,10.851647579));
#223990=CARTESIAN_POINT('Ctrl Pts',(0.259648296999944,15.2,10.84902803));
#223991=CARTESIAN_POINT('Ctrl Pts',(0.259648296999944,11.6,10.84902803));
#223992=CARTESIAN_POINT('Ctrl Pts',(0.258743930999945,15.2,10.846413139));
#223993=CARTESIAN_POINT('Ctrl Pts',(0.258743930999945,11.6,10.846413139));
#223994=CARTESIAN_POINT('Ctrl Pts',(0.257843629999943,15.2,10.843802919));
#223995=CARTESIAN_POINT('Ctrl Pts',(0.257843629999943,11.6,10.843802919));
#223996=CARTESIAN_POINT('Ctrl Pts',(0.256947389999944,15.2,10.841197381));
#223997=CARTESIAN_POINT('Ctrl Pts',(0.256947389999944,11.6,10.841197381));
#223998=CARTESIAN_POINT('Ctrl Pts',(0.256055205999944,15.2,10.838596539));
#223999=CARTESIAN_POINT('Ctrl Pts',(0.256055205999944,11.6,10.838596539));
#224000=CARTESIAN_POINT('Ctrl Pts',(0.255167071999944,15.2,10.836000406));
#224001=CARTESIAN_POINT('Ctrl Pts',(0.255167071999944,11.6,10.836000406));
#224002=CARTESIAN_POINT('Ctrl Pts',(0.254282986999945,15.2,10.833408995));
#224003=CARTESIAN_POINT('Ctrl Pts',(0.254282986999945,11.6,10.833408995));
#224004=CARTESIAN_POINT('Ctrl Pts',(0.253402944999944,15.2,10.830822318));
#224005=CARTESIAN_POINT('Ctrl Pts',(0.253402944999944,11.6,10.830822318));
#224006=CARTESIAN_POINT('Ctrl Pts',(0.252526938999944,15.2,10.828240388));
#224007=CARTESIAN_POINT('Ctrl Pts',(0.252526938999944,11.6,10.828240388));
#224008=CARTESIAN_POINT('Ctrl Pts',(0.251654968999944,15.2,10.825663219));
#224009=CARTESIAN_POINT('Ctrl Pts',(0.251654968999944,11.6,10.825663219));
#224010=CARTESIAN_POINT('Ctrl Pts',(0.250787026999945,15.2,10.823090823));
#224011=CARTESIAN_POINT('Ctrl Pts',(0.250787026999945,11.6,10.823090823));
#224012=CARTESIAN_POINT('Ctrl Pts',(0.249923107999944,15.2,10.820523213));
#224013=CARTESIAN_POINT('Ctrl Pts',(0.249923107999944,11.6,10.820523213));
#224014=CARTESIAN_POINT('Ctrl Pts',(0.249063209999945,15.2,10.817960403));
#224015=CARTESIAN_POINT('Ctrl Pts',(0.249063209999945,11.6,10.817960403));
#224016=CARTESIAN_POINT('Ctrl Pts',(0.248207326999944,15.2,10.815402405));
#224017=CARTESIAN_POINT('Ctrl Pts',(0.248207326999944,11.6,10.815402405));
#224018=CARTESIAN_POINT('Ctrl Pts',(0.247355453999945,15.2,10.812849232));
#224019=CARTESIAN_POINT('Ctrl Pts',(0.247355453999945,11.6,10.812849232));
#224020=CARTESIAN_POINT('Ctrl Pts',(0.246507586999943,15.2,10.810300898));
#224021=CARTESIAN_POINT('Ctrl Pts',(0.246507586999943,11.6,10.810300898));
#224022=CARTESIAN_POINT('Ctrl Pts',(0.245663720999945,15.2,10.807757416));
#224023=CARTESIAN_POINT('Ctrl Pts',(0.245663720999945,11.6,10.807757416));
#224024=CARTESIAN_POINT('Ctrl Pts',(0.244823849999944,15.2,10.805218799));
#224025=CARTESIAN_POINT('Ctrl Pts',(0.244823849999944,11.6,10.805218799));
#224026=CARTESIAN_POINT('Ctrl Pts',(0.243987971999945,15.2,10.80268506));
#224027=CARTESIAN_POINT('Ctrl Pts',(0.243987971999945,11.6,10.80268506));
#224028=CARTESIAN_POINT('Ctrl Pts',(0.243156079999943,15.2,10.800156212));
#224029=CARTESIAN_POINT('Ctrl Pts',(0.243156079999943,11.6,10.800156212));
#224030=CARTESIAN_POINT('Ctrl Pts',(0.242328170999944,15.2,10.797632269));
#224031=CARTESIAN_POINT('Ctrl Pts',(0.242328170999944,11.6,10.797632269));
#224032=CARTESIAN_POINT('Ctrl Pts',(0.241504236999944,15.2,10.795113244));
#224033=CARTESIAN_POINT('Ctrl Pts',(0.241504236999944,11.6,10.795113244));
#224034=CARTESIAN_POINT('Ctrl Pts',(0.240684276999945,15.2,10.79259915));
#224035=CARTESIAN_POINT('Ctrl Pts',(0.240684276999945,11.6,10.79259915));
#224036=CARTESIAN_POINT('Ctrl Pts',(0.239868283999943,15.2,10.790090001));
#224037=CARTESIAN_POINT('Ctrl Pts',(0.239868283999943,11.6,10.790090001));
#224038=CARTESIAN_POINT('Ctrl Pts',(0.239056252999944,15.2,10.78758581));
#224039=CARTESIAN_POINT('Ctrl Pts',(0.239056252999944,11.6,10.78758581));
#224040=CARTESIAN_POINT('Ctrl Pts',(0.238248179999945,15.2,10.78508659));
#224041=CARTESIAN_POINT('Ctrl Pts',(0.238248179999945,11.6,10.78508659));
#224042=CARTESIAN_POINT('Ctrl Pts',(0.237444059999945,15.2,10.782592356));
#224043=CARTESIAN_POINT('Ctrl Pts',(0.237444059999945,11.6,10.782592356));
#224044=CARTESIAN_POINT('Ctrl Pts',(0.236643886999944,15.2,10.780103119));
#224045=CARTESIAN_POINT('Ctrl Pts',(0.236643886999944,11.6,10.780103119));
#224046=CARTESIAN_POINT('Ctrl Pts',(0.235847656999945,15.2,10.777618895));
#224047=CARTESIAN_POINT('Ctrl Pts',(0.235847656999945,11.6,10.777618895));
#224048=CARTESIAN_POINT('Ctrl Pts',(0.235055364999944,15.2,10.775139696));
#224049=CARTESIAN_POINT('Ctrl Pts',(0.235055364999944,11.6,10.775139696));
#224050=CARTESIAN_POINT('Ctrl Pts',(0.234267004999945,15.2,10.772665536));
#224051=CARTESIAN_POINT('Ctrl Pts',(0.234267004999945,11.6,10.772665536));
#224052=CARTESIAN_POINT('Ctrl Pts',(0.233482572999945,15.2,10.770196429));
#224053=CARTESIAN_POINT('Ctrl Pts',(0.233482572999945,11.6,10.770196429));
#224054=CARTESIAN_POINT('Ctrl Pts',(0.232702063999944,15.2,10.767732388));
#224055=CARTESIAN_POINT('Ctrl Pts',(0.232702063999944,11.6,10.767732388));
#224056=CARTESIAN_POINT('Ctrl Pts',(0.231925471999944,15.2,10.765273427));
#224057=CARTESIAN_POINT('Ctrl Pts',(0.231925471999944,11.6,10.765273427));
#224058=CARTESIAN_POINT('Ctrl Pts',(0.231152791999945,15.2,10.762819561));
#224059=CARTESIAN_POINT('Ctrl Pts',(0.231152791999945,11.6,10.762819561));
#224060=CARTESIAN_POINT('Ctrl Pts',(0.230384019999944,15.2,10.760370801));
#224061=CARTESIAN_POINT('Ctrl Pts',(0.230384019999944,11.6,10.760370801));
#224062=CARTESIAN_POINT('Ctrl Pts',(0.229619148999944,15.2,10.757927164));
#224063=CARTESIAN_POINT('Ctrl Pts',(0.229619148999944,11.6,10.757927164));
#224064=CARTESIAN_POINT('Ctrl Pts',(0.228858174999944,15.2,10.755488661));
#224065=CARTESIAN_POINT('Ctrl Pts',(0.228858174999944,11.6,10.755488661));
#224066=CARTESIAN_POINT('Ctrl Pts',(0.228101093999945,15.2,10.753055306));
#224067=CARTESIAN_POINT('Ctrl Pts',(0.228101093999945,11.6,10.753055306));
#224068=CARTESIAN_POINT('Ctrl Pts',(0.227347897999944,15.2,10.750627115));
#224069=CARTESIAN_POINT('Ctrl Pts',(0.227347897999944,11.6,10.750627115));
#224070=CARTESIAN_POINT('Ctrl Pts',(0.226598583999945,15.2,10.748204101));
#224071=CARTESIAN_POINT('Ctrl Pts',(0.226598583999945,11.6,10.748204101));
#224072=CARTESIAN_POINT('Ctrl Pts',(0.225853144999943,15.2,10.745786278));
#224073=CARTESIAN_POINT('Ctrl Pts',(0.225853144999943,11.6,10.745786278));
#224074=CARTESIAN_POINT('Ctrl Pts',(0.225111577999944,15.2,10.743373659));
#224075=CARTESIAN_POINT('Ctrl Pts',(0.225111577999944,11.6,10.743373659));
#224076=CARTESIAN_POINT('Ctrl Pts',(0.224373874999945,15.2,10.740966259));
#224077=CARTESIAN_POINT('Ctrl Pts',(0.224373874999945,11.6,10.740966259));
#224078=CARTESIAN_POINT('Ctrl Pts',(0.223640032999944,15.2,10.738564091));
#224079=CARTESIAN_POINT('Ctrl Pts',(0.223640032999944,11.6,10.738564091));
#224080=CARTESIAN_POINT('Ctrl Pts',(0.222910043999944,15.2,10.736167171));
#224081=CARTESIAN_POINT('Ctrl Pts',(0.222910043999944,11.6,10.736167171));
#224082=CARTESIAN_POINT('Ctrl Pts',(0.222183904999945,15.2,10.733775512));
#224083=CARTESIAN_POINT('Ctrl Pts',(0.222183904999945,11.6,10.733775512));
#224084=CARTESIAN_POINT('Ctrl Pts',(0.221461608999943,15.2,10.731389127));
#224085=CARTESIAN_POINT('Ctrl Pts',(0.221461608999943,11.6,10.731389127));
#224086=CARTESIAN_POINT('Ctrl Pts',(0.220743151999944,15.2,10.729008033));
#224087=CARTESIAN_POINT('Ctrl Pts',(0.220743151999944,11.6,10.729008033));
#224088=CARTESIAN_POINT('Ctrl Pts',(0.220028526999944,15.2,10.726632242));
#224089=CARTESIAN_POINT('Ctrl Pts',(0.220028526999944,11.6,10.726632242));
#224090=CARTESIAN_POINT('Ctrl Pts',(0.219317728999944,15.2,10.724261769));
#224091=CARTESIAN_POINT('Ctrl Pts',(0.219317728999944,11.6,10.724261769));
#224092=CARTESIAN_POINT('Ctrl Pts',(0.218610752999944,15.2,10.721896627));
#224093=CARTESIAN_POINT('Ctrl Pts',(0.218610752999944,11.6,10.721896627));
#224094=CARTESIAN_POINT('Ctrl Pts',(0.217907592999945,15.2,10.719536832));
#224095=CARTESIAN_POINT('Ctrl Pts',(0.217907592999945,11.6,10.719536832));
#224096=CARTESIAN_POINT('Ctrl Pts',(0.217208243999943,15.2,10.717182399));
#224097=CARTESIAN_POINT('Ctrl Pts',(0.217208243999943,11.6,10.717182399));
#224098=CARTESIAN_POINT('Ctrl Pts',(0.216512699999944,15.2,10.71483334));
#224099=CARTESIAN_POINT('Ctrl Pts',(0.216512699999944,11.6,10.71483334));
#224100=CARTESIAN_POINT('Ctrl Pts',(0.215820953999944,15.2,10.712489672));
#224101=CARTESIAN_POINT('Ctrl Pts',(0.215820953999944,11.6,10.712489672));
#224102=CARTESIAN_POINT('Ctrl Pts',(0.215133002999943,15.2,10.710151408));
#224103=CARTESIAN_POINT('Ctrl Pts',(0.215133002999943,11.6,10.710151408));
#224104=CARTESIAN_POINT('Ctrl Pts',(0.214448838999944,15.2,10.707818563));
#224105=CARTESIAN_POINT('Ctrl Pts',(0.214448838999944,11.6,10.707818563));
#224106=CARTESIAN_POINT('Ctrl Pts',(0.213768457999944,15.2,10.70549115));
#224107=CARTESIAN_POINT('Ctrl Pts',(0.213768457999944,11.6,10.70549115));
#224108=CARTESIAN_POINT('Ctrl Pts',(0.213091851999945,15.2,10.703169186));
#224109=CARTESIAN_POINT('Ctrl Pts',(0.213091851999945,11.6,10.703169186));
#224110=CARTESIAN_POINT('Ctrl Pts',(0.212419017999944,15.2,10.700852684));
#224111=CARTESIAN_POINT('Ctrl Pts',(0.212419017999944,11.6,10.700852684));
#224112=CARTESIAN_POINT('Ctrl Pts',(0.211749947999945,15.2,10.69854166));
#224113=CARTESIAN_POINT('Ctrl Pts',(0.211749947999945,11.6,10.69854166));
#224114=CARTESIAN_POINT('Ctrl Pts',(0.211084637999944,15.2,10.696236128));
#224115=CARTESIAN_POINT('Ctrl Pts',(0.211084637999944,11.6,10.696236128));
#224116=CARTESIAN_POINT('Ctrl Pts',(0.210423080999943,15.2,10.693936102));
#224117=CARTESIAN_POINT('Ctrl Pts',(0.210423080999943,11.6,10.693936102));
#224118=CARTESIAN_POINT('Ctrl Pts',(0.209765270999943,15.2,10.691641598));
#224119=CARTESIAN_POINT('Ctrl Pts',(0.209765270999943,11.6,10.691641598));
#224120=CARTESIAN_POINT('Ctrl Pts',(0.209111202999944,15.2,10.68935263));
#224121=CARTESIAN_POINT('Ctrl Pts',(0.209111202999944,11.6,10.68935263));
#224122=CARTESIAN_POINT('Ctrl Pts',(0.208460869999945,15.2,10.687069213));
#224123=CARTESIAN_POINT('Ctrl Pts',(0.208460869999945,11.6,10.687069213));
#224124=CARTESIAN_POINT('Ctrl Pts',(0.207814266999945,15.2,10.684791362));
#224125=CARTESIAN_POINT('Ctrl Pts',(0.207814266999945,11.6,10.684791362));
#224126=CARTESIAN_POINT('Ctrl Pts',(0.207171385999944,15.2,10.682519093));
#224127=CARTESIAN_POINT('Ctrl Pts',(0.207171385999944,11.6,10.682519093));
#224128=CARTESIAN_POINT('Ctrl Pts',(0.206532223999943,15.2,10.680252419));
#224129=CARTESIAN_POINT('Ctrl Pts',(0.206532223999943,11.6,10.680252419));
#224130=CARTESIAN_POINT('Ctrl Pts',(0.205896773999944,15.2,10.677991356));
#224131=CARTESIAN_POINT('Ctrl Pts',(0.205896773999944,11.6,10.677991356));
#224132=CARTESIAN_POINT('Ctrl Pts',(0.205265027999945,15.2,10.67573592));
#224133=CARTESIAN_POINT('Ctrl Pts',(0.205265027999945,11.6,10.67573592));
#224134=CARTESIAN_POINT('Ctrl Pts',(0.204636982999944,15.2,10.673486125));
#224135=CARTESIAN_POINT('Ctrl Pts',(0.204636982999944,11.6,10.673486125));
#224136=CARTESIAN_POINT('Ctrl Pts',(0.204012629999945,15.2,10.671241985));
#224137=CARTESIAN_POINT('Ctrl Pts',(0.204012629999945,11.6,10.671241985));
#224138=CARTESIAN_POINT('Ctrl Pts',(0.203391963999945,15.2,10.669003518));
#224139=CARTESIAN_POINT('Ctrl Pts',(0.203391963999945,11.6,10.669003518));
#224140=CARTESIAN_POINT('Ctrl Pts',(0.202774978999944,15.2,10.666770738));
#224141=CARTESIAN_POINT('Ctrl Pts',(0.202774978999944,11.6,10.666770738));
#224142=CARTESIAN_POINT('Ctrl Pts',(0.202161669999944,15.2,10.664543659));
#224143=CARTESIAN_POINT('Ctrl Pts',(0.202161669999944,11.6,10.664543659));
#224144=CARTESIAN_POINT('Ctrl Pts',(0.201552027999944,15.2,10.662322298));
#224145=CARTESIAN_POINT('Ctrl Pts',(0.201552027999944,11.6,10.662322298));
#224146=CARTESIAN_POINT('Ctrl Pts',(0.200946048999944,15.2,10.660106669));
#224147=CARTESIAN_POINT('Ctrl Pts',(0.200946048999944,11.6,10.660106669));
#224148=CARTESIAN_POINT('Ctrl Pts',(0.200343724999945,15.2,10.657896788));
#224149=CARTESIAN_POINT('Ctrl Pts',(0.200343724999945,11.6,10.657896788));
#224150=CARTESIAN_POINT('Ctrl Pts',(0.199745050999944,15.2,10.655692671));
#224151=CARTESIAN_POINT('Ctrl Pts',(0.199745050999944,11.6,10.655692671));
#224152=CARTESIAN_POINT('Ctrl Pts',(0.199150019999944,15.2,10.653494334));
#224153=CARTESIAN_POINT('Ctrl Pts',(0.199150019999944,11.6,10.653494334));
#224154=CARTESIAN_POINT('Ctrl Pts',(0.198558625999944,15.2,10.651301789));
#224155=CARTESIAN_POINT('Ctrl Pts',(0.198558625999944,11.6,10.651301789));
#224156=CARTESIAN_POINT('Ctrl Pts',(0.197970861999943,15.2,10.649115056));
#224157=CARTESIAN_POINT('Ctrl Pts',(0.197970861999943,11.6,10.649115056));
#224158=CARTESIAN_POINT('Ctrl Pts',(0.197386722999945,15.2,10.646934148));
#224159=CARTESIAN_POINT('Ctrl Pts',(0.197386722999945,11.6,10.646934148));
#224160=CARTESIAN_POINT('Ctrl Pts',(0.196806200999945,15.2,10.644759081));
#224161=CARTESIAN_POINT('Ctrl Pts',(0.196806200999945,11.6,10.644759081));
#224162=CARTESIAN_POINT('Ctrl Pts',(0.196229288999945,15.2,10.642589871));
#224163=CARTESIAN_POINT('Ctrl Pts',(0.196229288999945,11.6,10.642589871));
#224164=CARTESIAN_POINT('Ctrl Pts',(0.195655981999945,15.2,10.640426535));
#224165=CARTESIAN_POINT('Ctrl Pts',(0.195655981999945,11.6,10.640426535));
#224166=CARTESIAN_POINT('Ctrl Pts',(0.195086272999945,15.2,10.638269086));
#224167=CARTESIAN_POINT('Ctrl Pts',(0.195086272999945,11.6,10.638269086));
#224168=CARTESIAN_POINT('Ctrl Pts',(0.194520154999944,15.2,10.636117541));
#224169=CARTESIAN_POINT('Ctrl Pts',(0.194520154999944,11.6,10.636117541));
#224170=CARTESIAN_POINT('Ctrl Pts',(0.193957621999944,15.2,10.633971917));
#224171=CARTESIAN_POINT('Ctrl Pts',(0.193957621999944,11.6,10.633971917));
#224172=CARTESIAN_POINT('Ctrl Pts',(0.193398666999943,15.2,10.631832228));
#224173=CARTESIAN_POINT('Ctrl Pts',(0.193398666999943,11.6,10.631832228));
#224174=CARTESIAN_POINT('Ctrl Pts',(0.192843282999944,15.2,10.629698493));
#224175=CARTESIAN_POINT('Ctrl Pts',(0.192843282999944,11.6,10.629698493));
#224176=CARTESIAN_POINT('Ctrl Pts',(0.192291463999944,15.2,10.627570724));
#224177=CARTESIAN_POINT('Ctrl Pts',(0.192291463999944,11.6,10.627570724));
#224178=CARTESIAN_POINT('Ctrl Pts',(0.191743202999944,15.2,10.62544894));
#224179=CARTESIAN_POINT('Ctrl Pts',(0.191743202999944,11.6,10.62544894));
#224180=CARTESIAN_POINT('Ctrl Pts',(0.191198490999945,15.2,10.623333156));
#224181=CARTESIAN_POINT('Ctrl Pts',(0.191198490999945,11.6,10.623333156));
#224182=CARTESIAN_POINT('Ctrl Pts',(0.190657324999943,15.2,10.621223388));
#224183=CARTESIAN_POINT('Ctrl Pts',(0.190657324999943,11.6,10.621223388));
#224184=CARTESIAN_POINT('Ctrl Pts',(0.190119695999943,15.2,10.619119652));
#224185=CARTESIAN_POINT('Ctrl Pts',(0.190119695999943,11.6,10.619119652));
#224186=CARTESIAN_POINT('Ctrl Pts',(0.189585597999944,15.2,10.617021966));
#224187=CARTESIAN_POINT('Ctrl Pts',(0.189585597999944,11.6,10.617021966));
#224188=CARTESIAN_POINT('Ctrl Pts',(0.189055023999943,15.2,10.614930343));
#224189=CARTESIAN_POINT('Ctrl Pts',(0.189055023999943,11.6,10.614930343));
#224190=CARTESIAN_POINT('Ctrl Pts',(0.188527964999944,15.2,10.612844803));
#224191=CARTESIAN_POINT('Ctrl Pts',(0.188527964999944,11.6,10.612844803));
#224192=CARTESIAN_POINT('Ctrl Pts',(0.188004415999944,15.2,10.61076536));
#224193=CARTESIAN_POINT('Ctrl Pts',(0.188004415999944,11.6,10.61076536));
#224194=CARTESIAN_POINT('Ctrl Pts',(0.187484369999943,15.2,10.608692031));
#224195=CARTESIAN_POINT('Ctrl Pts',(0.187484369999943,11.6,10.608692031));
#224196=CARTESIAN_POINT('Ctrl Pts',(0.186967819999945,15.2,10.606624832));
#224197=CARTESIAN_POINT('Ctrl Pts',(0.186967819999945,11.6,10.606624832));
#224198=CARTESIAN_POINT('Ctrl Pts',(0.186454757999943,15.2,10.604563781));
#224199=CARTESIAN_POINT('Ctrl Pts',(0.186454757999943,11.6,10.604563781));
#224200=CARTESIAN_POINT('Ctrl Pts',(0.185945176999944,15.2,10.602508892));
#224201=CARTESIAN_POINT('Ctrl Pts',(0.185945176999944,11.6,10.602508892));
#224202=CARTESIAN_POINT('Ctrl Pts',(0.185439070999944,15.2,10.600460184));
#224203=CARTESIAN_POINT('Ctrl Pts',(0.185439070999944,11.6,10.600460184));
#224204=CARTESIAN_POINT('Ctrl Pts',(0.184936431999944,15.2,10.598417673));
#224205=CARTESIAN_POINT('Ctrl Pts',(0.184936431999944,11.6,10.598417673));
#224206=CARTESIAN_POINT('Ctrl Pts',(0.184437252999944,15.2,10.596381375));
#224207=CARTESIAN_POINT('Ctrl Pts',(0.184437252999944,11.6,10.596381375));
#224208=CARTESIAN_POINT('Ctrl Pts',(0.183941525999943,15.2,10.594351307));
#224209=CARTESIAN_POINT('Ctrl Pts',(0.183941525999943,11.6,10.594351307));
#224210=CARTESIAN_POINT('Ctrl Pts',(0.183449243999944,15.2,10.592327487));
#224211=CARTESIAN_POINT('Ctrl Pts',(0.183449243999944,11.6,10.592327487));
#224212=CARTESIAN_POINT('Ctrl Pts',(0.182960400999944,15.2,10.59030993));
#224213=CARTESIAN_POINT('Ctrl Pts',(0.182960400999944,11.6,10.59030993));
#224214=CARTESIAN_POINT('Ctrl Pts',(0.182474987999944,15.2,10.588298654));
#224215=CARTESIAN_POINT('Ctrl Pts',(0.182474987999944,11.6,10.588298654));
#224216=CARTESIAN_POINT('Ctrl Pts',(0.181992997999944,15.2,10.586293676));
#224217=CARTESIAN_POINT('Ctrl Pts',(0.181992997999944,11.6,10.586293676));
#224218=CARTESIAN_POINT('Ctrl Pts',(0.181514424999945,15.2,10.584295013));
#224219=CARTESIAN_POINT('Ctrl Pts',(0.181514424999945,11.6,10.584295013));
#224220=CARTESIAN_POINT('Ctrl Pts',(0.181039259999943,15.2,10.582302681));
#224221=CARTESIAN_POINT('Ctrl Pts',(0.181039259999943,11.6,10.582302681));
#224222=CARTESIAN_POINT('Ctrl Pts',(0.180567494999944,15.2,10.580316698));
#224223=CARTESIAN_POINT('Ctrl Pts',(0.180567494999944,11.6,10.580316698));
#224224=CARTESIAN_POINT('Ctrl Pts',(0.180099123999945,15.2,10.578337082));
#224225=CARTESIAN_POINT('Ctrl Pts',(0.180099123999945,11.6,10.578337082));
#224226=CARTESIAN_POINT('Ctrl Pts',(0.179634138999945,15.2,10.576363848));
#224227=CARTESIAN_POINT('Ctrl Pts',(0.179634138999945,11.6,10.576363848));
#224228=CARTESIAN_POINT('Ctrl Pts',(0.179172531999944,15.2,10.574397014));
#224229=CARTESIAN_POINT('Ctrl Pts',(0.179172531999944,11.6,10.574397014));
#224230=CARTESIAN_POINT('Ctrl Pts',(0.178714295999944,15.2,10.5724366));
#224231=CARTESIAN_POINT('Ctrl Pts',(0.178714295999944,11.6,10.5724366));
#224232=CARTESIAN_POINT('Ctrl Pts',(0.178259421999943,15.2,10.570482619));
#224233=CARTESIAN_POINT('Ctrl Pts',(0.178259421999943,11.6,10.570482619));
#224234=CARTESIAN_POINT('Ctrl Pts',(0.177807903999945,15.2,10.568535092));
#224235=CARTESIAN_POINT('Ctrl Pts',(0.177807903999945,11.6,10.568535092));
#224236=CARTESIAN_POINT('Ctrl Pts',(0.177359733999944,15.2,10.566594034));
#224237=CARTESIAN_POINT('Ctrl Pts',(0.177359733999944,11.6,10.566594034));
#224238=CARTESIAN_POINT('Ctrl Pts',(0.176914901999944,15.2,10.564659464));
#224239=CARTESIAN_POINT('Ctrl Pts',(0.176914901999944,11.6,10.564659464));
#224240=CARTESIAN_POINT('Ctrl Pts',(0.176473402999945,15.2,10.5627314));
#224241=CARTESIAN_POINT('Ctrl Pts',(0.176473402999945,11.6,10.5627314));
#224242=CARTESIAN_POINT('Ctrl Pts',(0.176035227999943,15.2,10.560809858));
#224243=CARTESIAN_POINT('Ctrl Pts',(0.176035227999943,11.6,10.560809858));
#224244=CARTESIAN_POINT('Ctrl Pts',(0.175600368999945,15.2,10.558894856));
#224245=CARTESIAN_POINT('Ctrl Pts',(0.175600368999945,11.6,10.558894856));
#224246=CARTESIAN_POINT('Ctrl Pts',(0.175168817999944,15.2,10.556986414));
#224247=CARTESIAN_POINT('Ctrl Pts',(0.175168817999944,11.6,10.556986414));
#224248=CARTESIAN_POINT('Ctrl Pts',(0.174740566999944,15.2,10.555084546));
#224249=CARTESIAN_POINT('Ctrl Pts',(0.174740566999944,11.6,10.555084546));
#224250=CARTESIAN_POINT('Ctrl Pts',(0.174315608999944,15.2,10.553189272));
#224251=CARTESIAN_POINT('Ctrl Pts',(0.174315608999944,11.6,10.553189272));
#224252=CARTESIAN_POINT('Ctrl Pts',(0.173893933999943,15.2,10.551300611));
#224253=CARTESIAN_POINT('Ctrl Pts',(0.173893933999943,11.6,10.551300611));
#224254=CARTESIAN_POINT('Ctrl Pts',(0.173475535999945,15.2,10.549418579));
#224255=CARTESIAN_POINT('Ctrl Pts',(0.173475535999945,11.6,10.549418579));
#224256=CARTESIAN_POINT('Ctrl Pts',(0.173060405999944,15.2,10.547543196));
#224257=CARTESIAN_POINT('Ctrl Pts',(0.173060405999944,11.6,10.547543196));
#224258=CARTESIAN_POINT('Ctrl Pts',(0.172648535999944,15.2,10.545674477));
#224259=CARTESIAN_POINT('Ctrl Pts',(0.172648535999944,11.6,10.545674477));
#224260=CARTESIAN_POINT('Ctrl Pts',(0.172239915999944,15.2,10.543812444));
#224261=CARTESIAN_POINT('Ctrl Pts',(0.172239915999944,11.6,10.543812444));
#224262=CARTESIAN_POINT('Ctrl Pts',(0.171834540999944,15.2,10.541957111));
#224263=CARTESIAN_POINT('Ctrl Pts',(0.171834540999944,11.6,10.541957111));
#224264=CARTESIAN_POINT('Ctrl Pts',(0.171432399999943,15.2,10.5401085));
#224265=CARTESIAN_POINT('Ctrl Pts',(0.171432399999943,11.6,10.5401085));
#224266=CARTESIAN_POINT('Ctrl Pts',(0.171033485999944,15.2,10.538266627));
#224267=CARTESIAN_POINT('Ctrl Pts',(0.171033485999944,11.6,10.538266627));
#224268=CARTESIAN_POINT('Ctrl Pts',(0.170637789999945,15.2,10.536431512));
#224269=CARTESIAN_POINT('Ctrl Pts',(0.170637789999945,11.6,10.536431512));
#224270=CARTESIAN_POINT('Ctrl Pts',(0.170245304999943,15.2,10.534603171));
#224271=CARTESIAN_POINT('Ctrl Pts',(0.170245304999943,11.6,10.534603171));
#224272=CARTESIAN_POINT('Ctrl Pts',(0.169856019999944,15.2,10.532781625));
#224273=CARTESIAN_POINT('Ctrl Pts',(0.169856019999944,11.6,10.532781625));
#224274=CARTESIAN_POINT('Ctrl Pts',(0.169469929999944,15.2,10.530966892));
#224275=CARTESIAN_POINT('Ctrl Pts',(0.169469929999944,11.6,10.530966892));
#224276=CARTESIAN_POINT('Ctrl Pts',(0.169087021999944,15.2,10.52915899));
#224277=CARTESIAN_POINT('Ctrl Pts',(0.169087021999944,11.6,10.52915899));
#224278=CARTESIAN_POINT('Ctrl Pts',(0.168707291999944,15.2,10.527357938));
#224279=CARTESIAN_POINT('Ctrl Pts',(0.168707291999944,11.6,10.527357938));
#224280=CARTESIAN_POINT('Ctrl Pts',(0.168330727999945,15.2,10.525563754));
#224281=CARTESIAN_POINT('Ctrl Pts',(0.168330727999945,11.6,10.525563754));
#224282=CARTESIAN_POINT('Ctrl Pts',(0.167957322999944,15.2,10.523776458));
#224283=CARTESIAN_POINT('Ctrl Pts',(0.167957322999944,11.6,10.523776458));
#224284=CARTESIAN_POINT('Ctrl Pts',(0.167587068999945,15.2,10.521996069));
#224285=CARTESIAN_POINT('Ctrl Pts',(0.167587068999945,11.6,10.521996069));
#224286=CARTESIAN_POINT('Ctrl Pts',(0.167219954999943,15.2,10.520222605));
#224287=CARTESIAN_POINT('Ctrl Pts',(0.167219954999943,11.6,10.520222605));
#224288=CARTESIAN_POINT('Ctrl Pts',(0.166855973999944,15.2,10.518456083));
#224289=CARTESIAN_POINT('Ctrl Pts',(0.166855973999944,11.6,10.518456083));
#224290=CARTESIAN_POINT('Ctrl Pts',(0.166495116999944,15.2,10.516696527));
#224291=CARTESIAN_POINT('Ctrl Pts',(0.166495116999944,11.6,10.516696527));
#224292=CARTESIAN_POINT('Ctrl Pts',(0.166137373999945,15.2,10.514943952));
#224293=CARTESIAN_POINT('Ctrl Pts',(0.166137373999945,11.6,10.514943952));
#224294=CARTESIAN_POINT('Ctrl Pts',(0.165782736999944,15.2,10.513198379));
#224295=CARTESIAN_POINT('Ctrl Pts',(0.165782736999944,11.6,10.513198379));
#224296=CARTESIAN_POINT('Ctrl Pts',(0.165431195999943,15.2,10.511459827));
#224297=CARTESIAN_POINT('Ctrl Pts',(0.165431195999943,11.6,10.511459827));
#224298=CARTESIAN_POINT('Ctrl Pts',(0.165082743999945,15.2,10.509728314));
#224299=CARTESIAN_POINT('Ctrl Pts',(0.165082743999945,11.6,10.509728314));
#224300=CARTESIAN_POINT('Ctrl Pts',(0.164737370999944,15.2,10.508003861));
#224301=CARTESIAN_POINT('Ctrl Pts',(0.164737370999944,11.6,10.508003861));
#224302=CARTESIAN_POINT('Ctrl Pts',(0.164395066999944,15.2,10.506286488));
#224303=CARTESIAN_POINT('Ctrl Pts',(0.164395066999944,11.6,10.506286488));
#224304=CARTESIAN_POINT('Ctrl Pts',(0.164055823999943,15.2,10.504576213));
#224305=CARTESIAN_POINT('Ctrl Pts',(0.164055823999943,11.6,10.504576213));
#224306=CARTESIAN_POINT('Ctrl Pts',(0.163719631999945,15.2,10.502873055));
#224307=CARTESIAN_POINT('Ctrl Pts',(0.163719631999945,11.6,10.502873055));
#224308=CARTESIAN_POINT('Ctrl Pts',(0.163386482999943,15.2,10.501177035));
#224309=CARTESIAN_POINT('Ctrl Pts',(0.163386482999943,11.6,10.501177035));
#224310=CARTESIAN_POINT('Ctrl Pts',(0.163056365999944,15.2,10.499488173));
#224311=CARTESIAN_POINT('Ctrl Pts',(0.163056365999944,11.6,10.499488173));
#224312=CARTESIAN_POINT('Ctrl Pts',(0.162729271999943,15.2,10.497806487));
#224313=CARTESIAN_POINT('Ctrl Pts',(0.162729271999943,11.6,10.497806487));
#224314=CARTESIAN_POINT('Ctrl Pts',(0.162405193999945,15.2,10.496131999));
#224315=CARTESIAN_POINT('Ctrl Pts',(0.162405193999945,11.6,10.496131999));
#224316=CARTESIAN_POINT('Ctrl Pts',(0.162084119999945,15.2,10.494464727));
#224317=CARTESIAN_POINT('Ctrl Pts',(0.162084119999945,11.6,10.494464727));
#224318=CARTESIAN_POINT('Ctrl Pts',(0.161766040999943,15.2,10.492804693));
#224319=CARTESIAN_POINT('Ctrl Pts',(0.161766040999943,11.6,10.492804693));
#224320=CARTESIAN_POINT('Ctrl Pts',(0.161450947999944,15.2,10.491151915));
#224321=CARTESIAN_POINT('Ctrl Pts',(0.161450947999944,11.6,10.491151915));
#224322=CARTESIAN_POINT('Ctrl Pts',(0.161138831999944,15.2,10.489506414));
#224323=CARTESIAN_POINT('Ctrl Pts',(0.161138831999944,11.6,10.489506414));
#224324=CARTESIAN_POINT('Ctrl Pts',(0.160829681999944,15.2,10.487868211));
#224325=CARTESIAN_POINT('Ctrl Pts',(0.160829681999944,11.6,10.487868211));
#224326=CARTESIAN_POINT('Ctrl Pts',(0.160523488999944,15.2,10.486237324));
#224327=CARTESIAN_POINT('Ctrl Pts',(0.160523488999944,11.6,10.486237324));
#224328=CARTESIAN_POINT('Ctrl Pts',(0.160220243999945,15.2,10.484613776));
#224329=CARTESIAN_POINT('Ctrl Pts',(0.160220243999945,11.6,10.484613776));
#224330=CARTESIAN_POINT('Ctrl Pts',(0.159919935999945,15.2,10.482997587));
#224331=CARTESIAN_POINT('Ctrl Pts',(0.159919935999945,11.6,10.482997587));
#224332=CARTESIAN_POINT('Ctrl Pts',(0.159622555999944,15.2,10.481388775));
#224333=CARTESIAN_POINT('Ctrl Pts',(0.159622555999944,11.6,10.481388775));
#224334=CARTESIAN_POINT('Ctrl Pts',(0.159328093999944,15.2,10.479787363));
#224335=CARTESIAN_POINT('Ctrl Pts',(0.159328093999944,11.6,10.479787363));
#224336=CARTESIAN_POINT('Ctrl Pts',(0.159036538999944,15.2,10.478193371));
#224337=CARTESIAN_POINT('Ctrl Pts',(0.159036538999944,11.6,10.478193371));
#224338=CARTESIAN_POINT('Ctrl Pts',(0.158747883999943,15.2,10.476606819));
#224339=CARTESIAN_POINT('Ctrl Pts',(0.158747883999943,11.6,10.476606819));
#224340=CARTESIAN_POINT('Ctrl Pts',(0.158462115999944,15.2,10.475027729));
#224341=CARTESIAN_POINT('Ctrl Pts',(0.158462115999944,11.6,10.475027729));
#224342=CARTESIAN_POINT('Ctrl Pts',(0.158179225999945,15.2,10.473456121));
#224343=CARTESIAN_POINT('Ctrl Pts',(0.158179225999945,11.6,10.473456121));
#224344=CARTESIAN_POINT('Ctrl Pts',(0.157899203999945,15.2,10.471892016));
#224345=CARTESIAN_POINT('Ctrl Pts',(0.157899203999945,11.6,10.471892016));
#224346=CARTESIAN_POINT('Ctrl Pts',(0.157622040999945,15.2,10.470335436));
#224347=CARTESIAN_POINT('Ctrl Pts',(0.157622040999945,11.6,10.470335436));
#224348=CARTESIAN_POINT('Ctrl Pts',(0.157347723999944,15.2,10.4687864));
#224349=CARTESIAN_POINT('Ctrl Pts',(0.157347723999944,11.6,10.4687864));
#224350=CARTESIAN_POINT('Ctrl Pts',(0.157076244999944,15.2,10.467244932));
#224351=CARTESIAN_POINT('Ctrl Pts',(0.157076244999944,11.6,10.467244932));
#224352=CARTESIAN_POINT('Ctrl Pts',(0.156807592999944,15.2,10.46571105));
#224353=CARTESIAN_POINT('Ctrl Pts',(0.156807592999944,11.6,10.46571105));
#224354=CARTESIAN_POINT('Ctrl Pts',(0.156541757999945,15.2,10.464184777));
#224355=CARTESIAN_POINT('Ctrl Pts',(0.156541757999945,11.6,10.464184777));
#224356=CARTESIAN_POINT('Ctrl Pts',(0.156278728999943,15.2,10.462666136));
#224357=CARTESIAN_POINT('Ctrl Pts',(0.156278728999943,11.6,10.462666136));
#224358=CARTESIAN_POINT('Ctrl Pts',(0.156018494999944,15.2,10.461155145));
#224359=CARTESIAN_POINT('Ctrl Pts',(0.156018494999944,11.6,10.461155145));
#224360=CARTESIAN_POINT('Ctrl Pts',(0.155761047999944,15.2,10.459651829));
#224361=CARTESIAN_POINT('Ctrl Pts',(0.155761047999944,11.6,10.459651829));
#224362=CARTESIAN_POINT('Ctrl Pts',(0.155506374999945,15.2,10.458156207));
#224363=CARTESIAN_POINT('Ctrl Pts',(0.155506374999945,11.6,10.458156207));
#224364=CARTESIAN_POINT('Ctrl Pts',(0.155254464999944,15.2,10.456668303));
#224365=CARTESIAN_POINT('Ctrl Pts',(0.155254464999944,11.6,10.456668303));
#224366=CARTESIAN_POINT('Ctrl Pts',(0.155005309999944,15.2,10.455188137));
#224367=CARTESIAN_POINT('Ctrl Pts',(0.155005309999944,11.6,10.455188137));
#224368=CARTESIAN_POINT('Ctrl Pts',(0.154758896999944,15.2,10.45371573));
#224369=CARTESIAN_POINT('Ctrl Pts',(0.154758896999944,11.6,10.45371573));
#224370=CARTESIAN_POINT('Ctrl Pts',(0.154515215999943,15.2,10.452251107));
#224371=CARTESIAN_POINT('Ctrl Pts',(0.154515215999943,11.6,10.452251107));
#224372=CARTESIAN_POINT('Ctrl Pts',(0.154274255999944,15.2,10.450794288));
#224373=CARTESIAN_POINT('Ctrl Pts',(0.154274255999944,11.6,10.450794288));
#224374=CARTESIAN_POINT('Ctrl Pts',(0.154036005999943,15.2,10.449345296));
#224375=CARTESIAN_POINT('Ctrl Pts',(0.154036005999943,11.6,10.449345296));
#224376=CARTESIAN_POINT('Ctrl Pts',(0.153800454999944,15.2,10.447904152));
#224377=CARTESIAN_POINT('Ctrl Pts',(0.153800454999944,11.6,10.447904152));
#224378=CARTESIAN_POINT('Ctrl Pts',(0.153567591999944,15.2,10.44647088));
#224379=CARTESIAN_POINT('Ctrl Pts',(0.153567591999944,11.6,10.44647088));
#224380=CARTESIAN_POINT('Ctrl Pts',(0.153337406999944,15.2,10.445045501));
#224381=CARTESIAN_POINT('Ctrl Pts',(0.153337406999944,11.6,10.445045501));
#224382=CARTESIAN_POINT('Ctrl Pts',(0.153109886999945,15.2,10.443628039));
#224383=CARTESIAN_POINT('Ctrl Pts',(0.153109886999945,11.6,10.443628039));
#224384=CARTESIAN_POINT('Ctrl Pts',(0.152885021999944,15.2,10.442218514));
#224385=CARTESIAN_POINT('Ctrl Pts',(0.152885021999944,11.6,10.442218514));
#224386=CARTESIAN_POINT('Ctrl Pts',(0.152662799999945,15.2,10.440816951));
#224387=CARTESIAN_POINT('Ctrl Pts',(0.152662799999945,11.6,10.440816951));
#224388=CARTESIAN_POINT('Ctrl Pts',(0.152443210999945,15.2,10.439423373));
#224389=CARTESIAN_POINT('Ctrl Pts',(0.152443210999945,11.6,10.439423373));
#224390=CARTESIAN_POINT('Ctrl Pts',(0.152226241999944,15.2,10.4380378));
#224391=CARTESIAN_POINT('Ctrl Pts',(0.152226241999944,11.6,10.4380378));
#224392=CARTESIAN_POINT('Ctrl Pts',(0.152011882999944,15.2,10.436660258));
#224393=CARTESIAN_POINT('Ctrl Pts',(0.152011882999944,11.6,10.436660258));
#224394=CARTESIAN_POINT('Ctrl Pts',(0.151800121999944,15.2,10.435290769));
#224395=CARTESIAN_POINT('Ctrl Pts',(0.151800121999944,11.6,10.435290769));
#224396=CARTESIAN_POINT('Ctrl Pts',(0.151590946999944,15.2,10.433929355));
#224397=CARTESIAN_POINT('Ctrl Pts',(0.151590946999944,11.6,10.433929355));
#224398=CARTESIAN_POINT('Ctrl Pts',(0.151384345999944,15.2,10.432576041));
#224399=CARTESIAN_POINT('Ctrl Pts',(0.151384345999944,11.6,10.432576041));
#224400=CARTESIAN_POINT('Ctrl Pts',(0.151180308999944,15.2,10.431230849));
#224401=CARTESIAN_POINT('Ctrl Pts',(0.151180308999944,11.6,10.431230849));
#224402=CARTESIAN_POINT('Ctrl Pts',(0.150978822999944,15.2,10.429893802));
#224403=CARTESIAN_POINT('Ctrl Pts',(0.150978822999944,11.6,10.429893802));
#224404=CARTESIAN_POINT('Ctrl Pts',(0.150779875999945,15.2,10.428564925));
#224405=CARTESIAN_POINT('Ctrl Pts',(0.150779875999945,11.6,10.428564925));
#224406=CARTESIAN_POINT('Ctrl Pts',(0.150583456999945,15.2,10.427244241));
#224407=CARTESIAN_POINT('Ctrl Pts',(0.150583456999945,11.6,10.427244241));
#224408=CARTESIAN_POINT('Ctrl Pts',(0.150389552999943,15.2,10.425931773));
#224409=CARTESIAN_POINT('Ctrl Pts',(0.150389552999943,11.6,10.425931773));
#224410=CARTESIAN_POINT('Ctrl Pts',(0.150198153999943,15.2,10.424627546));
#224411=CARTESIAN_POINT('Ctrl Pts',(0.150198153999943,11.6,10.424627546));
#224412=CARTESIAN_POINT('Ctrl Pts',(0.150009245999945,15.2,10.423331583));
#224413=CARTESIAN_POINT('Ctrl Pts',(0.150009245999945,11.6,10.423331583));
#224414=CARTESIAN_POINT('Ctrl Pts',(0.149822815999944,15.2,10.422043908));
#224415=CARTESIAN_POINT('Ctrl Pts',(0.149822815999944,11.6,10.422043908));
#224416=CARTESIAN_POINT('Ctrl Pts',(0.149638854999944,15.2,10.420764544));
#224417=CARTESIAN_POINT('Ctrl Pts',(0.149638854999944,11.6,10.420764544));
#224418=CARTESIAN_POINT('Ctrl Pts',(0.149457348999944,15.2,10.419493518));
#224419=CARTESIAN_POINT('Ctrl Pts',(0.149457348999944,11.6,10.419493518));
#224420=CARTESIAN_POINT('Ctrl Pts',(0.149278284999944,15.2,10.418230853));
#224421=CARTESIAN_POINT('Ctrl Pts',(0.149278284999944,11.6,10.418230853));
#224422=CARTESIAN_POINT('Ctrl Pts',(0.149101651999944,15.2,10.416976571));
#224423=CARTESIAN_POINT('Ctrl Pts',(0.149101651999944,11.6,10.416976571));
#224424=CARTESIAN_POINT('Ctrl Pts',(0.148927436999945,15.2,10.4157307));
#224425=CARTESIAN_POINT('Ctrl Pts',(0.148927436999945,11.6,10.4157307));
#224426=CARTESIAN_POINT('Ctrl Pts',(0.148755626999945,15.2,10.414493263));
#224427=CARTESIAN_POINT('Ctrl Pts',(0.148755626999945,11.6,10.414493263));
#224428=CARTESIAN_POINT('Ctrl Pts',(0.148586208999945,15.2,10.413264284));
#224429=CARTESIAN_POINT('Ctrl Pts',(0.148586208999945,11.6,10.413264284));
#224430=CARTESIAN_POINT('Ctrl Pts',(0.148419171999944,15.2,10.412043789));
#224431=CARTESIAN_POINT('Ctrl Pts',(0.148419171999944,11.6,10.412043789));
#224432=CARTESIAN_POINT('Ctrl Pts',(0.148254501999944,15.2,10.410831802));
#224433=CARTESIAN_POINT('Ctrl Pts',(0.148254501999944,11.6,10.410831802));
#224434=CARTESIAN_POINT('Ctrl Pts',(0.148092186999945,15.2,10.409628349));
#224435=CARTESIAN_POINT('Ctrl Pts',(0.148092186999945,11.6,10.409628349));
#224436=CARTESIAN_POINT('Ctrl Pts',(0.147932212999944,15.2,10.408433454));
#224437=CARTESIAN_POINT('Ctrl Pts',(0.147932212999944,11.6,10.408433454));
#224438=CARTESIAN_POINT('Ctrl Pts',(0.147774568999944,15.2,10.407247143));
#224439=CARTESIAN_POINT('Ctrl Pts',(0.147774568999944,11.6,10.407247143));
#224440=CARTESIAN_POINT('Ctrl Pts',(0.147619239999944,15.2,10.40606944));
#224441=CARTESIAN_POINT('Ctrl Pts',(0.147619239999944,11.6,10.40606944));
#224442=CARTESIAN_POINT('Ctrl Pts',(0.147466212999945,15.2,10.404900372));
#224443=CARTESIAN_POINT('Ctrl Pts',(0.147466212999945,11.6,10.404900372));
#224444=CARTESIAN_POINT('Ctrl Pts',(0.147315476999944,15.2,10.403739964));
#224445=CARTESIAN_POINT('Ctrl Pts',(0.147315476999944,11.6,10.403739964));
#224446=CARTESIAN_POINT('Ctrl Pts',(0.147167015999944,15.2,10.402588242));
#224447=CARTESIAN_POINT('Ctrl Pts',(0.147167015999944,11.6,10.402588242));
#224448=CARTESIAN_POINT('Ctrl Pts',(0.147020819999945,15.2,10.401445231));
#224449=CARTESIAN_POINT('Ctrl Pts',(0.147020819999945,11.6,10.401445231));
#224450=CARTESIAN_POINT('Ctrl Pts',(0.146876870999944,15.2,10.400310958));
#224451=CARTESIAN_POINT('Ctrl Pts',(0.146876870999944,11.6,10.400310958));
#224452=CARTESIAN_POINT('Ctrl Pts',(0.146735159999943,15.2,10.399185447));
#224453=CARTESIAN_POINT('Ctrl Pts',(0.146735159999943,11.6,10.399185447));
#224454=CARTESIAN_POINT('Ctrl Pts',(0.146595670999944,15.2,10.398068726));
#224455=CARTESIAN_POINT('Ctrl Pts',(0.146595670999944,11.6,10.398068726));
#224456=CARTESIAN_POINT('Ctrl Pts',(0.146458390999945,15.2,10.39696082));
#224457=CARTESIAN_POINT('Ctrl Pts',(0.146458390999945,11.6,10.39696082));
#224458=CARTESIAN_POINT('Ctrl Pts',(0.146323305999945,15.2,10.395861757));
#224459=CARTESIAN_POINT('Ctrl Pts',(0.146323305999945,11.6,10.395861757));
#224460=CARTESIAN_POINT('Ctrl Pts',(0.146190402999944,15.2,10.39477156));
#224461=CARTESIAN_POINT('Ctrl Pts',(0.146190402999944,11.6,10.39477156));
#224462=CARTESIAN_POINT('Ctrl Pts',(0.146059667999945,15.2,10.39369026));
#224463=CARTESIAN_POINT('Ctrl Pts',(0.146059667999945,11.6,10.39369026));
#224464=CARTESIAN_POINT('Ctrl Pts',(0.145931086999944,15.2,10.392617881));
#224465=CARTESIAN_POINT('Ctrl Pts',(0.145931086999944,11.6,10.392617881));
#224466=CARTESIAN_POINT('Ctrl Pts',(0.145804644999944,15.2,10.391554451));
#224467=CARTESIAN_POINT('Ctrl Pts',(0.145804644999944,11.6,10.391554451));
#224468=CARTESIAN_POINT('Ctrl Pts',(0.145680329999944,15.2,10.390499995));
#224469=CARTESIAN_POINT('Ctrl Pts',(0.145680329999944,11.6,10.390499995));
#224470=CARTESIAN_POINT('Ctrl Pts',(0.145558125999944,15.2,10.389454543));
#224471=CARTESIAN_POINT('Ctrl Pts',(0.145558125999944,11.6,10.389454543));
#224472=CARTESIAN_POINT('Ctrl Pts',(0.145438019999944,15.2,10.38841812));
#224473=CARTESIAN_POINT('Ctrl Pts',(0.145438019999944,11.6,10.38841812));
#224474=CARTESIAN_POINT('Ctrl Pts',(0.145319995999945,15.2,10.387390753));
#224475=CARTESIAN_POINT('Ctrl Pts',(0.145319995999945,11.6,10.387390753));
#224476=CARTESIAN_POINT('Ctrl Pts',(0.145204040999944,15.2,10.386372471));
#224477=CARTESIAN_POINT('Ctrl Pts',(0.145204040999944,11.6,10.386372471));
#224478=CARTESIAN_POINT('Ctrl Pts',(0.145090141999944,15.2,10.3853633));
#224479=CARTESIAN_POINT('Ctrl Pts',(0.145090141999944,11.6,10.3853633));
#224480=CARTESIAN_POINT('Ctrl Pts',(0.144978279999943,15.2,10.384363269));
#224481=CARTESIAN_POINT('Ctrl Pts',(0.144978279999943,11.6,10.384363269));
#224482=CARTESIAN_POINT('Ctrl Pts',(0.144868444999944,15.2,10.383372406));
#224483=CARTESIAN_POINT('Ctrl Pts',(0.144868444999944,11.6,10.383372406));
#224484=CARTESIAN_POINT('Ctrl Pts',(0.144760618999945,15.2,10.382390738));
#224485=CARTESIAN_POINT('Ctrl Pts',(0.144760618999945,11.6,10.382390738));
#224486=CARTESIAN_POINT('Ctrl Pts',(0.144654789999944,15.2,10.381418293));
#224487=CARTESIAN_POINT('Ctrl Pts',(0.144654789999944,11.6,10.381418293));
#224488=CARTESIAN_POINT('Ctrl Pts',(0.144550940999943,15.2,10.3804551));
#224489=CARTESIAN_POINT('Ctrl Pts',(0.144550940999943,11.6,10.3804551));
#224490=CARTESIAN_POINT('Ctrl Pts',(0.144449056999945,15.2,10.379501187));
#224491=CARTESIAN_POINT('Ctrl Pts',(0.144449056999945,11.6,10.379501187));
#224492=CARTESIAN_POINT('Ctrl Pts',(0.144349124999945,15.2,10.378556581));
#224493=CARTESIAN_POINT('Ctrl Pts',(0.144349124999945,11.6,10.378556581));
#224494=CARTESIAN_POINT('Ctrl Pts',(0.144251126999944,15.2,10.377621314));
#224495=CARTESIAN_POINT('Ctrl Pts',(0.144251126999944,11.6,10.377621314));
#224496=CARTESIAN_POINT('Ctrl Pts',(0.144155048999943,15.2,10.376695411));
#224497=CARTESIAN_POINT('Ctrl Pts',(0.144155048999943,11.6,10.376695411));
#224498=CARTESIAN_POINT('Ctrl Pts',(0.144061419999945,15.2,10.375784182));
#224499=CARTESIAN_POINT('Ctrl Pts',(0.144061419999945,11.6,10.375784182));
#224500=CARTESIAN_POINT('Ctrl Pts',(0.143988113999944,15.2,10.375063685));
#224501=CARTESIAN_POINT('Ctrl Pts',(0.143988113999944,11.6,10.375063685));
#224502=CARTESIAN_POINT('Ctrl Pts',(0.143934094999943,15.2,10.374528791));
#224503=CARTESIAN_POINT('Ctrl Pts',(0.143934094999943,11.6,10.374528791));
#224504=CARTESIAN_POINT('Ctrl Pts',(0.143898617999945,15.2,10.374175763));
#224505=CARTESIAN_POINT('Ctrl Pts',(0.143898617999945,11.6,10.374175763));
#224506=CARTESIAN_POINT('Ctrl Pts',(0.143881226999945,15.2,10.374002275));
#224507=CARTESIAN_POINT('Ctrl Pts',(0.143881226999945,11.6,10.374002275));
#224508=CARTESIAN_POINT('',(0.143881226999945,12.2,10.374002275));
#224509=CARTESIAN_POINT('',(0.143881226999945,15.2,10.374002275));
#224510=CARTESIAN_POINT('',(0.143881226999945,12.2,10.374002275));
#224511=CARTESIAN_POINT('Ctrl Pts',(0.546958305999944,12.2,11.486985532));
#224512=CARTESIAN_POINT('Ctrl Pts',(0.546590898999945,12.2,11.486315008));
#224513=CARTESIAN_POINT('Ctrl Pts',(0.545856550999945,12.2,11.484974209));
#224514=CARTESIAN_POINT('Ctrl Pts',(0.544756420999944,12.2,11.482963756));
#224515=CARTESIAN_POINT('Ctrl Pts',(0.543292368999944,12.2,11.480284644));
#224516=CARTESIAN_POINT('Ctrl Pts',(0.541466945999944,12.2,11.476938237));
#224517=CARTESIAN_POINT('Ctrl Pts',(0.539646165999944,12.2,11.473594318));
#224518=CARTESIAN_POINT('Ctrl Pts',(0.537830029999945,12.2,11.470252887));
#224519=CARTESIAN_POINT('Ctrl Pts',(0.536018536999944,12.2,11.466913949));
#224520=CARTESIAN_POINT('Ctrl Pts',(0.534211683999944,12.2,11.46357751));
#224521=CARTESIAN_POINT('Ctrl Pts',(0.532409473999944,12.2,11.460243578));
#224522=CARTESIAN_POINT('Ctrl Pts',(0.530611901999943,12.2,11.456912161));
#224523=CARTESIAN_POINT('Ctrl Pts',(0.528818964999944,12.2,11.453583273));
#224524=CARTESIAN_POINT('Ctrl Pts',(0.527030663999944,12.2,11.450256921));
#224525=CARTESIAN_POINT('Ctrl Pts',(0.525246995999944,12.2,11.446933119));
#224526=CARTESIAN_POINT('Ctrl Pts',(0.523467958999944,12.2,11.443611876));
#224527=CARTESIAN_POINT('Ctrl Pts',(0.521693550999944,12.2,11.440293201));
#224528=CARTESIAN_POINT('Ctrl Pts',(0.519923770999945,12.2,11.436977102));
#224529=CARTESIAN_POINT('Ctrl Pts',(0.518158616999944,12.2,11.43366359));
#224530=CARTESIAN_POINT('Ctrl Pts',(0.516398088999944,12.2,11.43035267));
#224531=CARTESIAN_POINT('Ctrl Pts',(0.514642183999944,12.2,11.427044351));
#224532=CARTESIAN_POINT('Ctrl Pts',(0.512890899999944,12.2,11.423738642));
#224533=CARTESIAN_POINT('Ctrl Pts',(0.511144237999944,12.2,11.420435552));
#224534=CARTESIAN_POINT('Ctrl Pts',(0.509402193999944,12.2,11.417135088));
#224535=CARTESIAN_POINT('Ctrl Pts',(0.507664765999943,12.2,11.413837262));
#224536=CARTESIAN_POINT('Ctrl Pts',(0.505931953999944,12.2,11.410542081));
#224537=CARTESIAN_POINT('Ctrl Pts',(0.504203755999945,12.2,11.407249557));
#224538=CARTESIAN_POINT('Ctrl Pts',(0.502480167999945,12.2,11.403959697));
#224539=CARTESIAN_POINT('Ctrl Pts',(0.500761191999944,12.2,11.400672511));
#224540=CARTESIAN_POINT('Ctrl Pts',(0.499046822999943,12.2,11.397388008));
#224541=CARTESIAN_POINT('Ctrl Pts',(0.497337059999945,12.2,11.394106196));
#224542=CARTESIAN_POINT('Ctrl Pts',(0.495631902999945,12.2,11.390827085));
#224543=CARTESIAN_POINT('Ctrl Pts',(0.493931348999944,12.2,11.387550685));
#224544=CARTESIAN_POINT('Ctrl Pts',(0.492235395999945,12.2,11.384277002));
#224545=CARTESIAN_POINT('Ctrl Pts',(0.490544042999945,12.2,11.381006048));
#224546=CARTESIAN_POINT('Ctrl Pts',(0.488857286999943,12.2,11.37773783));
#224547=CARTESIAN_POINT('Ctrl Pts',(0.487175127999944,12.2,11.374472358));
#224548=CARTESIAN_POINT('Ctrl Pts',(0.485497562999945,12.2,11.371209642));
#224549=CARTESIAN_POINT('Ctrl Pts',(0.483824590999945,12.2,11.36794969));
#224550=CARTESIAN_POINT('Ctrl Pts',(0.482156208999944,12.2,11.364692512));
#224551=CARTESIAN_POINT('Ctrl Pts',(0.480492415999944,12.2,11.361438117));
#224552=CARTESIAN_POINT('Ctrl Pts',(0.478833209999945,12.2,11.358186515));
#224553=CARTESIAN_POINT('Ctrl Pts',(0.477178588999945,12.2,11.354937714));
#224554=CARTESIAN_POINT('Ctrl Pts',(0.475528549999943,12.2,11.351691724));
#224555=CARTESIAN_POINT('Ctrl Pts',(0.473883093999945,12.2,11.348448553));
#224556=CARTESIAN_POINT('Ctrl Pts',(0.472242216999945,12.2,11.345208212));
#224557=CARTESIAN_POINT('Ctrl Pts',(0.470605917999943,12.2,11.34197071));
#224558=CARTESIAN_POINT('Ctrl Pts',(0.468974193999945,12.2,11.338736055));
#224559=CARTESIAN_POINT('Ctrl Pts',(0.467347043999944,12.2,11.335504256));
#224560=CARTESIAN_POINT('Ctrl Pts',(0.465724464999945,12.2,11.332275324));
#224561=CARTESIAN_POINT('Ctrl Pts',(0.464106456999945,12.2,11.329049269));
#224562=CARTESIAN_POINT('Ctrl Pts',(0.462493016999945,12.2,11.325826099));
#224563=CARTESIAN_POINT('Ctrl Pts',(0.460884141999944,12.2,11.322605823));
#224564=CARTESIAN_POINT('Ctrl Pts',(0.459279831999944,12.2,11.319388451));
#224565=CARTESIAN_POINT('Ctrl Pts',(0.457680083999945,12.2,11.316173992));
#224566=CARTESIAN_POINT('Ctrl Pts',(0.456084895999943,12.2,11.312962457));
#224567=CARTESIAN_POINT('Ctrl Pts',(0.454494264999944,12.2,11.309753854));
#224568=CARTESIAN_POINT('Ctrl Pts',(0.452908190999944,12.2,11.306548191));
#224569=CARTESIAN_POINT('Ctrl Pts',(0.451326669999944,12.2,11.303345481));
#224570=CARTESIAN_POINT('Ctrl Pts',(0.449749701999943,12.2,11.300145732));
#224571=CARTESIAN_POINT('Ctrl Pts',(0.448177283999945,12.2,11.296948952));
#224572=CARTESIAN_POINT('Ctrl Pts',(0.446609412999944,12.2,11.293755151));
#224573=CARTESIAN_POINT('Ctrl Pts',(0.445046087999945,12.2,11.290564341));
#224574=CARTESIAN_POINT('Ctrl Pts',(0.443487306999945,12.2,11.287376529));
#224575=CARTESIAN_POINT('Ctrl Pts',(0.441933066999944,12.2,11.284191726));
#224576=CARTESIAN_POINT('Ctrl Pts',(0.440383366999945,12.2,11.28100994));
#224577=CARTESIAN_POINT('Ctrl Pts',(0.438838203999945,12.2,11.277831182));
#224578=CARTESIAN_POINT('Ctrl Pts',(0.437297575999944,12.2,11.27465546));
#224579=CARTESIAN_POINT('Ctrl Pts',(0.435761481999943,12.2,11.271482787));
#224580=CARTESIAN_POINT('Ctrl Pts',(0.434229916999945,12.2,11.268313168));
#224581=CARTESIAN_POINT('Ctrl Pts',(0.432397475066523,12.2,11.2645133069381));
#224582=CARTESIAN_POINT('Ctrl Pts',(0.430571823466653,12.2,11.260718059531));
#224583=CARTESIAN_POINT('Ctrl Pts',(0.428752956533235,12.2,11.256927442469));
#224584=CARTESIAN_POINT('Ctrl Pts',(0.426940870933362,12.2,11.2531414800619));
#224585=CARTESIAN_POINT('Ctrl Pts',(0.425135560999944,12.2,11.249360189));
#224586=CARTESIAN_POINT('Ctrl Pts',(0.423635651999945,12.2,11.246212238));
#224587=CARTESIAN_POINT('Ctrl Pts',(0.422140256999944,12.2,11.24306742));
#224588=CARTESIAN_POINT('Ctrl Pts',(0.420649371999945,12.2,11.239925747));
#224589=CARTESIAN_POINT('Ctrl Pts',(0.419162995999944,12.2,11.236787228));
#224590=CARTESIAN_POINT('Ctrl Pts',(0.417681126999945,12.2,11.233651872));
#224591=CARTESIAN_POINT('Ctrl Pts',(0.416203760999944,12.2,11.230519689));
#224592=CARTESIAN_POINT('Ctrl Pts',(0.414730897999943,12.2,11.227390689));
#224593=CARTESIAN_POINT('Ctrl Pts',(0.413262533999944,12.2,11.224264884));
#224594=CARTESIAN_POINT('Ctrl Pts',(0.411798665999944,12.2,11.22114228));
#224595=CARTESIAN_POINT('Ctrl Pts',(0.410339294999943,12.2,11.21802289));
#224596=CARTESIAN_POINT('Ctrl Pts',(0.408884414999945,12.2,11.214906723));
#224597=CARTESIAN_POINT('Ctrl Pts',(0.407434024999944,12.2,11.211793789));
#224598=CARTESIAN_POINT('Ctrl Pts',(0.405988121999944,12.2,11.208684097));
#224599=CARTESIAN_POINT('Ctrl Pts',(0.404546704999945,12.2,11.205577658));
#224600=CARTESIAN_POINT('Ctrl Pts',(0.403109770999944,12.2,11.202474482));
#224601=CARTESIAN_POINT('Ctrl Pts',(0.401677316999944,12.2,11.199374578));
#224602=CARTESIAN_POINT('Ctrl Pts',(0.400249340999944,12.2,11.196277957));
#224603=CARTESIAN_POINT('Ctrl Pts',(0.398825840999945,12.2,11.193184629));
#224604=CARTESIAN_POINT('Ctrl Pts',(0.397406813999943,12.2,11.190094604));
#224605=CARTESIAN_POINT('Ctrl Pts',(0.395992257999945,12.2,11.187007891));
#224606=CARTESIAN_POINT('Ctrl Pts',(0.394582168999945,12.2,11.183924503));
#224607=CARTESIAN_POINT('Ctrl Pts',(0.393176546999945,12.2,11.180844446));
#224608=CARTESIAN_POINT('Ctrl Pts',(0.391775385999944,12.2,11.177767734));
#224609=CARTESIAN_POINT('Ctrl Pts',(0.390378687999944,12.2,11.174694374));
#224610=CARTESIAN_POINT('Ctrl Pts',(0.388986445999944,12.2,11.171624378));
#224611=CARTESIAN_POINT('Ctrl Pts',(0.387598660999944,12.2,11.168557757));
#224612=CARTESIAN_POINT('Ctrl Pts',(0.386215327999944,12.2,11.165494518));
#224613=CARTESIAN_POINT('Ctrl Pts',(0.384836444999944,12.2,11.162434674));
#224614=CARTESIAN_POINT('Ctrl Pts',(0.383462009999944,12.2,11.159378235));
#224615=CARTESIAN_POINT('Ctrl Pts',(0.382092020999943,12.2,11.15632521));
#224616=CARTESIAN_POINT('Ctrl Pts',(0.380726473999945,12.2,11.15327561));
#224617=CARTESIAN_POINT('Ctrl Pts',(0.379365366999943,12.2,11.150229446));
#224618=CARTESIAN_POINT('Ctrl Pts',(0.378008696999944,12.2,11.147186727));
#224619=CARTESIAN_POINT('Ctrl Pts',(0.376656460999945,12.2,11.144147463));
#224620=CARTESIAN_POINT('Ctrl Pts',(0.375308657999945,12.2,11.141111667));
#224621=CARTESIAN_POINT('Ctrl Pts',(0.373965283999944,12.2,11.138079346));
#224622=CARTESIAN_POINT('Ctrl Pts',(0.372626335999945,12.2,11.135050513));
#224623=CARTESIAN_POINT('Ctrl Pts',(0.371291811999944,12.2,11.132025177));
#224624=CARTESIAN_POINT('Ctrl Pts',(0.369961708999943,12.2,11.129003348));
#224625=CARTESIAN_POINT('Ctrl Pts',(0.368636023999944,12.2,11.125985039));
#224626=CARTESIAN_POINT('Ctrl Pts',(0.367314755999945,12.2,11.122970257));
#224627=CARTESIAN_POINT('Ctrl Pts',(0.365997898999944,12.2,11.119959015));
#224628=CARTESIAN_POINT('Ctrl Pts',(0.364685451999945,12.2,11.116951322));
#224629=CARTESIAN_POINT('Ctrl Pts',(0.363377412999943,12.2,11.11394719));
#224630=CARTESIAN_POINT('Ctrl Pts',(0.362073778999944,12.2,11.110946629));
#224631=CARTESIAN_POINT('Ctrl Pts',(0.360774545999943,12.2,11.107949648));
#224632=CARTESIAN_POINT('Ctrl Pts',(0.359479711999944,12.2,11.104956259));
#224633=CARTESIAN_POINT('Ctrl Pts',(0.358189272999944,12.2,11.101966473));
#224634=CARTESIAN_POINT('Ctrl Pts',(0.356903226999944,12.2,11.0989803));
#224635=CARTESIAN_POINT('Ctrl Pts',(0.355621571999943,12.2,11.095997751));
#224636=CARTESIAN_POINT('Ctrl Pts',(0.354344304999945,12.2,11.093018835));
#224637=CARTESIAN_POINT('Ctrl Pts',(0.353071419999944,12.2,11.090043565));
#224638=CARTESIAN_POINT('Ctrl Pts',(0.351802917999944,12.2,11.087071951));
#224639=CARTESIAN_POINT('Ctrl Pts',(0.350538794999944,12.2,11.084104002));
#224640=CARTESIAN_POINT('Ctrl Pts',(0.349279045999945,12.2,11.081139731));
#224641=CARTESIAN_POINT('Ctrl Pts',(0.348023670999943,12.2,11.078179147));
#224642=CARTESIAN_POINT('Ctrl Pts',(0.346772663999945,12.2,11.075222263));
#224643=CARTESIAN_POINT('Ctrl Pts',(0.345526024999945,12.2,11.072269087));
#224644=CARTESIAN_POINT('Ctrl Pts',(0.344283748999944,12.2,11.069319631));
#224645=CARTESIAN_POINT('Ctrl Pts',(0.343045832999945,12.2,11.066373907));
#224646=CARTESIAN_POINT('Ctrl Pts',(0.341812274999944,12.2,11.063431924));
#224647=CARTESIAN_POINT('Ctrl Pts',(0.340583071999945,12.2,11.060493695));
#224648=CARTESIAN_POINT('Ctrl Pts',(0.339358218999944,12.2,11.057559229));
#224649=CARTESIAN_POINT('Ctrl Pts',(0.338137715999943,12.2,11.054628538));
#224650=CARTESIAN_POINT('Ctrl Pts',(0.336921556999944,12.2,11.051701632));
#224651=CARTESIAN_POINT('Ctrl Pts',(0.335709739999944,12.2,11.048778522));
#224652=CARTESIAN_POINT('Ctrl Pts',(0.334502261999944,12.2,11.04585922));
#224653=CARTESIAN_POINT('Ctrl Pts',(0.333299119999945,12.2,11.042943736));
#224654=CARTESIAN_POINT('Ctrl Pts',(0.332100310999944,12.2,11.040032081));
#224655=CARTESIAN_POINT('Ctrl Pts',(0.330905830999945,12.2,11.037124267));
#224656=CARTESIAN_POINT('Ctrl Pts',(0.329715676999944,12.2,11.034220304));
#224657=CARTESIAN_POINT('Ctrl Pts',(0.328529845999944,12.2,11.031320203));
#224658=CARTESIAN_POINT('Ctrl Pts',(0.327348334999943,12.2,11.028423977));
#224659=CARTESIAN_POINT('Ctrl Pts',(0.326171140999945,12.2,11.025531635));
#224660=CARTESIAN_POINT('Ctrl Pts',(0.324998259999945,12.2,11.02264319));
#224661=CARTESIAN_POINT('Ctrl Pts',(0.323829688999944,12.2,11.01975865));
#224662=CARTESIAN_POINT('Ctrl Pts',(0.322665423999944,12.2,11.016878029));
#224663=CARTESIAN_POINT('Ctrl Pts',(0.321505462999945,12.2,11.014001339));
#224664=CARTESIAN_POINT('Ctrl Pts',(0.320349802999944,12.2,11.011128587));
#224665=CARTESIAN_POINT('Ctrl Pts',(0.319198438999945,12.2,11.008259789));
#224666=CARTESIAN_POINT('Ctrl Pts',(0.318051368999944,12.2,11.005394953));
#224667=CARTESIAN_POINT('Ctrl Pts',(0.316908587999943,12.2,11.002534092));
#224668=CARTESIAN_POINT('Ctrl Pts',(0.315770094999944,12.2,10.999677217));
#224669=CARTESIAN_POINT('Ctrl Pts',(0.314635883999944,12.2,10.996824338));
#224670=CARTESIAN_POINT('Ctrl Pts',(0.313505953999943,12.2,10.993975469));
#224671=CARTESIAN_POINT('Ctrl Pts',(0.312380299999945,12.2,10.991130619));
#224672=CARTESIAN_POINT('Ctrl Pts',(0.311258918999944,12.2,10.988289801));
#224673=CARTESIAN_POINT('Ctrl Pts',(0.310141807999944,12.2,10.985453024));
#224674=CARTESIAN_POINT('Ctrl Pts',(0.309028961999944,12.2,10.982620303));
#224675=CARTESIAN_POINT('Ctrl Pts',(0.307920378999944,12.2,10.979791646));
#224676=CARTESIAN_POINT('Ctrl Pts',(0.306816055999944,12.2,10.976967067));
#224677=CARTESIAN_POINT('Ctrl Pts',(0.305715986999945,12.2,10.974146576));
#224678=CARTESIAN_POINT('Ctrl Pts',(0.304620169999945,12.2,10.971330186));
#224679=CARTESIAN_POINT('Ctrl Pts',(0.303528602999944,12.2,10.968517908));
#224680=CARTESIAN_POINT('Ctrl Pts',(0.302441278999943,12.2,10.965709751));
#224681=CARTESIAN_POINT('Ctrl Pts',(0.301358196999945,12.2,10.962905732));
#224682=CARTESIAN_POINT('Ctrl Pts',(0.300279352999944,12.2,10.960105857));
#224683=CARTESIAN_POINT('Ctrl Pts',(0.299204742999944,12.2,10.957310141));
#224684=CARTESIAN_POINT('Ctrl Pts',(0.298134362999944,12.2,10.954518595));
#224685=CARTESIAN_POINT('Ctrl Pts',(0.297068208999944,12.2,10.951731231));
#224686=CARTESIAN_POINT('Ctrl Pts',(0.296006278999944,12.2,10.94894806));
#224687=CARTESIAN_POINT('Ctrl Pts',(0.294948567999944,12.2,10.946169093));
#224688=CARTESIAN_POINT('Ctrl Pts',(0.293895072999945,12.2,10.943394344));
#224689=CARTESIAN_POINT('Ctrl Pts',(0.292845787999945,12.2,10.940623824));
#224690=CARTESIAN_POINT('Ctrl Pts',(0.291800711999944,12.2,10.937857544));
#224691=CARTESIAN_POINT('Ctrl Pts',(0.290759841999944,12.2,10.935095515));
#224692=CARTESIAN_POINT('Ctrl Pts',(0.289723169999944,12.2,10.932337751));
#224693=CARTESIAN_POINT('Ctrl Pts',(0.288690695999945,12.2,10.929584263));
#224694=CARTESIAN_POINT('Ctrl Pts',(0.287662414999945,12.2,10.926835064));
#224695=CARTESIAN_POINT('Ctrl Pts',(0.286638321999944,12.2,10.924090164));
#224696=CARTESIAN_POINT('Ctrl Pts',(0.285618414999943,12.2,10.921349576));
#224697=CARTESIAN_POINT('Ctrl Pts',(0.284602689999945,12.2,10.918613312));
#224698=CARTESIAN_POINT('Ctrl Pts',(0.283591139999944,12.2,10.915881383));
#224699=CARTESIAN_POINT('Ctrl Pts',(0.282583764999943,12.2,10.913153803));
#224700=CARTESIAN_POINT('Ctrl Pts',(0.281580559999943,12.2,10.910430582));
#224701=CARTESIAN_POINT('Ctrl Pts',(0.280581519999944,12.2,10.907711735));
#224702=CARTESIAN_POINT('Ctrl Pts',(0.279586641999944,12.2,10.904997271));
#224703=CARTESIAN_POINT('Ctrl Pts',(0.278595920999944,12.2,10.902287203));
#224704=CARTESIAN_POINT('Ctrl Pts',(0.277609353999945,12.2,10.899581544));
#224705=CARTESIAN_POINT('Ctrl Pts',(0.276626936999945,12.2,10.896880306));
#224706=CARTESIAN_POINT('Ctrl Pts',(0.275648663999943,12.2,10.894183501));
#224707=CARTESIAN_POINT('Ctrl Pts',(0.274674533999945,12.2,10.89149114));
#224708=CARTESIAN_POINT('Ctrl Pts',(0.273704539999944,12.2,10.888803238));
#224709=CARTESIAN_POINT('Ctrl Pts',(0.272738680999945,12.2,10.886119805));
#224710=CARTESIAN_POINT('Ctrl Pts',(0.271776950999945,12.2,10.883440855));
#224711=CARTESIAN_POINT('Ctrl Pts',(0.270819344999945,12.2,10.880766399));
#224712=CARTESIAN_POINT('Ctrl Pts',(0.269865859999945,12.2,10.878096449));
#224713=CARTESIAN_POINT('Ctrl Pts',(0.268916491999944,12.2,10.875431019));
#224714=CARTESIAN_POINT('Ctrl Pts',(0.267971236999944,12.2,10.872770121));
#224715=CARTESIAN_POINT('Ctrl Pts',(0.267030088999943,12.2,10.870113767));
#224716=CARTESIAN_POINT('Ctrl Pts',(0.266093045999943,12.2,10.867461969));
#224717=CARTESIAN_POINT('Ctrl Pts',(0.265160102999945,12.2,10.864814741));
#224718=CARTESIAN_POINT('Ctrl Pts',(0.264231254999944,12.2,10.862172095));
#224719=CARTESIAN_POINT('Ctrl Pts',(0.263306497999943,12.2,10.859534043));
#224720=CARTESIAN_POINT('Ctrl Pts',(0.262385827999945,12.2,10.856900597));
#224721=CARTESIAN_POINT('Ctrl Pts',(0.261469239999944,12.2,10.854271772));
#224722=CARTESIAN_POINT('Ctrl Pts',(0.260556730999945,12.2,10.851647579));
#224723=CARTESIAN_POINT('Ctrl Pts',(0.259648296999944,12.2,10.84902803));
#224724=CARTESIAN_POINT('Ctrl Pts',(0.258743930999945,12.2,10.846413139));
#224725=CARTESIAN_POINT('Ctrl Pts',(0.257843629999943,12.2,10.843802919));
#224726=CARTESIAN_POINT('Ctrl Pts',(0.256947389999944,12.2,10.841197381));
#224727=CARTESIAN_POINT('Ctrl Pts',(0.256055205999944,12.2,10.838596539));
#224728=CARTESIAN_POINT('Ctrl Pts',(0.255167071999944,12.2,10.836000406));
#224729=CARTESIAN_POINT('Ctrl Pts',(0.254282986999945,12.2,10.833408995));
#224730=CARTESIAN_POINT('Ctrl Pts',(0.253402944999944,12.2,10.830822318));
#224731=CARTESIAN_POINT('Ctrl Pts',(0.252526938999944,12.2,10.828240388));
#224732=CARTESIAN_POINT('Ctrl Pts',(0.251654968999944,12.2,10.825663219));
#224733=CARTESIAN_POINT('Ctrl Pts',(0.250787026999945,12.2,10.823090823));
#224734=CARTESIAN_POINT('Ctrl Pts',(0.249923107999944,12.2,10.820523213));
#224735=CARTESIAN_POINT('Ctrl Pts',(0.249063209999945,12.2,10.817960403));
#224736=CARTESIAN_POINT('Ctrl Pts',(0.248207326999944,12.2,10.815402405));
#224737=CARTESIAN_POINT('Ctrl Pts',(0.247355453999945,12.2,10.812849232));
#224738=CARTESIAN_POINT('Ctrl Pts',(0.246507586999943,12.2,10.810300898));
#224739=CARTESIAN_POINT('Ctrl Pts',(0.245663720999945,12.2,10.807757416));
#224740=CARTESIAN_POINT('Ctrl Pts',(0.244823849999944,12.2,10.805218799));
#224741=CARTESIAN_POINT('Ctrl Pts',(0.243987971999945,12.2,10.80268506));
#224742=CARTESIAN_POINT('Ctrl Pts',(0.243156079999943,12.2,10.800156212));
#224743=CARTESIAN_POINT('Ctrl Pts',(0.242328170999944,12.2,10.797632269));
#224744=CARTESIAN_POINT('Ctrl Pts',(0.241504236999944,12.2,10.795113244));
#224745=CARTESIAN_POINT('Ctrl Pts',(0.240684276999945,12.2,10.79259915));
#224746=CARTESIAN_POINT('Ctrl Pts',(0.239868283999943,12.2,10.790090001));
#224747=CARTESIAN_POINT('Ctrl Pts',(0.239056252999944,12.2,10.78758581));
#224748=CARTESIAN_POINT('Ctrl Pts',(0.238248179999945,12.2,10.78508659));
#224749=CARTESIAN_POINT('Ctrl Pts',(0.237444059999945,12.2,10.782592356));
#224750=CARTESIAN_POINT('Ctrl Pts',(0.236643886999944,12.2,10.780103119));
#224751=CARTESIAN_POINT('Ctrl Pts',(0.235847656999945,12.2,10.777618895));
#224752=CARTESIAN_POINT('Ctrl Pts',(0.235055364999944,12.2,10.775139696));
#224753=CARTESIAN_POINT('Ctrl Pts',(0.234267004999945,12.2,10.772665536));
#224754=CARTESIAN_POINT('Ctrl Pts',(0.233482572999945,12.2,10.770196429));
#224755=CARTESIAN_POINT('Ctrl Pts',(0.232702063999944,12.2,10.767732388));
#224756=CARTESIAN_POINT('Ctrl Pts',(0.231925471999944,12.2,10.765273427));
#224757=CARTESIAN_POINT('Ctrl Pts',(0.231152791999945,12.2,10.762819561));
#224758=CARTESIAN_POINT('Ctrl Pts',(0.230384019999944,12.2,10.760370801));
#224759=CARTESIAN_POINT('Ctrl Pts',(0.229619148999944,12.2,10.757927164));
#224760=CARTESIAN_POINT('Ctrl Pts',(0.228858174999944,12.2,10.755488661));
#224761=CARTESIAN_POINT('Ctrl Pts',(0.228101093999945,12.2,10.753055306));
#224762=CARTESIAN_POINT('Ctrl Pts',(0.227347897999944,12.2,10.750627115));
#224763=CARTESIAN_POINT('Ctrl Pts',(0.226598583999945,12.2,10.748204101));
#224764=CARTESIAN_POINT('Ctrl Pts',(0.225853144999943,12.2,10.745786278));
#224765=CARTESIAN_POINT('Ctrl Pts',(0.225111577999944,12.2,10.743373659));
#224766=CARTESIAN_POINT('Ctrl Pts',(0.224373874999945,12.2,10.740966259));
#224767=CARTESIAN_POINT('Ctrl Pts',(0.223640032999944,12.2,10.738564091));
#224768=CARTESIAN_POINT('Ctrl Pts',(0.222910043999944,12.2,10.736167171));
#224769=CARTESIAN_POINT('Ctrl Pts',(0.222183904999945,12.2,10.733775512));
#224770=CARTESIAN_POINT('Ctrl Pts',(0.221461608999943,12.2,10.731389127));
#224771=CARTESIAN_POINT('Ctrl Pts',(0.220743151999944,12.2,10.729008033));
#224772=CARTESIAN_POINT('Ctrl Pts',(0.220028526999944,12.2,10.726632242));
#224773=CARTESIAN_POINT('Ctrl Pts',(0.219317728999944,12.2,10.724261769));
#224774=CARTESIAN_POINT('Ctrl Pts',(0.218610752999944,12.2,10.721896627));
#224775=CARTESIAN_POINT('Ctrl Pts',(0.217907592999945,12.2,10.719536832));
#224776=CARTESIAN_POINT('Ctrl Pts',(0.217208243999943,12.2,10.717182399));
#224777=CARTESIAN_POINT('Ctrl Pts',(0.216512699999944,12.2,10.71483334));
#224778=CARTESIAN_POINT('Ctrl Pts',(0.215820953999944,12.2,10.712489672));
#224779=CARTESIAN_POINT('Ctrl Pts',(0.215133002999943,12.2,10.710151408));
#224780=CARTESIAN_POINT('Ctrl Pts',(0.214448838999944,12.2,10.707818563));
#224781=CARTESIAN_POINT('Ctrl Pts',(0.213768457999944,12.2,10.70549115));
#224782=CARTESIAN_POINT('Ctrl Pts',(0.213091851999945,12.2,10.703169186));
#224783=CARTESIAN_POINT('Ctrl Pts',(0.212419017999944,12.2,10.700852684));
#224784=CARTESIAN_POINT('Ctrl Pts',(0.211749947999945,12.2,10.69854166));
#224785=CARTESIAN_POINT('Ctrl Pts',(0.211084637999944,12.2,10.696236128));
#224786=CARTESIAN_POINT('Ctrl Pts',(0.210423080999943,12.2,10.693936102));
#224787=CARTESIAN_POINT('Ctrl Pts',(0.209765270999943,12.2,10.691641598));
#224788=CARTESIAN_POINT('Ctrl Pts',(0.209111202999944,12.2,10.68935263));
#224789=CARTESIAN_POINT('Ctrl Pts',(0.208460869999945,12.2,10.687069213));
#224790=CARTESIAN_POINT('Ctrl Pts',(0.207814266999945,12.2,10.684791362));
#224791=CARTESIAN_POINT('Ctrl Pts',(0.207171385999944,12.2,10.682519093));
#224792=CARTESIAN_POINT('Ctrl Pts',(0.206532223999943,12.2,10.680252419));
#224793=CARTESIAN_POINT('Ctrl Pts',(0.205896773999944,12.2,10.677991356));
#224794=CARTESIAN_POINT('Ctrl Pts',(0.205265027999945,12.2,10.67573592));
#224795=CARTESIAN_POINT('Ctrl Pts',(0.204636982999944,12.2,10.673486125));
#224796=CARTESIAN_POINT('Ctrl Pts',(0.204012629999945,12.2,10.671241985));
#224797=CARTESIAN_POINT('Ctrl Pts',(0.203391963999945,12.2,10.669003518));
#224798=CARTESIAN_POINT('Ctrl Pts',(0.202774978999944,12.2,10.666770738));
#224799=CARTESIAN_POINT('Ctrl Pts',(0.202161669999944,12.2,10.664543659));
#224800=CARTESIAN_POINT('Ctrl Pts',(0.201552027999944,12.2,10.662322298));
#224801=CARTESIAN_POINT('Ctrl Pts',(0.200946048999944,12.2,10.660106669));
#224802=CARTESIAN_POINT('Ctrl Pts',(0.200343724999945,12.2,10.657896788));
#224803=CARTESIAN_POINT('Ctrl Pts',(0.199745050999944,12.2,10.655692671));
#224804=CARTESIAN_POINT('Ctrl Pts',(0.199150019999944,12.2,10.653494334));
#224805=CARTESIAN_POINT('Ctrl Pts',(0.198558625999944,12.2,10.651301789));
#224806=CARTESIAN_POINT('Ctrl Pts',(0.197970861999943,12.2,10.649115056));
#224807=CARTESIAN_POINT('Ctrl Pts',(0.197386722999945,12.2,10.646934148));
#224808=CARTESIAN_POINT('Ctrl Pts',(0.196806200999945,12.2,10.644759081));
#224809=CARTESIAN_POINT('Ctrl Pts',(0.196229288999945,12.2,10.642589871));
#224810=CARTESIAN_POINT('Ctrl Pts',(0.195655981999945,12.2,10.640426535));
#224811=CARTESIAN_POINT('Ctrl Pts',(0.195086272999945,12.2,10.638269086));
#224812=CARTESIAN_POINT('Ctrl Pts',(0.194520154999944,12.2,10.636117541));
#224813=CARTESIAN_POINT('Ctrl Pts',(0.193957621999944,12.2,10.633971917));
#224814=CARTESIAN_POINT('Ctrl Pts',(0.193398666999943,12.2,10.631832228));
#224815=CARTESIAN_POINT('Ctrl Pts',(0.192843282999944,12.2,10.629698493));
#224816=CARTESIAN_POINT('Ctrl Pts',(0.192291463999944,12.2,10.627570724));
#224817=CARTESIAN_POINT('Ctrl Pts',(0.191743202999944,12.2,10.62544894));
#224818=CARTESIAN_POINT('Ctrl Pts',(0.191198490999945,12.2,10.623333156));
#224819=CARTESIAN_POINT('Ctrl Pts',(0.190657324999943,12.2,10.621223388));
#224820=CARTESIAN_POINT('Ctrl Pts',(0.190119695999943,12.2,10.619119652));
#224821=CARTESIAN_POINT('Ctrl Pts',(0.189585597999944,12.2,10.617021966));
#224822=CARTESIAN_POINT('Ctrl Pts',(0.189055023999943,12.2,10.614930343));
#224823=CARTESIAN_POINT('Ctrl Pts',(0.188527964999944,12.2,10.612844803));
#224824=CARTESIAN_POINT('Ctrl Pts',(0.188004415999944,12.2,10.61076536));
#224825=CARTESIAN_POINT('Ctrl Pts',(0.187484369999943,12.2,10.608692031));
#224826=CARTESIAN_POINT('Ctrl Pts',(0.186967819999945,12.2,10.606624832));
#224827=CARTESIAN_POINT('Ctrl Pts',(0.186454757999943,12.2,10.604563781));
#224828=CARTESIAN_POINT('Ctrl Pts',(0.185945176999944,12.2,10.602508892));
#224829=CARTESIAN_POINT('Ctrl Pts',(0.185439070999944,12.2,10.600460184));
#224830=CARTESIAN_POINT('Ctrl Pts',(0.184936431999944,12.2,10.598417673));
#224831=CARTESIAN_POINT('Ctrl Pts',(0.184437252999944,12.2,10.596381375));
#224832=CARTESIAN_POINT('Ctrl Pts',(0.183941525999943,12.2,10.594351307));
#224833=CARTESIAN_POINT('Ctrl Pts',(0.183449243999944,12.2,10.592327487));
#224834=CARTESIAN_POINT('Ctrl Pts',(0.182960400999944,12.2,10.59030993));
#224835=CARTESIAN_POINT('Ctrl Pts',(0.182474987999944,12.2,10.588298654));
#224836=CARTESIAN_POINT('Ctrl Pts',(0.181992997999944,12.2,10.586293676));
#224837=CARTESIAN_POINT('Ctrl Pts',(0.181514424999945,12.2,10.584295013));
#224838=CARTESIAN_POINT('Ctrl Pts',(0.181039259999943,12.2,10.582302681));
#224839=CARTESIAN_POINT('Ctrl Pts',(0.180567494999944,12.2,10.580316698));
#224840=CARTESIAN_POINT('Ctrl Pts',(0.180099123999945,12.2,10.578337082));
#224841=CARTESIAN_POINT('Ctrl Pts',(0.179634138999945,12.2,10.576363848));
#224842=CARTESIAN_POINT('Ctrl Pts',(0.179172531999944,12.2,10.574397014));
#224843=CARTESIAN_POINT('Ctrl Pts',(0.178714295999944,12.2,10.5724366));
#224844=CARTESIAN_POINT('Ctrl Pts',(0.178259421999943,12.2,10.570482619));
#224845=CARTESIAN_POINT('Ctrl Pts',(0.177807903999945,12.2,10.568535092));
#224846=CARTESIAN_POINT('Ctrl Pts',(0.177359733999944,12.2,10.566594034));
#224847=CARTESIAN_POINT('Ctrl Pts',(0.176914901999944,12.2,10.564659464));
#224848=CARTESIAN_POINT('Ctrl Pts',(0.176473402999945,12.2,10.5627314));
#224849=CARTESIAN_POINT('Ctrl Pts',(0.176035227999943,12.2,10.560809858));
#224850=CARTESIAN_POINT('Ctrl Pts',(0.175600368999945,12.2,10.558894856));
#224851=CARTESIAN_POINT('Ctrl Pts',(0.175168817999944,12.2,10.556986414));
#224852=CARTESIAN_POINT('Ctrl Pts',(0.174740566999944,12.2,10.555084546));
#224853=CARTESIAN_POINT('Ctrl Pts',(0.174315608999944,12.2,10.553189272));
#224854=CARTESIAN_POINT('Ctrl Pts',(0.173893933999943,12.2,10.551300611));
#224855=CARTESIAN_POINT('Ctrl Pts',(0.173475535999945,12.2,10.549418579));
#224856=CARTESIAN_POINT('Ctrl Pts',(0.173060405999944,12.2,10.547543196));
#224857=CARTESIAN_POINT('Ctrl Pts',(0.172648535999944,12.2,10.545674477));
#224858=CARTESIAN_POINT('Ctrl Pts',(0.172239915999944,12.2,10.543812444));
#224859=CARTESIAN_POINT('Ctrl Pts',(0.171834540999944,12.2,10.541957111));
#224860=CARTESIAN_POINT('Ctrl Pts',(0.171432399999943,12.2,10.5401085));
#224861=CARTESIAN_POINT('Ctrl Pts',(0.171033485999944,12.2,10.538266627));
#224862=CARTESIAN_POINT('Ctrl Pts',(0.170637789999945,12.2,10.536431512));
#224863=CARTESIAN_POINT('Ctrl Pts',(0.170245304999943,12.2,10.534603171));
#224864=CARTESIAN_POINT('Ctrl Pts',(0.169856019999944,12.2,10.532781625));
#224865=CARTESIAN_POINT('Ctrl Pts',(0.169469929999944,12.2,10.530966892));
#224866=CARTESIAN_POINT('Ctrl Pts',(0.169087021999944,12.2,10.52915899));
#224867=CARTESIAN_POINT('Ctrl Pts',(0.168707291999944,12.2,10.527357938));
#224868=CARTESIAN_POINT('Ctrl Pts',(0.168330727999945,12.2,10.525563754));
#224869=CARTESIAN_POINT('Ctrl Pts',(0.167957322999944,12.2,10.523776458));
#224870=CARTESIAN_POINT('Ctrl Pts',(0.167587068999945,12.2,10.521996069));
#224871=CARTESIAN_POINT('Ctrl Pts',(0.167219954999943,12.2,10.520222605));
#224872=CARTESIAN_POINT('Ctrl Pts',(0.166855973999944,12.2,10.518456083));
#224873=CARTESIAN_POINT('Ctrl Pts',(0.166495116999944,12.2,10.516696527));
#224874=CARTESIAN_POINT('Ctrl Pts',(0.166137373999945,12.2,10.514943952));
#224875=CARTESIAN_POINT('Ctrl Pts',(0.165782736999944,12.2,10.513198379));
#224876=CARTESIAN_POINT('Ctrl Pts',(0.165431195999943,12.2,10.511459827));
#224877=CARTESIAN_POINT('Ctrl Pts',(0.165082743999945,12.2,10.509728314));
#224878=CARTESIAN_POINT('Ctrl Pts',(0.164737370999944,12.2,10.508003861));
#224879=CARTESIAN_POINT('Ctrl Pts',(0.164395066999944,12.2,10.506286488));
#224880=CARTESIAN_POINT('Ctrl Pts',(0.164055823999943,12.2,10.504576213));
#224881=CARTESIAN_POINT('Ctrl Pts',(0.163719631999945,12.2,10.502873055));
#224882=CARTESIAN_POINT('Ctrl Pts',(0.163386482999943,12.2,10.501177035));
#224883=CARTESIAN_POINT('Ctrl Pts',(0.163056365999944,12.2,10.499488173));
#224884=CARTESIAN_POINT('Ctrl Pts',(0.162729271999943,12.2,10.497806487));
#224885=CARTESIAN_POINT('Ctrl Pts',(0.162405193999945,12.2,10.496131999));
#224886=CARTESIAN_POINT('Ctrl Pts',(0.162084119999945,12.2,10.494464727));
#224887=CARTESIAN_POINT('Ctrl Pts',(0.161766040999943,12.2,10.492804693));
#224888=CARTESIAN_POINT('Ctrl Pts',(0.161450947999944,12.2,10.491151915));
#224889=CARTESIAN_POINT('Ctrl Pts',(0.161138831999944,12.2,10.489506414));
#224890=CARTESIAN_POINT('Ctrl Pts',(0.160829681999944,12.2,10.487868211));
#224891=CARTESIAN_POINT('Ctrl Pts',(0.160523488999944,12.2,10.486237324));
#224892=CARTESIAN_POINT('Ctrl Pts',(0.160220243999945,12.2,10.484613776));
#224893=CARTESIAN_POINT('Ctrl Pts',(0.159919935999945,12.2,10.482997587));
#224894=CARTESIAN_POINT('Ctrl Pts',(0.159622555999944,12.2,10.481388775));
#224895=CARTESIAN_POINT('Ctrl Pts',(0.159328093999944,12.2,10.479787363));
#224896=CARTESIAN_POINT('Ctrl Pts',(0.159036538999944,12.2,10.478193371));
#224897=CARTESIAN_POINT('Ctrl Pts',(0.158747883999943,12.2,10.476606819));
#224898=CARTESIAN_POINT('Ctrl Pts',(0.158462115999944,12.2,10.475027729));
#224899=CARTESIAN_POINT('Ctrl Pts',(0.158179225999945,12.2,10.473456121));
#224900=CARTESIAN_POINT('Ctrl Pts',(0.157899203999945,12.2,10.471892016));
#224901=CARTESIAN_POINT('Ctrl Pts',(0.157622040999945,12.2,10.470335436));
#224902=CARTESIAN_POINT('Ctrl Pts',(0.157347723999944,12.2,10.4687864));
#224903=CARTESIAN_POINT('Ctrl Pts',(0.157076244999944,12.2,10.467244932));
#224904=CARTESIAN_POINT('Ctrl Pts',(0.156807592999944,12.2,10.46571105));
#224905=CARTESIAN_POINT('Ctrl Pts',(0.156541757999945,12.2,10.464184777));
#224906=CARTESIAN_POINT('Ctrl Pts',(0.156278728999943,12.2,10.462666136));
#224907=CARTESIAN_POINT('Ctrl Pts',(0.156018494999944,12.2,10.461155145));
#224908=CARTESIAN_POINT('Ctrl Pts',(0.155761047999944,12.2,10.459651829));
#224909=CARTESIAN_POINT('Ctrl Pts',(0.155506374999945,12.2,10.458156207));
#224910=CARTESIAN_POINT('Ctrl Pts',(0.155254464999944,12.2,10.456668303));
#224911=CARTESIAN_POINT('Ctrl Pts',(0.155005309999944,12.2,10.455188137));
#224912=CARTESIAN_POINT('Ctrl Pts',(0.154758896999944,12.2,10.45371573));
#224913=CARTESIAN_POINT('Ctrl Pts',(0.154515215999943,12.2,10.452251107));
#224914=CARTESIAN_POINT('Ctrl Pts',(0.154274255999944,12.2,10.450794288));
#224915=CARTESIAN_POINT('Ctrl Pts',(0.154036005999943,12.2,10.449345296));
#224916=CARTESIAN_POINT('Ctrl Pts',(0.153800454999944,12.2,10.447904152));
#224917=CARTESIAN_POINT('Ctrl Pts',(0.153567591999944,12.2,10.44647088));
#224918=CARTESIAN_POINT('Ctrl Pts',(0.153337406999944,12.2,10.445045501));
#224919=CARTESIAN_POINT('Ctrl Pts',(0.153109886999945,12.2,10.443628039));
#224920=CARTESIAN_POINT('Ctrl Pts',(0.152885021999944,12.2,10.442218514));
#224921=CARTESIAN_POINT('Ctrl Pts',(0.152662799999945,12.2,10.440816951));
#224922=CARTESIAN_POINT('Ctrl Pts',(0.152443210999945,12.2,10.439423373));
#224923=CARTESIAN_POINT('Ctrl Pts',(0.152226241999944,12.2,10.4380378));
#224924=CARTESIAN_POINT('Ctrl Pts',(0.152011882999944,12.2,10.436660258));
#224925=CARTESIAN_POINT('Ctrl Pts',(0.151800121999944,12.2,10.435290769));
#224926=CARTESIAN_POINT('Ctrl Pts',(0.151590946999944,12.2,10.433929355));
#224927=CARTESIAN_POINT('Ctrl Pts',(0.151384345999944,12.2,10.432576041));
#224928=CARTESIAN_POINT('Ctrl Pts',(0.151180308999944,12.2,10.431230849));
#224929=CARTESIAN_POINT('Ctrl Pts',(0.150978822999944,12.2,10.429893802));
#224930=CARTESIAN_POINT('Ctrl Pts',(0.150779875999945,12.2,10.428564925));
#224931=CARTESIAN_POINT('Ctrl Pts',(0.150583456999945,12.2,10.427244241));
#224932=CARTESIAN_POINT('Ctrl Pts',(0.150389552999943,12.2,10.425931773));
#224933=CARTESIAN_POINT('Ctrl Pts',(0.150198153999943,12.2,10.424627546));
#224934=CARTESIAN_POINT('Ctrl Pts',(0.150009245999945,12.2,10.423331583));
#224935=CARTESIAN_POINT('Ctrl Pts',(0.149822815999944,12.2,10.422043908));
#224936=CARTESIAN_POINT('Ctrl Pts',(0.149638854999944,12.2,10.420764544));
#224937=CARTESIAN_POINT('Ctrl Pts',(0.149457348999944,12.2,10.419493518));
#224938=CARTESIAN_POINT('Ctrl Pts',(0.149278284999944,12.2,10.418230853));
#224939=CARTESIAN_POINT('Ctrl Pts',(0.149101651999944,12.2,10.416976571));
#224940=CARTESIAN_POINT('Ctrl Pts',(0.148927436999945,12.2,10.4157307));
#224941=CARTESIAN_POINT('Ctrl Pts',(0.148755626999945,12.2,10.414493263));
#224942=CARTESIAN_POINT('Ctrl Pts',(0.148586208999945,12.2,10.413264284));
#224943=CARTESIAN_POINT('Ctrl Pts',(0.148419171999944,12.2,10.412043789));
#224944=CARTESIAN_POINT('Ctrl Pts',(0.148254501999944,12.2,10.410831802));
#224945=CARTESIAN_POINT('Ctrl Pts',(0.148092186999945,12.2,10.409628349));
#224946=CARTESIAN_POINT('Ctrl Pts',(0.147932212999944,12.2,10.408433454));
#224947=CARTESIAN_POINT('Ctrl Pts',(0.147774568999944,12.2,10.407247143));
#224948=CARTESIAN_POINT('Ctrl Pts',(0.147619239999944,12.2,10.40606944));
#224949=CARTESIAN_POINT('Ctrl Pts',(0.147466212999945,12.2,10.404900372));
#224950=CARTESIAN_POINT('Ctrl Pts',(0.147315476999944,12.2,10.403739964));
#224951=CARTESIAN_POINT('Ctrl Pts',(0.147167015999944,12.2,10.402588242));
#224952=CARTESIAN_POINT('Ctrl Pts',(0.147020819999945,12.2,10.401445231));
#224953=CARTESIAN_POINT('Ctrl Pts',(0.146876870999944,12.2,10.400310958));
#224954=CARTESIAN_POINT('Ctrl Pts',(0.146735159999943,12.2,10.399185447));
#224955=CARTESIAN_POINT('Ctrl Pts',(0.146595670999944,12.2,10.398068726));
#224956=CARTESIAN_POINT('Ctrl Pts',(0.146458390999945,12.2,10.39696082));
#224957=CARTESIAN_POINT('Ctrl Pts',(0.146323305999945,12.2,10.395861757));
#224958=CARTESIAN_POINT('Ctrl Pts',(0.146190402999944,12.2,10.39477156));
#224959=CARTESIAN_POINT('Ctrl Pts',(0.146059667999945,12.2,10.39369026));
#224960=CARTESIAN_POINT('Ctrl Pts',(0.145931086999944,12.2,10.392617881));
#224961=CARTESIAN_POINT('Ctrl Pts',(0.145804644999944,12.2,10.391554451));
#224962=CARTESIAN_POINT('Ctrl Pts',(0.145680329999944,12.2,10.390499995));
#224963=CARTESIAN_POINT('Ctrl Pts',(0.145558125999944,12.2,10.389454543));
#224964=CARTESIAN_POINT('Ctrl Pts',(0.145438019999944,12.2,10.38841812));
#224965=CARTESIAN_POINT('Ctrl Pts',(0.145319995999945,12.2,10.387390753));
#224966=CARTESIAN_POINT('Ctrl Pts',(0.145204040999944,12.2,10.386372471));
#224967=CARTESIAN_POINT('Ctrl Pts',(0.145090141999944,12.2,10.3853633));
#224968=CARTESIAN_POINT('Ctrl Pts',(0.144978279999943,12.2,10.384363269));
#224969=CARTESIAN_POINT('Ctrl Pts',(0.144868444999944,12.2,10.383372406));
#224970=CARTESIAN_POINT('Ctrl Pts',(0.144760618999945,12.2,10.382390738));
#224971=CARTESIAN_POINT('Ctrl Pts',(0.144654789999944,12.2,10.381418293));
#224972=CARTESIAN_POINT('Ctrl Pts',(0.144550940999943,12.2,10.3804551));
#224973=CARTESIAN_POINT('Ctrl Pts',(0.144449056999945,12.2,10.379501187));
#224974=CARTESIAN_POINT('Ctrl Pts',(0.144349124999945,12.2,10.378556581));
#224975=CARTESIAN_POINT('Ctrl Pts',(0.144251126999944,12.2,10.377621314));
#224976=CARTESIAN_POINT('Ctrl Pts',(0.144155048999943,12.2,10.376695411));
#224977=CARTESIAN_POINT('Ctrl Pts',(0.144061419999945,12.2,10.375784182));
#224978=CARTESIAN_POINT('Ctrl Pts',(0.143988113999944,12.2,10.375063685));
#224979=CARTESIAN_POINT('Ctrl Pts',(0.143934094999943,12.2,10.374528791));
#224980=CARTESIAN_POINT('Ctrl Pts',(0.143898617999945,12.2,10.374175763));
#224981=CARTESIAN_POINT('Ctrl Pts',(0.143881226999945,12.2,10.374002275));
#224982=CARTESIAN_POINT('Ctrl Pts',(0.143881226999945,15.2,10.374002275));
#224983=CARTESIAN_POINT('Ctrl Pts',(0.143898617999945,15.2,10.374175763));
#224984=CARTESIAN_POINT('Ctrl Pts',(0.143934094999943,15.2,10.374528791));
#224985=CARTESIAN_POINT('Ctrl Pts',(0.143988113999944,15.2,10.375063685));
#224986=CARTESIAN_POINT('Ctrl Pts',(0.144061419999945,15.2,10.375784182));
#224987=CARTESIAN_POINT('Ctrl Pts',(0.144155048999943,15.2,10.376695411));
#224988=CARTESIAN_POINT('Ctrl Pts',(0.144251126999944,15.2,10.377621314));
#224989=CARTESIAN_POINT('Ctrl Pts',(0.144349124999945,15.2,10.378556581));
#224990=CARTESIAN_POINT('Ctrl Pts',(0.144449056999945,15.2,10.379501187));
#224991=CARTESIAN_POINT('Ctrl Pts',(0.144550940999943,15.2,10.3804551));
#224992=CARTESIAN_POINT('Ctrl Pts',(0.144654789999944,15.2,10.381418293));
#224993=CARTESIAN_POINT('Ctrl Pts',(0.144760618999945,15.2,10.382390738));
#224994=CARTESIAN_POINT('Ctrl Pts',(0.144868444999944,15.2,10.383372406));
#224995=CARTESIAN_POINT('Ctrl Pts',(0.144978279999943,15.2,10.384363269));
#224996=CARTESIAN_POINT('Ctrl Pts',(0.145090141999944,15.2,10.3853633));
#224997=CARTESIAN_POINT('Ctrl Pts',(0.145204040999944,15.2,10.386372471));
#224998=CARTESIAN_POINT('Ctrl Pts',(0.145319995999945,15.2,10.387390753));
#224999=CARTESIAN_POINT('Ctrl Pts',(0.145438019999944,15.2,10.38841812));
#225000=CARTESIAN_POINT('Ctrl Pts',(0.145558125999944,15.2,10.389454543));
#225001=CARTESIAN_POINT('Ctrl Pts',(0.145680329999944,15.2,10.390499995));
#225002=CARTESIAN_POINT('Ctrl Pts',(0.145804644999944,15.2,10.391554451));
#225003=CARTESIAN_POINT('Ctrl Pts',(0.145931086999944,15.2,10.392617881));
#225004=CARTESIAN_POINT('Ctrl Pts',(0.146059667999945,15.2,10.39369026));
#225005=CARTESIAN_POINT('Ctrl Pts',(0.146190402999944,15.2,10.39477156));
#225006=CARTESIAN_POINT('Ctrl Pts',(0.146323305999945,15.2,10.395861757));
#225007=CARTESIAN_POINT('Ctrl Pts',(0.146458390999945,15.2,10.39696082));
#225008=CARTESIAN_POINT('Ctrl Pts',(0.146595670999944,15.2,10.398068726));
#225009=CARTESIAN_POINT('Ctrl Pts',(0.146735159999943,15.2,10.399185447));
#225010=CARTESIAN_POINT('Ctrl Pts',(0.146876870999944,15.2,10.400310958));
#225011=CARTESIAN_POINT('Ctrl Pts',(0.147020819999945,15.2,10.401445231));
#225012=CARTESIAN_POINT('Ctrl Pts',(0.147167015999944,15.2,10.402588242));
#225013=CARTESIAN_POINT('Ctrl Pts',(0.147315476999944,15.2,10.403739964));
#225014=CARTESIAN_POINT('Ctrl Pts',(0.147466212999945,15.2,10.404900372));
#225015=CARTESIAN_POINT('Ctrl Pts',(0.147619239999944,15.2,10.40606944));
#225016=CARTESIAN_POINT('Ctrl Pts',(0.147774568999944,15.2,10.407247143));
#225017=CARTESIAN_POINT('Ctrl Pts',(0.147932212999944,15.2,10.408433454));
#225018=CARTESIAN_POINT('Ctrl Pts',(0.148092186999945,15.2,10.409628349));
#225019=CARTESIAN_POINT('Ctrl Pts',(0.148254501999944,15.2,10.410831802));
#225020=CARTESIAN_POINT('Ctrl Pts',(0.148419171999944,15.2,10.412043789));
#225021=CARTESIAN_POINT('Ctrl Pts',(0.148586208999945,15.2,10.413264284));
#225022=CARTESIAN_POINT('Ctrl Pts',(0.148755626999945,15.2,10.414493263));
#225023=CARTESIAN_POINT('Ctrl Pts',(0.148927436999945,15.2,10.4157307));
#225024=CARTESIAN_POINT('Ctrl Pts',(0.149101651999944,15.2,10.416976571));
#225025=CARTESIAN_POINT('Ctrl Pts',(0.149278284999944,15.2,10.418230853));
#225026=CARTESIAN_POINT('Ctrl Pts',(0.149457348999944,15.2,10.419493518));
#225027=CARTESIAN_POINT('Ctrl Pts',(0.149638854999944,15.2,10.420764544));
#225028=CARTESIAN_POINT('Ctrl Pts',(0.149822815999944,15.2,10.422043908));
#225029=CARTESIAN_POINT('Ctrl Pts',(0.150009245999945,15.2,10.423331583));
#225030=CARTESIAN_POINT('Ctrl Pts',(0.150198153999943,15.2,10.424627546));
#225031=CARTESIAN_POINT('Ctrl Pts',(0.150389552999943,15.2,10.425931773));
#225032=CARTESIAN_POINT('Ctrl Pts',(0.150583456999945,15.2,10.427244241));
#225033=CARTESIAN_POINT('Ctrl Pts',(0.150779875999945,15.2,10.428564925));
#225034=CARTESIAN_POINT('Ctrl Pts',(0.150978822999944,15.2,10.429893802));
#225035=CARTESIAN_POINT('Ctrl Pts',(0.151180308999944,15.2,10.431230849));
#225036=CARTESIAN_POINT('Ctrl Pts',(0.151384345999944,15.2,10.432576041));
#225037=CARTESIAN_POINT('Ctrl Pts',(0.151590946999944,15.2,10.433929355));
#225038=CARTESIAN_POINT('Ctrl Pts',(0.151800121999944,15.2,10.435290769));
#225039=CARTESIAN_POINT('Ctrl Pts',(0.152011882999944,15.2,10.436660258));
#225040=CARTESIAN_POINT('Ctrl Pts',(0.152226241999944,15.2,10.4380378));
#225041=CARTESIAN_POINT('Ctrl Pts',(0.152443210999945,15.2,10.439423373));
#225042=CARTESIAN_POINT('Ctrl Pts',(0.152662799999945,15.2,10.440816951));
#225043=CARTESIAN_POINT('Ctrl Pts',(0.152885021999944,15.2,10.442218514));
#225044=CARTESIAN_POINT('Ctrl Pts',(0.153109886999945,15.2,10.443628039));
#225045=CARTESIAN_POINT('Ctrl Pts',(0.153337406999944,15.2,10.445045501));
#225046=CARTESIAN_POINT('Ctrl Pts',(0.153567591999944,15.2,10.44647088));
#225047=CARTESIAN_POINT('Ctrl Pts',(0.153800454999944,15.2,10.447904152));
#225048=CARTESIAN_POINT('Ctrl Pts',(0.154036005999943,15.2,10.449345296));
#225049=CARTESIAN_POINT('Ctrl Pts',(0.154274255999944,15.2,10.450794288));
#225050=CARTESIAN_POINT('Ctrl Pts',(0.154515215999943,15.2,10.452251107));
#225051=CARTESIAN_POINT('Ctrl Pts',(0.154758896999944,15.2,10.45371573));
#225052=CARTESIAN_POINT('Ctrl Pts',(0.155005309999944,15.2,10.455188137));
#225053=CARTESIAN_POINT('Ctrl Pts',(0.155254464999944,15.2,10.456668303));
#225054=CARTESIAN_POINT('Ctrl Pts',(0.155506374999945,15.2,10.458156207));
#225055=CARTESIAN_POINT('Ctrl Pts',(0.155761047999944,15.2,10.459651829));
#225056=CARTESIAN_POINT('Ctrl Pts',(0.156018494999944,15.2,10.461155145));
#225057=CARTESIAN_POINT('Ctrl Pts',(0.156278728999943,15.2,10.462666136));
#225058=CARTESIAN_POINT('Ctrl Pts',(0.156541757999945,15.2,10.464184777));
#225059=CARTESIAN_POINT('Ctrl Pts',(0.156807592999944,15.2,10.46571105));
#225060=CARTESIAN_POINT('Ctrl Pts',(0.157076244999944,15.2,10.467244932));
#225061=CARTESIAN_POINT('Ctrl Pts',(0.157347723999944,15.2,10.4687864));
#225062=CARTESIAN_POINT('Ctrl Pts',(0.157622040999945,15.2,10.470335436));
#225063=CARTESIAN_POINT('Ctrl Pts',(0.157899203999945,15.2,10.471892016));
#225064=CARTESIAN_POINT('Ctrl Pts',(0.158179225999945,15.2,10.473456121));
#225065=CARTESIAN_POINT('Ctrl Pts',(0.158462115999944,15.2,10.475027729));
#225066=CARTESIAN_POINT('Ctrl Pts',(0.158747883999943,15.2,10.476606819));
#225067=CARTESIAN_POINT('Ctrl Pts',(0.159036538999944,15.2,10.478193371));
#225068=CARTESIAN_POINT('Ctrl Pts',(0.159328093999944,15.2,10.479787363));
#225069=CARTESIAN_POINT('Ctrl Pts',(0.159622555999944,15.2,10.481388775));
#225070=CARTESIAN_POINT('Ctrl Pts',(0.159919935999945,15.2,10.482997587));
#225071=CARTESIAN_POINT('Ctrl Pts',(0.160220243999945,15.2,10.484613776));
#225072=CARTESIAN_POINT('Ctrl Pts',(0.160523488999944,15.2,10.486237324));
#225073=CARTESIAN_POINT('Ctrl Pts',(0.160829681999944,15.2,10.487868211));
#225074=CARTESIAN_POINT('Ctrl Pts',(0.161138831999944,15.2,10.489506414));
#225075=CARTESIAN_POINT('Ctrl Pts',(0.161450947999944,15.2,10.491151915));
#225076=CARTESIAN_POINT('Ctrl Pts',(0.161766040999943,15.2,10.492804693));
#225077=CARTESIAN_POINT('Ctrl Pts',(0.162084119999945,15.2,10.494464727));
#225078=CARTESIAN_POINT('Ctrl Pts',(0.162405193999945,15.2,10.496131999));
#225079=CARTESIAN_POINT('Ctrl Pts',(0.162729271999943,15.2,10.497806487));
#225080=CARTESIAN_POINT('Ctrl Pts',(0.163056365999944,15.2,10.499488173));
#225081=CARTESIAN_POINT('Ctrl Pts',(0.163386482999943,15.2,10.501177035));
#225082=CARTESIAN_POINT('Ctrl Pts',(0.163719631999945,15.2,10.502873055));
#225083=CARTESIAN_POINT('Ctrl Pts',(0.164055823999943,15.2,10.504576213));
#225084=CARTESIAN_POINT('Ctrl Pts',(0.164395066999944,15.2,10.506286488));
#225085=CARTESIAN_POINT('Ctrl Pts',(0.164737370999944,15.2,10.508003861));
#225086=CARTESIAN_POINT('Ctrl Pts',(0.165082743999945,15.2,10.509728314));
#225087=CARTESIAN_POINT('Ctrl Pts',(0.165431195999943,15.2,10.511459827));
#225088=CARTESIAN_POINT('Ctrl Pts',(0.165782736999944,15.2,10.513198379));
#225089=CARTESIAN_POINT('Ctrl Pts',(0.166137373999945,15.2,10.514943952));
#225090=CARTESIAN_POINT('Ctrl Pts',(0.166495116999944,15.2,10.516696527));
#225091=CARTESIAN_POINT('Ctrl Pts',(0.166855973999944,15.2,10.518456083));
#225092=CARTESIAN_POINT('Ctrl Pts',(0.167219954999943,15.2,10.520222605));
#225093=CARTESIAN_POINT('Ctrl Pts',(0.167587068999945,15.2,10.521996069));
#225094=CARTESIAN_POINT('Ctrl Pts',(0.167957322999944,15.2,10.523776458));
#225095=CARTESIAN_POINT('Ctrl Pts',(0.168330727999945,15.2,10.525563754));
#225096=CARTESIAN_POINT('Ctrl Pts',(0.168707291999944,15.2,10.527357938));
#225097=CARTESIAN_POINT('Ctrl Pts',(0.169087021999944,15.2,10.52915899));
#225098=CARTESIAN_POINT('Ctrl Pts',(0.169469929999944,15.2,10.530966892));
#225099=CARTESIAN_POINT('Ctrl Pts',(0.169856019999944,15.2,10.532781625));
#225100=CARTESIAN_POINT('Ctrl Pts',(0.170245304999943,15.2,10.534603171));
#225101=CARTESIAN_POINT('Ctrl Pts',(0.170637789999945,15.2,10.536431512));
#225102=CARTESIAN_POINT('Ctrl Pts',(0.171033485999944,15.2,10.538266627));
#225103=CARTESIAN_POINT('Ctrl Pts',(0.171432399999943,15.2,10.5401085));
#225104=CARTESIAN_POINT('Ctrl Pts',(0.171834540999944,15.2,10.541957111));
#225105=CARTESIAN_POINT('Ctrl Pts',(0.172239915999944,15.2,10.543812444));
#225106=CARTESIAN_POINT('Ctrl Pts',(0.172648535999944,15.2,10.545674477));
#225107=CARTESIAN_POINT('Ctrl Pts',(0.173060405999944,15.2,10.547543196));
#225108=CARTESIAN_POINT('Ctrl Pts',(0.173475535999945,15.2,10.549418579));
#225109=CARTESIAN_POINT('Ctrl Pts',(0.173893933999943,15.2,10.551300611));
#225110=CARTESIAN_POINT('Ctrl Pts',(0.174315608999944,15.2,10.553189272));
#225111=CARTESIAN_POINT('Ctrl Pts',(0.174740566999944,15.2,10.555084546));
#225112=CARTESIAN_POINT('Ctrl Pts',(0.175168817999944,15.2,10.556986414));
#225113=CARTESIAN_POINT('Ctrl Pts',(0.175600368999945,15.2,10.558894856));
#225114=CARTESIAN_POINT('Ctrl Pts',(0.176035227999943,15.2,10.560809858));
#225115=CARTESIAN_POINT('Ctrl Pts',(0.176473402999945,15.2,10.5627314));
#225116=CARTESIAN_POINT('Ctrl Pts',(0.176914901999944,15.2,10.564659464));
#225117=CARTESIAN_POINT('Ctrl Pts',(0.177359733999944,15.2,10.566594034));
#225118=CARTESIAN_POINT('Ctrl Pts',(0.177807903999945,15.2,10.568535092));
#225119=CARTESIAN_POINT('Ctrl Pts',(0.178259421999943,15.2,10.570482619));
#225120=CARTESIAN_POINT('Ctrl Pts',(0.178714295999944,15.2,10.5724366));
#225121=CARTESIAN_POINT('Ctrl Pts',(0.179172531999944,15.2,10.574397014));
#225122=CARTESIAN_POINT('Ctrl Pts',(0.179634138999945,15.2,10.576363848));
#225123=CARTESIAN_POINT('Ctrl Pts',(0.180099123999945,15.2,10.578337082));
#225124=CARTESIAN_POINT('Ctrl Pts',(0.180567494999944,15.2,10.580316698));
#225125=CARTESIAN_POINT('Ctrl Pts',(0.181039259999943,15.2,10.582302681));
#225126=CARTESIAN_POINT('Ctrl Pts',(0.181514424999945,15.2,10.584295013));
#225127=CARTESIAN_POINT('Ctrl Pts',(0.181992997999944,15.2,10.586293676));
#225128=CARTESIAN_POINT('Ctrl Pts',(0.182474987999944,15.2,10.588298654));
#225129=CARTESIAN_POINT('Ctrl Pts',(0.182960400999944,15.2,10.59030993));
#225130=CARTESIAN_POINT('Ctrl Pts',(0.183449243999944,15.2,10.592327487));
#225131=CARTESIAN_POINT('Ctrl Pts',(0.183941525999943,15.2,10.594351307));
#225132=CARTESIAN_POINT('Ctrl Pts',(0.184437252999944,15.2,10.596381375));
#225133=CARTESIAN_POINT('Ctrl Pts',(0.184936431999944,15.2,10.598417673));
#225134=CARTESIAN_POINT('Ctrl Pts',(0.185439070999944,15.2,10.600460184));
#225135=CARTESIAN_POINT('Ctrl Pts',(0.185945176999944,15.2,10.602508892));
#225136=CARTESIAN_POINT('Ctrl Pts',(0.186454757999943,15.2,10.604563781));
#225137=CARTESIAN_POINT('Ctrl Pts',(0.186967819999945,15.2,10.606624832));
#225138=CARTESIAN_POINT('Ctrl Pts',(0.187484369999943,15.2,10.608692031));
#225139=CARTESIAN_POINT('Ctrl Pts',(0.188004415999944,15.2,10.61076536));
#225140=CARTESIAN_POINT('Ctrl Pts',(0.188527964999944,15.2,10.612844803));
#225141=CARTESIAN_POINT('Ctrl Pts',(0.189055023999943,15.2,10.614930343));
#225142=CARTESIAN_POINT('Ctrl Pts',(0.189585597999944,15.2,10.617021966));
#225143=CARTESIAN_POINT('Ctrl Pts',(0.190119695999943,15.2,10.619119652));
#225144=CARTESIAN_POINT('Ctrl Pts',(0.190657324999943,15.2,10.621223388));
#225145=CARTESIAN_POINT('Ctrl Pts',(0.191198490999945,15.2,10.623333156));
#225146=CARTESIAN_POINT('Ctrl Pts',(0.191743202999944,15.2,10.62544894));
#225147=CARTESIAN_POINT('Ctrl Pts',(0.192291463999944,15.2,10.627570724));
#225148=CARTESIAN_POINT('Ctrl Pts',(0.192843282999944,15.2,10.629698493));
#225149=CARTESIAN_POINT('Ctrl Pts',(0.193398666999943,15.2,10.631832228));
#225150=CARTESIAN_POINT('Ctrl Pts',(0.193957621999944,15.2,10.633971917));
#225151=CARTESIAN_POINT('Ctrl Pts',(0.194520154999944,15.2,10.636117541));
#225152=CARTESIAN_POINT('Ctrl Pts',(0.195086272999945,15.2,10.638269086));
#225153=CARTESIAN_POINT('Ctrl Pts',(0.195655981999945,15.2,10.640426535));
#225154=CARTESIAN_POINT('Ctrl Pts',(0.196229288999945,15.2,10.642589871));
#225155=CARTESIAN_POINT('Ctrl Pts',(0.196806200999945,15.2,10.644759081));
#225156=CARTESIAN_POINT('Ctrl Pts',(0.197386722999945,15.2,10.646934148));
#225157=CARTESIAN_POINT('Ctrl Pts',(0.197970861999943,15.2,10.649115056));
#225158=CARTESIAN_POINT('Ctrl Pts',(0.198558625999944,15.2,10.651301789));
#225159=CARTESIAN_POINT('Ctrl Pts',(0.199150019999944,15.2,10.653494334));
#225160=CARTESIAN_POINT('Ctrl Pts',(0.199745050999944,15.2,10.655692671));
#225161=CARTESIAN_POINT('Ctrl Pts',(0.200343724999945,15.2,10.657896788));
#225162=CARTESIAN_POINT('Ctrl Pts',(0.200946048999944,15.2,10.660106669));
#225163=CARTESIAN_POINT('Ctrl Pts',(0.201552027999944,15.2,10.662322298));
#225164=CARTESIAN_POINT('Ctrl Pts',(0.202161669999944,15.2,10.664543659));
#225165=CARTESIAN_POINT('Ctrl Pts',(0.202774978999944,15.2,10.666770738));
#225166=CARTESIAN_POINT('Ctrl Pts',(0.203391963999945,15.2,10.669003518));
#225167=CARTESIAN_POINT('Ctrl Pts',(0.204012629999945,15.2,10.671241985));
#225168=CARTESIAN_POINT('Ctrl Pts',(0.204636982999944,15.2,10.673486125));
#225169=CARTESIAN_POINT('Ctrl Pts',(0.205265027999945,15.2,10.67573592));
#225170=CARTESIAN_POINT('Ctrl Pts',(0.205896773999944,15.2,10.677991356));
#225171=CARTESIAN_POINT('Ctrl Pts',(0.206532223999943,15.2,10.680252419));
#225172=CARTESIAN_POINT('Ctrl Pts',(0.207171385999944,15.2,10.682519093));
#225173=CARTESIAN_POINT('Ctrl Pts',(0.207814266999945,15.2,10.684791362));
#225174=CARTESIAN_POINT('Ctrl Pts',(0.208460869999945,15.2,10.687069213));
#225175=CARTESIAN_POINT('Ctrl Pts',(0.209111202999944,15.2,10.68935263));
#225176=CARTESIAN_POINT('Ctrl Pts',(0.209765270999943,15.2,10.691641598));
#225177=CARTESIAN_POINT('Ctrl Pts',(0.210423080999943,15.2,10.693936102));
#225178=CARTESIAN_POINT('Ctrl Pts',(0.211084637999944,15.2,10.696236128));
#225179=CARTESIAN_POINT('Ctrl Pts',(0.211749947999945,15.2,10.69854166));
#225180=CARTESIAN_POINT('Ctrl Pts',(0.212419017999944,15.2,10.700852684));
#225181=CARTESIAN_POINT('Ctrl Pts',(0.213091851999945,15.2,10.703169186));
#225182=CARTESIAN_POINT('Ctrl Pts',(0.213768457999944,15.2,10.70549115));
#225183=CARTESIAN_POINT('Ctrl Pts',(0.214448838999944,15.2,10.707818563));
#225184=CARTESIAN_POINT('Ctrl Pts',(0.215133002999943,15.2,10.710151408));
#225185=CARTESIAN_POINT('Ctrl Pts',(0.215820953999944,15.2,10.712489672));
#225186=CARTESIAN_POINT('Ctrl Pts',(0.216512699999944,15.2,10.71483334));
#225187=CARTESIAN_POINT('Ctrl Pts',(0.217208243999943,15.2,10.717182399));
#225188=CARTESIAN_POINT('Ctrl Pts',(0.217907592999945,15.2,10.719536832));
#225189=CARTESIAN_POINT('Ctrl Pts',(0.218610752999944,15.2,10.721896627));
#225190=CARTESIAN_POINT('Ctrl Pts',(0.219317728999944,15.2,10.724261769));
#225191=CARTESIAN_POINT('Ctrl Pts',(0.220028526999944,15.2,10.726632242));
#225192=CARTESIAN_POINT('Ctrl Pts',(0.220743151999944,15.2,10.729008033));
#225193=CARTESIAN_POINT('Ctrl Pts',(0.221461608999943,15.2,10.731389127));
#225194=CARTESIAN_POINT('Ctrl Pts',(0.222183904999945,15.2,10.733775512));
#225195=CARTESIAN_POINT('Ctrl Pts',(0.222910043999944,15.2,10.736167171));
#225196=CARTESIAN_POINT('Ctrl Pts',(0.223640032999944,15.2,10.738564091));
#225197=CARTESIAN_POINT('Ctrl Pts',(0.224373874999945,15.2,10.740966259));
#225198=CARTESIAN_POINT('Ctrl Pts',(0.225111577999944,15.2,10.743373659));
#225199=CARTESIAN_POINT('Ctrl Pts',(0.225853144999943,15.2,10.745786278));
#225200=CARTESIAN_POINT('Ctrl Pts',(0.226598583999945,15.2,10.748204101));
#225201=CARTESIAN_POINT('Ctrl Pts',(0.227347897999944,15.2,10.750627115));
#225202=CARTESIAN_POINT('Ctrl Pts',(0.228101093999945,15.2,10.753055306));
#225203=CARTESIAN_POINT('Ctrl Pts',(0.228858174999944,15.2,10.755488661));
#225204=CARTESIAN_POINT('Ctrl Pts',(0.229619148999944,15.2,10.757927164));
#225205=CARTESIAN_POINT('Ctrl Pts',(0.230384019999944,15.2,10.760370801));
#225206=CARTESIAN_POINT('Ctrl Pts',(0.231152791999945,15.2,10.762819561));
#225207=CARTESIAN_POINT('Ctrl Pts',(0.231925471999944,15.2,10.765273427));
#225208=CARTESIAN_POINT('Ctrl Pts',(0.232702063999944,15.2,10.767732388));
#225209=CARTESIAN_POINT('Ctrl Pts',(0.233482572999945,15.2,10.770196429));
#225210=CARTESIAN_POINT('Ctrl Pts',(0.234267004999945,15.2,10.772665536));
#225211=CARTESIAN_POINT('Ctrl Pts',(0.235055364999944,15.2,10.775139696));
#225212=CARTESIAN_POINT('Ctrl Pts',(0.235847656999945,15.2,10.777618895));
#225213=CARTESIAN_POINT('Ctrl Pts',(0.236643886999944,15.2,10.780103119));
#225214=CARTESIAN_POINT('Ctrl Pts',(0.237444059999945,15.2,10.782592356));
#225215=CARTESIAN_POINT('Ctrl Pts',(0.238248179999945,15.2,10.78508659));
#225216=CARTESIAN_POINT('Ctrl Pts',(0.239056252999944,15.2,10.78758581));
#225217=CARTESIAN_POINT('Ctrl Pts',(0.239868283999943,15.2,10.790090001));
#225218=CARTESIAN_POINT('Ctrl Pts',(0.240684276999945,15.2,10.79259915));
#225219=CARTESIAN_POINT('Ctrl Pts',(0.241504236999944,15.2,10.795113244));
#225220=CARTESIAN_POINT('Ctrl Pts',(0.242328170999944,15.2,10.797632269));
#225221=CARTESIAN_POINT('Ctrl Pts',(0.243156079999943,15.2,10.800156212));
#225222=CARTESIAN_POINT('Ctrl Pts',(0.243987971999945,15.2,10.80268506));
#225223=CARTESIAN_POINT('Ctrl Pts',(0.244823849999944,15.2,10.805218799));
#225224=CARTESIAN_POINT('Ctrl Pts',(0.245663720999945,15.2,10.807757416));
#225225=CARTESIAN_POINT('Ctrl Pts',(0.246507586999943,15.2,10.810300898));
#225226=CARTESIAN_POINT('Ctrl Pts',(0.247355453999945,15.2,10.812849232));
#225227=CARTESIAN_POINT('Ctrl Pts',(0.248207326999944,15.2,10.815402405));
#225228=CARTESIAN_POINT('Ctrl Pts',(0.249063209999945,15.2,10.817960403));
#225229=CARTESIAN_POINT('Ctrl Pts',(0.249923107999944,15.2,10.820523213));
#225230=CARTESIAN_POINT('Ctrl Pts',(0.250787026999945,15.2,10.823090823));
#225231=CARTESIAN_POINT('Ctrl Pts',(0.251654968999944,15.2,10.825663219));
#225232=CARTESIAN_POINT('Ctrl Pts',(0.252526938999944,15.2,10.828240388));
#225233=CARTESIAN_POINT('Ctrl Pts',(0.253402944999944,15.2,10.830822318));
#225234=CARTESIAN_POINT('Ctrl Pts',(0.254282986999945,15.2,10.833408995));
#225235=CARTESIAN_POINT('Ctrl Pts',(0.255167071999944,15.2,10.836000406));
#225236=CARTESIAN_POINT('Ctrl Pts',(0.256055205999944,15.2,10.838596539));
#225237=CARTESIAN_POINT('Ctrl Pts',(0.256947389999944,15.2,10.841197381));
#225238=CARTESIAN_POINT('Ctrl Pts',(0.257843629999943,15.2,10.843802919));
#225239=CARTESIAN_POINT('Ctrl Pts',(0.258743930999945,15.2,10.846413139));
#225240=CARTESIAN_POINT('Ctrl Pts',(0.259648296999944,15.2,10.84902803));
#225241=CARTESIAN_POINT('Ctrl Pts',(0.260556730999945,15.2,10.851647579));
#225242=CARTESIAN_POINT('Ctrl Pts',(0.261469239999944,15.2,10.854271772));
#225243=CARTESIAN_POINT('Ctrl Pts',(0.262385827999945,15.2,10.856900597));
#225244=CARTESIAN_POINT('Ctrl Pts',(0.263306497999943,15.2,10.859534043));
#225245=CARTESIAN_POINT('Ctrl Pts',(0.264231254999944,15.2,10.862172095));
#225246=CARTESIAN_POINT('Ctrl Pts',(0.265160102999945,15.2,10.864814741));
#225247=CARTESIAN_POINT('Ctrl Pts',(0.266093045999943,15.2,10.867461969));
#225248=CARTESIAN_POINT('Ctrl Pts',(0.267030088999943,15.2,10.870113767));
#225249=CARTESIAN_POINT('Ctrl Pts',(0.267971236999944,15.2,10.872770121));
#225250=CARTESIAN_POINT('Ctrl Pts',(0.268916491999944,15.2,10.875431019));
#225251=CARTESIAN_POINT('Ctrl Pts',(0.269865859999945,15.2,10.878096449));
#225252=CARTESIAN_POINT('Ctrl Pts',(0.270819344999945,15.2,10.880766399));
#225253=CARTESIAN_POINT('Ctrl Pts',(0.271776950999945,15.2,10.883440855));
#225254=CARTESIAN_POINT('Ctrl Pts',(0.272738680999945,15.2,10.886119805));
#225255=CARTESIAN_POINT('Ctrl Pts',(0.273704539999944,15.2,10.888803238));
#225256=CARTESIAN_POINT('Ctrl Pts',(0.274674533999945,15.2,10.89149114));
#225257=CARTESIAN_POINT('Ctrl Pts',(0.275648663999943,15.2,10.894183501));
#225258=CARTESIAN_POINT('Ctrl Pts',(0.276626936999945,15.2,10.896880306));
#225259=CARTESIAN_POINT('Ctrl Pts',(0.277609353999945,15.2,10.899581544));
#225260=CARTESIAN_POINT('Ctrl Pts',(0.278595920999944,15.2,10.902287203));
#225261=CARTESIAN_POINT('Ctrl Pts',(0.279586641999944,15.2,10.904997271));
#225262=CARTESIAN_POINT('Ctrl Pts',(0.280581519999944,15.2,10.907711735));
#225263=CARTESIAN_POINT('Ctrl Pts',(0.281580559999943,15.2,10.910430582));
#225264=CARTESIAN_POINT('Ctrl Pts',(0.282583764999943,15.2,10.913153803));
#225265=CARTESIAN_POINT('Ctrl Pts',(0.283591139999944,15.2,10.915881383));
#225266=CARTESIAN_POINT('Ctrl Pts',(0.284602689999945,15.2,10.918613312));
#225267=CARTESIAN_POINT('Ctrl Pts',(0.285618414999943,15.2,10.921349576));
#225268=CARTESIAN_POINT('Ctrl Pts',(0.286638321999944,15.2,10.924090164));
#225269=CARTESIAN_POINT('Ctrl Pts',(0.287662414999945,15.2,10.926835064));
#225270=CARTESIAN_POINT('Ctrl Pts',(0.288690695999945,15.2,10.929584263));
#225271=CARTESIAN_POINT('Ctrl Pts',(0.289723169999944,15.2,10.932337751));
#225272=CARTESIAN_POINT('Ctrl Pts',(0.290759841999944,15.2,10.935095515));
#225273=CARTESIAN_POINT('Ctrl Pts',(0.291800711999944,15.2,10.937857544));
#225274=CARTESIAN_POINT('Ctrl Pts',(0.292845787999945,15.2,10.940623824));
#225275=CARTESIAN_POINT('Ctrl Pts',(0.293895072999945,15.2,10.943394344));
#225276=CARTESIAN_POINT('Ctrl Pts',(0.294948567999944,15.2,10.946169093));
#225277=CARTESIAN_POINT('Ctrl Pts',(0.296006278999944,15.2,10.94894806));
#225278=CARTESIAN_POINT('Ctrl Pts',(0.297068208999944,15.2,10.951731231));
#225279=CARTESIAN_POINT('Ctrl Pts',(0.298134362999944,15.2,10.954518595));
#225280=CARTESIAN_POINT('Ctrl Pts',(0.299204742999944,15.2,10.957310141));
#225281=CARTESIAN_POINT('Ctrl Pts',(0.300279352999944,15.2,10.960105857));
#225282=CARTESIAN_POINT('Ctrl Pts',(0.301358196999945,15.2,10.962905732));
#225283=CARTESIAN_POINT('Ctrl Pts',(0.302441278999943,15.2,10.965709751));
#225284=CARTESIAN_POINT('Ctrl Pts',(0.303528602999944,15.2,10.968517908));
#225285=CARTESIAN_POINT('Ctrl Pts',(0.304620169999945,15.2,10.971330186));
#225286=CARTESIAN_POINT('Ctrl Pts',(0.305715986999945,15.2,10.974146576));
#225287=CARTESIAN_POINT('Ctrl Pts',(0.306816055999944,15.2,10.976967067));
#225288=CARTESIAN_POINT('Ctrl Pts',(0.307920378999944,15.2,10.979791646));
#225289=CARTESIAN_POINT('Ctrl Pts',(0.309028961999944,15.2,10.982620303));
#225290=CARTESIAN_POINT('Ctrl Pts',(0.310141807999944,15.2,10.985453024));
#225291=CARTESIAN_POINT('Ctrl Pts',(0.311258918999944,15.2,10.988289801));
#225292=CARTESIAN_POINT('Ctrl Pts',(0.312380299999945,15.2,10.991130619));
#225293=CARTESIAN_POINT('Ctrl Pts',(0.313505953999943,15.2,10.993975469));
#225294=CARTESIAN_POINT('Ctrl Pts',(0.314635883999944,15.2,10.996824338));
#225295=CARTESIAN_POINT('Ctrl Pts',(0.315770094999944,15.2,10.999677217));
#225296=CARTESIAN_POINT('Ctrl Pts',(0.316908587999943,15.2,11.002534092));
#225297=CARTESIAN_POINT('Ctrl Pts',(0.318051368999944,15.2,11.005394953));
#225298=CARTESIAN_POINT('Ctrl Pts',(0.319198438999945,15.2,11.008259789));
#225299=CARTESIAN_POINT('Ctrl Pts',(0.320349802999944,15.2,11.011128587));
#225300=CARTESIAN_POINT('Ctrl Pts',(0.321505462999945,15.2,11.014001339));
#225301=CARTESIAN_POINT('Ctrl Pts',(0.322665423999944,15.2,11.016878029));
#225302=CARTESIAN_POINT('Ctrl Pts',(0.323829688999944,15.2,11.01975865));
#225303=CARTESIAN_POINT('Ctrl Pts',(0.324998259999945,15.2,11.02264319));
#225304=CARTESIAN_POINT('Ctrl Pts',(0.326171140999945,15.2,11.025531635));
#225305=CARTESIAN_POINT('Ctrl Pts',(0.327348334999943,15.2,11.028423977));
#225306=CARTESIAN_POINT('Ctrl Pts',(0.328529845999944,15.2,11.031320203));
#225307=CARTESIAN_POINT('Ctrl Pts',(0.329715676999944,15.2,11.034220304));
#225308=CARTESIAN_POINT('Ctrl Pts',(0.330905830999945,15.2,11.037124267));
#225309=CARTESIAN_POINT('Ctrl Pts',(0.332100310999944,15.2,11.040032081));
#225310=CARTESIAN_POINT('Ctrl Pts',(0.333299119999945,15.2,11.042943736));
#225311=CARTESIAN_POINT('Ctrl Pts',(0.334502261999944,15.2,11.04585922));
#225312=CARTESIAN_POINT('Ctrl Pts',(0.335709739999944,15.2,11.048778522));
#225313=CARTESIAN_POINT('Ctrl Pts',(0.336921556999944,15.2,11.051701632));
#225314=CARTESIAN_POINT('Ctrl Pts',(0.338137715999943,15.2,11.054628538));
#225315=CARTESIAN_POINT('Ctrl Pts',(0.339358218999944,15.2,11.057559229));
#225316=CARTESIAN_POINT('Ctrl Pts',(0.340583071999945,15.2,11.060493695));
#225317=CARTESIAN_POINT('Ctrl Pts',(0.341812274999944,15.2,11.063431924));
#225318=CARTESIAN_POINT('Ctrl Pts',(0.343045832999945,15.2,11.066373907));
#225319=CARTESIAN_POINT('Ctrl Pts',(0.344283748999944,15.2,11.069319631));
#225320=CARTESIAN_POINT('Ctrl Pts',(0.345526024999945,15.2,11.072269087));
#225321=CARTESIAN_POINT('Ctrl Pts',(0.346772663999945,15.2,11.075222263));
#225322=CARTESIAN_POINT('Ctrl Pts',(0.348023670999943,15.2,11.078179147));
#225323=CARTESIAN_POINT('Ctrl Pts',(0.349279045999945,15.2,11.081139731));
#225324=CARTESIAN_POINT('Ctrl Pts',(0.350538794999944,15.2,11.084104002));
#225325=CARTESIAN_POINT('Ctrl Pts',(0.351802917999944,15.2,11.087071951));
#225326=CARTESIAN_POINT('Ctrl Pts',(0.353071419999944,15.2,11.090043565));
#225327=CARTESIAN_POINT('Ctrl Pts',(0.354344304999945,15.2,11.093018835));
#225328=CARTESIAN_POINT('Ctrl Pts',(0.355621571999943,15.2,11.095997751));
#225329=CARTESIAN_POINT('Ctrl Pts',(0.356903226999944,15.2,11.0989803));
#225330=CARTESIAN_POINT('Ctrl Pts',(0.358189272999944,15.2,11.101966473));
#225331=CARTESIAN_POINT('Ctrl Pts',(0.359479711999944,15.2,11.104956259));
#225332=CARTESIAN_POINT('Ctrl Pts',(0.360774545999943,15.2,11.107949648));
#225333=CARTESIAN_POINT('Ctrl Pts',(0.362073778999944,15.2,11.110946629));
#225334=CARTESIAN_POINT('Ctrl Pts',(0.363377412999943,15.2,11.11394719));
#225335=CARTESIAN_POINT('Ctrl Pts',(0.364685451999945,15.2,11.116951322));
#225336=CARTESIAN_POINT('Ctrl Pts',(0.365997898999944,15.2,11.119959015));
#225337=CARTESIAN_POINT('Ctrl Pts',(0.367314755999945,15.2,11.122970257));
#225338=CARTESIAN_POINT('Ctrl Pts',(0.368636023999944,15.2,11.125985039));
#225339=CARTESIAN_POINT('Ctrl Pts',(0.369961708999943,15.2,11.129003348));
#225340=CARTESIAN_POINT('Ctrl Pts',(0.371291811999944,15.2,11.132025177));
#225341=CARTESIAN_POINT('Ctrl Pts',(0.372626335999945,15.2,11.135050513));
#225342=CARTESIAN_POINT('Ctrl Pts',(0.373965283999944,15.2,11.138079346));
#225343=CARTESIAN_POINT('Ctrl Pts',(0.375308657999945,15.2,11.141111667));
#225344=CARTESIAN_POINT('Ctrl Pts',(0.376656460999945,15.2,11.144147463));
#225345=CARTESIAN_POINT('Ctrl Pts',(0.378008696999944,15.2,11.147186727));
#225346=CARTESIAN_POINT('Ctrl Pts',(0.379365366999943,15.2,11.150229446));
#225347=CARTESIAN_POINT('Ctrl Pts',(0.380726473999945,15.2,11.15327561));
#225348=CARTESIAN_POINT('Ctrl Pts',(0.382092020999943,15.2,11.15632521));
#225349=CARTESIAN_POINT('Ctrl Pts',(0.383462009999944,15.2,11.159378235));
#225350=CARTESIAN_POINT('Ctrl Pts',(0.384836444999944,15.2,11.162434674));
#225351=CARTESIAN_POINT('Ctrl Pts',(0.386215327999944,15.2,11.165494518));
#225352=CARTESIAN_POINT('Ctrl Pts',(0.387598660999944,15.2,11.168557757));
#225353=CARTESIAN_POINT('Ctrl Pts',(0.388986445999944,15.2,11.171624378));
#225354=CARTESIAN_POINT('Ctrl Pts',(0.390378687999944,15.2,11.174694374));
#225355=CARTESIAN_POINT('Ctrl Pts',(0.391775385999944,15.2,11.177767734));
#225356=CARTESIAN_POINT('Ctrl Pts',(0.393176546999945,15.2,11.180844446));
#225357=CARTESIAN_POINT('Ctrl Pts',(0.394582168999945,15.2,11.183924503));
#225358=CARTESIAN_POINT('Ctrl Pts',(0.395992257999945,15.2,11.187007891));
#225359=CARTESIAN_POINT('Ctrl Pts',(0.397406813999943,15.2,11.190094604));
#225360=CARTESIAN_POINT('Ctrl Pts',(0.398825840999945,15.2,11.193184629));
#225361=CARTESIAN_POINT('Ctrl Pts',(0.400249340999944,15.2,11.196277957));
#225362=CARTESIAN_POINT('Ctrl Pts',(0.401677316999944,15.2,11.199374578));
#225363=CARTESIAN_POINT('Ctrl Pts',(0.403109770999944,15.2,11.202474482));
#225364=CARTESIAN_POINT('Ctrl Pts',(0.404546704999945,15.2,11.205577658));
#225365=CARTESIAN_POINT('Ctrl Pts',(0.405988121999944,15.2,11.208684097));
#225366=CARTESIAN_POINT('Ctrl Pts',(0.407434024999944,15.2,11.211793789));
#225367=CARTESIAN_POINT('Ctrl Pts',(0.408884414999945,15.2,11.214906723));
#225368=CARTESIAN_POINT('Ctrl Pts',(0.410339294999943,15.2,11.21802289));
#225369=CARTESIAN_POINT('Ctrl Pts',(0.411798665999944,15.2,11.22114228));
#225370=CARTESIAN_POINT('Ctrl Pts',(0.413262533999944,15.2,11.224264884));
#225371=CARTESIAN_POINT('Ctrl Pts',(0.414730897999943,15.2,11.227390689));
#225372=CARTESIAN_POINT('Ctrl Pts',(0.416203760999944,15.2,11.230519689));
#225373=CARTESIAN_POINT('Ctrl Pts',(0.417681126999945,15.2,11.233651872));
#225374=CARTESIAN_POINT('Ctrl Pts',(0.419162995999944,15.2,11.236787228));
#225375=CARTESIAN_POINT('Ctrl Pts',(0.420649371999945,15.2,11.239925747));
#225376=CARTESIAN_POINT('Ctrl Pts',(0.422140256999944,15.2,11.24306742));
#225377=CARTESIAN_POINT('Ctrl Pts',(0.423635651999945,15.2,11.246212238));
#225378=CARTESIAN_POINT('Ctrl Pts',(0.425135560999944,15.2,11.249360189));
#225379=CARTESIAN_POINT('Ctrl Pts',(0.426940870934353,15.2,11.2531414800626));
#225380=CARTESIAN_POINT('Ctrl Pts',(0.42875295653274,15.2,11.2569274424687));
#225381=CARTESIAN_POINT('Ctrl Pts',(0.430571823467149,15.2,11.2607180595313));
#225382=CARTESIAN_POINT('Ctrl Pts',(0.432397475065532,15.2,11.2645133069374));
#225383=CARTESIAN_POINT('Ctrl Pts',(0.434229916999945,15.2,11.268313168));
#225384=CARTESIAN_POINT('Ctrl Pts',(0.435761481999943,15.2,11.271482787));
#225385=CARTESIAN_POINT('Ctrl Pts',(0.437297575999944,15.2,11.27465546));
#225386=CARTESIAN_POINT('Ctrl Pts',(0.438838203999945,15.2,11.277831182));
#225387=CARTESIAN_POINT('Ctrl Pts',(0.440383366999945,15.2,11.28100994));
#225388=CARTESIAN_POINT('Ctrl Pts',(0.441933066999944,15.2,11.284191726));
#225389=CARTESIAN_POINT('Ctrl Pts',(0.443487306999945,15.2,11.287376529));
#225390=CARTESIAN_POINT('Ctrl Pts',(0.445046087999945,15.2,11.290564341));
#225391=CARTESIAN_POINT('Ctrl Pts',(0.446609412999944,15.2,11.293755151));
#225392=CARTESIAN_POINT('Ctrl Pts',(0.448177283999945,15.2,11.296948952));
#225393=CARTESIAN_POINT('Ctrl Pts',(0.449749701999943,15.2,11.300145732));
#225394=CARTESIAN_POINT('Ctrl Pts',(0.451326669999944,15.2,11.303345481));
#225395=CARTESIAN_POINT('Ctrl Pts',(0.452908190999944,15.2,11.306548191));
#225396=CARTESIAN_POINT('Ctrl Pts',(0.454494264999944,15.2,11.309753854));
#225397=CARTESIAN_POINT('Ctrl Pts',(0.456084895999943,15.2,11.312962457));
#225398=CARTESIAN_POINT('Ctrl Pts',(0.457680083999945,15.2,11.316173992));
#225399=CARTESIAN_POINT('Ctrl Pts',(0.459279831999944,15.2,11.319388451));
#225400=CARTESIAN_POINT('Ctrl Pts',(0.460884141999944,15.2,11.322605823));
#225401=CARTESIAN_POINT('Ctrl Pts',(0.462493016999945,15.2,11.325826099));
#225402=CARTESIAN_POINT('Ctrl Pts',(0.464106456999945,15.2,11.329049269));
#225403=CARTESIAN_POINT('Ctrl Pts',(0.465724464999945,15.2,11.332275324));
#225404=CARTESIAN_POINT('Ctrl Pts',(0.467347043999944,15.2,11.335504256));
#225405=CARTESIAN_POINT('Ctrl Pts',(0.468974193999945,15.2,11.338736055));
#225406=CARTESIAN_POINT('Ctrl Pts',(0.470605917999943,15.2,11.34197071));
#225407=CARTESIAN_POINT('Ctrl Pts',(0.472242216999945,15.2,11.345208212));
#225408=CARTESIAN_POINT('Ctrl Pts',(0.473883093999945,15.2,11.348448553));
#225409=CARTESIAN_POINT('Ctrl Pts',(0.475528549999943,15.2,11.351691724));
#225410=CARTESIAN_POINT('Ctrl Pts',(0.477178588999945,15.2,11.354937714));
#225411=CARTESIAN_POINT('Ctrl Pts',(0.478833209999945,15.2,11.358186515));
#225412=CARTESIAN_POINT('Ctrl Pts',(0.480492415999944,15.2,11.361438117));
#225413=CARTESIAN_POINT('Ctrl Pts',(0.482156208999944,15.2,11.364692512));
#225414=CARTESIAN_POINT('Ctrl Pts',(0.483824590999945,15.2,11.36794969));
#225415=CARTESIAN_POINT('Ctrl Pts',(0.485497562999945,15.2,11.371209642));
#225416=CARTESIAN_POINT('Ctrl Pts',(0.487175127999944,15.2,11.374472358));
#225417=CARTESIAN_POINT('Ctrl Pts',(0.488857286999943,15.2,11.37773783));
#225418=CARTESIAN_POINT('Ctrl Pts',(0.490544042999945,15.2,11.381006048));
#225419=CARTESIAN_POINT('Ctrl Pts',(0.492235395999945,15.2,11.384277002));
#225420=CARTESIAN_POINT('Ctrl Pts',(0.493931348999944,15.2,11.387550685));
#225421=CARTESIAN_POINT('Ctrl Pts',(0.495631902999945,15.2,11.390827085));
#225422=CARTESIAN_POINT('Ctrl Pts',(0.497337059999945,15.2,11.394106196));
#225423=CARTESIAN_POINT('Ctrl Pts',(0.499046822999943,15.2,11.397388008));
#225424=CARTESIAN_POINT('Ctrl Pts',(0.500761191999944,15.2,11.400672511));
#225425=CARTESIAN_POINT('Ctrl Pts',(0.502480167999945,15.2,11.403959697));
#225426=CARTESIAN_POINT('Ctrl Pts',(0.504203755999945,15.2,11.407249557));
#225427=CARTESIAN_POINT('Ctrl Pts',(0.505931953999944,15.2,11.410542081));
#225428=CARTESIAN_POINT('Ctrl Pts',(0.507664765999943,15.2,11.413837262));
#225429=CARTESIAN_POINT('Ctrl Pts',(0.509402193999944,15.2,11.417135088));
#225430=CARTESIAN_POINT('Ctrl Pts',(0.511144237999944,15.2,11.420435552));
#225431=CARTESIAN_POINT('Ctrl Pts',(0.512890899999944,15.2,11.423738642));
#225432=CARTESIAN_POINT('Ctrl Pts',(0.514642183999944,15.2,11.427044351));
#225433=CARTESIAN_POINT('Ctrl Pts',(0.516398088999944,15.2,11.43035267));
#225434=CARTESIAN_POINT('Ctrl Pts',(0.518158616999944,15.2,11.43366359));
#225435=CARTESIAN_POINT('Ctrl Pts',(0.519923770999945,15.2,11.436977102));
#225436=CARTESIAN_POINT('Ctrl Pts',(0.521693550999944,15.2,11.440293201));
#225437=CARTESIAN_POINT('Ctrl Pts',(0.523467958999944,15.2,11.443611876));
#225438=CARTESIAN_POINT('Ctrl Pts',(0.525246995999944,15.2,11.446933119));
#225439=CARTESIAN_POINT('Ctrl Pts',(0.527030663999944,15.2,11.450256921));
#225440=CARTESIAN_POINT('Ctrl Pts',(0.528818964999944,15.2,11.453583273));
#225441=CARTESIAN_POINT('Ctrl Pts',(0.530611901999943,15.2,11.456912161));
#225442=CARTESIAN_POINT('Ctrl Pts',(0.532409473999944,15.2,11.460243578));
#225443=CARTESIAN_POINT('Ctrl Pts',(0.534211683999944,15.2,11.46357751));
#225444=CARTESIAN_POINT('Ctrl Pts',(0.536018536999944,15.2,11.466913949));
#225445=CARTESIAN_POINT('Ctrl Pts',(0.537830029999945,15.2,11.470252887));
#225446=CARTESIAN_POINT('Ctrl Pts',(0.539646165999944,15.2,11.473594318));
#225447=CARTESIAN_POINT('Ctrl Pts',(0.541466945999944,15.2,11.476938237));
#225448=CARTESIAN_POINT('Ctrl Pts',(0.543292368999944,15.2,11.480284644));
#225449=CARTESIAN_POINT('Ctrl Pts',(0.544756420999944,15.2,11.482963756));
#225450=CARTESIAN_POINT('Ctrl Pts',(0.545856550999945,15.2,11.484974209));
#225451=CARTESIAN_POINT('Ctrl Pts',(0.546590898999945,15.2,11.486315008));
#225452=CARTESIAN_POINT('Ctrl Pts',(0.546958305999944,15.2,11.486985532));
#225453=CARTESIAN_POINT('Ctrl Pts',(1.18690176599994,15.2,10.306885525));
#225454=CARTESIAN_POINT('Ctrl Pts',(1.18690176599994,11.6,10.306885525));
#225455=CARTESIAN_POINT('Ctrl Pts',(1.18690675299994,15.2,10.307059811));
#225456=CARTESIAN_POINT('Ctrl Pts',(1.18690675299994,11.6,10.307059811));
#225457=CARTESIAN_POINT('Ctrl Pts',(1.18691681599994,15.2,10.307414474));
#225458=CARTESIAN_POINT('Ctrl Pts',(1.18691681599994,11.6,10.307414474));
#225459=CARTESIAN_POINT('Ctrl Pts',(1.18693179799994,15.2,10.30795188));
#225460=CARTESIAN_POINT('Ctrl Pts',(1.18693179799994,11.6,10.30795188));
#225461=CARTESIAN_POINT('Ctrl Pts',(1.18695143899994,15.2,10.30867583));
#225462=CARTESIAN_POINT('Ctrl Pts',(1.18695143899994,11.6,10.30867583));
#225463=CARTESIAN_POINT('Ctrl Pts',(1.18697536999994,15.2,10.309591544));
#225464=CARTESIAN_POINT('Ctrl Pts',(1.18697536999994,11.6,10.309591544));
#225465=CARTESIAN_POINT('Ctrl Pts',(1.18699875399994,15.2,10.310522124));
#225466=CARTESIAN_POINT('Ctrl Pts',(1.18699875399994,11.6,10.310522124));
#225467=CARTESIAN_POINT('Ctrl Pts',(1.18702143499994,15.2,10.311462238));
#225468=CARTESIAN_POINT('Ctrl Pts',(1.18702143499994,11.6,10.311462238));
#225469=CARTESIAN_POINT('Ctrl Pts',(1.18704339299994,15.2,10.312411862));
#225470=CARTESIAN_POINT('Ctrl Pts',(1.18704339299994,11.6,10.312411862));
#225471=CARTESIAN_POINT('Ctrl Pts',(1.18706460899994,15.2,10.313370965));
#225472=CARTESIAN_POINT('Ctrl Pts',(1.18706460899994,11.6,10.313370965));
#225473=CARTESIAN_POINT('Ctrl Pts',(1.18708506599994,15.2,10.314339525));
#225474=CARTESIAN_POINT('Ctrl Pts',(1.18708506599994,11.6,10.314339525));
#225475=CARTESIAN_POINT('Ctrl Pts',(1.18710474299994,15.2,10.315317514));
#225476=CARTESIAN_POINT('Ctrl Pts',(1.18710474299994,11.6,10.315317514));
#225477=CARTESIAN_POINT('Ctrl Pts',(1.18712362299994,15.2,10.316304905));
#225478=CARTESIAN_POINT('Ctrl Pts',(1.18712362299994,11.6,10.316304905));
#225479=CARTESIAN_POINT('Ctrl Pts',(1.18714168899994,15.2,10.317301674));
#225480=CARTESIAN_POINT('Ctrl Pts',(1.18714168899994,11.6,10.317301674));
#225481=CARTESIAN_POINT('Ctrl Pts',(1.18715892199994,15.2,10.318307794));
#225482=CARTESIAN_POINT('Ctrl Pts',(1.18715892199994,11.6,10.318307794));
#225483=CARTESIAN_POINT('Ctrl Pts',(1.18717530199994,15.2,10.319323239));
#225484=CARTESIAN_POINT('Ctrl Pts',(1.18717530199994,11.6,10.319323239));
#225485=CARTESIAN_POINT('Ctrl Pts',(1.18719081299994,15.2,10.320347985));
#225486=CARTESIAN_POINT('Ctrl Pts',(1.18719081299994,11.6,10.320347985));
#225487=CARTESIAN_POINT('Ctrl Pts',(1.18720543699994,15.2,10.321382005));
#225488=CARTESIAN_POINT('Ctrl Pts',(1.18720543699994,11.6,10.321382005));
#225489=CARTESIAN_POINT('Ctrl Pts',(1.18721915499994,15.2,10.322425274));
#225490=CARTESIAN_POINT('Ctrl Pts',(1.18721915499994,11.6,10.322425274));
#225491=CARTESIAN_POINT('Ctrl Pts',(1.18723195099994,15.2,10.323477767));
#225492=CARTESIAN_POINT('Ctrl Pts',(1.18723195099994,11.6,10.323477767));
#225493=CARTESIAN_POINT('Ctrl Pts',(1.18724380599994,15.2,10.324539459));
#225494=CARTESIAN_POINT('Ctrl Pts',(1.18724380599994,11.6,10.324539459));
#225495=CARTESIAN_POINT('Ctrl Pts',(1.18725470299994,15.2,10.325610325));
#225496=CARTESIAN_POINT('Ctrl Pts',(1.18725470299994,11.6,10.325610325));
#225497=CARTESIAN_POINT('Ctrl Pts',(1.18726462499994,15.2,10.326690339));
#225498=CARTESIAN_POINT('Ctrl Pts',(1.18726462499994,11.6,10.326690339));
#225499=CARTESIAN_POINT('Ctrl Pts',(1.18727355399994,15.2,10.327779478));
#225500=CARTESIAN_POINT('Ctrl Pts',(1.18727355399994,11.6,10.327779478));
#225501=CARTESIAN_POINT('Ctrl Pts',(1.18728147299994,15.2,10.328877715));
#225502=CARTESIAN_POINT('Ctrl Pts',(1.18728147299994,11.6,10.328877715));
#225503=CARTESIAN_POINT('Ctrl Pts',(1.18728836599994,15.2,10.329985029));
#225504=CARTESIAN_POINT('Ctrl Pts',(1.18728836599994,11.6,10.329985029));
#225505=CARTESIAN_POINT('Ctrl Pts',(1.18729421399994,15.2,10.331101392));
#225506=CARTESIAN_POINT('Ctrl Pts',(1.18729421399994,11.6,10.331101392));
#225507=CARTESIAN_POINT('Ctrl Pts',(1.18729900199994,15.2,10.332226781));
#225508=CARTESIAN_POINT('Ctrl Pts',(1.18729900199994,11.6,10.332226781));
#225509=CARTESIAN_POINT('Ctrl Pts',(1.18730271099994,15.2,10.333361172));
#225510=CARTESIAN_POINT('Ctrl Pts',(1.18730271099994,11.6,10.333361172));
#225511=CARTESIAN_POINT('Ctrl Pts',(1.18730532599994,15.2,10.334504539));
#225512=CARTESIAN_POINT('Ctrl Pts',(1.18730532599994,11.6,10.334504539));
#225513=CARTESIAN_POINT('Ctrl Pts',(1.18730682999994,15.2,10.335656861));
#225514=CARTESIAN_POINT('Ctrl Pts',(1.18730682999994,11.6,10.335656861));
#225515=CARTESIAN_POINT('Ctrl Pts',(1.18730720499994,15.2,10.336818113));
#225516=CARTESIAN_POINT('Ctrl Pts',(1.18730720499994,11.6,10.336818113));
#225517=CARTESIAN_POINT('Ctrl Pts',(1.18730643699994,15.2,10.33798827));
#225518=CARTESIAN_POINT('Ctrl Pts',(1.18730643699994,11.6,10.33798827));
#225519=CARTESIAN_POINT('Ctrl Pts',(1.18730450699994,15.2,10.339167309));
#225520=CARTESIAN_POINT('Ctrl Pts',(1.18730450699994,11.6,10.339167309));
#225521=CARTESIAN_POINT('Ctrl Pts',(1.18730140099994,15.2,10.340355206));
#225522=CARTESIAN_POINT('Ctrl Pts',(1.18730140099994,11.6,10.340355206));
#225523=CARTESIAN_POINT('Ctrl Pts',(1.18729710199994,15.2,10.341551938));
#225524=CARTESIAN_POINT('Ctrl Pts',(1.18729710199994,11.6,10.341551938));
#225525=CARTESIAN_POINT('Ctrl Pts',(1.18729159299995,15.2,10.342757482));
#225526=CARTESIAN_POINT('Ctrl Pts',(1.18729159299995,11.6,10.342757482));
#225527=CARTESIAN_POINT('Ctrl Pts',(1.18728485799994,15.2,10.343971813));
#225528=CARTESIAN_POINT('Ctrl Pts',(1.18728485799994,11.6,10.343971813));
#225529=CARTESIAN_POINT('Ctrl Pts',(1.18727688199994,15.2,10.345194909));
#225530=CARTESIAN_POINT('Ctrl Pts',(1.18727688199994,11.6,10.345194909));
#225531=CARTESIAN_POINT('Ctrl Pts',(1.18726764899994,15.2,10.346426747));
#225532=CARTESIAN_POINT('Ctrl Pts',(1.18726764899994,11.6,10.346426747));
#225533=CARTESIAN_POINT('Ctrl Pts',(1.18725714199994,15.2,10.347667304));
#225534=CARTESIAN_POINT('Ctrl Pts',(1.18725714199994,11.6,10.347667304));
#225535=CARTESIAN_POINT('Ctrl Pts',(1.18724534799994,15.2,10.348916556));
#225536=CARTESIAN_POINT('Ctrl Pts',(1.18724534799994,11.6,10.348916556));
#225537=CARTESIAN_POINT('Ctrl Pts',(1.18723224699994,15.2,10.350174481));
#225538=CARTESIAN_POINT('Ctrl Pts',(1.18723224699994,11.6,10.350174481));
#225539=CARTESIAN_POINT('Ctrl Pts',(1.18721782699994,15.2,10.351441056));
#225540=CARTESIAN_POINT('Ctrl Pts',(1.18721782699994,11.6,10.351441056));
#225541=CARTESIAN_POINT('Ctrl Pts',(1.18720207099994,15.2,10.352716258));
#225542=CARTESIAN_POINT('Ctrl Pts',(1.18720207099994,11.6,10.352716258));
#225543=CARTESIAN_POINT('Ctrl Pts',(1.18718496499994,15.2,10.354000065));
#225544=CARTESIAN_POINT('Ctrl Pts',(1.18718496499994,11.6,10.354000065));
#225545=CARTESIAN_POINT('Ctrl Pts',(1.18716649099994,15.2,10.355292454));
#225546=CARTESIAN_POINT('Ctrl Pts',(1.18716649099994,11.6,10.355292454));
#225547=CARTESIAN_POINT('Ctrl Pts',(1.18714663599994,15.2,10.356593403));
#225548=CARTESIAN_POINT('Ctrl Pts',(1.18714663599994,11.6,10.356593403));
#225549=CARTESIAN_POINT('Ctrl Pts',(1.18712538499994,15.2,10.35790289));
#225550=CARTESIAN_POINT('Ctrl Pts',(1.18712538499994,11.6,10.35790289));
#225551=CARTESIAN_POINT('Ctrl Pts',(1.18710272199994,15.2,10.359220892));
#225552=CARTESIAN_POINT('Ctrl Pts',(1.18710272199994,11.6,10.359220892));
#225553=CARTESIAN_POINT('Ctrl Pts',(1.18707863099994,15.2,10.360547387));
#225554=CARTESIAN_POINT('Ctrl Pts',(1.18707863099994,11.6,10.360547387));
#225555=CARTESIAN_POINT('Ctrl Pts',(1.18705309899994,15.2,10.361882353));
#225556=CARTESIAN_POINT('Ctrl Pts',(1.18705309899994,11.6,10.361882353));
#225557=CARTESIAN_POINT('Ctrl Pts',(1.18702610999994,15.2,10.363225769));
#225558=CARTESIAN_POINT('Ctrl Pts',(1.18702610999994,11.6,10.363225769));
#225559=CARTESIAN_POINT('Ctrl Pts',(1.18699764999994,15.2,10.364577612));
#225560=CARTESIAN_POINT('Ctrl Pts',(1.18699764999994,11.6,10.364577612));
#225561=CARTESIAN_POINT('Ctrl Pts',(1.18696770299994,15.2,10.365937861));
#225562=CARTESIAN_POINT('Ctrl Pts',(1.18696770299994,11.6,10.365937861));
#225563=CARTESIAN_POINT('Ctrl Pts',(1.18693625599994,15.2,10.367306493));
#225564=CARTESIAN_POINT('Ctrl Pts',(1.18693625599994,11.6,10.367306493));
#225565=CARTESIAN_POINT('Ctrl Pts',(1.18690329299994,15.2,10.368683488));
#225566=CARTESIAN_POINT('Ctrl Pts',(1.18690329299994,11.6,10.368683488));
#225567=CARTESIAN_POINT('Ctrl Pts',(1.18686879999994,15.2,10.370068824));
#225568=CARTESIAN_POINT('Ctrl Pts',(1.18686879999994,11.6,10.370068824));
#225569=CARTESIAN_POINT('Ctrl Pts',(1.18683276299994,15.2,10.371462478));
#225570=CARTESIAN_POINT('Ctrl Pts',(1.18683276299994,11.6,10.371462478));
#225571=CARTESIAN_POINT('Ctrl Pts',(1.18679516799994,15.2,10.372864432));
#225572=CARTESIAN_POINT('Ctrl Pts',(1.18679516799994,11.6,10.372864432));
#225573=CARTESIAN_POINT('Ctrl Pts',(1.18675599899994,15.2,10.37427466));
#225574=CARTESIAN_POINT('Ctrl Pts',(1.18675599899994,11.6,10.37427466));
#225575=CARTESIAN_POINT('Ctrl Pts',(1.18671524299994,15.2,10.375693146));
#225576=CARTESIAN_POINT('Ctrl Pts',(1.18671524299994,11.6,10.375693146));
#225577=CARTESIAN_POINT('Ctrl Pts',(1.18667288599994,15.2,10.377119865));
#225578=CARTESIAN_POINT('Ctrl Pts',(1.18667288599994,11.6,10.377119865));
#225579=CARTESIAN_POINT('Ctrl Pts',(1.18662891299994,15.2,10.378554798));
#225580=CARTESIAN_POINT('Ctrl Pts',(1.18662891299994,11.6,10.378554798));
#225581=CARTESIAN_POINT('Ctrl Pts',(1.18658331199994,15.2,10.379997924));
#225582=CARTESIAN_POINT('Ctrl Pts',(1.18658331199994,11.6,10.379997924));
#225583=CARTESIAN_POINT('Ctrl Pts',(1.18653606599994,15.2,10.38144922));
#225584=CARTESIAN_POINT('Ctrl Pts',(1.18653606599994,11.6,10.38144922));
#225585=CARTESIAN_POINT('Ctrl Pts',(1.18648716499994,15.2,10.382908668));
#225586=CARTESIAN_POINT('Ctrl Pts',(1.18648716499994,11.6,10.382908668));
#225587=CARTESIAN_POINT('Ctrl Pts',(1.18643659099994,15.2,10.384376246));
#225588=CARTESIAN_POINT('Ctrl Pts',(1.18643659099994,11.6,10.384376246));
#225589=CARTESIAN_POINT('Ctrl Pts',(1.18638433299994,15.2,10.385851932));
#225590=CARTESIAN_POINT('Ctrl Pts',(1.18638433299994,11.6,10.385851932));
#225591=CARTESIAN_POINT('Ctrl Pts',(1.18633037699994,15.2,10.387335709));
#225592=CARTESIAN_POINT('Ctrl Pts',(1.18633037699994,11.6,10.387335709));
#225593=CARTESIAN_POINT('Ctrl Pts',(1.18627470899994,15.2,10.388827552));
#225594=CARTESIAN_POINT('Ctrl Pts',(1.18627470899994,11.6,10.388827552));
#225595=CARTESIAN_POINT('Ctrl Pts',(1.18621731499994,15.2,10.390327445));
#225596=CARTESIAN_POINT('Ctrl Pts',(1.18621731499994,11.6,10.390327445));
#225597=CARTESIAN_POINT('Ctrl Pts',(1.18615818399994,15.2,10.391835364));
#225598=CARTESIAN_POINT('Ctrl Pts',(1.18615818399994,11.6,10.391835364));
#225599=CARTESIAN_POINT('Ctrl Pts',(1.18609729899994,15.2,10.393351292));
#225600=CARTESIAN_POINT('Ctrl Pts',(1.18609729899994,11.6,10.393351292));
#225601=CARTESIAN_POINT('Ctrl Pts',(1.18603464799994,15.2,10.394875207));
#225602=CARTESIAN_POINT('Ctrl Pts',(1.18603464799994,11.6,10.394875207));
#225603=CARTESIAN_POINT('Ctrl Pts',(1.18597021899994,15.2,10.396407089));
#225604=CARTESIAN_POINT('Ctrl Pts',(1.18597021899994,11.6,10.396407089));
#225605=CARTESIAN_POINT('Ctrl Pts',(1.18590399799994,15.2,10.397946917));
#225606=CARTESIAN_POINT('Ctrl Pts',(1.18590399799994,11.6,10.397946917));
#225607=CARTESIAN_POINT('Ctrl Pts',(1.18583597199994,15.2,10.399494672));
#225608=CARTESIAN_POINT('Ctrl Pts',(1.18583597199994,11.6,10.399494672));
#225609=CARTESIAN_POINT('Ctrl Pts',(1.18576612699994,15.2,10.401050336));
#225610=CARTESIAN_POINT('Ctrl Pts',(1.18576612699994,11.6,10.401050336));
#225611=CARTESIAN_POINT('Ctrl Pts',(1.18569445199994,15.2,10.402613886));
#225612=CARTESIAN_POINT('Ctrl Pts',(1.18569445199994,11.6,10.402613886));
#225613=CARTESIAN_POINT('Ctrl Pts',(1.18562093099994,15.2,10.404185304));
#225614=CARTESIAN_POINT('Ctrl Pts',(1.18562093099994,11.6,10.404185304));
#225615=CARTESIAN_POINT('Ctrl Pts',(1.18554555399994,15.2,10.405764571));
#225616=CARTESIAN_POINT('Ctrl Pts',(1.18554555399994,11.6,10.405764571));
#225617=CARTESIAN_POINT('Ctrl Pts',(1.18546830699994,15.2,10.407351665));
#225618=CARTESIAN_POINT('Ctrl Pts',(1.18546830699994,11.6,10.407351665));
#225619=CARTESIAN_POINT('Ctrl Pts',(1.18538917699994,15.2,10.408946569));
#225620=CARTESIAN_POINT('Ctrl Pts',(1.18538917699994,11.6,10.408946569));
#225621=CARTESIAN_POINT('Ctrl Pts',(1.18530815299994,15.2,10.410549261));
#225622=CARTESIAN_POINT('Ctrl Pts',(1.18530815299994,11.6,10.410549261));
#225623=CARTESIAN_POINT('Ctrl Pts',(1.18522521999994,15.2,10.412159724));
#225624=CARTESIAN_POINT('Ctrl Pts',(1.18522521999994,11.6,10.412159724));
#225625=CARTESIAN_POINT('Ctrl Pts',(1.18514036599994,15.2,10.413777937));
#225626=CARTESIAN_POINT('Ctrl Pts',(1.18514036599994,11.6,10.413777937));
#225627=CARTESIAN_POINT('Ctrl Pts',(1.18505357899994,15.2,10.415403882));
#225628=CARTESIAN_POINT('Ctrl Pts',(1.18505357899994,11.6,10.415403882));
#225629=CARTESIAN_POINT('Ctrl Pts',(1.18496484699994,15.2,10.417037539));
#225630=CARTESIAN_POINT('Ctrl Pts',(1.18496484699994,11.6,10.417037539));
#225631=CARTESIAN_POINT('Ctrl Pts',(1.18487415699994,15.2,10.418678889));
#225632=CARTESIAN_POINT('Ctrl Pts',(1.18487415699994,11.6,10.418678889));
#225633=CARTESIAN_POINT('Ctrl Pts',(1.18478149599994,15.2,10.420327914));
#225634=CARTESIAN_POINT('Ctrl Pts',(1.18478149599994,11.6,10.420327914));
#225635=CARTESIAN_POINT('Ctrl Pts',(1.18468685299994,15.2,10.421984593));
#225636=CARTESIAN_POINT('Ctrl Pts',(1.18468685299994,11.6,10.421984593));
#225637=CARTESIAN_POINT('Ctrl Pts',(1.18459021499994,15.2,10.423648908));
#225638=CARTESIAN_POINT('Ctrl Pts',(1.18459021499994,11.6,10.423648908));
#225639=CARTESIAN_POINT('Ctrl Pts',(1.18449156999994,15.2,10.42532084));
#225640=CARTESIAN_POINT('Ctrl Pts',(1.18449156999994,11.6,10.42532084));
#225641=CARTESIAN_POINT('Ctrl Pts',(1.18439090699994,15.2,10.427000372));
#225642=CARTESIAN_POINT('Ctrl Pts',(1.18439090699994,11.6,10.427000372));
#225643=CARTESIAN_POINT('Ctrl Pts',(1.18428821199994,15.2,10.428687483));
#225644=CARTESIAN_POINT('Ctrl Pts',(1.18428821199994,11.6,10.428687483));
#225645=CARTESIAN_POINT('Ctrl Pts',(1.18418347299994,15.2,10.430382155));
#225646=CARTESIAN_POINT('Ctrl Pts',(1.18418347299994,11.6,10.430382155));
#225647=CARTESIAN_POINT('Ctrl Pts',(1.18407667999994,15.2,10.432084369));
#225648=CARTESIAN_POINT('Ctrl Pts',(1.18407667999994,11.6,10.432084369));
#225649=CARTESIAN_POINT('Ctrl Pts',(1.18396781899994,15.2,10.433794108));
#225650=CARTESIAN_POINT('Ctrl Pts',(1.18396781899994,11.6,10.433794108));
#225651=CARTESIAN_POINT('Ctrl Pts',(1.18385688099994,15.2,10.435511351));
#225652=CARTESIAN_POINT('Ctrl Pts',(1.18385688099994,11.6,10.435511351));
#225653=CARTESIAN_POINT('Ctrl Pts',(1.18374385099994,15.2,10.437236081));
#225654=CARTESIAN_POINT('Ctrl Pts',(1.18374385099994,11.6,10.437236081));
#225655=CARTESIAN_POINT('Ctrl Pts',(1.18362871899994,15.2,10.438968281));
#225656=CARTESIAN_POINT('Ctrl Pts',(1.18362871899994,11.6,10.438968281));
#225657=CARTESIAN_POINT('Ctrl Pts',(1.18351147299994,15.2,10.440707931));
#225658=CARTESIAN_POINT('Ctrl Pts',(1.18351147299994,11.6,10.440707931));
#225659=CARTESIAN_POINT('Ctrl Pts',(1.18339210199994,15.2,10.442455013));
#225660=CARTESIAN_POINT('Ctrl Pts',(1.18339210199994,11.6,10.442455013));
#225661=CARTESIAN_POINT('Ctrl Pts',(1.18327059299994,15.2,10.444209509));
#225662=CARTESIAN_POINT('Ctrl Pts',(1.18327059299994,11.6,10.444209509));
#225663=CARTESIAN_POINT('Ctrl Pts',(1.18314693599994,15.2,10.445971401));
#225664=CARTESIAN_POINT('Ctrl Pts',(1.18314693599994,11.6,10.445971401));
#225665=CARTESIAN_POINT('Ctrl Pts',(1.18302111899994,15.2,10.44774067));
#225666=CARTESIAN_POINT('Ctrl Pts',(1.18302111899994,11.6,10.44774067));
#225667=CARTESIAN_POINT('Ctrl Pts',(1.18289312999994,15.2,10.4495173));
#225668=CARTESIAN_POINT('Ctrl Pts',(1.18289312999994,11.6,10.4495173));
#225669=CARTESIAN_POINT('Ctrl Pts',(1.18276295899994,15.2,10.45130127));
#225670=CARTESIAN_POINT('Ctrl Pts',(1.18276295899994,11.6,10.45130127));
#225671=CARTESIAN_POINT('Ctrl Pts',(1.18263059299994,15.2,10.453092566));
#225672=CARTESIAN_POINT('Ctrl Pts',(1.18263059299994,11.6,10.453092566));
#225673=CARTESIAN_POINT('Ctrl Pts',(1.18249602099994,15.2,10.454891167));
#225674=CARTESIAN_POINT('Ctrl Pts',(1.18249602099994,11.6,10.454891167));
#225675=CARTESIAN_POINT('Ctrl Pts',(1.18235923399994,15.2,10.456697057));
#225676=CARTESIAN_POINT('Ctrl Pts',(1.18235923399994,11.6,10.456697057));
#225677=CARTESIAN_POINT('Ctrl Pts',(1.18222021799994,15.2,10.458510218));
#225678=CARTESIAN_POINT('Ctrl Pts',(1.18222021799994,11.6,10.458510218));
#225679=CARTESIAN_POINT('Ctrl Pts',(1.18207896399994,15.2,10.460330631));
#225680=CARTESIAN_POINT('Ctrl Pts',(1.18207896399994,11.6,10.460330631));
#225681=CARTESIAN_POINT('Ctrl Pts',(1.18193546099994,15.2,10.46215828));
#225682=CARTESIAN_POINT('Ctrl Pts',(1.18193546099994,11.6,10.46215828));
#225683=CARTESIAN_POINT('Ctrl Pts',(1.18178969499994,15.2,10.463993147));
#225684=CARTESIAN_POINT('Ctrl Pts',(1.18178969499994,11.6,10.463993147));
#225685=CARTESIAN_POINT('Ctrl Pts',(1.18164165899994,15.2,10.465835214));
#225686=CARTESIAN_POINT('Ctrl Pts',(1.18164165899994,11.6,10.465835214));
#225687=CARTESIAN_POINT('Ctrl Pts',(1.18149133899994,15.2,10.467684465));
#225688=CARTESIAN_POINT('Ctrl Pts',(1.18149133899994,11.6,10.467684465));
#225689=CARTESIAN_POINT('Ctrl Pts',(1.18133872599994,15.2,10.469540881));
#225690=CARTESIAN_POINT('Ctrl Pts',(1.18133872599994,11.6,10.469540881));
#225691=CARTESIAN_POINT('Ctrl Pts',(1.18118380799994,15.2,10.471404446));
#225692=CARTESIAN_POINT('Ctrl Pts',(1.18118380799994,11.6,10.471404446));
#225693=CARTESIAN_POINT('Ctrl Pts',(1.18102657599994,15.2,10.473275141));
#225694=CARTESIAN_POINT('Ctrl Pts',(1.18102657599994,11.6,10.473275141));
#225695=CARTESIAN_POINT('Ctrl Pts',(1.18086701799994,15.2,10.475152951));
#225696=CARTESIAN_POINT('Ctrl Pts',(1.18086701799994,11.6,10.475152951));
#225697=CARTESIAN_POINT('Ctrl Pts',(1.18070512299994,15.2,10.477037857));
#225698=CARTESIAN_POINT('Ctrl Pts',(1.18070512299994,11.6,10.477037857));
#225699=CARTESIAN_POINT('Ctrl Pts',(1.18054088199994,15.2,10.478929843));
#225700=CARTESIAN_POINT('Ctrl Pts',(1.18054088199994,11.6,10.478929843));
#225701=CARTESIAN_POINT('Ctrl Pts',(1.18037428299994,15.2,10.480828891));
#225702=CARTESIAN_POINT('Ctrl Pts',(1.18037428299994,11.6,10.480828891));
#225703=CARTESIAN_POINT('Ctrl Pts',(1.18020531499994,15.2,10.482734986));
#225704=CARTESIAN_POINT('Ctrl Pts',(1.18020531499994,11.6,10.482734986));
#225705=CARTESIAN_POINT('Ctrl Pts',(1.18003396899994,15.2,10.484648108));
#225706=CARTESIAN_POINT('Ctrl Pts',(1.18003396899994,11.6,10.484648108));
#225707=CARTESIAN_POINT('Ctrl Pts',(1.17986023499994,15.2,10.486568243));
#225708=CARTESIAN_POINT('Ctrl Pts',(1.17986023499994,11.6,10.486568243));
#225709=CARTESIAN_POINT('Ctrl Pts',(1.17968410099994,15.2,10.488495372));
#225710=CARTESIAN_POINT('Ctrl Pts',(1.17968410099994,11.6,10.488495372));
#225711=CARTESIAN_POINT('Ctrl Pts',(1.17950555699994,15.2,10.49042948));
#225712=CARTESIAN_POINT('Ctrl Pts',(1.17950555699994,11.6,10.49042948));
#225713=CARTESIAN_POINT('Ctrl Pts',(1.17932459299994,15.2,10.492370549));
#225714=CARTESIAN_POINT('Ctrl Pts',(1.17932459299994,11.6,10.492370549));
#225715=CARTESIAN_POINT('Ctrl Pts',(1.17914119899994,15.2,10.494318564));
#225716=CARTESIAN_POINT('Ctrl Pts',(1.17914119899994,11.6,10.494318564));
#225717=CARTESIAN_POINT('Ctrl Pts',(1.17895536499994,15.2,10.496273505));
#225718=CARTESIAN_POINT('Ctrl Pts',(1.17895536499994,11.6,10.496273505));
#225719=CARTESIAN_POINT('Ctrl Pts',(1.17876707999994,15.2,10.498235359));
#225720=CARTESIAN_POINT('Ctrl Pts',(1.17876707999994,11.6,10.498235359));
#225721=CARTESIAN_POINT('Ctrl Pts',(1.17857633499994,15.2,10.500204107));
#225722=CARTESIAN_POINT('Ctrl Pts',(1.17857633499994,11.6,10.500204107));
#225723=CARTESIAN_POINT('Ctrl Pts',(1.17838311899994,15.2,10.502179735));
#225724=CARTESIAN_POINT('Ctrl Pts',(1.17838311899994,11.6,10.502179735));
#225725=CARTESIAN_POINT('Ctrl Pts',(1.17818742199994,15.2,10.504162224));
#225726=CARTESIAN_POINT('Ctrl Pts',(1.17818742199994,11.6,10.504162224));
#225727=CARTESIAN_POINT('Ctrl Pts',(1.17798923499994,15.2,10.50615156));
#225728=CARTESIAN_POINT('Ctrl Pts',(1.17798923499994,11.6,10.50615156));
#225729=CARTESIAN_POINT('Ctrl Pts',(1.17778854699994,15.2,10.508147724));
#225730=CARTESIAN_POINT('Ctrl Pts',(1.17778854699994,11.6,10.508147724));
#225731=CARTESIAN_POINT('Ctrl Pts',(1.17758534899994,15.2,10.510150701));
#225732=CARTESIAN_POINT('Ctrl Pts',(1.17758534899994,11.6,10.510150701));
#225733=CARTESIAN_POINT('Ctrl Pts',(1.17737963099994,15.2,10.512160476));
#225734=CARTESIAN_POINT('Ctrl Pts',(1.17737963099994,11.6,10.512160476));
#225735=CARTESIAN_POINT('Ctrl Pts',(1.17717138199994,15.2,10.514177031));
#225736=CARTESIAN_POINT('Ctrl Pts',(1.17717138199994,11.6,10.514177031));
#225737=CARTESIAN_POINT('Ctrl Pts',(1.17696059399994,15.2,10.51620035));
#225738=CARTESIAN_POINT('Ctrl Pts',(1.17696059399994,11.6,10.51620035));
#225739=CARTESIAN_POINT('Ctrl Pts',(1.17674725699994,15.2,10.518230418));
#225740=CARTESIAN_POINT('Ctrl Pts',(1.17674725699994,11.6,10.518230418));
#225741=CARTESIAN_POINT('Ctrl Pts',(1.17653135999994,15.2,10.520267219));
#225742=CARTESIAN_POINT('Ctrl Pts',(1.17653135999994,11.6,10.520267219));
#225743=CARTESIAN_POINT('Ctrl Pts',(1.17631289399994,15.2,10.522310736));
#225744=CARTESIAN_POINT('Ctrl Pts',(1.17631289399994,11.6,10.522310736));
#225745=CARTESIAN_POINT('Ctrl Pts',(1.17609184899994,15.2,10.524360953));
#225746=CARTESIAN_POINT('Ctrl Pts',(1.17609184899994,11.6,10.524360953));
#225747=CARTESIAN_POINT('Ctrl Pts',(1.17586821799994,15.2,10.526417855));
#225748=CARTESIAN_POINT('Ctrl Pts',(1.17586821799994,11.6,10.526417855));
#225749=CARTESIAN_POINT('Ctrl Pts',(1.17564198899994,15.2,10.528481426));
#225750=CARTESIAN_POINT('Ctrl Pts',(1.17564198899994,11.6,10.528481426));
#225751=CARTESIAN_POINT('Ctrl Pts',(1.17541315199994,15.2,10.530551649));
#225752=CARTESIAN_POINT('Ctrl Pts',(1.17541315199994,11.6,10.530551649));
#225753=CARTESIAN_POINT('Ctrl Pts',(1.17518169999994,15.2,10.53262851));
#225754=CARTESIAN_POINT('Ctrl Pts',(1.17518169999994,11.6,10.53262851));
#225755=CARTESIAN_POINT('Ctrl Pts',(1.17494762299994,15.2,10.534711991));
#225756=CARTESIAN_POINT('Ctrl Pts',(1.17494762299994,11.6,10.534711991));
#225757=CARTESIAN_POINT('Ctrl Pts',(1.17471090899994,15.2,10.536802079));
#225758=CARTESIAN_POINT('Ctrl Pts',(1.17471090899994,11.6,10.536802079));
#225759=CARTESIAN_POINT('Ctrl Pts',(1.17447155199994,15.2,10.538898756));
#225760=CARTESIAN_POINT('Ctrl Pts',(1.17447155199994,11.6,10.538898756));
#225761=CARTESIAN_POINT('Ctrl Pts',(1.17422954199994,15.2,10.541002008));
#225762=CARTESIAN_POINT('Ctrl Pts',(1.17422954199994,11.6,10.541002008));
#225763=CARTESIAN_POINT('Ctrl Pts',(1.17398486799994,15.2,10.543111819));
#225764=CARTESIAN_POINT('Ctrl Pts',(1.17398486799994,11.6,10.543111819));
#225765=CARTESIAN_POINT('Ctrl Pts',(1.17373752299994,15.2,10.545228173));
#225766=CARTESIAN_POINT('Ctrl Pts',(1.17373752299994,11.6,10.545228173));
#225767=CARTESIAN_POINT('Ctrl Pts',(1.17348749699994,15.2,10.547351055));
#225768=CARTESIAN_POINT('Ctrl Pts',(1.17348749699994,11.6,10.547351055));
#225769=CARTESIAN_POINT('Ctrl Pts',(1.17323478099994,15.2,10.549480449));
#225770=CARTESIAN_POINT('Ctrl Pts',(1.17323478099994,11.6,10.549480449));
#225771=CARTESIAN_POINT('Ctrl Pts',(1.17297936399994,15.2,10.551616341));
#225772=CARTESIAN_POINT('Ctrl Pts',(1.17297936399994,11.6,10.551616341));
#225773=CARTESIAN_POINT('Ctrl Pts',(1.17272123999994,15.2,10.553758715));
#225774=CARTESIAN_POINT('Ctrl Pts',(1.17272123999994,11.6,10.553758715));
#225775=CARTESIAN_POINT('Ctrl Pts',(1.17246039899994,15.2,10.555907554));
#225776=CARTESIAN_POINT('Ctrl Pts',(1.17246039899994,11.6,10.555907554));
#225777=CARTESIAN_POINT('Ctrl Pts',(1.17219683199994,15.2,10.558062846));
#225778=CARTESIAN_POINT('Ctrl Pts',(1.17219683199994,11.6,10.558062846));
#225779=CARTESIAN_POINT('Ctrl Pts',(1.17193052999994,15.2,10.560224573));
#225780=CARTESIAN_POINT('Ctrl Pts',(1.17193052999994,11.6,10.560224573));
#225781=CARTESIAN_POINT('Ctrl Pts',(1.17166148399994,15.2,10.562392721));
#225782=CARTESIAN_POINT('Ctrl Pts',(1.17166148399994,11.6,10.562392721));
#225783=CARTESIAN_POINT('Ctrl Pts',(1.17138968499995,15.2,10.564567275));
#225784=CARTESIAN_POINT('Ctrl Pts',(1.17138968499995,11.6,10.564567275));
#225785=CARTESIAN_POINT('Ctrl Pts',(1.17111512399994,15.2,10.566748219));
#225786=CARTESIAN_POINT('Ctrl Pts',(1.17111512399994,11.6,10.566748219));
#225787=CARTESIAN_POINT('Ctrl Pts',(1.17083779399994,15.2,10.56893554));
#225788=CARTESIAN_POINT('Ctrl Pts',(1.17083779399994,11.6,10.56893554));
#225789=CARTESIAN_POINT('Ctrl Pts',(1.17055768399994,15.2,10.57112922));
#225790=CARTESIAN_POINT('Ctrl Pts',(1.17055768399994,11.6,10.57112922));
#225791=CARTESIAN_POINT('Ctrl Pts',(1.17027478699994,15.2,10.573329246));
#225792=CARTESIAN_POINT('Ctrl Pts',(1.17027478699994,11.6,10.573329246));
#225793=CARTESIAN_POINT('Ctrl Pts',(1.16998909399994,15.2,10.575535604));
#225794=CARTESIAN_POINT('Ctrl Pts',(1.16998909399994,11.6,10.575535604));
#225795=CARTESIAN_POINT('Ctrl Pts',(1.16970059499994,15.2,10.577748277));
#225796=CARTESIAN_POINT('Ctrl Pts',(1.16970059499994,11.6,10.577748277));
#225797=CARTESIAN_POINT('Ctrl Pts',(1.16940928299994,15.2,10.579967251));
#225798=CARTESIAN_POINT('Ctrl Pts',(1.16940928299994,11.6,10.579967251));
#225799=CARTESIAN_POINT('Ctrl Pts',(1.16911514899994,15.2,10.582192511));
#225800=CARTESIAN_POINT('Ctrl Pts',(1.16911514899994,11.6,10.582192511));
#225801=CARTESIAN_POINT('Ctrl Pts',(1.16881818499994,15.2,10.584424043));
#225802=CARTESIAN_POINT('Ctrl Pts',(1.16881818499994,11.6,10.584424043));
#225803=CARTESIAN_POINT('Ctrl Pts',(1.16851838099994,15.2,10.586661831));
#225804=CARTESIAN_POINT('Ctrl Pts',(1.16851838099994,11.6,10.586661831));
#225805=CARTESIAN_POINT('Ctrl Pts',(1.16821573099994,15.2,10.588905861));
#225806=CARTESIAN_POINT('Ctrl Pts',(1.16821573099994,11.6,10.588905861));
#225807=CARTESIAN_POINT('Ctrl Pts',(1.16791022399994,15.2,10.59115612));
#225808=CARTESIAN_POINT('Ctrl Pts',(1.16791022399994,11.6,10.59115612));
#225809=CARTESIAN_POINT('Ctrl Pts',(1.16760185299994,15.2,10.59341259));
#225810=CARTESIAN_POINT('Ctrl Pts',(1.16760185299994,11.6,10.59341259));
#225811=CARTESIAN_POINT('Ctrl Pts',(1.16729060999994,15.2,10.595675259));
#225812=CARTESIAN_POINT('Ctrl Pts',(1.16729060999994,11.6,10.595675259));
#225813=CARTESIAN_POINT('Ctrl Pts',(1.16697648499994,15.2,10.597944112));
#225814=CARTESIAN_POINT('Ctrl Pts',(1.16697648499994,11.6,10.597944112));
#225815=CARTESIAN_POINT('Ctrl Pts',(1.16665947299994,15.2,10.600219134));
#225816=CARTESIAN_POINT('Ctrl Pts',(1.16665947299994,11.6,10.600219134));
#225817=CARTESIAN_POINT('Ctrl Pts',(1.16633956199994,15.2,10.602500311));
#225818=CARTESIAN_POINT('Ctrl Pts',(1.16633956199994,11.6,10.602500311));
#225819=CARTESIAN_POINT('Ctrl Pts',(1.16601674699994,15.2,10.604787627));
#225820=CARTESIAN_POINT('Ctrl Pts',(1.16601674699994,11.6,10.604787627));
#225821=CARTESIAN_POINT('Ctrl Pts',(1.16569101699994,15.2,10.60708107));
#225822=CARTESIAN_POINT('Ctrl Pts',(1.16569101699994,11.6,10.60708107));
#225823=CARTESIAN_POINT('Ctrl Pts',(1.16536236599994,15.2,10.609380625));
#225824=CARTESIAN_POINT('Ctrl Pts',(1.16536236599994,11.6,10.609380625));
#225825=CARTESIAN_POINT('Ctrl Pts',(1.16503078499994,15.2,10.611686276));
#225826=CARTESIAN_POINT('Ctrl Pts',(1.16503078499994,11.6,10.611686276));
#225827=CARTESIAN_POINT('Ctrl Pts',(1.16469626699994,15.2,10.61399801));
#225828=CARTESIAN_POINT('Ctrl Pts',(1.16469626699994,11.6,10.61399801));
#225829=CARTESIAN_POINT('Ctrl Pts',(1.16435880199994,15.2,10.616315815));
#225830=CARTESIAN_POINT('Ctrl Pts',(1.16435880199994,11.6,10.616315815));
#225831=CARTESIAN_POINT('Ctrl Pts',(1.16401838399994,15.2,10.618639673));
#225832=CARTESIAN_POINT('Ctrl Pts',(1.16401838399994,11.6,10.618639673));
#225833=CARTESIAN_POINT('Ctrl Pts',(1.16367500499994,15.2,10.620969571));
#225834=CARTESIAN_POINT('Ctrl Pts',(1.16367500499994,11.6,10.620969571));
#225835=CARTESIAN_POINT('Ctrl Pts',(1.16332865499994,15.2,10.623305496));
#225836=CARTESIAN_POINT('Ctrl Pts',(1.16332865499994,11.6,10.623305496));
#225837=CARTESIAN_POINT('Ctrl Pts',(1.16297932699994,15.2,10.625647434));
#225838=CARTESIAN_POINT('Ctrl Pts',(1.16297932699994,11.6,10.625647434));
#225839=CARTESIAN_POINT('Ctrl Pts',(1.16262701499994,15.2,10.627995369));
#225840=CARTESIAN_POINT('Ctrl Pts',(1.16262701499994,11.6,10.627995369));
#225841=CARTESIAN_POINT('Ctrl Pts',(1.16227170899994,15.2,10.630349289));
#225842=CARTESIAN_POINT('Ctrl Pts',(1.16227170899994,11.6,10.630349289));
#225843=CARTESIAN_POINT('Ctrl Pts',(1.16191340199994,15.2,10.632709178));
#225844=CARTESIAN_POINT('Ctrl Pts',(1.16191340199994,11.6,10.632709178));
#225845=CARTESIAN_POINT('Ctrl Pts',(1.16155208699994,15.2,10.635075024));
#225846=CARTESIAN_POINT('Ctrl Pts',(1.16155208699994,11.6,10.635075024));
#225847=CARTESIAN_POINT('Ctrl Pts',(1.16118775499994,15.2,10.637446813));
#225848=CARTESIAN_POINT('Ctrl Pts',(1.16118775499994,11.6,10.637446813));
#225849=CARTESIAN_POINT('Ctrl Pts',(1.16082039799994,15.2,10.639824529));
#225850=CARTESIAN_POINT('Ctrl Pts',(1.16082039799994,11.6,10.639824529));
#225851=CARTESIAN_POINT('Ctrl Pts',(1.16045000999994,15.2,10.642208161));
#225852=CARTESIAN_POINT('Ctrl Pts',(1.16045000999994,11.6,10.642208161));
#225853=CARTESIAN_POINT('Ctrl Pts',(1.16007658299994,15.2,10.644597693));
#225854=CARTESIAN_POINT('Ctrl Pts',(1.16007658299994,11.6,10.644597693));
#225855=CARTESIAN_POINT('Ctrl Pts',(1.15970010799994,15.2,10.646993112));
#225856=CARTESIAN_POINT('Ctrl Pts',(1.15970010799994,11.6,10.646993112));
#225857=CARTESIAN_POINT('Ctrl Pts',(1.15932057899994,15.2,10.649394405));
#225858=CARTESIAN_POINT('Ctrl Pts',(1.15932057899994,11.6,10.649394405));
#225859=CARTESIAN_POINT('Ctrl Pts',(1.15893798699994,15.2,10.651801557));
#225860=CARTESIAN_POINT('Ctrl Pts',(1.15893798699994,11.6,10.651801557));
#225861=CARTESIAN_POINT('Ctrl Pts',(1.15855232599994,15.2,10.654214555));
#225862=CARTESIAN_POINT('Ctrl Pts',(1.15855232599994,11.6,10.654214555));
#225863=CARTESIAN_POINT('Ctrl Pts',(1.15816358799994,15.2,10.656633385));
#225864=CARTESIAN_POINT('Ctrl Pts',(1.15816358799994,11.6,10.656633385));
#225865=CARTESIAN_POINT('Ctrl Pts',(1.15777176599994,15.2,10.659058034));
#225866=CARTESIAN_POINT('Ctrl Pts',(1.15777176599994,11.6,10.659058034));
#225867=CARTESIAN_POINT('Ctrl Pts',(1.15737685099994,15.2,10.661488488));
#225868=CARTESIAN_POINT('Ctrl Pts',(1.15737685099994,11.6,10.661488488));
#225869=CARTESIAN_POINT('Ctrl Pts',(1.15697883699994,15.2,10.663924734));
#225870=CARTESIAN_POINT('Ctrl Pts',(1.15697883699994,11.6,10.663924734));
#225871=CARTESIAN_POINT('Ctrl Pts',(1.15657771599994,15.2,10.666366756));
#225872=CARTESIAN_POINT('Ctrl Pts',(1.15657771599994,11.6,10.666366756));
#225873=CARTESIAN_POINT('Ctrl Pts',(1.15617348099994,15.2,10.668814545));
#225874=CARTESIAN_POINT('Ctrl Pts',(1.15617348099994,11.6,10.668814545));
#225875=CARTESIAN_POINT('Ctrl Pts',(1.15576612399995,15.2,10.671268084));
#225876=CARTESIAN_POINT('Ctrl Pts',(1.15576612399995,11.6,10.671268084));
#225877=CARTESIAN_POINT('Ctrl Pts',(1.15535563899994,15.2,10.67372736));
#225878=CARTESIAN_POINT('Ctrl Pts',(1.15535563899994,11.6,10.67372736));
#225879=CARTESIAN_POINT('Ctrl Pts',(1.15494201899994,15.2,10.676192361));
#225880=CARTESIAN_POINT('Ctrl Pts',(1.15494201899994,11.6,10.676192361));
#225881=CARTESIAN_POINT('Ctrl Pts',(1.15452525499994,15.2,10.678663074));
#225882=CARTESIAN_POINT('Ctrl Pts',(1.15452525499994,11.6,10.678663074));
#225883=CARTESIAN_POINT('Ctrl Pts',(1.15410534099994,15.2,10.681139484));
#225884=CARTESIAN_POINT('Ctrl Pts',(1.15410534099994,11.6,10.681139484));
#225885=CARTESIAN_POINT('Ctrl Pts',(1.15368226999994,15.2,10.683621578));
#225886=CARTESIAN_POINT('Ctrl Pts',(1.15368226999994,11.6,10.683621578));
#225887=CARTESIAN_POINT('Ctrl Pts',(1.15325603399994,15.2,10.686109343));
#225888=CARTESIAN_POINT('Ctrl Pts',(1.15325603399994,11.6,10.686109343));
#225889=CARTESIAN_POINT('Ctrl Pts',(1.15282662699994,15.2,10.688602766));
#225890=CARTESIAN_POINT('Ctrl Pts',(1.15282662699994,11.6,10.688602766));
#225891=CARTESIAN_POINT('Ctrl Pts',(1.15239403999994,15.2,10.691101834));
#225892=CARTESIAN_POINT('Ctrl Pts',(1.15239403999994,11.6,10.691101834));
#225893=CARTESIAN_POINT('Ctrl Pts',(1.15195826899994,15.2,10.693606533));
#225894=CARTESIAN_POINT('Ctrl Pts',(1.15195826899994,11.6,10.693606533));
#225895=CARTESIAN_POINT('Ctrl Pts',(1.15151930399994,15.2,10.696116851));
#225896=CARTESIAN_POINT('Ctrl Pts',(1.15151930399994,11.6,10.696116851));
#225897=CARTESIAN_POINT('Ctrl Pts',(1.15107714099994,15.2,10.698632774));
#225898=CARTESIAN_POINT('Ctrl Pts',(1.15107714099994,11.6,10.698632774));
#225899=CARTESIAN_POINT('Ctrl Pts',(1.15063176999994,15.2,10.701154289));
#225900=CARTESIAN_POINT('Ctrl Pts',(1.15063176999994,11.6,10.701154289));
#225901=CARTESIAN_POINT('Ctrl Pts',(1.15018318599994,15.2,10.703681383));
#225902=CARTESIAN_POINT('Ctrl Pts',(1.15018318599994,11.6,10.703681383));
#225903=CARTESIAN_POINT('Ctrl Pts',(1.14973138199994,15.2,10.706214044));
#225904=CARTESIAN_POINT('Ctrl Pts',(1.14973138199994,11.6,10.706214044));
#225905=CARTESIAN_POINT('Ctrl Pts',(1.14927634999994,15.2,10.708752258));
#225906=CARTESIAN_POINT('Ctrl Pts',(1.14927634999994,11.6,10.708752258));
#225907=CARTESIAN_POINT('Ctrl Pts',(1.14881808499994,15.2,10.711296011));
#225908=CARTESIAN_POINT('Ctrl Pts',(1.14881808499994,11.6,10.711296011));
#225909=CARTESIAN_POINT('Ctrl Pts',(1.14835657799994,15.2,10.713845293));
#225910=CARTESIAN_POINT('Ctrl Pts',(1.14835657799994,11.6,10.713845293));
#225911=CARTESIAN_POINT('Ctrl Pts',(1.14789182399994,15.2,10.716400089));
#225912=CARTESIAN_POINT('Ctrl Pts',(1.14789182399994,11.6,10.716400089));
#225913=CARTESIAN_POINT('Ctrl Pts',(1.14742381599994,15.2,10.718960386));
#225914=CARTESIAN_POINT('Ctrl Pts',(1.14742381599994,11.6,10.718960386));
#225915=CARTESIAN_POINT('Ctrl Pts',(1.14695254499994,15.2,10.721526172));
#225916=CARTESIAN_POINT('Ctrl Pts',(1.14695254499994,11.6,10.721526172));
#225917=CARTESIAN_POINT('Ctrl Pts',(1.14647800799994,15.2,10.724097434));
#225918=CARTESIAN_POINT('Ctrl Pts',(1.14647800799994,11.6,10.724097434));
#225919=CARTESIAN_POINT('Ctrl Pts',(1.14600019599994,15.2,10.726674159));
#225920=CARTESIAN_POINT('Ctrl Pts',(1.14600019599994,11.6,10.726674159));
#225921=CARTESIAN_POINT('Ctrl Pts',(1.14551910299994,15.2,10.729256335));
#225922=CARTESIAN_POINT('Ctrl Pts',(1.14551910299994,11.6,10.729256335));
#225923=CARTESIAN_POINT('Ctrl Pts',(1.14503472199994,15.2,10.731843948));
#225924=CARTESIAN_POINT('Ctrl Pts',(1.14503472199994,11.6,10.731843948));
#225925=CARTESIAN_POINT('Ctrl Pts',(1.14454704599994,15.2,10.734436985));
#225926=CARTESIAN_POINT('Ctrl Pts',(1.14454704599994,11.6,10.734436985));
#225927=CARTESIAN_POINT('Ctrl Pts',(1.14405606999994,15.2,10.737035436));
#225928=CARTESIAN_POINT('Ctrl Pts',(1.14405606999994,11.6,10.737035436));
#225929=CARTESIAN_POINT('Ctrl Pts',(1.14356178599994,15.2,10.739639287));
#225930=CARTESIAN_POINT('Ctrl Pts',(1.14356178599994,11.6,10.739639287));
#225931=CARTESIAN_POINT('Ctrl Pts',(1.14306418799994,15.2,10.742248524));
#225932=CARTESIAN_POINT('Ctrl Pts',(1.14306418799994,11.6,10.742248524));
#225933=CARTESIAN_POINT('Ctrl Pts',(1.14256327099994,15.2,10.744863136));
#225934=CARTESIAN_POINT('Ctrl Pts',(1.14256327099994,11.6,10.744863136));
#225935=CARTESIAN_POINT('Ctrl Pts',(1.14205902599994,15.2,10.74748311));
#225936=CARTESIAN_POINT('Ctrl Pts',(1.14205902599994,11.6,10.74748311));
#225937=CARTESIAN_POINT('Ctrl Pts',(1.14155144699994,15.2,10.750108434));
#225938=CARTESIAN_POINT('Ctrl Pts',(1.14155144699994,11.6,10.750108434));
#225939=CARTESIAN_POINT('Ctrl Pts',(1.14104052899994,15.2,10.752739094));
#225940=CARTESIAN_POINT('Ctrl Pts',(1.14104052899994,11.6,10.752739094));
#225941=CARTESIAN_POINT('Ctrl Pts',(1.14052626499994,15.2,10.755375079));
#225942=CARTESIAN_POINT('Ctrl Pts',(1.14052626499994,11.6,10.755375079));
#225943=CARTESIAN_POINT('Ctrl Pts',(1.14000864799994,15.2,10.758016376));
#225944=CARTESIAN_POINT('Ctrl Pts',(1.14000864799994,11.6,10.758016376));
#225945=CARTESIAN_POINT('Ctrl Pts',(1.13948767199994,15.2,10.760662973));
#225946=CARTESIAN_POINT('Ctrl Pts',(1.13948767199994,11.6,10.760662973));
#225947=CARTESIAN_POINT('Ctrl Pts',(1.13896333099994,15.2,10.763314857));
#225948=CARTESIAN_POINT('Ctrl Pts',(1.13896333099994,11.6,10.763314857));
#225949=CARTESIAN_POINT('Ctrl Pts',(1.13843561899994,15.2,10.765972015));
#225950=CARTESIAN_POINT('Ctrl Pts',(1.13843561899994,11.6,10.765972015));
#225951=CARTESIAN_POINT('Ctrl Pts',(1.13790452899994,15.2,10.768634437));
#225952=CARTESIAN_POINT('Ctrl Pts',(1.13790452899994,11.6,10.768634437));
#225953=CARTESIAN_POINT('Ctrl Pts',(1.13737005499994,15.2,10.771302109));
#225954=CARTESIAN_POINT('Ctrl Pts',(1.13737005499994,11.6,10.771302109));
#225955=CARTESIAN_POINT('Ctrl Pts',(1.13683219099994,15.2,10.773975018));
#225956=CARTESIAN_POINT('Ctrl Pts',(1.13683219099994,11.6,10.773975018));
#225957=CARTESIAN_POINT('Ctrl Pts',(1.13629093099994,15.2,10.776653154));
#225958=CARTESIAN_POINT('Ctrl Pts',(1.13629093099994,11.6,10.776653154));
#225959=CARTESIAN_POINT('Ctrl Pts',(1.13574626799994,15.2,10.779336503));
#225960=CARTESIAN_POINT('Ctrl Pts',(1.13574626799994,11.6,10.779336503));
#225961=CARTESIAN_POINT('Ctrl Pts',(1.13519819699994,15.2,10.782025053));
#225962=CARTESIAN_POINT('Ctrl Pts',(1.13519819699994,11.6,10.782025053));
#225963=CARTESIAN_POINT('Ctrl Pts',(1.13464671099994,15.2,10.784718793));
#225964=CARTESIAN_POINT('Ctrl Pts',(1.13464671099994,11.6,10.784718793));
#225965=CARTESIAN_POINT('Ctrl Pts',(1.13409180399994,15.2,10.787417709));
#225966=CARTESIAN_POINT('Ctrl Pts',(1.13409180399994,11.6,10.787417709));
#225967=CARTESIAN_POINT('Ctrl Pts',(1.13353346999994,15.2,10.790121791));
#225968=CARTESIAN_POINT('Ctrl Pts',(1.13353346999994,11.6,10.790121791));
#225969=CARTESIAN_POINT('Ctrl Pts',(1.13297170399994,15.2,10.792831025));
#225970=CARTESIAN_POINT('Ctrl Pts',(1.13297170399994,11.6,10.792831025));
#225971=CARTESIAN_POINT('Ctrl Pts',(1.13240649799994,15.2,10.7955454));
#225972=CARTESIAN_POINT('Ctrl Pts',(1.13240649799994,11.6,10.7955454));
#225973=CARTESIAN_POINT('Ctrl Pts',(1.13183784799994,15.2,10.798264905));
#225974=CARTESIAN_POINT('Ctrl Pts',(1.13183784799994,11.6,10.798264905));
#225975=CARTESIAN_POINT('Ctrl Pts',(1.13126574599994,15.2,10.800989525));
#225976=CARTESIAN_POINT('Ctrl Pts',(1.13126574599994,11.6,10.800989525));
#225977=CARTESIAN_POINT('Ctrl Pts',(1.13069018799994,15.2,10.803719251));
#225978=CARTESIAN_POINT('Ctrl Pts',(1.13069018799994,11.6,10.803719251));
#225979=CARTESIAN_POINT('Ctrl Pts',(1.13011116699994,15.2,10.806454068));
#225980=CARTESIAN_POINT('Ctrl Pts',(1.13011116699994,11.6,10.806454068));
#225981=CARTESIAN_POINT('Ctrl Pts',(1.12952867699994,15.2,10.809193967));
#225982=CARTESIAN_POINT('Ctrl Pts',(1.12952867699994,11.6,10.809193967));
#225983=CARTESIAN_POINT('Ctrl Pts',(1.12894271299994,15.2,10.811938934));
#225984=CARTESIAN_POINT('Ctrl Pts',(1.12894271299994,11.6,10.811938934));
#225985=CARTESIAN_POINT('Ctrl Pts',(1.12835326899994,15.2,10.814688958));
#225986=CARTESIAN_POINT('Ctrl Pts',(1.12835326899994,11.6,10.814688958));
#225987=CARTESIAN_POINT('Ctrl Pts',(1.12776033799994,15.2,10.817444028));
#225988=CARTESIAN_POINT('Ctrl Pts',(1.12776033799994,11.6,10.817444028));
#225989=CARTESIAN_POINT('Ctrl Pts',(1.12716391599994,15.2,10.820204131));
#225990=CARTESIAN_POINT('Ctrl Pts',(1.12716391599994,11.6,10.820204131));
#225991=CARTESIAN_POINT('Ctrl Pts',(1.12656399599994,15.2,10.822969256));
#225992=CARTESIAN_POINT('Ctrl Pts',(1.12656399599994,11.6,10.822969256));
#225993=CARTESIAN_POINT('Ctrl Pts',(1.12596057199994,15.2,10.825739389));
#225994=CARTESIAN_POINT('Ctrl Pts',(1.12596057199994,11.6,10.825739389));
#225995=CARTESIAN_POINT('Ctrl Pts',(1.12535363899994,15.2,10.828514521));
#225996=CARTESIAN_POINT('Ctrl Pts',(1.12535363899994,11.6,10.828514521));
#225997=CARTESIAN_POINT('Ctrl Pts',(1.12474319099995,15.2,10.831294639));
#225998=CARTESIAN_POINT('Ctrl Pts',(1.12474319099995,11.6,10.831294639));
#225999=CARTESIAN_POINT('Ctrl Pts',(1.12412922199994,15.2,10.834079731));
#226000=CARTESIAN_POINT('Ctrl Pts',(1.12412922199994,11.6,10.834079731));
#226001=CARTESIAN_POINT('Ctrl Pts',(1.12351172699994,15.2,10.836869786));
#226002=CARTESIAN_POINT('Ctrl Pts',(1.12351172699994,11.6,10.836869786));
#226003=CARTESIAN_POINT('Ctrl Pts',(1.12289069999994,15.2,10.839664792));
#226004=CARTESIAN_POINT('Ctrl Pts',(1.12289069999994,11.6,10.839664792));
#226005=CARTESIAN_POINT('Ctrl Pts',(1.12226613599994,15.2,10.842464738));
#226006=CARTESIAN_POINT('Ctrl Pts',(1.12226613599994,11.6,10.842464738));
#226007=CARTESIAN_POINT('Ctrl Pts',(1.12163802699994,15.2,10.84526961));
#226008=CARTESIAN_POINT('Ctrl Pts',(1.12163802699994,11.6,10.84526961));
#226009=CARTESIAN_POINT('Ctrl Pts',(1.12100637099994,15.2,10.848079399));
#226010=CARTESIAN_POINT('Ctrl Pts',(1.12100637099994,11.6,10.848079399));
#226011=CARTESIAN_POINT('Ctrl Pts',(1.12037115999994,15.2,10.850894093));
#226012=CARTESIAN_POINT('Ctrl Pts',(1.12037115999994,11.6,10.850894093));
#226013=CARTESIAN_POINT('Ctrl Pts',(1.11973238899994,15.2,10.85371368));
#226014=CARTESIAN_POINT('Ctrl Pts',(1.11973238899994,11.6,10.85371368));
#226015=CARTESIAN_POINT('Ctrl Pts',(1.11909005399994,15.2,10.856538148));
#226016=CARTESIAN_POINT('Ctrl Pts',(1.11909005399994,11.6,10.856538148));
#226017=CARTESIAN_POINT('Ctrl Pts',(1.11844414599994,15.2,10.859367487));
#226018=CARTESIAN_POINT('Ctrl Pts',(1.11844414599994,11.6,10.859367487));
#226019=CARTESIAN_POINT('Ctrl Pts',(1.11779466299994,15.2,10.862201683));
#226020=CARTESIAN_POINT('Ctrl Pts',(1.11779466299994,11.6,10.862201683));
#226021=CARTESIAN_POINT('Ctrl Pts',(1.11714159699994,15.2,10.865040727));
#226022=CARTESIAN_POINT('Ctrl Pts',(1.11714159699994,11.6,10.865040727));
#226023=CARTESIAN_POINT('Ctrl Pts',(1.11648494499994,15.2,10.867884606));
#226024=CARTESIAN_POINT('Ctrl Pts',(1.11648494499994,11.6,10.867884606));
#226025=CARTESIAN_POINT('Ctrl Pts',(1.11582469999994,15.2,10.870733309));
#226026=CARTESIAN_POINT('Ctrl Pts',(1.11582469999994,11.6,10.870733309));
#226027=CARTESIAN_POINT('Ctrl Pts',(1.11516085699994,15.2,10.873586825));
#226028=CARTESIAN_POINT('Ctrl Pts',(1.11516085699994,11.6,10.873586825));
#226029=CARTESIAN_POINT('Ctrl Pts',(1.11449341099994,15.2,10.876445142));
#226030=CARTESIAN_POINT('Ctrl Pts',(1.11449341099994,11.6,10.876445142));
#226031=CARTESIAN_POINT('Ctrl Pts',(1.11382235499994,15.2,10.879308249));
#226032=CARTESIAN_POINT('Ctrl Pts',(1.11382235499994,11.6,10.879308249));
#226033=CARTESIAN_POINT('Ctrl Pts',(1.11314768699994,15.2,10.882176136));
#226034=CARTESIAN_POINT('Ctrl Pts',(1.11314768699994,11.6,10.882176136));
#226035=CARTESIAN_POINT('Ctrl Pts',(1.11246939799994,15.2,10.885048788));
#226036=CARTESIAN_POINT('Ctrl Pts',(1.11246939799994,11.6,10.885048788));
#226037=CARTESIAN_POINT('Ctrl Pts',(1.11178748599994,15.2,10.887926198));
#226038=CARTESIAN_POINT('Ctrl Pts',(1.11178748599994,11.6,10.887926198));
#226039=CARTESIAN_POINT('Ctrl Pts',(1.11110194299994,15.2,10.890808352));
#226040=CARTESIAN_POINT('Ctrl Pts',(1.11110194299994,11.6,10.890808352));
#226041=CARTESIAN_POINT('Ctrl Pts',(1.11041276399995,15.2,10.89369524));
#226042=CARTESIAN_POINT('Ctrl Pts',(1.11041276399995,11.6,10.89369524));
#226043=CARTESIAN_POINT('Ctrl Pts',(1.10971994499994,15.2,10.89658685));
#226044=CARTESIAN_POINT('Ctrl Pts',(1.10971994499994,11.6,10.89658685));
#226045=CARTESIAN_POINT('Ctrl Pts',(1.10902348199994,15.2,10.899483171));
#226046=CARTESIAN_POINT('Ctrl Pts',(1.10902348199994,11.6,10.899483171));
#226047=CARTESIAN_POINT('Ctrl Pts',(1.10832336799994,15.2,10.902384192));
#226048=CARTESIAN_POINT('Ctrl Pts',(1.10832336799994,11.6,10.902384192));
#226049=CARTESIAN_POINT('Ctrl Pts',(1.10761959699994,15.2,10.905289901));
#226050=CARTESIAN_POINT('Ctrl Pts',(1.10761959699994,11.6,10.905289901));
#226051=CARTESIAN_POINT('Ctrl Pts',(1.10691216499994,15.2,10.908200289));
#226052=CARTESIAN_POINT('Ctrl Pts',(1.10691216499994,11.6,10.908200289));
#226053=CARTESIAN_POINT('Ctrl Pts',(1.10620106799994,15.2,10.911115343));
#226054=CARTESIAN_POINT('Ctrl Pts',(1.10620106799994,11.6,10.911115343));
#226055=CARTESIAN_POINT('Ctrl Pts',(1.10548629899994,15.2,10.914035053));
#226056=CARTESIAN_POINT('Ctrl Pts',(1.10548629899994,11.6,10.914035053));
#226057=CARTESIAN_POINT('Ctrl Pts',(1.10476785399995,15.2,10.916959407));
#226058=CARTESIAN_POINT('Ctrl Pts',(1.10476785399995,11.6,10.916959407));
#226059=CARTESIAN_POINT('Ctrl Pts',(1.10404572799994,15.2,10.919888394));
#226060=CARTESIAN_POINT('Ctrl Pts',(1.10404572799994,11.6,10.919888394));
#226061=CARTESIAN_POINT('Ctrl Pts',(1.10331991399994,15.2,10.922822003));
#226062=CARTESIAN_POINT('Ctrl Pts',(1.10331991399994,11.6,10.922822003));
#226063=CARTESIAN_POINT('Ctrl Pts',(1.10259040999994,15.2,10.925760224));
#226064=CARTESIAN_POINT('Ctrl Pts',(1.10259040999994,11.6,10.925760224));
#226065=CARTESIAN_POINT('Ctrl Pts',(1.10185720999994,15.2,10.928703045));
#226066=CARTESIAN_POINT('Ctrl Pts',(1.10185720999994,11.6,10.928703045));
#226067=CARTESIAN_POINT('Ctrl Pts',(1.10112030699994,15.2,10.931650455));
#226068=CARTESIAN_POINT('Ctrl Pts',(1.10112030699994,11.6,10.931650455));
#226069=CARTESIAN_POINT('Ctrl Pts',(1.10037969999994,15.2,10.934602444));
#226070=CARTESIAN_POINT('Ctrl Pts',(1.10037969999994,11.6,10.934602444));
#226071=CARTESIAN_POINT('Ctrl Pts',(1.09963537999994,15.2,10.937559));
#226072=CARTESIAN_POINT('Ctrl Pts',(1.09963537999994,11.6,10.937559));
#226073=CARTESIAN_POINT('Ctrl Pts',(1.09888734499994,15.2,10.940520113));
#226074=CARTESIAN_POINT('Ctrl Pts',(1.09888734499994,11.6,10.940520113));
#226075=CARTESIAN_POINT('Ctrl Pts',(1.09813558699994,15.2,10.943485772));
#226076=CARTESIAN_POINT('Ctrl Pts',(1.09813558699994,11.6,10.943485772));
#226077=CARTESIAN_POINT('Ctrl Pts',(1.09738010399994,15.2,10.946455965));
#226078=CARTESIAN_POINT('Ctrl Pts',(1.09738010399994,11.6,10.946455965));
#226079=CARTESIAN_POINT('Ctrl Pts',(1.09662089099994,15.2,10.949430682));
#226080=CARTESIAN_POINT('Ctrl Pts',(1.09662089099994,11.6,10.949430682));
#226081=CARTESIAN_POINT('Ctrl Pts',(1.09585794199994,15.2,10.952409912));
#226082=CARTESIAN_POINT('Ctrl Pts',(1.09585794199994,11.6,10.952409912));
#226083=CARTESIAN_POINT('Ctrl Pts',(1.09509125199994,15.2,10.955393644));
#226084=CARTESIAN_POINT('Ctrl Pts',(1.09509125199994,11.6,10.955393644));
#226085=CARTESIAN_POINT('Ctrl Pts',(1.09432081599994,15.2,10.958381869));
#226086=CARTESIAN_POINT('Ctrl Pts',(1.09432081599994,11.6,10.958381869));
#226087=CARTESIAN_POINT('Ctrl Pts',(1.09354663099994,15.2,10.961374573));
#226088=CARTESIAN_POINT('Ctrl Pts',(1.09354663099994,11.6,10.961374573));
#226089=CARTESIAN_POINT('Ctrl Pts',(1.09276869099994,15.2,10.964371748));
#226090=CARTESIAN_POINT('Ctrl Pts',(1.09276869099994,11.6,10.964371748));
#226091=CARTESIAN_POINT('Ctrl Pts',(1.09198699099994,15.2,10.967373382));
#226092=CARTESIAN_POINT('Ctrl Pts',(1.09198699099994,11.6,10.967373382));
#226093=CARTESIAN_POINT('Ctrl Pts',(1.09120152699994,15.2,10.970379465));
#226094=CARTESIAN_POINT('Ctrl Pts',(1.09120152699994,11.6,10.970379465));
#226095=CARTESIAN_POINT('Ctrl Pts',(1.09041229399994,15.2,10.973389986));
#226096=CARTESIAN_POINT('Ctrl Pts',(1.09041229399994,11.6,10.973389986));
#226097=CARTESIAN_POINT('Ctrl Pts',(1.08961928699994,15.2,10.976404933));
#226098=CARTESIAN_POINT('Ctrl Pts',(1.08961928699994,11.6,10.976404933));
#226099=CARTESIAN_POINT('Ctrl Pts',(1.08882250299994,15.2,10.979424298));
#226100=CARTESIAN_POINT('Ctrl Pts',(1.08882250299994,11.6,10.979424298));
#226101=CARTESIAN_POINT('Ctrl Pts',(1.08802193399994,15.2,10.982448068));
#226102=CARTESIAN_POINT('Ctrl Pts',(1.08802193399994,11.6,10.982448068));
#226103=CARTESIAN_POINT('Ctrl Pts',(1.08721757799994,15.2,10.985476233));
#226104=CARTESIAN_POINT('Ctrl Pts',(1.08721757799994,11.6,10.985476233));
#226105=CARTESIAN_POINT('Ctrl Pts',(1.08640942899994,15.2,10.988508784));
#226106=CARTESIAN_POINT('Ctrl Pts',(1.08640942899994,11.6,10.988508784));
#226107=CARTESIAN_POINT('Ctrl Pts',(1.08559748399994,15.2,10.991545709));
#226108=CARTESIAN_POINT('Ctrl Pts',(1.08559748399994,11.6,10.991545709));
#226109=CARTESIAN_POINT('Ctrl Pts',(1.08478173699994,15.2,10.994586997));
#226110=CARTESIAN_POINT('Ctrl Pts',(1.08478173699994,11.6,10.994586997));
#226111=CARTESIAN_POINT('Ctrl Pts',(1.08396218399994,15.2,10.997632638));
#226112=CARTESIAN_POINT('Ctrl Pts',(1.08396218399994,11.6,10.997632638));
#226113=CARTESIAN_POINT('Ctrl Pts',(1.08313882099994,15.2,11.000682622));
#226114=CARTESIAN_POINT('Ctrl Pts',(1.08313882099994,11.6,11.000682622));
#226115=CARTESIAN_POINT('Ctrl Pts',(1.08231164199994,15.2,11.003736938));
#226116=CARTESIAN_POINT('Ctrl Pts',(1.08231164199994,11.6,11.003736938));
#226117=CARTESIAN_POINT('Ctrl Pts',(1.08148064399994,15.2,11.006795575));
#226118=CARTESIAN_POINT('Ctrl Pts',(1.08148064399994,11.6,11.006795575));
#226119=CARTESIAN_POINT('Ctrl Pts',(1.08064582099994,15.2,11.009858524));
#226120=CARTESIAN_POINT('Ctrl Pts',(1.08064582099994,11.6,11.009858524));
#226121=CARTESIAN_POINT('Ctrl Pts',(1.07980716999994,15.2,11.012925773));
#226122=CARTESIAN_POINT('Ctrl Pts',(1.07980716999994,11.6,11.012925773));
#226123=CARTESIAN_POINT('Ctrl Pts',(1.07896468599994,15.2,11.015997312));
#226124=CARTESIAN_POINT('Ctrl Pts',(1.07896468599994,11.6,11.015997312));
#226125=CARTESIAN_POINT('Ctrl Pts',(1.07811836399994,15.2,11.019073132));
#226126=CARTESIAN_POINT('Ctrl Pts',(1.07811836399994,11.6,11.019073132));
#226127=CARTESIAN_POINT('Ctrl Pts',(1.07726819999994,15.2,11.022153221));
#226128=CARTESIAN_POINT('Ctrl Pts',(1.07726819999994,11.6,11.022153221));
#226129=CARTESIAN_POINT('Ctrl Pts',(1.07641418999994,15.2,11.025237569));
#226130=CARTESIAN_POINT('Ctrl Pts',(1.07641418999994,11.6,11.025237569));
#226131=CARTESIAN_POINT('Ctrl Pts',(1.07555632999994,15.2,11.028326166));
#226132=CARTESIAN_POINT('Ctrl Pts',(1.07555632999994,11.6,11.028326166));
#226133=CARTESIAN_POINT('Ctrl Pts',(1.07469461299994,15.2,11.031419001));
#226134=CARTESIAN_POINT('Ctrl Pts',(1.07469461299994,11.6,11.031419001));
#226135=CARTESIAN_POINT('Ctrl Pts',(1.07382903699994,15.2,11.034516064));
#226136=CARTESIAN_POINT('Ctrl Pts',(1.07382903699994,11.6,11.034516064));
#226137=CARTESIAN_POINT('Ctrl Pts',(1.07295959799994,15.2,11.037617346));
#226138=CARTESIAN_POINT('Ctrl Pts',(1.07295959799994,11.6,11.037617346));
#226139=CARTESIAN_POINT('Ctrl Pts',(1.07208628999994,15.2,11.040722834));
#226140=CARTESIAN_POINT('Ctrl Pts',(1.07208628999994,11.6,11.040722834));
#226141=CARTESIAN_POINT('Ctrl Pts',(1.07120910999994,15.2,11.043832521));
#226142=CARTESIAN_POINT('Ctrl Pts',(1.07120910999994,11.6,11.043832521));
#226143=CARTESIAN_POINT('Ctrl Pts',(1.07032805399994,15.2,11.046946393));
#226144=CARTESIAN_POINT('Ctrl Pts',(1.07032805399994,11.6,11.046946393));
#226145=CARTESIAN_POINT('Ctrl Pts',(1.06944311599994,15.2,11.050064443));
#226146=CARTESIAN_POINT('Ctrl Pts',(1.06944311599994,11.6,11.050064443));
#226147=CARTESIAN_POINT('Ctrl Pts',(1.06855429299994,15.2,11.05318666));
#226148=CARTESIAN_POINT('Ctrl Pts',(1.06855429299994,11.6,11.05318666));
#226149=CARTESIAN_POINT('Ctrl Pts',(1.06766158099994,15.2,11.056313033));
#226150=CARTESIAN_POINT('Ctrl Pts',(1.06766158099994,11.6,11.056313033));
#226151=CARTESIAN_POINT('Ctrl Pts',(1.06676497399994,15.2,11.059443552));
#226152=CARTESIAN_POINT('Ctrl Pts',(1.06676497399994,11.6,11.059443552));
#226153=CARTESIAN_POINT('Ctrl Pts',(1.06586446999994,15.2,11.062578207));
#226154=CARTESIAN_POINT('Ctrl Pts',(1.06586446999994,11.6,11.062578207));
#226155=CARTESIAN_POINT('Ctrl Pts',(1.06496006399994,15.2,11.065716989));
#226156=CARTESIAN_POINT('Ctrl Pts',(1.06496006399994,11.6,11.065716989));
#226157=CARTESIAN_POINT('Ctrl Pts',(1.06405175099994,15.2,11.068859885));
#226158=CARTESIAN_POINT('Ctrl Pts',(1.06405175099994,11.6,11.068859885));
#226159=CARTESIAN_POINT('Ctrl Pts',(1.06313952799994,15.2,11.072006888));
#226160=CARTESIAN_POINT('Ctrl Pts',(1.06313952799994,11.6,11.072006888));
#226161=CARTESIAN_POINT('Ctrl Pts',(1.06222338999994,15.2,11.075157987));
#226162=CARTESIAN_POINT('Ctrl Pts',(1.06222338999994,11.6,11.075157987));
#226163=CARTESIAN_POINT('Ctrl Pts',(1.06130333399994,15.2,11.078313171));
#226164=CARTESIAN_POINT('Ctrl Pts',(1.06130333399994,11.6,11.078313171));
#226165=CARTESIAN_POINT('Ctrl Pts',(1.06037935499994,15.2,11.081472431));
#226166=CARTESIAN_POINT('Ctrl Pts',(1.06037935499994,11.6,11.081472431));
#226167=CARTESIAN_POINT('Ctrl Pts',(1.05945144799994,15.2,11.084635756));
#226168=CARTESIAN_POINT('Ctrl Pts',(1.05945144799994,11.6,11.084635756));
#226169=CARTESIAN_POINT('Ctrl Pts',(1.05851961199994,15.2,11.087803136));
#226170=CARTESIAN_POINT('Ctrl Pts',(1.05851961199994,11.6,11.087803136));
#226171=CARTESIAN_POINT('Ctrl Pts',(1.05758383899994,15.2,11.090974562));
#226172=CARTESIAN_POINT('Ctrl Pts',(1.05758383899994,11.6,11.090974562));
#226173=CARTESIAN_POINT('Ctrl Pts',(1.05664412899994,15.2,11.094150023));
#226174=CARTESIAN_POINT('Ctrl Pts',(1.05664412899994,11.6,11.094150023));
#226175=CARTESIAN_POINT('Ctrl Pts',(1.05570047399994,15.2,11.097329511));
#226176=CARTESIAN_POINT('Ctrl Pts',(1.05570047399994,11.6,11.097329511));
#226177=CARTESIAN_POINT('Ctrl Pts',(1.05475287399994,15.2,11.100513013));
#226178=CARTESIAN_POINT('Ctrl Pts',(1.05475287399994,11.6,11.100513013));
#226179=CARTESIAN_POINT('Ctrl Pts',(1.05380132099994,15.2,11.103700521));
#226180=CARTESIAN_POINT('Ctrl Pts',(1.05380132099994,11.6,11.103700521));
#226181=CARTESIAN_POINT('Ctrl Pts',(1.05284581299994,15.2,11.106892026));
#226182=CARTESIAN_POINT('Ctrl Pts',(1.05284581299994,11.6,11.106892026));
#226183=CARTESIAN_POINT('Ctrl Pts',(1.05188634699994,15.2,11.110087516));
#226184=CARTESIAN_POINT('Ctrl Pts',(1.05188634699994,11.6,11.110087516));
#226185=CARTESIAN_POINT('Ctrl Pts',(1.05092291799994,15.2,11.113286982));
#226186=CARTESIAN_POINT('Ctrl Pts',(1.05092291799994,11.6,11.113286982));
#226187=CARTESIAN_POINT('Ctrl Pts',(1.04995552099994,15.2,11.116490413));
#226188=CARTESIAN_POINT('Ctrl Pts',(1.04995552099994,11.6,11.116490413));
#226189=CARTESIAN_POINT('Ctrl Pts',(1.04898415399994,15.2,11.119697801));
#226190=CARTESIAN_POINT('Ctrl Pts',(1.04898415399994,11.6,11.119697801));
#226191=CARTESIAN_POINT('Ctrl Pts',(1.04800881199994,15.2,11.122909136));
#226192=CARTESIAN_POINT('Ctrl Pts',(1.04800881199994,11.6,11.122909136));
#226193=CARTESIAN_POINT('Ctrl Pts',(1.04702949199994,15.2,11.126124407));
#226194=CARTESIAN_POINT('Ctrl Pts',(1.04702949199994,11.6,11.126124407));
#226195=CARTESIAN_POINT('Ctrl Pts',(1.04604618899994,15.2,11.129343605));
#226196=CARTESIAN_POINT('Ctrl Pts',(1.04604618899994,11.6,11.129343605));
#226197=CARTESIAN_POINT('Ctrl Pts',(1.04505889899994,15.2,11.13256672));
#226198=CARTESIAN_POINT('Ctrl Pts',(1.04505889899994,11.6,11.13256672));
#226199=CARTESIAN_POINT('Ctrl Pts',(1.04406761999994,15.2,11.135793742));
#226200=CARTESIAN_POINT('Ctrl Pts',(1.04406761999994,11.6,11.135793742));
#226201=CARTESIAN_POINT('Ctrl Pts',(1.04307234599994,15.2,11.139024661));
#226202=CARTESIAN_POINT('Ctrl Pts',(1.04307234599994,11.6,11.139024661));
#226203=CARTESIAN_POINT('Ctrl Pts',(1.04207307499994,15.2,11.142259469));
#226204=CARTESIAN_POINT('Ctrl Pts',(1.04207307499994,11.6,11.142259469));
#226205=CARTESIAN_POINT('Ctrl Pts',(1.04106980299994,15.2,11.145498154));
#226206=CARTESIAN_POINT('Ctrl Pts',(1.04106980299994,11.6,11.145498154));
#226207=CARTESIAN_POINT('Ctrl Pts',(1.04006252399994,15.2,11.148740708));
#226208=CARTESIAN_POINT('Ctrl Pts',(1.04006252399994,11.6,11.148740708));
#226209=CARTESIAN_POINT('Ctrl Pts',(1.03905123799994,15.2,11.15198712));
#226210=CARTESIAN_POINT('Ctrl Pts',(1.03905123799994,11.6,11.15198712));
#226211=CARTESIAN_POINT('Ctrl Pts',(1.03803593699994,15.2,11.15523738));
#226212=CARTESIAN_POINT('Ctrl Pts',(1.03803593699994,11.6,11.15523738));
#226213=CARTESIAN_POINT('Ctrl Pts',(1.03701662099994,15.2,11.158491481));
#226214=CARTESIAN_POINT('Ctrl Pts',(1.03701662099994,11.6,11.158491481));
#226215=CARTESIAN_POINT('Ctrl Pts',(1.03599328299994,15.2,11.161749411));
#226216=CARTESIAN_POINT('Ctrl Pts',(1.03599328299994,11.6,11.161749411));
#226217=CARTESIAN_POINT('Ctrl Pts',(1.03496592299994,15.2,11.165011161));
#226218=CARTESIAN_POINT('Ctrl Pts',(1.03496592299994,11.6,11.165011161));
#226219=CARTESIAN_POINT('Ctrl Pts',(1.03393453399994,15.2,11.168276721));
#226220=CARTESIAN_POINT('Ctrl Pts',(1.03393453399994,11.6,11.168276721));
#226221=CARTESIAN_POINT('Ctrl Pts',(1.03289911299994,15.2,11.171546082));
#226222=CARTESIAN_POINT('Ctrl Pts',(1.03289911299994,11.6,11.171546082));
#226223=CARTESIAN_POINT('Ctrl Pts',(1.03185965899994,15.2,11.174819234));
#226224=CARTESIAN_POINT('Ctrl Pts',(1.03185965899994,11.6,11.174819234));
#226225=CARTESIAN_POINT('Ctrl Pts',(1.03081616499994,15.2,11.178096167));
#226226=CARTESIAN_POINT('Ctrl Pts',(1.03081616499994,11.6,11.178096167));
#226227=CARTESIAN_POINT('Ctrl Pts',(1.02976862899994,15.2,11.181376874));
#226228=CARTESIAN_POINT('Ctrl Pts',(1.02976862899994,11.6,11.181376874));
#226229=CARTESIAN_POINT('Ctrl Pts',(1.02871704699994,15.2,11.184661342));
#226230=CARTESIAN_POINT('Ctrl Pts',(1.02871704699994,11.6,11.184661342));
#226231=CARTESIAN_POINT('Ctrl Pts',(1.02766141499994,15.2,11.187949564));
#226232=CARTESIAN_POINT('Ctrl Pts',(1.02766141499994,11.6,11.187949564));
#226233=CARTESIAN_POINT('Ctrl Pts',(1.02660172999994,15.2,11.191241528));
#226234=CARTESIAN_POINT('Ctrl Pts',(1.02660172999994,11.6,11.191241528));
#226235=CARTESIAN_POINT('Ctrl Pts',(1.02553798899994,15.2,11.194537227));
#226236=CARTESIAN_POINT('Ctrl Pts',(1.02553798899994,11.6,11.194537227));
#226237=CARTESIAN_POINT('Ctrl Pts',(1.02447018799994,15.2,11.19783665));
#226238=CARTESIAN_POINT('Ctrl Pts',(1.02447018799994,11.6,11.19783665));
#226239=CARTESIAN_POINT('Ctrl Pts',(1.02339832299994,15.2,11.201139789));
#226240=CARTESIAN_POINT('Ctrl Pts',(1.02339832299994,11.6,11.201139789));
#226241=CARTESIAN_POINT('Ctrl Pts',(1.02232238999994,15.2,11.204446633));
#226242=CARTESIAN_POINT('Ctrl Pts',(1.02232238999994,11.6,11.204446633));
#226243=CARTESIAN_POINT('Ctrl Pts',(1.02124238599994,15.2,11.207757173));
#226244=CARTESIAN_POINT('Ctrl Pts',(1.02124238599994,11.6,11.207757173));
#226245=CARTESIAN_POINT('Ctrl Pts',(1.02015830899994,15.2,11.2110714));
#226246=CARTESIAN_POINT('Ctrl Pts',(1.02015830899994,11.6,11.2110714));
#226247=CARTESIAN_POINT('Ctrl Pts',(1.01907015299994,15.2,11.214389305));
#226248=CARTESIAN_POINT('Ctrl Pts',(1.01907015299994,11.6,11.214389305));
#226249=CARTESIAN_POINT('Ctrl Pts',(1.01797791699994,15.2,11.217710876));
#226250=CARTESIAN_POINT('Ctrl Pts',(1.01797791699994,11.6,11.217710876));
#226251=CARTESIAN_POINT('Ctrl Pts',(1.01688159499994,15.2,11.221036107));
#226252=CARTESIAN_POINT('Ctrl Pts',(1.01688159499994,11.6,11.221036107));
#226253=CARTESIAN_POINT('Ctrl Pts',(1.01578118499994,15.2,11.224364988));
#226254=CARTESIAN_POINT('Ctrl Pts',(1.01578118499994,11.6,11.224364988));
#226255=CARTESIAN_POINT('Ctrl Pts',(1.01467668399994,15.2,11.227697508));
#226256=CARTESIAN_POINT('Ctrl Pts',(1.01467668399994,11.6,11.227697508));
#226257=CARTESIAN_POINT('Ctrl Pts',(1.01356808799994,15.2,11.231033658));
#226258=CARTESIAN_POINT('Ctrl Pts',(1.01356808799994,11.6,11.231033658));
#226259=CARTESIAN_POINT('Ctrl Pts',(1.01245539399994,15.2,11.23437343));
#226260=CARTESIAN_POINT('Ctrl Pts',(1.01245539399994,11.6,11.23437343));
#226261=CARTESIAN_POINT('Ctrl Pts',(1.01133859699994,15.2,11.237716814));
#226262=CARTESIAN_POINT('Ctrl Pts',(1.01133859699994,11.6,11.237716814));
#226263=CARTESIAN_POINT('Ctrl Pts',(1.01021769499994,15.2,11.2410638));
#226264=CARTESIAN_POINT('Ctrl Pts',(1.01021769499994,11.6,11.2410638));
#226265=CARTESIAN_POINT('Ctrl Pts',(1.00909268499994,15.2,11.244414379));
#226266=CARTESIAN_POINT('Ctrl Pts',(1.00909268499994,11.6,11.244414379));
#226267=CARTESIAN_POINT('Ctrl Pts',(1.00796356299994,15.2,11.247768542));
#226268=CARTESIAN_POINT('Ctrl Pts',(1.00796356299994,11.6,11.247768542));
#226269=CARTESIAN_POINT('Ctrl Pts',(1.00683032599994,15.2,11.251126281));
#226270=CARTESIAN_POINT('Ctrl Pts',(1.00683032599994,11.6,11.251126281));
#226271=CARTESIAN_POINT('Ctrl Pts',(1.00569296899994,15.2,11.254487586));
#226272=CARTESIAN_POINT('Ctrl Pts',(1.00569296899994,11.6,11.254487586));
#226273=CARTESIAN_POINT('Ctrl Pts',(1.00455149199994,15.2,11.257852446));
#226274=CARTESIAN_POINT('Ctrl Pts',(1.00455149199994,11.6,11.257852446));
#226275=CARTESIAN_POINT('Ctrl Pts',(1.00340588899994,15.2,11.261220854));
#226276=CARTESIAN_POINT('Ctrl Pts',(1.00340588899994,11.6,11.261220854));
#226277=CARTESIAN_POINT('Ctrl Pts',(1.00225615799994,15.2,11.2645928));
#226278=CARTESIAN_POINT('Ctrl Pts',(1.00225615799994,11.6,11.2645928));
#226279=CARTESIAN_POINT('Ctrl Pts',(1.00110229499994,15.2,11.267968273));
#226280=CARTESIAN_POINT('Ctrl Pts',(1.00110229499994,11.6,11.267968273));
#226281=CARTESIAN_POINT('Ctrl Pts',(0.999944296999944,15.2,11.271347268));
#226282=CARTESIAN_POINT('Ctrl Pts',(0.999944296999944,11.6,11.271347268));
#226283=CARTESIAN_POINT('Ctrl Pts',(0.998782160999945,15.2,11.274729773));
#226284=CARTESIAN_POINT('Ctrl Pts',(0.998782160999945,11.6,11.274729773));
#226285=CARTESIAN_POINT('Ctrl Pts',(0.997615883999944,15.2,11.278115779));
#226286=CARTESIAN_POINT('Ctrl Pts',(0.997615883999944,11.6,11.278115779));
#226287=CARTESIAN_POINT('Ctrl Pts',(0.996445460999944,15.2,11.281505278));
#226288=CARTESIAN_POINT('Ctrl Pts',(0.996445460999944,11.6,11.281505278));
#226289=CARTESIAN_POINT('Ctrl Pts',(0.995270891999944,15.2,11.284898259));
#226290=CARTESIAN_POINT('Ctrl Pts',(0.995270891999944,11.6,11.284898259));
#226291=CARTESIAN_POINT('Ctrl Pts',(0.994092170999944,15.2,11.288294714));
#226292=CARTESIAN_POINT('Ctrl Pts',(0.994092170999944,11.6,11.288294714));
#226293=CARTESIAN_POINT('Ctrl Pts',(0.992909295999944,15.2,11.291694635));
#226294=CARTESIAN_POINT('Ctrl Pts',(0.992909295999944,11.6,11.291694635));
#226295=CARTESIAN_POINT('Ctrl Pts',(0.991722263999945,15.2,11.295098011));
#226296=CARTESIAN_POINT('Ctrl Pts',(0.991722263999945,11.6,11.295098011));
#226297=CARTESIAN_POINT('Ctrl Pts',(0.990531070999944,15.2,11.298504835));
#226298=CARTESIAN_POINT('Ctrl Pts',(0.990531070999944,11.6,11.298504835));
#226299=CARTESIAN_POINT('Ctrl Pts',(0.989335713999945,15.2,11.301915096));
#226300=CARTESIAN_POINT('Ctrl Pts',(0.989335713999945,11.6,11.301915096));
#226301=CARTESIAN_POINT('Ctrl Pts',(0.988136190999944,15.2,11.305328786));
#226302=CARTESIAN_POINT('Ctrl Pts',(0.988136190999944,11.6,11.305328786));
#226303=CARTESIAN_POINT('Ctrl Pts',(0.986932497999944,15.2,11.308745896));
#226304=CARTESIAN_POINT('Ctrl Pts',(0.986932497999944,11.6,11.308745896));
#226305=CARTESIAN_POINT('Ctrl Pts',(0.985724631999945,15.2,11.312166416));
#226306=CARTESIAN_POINT('Ctrl Pts',(0.985724631999945,11.6,11.312166416));
#226307=CARTESIAN_POINT('Ctrl Pts',(0.984512589999944,15.2,11.315590338));
#226308=CARTESIAN_POINT('Ctrl Pts',(0.984512589999944,11.6,11.315590338));
#226309=CARTESIAN_POINT('Ctrl Pts',(0.983296368999944,15.2,11.319017653));
#226310=CARTESIAN_POINT('Ctrl Pts',(0.983296368999944,11.6,11.319017653));
#226311=CARTESIAN_POINT('Ctrl Pts',(0.982075964999944,15.2,11.322448352));
#226312=CARTESIAN_POINT('Ctrl Pts',(0.982075964999944,11.6,11.322448352));
#226313=CARTESIAN_POINT('Ctrl Pts',(0.980851376999944,15.2,11.325882426));
#226314=CARTESIAN_POINT('Ctrl Pts',(0.980851376999944,11.6,11.325882426));
#226315=CARTESIAN_POINT('Ctrl Pts',(0.979622599999944,15.2,11.329319866));
#226316=CARTESIAN_POINT('Ctrl Pts',(0.979622599999944,11.6,11.329319866));
#226317=CARTESIAN_POINT('Ctrl Pts',(0.978389631999944,15.2,11.332760663));
#226318=CARTESIAN_POINT('Ctrl Pts',(0.978389631999944,11.6,11.332760663));
#226319=CARTESIAN_POINT('Ctrl Pts',(0.977152469999945,15.2,11.336204808));
#226320=CARTESIAN_POINT('Ctrl Pts',(0.977152469999945,11.6,11.336204808));
#226321=CARTESIAN_POINT('Ctrl Pts',(0.975911110999944,15.2,11.339652292));
#226322=CARTESIAN_POINT('Ctrl Pts',(0.975911110999944,11.6,11.339652292));
#226323=CARTESIAN_POINT('Ctrl Pts',(0.974665549999945,15.2,11.343103107));
#226324=CARTESIAN_POINT('Ctrl Pts',(0.974665549999945,11.6,11.343103107));
#226325=CARTESIAN_POINT('Ctrl Pts',(0.973415787999944,15.2,11.346557243));
#226326=CARTESIAN_POINT('Ctrl Pts',(0.973415787999944,11.6,11.346557243));
#226327=CARTESIAN_POINT('Ctrl Pts',(0.972161818999945,15.2,11.350014692));
#226328=CARTESIAN_POINT('Ctrl Pts',(0.972161818999945,11.6,11.350014692));
#226329=CARTESIAN_POINT('Ctrl Pts',(0.970903640999944,15.2,11.353475445));
#226330=CARTESIAN_POINT('Ctrl Pts',(0.970903640999944,11.6,11.353475445));
#226331=CARTESIAN_POINT('Ctrl Pts',(0.969641250999944,15.2,11.356939492));
#226332=CARTESIAN_POINT('Ctrl Pts',(0.969641250999944,11.6,11.356939492));
#226333=CARTESIAN_POINT('Ctrl Pts',(0.968374644999944,15.2,11.360406825));
#226334=CARTESIAN_POINT('Ctrl Pts',(0.968374644999944,11.6,11.360406825));
#226335=CARTESIAN_POINT('Ctrl Pts',(0.967103821999945,15.2,11.363877435));
#226336=CARTESIAN_POINT('Ctrl Pts',(0.967103821999945,11.6,11.363877435));
#226337=CARTESIAN_POINT('Ctrl Pts',(0.965828776999944,15.2,11.367351315));
#226338=CARTESIAN_POINT('Ctrl Pts',(0.965828776999944,11.6,11.367351315));
#226339=CARTESIAN_POINT('Ctrl Pts',(0.964549509999945,15.2,11.370828453));
#226340=CARTESIAN_POINT('Ctrl Pts',(0.964549509999945,11.6,11.370828453));
#226341=CARTESIAN_POINT('Ctrl Pts',(0.963266015999944,15.2,11.374308844));
#226342=CARTESIAN_POINT('Ctrl Pts',(0.963266015999944,11.6,11.374308844));
#226343=CARTESIAN_POINT('Ctrl Pts',(0.961978292999944,15.2,11.377792477));
#226344=CARTESIAN_POINT('Ctrl Pts',(0.961978292999944,11.6,11.377792477));
#226345=CARTESIAN_POINT('Ctrl Pts',(0.960686336999944,15.2,11.381279343));
#226346=CARTESIAN_POINT('Ctrl Pts',(0.960686336999944,11.6,11.381279343));
#226347=CARTESIAN_POINT('Ctrl Pts',(0.959390145999944,15.2,11.384769435));
#226348=CARTESIAN_POINT('Ctrl Pts',(0.959390145999944,11.6,11.384769435));
#226349=CARTESIAN_POINT('Ctrl Pts',(0.958089717999945,15.2,11.388262743));
#226350=CARTESIAN_POINT('Ctrl Pts',(0.958089717999945,11.6,11.388262743));
#226351=CARTESIAN_POINT('Ctrl Pts',(0.956785049999944,15.2,11.391759258));
#226352=CARTESIAN_POINT('Ctrl Pts',(0.956785049999944,11.6,11.391759258));
#226353=CARTESIAN_POINT('Ctrl Pts',(0.955476135999944,15.2,11.395258971));
#226354=CARTESIAN_POINT('Ctrl Pts',(0.955476135999944,11.6,11.395258971));
#226355=CARTESIAN_POINT('Ctrl Pts',(0.954162975999945,15.2,11.398761871));
#226356=CARTESIAN_POINT('Ctrl Pts',(0.954162975999945,11.6,11.398761871));
#226357=CARTESIAN_POINT('Ctrl Pts',(0.952845566999944,15.2,11.402267953));
#226358=CARTESIAN_POINT('Ctrl Pts',(0.952845566999944,11.6,11.402267953));
#226359=CARTESIAN_POINT('Ctrl Pts',(0.951523905999945,15.2,11.405777206));
#226360=CARTESIAN_POINT('Ctrl Pts',(0.951523905999945,11.6,11.405777206));
#226361=CARTESIAN_POINT('Ctrl Pts',(0.950197990999944,15.2,11.409289625));
#226362=CARTESIAN_POINT('Ctrl Pts',(0.950197990999944,11.6,11.409289625));
#226363=CARTESIAN_POINT('Ctrl Pts',(0.948867817999944,15.2,11.4128052));
#226364=CARTESIAN_POINT('Ctrl Pts',(0.948867817999944,11.6,11.4128052));
#226365=CARTESIAN_POINT('Ctrl Pts',(0.947533385999945,15.2,11.416323924));
#226366=CARTESIAN_POINT('Ctrl Pts',(0.947533385999945,11.6,11.416323924));
#226367=CARTESIAN_POINT('Ctrl Pts',(0.946194692999944,15.2,11.419845788));
#226368=CARTESIAN_POINT('Ctrl Pts',(0.946194692999944,11.6,11.419845788));
#226369=CARTESIAN_POINT('Ctrl Pts',(0.944851733999944,15.2,11.423370785));
#226370=CARTESIAN_POINT('Ctrl Pts',(0.944851733999944,11.6,11.423370785));
#226371=CARTESIAN_POINT('Ctrl Pts',(0.943504507999945,15.2,11.426898902));
#226372=CARTESIAN_POINT('Ctrl Pts',(0.943504507999945,11.6,11.426898902));
#226373=CARTESIAN_POINT('Ctrl Pts',(0.942153009999944,15.2,11.430430131));
#226374=CARTESIAN_POINT('Ctrl Pts',(0.942153009999944,11.6,11.430430131));
#226375=CARTESIAN_POINT('Ctrl Pts',(0.940797236999944,15.2,11.43396446));
#226376=CARTESIAN_POINT('Ctrl Pts',(0.940797236999944,11.6,11.43396446));
#226377=CARTESIAN_POINT('Ctrl Pts',(0.939437186999944,15.2,11.437501879));
#226378=CARTESIAN_POINT('Ctrl Pts',(0.939437186999944,11.6,11.437501879));
#226379=CARTESIAN_POINT('Ctrl Pts',(0.938072854999944,15.2,11.441042379));
#226380=CARTESIAN_POINT('Ctrl Pts',(0.938072854999944,11.6,11.441042379));
#226381=CARTESIAN_POINT('Ctrl Pts',(0.936704240999945,15.2,11.444585952));
#226382=CARTESIAN_POINT('Ctrl Pts',(0.936704240999945,11.6,11.444585952));
#226383=CARTESIAN_POINT('Ctrl Pts',(0.935331340999944,15.2,11.448132591));
#226384=CARTESIAN_POINT('Ctrl Pts',(0.935331340999944,11.6,11.448132591));
#226385=CARTESIAN_POINT('Ctrl Pts',(0.933954155999944,15.2,11.451682296));
#226386=CARTESIAN_POINT('Ctrl Pts',(0.933954155999944,11.6,11.451682296));
#226387=CARTESIAN_POINT('Ctrl Pts',(0.932572683999945,15.2,11.45523506));
#226388=CARTESIAN_POINT('Ctrl Pts',(0.932572683999945,11.6,11.45523506));
#226389=CARTESIAN_POINT('Ctrl Pts',(0.931464076999945,15.2,11.458079719));
#226390=CARTESIAN_POINT('Ctrl Pts',(0.931464076999945,11.6,11.458079719));
#226391=CARTESIAN_POINT('Ctrl Pts',(0.930630692999944,15.2,11.460214592));
#226392=CARTESIAN_POINT('Ctrl Pts',(0.930630692999944,11.6,11.460214592));
#226393=CARTESIAN_POINT('Ctrl Pts',(0.930074245999944,15.2,11.461638451));
#226394=CARTESIAN_POINT('Ctrl Pts',(0.930074245999944,11.6,11.461638451));
#226395=CARTESIAN_POINT('Ctrl Pts',(0.929795807999944,15.2,11.462350533));
#226396=CARTESIAN_POINT('Ctrl Pts',(0.929795807999944,11.6,11.462350533));
#226397=CARTESIAN_POINT('Ctrl Pts',(1.18690176599994,15.2,10.306885525));
#226398=CARTESIAN_POINT('Ctrl Pts',(1.18695286801371,15.2,10.3086714414971));
#226399=CARTESIAN_POINT('Ctrl Pts',(1.18700024370246,15.2,10.3105146695817));
#226400=CARTESIAN_POINT('Ctrl Pts',(1.18704320751191,15.2,10.3124142316168));
#226401=CARTESIAN_POINT('Ctrl Pts',(1.18708637851457,15.2,10.3143229543003));
#226402=CARTESIAN_POINT('Ctrl Pts',(1.18712509878331,15.2,10.3162885644145));
#226403=CARTESIAN_POINT('Ctrl Pts',(1.18715870878653,15.2,10.3183101254623));
#226404=CARTESIAN_POINT('Ctrl Pts',(1.18720912378677,15.2,10.3213424667585));
#226405=CARTESIAN_POINT('Ctrl Pts',(1.18724803363287,15.2,10.3245006945537));
#226406=CARTESIAN_POINT('Ctrl Pts',(1.18727330150735,15.2,10.3277817524309));
#226407=CARTESIAN_POINT('Ctrl Pts',(1.18729014675699,15.2,10.329969124349));
#226408=CARTESIAN_POINT('Ctrl Pts',(1.18730093215753,15.2,10.3322110923867));
#226409=CARTESIAN_POINT('Ctrl Pts',(1.18730504824117,15.2,10.3345067774663));
#226410=CARTESIAN_POINT('Ctrl Pts',(1.18730916432518,15.2,10.3368024627545));
#226411=CARTESIAN_POINT('Ctrl Pts',(1.18730661025857,15.2,10.3391518689812));
#226412=CARTESIAN_POINT('Ctrl Pts',(1.18729679950772,15.2,10.3415541411144));
#226413=CARTESIAN_POINT('Ctrl Pts',(1.18728698875776,15.2,10.3439564130294));
#226414=CARTESIAN_POINT('Ctrl Pts',(1.18726991898249,15.2,10.3464115510702));
#226415=CARTESIAN_POINT('Ctrl Pts',(1.18724502131664,15.2,10.3489187242404));
#226416=CARTESIAN_POINT('Ctrl Pts',(1.18720767481559,15.2,10.3526794842235));
#226417=CARTESIAN_POINT('Ctrl Pts',(1.18715270884723,15.2,10.3565573188216));
#226418=CARTESIAN_POINT('Ctrl Pts',(1.18707827071955,15.2,10.3605495050483));
#226419=CARTESIAN_POINT('Ctrl Pts',(1.1870286453041,15.2,10.3632109623717));
#226420=CARTESIAN_POINT('Ctrl Pts',(1.18697036882753,15.2,10.3659232462405));
#226421=CARTESIAN_POINT('Ctrl Pts',(1.18690291049625,15.2,10.3686855733923));
#226422=CARTESIAN_POINT('Ctrl Pts',(1.18683545216496,15.2,10.3714479005441));
#226423=CARTESIAN_POINT('Ctrl Pts',(1.18675881427607,15.2,10.3742602697669));
#226424=CARTESIAN_POINT('Ctrl Pts',(1.18667248202963,15.2,10.3771219183275));
#226425=CARTESIAN_POINT('Ctrl Pts',(1.18657176107022,15.2,10.3804605084881));
#226426=CARTESIAN_POINT('Ctrl Pts',(1.18645784638535,15.2,10.3838661730002));
#226427=CARTESIAN_POINT('Ctrl Pts',(1.18632994899394,15.2,10.3873377257373));
#226428=CARTESIAN_POINT('Ctrl Pts',(1.18622032266415,15.2,10.3903133422146));
#226429=CARTESIAN_POINT('Ctrl Pts',(1.18610042326015,15.2,10.3933373687964));
#226430=CARTESIAN_POINT('Ctrl Pts',(1.18596977101537,15.2,10.3964090753493));
#226431=CARTESIAN_POINT('Ctrl Pts',(1.18579556801838,15.2,10.4005046841795));
#226432=CARTESIAN_POINT('Ctrl Pts',(1.1856022450273,15.2,10.4046850589283));
#226433=CARTESIAN_POINT('Ctrl Pts',(1.18538870347531,15.2,10.4089485158675));
#226434=CARTESIAN_POINT('Ctrl Pts',(1.18522854730041,15.2,10.4121461087897));
#226435=CARTESIAN_POINT('Ctrl Pts',(1.18505701725744,15.2,10.4153904361511));
#226436=CARTESIAN_POINT('Ctrl Pts',(1.18487366424664,15.2,10.4186808080836));
#226437=CARTESIAN_POINT('Ctrl Pts',(1.18453751708517,15.1999999999999,10.424713156178));
#226438=CARTESIAN_POINT('Ctrl Pts',(1.18416162582464,15.2,10.4309002494383));
#226439=CARTESIAN_POINT('Ctrl Pts',(1.18374332547081,15.2,10.4372379486635));
#226440=CARTESIAN_POINT('Ctrl Pts',(1.18347713432714,15.2,10.4412710301313));
#226441=CARTESIAN_POINT('Ctrl Pts',(1.18319377335533,15.2,10.4453651054476));
#226442=CARTESIAN_POINT('Ctrl Pts',(1.18289258444682,15.2,10.4495191354464));
#226443=CARTESIAN_POINT('Ctrl Pts',(1.18263442253865,15.2,10.4530797324033));
#226444=CARTESIAN_POINT('Ctrl Pts',(1.18236316078296,15.2,10.4566843811463));
#226445=CARTESIAN_POINT('Ctrl Pts',(1.18207840170939,15.2,10.4603324401822));
#226446=CARTESIAN_POINT('Ctrl Pts',(1.18174618277298,15.2,10.4645885092785));
#226447=CARTESIAN_POINT('Ctrl Pts',(1.18139558505007,15.2,10.4689036675259));
#226448=CARTESIAN_POINT('Ctrl Pts',(1.18102599447377,15.2,10.4732769201252));
#226449=CARTESIAN_POINT('Ctrl Pts',(1.18070920256766,15.2,10.4770254221585));
#226450=CARTESIAN_POINT('Ctrl Pts',(1.18037845378586,15.2,10.4808166073047));
#226451=CARTESIAN_POINT('Ctrl Pts',(1.18003337196443,15.2,10.4846498614173));
#226452=CARTESIAN_POINT('Ctrl Pts',(1.17963077648521,15.2,10.4891219914475));
#226453=CARTESIAN_POINT('Ctrl Pts',(1.17920866856116,15.2,10.4936513837703));
#226454=CARTESIAN_POINT('Ctrl Pts',(1.17876646494199,15.2,10.49823708297));
#226455=CARTESIAN_POINT('Ctrl Pts',(1.17838743328808,15.2,10.5021676820801));
#226456=CARTESIAN_POINT('Ctrl Pts',(1.17799363670509,15.2,10.5061396515878));
#226457=CARTESIAN_POINT('Ctrl Pts',(1.17758471896929,15.2,10.5101524006938));
#226458=CARTESIAN_POINT('Ctrl Pts',(1.17717580123348,15.2,10.5141651497998));
#226459=CARTESIAN_POINT('Ctrl Pts',(1.1767517616989,15.2,10.518218679519));
#226460=CARTESIAN_POINT('Ctrl Pts',(1.17631224929886,15.2,10.5223124107853));
#226461=CARTESIAN_POINT('Ctrl Pts',(1.17594598895219,15.2,10.5257238536312));
#226462=CARTESIAN_POINT('Ctrl Pts',(1.17556898609636,15.2,10.5291632155101));
#226463=CARTESIAN_POINT('Ctrl Pts',(1.17518104373351,15.2,10.5326301650397));
#226464=CARTESIAN_POINT('Ctrl Pts',(1.17479310137067,15.2,10.5360971145692));
#226465=CARTESIAN_POINT('Ctrl Pts',(1.17439421723886,15.2,10.5395916527444));
#226466=CARTESIAN_POINT('Ctrl Pts',(1.17398420022497,15.2,10.5431134547582));
#226467=CARTESIAN_POINT('Ctrl Pts',(1.17357418321109,15.2,10.5466352567721));
#226468=CARTESIAN_POINT('Ctrl Pts',(1.17315303291284,15.2,10.5501843224578));
#226469=CARTESIAN_POINT('Ctrl Pts',(1.17272056075807,15.2,10.5537603312935));
#226470=CARTESIAN_POINT('Ctrl Pts',(1.1722015941912,15.2,10.5580515417405));
#226471=CARTESIAN_POINT('Ctrl Pts',(1.17166632422587,15.2,10.5623815507141));
#226472=CARTESIAN_POINT('Ctrl Pts',(1.17111443174665,15.2,10.5667498129703));
#226473=CARTESIAN_POINT('Ctrl Pts',(1.17056253921729,15.2,10.5711180756234));
#226474=CARTESIAN_POINT('Ctrl Pts',(1.16999402489421,15.2,10.5755245911646));
#226475=CARTESIAN_POINT('Ctrl Pts',(1.16940857744449,15.2,10.5799688229927));
#226476=CARTESIAN_POINT('Ctrl Pts',(1.16892070464949,15.2,10.5836723489106));
#226477=CARTESIAN_POINT('Ctrl Pts',(1.16842107404348,15.2,10.5874020673035));
#226478=CARTESIAN_POINT('Ctrl Pts',(1.16790950805855,15.2,10.5911576723087));
#226479=CARTESIAN_POINT('Ctrl Pts',(1.16719331559044,15.2,10.5964155199709));
#226480=CARTESIAN_POINT('Ctrl Pts',(1.16645373272989,15.2,10.6017241030071));
#226481=CARTESIAN_POINT('Ctrl Pts',(1.16569028676057,15.2,10.6070825977414));
#226482=CARTESIAN_POINT('Ctrl Pts',(1.16514496821954,15.2,10.6109100939206));
#226483=CARTESIAN_POINT('Ctrl Pts',(1.16458747581952,15.2,10.6147630547858));
#226484=CARTESIAN_POINT('Ctrl Pts',(1.16401764373362,15.2,10.6186411829978));
#226485=CARTESIAN_POINT('Ctrl Pts',(1.16333384525538,15.2,10.6232949366832));
#226486=CARTESIAN_POINT('Ctrl Pts',(1.16263227336771,15.2,10.6279849340589));
#226487=CARTESIAN_POINT('Ctrl Pts',(1.16191265006174,15.2,10.6327106667182));
#226488=CARTESIAN_POINT('Ctrl Pts',(1.16119302669041,15.2,10.6374363998066));
#226489=CARTESIAN_POINT('Ctrl Pts',(1.16045534972569,15.2,10.6421978708152));
#226490=CARTESIAN_POINT('Ctrl Pts',(1.1596993444337,15.2,10.6469945807448));
#226491=CARTESIAN_POINT('Ctrl Pts',(1.15906934005804,15.2,10.6509918388016));
#226492=CARTESIAN_POINT('Ctrl Pts',(1.15842660794081,15.2,10.6550135682326));
#226493=CARTESIAN_POINT('Ctrl Pts',(1.15777099269882,15.2,10.659059485728));
#226494=CARTESIAN_POINT('Ctrl Pts',(1.15711537745684,15.2,10.6631054032235));
#226495=CARTESIAN_POINT('Ctrl Pts',(1.15644687780632,15.2,10.667175508028));
#226496=CARTESIAN_POINT('Ctrl Pts',(1.15576534190249,15.2,10.6712695187938));
#226497=CARTESIAN_POINT('Ctrl Pts',(1.155220113224,15.2,10.6745447271386));
#226498=CARTESIAN_POINT('Ctrl Pts',(1.15466654257434,15.2,10.6778352371122));
#226499=CARTESIAN_POINT('Ctrl Pts',(1.15410455178751,15.2,10.6811409047298));
#226500=CARTESIAN_POINT('Ctrl Pts',(1.1535425609241,15.2,10.6844465727978));
#226501=CARTESIAN_POINT('Ctrl Pts',(1.15297215003825,15.2,10.6877673986787));
#226502=CARTESIAN_POINT('Ctrl Pts',(1.15239324386593,15.2,10.6911032422507));
#226503=CARTESIAN_POINT('Ctrl Pts',(1.15166961118997,15.2,10.6952730464885));
#226504=CARTESIAN_POINT('Ctrl Pts',(1.1509327052696,15.2,10.6994663145884));
#226505=CARTESIAN_POINT('Ctrl Pts',(1.1501823808935,15.2,10.7036827752848));
#226506=CARTESIAN_POINT('Ctrl Pts',(1.14928199167489,15.2,10.7087425279366));
#226507=CARTESIAN_POINT('Ctrl Pts',(1.14836228026973,15.2,10.7138356774902));
#226508=CARTESIAN_POINT('Ctrl Pts',(1.14742300029955,15.2,10.7189617582439));
#226509=CARTESIAN_POINT('Ctrl Pts',(1.1467968136812,15.2,10.7223791452579));
#226510=CARTESIAN_POINT('Ctrl Pts',(1.1461619311628,15.2,10.725811169478));
#226511=CARTESIAN_POINT('Ctrl Pts',(1.14551828110521,15.2,10.7292576936948));
#226512=CARTESIAN_POINT('Ctrl Pts',(1.1443918933948,15.2,10.7352891116611));
#226513=CARTESIAN_POINT('Ctrl Pts',(1.14323865498352,15.2,10.7413649352983));
#226514=CARTESIAN_POINT('Ctrl Pts',(1.14205819256337,15.2,10.7474844471975));
#226515=CARTESIAN_POINT('Ctrl Pts',(1.14138364258275,15.2,10.7509813112761));
#226516=CARTESIAN_POINT('Ctrl Pts',(1.14070020422257,15.2,10.7544924398559));
#226517=CARTESIAN_POINT('Ctrl Pts',(1.14000780814946,15.2,10.7580177015032));
#226518=CARTESIAN_POINT('Ctrl Pts',(1.13896921413414,15.2,10.7633055934938));
#226519=CARTESIAN_POINT('Ctrl Pts',(1.13791046703578,15.2,10.768625281911));
#226520=CARTESIAN_POINT('Ctrl Pts',(1.13683134199165,15.2,10.7739763247166));
#226521=CARTESIAN_POINT('Ctrl Pts',(1.13611192523021,15.2,10.7775436869111));
#226522=CARTESIAN_POINT('Ctrl Pts',(1.13538345167051,15.2,10.7811249847571));
#226523=CARTESIAN_POINT('Ctrl Pts',(1.13464585562938,15.2,10.7847200876211));
#226524=CARTESIAN_POINT('Ctrl Pts',(1.13372386072871,15.2,10.7892139654663));
#226525=CARTESIAN_POINT('Ctrl Pts',(1.13278761255285,15.2,10.7937294145361));
#226526=CARTESIAN_POINT('Ctrl Pts',(1.13183698515765,15.2,10.7982661832065));
#226527=CARTESIAN_POINT('Ctrl Pts',(1.13107648311716,15.2,10.8018955987362));
#226528=CARTESIAN_POINT('Ctrl Pts',(1.13030677847856,15.2,10.8055386578811));
#226529=CARTESIAN_POINT('Ctrl Pts',(1.12952780849165,15.2,10.8091952340249));
#226530=CARTESIAN_POINT('Ctrl Pts',(1.12835935361742,15.2,10.8146800977424));
#226531=CARTESIAN_POINT('Ctrl Pts',(1.12717005279062,15.2,10.8201953749398));
#226532=CARTESIAN_POINT('Ctrl Pts',(1.12595969485868,15.2,10.8257406381802));
#226533=CARTESIAN_POINT('Ctrl Pts',(1.12474933681681,15.2,10.8312859019244));
#226534=CARTESIAN_POINT('Ctrl Pts',(1.12351792356648,15.2,10.8368611537618));
#226535=CARTESIAN_POINT('Ctrl Pts',(1.12226524966344,15.2,10.8424659701525));
#226536=CARTESIAN_POINT('Ctrl Pts',(1.12122135480113,15.2,10.8471366502236));
#226537=CARTESIAN_POINT('Ctrl Pts',(1.12016269726633,15.2,10.8518278621646));
#226538=CARTESIAN_POINT('Ctrl Pts',(1.11908916066789,15.2,10.8565393663329));
#226539=CARTESIAN_POINT('Ctrl Pts',(1.11801562418647,15.2,10.8612508699876));
#226540=CARTESIAN_POINT('Ctrl Pts',(1.11692720788392,15.2,10.8659826645702));
#226541=CARTESIAN_POINT('Ctrl Pts',(1.1158238006443,15.2,10.8707345116201));
#226542=CARTESIAN_POINT('Ctrl Pts',(1.11494107470829,15.2,10.8745359898815));
#226543=CARTESIAN_POINT('Ctrl Pts',(1.11404875380192,15.2,10.8783503023303));
#226544=CARTESIAN_POINT('Ctrl Pts',(1.11314678180832,15.2,10.8821773273166));
#226545=CARTESIAN_POINT('Ctrl Pts',(1.11179382394082,15.2,10.8879178642746));
#226546=CARTESIAN_POINT('Ctrl Pts',(1.11041914749445,15.2,10.8936870052702));
#226547=CARTESIAN_POINT('Ctrl Pts',(1.10902256939336,15.2,10.8994843454308));
#226548=CARTESIAN_POINT('Ctrl Pts',(1.10785875426684,15.2,10.9043154624069));
#226549=CARTESIAN_POINT('Ctrl Pts',(1.10667972569385,15.2,10.9091661619548));
#226550=CARTESIAN_POINT('Ctrl Pts',(1.10548538006967,15.2,10.9140362136899));
#226551=CARTESIAN_POINT('Ctrl Pts',(1.10429103444549,15.2,10.9189062654249));
#226552=CARTESIAN_POINT('Ctrl Pts',(1.1030813707681,15.2,10.9237956675634));
#226553=CARTESIAN_POINT('Ctrl Pts',(1.10185628438001,15.2,10.9287041919374));
#226554=CARTESIAN_POINT('Ctrl Pts',(1.10014116340998,15.2,10.935576126168));
#226555=CARTESIAN_POINT('Ctrl Pts',(1.09839581377953,15.2,10.9424855407517));
#226556=CARTESIAN_POINT('Ctrl Pts',(1.09661995700762,15.2,10.9494318102527));
#226557=CARTESIAN_POINT('Ctrl Pts',(1.09509779413927,15.2,10.9553857552302));
#226558=CARTESIAN_POINT('Ctrl Pts',(1.09355321476903,15.2,10.9613667788838));
#226559=CARTESIAN_POINT('Ctrl Pts',(1.09198605007697,15.2,10.9673744939143));
#226560=CARTESIAN_POINT('Ctrl Pts',(1.09094127352069,15.2,10.9713796376318));
#226561=CARTESIAN_POINT('Ctrl Pts',(1.08988645932708,15.2,10.9753966439952));
#226562=CARTESIAN_POINT('Ctrl Pts',(1.08882155671283,15.2,10.9794253996044));
#226563=CARTESIAN_POINT('Ctrl Pts',(1.08775665424368,15.2,10.9834541546647));
#226564=CARTESIAN_POINT('Ctrl Pts',(1.08668166219425,15.2,10.9874946584668));
#226565=CARTESIAN_POINT('Ctrl Pts',(1.08559653367406,15.2,10.9915467991703));
#226566=CARTESIAN_POINT('Ctrl Pts',(1.08369755857891,15.2,10.9986380460917));
#226567=CARTESIAN_POINT('Ctrl Pts',(1.08176753691945,15.2,11.0057649279105));
#226568=CARTESIAN_POINT('Ctrl Pts',(1.07980621174998,15.2,11.0129268455083));
#226569=CARTESIAN_POINT('Ctrl Pts',(1.07868545446665,15.2,11.0170193700092));
#226570=CARTESIAN_POINT('Ctrl Pts',(1.07755447462942,15.2,11.021123336189));
#226571=CARTESIAN_POINT('Ctrl Pts',(1.07641322728838,15.2,11.0252386319145));
#226572=CARTESIAN_POINT('Ctrl Pts',(1.07527198010284,15.2,11.0293539270792));
#226573=CARTESIAN_POINT('Ctrl Pts',(1.07412046251936,15.2,11.0334805523111));
#226574=CARTESIAN_POINT('Ctrl Pts',(1.07295863077578,15.2,11.0376183975471));
#226575=CARTESIAN_POINT('Ctrl Pts',(1.0717967988739,15.2,11.0417562433469));
#226576=CARTESIAN_POINT('Ctrl Pts',(1.07062465233603,15.2,11.0459053084245));
#226577=CARTESIAN_POINT('Ctrl Pts',(1.06944214454831,15.2,11.0500654854301));
#226578=CARTESIAN_POINT('Ctrl Pts',(1.0682596369217,15.2,11.0542256618689));
#226579=CARTESIAN_POINT('Ctrl Pts',(1.06706676838811,15.2,11.0583969486063));
#226580=CARTESIAN_POINT('Ctrl Pts',(1.06586349459825,15.2,11.0625792383748));
#226581=CARTESIAN_POINT('Ctrl Pts',(1.06435940223797,15.2,11.0678071010129));
#226582=CARTESIAN_POINT('Ctrl Pts',(1.06283904978554,15.2,11.0730521546788));
#226583=CARTESIAN_POINT('Ctrl Pts',(1.06130235325082,15.2,11.0783141899804));
#226584=CARTESIAN_POINT('Ctrl Pts',(1.06007299595604,15.2,11.0825238184512));
#226585=CARTESIAN_POINT('Ctrl Pts',(1.05883317699255,15.2,11.0867443142906));
#226586=CARTESIAN_POINT('Ctrl Pts',(1.05758285447889,15.2,11.0909755714668));
#226587=CARTESIAN_POINT('Ctrl Pts',(1.05601995142198,15.2,11.0962646426487));
#226588=CARTESIAN_POINT('Ctrl Pts',(1.05444063549815,15.2,11.1015705285948));
#226589=CARTESIAN_POINT('Ctrl Pts',(1.05284482327458,15.2,11.1068930229711));
#226590=CARTESIAN_POINT('Ctrl Pts',(1.05156817360009,15.2,11.1111510181241));
#226591=CARTESIAN_POINT('Ctrl Pts',(1.05028096661174,15.2,11.1154196405691));
#226592=CARTESIAN_POINT('Ctrl Pts',(1.04898316026753,15.2,11.1196987877387));
#226593=CARTESIAN_POINT('Ctrl Pts',(1.04736090220466,15.2,11.1250477221379));
#226594=CARTESIAN_POINT('Ctrl Pts',(1.04572208267221,15.2,11.1304131000166));
#226595=CARTESIAN_POINT('Ctrl Pts',(1.04406662128332,15.2,11.1357947162666));
#226596=CARTESIAN_POINT('Ctrl Pts',(1.04307334448608,15.2,11.1390236858993));
#226597=CARTESIAN_POINT('Ctrl Pts',(1.0420740771224,15.2,11.1422585022818));
#226598=CARTESIAN_POINT('Ctrl Pts',(1.04106880140946,15.2,11.1454991208718));
#226599=CARTESIAN_POINT('Ctrl Pts',(1.03972843367046,15.2,11.149819946051));
#226600=CARTESIAN_POINT('Ctrl Pts',(1.03837738522607,15.2,11.1541510856172));
#226601=CARTESIAN_POINT('Ctrl Pts',(1.03701561536066,15.2,11.158492438905));
#226602=CARTESIAN_POINT('Ctrl Pts',(1.03565384568079,15.2,11.1628337916012));
#226603=CARTESIAN_POINT('Ctrl Pts',(1.03428135514361,15.2,11.1671853555285));
#226604=CARTESIAN_POINT('Ctrl Pts',(1.03289810481297,15.2,11.1715470293935));
#226605=CARTESIAN_POINT('Ctrl Pts',(1.03116904175831,15.2,11.1769991221704));
#226606=CARTESIAN_POINT('Ctrl Pts',(1.02942316644761,15.2,11.18246701217));
#226607=CARTESIAN_POINT('Ctrl Pts',(1.02766040186517,15.2,11.1879504991831));
#226608=CARTESIAN_POINT('Ctrl Pts',(1.02589763728273,15.2,11.1934339861961));
#226609=CARTESIAN_POINT('Ctrl Pts',(1.02411798678128,15.2,11.1989330715553));
#226610=CARTESIAN_POINT('Ctrl Pts',(1.0223213722593,15.2,11.2044475569969));
#226611=CARTESIAN_POINT('Ctrl Pts',(1.02124340358528,15.2,11.2077562481417));
#226612=CARTESIAN_POINT('Ctrl Pts',(1.02015932932857,15.2,11.2110704840593));
#226613=CARTESIAN_POINT('Ctrl Pts',(1.01906913307705,15.2,11.2143902211882));
#226614=CARTESIAN_POINT('Ctrl Pts',(1.01797893682553,15.2,11.2177099583171));
#226615=CARTESIAN_POINT('Ctrl Pts',(1.01688261823276,15.2,11.2210351974956));
#226616=CARTESIAN_POINT('Ctrl Pts',(1.01578016248198,15.2,11.2243658970405));
#226617=CARTESIAN_POINT('Ctrl Pts',(1.01467770653093,15.2,11.2276965971905));
#226618=CARTESIAN_POINT('Ctrl Pts',(1.01356911398648,15.2,11.2310327560754));
#226619=CARTESIAN_POINT('Ctrl Pts',(1.01245436803196,15.2,11.2343743337284));
#226620=CARTESIAN_POINT('Ctrl Pts',(1.01096804043012,15.2,11.2388297695874));
#226621=CARTESIAN_POINT('Ctrl Pts',(1.00947077389564,15.2,11.2432948359924));
#226622=CARTESIAN_POINT('Ctrl Pts',(1.00796253423434,15.2,11.2477694359802));
#226623=CARTESIAN_POINT('Ctrl Pts',(1.00683135443699,15.2,11.2511253861235));
#226624=CARTESIAN_POINT('Ctrl Pts',(1.0056940009491,15.2,11.2544866994392));
#226625=CARTESIAN_POINT('Ctrl Pts',(1.00455046065786,15.2,11.2578533326081));
#226626=CARTESIAN_POINT('Ctrl Pts',(1.00302574013104,15.2,11.262342177241));
#226627=CARTESIAN_POINT('Ctrl Pts',(1.00149001879179,15.2,11.2668404801473));
#226628=CARTESIAN_POINT('Ctrl Pts',(0.999943262373438,15.2,11.2713481458935));
#226629=CARTESIAN_POINT('Ctrl Pts',(0.998783195165049,15.2,11.2747288948962));
#226630=CARTESIAN_POINT('Ctrl Pts',(0.997616920657404,15.2,11.2781149094398));
#226631=CARTESIAN_POINT('Ctrl Pts',(0.996444424449991,15.2,11.2815061485249));
#226632=CARTESIAN_POINT('Ctrl Pts',(0.995271928242578,15.2,11.2848973876101));
#226633=CARTESIAN_POINT('Ctrl Pts',(0.994093210618774,15.2,11.2882938507866));
#226634=CARTESIAN_POINT('Ctrl Pts',(0.992908256870712,15.2,11.2916954984126));
#226635=CARTESIAN_POINT('Ctrl Pts',(0.99172330312265,15.2,11.2950971460385));
#226636=CARTESIAN_POINT('Ctrl Pts',(0.990532112980523,15.2,11.298503977744));
#226637=CARTESIAN_POINT('Ctrl Pts',(0.989334672714937,15.2,11.3019159525815));
#226638=CARTESIAN_POINT('Ctrl Pts',(0.988137232449352,15.2,11.3053279274191));
#226639=CARTESIAN_POINT('Ctrl Pts',(0.986933542468933,15.2,11.308745045579));
#226640=CARTESIAN_POINT('Ctrl Pts',(0.985723588263753,15.2,11.3121672657456));
#226641=CARTESIAN_POINT('Ctrl Pts',(0.984513633838765,15.2,11.3155894865339));
#226642=CARTESIAN_POINT('Ctrl Pts',(0.983297415128669,15.2,11.3190168102487));
#226643=CARTESIAN_POINT('Ctrl Pts',(0.982074918700141,15.2,11.3224491964982));
#226644=CARTESIAN_POINT('Ctrl Pts',(0.980852422493701,15.2,11.3258815821242));
#226645=CARTESIAN_POINT('Ctrl Pts',(0.979623648570926,15.2,11.3293190302499));
#226646=CARTESIAN_POINT('Ctrl Pts',(0.978388583365259,15.2,11.3327615003753));
#226647=CARTESIAN_POINT('Ctrl Pts',(0.976330141281025,15.2,11.3384989507926));
#226648=CARTESIAN_POINT('Ctrl Pts',(0.97425422278491,15.2,11.3442503513581));
#226649=CARTESIAN_POINT('Ctrl Pts',(0.972160766498573,15.2,11.3500155186609));
#226650=CARTESIAN_POINT('Ctrl Pts',(0.970067310212236,15.2,11.3557806859637));
#226651=CARTESIAN_POINT('Ctrl Pts',(0.967956314861861,15.2,11.3615596164955));
#226652=CARTESIAN_POINT('Ctrl Pts',(0.965827721179896,15.2,11.367352130316));
#226653=CARTESIAN_POINT('Ctrl Pts',(0.96455056501712,15.2,11.370827638482));
#226654=CARTESIAN_POINT('Ctrl Pts',(0.963267074329644,15.2,11.3743080369395));
#226655=CARTESIAN_POINT('Ctrl Pts',(0.961977234625954,15.2,11.3777932856466));
#226656=CARTESIAN_POINT('Ctrl Pts',(0.960687394922265,15.2,11.3812785343537));
#226657=CARTESIAN_POINT('Ctrl Pts',(0.959391206307425,15.2,11.3847686341142));
#226658=CARTESIAN_POINT('Ctrl Pts',(0.958088657973805,15.2,11.3882635447531));
#226659=CARTESIAN_POINT('Ctrl Pts',(0.956786109640184,15.2,11.391758455392));
#226660=CARTESIAN_POINT('Ctrl Pts',(0.955477198459337,15.2,11.3952581762249));
#226661=CARTESIAN_POINT('Ctrl Pts',(0.954161913751181,15.2,11.3987626664468));
#226662=CARTESIAN_POINT('Ctrl Pts',(0.951969772491273,15.2,11.4046034836955));
#226663=CARTESIAN_POINT('Ctrl Pts',(0.949759925377751,15.2,11.4104575534611));
#226664=CARTESIAN_POINT('Ctrl Pts',(0.947532320724996,15.2,11.4163247090166));
#226665=CARTESIAN_POINT('Ctrl Pts',(0.945750236905668,15.2,11.4210184337168));
#226666=CARTESIAN_POINT('Ctrl Pts',(0.943956788673861,15.2,11.4257205357515));
#226667=CARTESIAN_POINT('Ctrl Pts',(0.942151940963227,15.2,11.4304309067868));
#226668=CARTESIAN_POINT('Ctrl Pts',(0.940798305303206,15.2,11.4339636847424));
#226669=CARTESIAN_POINT('Ctrl Pts',(0.93943825738824,15.2,11.4375011120198));
#226670=CARTESIAN_POINT('Ctrl Pts',(0.938071784202212,15.2,11.4410431479436));
#226671=CARTESIAN_POINT('Ctrl Pts',(0.936705311016184,15.2,11.4445851838674));
#226672=CARTESIAN_POINT('Ctrl Pts',(0.935332412639122,15.2,11.4481318270972));
#226673=CARTESIAN_POINT('Ctrl Pts',(0.933953084118917,15.2,11.4516830612001));
#226674=CARTESIAN_POINT('Ctrl Pts',(0.932573755598712,15.2,11.4552342953029));
#226675=CARTESIAN_POINT('Ctrl Pts',(0.931187998930692,15.2,11.4587901206197));
#226676=CARTESIAN_POINT('Ctrl Pts',(0.929795807999944,15.2,11.462350533));
#226677=CARTESIAN_POINT('Ctrl Pts',(1.18690176599994,12.2,10.306885525));
#226678=CARTESIAN_POINT('Ctrl Pts',(1.18695286801371,12.2,10.3086714414971));
#226679=CARTESIAN_POINT('Ctrl Pts',(1.18700024370246,12.2,10.3105146695817));
#226680=CARTESIAN_POINT('Ctrl Pts',(1.18704320751191,12.2,10.3124142316168));
#226681=CARTESIAN_POINT('Ctrl Pts',(1.18708637851457,12.2,10.3143229543003));
#226682=CARTESIAN_POINT('Ctrl Pts',(1.18712509878331,12.2,10.3162885644145));
#226683=CARTESIAN_POINT('Ctrl Pts',(1.18715870878653,12.2,10.3183101254623));
#226684=CARTESIAN_POINT('Ctrl Pts',(1.18719792045236,12.2,10.3206686130759));
#226685=CARTESIAN_POINT('Ctrl Pts',(1.18723017380984,12.2,10.3231032567151));
#226686=CARTESIAN_POINT('Ctrl Pts',(1.18725445923935,12.2,10.3256126117905));
#226687=CARTESIAN_POINT('Ctrl Pts',(1.18727527532422,12.2,10.3277634878206));
#226688=CARTESIAN_POINT('Ctrl Pts',(1.18729023811691,12.2,10.3299692556294));
#226689=CARTESIAN_POINT('Ctrl Pts',(1.18729873228409,12.2,10.332229031702));
#226690=CARTESIAN_POINT('Ctrl Pts',(1.1873072264505,12.2,10.3344888075693));
#226691=CARTESIAN_POINT('Ctrl Pts',(1.18730925155811,12.2,10.3368025915109));
#226692=CARTESIAN_POINT('Ctrl Pts',(1.18730421297496,12.2,10.3391695235082));
#226693=CARTESIAN_POINT('Ctrl Pts',(1.18729917439181,12.2,10.3415364555056));
#226694=CARTESIAN_POINT('Ctrl Pts',(1.18728707303501,12.2,10.3439565353885));
#226695=CARTESIAN_POINT('Ctrl Pts',(1.18726733053518,12.2,10.3464289265025));
#226696=CARTESIAN_POINT('Ctrl Pts',(1.18724758803356,12.2,10.3489013178411));
#226697=CARTESIAN_POINT('Ctrl Pts',(1.18722020562358,12.2,10.3514260183951));
#226698=CARTESIAN_POINT('Ctrl Pts',(1.18718462303775,12.2,10.354002210789));
#226699=CARTESIAN_POINT('Ctrl Pts',(1.18714311002579,12.2,10.357007768231));
#226700=CARTESIAN_POINT('Ctrl Pts',(1.18709043565391,12.2,10.3600834109926));
#226701=CARTESIAN_POINT('Ctrl Pts',(1.18702574223863,12.2,10.363227875506));
#226702=CARTESIAN_POINT('Ctrl Pts',(1.18697029073335,12.2,10.3659231311179));
#226703=CARTESIAN_POINT('Ctrl Pts',(1.18690600797991,12.2,10.3686689487489));
#226704=CARTESIAN_POINT('Ctrl Pts',(1.18683237347527,12.2,10.371464553238));
#226705=CARTESIAN_POINT('Ctrl Pts',(1.1867587389773,12.2,10.3742601574731));
#226706=CARTESIAN_POINT('Ctrl Pts',(1.18667575005532,12.2,10.3771055480514));
#226707=CARTESIAN_POINT('Ctrl Pts',(1.18658290080825,12.2,10.3799999665429));
#226708=CARTESIAN_POINT('Ctrl Pts',(1.18649005156118,12.2,10.3828943850343));
#226709=CARTESIAN_POINT('Ctrl Pts',(1.18638734160986,12.2,10.3858378317145));
#226710=CARTESIAN_POINT('Ctrl Pts',(1.18627427753108,12.2,10.3888295642704));
#226711=CARTESIAN_POINT('Ctrl Pts',(1.18616121344203,12.2,10.391821297098));
#226712=CARTESIAN_POINT('Ctrl Pts',(1.18603779598505,12.2,10.3948613190067));
#226713=CARTESIAN_POINT('Ctrl Pts',(1.18590354672699,12.2,10.3979488990948));
#226714=CARTESIAN_POINT('Ctrl Pts',(1.18576929748114,12.2,10.4010364789024));
#226715=CARTESIAN_POINT('Ctrl Pts',(1.18562421525287,12.2,10.4041716229954));
#226716=CARTESIAN_POINT('Ctrl Pts',(1.18546783625806,12.2,10.4073536176319));
#226717=CARTESIAN_POINT('Ctrl Pts',(1.18531145726325,12.2,10.4105356122684));
#226718=CARTESIAN_POINT('Ctrl Pts',(1.18514378166932,12.2,10.4137644582844));
#226719=CARTESIAN_POINT('Ctrl Pts',(1.18496435750969,12.2,10.4170394620799));
#226720=CARTESIAN_POINT('Ctrl Pts',(1.18478493333377,12.2,10.420314466173));
#226721=CARTESIAN_POINT('Ctrl Pts',(1.18459375917304,12.2,10.4236356272053));
#226722=CARTESIAN_POINT('Ctrl Pts',(1.18439039899446,12.2,10.4270022671419));
#226723=CARTESIAN_POINT('Ctrl Pts',(1.18418703883435,12.2,10.4303689067727));
#226724=CARTESIAN_POINT('Ctrl Pts',(1.1839714892964,12.2,10.4337810218705));
#226725=CARTESIAN_POINT('Ctrl Pts',(1.18374332547081,12.2,10.4372379486635));
#226726=CARTESIAN_POINT('Ctrl Pts',(1.18351516164522,12.2,10.4406948754565));
#226727=CARTESIAN_POINT('Ctrl Pts',(1.18327438385395,12.2,10.4441966142294));
#226728=CARTESIAN_POINT('Ctrl Pts',(1.18302057603041,12.2,10.4477425100152));
#226729=CARTESIAN_POINT('Ctrl Pts',(1.18276676820687,12.2,10.451288405801));
#226730=CARTESIAN_POINT('Ctrl Pts',(1.18249993016942,12.2,10.4548784596805));
#226731=CARTESIAN_POINT('Ctrl Pts',(1.18221965851385,12.2,10.4585120306289));
#226732=CARTESIAN_POINT('Ctrl Pts',(1.18193938683282,12.2,10.4621456019073));
#226733=CARTESIAN_POINT('Ctrl Pts',(1.18164568252551,12.2,10.4658226901399));
#226734=CARTESIAN_POINT('Ctrl Pts',(1.18133814975815,12.2,10.4695426684278));
#226735=CARTESIAN_POINT('Ctrl Pts',(1.18097936157147,12.2,10.4738826425902));
#226736=CARTESIAN_POINT('Ctrl Pts',(1.18060175535009,12.2,10.4782809928034));
#226737=CARTESIAN_POINT('Ctrl Pts',(1.18020472052873,12.2,10.4827367423836));
#226738=CARTESIAN_POINT('Ctrl Pts',(1.17986440492782,12.2,10.4865559567556));
#226739=CARTESIAN_POINT('Ctrl Pts',(1.17950981874221,12.2,10.4904173423067));
#226740=CARTESIAN_POINT('Ctrl Pts',(1.17914058897145,12.2,10.4943202957711));
#226741=CARTESIAN_POINT('Ctrl Pts',(1.17870982095588,12.2,10.4988737409479));
#226742=CARTESIAN_POINT('Ctrl Pts',(1.17825912168566,12.2,10.5034837655246));
#226743=CARTESIAN_POINT('Ctrl Pts',(1.17778791953566,12.2,10.508149426814));
#226744=CARTESIAN_POINT('Ctrl Pts',(1.17745134655041,12.2,10.5114820422283));
#226745=CARTESIAN_POINT('Ctrl Pts',(1.17710431345143,12.2,10.5148430455923));
#226746=CARTESIAN_POINT('Ctrl Pts',(1.17674661706342,12.2,10.5182321007983));
#226747=CARTESIAN_POINT('Ctrl Pts',(1.17638892067541,12.2,10.5216211560043));
#226748=CARTESIAN_POINT('Ctrl Pts',(1.17602055993437,12.2,10.5250382622744));
#226749=CARTESIAN_POINT('Ctrl Pts',(1.17564133706896,12.2,10.5284830886251));
#226750=CARTESIAN_POINT('Ctrl Pts',(1.17526211420355,12.2,10.5319279149758));
#226751=CARTESIAN_POINT('Ctrl Pts',(1.17487202939223,12.2,10.5354004607559));
#226752=CARTESIAN_POINT('Ctrl Pts',(1.17447088876781,12.2,10.5389003995045));
#226753=CARTESIAN_POINT('Ctrl Pts',(1.17406974814338,12.2,10.5424003382531));
#226754=CARTESIAN_POINT('Ctrl Pts',(1.17365755116589,12.2,10.5459276703358));
#226755=CARTESIAN_POINT('Ctrl Pts',(1.17323410581927,12.2,10.5494820732509));
#226756=CARTESIAN_POINT('Ctrl Pts',(1.17281066047264,12.2,10.5530364761661));
#226757=CARTESIAN_POINT('Ctrl Pts',(1.17237596858554,12.2,10.5566179510706));
#226758=CARTESIAN_POINT('Ctrl Pts',(1.17192984400021,12.2,10.5602261782397));
#226759=CARTESIAN_POINT('Ctrl Pts',(1.17148371941488,12.2,10.5638344054087));
#226760=CARTESIAN_POINT('Ctrl Pts',(1.17102616084442,12.2,10.5674693866999));
#226761=CARTESIAN_POINT('Ctrl Pts',(1.17055698723331,12.2,10.5711308064916));
#226762=CARTESIAN_POINT('Ctrl Pts',(1.1700878136222,12.2,10.5747922262832));
#226763=CARTESIAN_POINT('Ctrl Pts',(1.16960702440198,12.2,10.5784800877183));
#226764=CARTESIAN_POINT('Ctrl Pts',(1.16911444148304,12.2,10.5821940789853));
#226765=CARTESIAN_POINT('Ctrl Pts',(1.1686218585641,12.2,10.5859080702522));
#226766=CARTESIAN_POINT('Ctrl Pts',(1.16811748120008,12.2,10.5896481926784));
#226767=CARTESIAN_POINT('Ctrl Pts',(1.16760113494947,12.2,10.5934141399714));
#226768=CARTESIAN_POINT('Ctrl Pts',(1.16698151947124,12.2,10.5979332765587));
#226769=CARTESIAN_POINT('Ctrl Pts',(1.16634466898602,12.2,10.6024896024933));
#226770=CARTESIAN_POINT('Ctrl Pts',(1.16569028676057,12.2,10.6070825977414));
#226771=CARTESIAN_POINT('Ctrl Pts',(1.16492684079125,12.2,10.6124410924757));
#226772=CARTESIAN_POINT('Ctrl Pts',(1.1641395360811,12.2,10.6178494954848));
#226773=CARTESIAN_POINT('Ctrl Pts',(1.16332791047032,12.2,10.6233069994883));
#226774=CARTESIAN_POINT('Ctrl Pts',(1.16263223141148,12.2,10.62798485982));
#226775=CARTESIAN_POINT('Ctrl Pts',(1.16191868894575,12.2,10.6326987919569));
#226776=CARTESIAN_POINT('Ctrl Pts',(1.16118699880644,12.2,10.6374482945329));
#226777=CARTESIAN_POINT('Ctrl Pts',(1.16057725700153,12.2,10.64140621349));
#226778=CARTESIAN_POINT('Ctrl Pts',(1.15995491519076,12.2,10.6453888339504));
#226779=CARTESIAN_POINT('Ctrl Pts',(1.15931981331644,12.2,10.6493958695047));
#226780=CARTESIAN_POINT('Ctrl Pts',(1.15868471144211,12.2,10.6534029050589));
#226781=CARTESIAN_POINT('Ctrl Pts',(1.15803685137552,12.2,10.6574343546349));
#226782=CARTESIAN_POINT('Ctrl Pts',(1.15737607623367,12.2,10.6614899359727));
#226783=CARTESIAN_POINT('Ctrl Pts',(1.15671530109181,12.2,10.6655455173105));
#226784=CARTESIAN_POINT('Ctrl Pts',(1.15604161051109,12.2,10.669625228811));
#226785=CARTESIAN_POINT('Ctrl Pts',(1.15535485523331,12.2,10.6737287912416));
#226786=CARTESIAN_POINT('Ctrl Pts',(1.15480545098114,12.2,10.677011641365));
#226787=CARTESIAN_POINT('Ctrl Pts',(1.15424768415023,12.2,10.6803097582206));
#226788=CARTESIAN_POINT('Ctrl Pts',(1.15368147867406,12.2,10.6836229962916));
#226789=CARTESIAN_POINT('Ctrl Pts',(1.15311527327504,12.2,10.6869362339113));
#226790=CARTESIAN_POINT('Ctrl Pts',(1.15254062861643,12.2,10.6902645947669));
#226791=CARTESIAN_POINT('Ctrl Pts',(1.15195747055037,12.2,10.693607937731));
#226792=CARTESIAN_POINT('Ctrl Pts',(1.15137431240486,12.2,10.6969512811505));
#226793=CARTESIAN_POINT('Ctrl Pts',(1.15078264042709,12.2,10.7003096065438));
#226794=CARTESIAN_POINT('Ctrl Pts',(1.1501823808935,12.2,10.7036827752848));
#226795=CARTESIAN_POINT('Ctrl Pts',(1.14958212144169,12.2,10.7070559435661));
#226796=CARTESIAN_POINT('Ctrl Pts',(1.14897327423266,12.2,10.7104439544066));
#226797=CARTESIAN_POINT('Ctrl Pts',(1.14835576628371,12.2,10.7138466712386));
#226798=CARTESIAN_POINT('Ctrl Pts',(1.14773825825063,12.2,10.7172493885341));
#226799=CARTESIAN_POINT('Ctrl Pts',(1.14711208941654,12.2,10.7206668099522));
#226800=CARTESIAN_POINT('Ctrl Pts',(1.1464771891828,12.2,10.7240988002563));
#226801=CARTESIAN_POINT('Ctrl Pts',(1.14584228903557,12.2,10.7275307900929));
#226802=CARTESIAN_POINT('Ctrl Pts',(1.14519865636321,12.2,10.730977347801));
#226803=CARTESIAN_POINT('Ctrl Pts',(1.14454622102823,12.2,10.7344383381838));
#226804=CARTESIAN_POINT('Ctrl Pts',(1.14373067679283,12.2,10.738764576516));
#226805=CARTESIAN_POINT('Ctrl Pts',(1.1429013799932,12.2,10.7431133673376));
#226806=CARTESIAN_POINT('Ctrl Pts',(1.14205819256337,12.2,10.7474844471975));
#226807=CARTESIAN_POINT('Ctrl Pts',(1.14138364258275,12.2,10.7509813112761));
#226808=CARTESIAN_POINT('Ctrl Pts',(1.14070020422257,12.2,10.7544924398559));
#226809=CARTESIAN_POINT('Ctrl Pts',(1.14000780814946,12.2,10.7580177015032));
#226810=CARTESIAN_POINT('Ctrl Pts',(1.13931541217069,12.2,10.7615429626701));
#226811=CARTESIAN_POINT('Ctrl Pts',(1.13861405966597,12.2,10.7650823550093));
#226812=CARTESIAN_POINT('Ctrl Pts',(1.13790368305797,12.2,10.7686357492179));
#226813=CARTESIAN_POINT('Ctrl Pts',(1.13719330635317,12.2,10.7721891439107));
#226814=CARTESIAN_POINT('Ctrl Pts',(1.13647390596397,12.2,10.7757565386328));
#226815=CARTESIAN_POINT('Ctrl Pts',(1.13574541592367,12.2,10.7793378035512));
#226816=CARTESIAN_POINT('Ctrl Pts',(1.13501692598263,12.2,10.7829190679815));
#226817=CARTESIAN_POINT('Ctrl Pts',(1.1342793461143,12.2,10.7865142026728));
#226818=CARTESIAN_POINT('Ctrl Pts',(1.13353261208329,12.2,10.7901230785013));
#226819=CARTESIAN_POINT('Ctrl Pts',(1.13278587795053,12.2,10.7937319548215));
#226820=CARTESIAN_POINT('Ctrl Pts',(1.13202998923243,12.2,10.7973545722149));
#226821=CARTESIAN_POINT('Ctrl Pts',(1.13126488191235,12.2,10.8009908017473));
#226822=CARTESIAN_POINT('Ctrl Pts',(1.13049977469651,12.2,10.8046270307843));
#226823=CARTESIAN_POINT('Ctrl Pts',(1.1297254491103,12.2,10.8082768718408));
#226824=CARTESIAN_POINT('Ctrl Pts',(1.12894184311976,12.2,10.811940197651));
#226825=CARTESIAN_POINT('Ctrl Pts',(1.12815823702246,12.2,10.8156035239603));
#226826=CARTESIAN_POINT('Ctrl Pts',(1.1273653499996,12.2,10.819280337104));
#226827=CARTESIAN_POINT('Ctrl Pts',(1.12656312000776,12.2,10.8229705080441));
#226828=CARTESIAN_POINT('Ctrl Pts',(1.12576089012523,12.2,10.8266606784815));
#226829=CARTESIAN_POINT('Ctrl Pts',(1.12494931716891,12.2,10.8303642080502));
#226830=CARTESIAN_POINT('Ctrl Pts',(1.12412834062587,12.2,10.8340809711339));
#226831=CARTESIAN_POINT('Ctrl Pts',(1.12330736397098,12.2,10.837797734724));
#226832=CARTESIAN_POINT('Ctrl Pts',(1.12247698413465,12.2,10.8415277328543));
#226833=CARTESIAN_POINT('Ctrl Pts',(1.12163714019998,12.2,10.845270839225));
#226834=CARTESIAN_POINT('Ctrl Pts',(1.12079729626531,12.2,10.8490139455957));
#226835=CARTESIAN_POINT('Ctrl Pts',(1.11994798999345,12.2,10.8527701627928));
#226836=CARTESIAN_POINT('Ctrl Pts',(1.11908916066789,12.2,10.8565393663329));
#226837=CARTESIAN_POINT('Ctrl Pts',(1.11801562418647,12.2,10.8612508699876));
#226838=CARTESIAN_POINT('Ctrl Pts',(1.11692720788392,12.2,10.8659826645702));
#226839=CARTESIAN_POINT('Ctrl Pts',(1.1158238006443,12.2,10.8707345116201));
#226840=CARTESIAN_POINT('Ctrl Pts',(1.11494107470829,12.2,10.8745359898815));
#226841=CARTESIAN_POINT('Ctrl Pts',(1.11404875380191,12.2,10.8783503023303));
#226842=CARTESIAN_POINT('Ctrl Pts',(1.11314678180832,12.2,10.8821773273166));
#226843=CARTESIAN_POINT('Ctrl Pts',(1.11224480981472,12.2,10.8860043523029));
#226844=CARTESIAN_POINT('Ctrl Pts',(1.11133318634499,12.2,10.8898440902047));
#226845=CARTESIAN_POINT('Ctrl Pts',(1.11041185384934,12.2,10.8936964211382));
#226846=CARTESIAN_POINT('Ctrl Pts',(1.10949052147921,12.2,10.8975487515468));
#226847=CARTESIAN_POINT('Ctrl Pts',(1.1085594841224,12.2,10.9014136742356));
#226848=CARTESIAN_POINT('Ctrl Pts',(1.10761868175062,12.2,10.905291070714));
#226849=CARTESIAN_POINT('Ctrl Pts',(1.10667787925066,12.2,10.9091684677206));
#226850=CARTESIAN_POINT('Ctrl Pts',(1.10572731496296,12.2,10.9130583395629));
#226851=CARTESIAN_POINT('Ctrl Pts',(1.10476693357629,12.2,10.916960565888));
#226852=CARTESIAN_POINT('Ctrl Pts',(1.10380655232046,12.2,10.9208627916813));
#226853=CARTESIAN_POINT('Ctrl Pts',(1.10283635341036,12.2,10.9247773727592));
#226854=CARTESIAN_POINT('Ctrl Pts',(1.10185628438001,12.2,10.9287041919374));
#226855=CARTESIAN_POINT('Ctrl Pts',(1.10063119799192,12.2,10.9336127163114));
#226856=CARTESIAN_POINT('Ctrl Pts',(1.09939069045902,12.2,10.9385403633886));
#226857=CARTESIAN_POINT('Ctrl Pts',(1.09813465580703,12.2,10.9434869051932));
#226858=CARTESIAN_POINT('Ctrl Pts',(1.09712982803067,12.2,10.9474441388526));
#226859=CARTESIAN_POINT('Ctrl Pts',(1.09611506658692,12.2,10.9514134639803));
#226860=CARTESIAN_POINT('Ctrl Pts',(1.09509031536789,12.2,10.9553947677861));
#226861=CARTESIAN_POINT('Ctrl Pts',(1.09406556428849,12.2,10.9593760710494));
#226862=CARTESIAN_POINT('Ctrl Pts',(1.09303082649089,12.2,10.9633693507425));
#226863=CARTESIAN_POINT('Ctrl Pts',(1.09198605007697,12.2,10.9673744939143));
#226864=CARTESIAN_POINT('Ctrl Pts',(1.09094127352069,12.2,10.9713796376318));
#226865=CARTESIAN_POINT('Ctrl Pts',(1.08988645932708,12.2,10.9753966439952));
#226866=CARTESIAN_POINT('Ctrl Pts',(1.08882155671283,12.2,10.9794253996044));
#226867=CARTESIAN_POINT('Ctrl Pts',(1.08775665424368,12.2,10.9834541546647));
#226868=CARTESIAN_POINT('Ctrl Pts',(1.08668166219425,12.2,10.9874946584668));
#226869=CARTESIAN_POINT('Ctrl Pts',(1.08559653367406,12.2,10.9915467991703));
#226870=CARTESIAN_POINT('Ctrl Pts',(1.08424012291293,12.2,10.9966119754639));
#226871=CARTESIAN_POINT('Ctrl Pts',(1.08286787265651,12.2,11.001695332434));
#226872=CARTESIAN_POINT('Ctrl Pts',(1.08147968786568,12.2,11.0067966526414));
#226873=CARTESIAN_POINT('Ctrl Pts',(1.08036913997248,12.2,11.0108777090298));
#226874=CARTESIAN_POINT('Ctrl Pts',(1.07924839458084,12.2,11.0149702612667));
#226875=CARTESIAN_POINT('Ctrl Pts',(1.07811740340743,12.2,11.0190741996022));
#226876=CARTESIAN_POINT('Ctrl Pts',(1.07698641238811,12.2,11.0231781373786));
#226877=CARTESIAN_POINT('Ctrl Pts',(1.07584517736287,12.2,11.0272934599305));
#226878=CARTESIAN_POINT('Ctrl Pts',(1.07469364840036,12.2,11.0314200574095));
#226879=CARTESIAN_POINT('Ctrl Pts',(1.07296635472125,12.2,11.0376099544714));
#226880=CARTESIAN_POINT('Ctrl Pts',(1.07121590622989,12.2,11.0438252199217));
#226881=CARTESIAN_POINT('Ctrl Pts',(1.06944214454831,12.2,11.0500654854301));
#226882=CARTESIAN_POINT('Ctrl Pts',(1.0682596369217,12.2,11.0542256618689));
#226883=CARTESIAN_POINT('Ctrl Pts',(1.06706676838811,12.2,11.0583969486063));
#226884=CARTESIAN_POINT('Ctrl Pts',(1.06586349459826,12.2,11.0625792383748));
#226885=CARTESIAN_POINT('Ctrl Pts',(1.06466022064445,12.2,11.0667615287132));
#226886=CARTESIAN_POINT('Ctrl Pts',(1.06344654021219,12.2,11.0709548208811));
#226887=CARTESIAN_POINT('Ctrl Pts',(1.06222241030563,12.2,11.0751590088767));
#226888=CARTESIAN_POINT('Ctrl Pts',(1.06099828056586,12.2,11.0793631962996));
#226889=CARTESIAN_POINT('Ctrl Pts',(1.05976370092697,12.2,11.0835782779285));
#226890=CARTESIAN_POINT('Ctrl Pts',(1.05851862791834,12.2,11.0878041471379));
#226891=CARTESIAN_POINT('Ctrl Pts',(1.05727355474007,12.2,11.0920300169231));
#226892=CARTESIAN_POINT('Ctrl Pts',(1.05601798832163,12.2,11.0962666755512));
#226893=CARTESIAN_POINT('Ctrl Pts',(1.05475188569638,12.2,11.1005140148389));
#226894=CARTESIAN_POINT('Ctrl Pts',(1.05348578324364,12.2,11.104761353548));
#226895=CARTESIAN_POINT('Ctrl Pts',(1.05220914389209,12.2,11.1090193758478));
#226896=CARTESIAN_POINT('Ctrl Pts',(1.05092192621171,12.2,11.1132879726556));
#226897=CARTESIAN_POINT('Ctrl Pts',(1.04995651290758,12.2,11.1164894204069));
#226898=CARTESIAN_POINT('Ctrl Pts',(1.04898514899338,12.2,11.119696817267));
#226899=CARTESIAN_POINT('Ctrl Pts',(1.04800781769637,12.2,11.1229101193161));
#226900=CARTESIAN_POINT('Ctrl Pts',(1.04703048622182,12.2,11.126123421949));
#226901=CARTESIAN_POINT('Ctrl Pts',(1.0460471864789,12.2,11.1293426293168));
#226902=CARTESIAN_POINT('Ctrl Pts',(1.04505790150098,12.2,11.132567697453));
#226903=CARTESIAN_POINT('Ctrl Pts',(1.04406861670277,12.2,11.1357927650033));
#226904=CARTESIAN_POINT('Ctrl Pts',(1.04307334650489,12.2,11.1390236930866));
#226905=CARTESIAN_POINT('Ctrl Pts',(1.04207207462408,12.2,11.1422604386362));
#226906=CARTESIAN_POINT('Ctrl Pts',(1.04107080274327,12.2,11.1454971841858));
#226907=CARTESIAN_POINT('Ctrl Pts',(1.04006352811688,12.2,11.1487397468395));
#226908=CARTESIAN_POINT('Ctrl Pts',(1.03905023431573,12.2,11.1519880820279));
#226909=CARTESIAN_POINT('Ctrl Pts',(1.03803694051458,12.2,11.1552364172163));
#226910=CARTESIAN_POINT('Ctrl Pts',(1.03701762670163,12.2,11.158490526884));
#226911=CARTESIAN_POINT('Ctrl Pts',(1.03599227744259,12.2,11.1617503659886));
#226912=CARTESIAN_POINT('Ctrl Pts',(1.03496692818354,12.2,11.1650102050933));
#226913=CARTESIAN_POINT('Ctrl Pts',(1.03393554260807,12.2,11.1682757738462));
#226914=CARTESIAN_POINT('Ctrl Pts',(1.03289810481297,12.2,11.1715470293935));
#226915=CARTESIAN_POINT('Ctrl Pts',(1.03186066701787,12.2,11.1748182849407));
#226916=CARTESIAN_POINT('Ctrl Pts',(1.03081717702315,12.2,11.1780952270377));
#226917=CARTESIAN_POINT('Ctrl Pts',(1.02976761772878,12.2,11.1813778135844));
#226918=CARTESIAN_POINT('Ctrl Pts',(1.02871805824375,12.2,11.1846604007273));
#226919=CARTESIAN_POINT('Ctrl Pts',(1.027662429207,12.2,11.1879486312052));
#226920=CARTESIAN_POINT('Ctrl Pts',(1.02660071576019,12.2,11.1912424624347));
#226921=CARTESIAN_POINT('Ctrl Pts',(1.02553900250626,12.2,11.1945362930658));
#226922=CARTESIAN_POINT('Ctrl Pts',(1.0244712051075,12.2,11.1978357251937));
#226923=CARTESIAN_POINT('Ctrl Pts',(1.02339730580049,12.2,11.2011407159061));
#226924=CARTESIAN_POINT('Ctrl Pts',(1.02196544012284,12.2,11.2055473699891));
#226925=CARTESIAN_POINT('Ctrl Pts',(1.02052272801306,12.2,11.2099639052174));
#226926=CARTESIAN_POINT('Ctrl Pts',(1.01906913307705,12.2,11.2143902211882));
#226927=CARTESIAN_POINT('Ctrl Pts',(1.01797893682553,12.2,11.2177099583171));
#226928=CARTESIAN_POINT('Ctrl Pts',(1.01688261823276,12.2,11.2210351974956));
#226929=CARTESIAN_POINT('Ctrl Pts',(1.01578016248198,12.2,11.2243658970405));
#226930=CARTESIAN_POINT('Ctrl Pts',(1.01467770653093,12.2,11.2276965971905));
#226931=CARTESIAN_POINT('Ctrl Pts',(1.01356911398648,12.2,11.2310327560754));
#226932=CARTESIAN_POINT('Ctrl Pts',(1.01245436803196,12.2,11.2343743337284));
#226933=CARTESIAN_POINT('Ctrl Pts',(1.01133962227995,12.2,11.2377159107744));
#226934=CARTESIAN_POINT('Ctrl Pts',(1.01021872309793,12.2,11.241062905319));
#226935=CARTESIAN_POINT('Ctrl Pts',(1.0090916567902,12.2,11.2444152756569));
#226936=CARTESIAN_POINT('Ctrl Pts',(1.00758890178147,12.2,11.2488851025712));
#226937=CARTESIAN_POINT('Ctrl Pts',(1.00607518097694,12.2,11.2533644885868));
#226938=CARTESIAN_POINT('Ctrl Pts',(1.00455046065786,12.2,11.2578533326081));
#226939=CARTESIAN_POINT('Ctrl Pts',(1.00340692036662,12.2,11.261219965777));
#226940=CARTESIAN_POINT('Ctrl Pts',(1.00225719220913,12.2,11.2645919195371));
#226941=CARTESIAN_POINT('Ctrl Pts',(1.00110126150197,12.2,11.2679691527054));
#226942=CARTESIAN_POINT('Ctrl Pts',(0.999945330584818,12.2,11.2713463864872));
#226943=CARTESIAN_POINT('Ctrl Pts',(0.998783197665939,12.2,11.2747289007621));
#226944=CARTESIAN_POINT('Ctrl Pts',(0.99761484728694,12.2,11.2781166529635));
#226945=CARTESIAN_POINT('Ctrl Pts',(0.996446497120191,12.2,11.2815044045495));
#226946=CARTESIAN_POINT('Ctrl Pts',(0.995271930528823,12.2,11.2848973937601));
#226947=CARTESIAN_POINT('Ctrl Pts',(0.994091132362839,12.2,11.2882955808454));
#226948=CARTESIAN_POINT('Ctrl Pts',(0.992910334196854,12.2,11.2916937679308));
#226949=CARTESIAN_POINT('Ctrl Pts',(0.991723305177649,12.2,11.2950971526781));
#226950=CARTESIAN_POINT('Ctrl Pts',(0.990530030007237,12.2,11.298505694278));
#226951=CARTESIAN_POINT('Ctrl Pts',(0.98893899651895,12.2,11.3030504162049));
#226952=CARTESIAN_POINT('Ctrl Pts',(0.987336860464056,12.2,11.3076043057307));
#226953=CARTESIAN_POINT('Ctrl Pts',(0.985723588263753,12.2,11.3121672657456));
#226954=CARTESIAN_POINT('Ctrl Pts',(0.984513633838765,12.2,11.3155894865339));
#226955=CARTESIAN_POINT('Ctrl Pts',(0.983297415128669,12.2,11.3190168102487));
#226956=CARTESIAN_POINT('Ctrl Pts',(0.982074918700141,12.2,11.3224491964982));
#226957=CARTESIAN_POINT('Ctrl Pts',(0.980444923832249,12.2,11.3270257104583));
#226958=CARTESIAN_POINT('Ctrl Pts',(0.97880376851027,12.2,11.33161122437));
#226959=CARTESIAN_POINT('Ctrl Pts',(0.977151420868294,12.2,11.3362056423828));
#226960=CARTESIAN_POINT('Ctrl Pts',(0.975912160080528,12.2,11.3396514560488));
#226961=CARTESIAN_POINT('Ctrl Pts',(0.974666602375131,12.2,11.3431022787349));
#226962=CARTESIAN_POINT('Ctrl Pts',(0.973414736525461,12.2,11.3465580705731));
#226963=CARTESIAN_POINT('Ctrl Pts',(0.972162870675792,12.2,11.3500138624113));
#226964=CARTESIAN_POINT('Ctrl Pts',(0.970904695462171,12.2,11.353474623571));
#226965=CARTESIAN_POINT('Ctrl Pts',(0.969640197300644,12.2,11.3569403127361));
#226966=CARTESIAN_POINT('Ctrl Pts',(0.968375698909399,12.2,11.3604060025308));
#226967=CARTESIAN_POINT('Ctrl Pts',(0.967104877574688,12.2,11.3638766215186));
#226968=CARTESIAN_POINT('Ctrl Pts',(0.965827721179895,12.2,11.367352130316));
#226969=CARTESIAN_POINT('Ctrl Pts',(0.964124846373533,12.2,11.3719861409935));
#226970=CARTESIAN_POINT('Ctrl Pts',(0.962410709804703,12.2,11.3766288450867));
#226971=CARTESIAN_POINT('Ctrl Pts',(0.960685278390935,12.2,11.3812801490948));
#226972=CARTESIAN_POINT('Ctrl Pts',(0.959391204771838,12.2,11.3847686272593));
#226973=CARTESIAN_POINT('Ctrl Pts',(0.95809078006983,12.2,11.3882619435928));
#226974=CARTESIAN_POINT('Ctrl Pts',(0.956783988802754,12.2,11.3917600568065));
#226975=CARTESIAN_POINT('Ctrl Pts',(0.955477197535678,12.2,11.3952581700203));
#226976=CARTESIAN_POINT('Ctrl Pts',(0.954164039455502,12.2,11.39876107833));
#226977=CARTESIAN_POINT('Ctrl Pts',(0.952844504295974,12.2,11.4022687450353));
#226978=CARTESIAN_POINT('Ctrl Pts',(0.951524968896731,12.2,11.4057764123778));
#226979=CARTESIAN_POINT('Ctrl Pts',(0.950199055770689,12.2,11.4092888386549));
#226980=CARTESIAN_POINT('Ctrl Pts',(0.948866752951208,12.2,11.412805988));
#226981=CARTESIAN_POINT('Ctrl Pts',(0.947534450373763,12.2,11.4163231367062));
#226982=CARTESIAN_POINT('Ctrl Pts',(0.946195759771612,12.2,11.4198450094288));
#226983=CARTESIAN_POINT('Ctrl Pts',(0.944850667069934,12.2,11.4233715654261));
#226984=CARTESIAN_POINT('Ctrl Pts',(0.943505574368256,12.2,11.4268981214234));
#226985=CARTESIAN_POINT('Ctrl Pts',(0.942154079472279,12.2,11.4304293594156));
#226986=CARTESIAN_POINT('Ctrl Pts',(0.940796167723754,12.2,11.4339652325115));
#226987=CARTESIAN_POINT('Ctrl Pts',(0.938532981393982,12.2,11.4398583545522));
#226988=CARTESIAN_POINT('Ctrl Pts',(0.936251965069451,12.2,11.4457643374802));
#226989=CARTESIAN_POINT('Ctrl Pts',(0.933953084118917,12.2,11.4516830612001));
#226990=CARTESIAN_POINT('Ctrl Pts',(0.932573755598712,12.2,11.4552342953029));
#226991=CARTESIAN_POINT('Ctrl Pts',(0.931187998930692,12.2,11.4587901206197));
#226992=CARTESIAN_POINT('Ctrl Pts',(0.929795807999944,12.2,11.462350533));
#226993=CARTESIAN_POINT('Origin',(-5.66257110645729E-14,15.2,-1.77635683940025E-14));
#226994=CARTESIAN_POINT('',(-0.292001929325956,15.2,10.370890023736));
#226995=CARTESIAN_POINT('',(-0.292001929325956,12.2,10.370890023736));
#226996=CARTESIAN_POINT('',(-0.292001929000056,15.2,10.370890024));
#226997=CARTESIAN_POINT('Origin',(-5.66257110645729E-14,12.2,-1.77635683940025E-14));
#226998=CARTESIAN_POINT('Origin',(-5.66257110645729E-14,15.2,-1.77635683940025E-14));
#226999=CARTESIAN_POINT('Origin',(-5.66257110645729E-14,15.2,-1.77635683940025E-14));
#227000=CARTESIAN_POINT('',(-0.710930735000056,15.2,11.478004073));
#227001=CARTESIAN_POINT('',(-1.09337743000006,15.2,11.447904865));
#227002=CARTESIAN_POINT('Origin',(-5.66257110645729E-14,15.2,-1.77635683940025E-14));
#227003=CARTESIAN_POINT('',(-1.09337743000006,12.2,11.447904865));
#227004=CARTESIAN_POINT('',(-1.09337743000006,15.2,11.447904865));
#227005=CARTESIAN_POINT('',(-0.710930735000056,12.2,11.478004073));
#227006=CARTESIAN_POINT('Origin',(-5.66257110645729E-14,12.2,-1.77635683940025E-14));
#227007=CARTESIAN_POINT('',(-0.710930735000056,15.2,11.478004073));
#227008=CARTESIAN_POINT('Ctrl Pts',(-0.292001930000056,15.2,10.370890024));
#227009=CARTESIAN_POINT('Ctrl Pts',(-0.292001930000056,11.6,10.370890024));
#227010=CARTESIAN_POINT('Ctrl Pts',(-0.292021796000055,15.2,10.371063246));
#227011=CARTESIAN_POINT('Ctrl Pts',(-0.292021796000055,11.6,10.371063246));
#227012=CARTESIAN_POINT('Ctrl Pts',(-0.292062309000055,15.2,10.371415731));
#227013=CARTESIAN_POINT('Ctrl Pts',(-0.292062309000055,11.6,10.371415731));
#227014=CARTESIAN_POINT('Ctrl Pts',(-0.292123962000056,15.2,10.3719498));
#227015=CARTESIAN_POINT('Ctrl Pts',(-0.292123962000056,11.6,10.3719498));
#227016=CARTESIAN_POINT('Ctrl Pts',(-0.292207548000055,15.2,10.372669177));
#227017=CARTESIAN_POINT('Ctrl Pts',(-0.292207548000055,11.6,10.372669177));
#227018=CARTESIAN_POINT('Ctrl Pts',(-0.292314181000056,15.2,10.373578975));
#227019=CARTESIAN_POINT('Ctrl Pts',(-0.292314181000056,11.6,10.373578975));
#227020=CARTESIAN_POINT('Ctrl Pts',(-0.292423470000056,15.2,10.374503411));
#227021=CARTESIAN_POINT('Ctrl Pts',(-0.292423470000056,11.6,10.374503411));
#227022=CARTESIAN_POINT('Ctrl Pts',(-0.292534812000056,15.2,10.375437185));
#227023=CARTESIAN_POINT('Ctrl Pts',(-0.292534812000056,11.6,10.375437185));
#227024=CARTESIAN_POINT('Ctrl Pts',(-0.292648223000055,15.2,10.376380267));
#227025=CARTESIAN_POINT('Ctrl Pts',(-0.292648223000055,11.6,10.376380267));
#227026=CARTESIAN_POINT('Ctrl Pts',(-0.292763718000056,15.2,10.377332628));
#227027=CARTESIAN_POINT('Ctrl Pts',(-0.292763718000056,11.6,10.377332628));
#227028=CARTESIAN_POINT('Ctrl Pts',(-0.292881311000055,15.2,10.37829424));
#227029=CARTESIAN_POINT('Ctrl Pts',(-0.292881311000055,11.6,10.37829424));
#227030=CARTESIAN_POINT('Ctrl Pts',(-0.293001016000056,15.2,10.379265074));
#227031=CARTESIAN_POINT('Ctrl Pts',(-0.293001016000056,11.6,10.379265074));
#227032=CARTESIAN_POINT('Ctrl Pts',(-0.293122847000056,15.2,10.380245102));
#227033=CARTESIAN_POINT('Ctrl Pts',(-0.293122847000056,11.6,10.380245102));
#227034=CARTESIAN_POINT('Ctrl Pts',(-0.293246820000055,15.2,10.381234296));
#227035=CARTESIAN_POINT('Ctrl Pts',(-0.293246820000055,11.6,10.381234296));
#227036=CARTESIAN_POINT('Ctrl Pts',(-0.293372949000055,15.2,10.382232628));
#227037=CARTESIAN_POINT('Ctrl Pts',(-0.293372949000055,11.6,10.382232628));
#227038=CARTESIAN_POINT('Ctrl Pts',(-0.293501249000055,15.2,10.383240069));
#227039=CARTESIAN_POINT('Ctrl Pts',(-0.293501249000055,11.6,10.383240069));
#227040=CARTESIAN_POINT('Ctrl Pts',(-0.293631732000056,15.2,10.384256592));
#227041=CARTESIAN_POINT('Ctrl Pts',(-0.293631732000056,11.6,10.384256592));
#227042=CARTESIAN_POINT('Ctrl Pts',(-0.293764414000056,15.2,10.385282169));
#227043=CARTESIAN_POINT('Ctrl Pts',(-0.293764414000056,11.6,10.385282169));
#227044=CARTESIAN_POINT('Ctrl Pts',(-0.293899307000055,15.2,10.38631677));
#227045=CARTESIAN_POINT('Ctrl Pts',(-0.293899307000055,11.6,10.38631677));
#227046=CARTESIAN_POINT('Ctrl Pts',(-0.294036428000056,15.2,10.387360372));
#227047=CARTESIAN_POINT('Ctrl Pts',(-0.294036428000056,11.6,10.387360372));
#227048=CARTESIAN_POINT('Ctrl Pts',(-0.294175788000055,15.2,10.388412944));
#227049=CARTESIAN_POINT('Ctrl Pts',(-0.294175788000055,11.6,10.388412944));
#227050=CARTESIAN_POINT('Ctrl Pts',(-0.294317401000056,15.2,10.389474461));
#227051=CARTESIAN_POINT('Ctrl Pts',(-0.294317401000056,11.6,10.389474461));
#227052=CARTESIAN_POINT('Ctrl Pts',(-0.294461282000055,15.2,10.390544895));
#227053=CARTESIAN_POINT('Ctrl Pts',(-0.294461282000055,11.6,10.390544895));
#227054=CARTESIAN_POINT('Ctrl Pts',(-0.294607445000056,15.2,10.391624218));
#227055=CARTESIAN_POINT('Ctrl Pts',(-0.294607445000056,11.6,10.391624218));
#227056=CARTESIAN_POINT('Ctrl Pts',(-0.294755901000056,15.2,10.392712405));
#227057=CARTESIAN_POINT('Ctrl Pts',(-0.294755901000056,11.6,10.392712405));
#227058=CARTESIAN_POINT('Ctrl Pts',(-0.294906666000055,15.2,10.393809428));
#227059=CARTESIAN_POINT('Ctrl Pts',(-0.294906666000055,11.6,10.393809428));
#227060=CARTESIAN_POINT('Ctrl Pts',(-0.295059753000055,15.2,10.39491526));
#227061=CARTESIAN_POINT('Ctrl Pts',(-0.295059753000055,11.6,10.39491526));
#227062=CARTESIAN_POINT('Ctrl Pts',(-0.295215174000055,15.2,10.396029876));
#227063=CARTESIAN_POINT('Ctrl Pts',(-0.295215174000055,11.6,10.396029876));
#227064=CARTESIAN_POINT('Ctrl Pts',(-0.295372942000055,15.2,10.397153247));
#227065=CARTESIAN_POINT('Ctrl Pts',(-0.295372942000055,11.6,10.397153247));
#227066=CARTESIAN_POINT('Ctrl Pts',(-0.295533072000056,15.2,10.398285351));
#227067=CARTESIAN_POINT('Ctrl Pts',(-0.295533072000056,11.6,10.398285351));
#227068=CARTESIAN_POINT('Ctrl Pts',(-0.295695577000057,15.2,10.399426157));
#227069=CARTESIAN_POINT('Ctrl Pts',(-0.295695577000057,11.6,10.399426157));
#227070=CARTESIAN_POINT('Ctrl Pts',(-0.295860468000055,15.2,10.400575642));
#227071=CARTESIAN_POINT('Ctrl Pts',(-0.295860468000055,11.6,10.400575642));
#227072=CARTESIAN_POINT('Ctrl Pts',(-0.296027759000056,15.2,10.401733779));
#227073=CARTESIAN_POINT('Ctrl Pts',(-0.296027759000056,11.6,10.401733779));
#227074=CARTESIAN_POINT('Ctrl Pts',(-0.296197463000055,15.2,10.402900543));
#227075=CARTESIAN_POINT('Ctrl Pts',(-0.296197463000055,11.6,10.402900543));
#227076=CARTESIAN_POINT('Ctrl Pts',(-0.296369593000056,15.2,10.404075907));
#227077=CARTESIAN_POINT('Ctrl Pts',(-0.296369593000056,11.6,10.404075907));
#227078=CARTESIAN_POINT('Ctrl Pts',(-0.296544162000056,15.2,10.405259846));
#227079=CARTESIAN_POINT('Ctrl Pts',(-0.296544162000056,11.6,10.405259846));
#227080=CARTESIAN_POINT('Ctrl Pts',(-0.296721182000056,15.2,10.406452335));
#227081=CARTESIAN_POINT('Ctrl Pts',(-0.296721182000056,11.6,10.406452335));
#227082=CARTESIAN_POINT('Ctrl Pts',(-0.296900665000056,15.2,10.407653348));
#227083=CARTESIAN_POINT('Ctrl Pts',(-0.296900665000056,11.6,10.407653348));
#227084=CARTESIAN_POINT('Ctrl Pts',(-0.297082625000057,15.2,10.408862859));
#227085=CARTESIAN_POINT('Ctrl Pts',(-0.297082625000057,11.6,10.408862859));
#227086=CARTESIAN_POINT('Ctrl Pts',(-0.297267073000055,15.2,10.410080845));
#227087=CARTESIAN_POINT('Ctrl Pts',(-0.297267073000055,11.6,10.410080845));
#227088=CARTESIAN_POINT('Ctrl Pts',(-0.297454022000055,15.2,10.411307279));
#227089=CARTESIAN_POINT('Ctrl Pts',(-0.297454022000055,11.6,10.411307279));
#227090=CARTESIAN_POINT('Ctrl Pts',(-0.297643484000056,15.2,10.412542136));
#227091=CARTESIAN_POINT('Ctrl Pts',(-0.297643484000056,11.6,10.412542136));
#227092=CARTESIAN_POINT('Ctrl Pts',(-0.297835473000055,15.2,10.413785393));
#227093=CARTESIAN_POINT('Ctrl Pts',(-0.297835473000055,11.6,10.413785393));
#227094=CARTESIAN_POINT('Ctrl Pts',(-0.298029998000056,15.2,10.415037024));
#227095=CARTESIAN_POINT('Ctrl Pts',(-0.298029998000056,11.6,10.415037024));
#227096=CARTESIAN_POINT('Ctrl Pts',(-0.298227074000056,15.2,10.416297004));
#227097=CARTESIAN_POINT('Ctrl Pts',(-0.298227074000056,11.6,10.416297004));
#227098=CARTESIAN_POINT('Ctrl Pts',(-0.298426711000056,15.2,10.41756531));
#227099=CARTESIAN_POINT('Ctrl Pts',(-0.298426711000056,11.6,10.41756531));
#227100=CARTESIAN_POINT('Ctrl Pts',(-0.298628923000056,15.2,10.418841915));
#227101=CARTESIAN_POINT('Ctrl Pts',(-0.298628923000056,11.6,10.418841915));
#227102=CARTESIAN_POINT('Ctrl Pts',(-0.298833720000056,15.2,10.420126797));
#227103=CARTESIAN_POINT('Ctrl Pts',(-0.298833720000056,11.6,10.420126797));
#227104=CARTESIAN_POINT('Ctrl Pts',(-0.299041114000056,15.2,10.42141993));
#227105=CARTESIAN_POINT('Ctrl Pts',(-0.299041114000056,11.6,10.42141993));
#227106=CARTESIAN_POINT('Ctrl Pts',(-0.299251119000056,15.2,10.422721291));
#227107=CARTESIAN_POINT('Ctrl Pts',(-0.299251119000056,11.6,10.422721291));
#227108=CARTESIAN_POINT('Ctrl Pts',(-0.299463743000056,15.2,10.424030857));
#227109=CARTESIAN_POINT('Ctrl Pts',(-0.299463743000056,11.6,10.424030857));
#227110=CARTESIAN_POINT('Ctrl Pts',(-0.299679001000056,15.2,10.425348601));
#227111=CARTESIAN_POINT('Ctrl Pts',(-0.299679001000056,11.6,10.425348601));
#227112=CARTESIAN_POINT('Ctrl Pts',(-0.299896903000055,15.2,10.426674502));
#227113=CARTESIAN_POINT('Ctrl Pts',(-0.299896903000055,11.6,10.426674502));
#227114=CARTESIAN_POINT('Ctrl Pts',(-0.300117461000056,15.2,10.428008535));
#227115=CARTESIAN_POINT('Ctrl Pts',(-0.300117461000056,11.6,10.428008535));
#227116=CARTESIAN_POINT('Ctrl Pts',(-0.300340687000055,15.2,10.429350676));
#227117=CARTESIAN_POINT('Ctrl Pts',(-0.300340687000055,11.6,10.429350676));
#227118=CARTESIAN_POINT('Ctrl Pts',(-0.300566590000055,15.2,10.430700903));
#227119=CARTESIAN_POINT('Ctrl Pts',(-0.300566590000055,11.6,10.430700903));
#227120=CARTESIAN_POINT('Ctrl Pts',(-0.300795185000055,15.2,10.432059191));
#227121=CARTESIAN_POINT('Ctrl Pts',(-0.300795185000055,11.6,10.432059191));
#227122=CARTESIAN_POINT('Ctrl Pts',(-0.301026480000056,15.2,10.433425517));
#227123=CARTESIAN_POINT('Ctrl Pts',(-0.301026480000056,11.6,10.433425517));
#227124=CARTESIAN_POINT('Ctrl Pts',(-0.301260488000056,15.2,10.434799857));
#227125=CARTESIAN_POINT('Ctrl Pts',(-0.301260488000056,11.6,10.434799857));
#227126=CARTESIAN_POINT('Ctrl Pts',(-0.301497220000057,15.2,10.43618219));
#227127=CARTESIAN_POINT('Ctrl Pts',(-0.301497220000057,11.6,10.43618219));
#227128=CARTESIAN_POINT('Ctrl Pts',(-0.301736686000057,15.2,10.437572491));
#227129=CARTESIAN_POINT('Ctrl Pts',(-0.301736686000057,11.6,10.437572491));
#227130=CARTESIAN_POINT('Ctrl Pts',(-0.301978899000056,15.2,10.438970738));
#227131=CARTESIAN_POINT('Ctrl Pts',(-0.301978899000056,11.6,10.438970738));
#227132=CARTESIAN_POINT('Ctrl Pts',(-0.302223868000056,15.2,10.440376907));
#227133=CARTESIAN_POINT('Ctrl Pts',(-0.302223868000056,11.6,10.440376907));
#227134=CARTESIAN_POINT('Ctrl Pts',(-0.302471605000055,15.2,10.441790977));
#227135=CARTESIAN_POINT('Ctrl Pts',(-0.302471605000055,11.6,10.441790977));
#227136=CARTESIAN_POINT('Ctrl Pts',(-0.302722121000055,15.2,10.443212923));
#227137=CARTESIAN_POINT('Ctrl Pts',(-0.302722121000055,11.6,10.443212923));
#227138=CARTESIAN_POINT('Ctrl Pts',(-0.302975427000056,15.2,10.444642724));
#227139=CARTESIAN_POINT('Ctrl Pts',(-0.302975427000056,11.6,10.444642724));
#227140=CARTESIAN_POINT('Ctrl Pts',(-0.303231532000057,15.2,10.446080358));
#227141=CARTESIAN_POINT('Ctrl Pts',(-0.303231532000057,11.6,10.446080358));
#227142=CARTESIAN_POINT('Ctrl Pts',(-0.303490448000057,15.2,10.4475258));
#227143=CARTESIAN_POINT('Ctrl Pts',(-0.303490448000057,11.6,10.4475258));
#227144=CARTESIAN_POINT('Ctrl Pts',(-0.303752187000056,15.2,10.44897903));
#227145=CARTESIAN_POINT('Ctrl Pts',(-0.303752187000056,11.6,10.44897903));
#227146=CARTESIAN_POINT('Ctrl Pts',(-0.304016757000056,15.2,10.450440024));
#227147=CARTESIAN_POINT('Ctrl Pts',(-0.304016757000056,11.6,10.450440024));
#227148=CARTESIAN_POINT('Ctrl Pts',(-0.304284170000055,15.2,10.451908761));
#227149=CARTESIAN_POINT('Ctrl Pts',(-0.304284170000055,11.6,10.451908761));
#227150=CARTESIAN_POINT('Ctrl Pts',(-0.304554437000055,15.2,10.453385219));
#227151=CARTESIAN_POINT('Ctrl Pts',(-0.304554437000055,11.6,10.453385219));
#227152=CARTESIAN_POINT('Ctrl Pts',(-0.304827566000055,15.2,10.454869375));
#227153=CARTESIAN_POINT('Ctrl Pts',(-0.304827566000055,11.6,10.454869375));
#227154=CARTESIAN_POINT('Ctrl Pts',(-0.305103570000057,15.2,10.456361207));
#227155=CARTESIAN_POINT('Ctrl Pts',(-0.305103570000057,11.6,10.456361207));
#227156=CARTESIAN_POINT('Ctrl Pts',(-0.305382458000055,15.2,10.457860694));
#227157=CARTESIAN_POINT('Ctrl Pts',(-0.305382458000055,11.6,10.457860694));
#227158=CARTESIAN_POINT('Ctrl Pts',(-0.305664241000055,15.2,10.459367814));
#227159=CARTESIAN_POINT('Ctrl Pts',(-0.305664241000055,11.6,10.459367814));
#227160=CARTESIAN_POINT('Ctrl Pts',(-0.305948929000056,15.2,10.460882546));
#227161=CARTESIAN_POINT('Ctrl Pts',(-0.305948929000056,11.6,10.460882546));
#227162=CARTESIAN_POINT('Ctrl Pts',(-0.306236530000056,15.2,10.462404866));
#227163=CARTESIAN_POINT('Ctrl Pts',(-0.306236530000056,11.6,10.462404866));
#227164=CARTESIAN_POINT('Ctrl Pts',(-0.306527058000056,15.2,10.463934755));
#227165=CARTESIAN_POINT('Ctrl Pts',(-0.306527058000056,11.6,10.463934755));
#227166=CARTESIAN_POINT('Ctrl Pts',(-0.306820521000055,15.2,10.465472191));
#227167=CARTESIAN_POINT('Ctrl Pts',(-0.306820521000055,11.6,10.465472191));
#227168=CARTESIAN_POINT('Ctrl Pts',(-0.307116929000056,15.2,10.467017151));
#227169=CARTESIAN_POINT('Ctrl Pts',(-0.307116929000056,11.6,10.467017151));
#227170=CARTESIAN_POINT('Ctrl Pts',(-0.307416292000056,15.2,10.468569615));
#227171=CARTESIAN_POINT('Ctrl Pts',(-0.307416292000056,11.6,10.468569615));
#227172=CARTESIAN_POINT('Ctrl Pts',(-0.307718620000056,15.2,10.470129562));
#227173=CARTESIAN_POINT('Ctrl Pts',(-0.307718620000056,11.6,10.470129562));
#227174=CARTESIAN_POINT('Ctrl Pts',(-0.308023922000055,15.2,10.47169697));
#227175=CARTESIAN_POINT('Ctrl Pts',(-0.308023922000055,11.6,10.47169697));
#227176=CARTESIAN_POINT('Ctrl Pts',(-0.308332210000056,15.2,10.473271818));
#227177=CARTESIAN_POINT('Ctrl Pts',(-0.308332210000056,11.6,10.473271818));
#227178=CARTESIAN_POINT('Ctrl Pts',(-0.308643491000057,15.2,10.474854086));
#227179=CARTESIAN_POINT('Ctrl Pts',(-0.308643491000057,11.6,10.474854086));
#227180=CARTESIAN_POINT('Ctrl Pts',(-0.308957777000056,15.2,10.476443753));
#227181=CARTESIAN_POINT('Ctrl Pts',(-0.308957777000056,11.6,10.476443753));
#227182=CARTESIAN_POINT('Ctrl Pts',(-0.309275077000055,15.2,10.478040797));
#227183=CARTESIAN_POINT('Ctrl Pts',(-0.309275077000055,11.6,10.478040797));
#227184=CARTESIAN_POINT('Ctrl Pts',(-0.309595400000056,15.2,10.479645197));
#227185=CARTESIAN_POINT('Ctrl Pts',(-0.309595400000056,11.6,10.479645197));
#227186=CARTESIAN_POINT('Ctrl Pts',(-0.309918755000057,15.2,10.481256935));
#227187=CARTESIAN_POINT('Ctrl Pts',(-0.309918755000057,11.6,10.481256935));
#227188=CARTESIAN_POINT('Ctrl Pts',(-0.310245153000055,15.2,10.482875987));
#227189=CARTESIAN_POINT('Ctrl Pts',(-0.310245153000055,11.6,10.482875987));
#227190=CARTESIAN_POINT('Ctrl Pts',(-0.310574603000056,15.2,10.484502335));
#227191=CARTESIAN_POINT('Ctrl Pts',(-0.310574603000056,11.6,10.484502335));
#227192=CARTESIAN_POINT('Ctrl Pts',(-0.310907114000055,15.2,10.486135956));
#227193=CARTESIAN_POINT('Ctrl Pts',(-0.310907114000055,11.6,10.486135956));
#227194=CARTESIAN_POINT('Ctrl Pts',(-0.311242695000056,15.2,10.487776833));
#227195=CARTESIAN_POINT('Ctrl Pts',(-0.311242695000056,11.6,10.487776833));
#227196=CARTESIAN_POINT('Ctrl Pts',(-0.311581357000056,15.2,10.489424943));
#227197=CARTESIAN_POINT('Ctrl Pts',(-0.311581357000056,11.6,10.489424943));
#227198=CARTESIAN_POINT('Ctrl Pts',(-0.311923108000055,15.2,10.491080266));
#227199=CARTESIAN_POINT('Ctrl Pts',(-0.311923108000055,11.6,10.491080266));
#227200=CARTESIAN_POINT('Ctrl Pts',(-0.312267957000056,15.2,10.492742783));
#227201=CARTESIAN_POINT('Ctrl Pts',(-0.312267957000056,11.6,10.492742783));
#227202=CARTESIAN_POINT('Ctrl Pts',(-0.312615913000055,15.2,10.494412473));
#227203=CARTESIAN_POINT('Ctrl Pts',(-0.312615913000055,11.6,10.494412473));
#227204=CARTESIAN_POINT('Ctrl Pts',(-0.312966986000056,15.2,10.496089317));
#227205=CARTESIAN_POINT('Ctrl Pts',(-0.312966986000056,11.6,10.496089317));
#227206=CARTESIAN_POINT('Ctrl Pts',(-0.313321186000056,15.2,10.497773292));
#227207=CARTESIAN_POINT('Ctrl Pts',(-0.313321186000056,11.6,10.497773292));
#227208=CARTESIAN_POINT('Ctrl Pts',(-0.313678519000057,15.2,10.499464382));
#227209=CARTESIAN_POINT('Ctrl Pts',(-0.313678519000057,11.6,10.499464382));
#227210=CARTESIAN_POINT('Ctrl Pts',(-0.314038998000056,15.2,10.501162565));
#227211=CARTESIAN_POINT('Ctrl Pts',(-0.314038998000056,11.6,10.501162565));
#227212=CARTESIAN_POINT('Ctrl Pts',(-0.314402627000057,15.2,10.502867822));
#227213=CARTESIAN_POINT('Ctrl Pts',(-0.314402627000057,11.6,10.502867822));
#227214=CARTESIAN_POINT('Ctrl Pts',(-0.314769419000056,15.2,10.504580133));
#227215=CARTESIAN_POINT('Ctrl Pts',(-0.314769419000056,11.6,10.504580133));
#227216=CARTESIAN_POINT('Ctrl Pts',(-0.315139383000057,15.2,10.506299478));
#227217=CARTESIAN_POINT('Ctrl Pts',(-0.315139383000057,11.6,10.506299478));
#227218=CARTESIAN_POINT('Ctrl Pts',(-0.315512524000056,15.2,10.508025839));
#227219=CARTESIAN_POINT('Ctrl Pts',(-0.315512524000056,11.6,10.508025839));
#227220=CARTESIAN_POINT('Ctrl Pts',(-0.315888854000056,15.2,10.509759194));
#227221=CARTESIAN_POINT('Ctrl Pts',(-0.315888854000056,11.6,10.509759194));
#227222=CARTESIAN_POINT('Ctrl Pts',(-0.316268381000055,15.2,10.511499524));
#227223=CARTESIAN_POINT('Ctrl Pts',(-0.316268381000055,11.6,10.511499524));
#227224=CARTESIAN_POINT('Ctrl Pts',(-0.316651113000056,15.2,10.513246813));
#227225=CARTESIAN_POINT('Ctrl Pts',(-0.316651113000056,11.6,10.513246813));
#227226=CARTESIAN_POINT('Ctrl Pts',(-0.317037059000055,15.2,10.515001037));
#227227=CARTESIAN_POINT('Ctrl Pts',(-0.317037059000055,11.6,10.515001037));
#227228=CARTESIAN_POINT('Ctrl Pts',(-0.317426228000055,15.2,10.51676218));
#227229=CARTESIAN_POINT('Ctrl Pts',(-0.317426228000055,11.6,10.51676218));
#227230=CARTESIAN_POINT('Ctrl Pts',(-0.317818629000056,15.2,10.518530221));
#227231=CARTESIAN_POINT('Ctrl Pts',(-0.317818629000056,11.6,10.518530221));
#227232=CARTESIAN_POINT('Ctrl Pts',(-0.318214269000056,15.2,10.520305142));
#227233=CARTESIAN_POINT('Ctrl Pts',(-0.318214269000056,11.6,10.520305142));
#227234=CARTESIAN_POINT('Ctrl Pts',(-0.318613157000056,15.2,10.522086924));
#227235=CARTESIAN_POINT('Ctrl Pts',(-0.318613157000056,11.6,10.522086924));
#227236=CARTESIAN_POINT('Ctrl Pts',(-0.319015302000055,15.2,10.523875548));
#227237=CARTESIAN_POINT('Ctrl Pts',(-0.319015302000055,11.6,10.523875548));
#227238=CARTESIAN_POINT('Ctrl Pts',(-0.319420712000056,15.2,10.525670994));
#227239=CARTESIAN_POINT('Ctrl Pts',(-0.319420712000056,11.6,10.525670994));
#227240=CARTESIAN_POINT('Ctrl Pts',(-0.319829395000056,15.2,10.527473244));
#227241=CARTESIAN_POINT('Ctrl Pts',(-0.319829395000056,11.6,10.527473244));
#227242=CARTESIAN_POINT('Ctrl Pts',(-0.320241361000055,15.2,10.529282278));
#227243=CARTESIAN_POINT('Ctrl Pts',(-0.320241361000055,11.6,10.529282278));
#227244=CARTESIAN_POINT('Ctrl Pts',(-0.320656616000056,15.2,10.53109808));
#227245=CARTESIAN_POINT('Ctrl Pts',(-0.320656616000056,11.6,10.53109808));
#227246=CARTESIAN_POINT('Ctrl Pts',(-0.321075169000055,15.2,10.53292063));
#227247=CARTESIAN_POINT('Ctrl Pts',(-0.321075169000055,11.6,10.53292063));
#227248=CARTESIAN_POINT('Ctrl Pts',(-0.321497030000056,15.2,10.534749908));
#227249=CARTESIAN_POINT('Ctrl Pts',(-0.321497030000056,11.6,10.534749908));
#227250=CARTESIAN_POINT('Ctrl Pts',(-0.321922204000057,15.2,10.536585896));
#227251=CARTESIAN_POINT('Ctrl Pts',(-0.321922204000057,11.6,10.536585896));
#227252=CARTESIAN_POINT('Ctrl Pts',(-0.322350700000056,15.2,10.538428577));
#227253=CARTESIAN_POINT('Ctrl Pts',(-0.322350700000056,11.6,10.538428577));
#227254=CARTESIAN_POINT('Ctrl Pts',(-0.322782528000056,15.2,10.540277931));
#227255=CARTESIAN_POINT('Ctrl Pts',(-0.322782528000056,11.6,10.540277931));
#227256=CARTESIAN_POINT('Ctrl Pts',(-0.323217694000055,15.2,10.542133941));
#227257=CARTESIAN_POINT('Ctrl Pts',(-0.323217694000055,11.6,10.542133941));
#227258=CARTESIAN_POINT('Ctrl Pts',(-0.323656207000056,15.2,10.543996587));
#227259=CARTESIAN_POINT('Ctrl Pts',(-0.323656207000056,11.6,10.543996587));
#227260=CARTESIAN_POINT('Ctrl Pts',(-0.324098075000055,15.2,10.545865852));
#227261=CARTESIAN_POINT('Ctrl Pts',(-0.324098075000055,11.6,10.545865852));
#227262=CARTESIAN_POINT('Ctrl Pts',(-0.324543305000056,15.2,10.547741717));
#227263=CARTESIAN_POINT('Ctrl Pts',(-0.324543305000056,11.6,10.547741717));
#227264=CARTESIAN_POINT('Ctrl Pts',(-0.324991905000056,15.2,10.549624165));
#227265=CARTESIAN_POINT('Ctrl Pts',(-0.324991905000056,11.6,10.549624165));
#227266=CARTESIAN_POINT('Ctrl Pts',(-0.325443884000055,15.2,10.551513177));
#227267=CARTESIAN_POINT('Ctrl Pts',(-0.325443884000055,11.6,10.551513177));
#227268=CARTESIAN_POINT('Ctrl Pts',(-0.325899249000056,15.2,10.553408734));
#227269=CARTESIAN_POINT('Ctrl Pts',(-0.325899249000056,11.6,10.553408734));
#227270=CARTESIAN_POINT('Ctrl Pts',(-0.326358007000056,15.2,10.555310822));
#227271=CARTESIAN_POINT('Ctrl Pts',(-0.326358007000056,11.6,10.555310822));
#227272=CARTESIAN_POINT('Ctrl Pts',(-0.326820167000056,15.2,10.557219418));
#227273=CARTESIAN_POINT('Ctrl Pts',(-0.326820167000056,11.6,10.557219418));
#227274=CARTESIAN_POINT('Ctrl Pts',(-0.327285737000055,15.2,10.559134507));
#227275=CARTESIAN_POINT('Ctrl Pts',(-0.327285737000055,11.6,10.559134507));
#227276=CARTESIAN_POINT('Ctrl Pts',(-0.327754722000057,15.2,10.561056071));
#227277=CARTESIAN_POINT('Ctrl Pts',(-0.327754722000057,11.6,10.561056071));
#227278=CARTESIAN_POINT('Ctrl Pts',(-0.328227133000055,15.2,10.562984091));
#227279=CARTESIAN_POINT('Ctrl Pts',(-0.328227133000055,11.6,10.562984091));
#227280=CARTESIAN_POINT('Ctrl Pts',(-0.328702975000056,15.2,10.564918551));
#227281=CARTESIAN_POINT('Ctrl Pts',(-0.328702975000056,11.6,10.564918551));
#227282=CARTESIAN_POINT('Ctrl Pts',(-0.329182257000056,15.2,10.566859433));
#227283=CARTESIAN_POINT('Ctrl Pts',(-0.329182257000056,11.6,10.566859433));
#227284=CARTESIAN_POINT('Ctrl Pts',(-0.329664986000056,15.2,10.568806718));
#227285=CARTESIAN_POINT('Ctrl Pts',(-0.329664986000056,11.6,10.568806718));
#227286=CARTESIAN_POINT('Ctrl Pts',(-0.330151168000056,15.2,10.57076039));
#227287=CARTESIAN_POINT('Ctrl Pts',(-0.330151168000056,11.6,10.57076039));
#227288=CARTESIAN_POINT('Ctrl Pts',(-0.330640814000055,15.2,10.572720431));
#227289=CARTESIAN_POINT('Ctrl Pts',(-0.330640814000055,11.6,10.572720431));
#227290=CARTESIAN_POINT('Ctrl Pts',(-0.331133929000057,15.2,10.574686824));
#227291=CARTESIAN_POINT('Ctrl Pts',(-0.331133929000057,11.6,10.574686824));
#227292=CARTESIAN_POINT('Ctrl Pts',(-0.331630520000056,15.2,10.576659551));
#227293=CARTESIAN_POINT('Ctrl Pts',(-0.331630520000056,11.6,10.576659551));
#227294=CARTESIAN_POINT('Ctrl Pts',(-0.332130595000055,15.2,10.578638594));
#227295=CARTESIAN_POINT('Ctrl Pts',(-0.332130595000055,11.6,10.578638594));
#227296=CARTESIAN_POINT('Ctrl Pts',(-0.332634161000056,15.2,10.580623938));
#227297=CARTESIAN_POINT('Ctrl Pts',(-0.332634161000056,11.6,10.580623938));
#227298=CARTESIAN_POINT('Ctrl Pts',(-0.333141226000055,15.2,10.582615563));
#227299=CARTESIAN_POINT('Ctrl Pts',(-0.333141226000055,11.6,10.582615563));
#227300=CARTESIAN_POINT('Ctrl Pts',(-0.333651796000056,15.2,10.584613455));
#227301=CARTESIAN_POINT('Ctrl Pts',(-0.333651796000056,11.6,10.584613455));
#227302=CARTESIAN_POINT('Ctrl Pts',(-0.334165879000056,15.2,10.586617594));
#227303=CARTESIAN_POINT('Ctrl Pts',(-0.334165879000056,11.6,10.586617594));
#227304=CARTESIAN_POINT('Ctrl Pts',(-0.334683483000056,15.2,10.588627965));
#227305=CARTESIAN_POINT('Ctrl Pts',(-0.334683483000056,11.6,10.588627965));
#227306=CARTESIAN_POINT('Ctrl Pts',(-0.335204614000055,15.2,10.590644549));
#227307=CARTESIAN_POINT('Ctrl Pts',(-0.335204614000055,11.6,10.590644549));
#227308=CARTESIAN_POINT('Ctrl Pts',(-0.335729278000055,15.2,10.592667331));
#227309=CARTESIAN_POINT('Ctrl Pts',(-0.335729278000055,11.6,10.592667331));
#227310=CARTESIAN_POINT('Ctrl Pts',(-0.336257484000055,15.2,10.594696294));
#227311=CARTESIAN_POINT('Ctrl Pts',(-0.336257484000055,11.6,10.594696294));
#227312=CARTESIAN_POINT('Ctrl Pts',(-0.336789237000056,15.2,10.596731419));
#227313=CARTESIAN_POINT('Ctrl Pts',(-0.336789237000056,11.6,10.596731419));
#227314=CARTESIAN_POINT('Ctrl Pts',(-0.337324546000056,15.2,10.598772692));
#227315=CARTESIAN_POINT('Ctrl Pts',(-0.337324546000056,11.6,10.598772692));
#227316=CARTESIAN_POINT('Ctrl Pts',(-0.337863418000056,15.2,10.600820093));
#227317=CARTESIAN_POINT('Ctrl Pts',(-0.337863418000056,11.6,10.600820093));
#227318=CARTESIAN_POINT('Ctrl Pts',(-0.338405859000056,15.2,10.602873609));
#227319=CARTESIAN_POINT('Ctrl Pts',(-0.338405859000056,11.6,10.602873609));
#227320=CARTESIAN_POINT('Ctrl Pts',(-0.338951875000056,15.2,10.604933221));
#227321=CARTESIAN_POINT('Ctrl Pts',(-0.338951875000056,11.6,10.604933221));
#227322=CARTESIAN_POINT('Ctrl Pts',(-0.339501474000056,15.2,10.606998913));
#227323=CARTESIAN_POINT('Ctrl Pts',(-0.339501474000056,11.6,10.606998913));
#227324=CARTESIAN_POINT('Ctrl Pts',(-0.340054663000057,15.2,10.609070668));
#227325=CARTESIAN_POINT('Ctrl Pts',(-0.340054663000057,11.6,10.609070668));
#227326=CARTESIAN_POINT('Ctrl Pts',(-0.340611447000055,15.2,10.61114847));
#227327=CARTESIAN_POINT('Ctrl Pts',(-0.340611447000055,11.6,10.61114847));
#227328=CARTESIAN_POINT('Ctrl Pts',(-0.341171835000056,15.2,10.613232302));
#227329=CARTESIAN_POINT('Ctrl Pts',(-0.341171835000056,11.6,10.613232302));
#227330=CARTESIAN_POINT('Ctrl Pts',(-0.341735833000056,15.2,10.615322148));
#227331=CARTESIAN_POINT('Ctrl Pts',(-0.341735833000056,11.6,10.615322148));
#227332=CARTESIAN_POINT('Ctrl Pts',(-0.342303447000055,15.2,10.617417992));
#227333=CARTESIAN_POINT('Ctrl Pts',(-0.342303447000055,11.6,10.617417992));
#227334=CARTESIAN_POINT('Ctrl Pts',(-0.342874686000056,15.2,10.619519817));
#227335=CARTESIAN_POINT('Ctrl Pts',(-0.342874686000056,11.6,10.619519817));
#227336=CARTESIAN_POINT('Ctrl Pts',(-0.343449552000056,15.2,10.621627607));
#227337=CARTESIAN_POINT('Ctrl Pts',(-0.343449552000056,11.6,10.621627607));
#227338=CARTESIAN_POINT('Ctrl Pts',(-0.344028056000055,15.2,10.623741346));
#227339=CARTESIAN_POINT('Ctrl Pts',(-0.344028056000055,11.6,10.623741346));
#227340=CARTESIAN_POINT('Ctrl Pts',(-0.344610203000055,15.2,10.625861018));
#227341=CARTESIAN_POINT('Ctrl Pts',(-0.344610203000055,11.6,10.625861018));
#227342=CARTESIAN_POINT('Ctrl Pts',(-0.345195998000056,15.2,10.627986606));
#227343=CARTESIAN_POINT('Ctrl Pts',(-0.345195998000056,11.6,10.627986606));
#227344=CARTESIAN_POINT('Ctrl Pts',(-0.345785451000056,15.2,10.630118095));
#227345=CARTESIAN_POINT('Ctrl Pts',(-0.345785451000056,11.6,10.630118095));
#227346=CARTESIAN_POINT('Ctrl Pts',(-0.346378564000055,15.2,10.632255468));
#227347=CARTESIAN_POINT('Ctrl Pts',(-0.346378564000055,11.6,10.632255468));
#227348=CARTESIAN_POINT('Ctrl Pts',(-0.346975348000056,15.2,10.634398709));
#227349=CARTESIAN_POINT('Ctrl Pts',(-0.346975348000056,11.6,10.634398709));
#227350=CARTESIAN_POINT('Ctrl Pts',(-0.347575806000057,15.2,10.636547802));
#227351=CARTESIAN_POINT('Ctrl Pts',(-0.347575806000057,11.6,10.636547802));
#227352=CARTESIAN_POINT('Ctrl Pts',(-0.348179945000057,15.2,10.638702733));
#227353=CARTESIAN_POINT('Ctrl Pts',(-0.348179945000057,11.6,10.638702733));
#227354=CARTESIAN_POINT('Ctrl Pts',(-0.348787773000057,15.2,10.640863484));
#227355=CARTESIAN_POINT('Ctrl Pts',(-0.348787773000057,11.6,10.640863484));
#227356=CARTESIAN_POINT('Ctrl Pts',(-0.349399295000056,15.2,10.643030039));
#227357=CARTESIAN_POINT('Ctrl Pts',(-0.349399295000056,11.6,10.643030039));
#227358=CARTESIAN_POINT('Ctrl Pts',(-0.350014517000057,15.2,10.645202383));
#227359=CARTESIAN_POINT('Ctrl Pts',(-0.350014517000057,11.6,10.645202383));
#227360=CARTESIAN_POINT('Ctrl Pts',(-0.350633446000056,15.2,10.6473805));
#227361=CARTESIAN_POINT('Ctrl Pts',(-0.350633446000056,11.6,10.6473805));
#227362=CARTESIAN_POINT('Ctrl Pts',(-0.351256088000056,15.2,10.649564376));
#227363=CARTESIAN_POINT('Ctrl Pts',(-0.351256088000056,11.6,10.649564376));
#227364=CARTESIAN_POINT('Ctrl Pts',(-0.351882450000056,15.2,10.651753994));
#227365=CARTESIAN_POINT('Ctrl Pts',(-0.351882450000056,11.6,10.651753994));
#227366=CARTESIAN_POINT('Ctrl Pts',(-0.352512536000056,15.2,10.653949337));
#227367=CARTESIAN_POINT('Ctrl Pts',(-0.352512536000056,11.6,10.653949337));
#227368=CARTESIAN_POINT('Ctrl Pts',(-0.353146354000057,15.2,10.656150391));
#227369=CARTESIAN_POINT('Ctrl Pts',(-0.353146354000057,11.6,10.656150391));
#227370=CARTESIAN_POINT('Ctrl Pts',(-0.353783911000055,15.2,10.658357142));
#227371=CARTESIAN_POINT('Ctrl Pts',(-0.353783911000055,11.6,10.658357142));
#227372=CARTESIAN_POINT('Ctrl Pts',(-0.354425210000056,15.2,10.66056957));
#227373=CARTESIAN_POINT('Ctrl Pts',(-0.354425210000056,11.6,10.66056957));
#227374=CARTESIAN_POINT('Ctrl Pts',(-0.355070259000057,15.2,10.662787665));
#227375=CARTESIAN_POINT('Ctrl Pts',(-0.355070259000057,11.6,10.662787665));
#227376=CARTESIAN_POINT('Ctrl Pts',(-0.355719064000055,15.2,10.665011408));
#227377=CARTESIAN_POINT('Ctrl Pts',(-0.355719064000055,11.6,10.665011408));
#227378=CARTESIAN_POINT('Ctrl Pts',(-0.356371630000056,15.2,10.667240784));
#227379=CARTESIAN_POINT('Ctrl Pts',(-0.356371630000056,11.6,10.667240784));
#227380=CARTESIAN_POINT('Ctrl Pts',(-0.357027964000055,15.2,10.669475779));
#227381=CARTESIAN_POINT('Ctrl Pts',(-0.357027964000055,11.6,10.669475779));
#227382=CARTESIAN_POINT('Ctrl Pts',(-0.357688072000055,15.2,10.671716376));
#227383=CARTESIAN_POINT('Ctrl Pts',(-0.357688072000055,11.6,10.671716376));
#227384=CARTESIAN_POINT('Ctrl Pts',(-0.358351960000055,15.2,10.673962562));
#227385=CARTESIAN_POINT('Ctrl Pts',(-0.358351960000055,11.6,10.673962562));
#227386=CARTESIAN_POINT('Ctrl Pts',(-0.359019632000056,15.2,10.67621432));
#227387=CARTESIAN_POINT('Ctrl Pts',(-0.359019632000056,11.6,10.67621432));
#227388=CARTESIAN_POINT('Ctrl Pts',(-0.359691096000055,15.2,10.678471636));
#227389=CARTESIAN_POINT('Ctrl Pts',(-0.359691096000055,11.6,10.678471636));
#227390=CARTESIAN_POINT('Ctrl Pts',(-0.360366357000055,15.2,10.680734494));
#227391=CARTESIAN_POINT('Ctrl Pts',(-0.360366357000055,11.6,10.680734494));
#227392=CARTESIAN_POINT('Ctrl Pts',(-0.361045421000057,15.2,10.683002879));
#227393=CARTESIAN_POINT('Ctrl Pts',(-0.361045421000057,11.6,10.683002879));
#227394=CARTESIAN_POINT('Ctrl Pts',(-0.361728294000055,15.2,10.685276776));
#227395=CARTESIAN_POINT('Ctrl Pts',(-0.361728294000055,11.6,10.685276776));
#227396=CARTESIAN_POINT('Ctrl Pts',(-0.362414981000055,15.2,10.687556171));
#227397=CARTESIAN_POINT('Ctrl Pts',(-0.362414981000055,11.6,10.687556171));
#227398=CARTESIAN_POINT('Ctrl Pts',(-0.363105488000055,15.2,10.689841048));
#227399=CARTESIAN_POINT('Ctrl Pts',(-0.363105488000055,11.6,10.689841048));
#227400=CARTESIAN_POINT('Ctrl Pts',(-0.363799821000056,15.2,10.692131392));
#227401=CARTESIAN_POINT('Ctrl Pts',(-0.363799821000056,11.6,10.692131392));
#227402=CARTESIAN_POINT('Ctrl Pts',(-0.364497985000056,15.2,10.694427189));
#227403=CARTESIAN_POINT('Ctrl Pts',(-0.364497985000056,11.6,10.694427189));
#227404=CARTESIAN_POINT('Ctrl Pts',(-0.365199987000056,15.2,10.696728424));
#227405=CARTESIAN_POINT('Ctrl Pts',(-0.365199987000056,11.6,10.696728424));
#227406=CARTESIAN_POINT('Ctrl Pts',(-0.365905831000056,15.2,10.699035082));
#227407=CARTESIAN_POINT('Ctrl Pts',(-0.365905831000056,11.6,10.699035082));
#227408=CARTESIAN_POINT('Ctrl Pts',(-0.366615524000055,15.2,10.701347148));
#227409=CARTESIAN_POINT('Ctrl Pts',(-0.366615524000055,11.6,10.701347148));
#227410=CARTESIAN_POINT('Ctrl Pts',(-0.367329070000055,15.2,10.703664608));
#227411=CARTESIAN_POINT('Ctrl Pts',(-0.367329070000055,11.6,10.703664608));
#227412=CARTESIAN_POINT('Ctrl Pts',(-0.368046475000057,15.2,10.705987446));
#227413=CARTESIAN_POINT('Ctrl Pts',(-0.368046475000057,11.6,10.705987446));
#227414=CARTESIAN_POINT('Ctrl Pts',(-0.368767746000056,15.2,10.708315648));
#227415=CARTESIAN_POINT('Ctrl Pts',(-0.368767746000056,11.6,10.708315648));
#227416=CARTESIAN_POINT('Ctrl Pts',(-0.369492887000057,15.2,10.7106492));
#227417=CARTESIAN_POINT('Ctrl Pts',(-0.369492887000057,11.6,10.7106492));
#227418=CARTESIAN_POINT('Ctrl Pts',(-0.370221904000055,15.2,10.712988087));
#227419=CARTESIAN_POINT('Ctrl Pts',(-0.370221904000055,11.6,10.712988087));
#227420=CARTESIAN_POINT('Ctrl Pts',(-0.370954802000056,15.2,10.715332294));
#227421=CARTESIAN_POINT('Ctrl Pts',(-0.370954802000056,11.6,10.715332294));
#227422=CARTESIAN_POINT('Ctrl Pts',(-0.371691587000056,15.2,10.717681807));
#227423=CARTESIAN_POINT('Ctrl Pts',(-0.371691587000056,11.6,10.717681807));
#227424=CARTESIAN_POINT('Ctrl Pts',(-0.372432264000055,15.2,10.720036611));
#227425=CARTESIAN_POINT('Ctrl Pts',(-0.372432264000055,11.6,10.720036611));
#227426=CARTESIAN_POINT('Ctrl Pts',(-0.373176838000056,15.2,10.722396693));
#227427=CARTESIAN_POINT('Ctrl Pts',(-0.373176838000056,11.6,10.722396693));
#227428=CARTESIAN_POINT('Ctrl Pts',(-0.373925315000055,15.2,10.724762038));
#227429=CARTESIAN_POINT('Ctrl Pts',(-0.373925315000055,11.6,10.724762038));
#227430=CARTESIAN_POINT('Ctrl Pts',(-0.374677700000056,15.2,10.72713263));
#227431=CARTESIAN_POINT('Ctrl Pts',(-0.374677700000056,11.6,10.72713263));
#227432=CARTESIAN_POINT('Ctrl Pts',(-0.375433998000055,15.2,10.729508458));
#227433=CARTESIAN_POINT('Ctrl Pts',(-0.375433998000055,11.6,10.729508458));
#227434=CARTESIAN_POINT('Ctrl Pts',(-0.376194216000056,15.2,10.731889504));
#227435=CARTESIAN_POINT('Ctrl Pts',(-0.376194216000056,11.6,10.731889504));
#227436=CARTESIAN_POINT('Ctrl Pts',(-0.376958356000056,15.2,10.734275756));
#227437=CARTESIAN_POINT('Ctrl Pts',(-0.376958356000056,11.6,10.734275756));
#227438=CARTESIAN_POINT('Ctrl Pts',(-0.377726425000056,15.2,10.7366672));
#227439=CARTESIAN_POINT('Ctrl Pts',(-0.377726425000056,11.6,10.7366672));
#227440=CARTESIAN_POINT('Ctrl Pts',(-0.378498429000055,15.2,10.739063821));
#227441=CARTESIAN_POINT('Ctrl Pts',(-0.378498429000055,11.6,10.739063821));
#227442=CARTESIAN_POINT('Ctrl Pts',(-0.379274373000056,15.2,10.741465604));
#227443=CARTESIAN_POINT('Ctrl Pts',(-0.379274373000056,11.6,10.741465604));
#227444=CARTESIAN_POINT('Ctrl Pts',(-0.380054260000057,15.2,10.743872536));
#227445=CARTESIAN_POINT('Ctrl Pts',(-0.380054260000057,11.6,10.743872536));
#227446=CARTESIAN_POINT('Ctrl Pts',(-0.380838098000057,15.2,10.746284603));
#227447=CARTESIAN_POINT('Ctrl Pts',(-0.380838098000057,11.6,10.746284603));
#227448=CARTESIAN_POINT('Ctrl Pts',(-0.381625890000056,15.2,10.748701792));
#227449=CARTESIAN_POINT('Ctrl Pts',(-0.381625890000056,11.6,10.748701792));
#227450=CARTESIAN_POINT('Ctrl Pts',(-0.382417641000057,15.2,10.751124087));
#227451=CARTESIAN_POINT('Ctrl Pts',(-0.382417641000057,11.6,10.751124087));
#227452=CARTESIAN_POINT('Ctrl Pts',(-0.383213358000055,15.2,10.753551475));
#227453=CARTESIAN_POINT('Ctrl Pts',(-0.383213358000055,11.6,10.753551475));
#227454=CARTESIAN_POINT('Ctrl Pts',(-0.384013044000057,15.2,10.755983943));
#227455=CARTESIAN_POINT('Ctrl Pts',(-0.384013044000057,11.6,10.755983943));
#227456=CARTESIAN_POINT('Ctrl Pts',(-0.384816706000055,15.2,10.758421474));
#227457=CARTESIAN_POINT('Ctrl Pts',(-0.384816706000055,11.6,10.758421474));
#227458=CARTESIAN_POINT('Ctrl Pts',(-0.385624346000055,15.2,10.760864058));
#227459=CARTESIAN_POINT('Ctrl Pts',(-0.385624346000055,11.6,10.760864058));
#227460=CARTESIAN_POINT('Ctrl Pts',(-0.386435972000055,15.2,10.763311678));
#227461=CARTESIAN_POINT('Ctrl Pts',(-0.386435972000055,11.6,10.763311678));
#227462=CARTESIAN_POINT('Ctrl Pts',(-0.387251587000056,15.2,10.765764322));
#227463=CARTESIAN_POINT('Ctrl Pts',(-0.387251587000056,11.6,10.765764322));
#227464=CARTESIAN_POINT('Ctrl Pts',(-0.388071197000055,15.2,10.768221976));
#227465=CARTESIAN_POINT('Ctrl Pts',(-0.388071197000055,11.6,10.768221976));
#227466=CARTESIAN_POINT('Ctrl Pts',(-0.388894805000056,15.2,10.770684627));
#227467=CARTESIAN_POINT('Ctrl Pts',(-0.388894805000056,11.6,10.770684627));
#227468=CARTESIAN_POINT('Ctrl Pts',(-0.389722418000057,15.2,10.773152259));
#227469=CARTESIAN_POINT('Ctrl Pts',(-0.389722418000057,11.6,10.773152259));
#227470=CARTESIAN_POINT('Ctrl Pts',(-0.390554041000056,15.2,10.77562486));
#227471=CARTESIAN_POINT('Ctrl Pts',(-0.390554041000056,11.6,10.77562486));
#227472=CARTESIAN_POINT('Ctrl Pts',(-0.391389677000056,15.2,10.778102417));
#227473=CARTESIAN_POINT('Ctrl Pts',(-0.391389677000056,11.6,10.778102417));
#227474=CARTESIAN_POINT('Ctrl Pts',(-0.392229332000056,15.2,10.780584915));
#227475=CARTESIAN_POINT('Ctrl Pts',(-0.392229332000056,11.6,10.780584915));
#227476=CARTESIAN_POINT('Ctrl Pts',(-0.393073010000055,15.2,10.783072341));
#227477=CARTESIAN_POINT('Ctrl Pts',(-0.393073010000055,11.6,10.783072341));
#227478=CARTESIAN_POINT('Ctrl Pts',(-0.393920716000055,15.2,10.785564682));
#227479=CARTESIAN_POINT('Ctrl Pts',(-0.393920716000055,11.6,10.785564682));
#227480=CARTESIAN_POINT('Ctrl Pts',(-0.394772455000056,15.2,10.788061923));
#227481=CARTESIAN_POINT('Ctrl Pts',(-0.394772455000056,11.6,10.788061923));
#227482=CARTESIAN_POINT('Ctrl Pts',(-0.395628232000057,15.2,10.790564052));
#227483=CARTESIAN_POINT('Ctrl Pts',(-0.395628232000057,11.6,10.790564052));
#227484=CARTESIAN_POINT('Ctrl Pts',(-0.396488052000056,15.2,10.793071055));
#227485=CARTESIAN_POINT('Ctrl Pts',(-0.396488052000056,11.6,10.793071055));
#227486=CARTESIAN_POINT('Ctrl Pts',(-0.397351918000056,15.2,10.795582918));
#227487=CARTESIAN_POINT('Ctrl Pts',(-0.397351918000056,11.6,10.795582918));
#227488=CARTESIAN_POINT('Ctrl Pts',(-0.398219836000056,15.2,10.798099629));
#227489=CARTESIAN_POINT('Ctrl Pts',(-0.398219836000056,11.6,10.798099629));
#227490=CARTESIAN_POINT('Ctrl Pts',(-0.399091809000056,15.2,10.800621175));
#227491=CARTESIAN_POINT('Ctrl Pts',(-0.399091809000056,11.6,10.800621175));
#227492=CARTESIAN_POINT('Ctrl Pts',(-0.399967843000055,15.2,10.80314754));
#227493=CARTESIAN_POINT('Ctrl Pts',(-0.399967843000055,11.6,10.80314754));
#227494=CARTESIAN_POINT('Ctrl Pts',(-0.400847943000056,15.2,10.805678712));
#227495=CARTESIAN_POINT('Ctrl Pts',(-0.400847943000056,11.6,10.805678712));
#227496=CARTESIAN_POINT('Ctrl Pts',(-0.401732113000056,15.2,10.80821468));
#227497=CARTESIAN_POINT('Ctrl Pts',(-0.401732113000056,11.6,10.80821468));
#227498=CARTESIAN_POINT('Ctrl Pts',(-0.402620357000056,15.2,10.810755427));
#227499=CARTESIAN_POINT('Ctrl Pts',(-0.402620357000056,11.6,10.810755427));
#227500=CARTESIAN_POINT('Ctrl Pts',(-0.403512680000055,15.2,10.813300943));
#227501=CARTESIAN_POINT('Ctrl Pts',(-0.403512680000055,11.6,10.813300943));
#227502=CARTESIAN_POINT('Ctrl Pts',(-0.404409086000056,15.2,10.815851213));
#227503=CARTESIAN_POINT('Ctrl Pts',(-0.404409086000056,11.6,10.815851213));
#227504=CARTESIAN_POINT('Ctrl Pts',(-0.405309580000056,15.2,10.818406224));
#227505=CARTESIAN_POINT('Ctrl Pts',(-0.405309580000056,11.6,10.818406224));
#227506=CARTESIAN_POINT('Ctrl Pts',(-0.406214167000056,15.2,10.820965965));
#227507=CARTESIAN_POINT('Ctrl Pts',(-0.406214167000056,11.6,10.820965965));
#227508=CARTESIAN_POINT('Ctrl Pts',(-0.407122850000056,15.2,10.82353042));
#227509=CARTESIAN_POINT('Ctrl Pts',(-0.407122850000056,11.6,10.82353042));
#227510=CARTESIAN_POINT('Ctrl Pts',(-0.408035634000056,15.2,10.826099577));
#227511=CARTESIAN_POINT('Ctrl Pts',(-0.408035634000056,11.6,10.826099577));
#227512=CARTESIAN_POINT('Ctrl Pts',(-0.408952523000057,15.2,10.828673423));
#227513=CARTESIAN_POINT('Ctrl Pts',(-0.408952523000057,11.6,10.828673423));
#227514=CARTESIAN_POINT('Ctrl Pts',(-0.409873522000056,15.2,10.831251946));
#227515=CARTESIAN_POINT('Ctrl Pts',(-0.409873522000056,11.6,10.831251946));
#227516=CARTESIAN_POINT('Ctrl Pts',(-0.410798636000056,15.2,10.833835133));
#227517=CARTESIAN_POINT('Ctrl Pts',(-0.410798636000056,11.6,10.833835133));
#227518=CARTESIAN_POINT('Ctrl Pts',(-0.411727868000057,15.2,10.836422969));
#227519=CARTESIAN_POINT('Ctrl Pts',(-0.411727868000057,11.6,10.836422969));
#227520=CARTESIAN_POINT('Ctrl Pts',(-0.412661222000056,15.2,10.839015444));
#227521=CARTESIAN_POINT('Ctrl Pts',(-0.412661222000056,11.6,10.839015444));
#227522=CARTESIAN_POINT('Ctrl Pts',(-0.413598704000057,15.2,10.841612542));
#227523=CARTESIAN_POINT('Ctrl Pts',(-0.413598704000057,11.6,10.841612542));
#227524=CARTESIAN_POINT('Ctrl Pts',(-0.414540317000055,15.2,10.844214253));
#227525=CARTESIAN_POINT('Ctrl Pts',(-0.414540317000055,11.6,10.844214253));
#227526=CARTESIAN_POINT('Ctrl Pts',(-0.415486065000056,15.2,10.846820562));
#227527=CARTESIAN_POINT('Ctrl Pts',(-0.415486065000056,11.6,10.846820562));
#227528=CARTESIAN_POINT('Ctrl Pts',(-0.416435953000055,15.2,10.849431458));
#227529=CARTESIAN_POINT('Ctrl Pts',(-0.416435953000055,11.6,10.849431458));
#227530=CARTESIAN_POINT('Ctrl Pts',(-0.417389986000056,15.2,10.852046927));
#227531=CARTESIAN_POINT('Ctrl Pts',(-0.417389986000056,11.6,10.852046927));
#227532=CARTESIAN_POINT('Ctrl Pts',(-0.418348166000057,15.2,10.854666957));
#227533=CARTESIAN_POINT('Ctrl Pts',(-0.418348166000057,11.6,10.854666957));
#227534=CARTESIAN_POINT('Ctrl Pts',(-0.419310498000056,15.2,10.857291536));
#227535=CARTESIAN_POINT('Ctrl Pts',(-0.419310498000056,11.6,10.857291536));
#227536=CARTESIAN_POINT('Ctrl Pts',(-0.420276987000056,15.2,10.859920649));
#227537=CARTESIAN_POINT('Ctrl Pts',(-0.420276987000056,11.6,10.859920649));
#227538=CARTESIAN_POINT('Ctrl Pts',(-0.421247636000055,15.2,10.862554285));
#227539=CARTESIAN_POINT('Ctrl Pts',(-0.421247636000055,11.6,10.862554285));
#227540=CARTESIAN_POINT('Ctrl Pts',(-0.422222450000056,15.2,10.865192432));
#227541=CARTESIAN_POINT('Ctrl Pts',(-0.422222450000056,11.6,10.865192432));
#227542=CARTESIAN_POINT('Ctrl Pts',(-0.423201433000056,15.2,10.867835076));
#227543=CARTESIAN_POINT('Ctrl Pts',(-0.423201433000056,11.6,10.867835076));
#227544=CARTESIAN_POINT('Ctrl Pts',(-0.424184589000056,15.2,10.870482205));
#227545=CARTESIAN_POINT('Ctrl Pts',(-0.424184589000056,11.6,10.870482205));
#227546=CARTESIAN_POINT('Ctrl Pts',(-0.425171920000055,15.2,10.873133807));
#227547=CARTESIAN_POINT('Ctrl Pts',(-0.425171920000055,11.6,10.873133807));
#227548=CARTESIAN_POINT('Ctrl Pts',(-0.426163434000056,15.2,10.875789869));
#227549=CARTESIAN_POINT('Ctrl Pts',(-0.426163434000056,11.6,10.875789869));
#227550=CARTESIAN_POINT('Ctrl Pts',(-0.427159131000057,15.2,10.878450378));
#227551=CARTESIAN_POINT('Ctrl Pts',(-0.427159131000057,11.6,10.878450378));
#227552=CARTESIAN_POINT('Ctrl Pts',(-0.428159019000055,15.2,10.881115323));
#227553=CARTESIAN_POINT('Ctrl Pts',(-0.428159019000055,11.6,10.881115323));
#227554=CARTESIAN_POINT('Ctrl Pts',(-0.429163097000057,15.2,10.88378469));
#227555=CARTESIAN_POINT('Ctrl Pts',(-0.429163097000057,11.6,10.88378469));
#227556=CARTESIAN_POINT('Ctrl Pts',(-0.430171373000056,15.2,10.886458467));
#227557=CARTESIAN_POINT('Ctrl Pts',(-0.430171373000056,11.6,10.886458467));
#227558=CARTESIAN_POINT('Ctrl Pts',(-0.431183850000056,15.2,10.889136642));
#227559=CARTESIAN_POINT('Ctrl Pts',(-0.431183850000056,11.6,10.889136642));
#227560=CARTESIAN_POINT('Ctrl Pts',(-0.432200532000057,15.2,10.891819204));
#227561=CARTESIAN_POINT('Ctrl Pts',(-0.432200532000057,11.6,10.891819204));
#227562=CARTESIAN_POINT('Ctrl Pts',(-0.433221421000055,15.2,10.894506138));
#227563=CARTESIAN_POINT('Ctrl Pts',(-0.433221421000055,11.6,10.894506138));
#227564=CARTESIAN_POINT('Ctrl Pts',(-0.434246523000056,15.2,10.897197433));
#227565=CARTESIAN_POINT('Ctrl Pts',(-0.434246523000056,11.6,10.897197433));
#227566=CARTESIAN_POINT('Ctrl Pts',(-0.435275841000056,15.2,10.899893078));
#227567=CARTESIAN_POINT('Ctrl Pts',(-0.435275841000056,11.6,10.899893078));
#227568=CARTESIAN_POINT('Ctrl Pts',(-0.436309379000056,15.2,10.902593058));
#227569=CARTESIAN_POINT('Ctrl Pts',(-0.436309379000056,11.6,10.902593058));
#227570=CARTESIAN_POINT('Ctrl Pts',(-0.437347140000056,15.2,10.905297364));
#227571=CARTESIAN_POINT('Ctrl Pts',(-0.437347140000056,11.6,10.905297364));
#227572=CARTESIAN_POINT('Ctrl Pts',(-0.438389130000055,15.2,10.908005982));
#227573=CARTESIAN_POINT('Ctrl Pts',(-0.438389130000055,11.6,10.908005982));
#227574=CARTESIAN_POINT('Ctrl Pts',(-0.439435351000055,15.2,10.910718899));
#227575=CARTESIAN_POINT('Ctrl Pts',(-0.439435351000055,11.6,10.910718899));
#227576=CARTESIAN_POINT('Ctrl Pts',(-0.440485807000056,15.2,10.913436104));
#227577=CARTESIAN_POINT('Ctrl Pts',(-0.440485807000056,11.6,10.913436104));
#227578=CARTESIAN_POINT('Ctrl Pts',(-0.441540501000055,15.2,10.916157585));
#227579=CARTESIAN_POINT('Ctrl Pts',(-0.441540501000055,11.6,10.916157585));
#227580=CARTESIAN_POINT('Ctrl Pts',(-0.442599439000055,15.2,10.91888333));
#227581=CARTESIAN_POINT('Ctrl Pts',(-0.442599439000055,11.6,10.91888333));
#227582=CARTESIAN_POINT('Ctrl Pts',(-0.443662622000056,15.2,10.921613326));
#227583=CARTESIAN_POINT('Ctrl Pts',(-0.443662622000056,11.6,10.921613326));
#227584=CARTESIAN_POINT('Ctrl Pts',(-0.444730056000056,15.2,10.924347563));
#227585=CARTESIAN_POINT('Ctrl Pts',(-0.444730056000056,11.6,10.924347563));
#227586=CARTESIAN_POINT('Ctrl Pts',(-0.445801744000055,15.2,10.927086027));
#227587=CARTESIAN_POINT('Ctrl Pts',(-0.445801744000055,11.6,10.927086027));
#227588=CARTESIAN_POINT('Ctrl Pts',(-0.446877689000056,15.2,10.929828706));
#227589=CARTESIAN_POINT('Ctrl Pts',(-0.446877689000056,11.6,10.929828706));
#227590=CARTESIAN_POINT('Ctrl Pts',(-0.447957894000056,15.2,10.932575589));
#227591=CARTESIAN_POINT('Ctrl Pts',(-0.447957894000056,11.6,10.932575589));
#227592=CARTESIAN_POINT('Ctrl Pts',(-0.449042364000055,15.2,10.935326665));
#227593=CARTESIAN_POINT('Ctrl Pts',(-0.449042364000055,11.6,10.935326665));
#227594=CARTESIAN_POINT('Ctrl Pts',(-0.450131103000055,15.2,10.938081919));
#227595=CARTESIAN_POINT('Ctrl Pts',(-0.450131103000055,11.6,10.938081919));
#227596=CARTESIAN_POINT('Ctrl Pts',(-0.451224113000055,15.2,10.940841342));
#227597=CARTESIAN_POINT('Ctrl Pts',(-0.451224113000055,11.6,10.940841342));
#227598=CARTESIAN_POINT('Ctrl Pts',(-0.452321398000055,15.2,10.943604922));
#227599=CARTESIAN_POINT('Ctrl Pts',(-0.452321398000055,11.6,10.943604922));
#227600=CARTESIAN_POINT('Ctrl Pts',(-0.453422963000056,15.2,10.946372645));
#227601=CARTESIAN_POINT('Ctrl Pts',(-0.453422963000056,11.6,10.946372645));
#227602=CARTESIAN_POINT('Ctrl Pts',(-0.454528809000055,15.2,10.949144502));
#227603=CARTESIAN_POINT('Ctrl Pts',(-0.454528809000055,11.6,10.949144502));
#227604=CARTESIAN_POINT('Ctrl Pts',(-0.455638942000055,15.2,10.951920479));
#227605=CARTESIAN_POINT('Ctrl Pts',(-0.455638942000055,11.6,10.951920479));
#227606=CARTESIAN_POINT('Ctrl Pts',(-0.456753365000055,15.2,10.954700564));
#227607=CARTESIAN_POINT('Ctrl Pts',(-0.456753365000055,11.6,10.954700564));
#227608=CARTESIAN_POINT('Ctrl Pts',(-0.457872079000056,15.2,10.957484748));
#227609=CARTESIAN_POINT('Ctrl Pts',(-0.457872079000056,11.6,10.957484748));
#227610=CARTESIAN_POINT('Ctrl Pts',(-0.458995091000055,15.2,10.960273017));
#227611=CARTESIAN_POINT('Ctrl Pts',(-0.458995091000055,11.6,10.960273017));
#227612=CARTESIAN_POINT('Ctrl Pts',(-0.460122403000056,15.2,10.963065359));
#227613=CARTESIAN_POINT('Ctrl Pts',(-0.460122403000056,11.6,10.963065359));
#227614=CARTESIAN_POINT('Ctrl Pts',(-0.461254017000057,15.2,10.965861764));
#227615=CARTESIAN_POINT('Ctrl Pts',(-0.461254017000057,11.6,10.965861764));
#227616=CARTESIAN_POINT('Ctrl Pts',(-0.462389938000056,15.2,10.96866222));
#227617=CARTESIAN_POINT('Ctrl Pts',(-0.462389938000056,11.6,10.96866222));
#227618=CARTESIAN_POINT('Ctrl Pts',(-0.463530169000055,15.2,10.971466714));
#227619=CARTESIAN_POINT('Ctrl Pts',(-0.463530169000055,11.6,10.971466714));
#227620=CARTESIAN_POINT('Ctrl Pts',(-0.464674714000056,15.2,10.974275236));
#227621=CARTESIAN_POINT('Ctrl Pts',(-0.464674714000056,11.6,10.974275236));
#227622=CARTESIAN_POINT('Ctrl Pts',(-0.465823576000056,15.2,10.977087774));
#227623=CARTESIAN_POINT('Ctrl Pts',(-0.465823576000056,11.6,10.977087774));
#227624=CARTESIAN_POINT('Ctrl Pts',(-0.466976757000056,15.2,10.979904316));
#227625=CARTESIAN_POINT('Ctrl Pts',(-0.466976757000056,11.6,10.979904316));
#227626=CARTESIAN_POINT('Ctrl Pts',(-0.468134263000056,15.2,10.982724851));
#227627=CARTESIAN_POINT('Ctrl Pts',(-0.468134263000056,11.6,10.982724851));
#227628=CARTESIAN_POINT('Ctrl Pts',(-0.469296095000056,15.2,10.985549367));
#227629=CARTESIAN_POINT('Ctrl Pts',(-0.469296095000056,11.6,10.985549367));
#227630=CARTESIAN_POINT('Ctrl Pts',(-0.470462257000056,15.2,10.988377854));
#227631=CARTESIAN_POINT('Ctrl Pts',(-0.470462257000056,11.6,10.988377854));
#227632=CARTESIAN_POINT('Ctrl Pts',(-0.471632753000056,15.2,10.991210298));
#227633=CARTESIAN_POINT('Ctrl Pts',(-0.471632753000056,11.6,10.991210298));
#227634=CARTESIAN_POINT('Ctrl Pts',(-0.472807585000057,15.2,10.99404669));
#227635=CARTESIAN_POINT('Ctrl Pts',(-0.472807585000057,11.6,10.99404669));
#227636=CARTESIAN_POINT('Ctrl Pts',(-0.473986758000056,15.2,10.996887017));
#227637=CARTESIAN_POINT('Ctrl Pts',(-0.473986758000056,11.6,10.996887017));
#227638=CARTESIAN_POINT('Ctrl Pts',(-0.475170273000056,15.2,10.999731268));
#227639=CARTESIAN_POINT('Ctrl Pts',(-0.475170273000056,11.6,10.999731268));
#227640=CARTESIAN_POINT('Ctrl Pts',(-0.476358135000057,15.2,11.002579432));
#227641=CARTESIAN_POINT('Ctrl Pts',(-0.476358135000057,11.6,11.002579432));
#227642=CARTESIAN_POINT('Ctrl Pts',(-0.477550347000056,15.2,11.005431497));
#227643=CARTESIAN_POINT('Ctrl Pts',(-0.477550347000056,11.6,11.005431497));
#227644=CARTESIAN_POINT('Ctrl Pts',(-0.478746911000056,15.2,11.008287452));
#227645=CARTESIAN_POINT('Ctrl Pts',(-0.478746911000056,11.6,11.008287452));
#227646=CARTESIAN_POINT('Ctrl Pts',(-0.479947831000055,15.2,11.011147286));
#227647=CARTESIAN_POINT('Ctrl Pts',(-0.479947831000055,11.6,11.011147286));
#227648=CARTESIAN_POINT('Ctrl Pts',(-0.481153110000055,15.2,11.014010989));
#227649=CARTESIAN_POINT('Ctrl Pts',(-0.481153110000055,11.6,11.014010989));
#227650=CARTESIAN_POINT('Ctrl Pts',(-0.482362752000055,15.2,11.016878547));
#227651=CARTESIAN_POINT('Ctrl Pts',(-0.482362752000055,11.6,11.016878547));
#227652=CARTESIAN_POINT('Ctrl Pts',(-0.483576758000056,15.2,11.01974995));
#227653=CARTESIAN_POINT('Ctrl Pts',(-0.483576758000056,11.6,11.01974995));
#227654=CARTESIAN_POINT('Ctrl Pts',(-0.484795134000056,15.2,11.022625187));
#227655=CARTESIAN_POINT('Ctrl Pts',(-0.484795134000056,11.6,11.022625187));
#227656=CARTESIAN_POINT('Ctrl Pts',(-0.486017882000055,15.2,11.025504248));
#227657=CARTESIAN_POINT('Ctrl Pts',(-0.486017882000055,11.6,11.025504248));
#227658=CARTESIAN_POINT('Ctrl Pts',(-0.487245003000056,15.2,11.028387119));
#227659=CARTESIAN_POINT('Ctrl Pts',(-0.487245003000056,11.6,11.028387119));
#227660=CARTESIAN_POINT('Ctrl Pts',(-0.488476503000056,15.2,11.031273791));
#227661=CARTESIAN_POINT('Ctrl Pts',(-0.488476503000056,11.6,11.031273791));
#227662=CARTESIAN_POINT('Ctrl Pts',(-0.489712382000055,15.2,11.034164252));
#227663=CARTESIAN_POINT('Ctrl Pts',(-0.489712382000055,11.6,11.034164252));
#227664=CARTESIAN_POINT('Ctrl Pts',(-0.490952647000055,15.2,11.037058492));
#227665=CARTESIAN_POINT('Ctrl Pts',(-0.490952647000055,11.6,11.037058492));
#227666=CARTESIAN_POINT('Ctrl Pts',(-0.492197298000056,15.2,11.039956498));
#227667=CARTESIAN_POINT('Ctrl Pts',(-0.492197298000056,11.6,11.039956498));
#227668=CARTESIAN_POINT('Ctrl Pts',(-0.493446339000055,15.2,11.042858261));
#227669=CARTESIAN_POINT('Ctrl Pts',(-0.493446339000055,11.6,11.042858261));
#227670=CARTESIAN_POINT('Ctrl Pts',(-0.494699772000056,15.2,11.045763768));
#227671=CARTESIAN_POINT('Ctrl Pts',(-0.494699772000056,11.6,11.045763768));
#227672=CARTESIAN_POINT('Ctrl Pts',(-0.495957601000055,15.2,11.04867301));
#227673=CARTESIAN_POINT('Ctrl Pts',(-0.495957601000055,11.6,11.04867301));
#227674=CARTESIAN_POINT('Ctrl Pts',(-0.497219830000055,15.2,11.051585974));
#227675=CARTESIAN_POINT('Ctrl Pts',(-0.497219830000055,11.6,11.051585974));
#227676=CARTESIAN_POINT('Ctrl Pts',(-0.498486460000055,15.2,11.054502651));
#227677=CARTESIAN_POINT('Ctrl Pts',(-0.498486460000055,11.6,11.054502651));
#227678=CARTESIAN_POINT('Ctrl Pts',(-0.499757495000056,15.2,11.057423028));
#227679=CARTESIAN_POINT('Ctrl Pts',(-0.499757495000056,11.6,11.057423028));
#227680=CARTESIAN_POINT('Ctrl Pts',(-0.501032937000057,15.2,11.060347096));
#227681=CARTESIAN_POINT('Ctrl Pts',(-0.501032937000057,11.6,11.060347096));
#227682=CARTESIAN_POINT('Ctrl Pts',(-0.502312790000056,15.2,11.063274844));
#227683=CARTESIAN_POINT('Ctrl Pts',(-0.502312790000056,11.6,11.063274844));
#227684=CARTESIAN_POINT('Ctrl Pts',(-0.503597056000055,15.2,11.06620626));
#227685=CARTESIAN_POINT('Ctrl Pts',(-0.503597056000055,11.6,11.06620626));
#227686=CARTESIAN_POINT('Ctrl Pts',(-0.504885739000055,15.2,11.069141332));
#227687=CARTESIAN_POINT('Ctrl Pts',(-0.504885739000055,11.6,11.069141332));
#227688=CARTESIAN_POINT('Ctrl Pts',(-0.506178839000055,15.2,11.072080052));
#227689=CARTESIAN_POINT('Ctrl Pts',(-0.506178839000055,11.6,11.072080052));
#227690=CARTESIAN_POINT('Ctrl Pts',(-0.507476363000056,15.2,11.075022407));
#227691=CARTESIAN_POINT('Ctrl Pts',(-0.507476363000056,11.6,11.075022407));
#227692=CARTESIAN_POINT('Ctrl Pts',(-0.508778311000055,15.2,11.077968388));
#227693=CARTESIAN_POINT('Ctrl Pts',(-0.508778311000055,11.6,11.077968388));
#227694=CARTESIAN_POINT('Ctrl Pts',(-0.510084686000055,15.2,11.080917983));
#227695=CARTESIAN_POINT('Ctrl Pts',(-0.510084686000055,11.6,11.080917983));
#227696=CARTESIAN_POINT('Ctrl Pts',(-0.511395493000055,15.2,11.08387118));
#227697=CARTESIAN_POINT('Ctrl Pts',(-0.511395493000055,11.6,11.08387118));
#227698=CARTESIAN_POINT('Ctrl Pts',(-0.512710732000056,15.2,11.086827971));
#227699=CARTESIAN_POINT('Ctrl Pts',(-0.512710732000056,11.6,11.086827971));
#227700=CARTESIAN_POINT('Ctrl Pts',(-0.514030407000057,15.2,11.089788344));
#227701=CARTESIAN_POINT('Ctrl Pts',(-0.514030407000057,11.6,11.089788344));
#227702=CARTESIAN_POINT('Ctrl Pts',(-0.515354521000055,15.2,11.092752288));
#227703=CARTESIAN_POINT('Ctrl Pts',(-0.515354521000055,11.6,11.092752288));
#227704=CARTESIAN_POINT('Ctrl Pts',(-0.516683076000056,15.2,11.095719793));
#227705=CARTESIAN_POINT('Ctrl Pts',(-0.516683076000056,11.6,11.095719793));
#227706=CARTESIAN_POINT('Ctrl Pts',(-0.518016075000055,15.2,11.098690848));
#227707=CARTESIAN_POINT('Ctrl Pts',(-0.518016075000055,11.6,11.098690848));
#227708=CARTESIAN_POINT('Ctrl Pts',(-0.519353523000056,15.2,11.101665442));
#227709=CARTESIAN_POINT('Ctrl Pts',(-0.519353523000056,11.6,11.101665442));
#227710=CARTESIAN_POINT('Ctrl Pts',(-0.520695418000056,15.2,11.104643565));
#227711=CARTESIAN_POINT('Ctrl Pts',(-0.520695418000056,11.6,11.104643565));
#227712=CARTESIAN_POINT('Ctrl Pts',(-0.522041766000055,15.2,11.107625205));
#227713=CARTESIAN_POINT('Ctrl Pts',(-0.522041766000055,11.6,11.107625205));
#227714=CARTESIAN_POINT('Ctrl Pts',(-0.523392569000055,15.2,11.110610353));
#227715=CARTESIAN_POINT('Ctrl Pts',(-0.523392569000055,11.6,11.110610353));
#227716=CARTESIAN_POINT('Ctrl Pts',(-0.524747830000055,15.2,11.113598997));
#227717=CARTESIAN_POINT('Ctrl Pts',(-0.524747830000055,11.6,11.113598997));
#227718=CARTESIAN_POINT('Ctrl Pts',(-0.526107551000056,15.2,11.116591128));
#227719=CARTESIAN_POINT('Ctrl Pts',(-0.526107551000056,11.6,11.116591128));
#227720=CARTESIAN_POINT('Ctrl Pts',(-0.527471735000056,15.2,11.119586736));
#227721=CARTESIAN_POINT('Ctrl Pts',(-0.527471735000056,11.6,11.119586736));
#227722=CARTESIAN_POINT('Ctrl Pts',(-0.528840384000056,15.2,11.122585808));
#227723=CARTESIAN_POINT('Ctrl Pts',(-0.528840384000056,11.6,11.122585808));
#227724=CARTESIAN_POINT('Ctrl Pts',(-0.530213502000055,15.2,11.125588335));
#227725=CARTESIAN_POINT('Ctrl Pts',(-0.530213502000055,11.6,11.125588335));
#227726=CARTESIAN_POINT('Ctrl Pts',(-0.531591090000055,15.2,11.128594306));
#227727=CARTESIAN_POINT('Ctrl Pts',(-0.531591090000055,11.6,11.128594306));
#227728=CARTESIAN_POINT('Ctrl Pts',(-0.532973152000055,15.2,11.131603711));
#227729=CARTESIAN_POINT('Ctrl Pts',(-0.532973152000055,11.6,11.131603711));
#227730=CARTESIAN_POINT('Ctrl Pts',(-0.534359689000056,15.2,11.134616539));
#227731=CARTESIAN_POINT('Ctrl Pts',(-0.534359689000056,11.6,11.134616539));
#227732=CARTESIAN_POINT('Ctrl Pts',(-0.535750704000056,15.2,11.137632782));
#227733=CARTESIAN_POINT('Ctrl Pts',(-0.535750704000056,11.6,11.137632782));
#227734=CARTESIAN_POINT('Ctrl Pts',(-0.537146201000055,15.2,11.140652425));
#227735=CARTESIAN_POINT('Ctrl Pts',(-0.537146201000055,11.6,11.140652425));
#227736=CARTESIAN_POINT('Ctrl Pts',(-0.538546181000056,15.2,11.143675461));
#227737=CARTESIAN_POINT('Ctrl Pts',(-0.538546181000056,11.6,11.143675461));
#227738=CARTESIAN_POINT('Ctrl Pts',(-0.539950647000056,15.2,11.14670188));
#227739=CARTESIAN_POINT('Ctrl Pts',(-0.539950647000056,11.6,11.14670188));
#227740=CARTESIAN_POINT('Ctrl Pts',(-0.541359602000057,15.2,11.149731669));
#227741=CARTESIAN_POINT('Ctrl Pts',(-0.541359602000057,11.6,11.149731669));
#227742=CARTESIAN_POINT('Ctrl Pts',(-0.542773047000056,15.2,11.15276482));
#227743=CARTESIAN_POINT('Ctrl Pts',(-0.542773047000056,11.6,11.15276482));
#227744=CARTESIAN_POINT('Ctrl Pts',(-0.544190986000055,15.2,11.155801321));
#227745=CARTESIAN_POINT('Ctrl Pts',(-0.544190986000055,11.6,11.155801321));
#227746=CARTESIAN_POINT('Ctrl Pts',(-0.545613422000055,15.2,11.158841163));
#227747=CARTESIAN_POINT('Ctrl Pts',(-0.545613422000055,11.6,11.158841163));
#227748=CARTESIAN_POINT('Ctrl Pts',(-0.547040355000057,15.2,11.161884336));
#227749=CARTESIAN_POINT('Ctrl Pts',(-0.547040355000057,11.6,11.161884336));
#227750=CARTESIAN_POINT('Ctrl Pts',(-0.548471788000056,15.2,11.164930828));
#227751=CARTESIAN_POINT('Ctrl Pts',(-0.548471788000056,11.6,11.164930828));
#227752=CARTESIAN_POINT('Ctrl Pts',(-0.549907726000055,15.2,11.167980631));
#227753=CARTESIAN_POINT('Ctrl Pts',(-0.549907726000055,11.6,11.167980631));
#227754=CARTESIAN_POINT('Ctrl Pts',(-0.551348168000055,15.2,11.171033732));
#227755=CARTESIAN_POINT('Ctrl Pts',(-0.551348168000055,11.6,11.171033732));
#227756=CARTESIAN_POINT('Ctrl Pts',(-0.552793119000056,15.2,11.174090124));
#227757=CARTESIAN_POINT('Ctrl Pts',(-0.552793119000056,11.6,11.174090124));
#227758=CARTESIAN_POINT('Ctrl Pts',(-0.554242580000055,15.2,11.177149794));
#227759=CARTESIAN_POINT('Ctrl Pts',(-0.554242580000055,11.6,11.177149794));
#227760=CARTESIAN_POINT('Ctrl Pts',(-0.555696553000056,15.2,11.180212734));
#227761=CARTESIAN_POINT('Ctrl Pts',(-0.555696553000056,11.6,11.180212734));
#227762=CARTESIAN_POINT('Ctrl Pts',(-0.557155043000056,15.2,11.183278932));
#227763=CARTESIAN_POINT('Ctrl Pts',(-0.557155043000056,11.6,11.183278932));
#227764=CARTESIAN_POINT('Ctrl Pts',(-0.558618050000056,15.2,11.18634838));
#227765=CARTESIAN_POINT('Ctrl Pts',(-0.558618050000056,11.6,11.18634838));
#227766=CARTESIAN_POINT('Ctrl Pts',(-0.560085576000056,15.2,11.189421065));
#227767=CARTESIAN_POINT('Ctrl Pts',(-0.560085576000056,11.6,11.189421065));
#227768=CARTESIAN_POINT('Ctrl Pts',(-0.561557624000055,15.2,11.192496979));
#227769=CARTESIAN_POINT('Ctrl Pts',(-0.561557624000055,11.6,11.192496979));
#227770=CARTESIAN_POINT('Ctrl Pts',(-0.563034196000055,15.2,11.195576112));
#227771=CARTESIAN_POINT('Ctrl Pts',(-0.563034196000055,11.6,11.195576112));
#227772=CARTESIAN_POINT('Ctrl Pts',(-0.564515296000057,15.2,11.198658454));
#227773=CARTESIAN_POINT('Ctrl Pts',(-0.564515296000057,11.6,11.198658454));
#227774=CARTESIAN_POINT('Ctrl Pts',(-0.566000924000055,15.2,11.201743993));
#227775=CARTESIAN_POINT('Ctrl Pts',(-0.566000924000055,11.6,11.201743993));
#227776=CARTESIAN_POINT('Ctrl Pts',(-0.567491083000055,15.2,11.204832722));
#227777=CARTESIAN_POINT('Ctrl Pts',(-0.567491083000055,11.6,11.204832722));
#227778=CARTESIAN_POINT('Ctrl Pts',(-0.568985776000056,15.2,11.207924627));
#227779=CARTESIAN_POINT('Ctrl Pts',(-0.568985776000056,11.6,11.207924627));
#227780=CARTESIAN_POINT('Ctrl Pts',(-0.570485006000055,15.2,11.211019702));
#227781=CARTESIAN_POINT('Ctrl Pts',(-0.570485006000055,11.6,11.211019702));
#227782=CARTESIAN_POINT('Ctrl Pts',(-0.571988772000056,15.2,11.214117935));
#227783=CARTESIAN_POINT('Ctrl Pts',(-0.571988772000056,11.6,11.214117935));
#227784=CARTESIAN_POINT('Ctrl Pts',(-0.573497080000056,15.2,11.217219317));
#227785=CARTESIAN_POINT('Ctrl Pts',(-0.573497080000056,11.6,11.217219317));
#227786=CARTESIAN_POINT('Ctrl Pts',(-0.575009929000055,15.2,11.220323837));
#227787=CARTESIAN_POINT('Ctrl Pts',(-0.575009929000055,11.6,11.220323837));
#227788=CARTESIAN_POINT('Ctrl Pts',(-0.576527323000056,15.2,11.223431485));
#227789=CARTESIAN_POINT('Ctrl Pts',(-0.576527323000056,11.6,11.223431485));
#227790=CARTESIAN_POINT('Ctrl Pts',(-0.578049263000056,15.2,11.226542252));
#227791=CARTESIAN_POINT('Ctrl Pts',(-0.578049263000056,11.6,11.226542252));
#227792=CARTESIAN_POINT('Ctrl Pts',(-0.579575753000056,15.2,11.229656129));
#227793=CARTESIAN_POINT('Ctrl Pts',(-0.579575753000056,11.6,11.229656129));
#227794=CARTESIAN_POINT('Ctrl Pts',(-0.581106795000055,15.2,11.232773103));
#227795=CARTESIAN_POINT('Ctrl Pts',(-0.581106795000055,11.6,11.232773103));
#227796=CARTESIAN_POINT('Ctrl Pts',(-0.582642388000056,15.2,11.235893167));
#227797=CARTESIAN_POINT('Ctrl Pts',(-0.582642388000056,11.6,11.235893167));
#227798=CARTESIAN_POINT('Ctrl Pts',(-0.584182538000055,15.2,11.239016311));
#227799=CARTESIAN_POINT('Ctrl Pts',(-0.584182538000055,11.6,11.239016311));
#227800=CARTESIAN_POINT('Ctrl Pts',(-0.585727245000056,15.2,11.242142523));
#227801=CARTESIAN_POINT('Ctrl Pts',(-0.585727245000056,11.6,11.242142523));
#227802=CARTESIAN_POINT('Ctrl Pts',(-0.587276512000056,15.2,11.245271795));
#227803=CARTESIAN_POINT('Ctrl Pts',(-0.587276512000056,11.6,11.245271795));
#227804=CARTESIAN_POINT('Ctrl Pts',(-0.588830340000056,15.2,11.248404117));
#227805=CARTESIAN_POINT('Ctrl Pts',(-0.588830340000056,11.6,11.248404117));
#227806=CARTESIAN_POINT('Ctrl Pts',(-0.590388732000056,15.2,11.251539479));
#227807=CARTESIAN_POINT('Ctrl Pts',(-0.590388732000056,11.6,11.251539479));
#227808=CARTESIAN_POINT('Ctrl Pts',(-0.591951691000056,15.2,11.254677871));
#227809=CARTESIAN_POINT('Ctrl Pts',(-0.591951691000056,11.6,11.254677871));
#227810=CARTESIAN_POINT('Ctrl Pts',(-0.593519216000056,15.2,11.257819284));
#227811=CARTESIAN_POINT('Ctrl Pts',(-0.593519216000056,11.6,11.257819284));
#227812=CARTESIAN_POINT('Ctrl Pts',(-0.595091313000056,15.2,11.260963708));
#227813=CARTESIAN_POINT('Ctrl Pts',(-0.595091313000056,11.6,11.260963708));
#227814=CARTESIAN_POINT('Ctrl Pts',(-0.596667980000056,15.2,11.264111132));
#227815=CARTESIAN_POINT('Ctrl Pts',(-0.596667980000056,11.6,11.264111132));
#227816=CARTESIAN_POINT('Ctrl Pts',(-0.598249223000057,15.2,11.267261549));
#227817=CARTESIAN_POINT('Ctrl Pts',(-0.598249223000057,11.6,11.267261549));
#227818=CARTESIAN_POINT('Ctrl Pts',(-0.599835040000055,15.2,11.270414946));
#227819=CARTESIAN_POINT('Ctrl Pts',(-0.599835040000055,11.6,11.270414946));
#227820=CARTESIAN_POINT('Ctrl Pts',(-0.601425437000056,15.2,11.273571316));
#227821=CARTESIAN_POINT('Ctrl Pts',(-0.601425437000056,11.6,11.273571316));
#227822=CARTESIAN_POINT('Ctrl Pts',(-0.603020414000056,15.2,11.276730648));
#227823=CARTESIAN_POINT('Ctrl Pts',(-0.603020414000056,11.6,11.276730648));
#227824=CARTESIAN_POINT('Ctrl Pts',(-0.604619973000055,15.2,11.279892933));
#227825=CARTESIAN_POINT('Ctrl Pts',(-0.604619973000055,11.6,11.279892933));
#227826=CARTESIAN_POINT('Ctrl Pts',(-0.606224115000057,15.2,11.283058162));
#227827=CARTESIAN_POINT('Ctrl Pts',(-0.606224115000057,11.6,11.283058162));
#227828=CARTESIAN_POINT('Ctrl Pts',(-0.607832844000056,15.2,11.286226324));
#227829=CARTESIAN_POINT('Ctrl Pts',(-0.607832844000056,11.6,11.286226324));
#227830=CARTESIAN_POINT('Ctrl Pts',(-0.609446161000056,15.2,11.28939741));
#227831=CARTESIAN_POINT('Ctrl Pts',(-0.609446161000056,11.6,11.28939741));
#227832=CARTESIAN_POINT('Ctrl Pts',(-0.611064067000056,15.2,11.29257141));
#227833=CARTESIAN_POINT('Ctrl Pts',(-0.611064067000056,11.6,11.29257141));
#227834=CARTESIAN_POINT('Ctrl Pts',(-0.612686566000056,15.2,11.295748316));
#227835=CARTESIAN_POINT('Ctrl Pts',(-0.612686566000056,11.6,11.295748316));
#227836=CARTESIAN_POINT('Ctrl Pts',(-0.614313657000055,15.2,11.298928116));
#227837=CARTESIAN_POINT('Ctrl Pts',(-0.614313657000055,11.6,11.298928116));
#227838=CARTESIAN_POINT('Ctrl Pts',(-0.615945345000056,15.2,11.302110802));
#227839=CARTESIAN_POINT('Ctrl Pts',(-0.615945345000056,11.6,11.302110802));
#227840=CARTESIAN_POINT('Ctrl Pts',(-0.617581631000055,15.2,11.305296366));
#227841=CARTESIAN_POINT('Ctrl Pts',(-0.617581631000055,11.6,11.305296366));
#227842=CARTESIAN_POINT('Ctrl Pts',(-0.619222515000055,15.2,11.308484795));
#227843=CARTESIAN_POINT('Ctrl Pts',(-0.619222515000055,11.6,11.308484795));
#227844=CARTESIAN_POINT('Ctrl Pts',(-0.620868001000057,15.2,11.311676083));
#227845=CARTESIAN_POINT('Ctrl Pts',(-0.620868001000057,11.6,11.311676083));
#227846=CARTESIAN_POINT('Ctrl Pts',(-0.622518091000056,15.2,11.314870218));
#227847=CARTESIAN_POINT('Ctrl Pts',(-0.622518091000056,11.6,11.314870218));
#227848=CARTESIAN_POINT('Ctrl Pts',(-0.624172785000056,15.2,11.318067191));
#227849=CARTESIAN_POINT('Ctrl Pts',(-0.624172785000056,11.6,11.318067191));
#227850=CARTESIAN_POINT('Ctrl Pts',(-0.625832086000055,15.2,11.321266994));
#227851=CARTESIAN_POINT('Ctrl Pts',(-0.625832086000055,11.6,11.321266994));
#227852=CARTESIAN_POINT('Ctrl Pts',(-0.627495995000055,15.2,11.324469616));
#227853=CARTESIAN_POINT('Ctrl Pts',(-0.627495995000055,11.6,11.324469616));
#227854=CARTESIAN_POINT('Ctrl Pts',(-0.629164516000056,15.2,11.327675048));
#227855=CARTESIAN_POINT('Ctrl Pts',(-0.629164516000056,11.6,11.327675048));
#227856=CARTESIAN_POINT('Ctrl Pts',(-0.630837649000057,15.2,11.330883282));
#227857=CARTESIAN_POINT('Ctrl Pts',(-0.630837649000057,11.6,11.330883282));
#227858=CARTESIAN_POINT('Ctrl Pts',(-0.632515395000055,15.2,11.334094308));
#227859=CARTESIAN_POINT('Ctrl Pts',(-0.632515395000055,11.6,11.334094308));
#227860=CARTESIAN_POINT('Ctrl Pts',(-0.634197757000056,15.2,11.337308114));
#227861=CARTESIAN_POINT('Ctrl Pts',(-0.634197757000056,11.6,11.337308114));
#227862=CARTESIAN_POINT('Ctrl Pts',(-0.635884738000057,15.2,11.340524695));
#227863=CARTESIAN_POINT('Ctrl Pts',(-0.635884738000057,11.6,11.340524695));
#227864=CARTESIAN_POINT('Ctrl Pts',(-0.637576337000055,15.2,11.343744039));
#227865=CARTESIAN_POINT('Ctrl Pts',(-0.637576337000055,11.6,11.343744039));
#227866=CARTESIAN_POINT('Ctrl Pts',(-0.639272558000057,15.2,11.346966136));
#227867=CARTESIAN_POINT('Ctrl Pts',(-0.639272558000057,11.6,11.346966136));
#227868=CARTESIAN_POINT('Ctrl Pts',(-0.640973402000055,15.2,11.350190979));
#227869=CARTESIAN_POINT('Ctrl Pts',(-0.640973402000055,11.6,11.350190979));
#227870=CARTESIAN_POINT('Ctrl Pts',(-0.642678870000056,15.2,11.353418558));
#227871=CARTESIAN_POINT('Ctrl Pts',(-0.642678870000056,11.6,11.353418558));
#227872=CARTESIAN_POINT('Ctrl Pts',(-0.644388964000056,15.2,11.356648862));
#227873=CARTESIAN_POINT('Ctrl Pts',(-0.644388964000056,11.6,11.356648862));
#227874=CARTESIAN_POINT('Ctrl Pts',(-0.646103687000057,15.2,11.359881884));
#227875=CARTESIAN_POINT('Ctrl Pts',(-0.646103687000057,11.6,11.359881884));
#227876=CARTESIAN_POINT('Ctrl Pts',(-0.647823040000055,15.2,11.363117614));
#227877=CARTESIAN_POINT('Ctrl Pts',(-0.647823040000055,11.6,11.363117614));
#227878=CARTESIAN_POINT('Ctrl Pts',(-0.649547023000056,15.2,11.366356043));
#227879=CARTESIAN_POINT('Ctrl Pts',(-0.649547023000056,11.6,11.366356043));
#227880=CARTESIAN_POINT('Ctrl Pts',(-0.651275640000056,15.2,11.369597161));
#227881=CARTESIAN_POINT('Ctrl Pts',(-0.651275640000056,11.6,11.369597161));
#227882=CARTESIAN_POINT('Ctrl Pts',(-0.653008892000055,15.2,11.37284096));
#227883=CARTESIAN_POINT('Ctrl Pts',(-0.653008892000055,11.6,11.37284096));
#227884=CARTESIAN_POINT('Ctrl Pts',(-0.654746780000056,15.2,11.37608743));
#227885=CARTESIAN_POINT('Ctrl Pts',(-0.654746780000056,11.6,11.37608743));
#227886=CARTESIAN_POINT('Ctrl Pts',(-0.656489306000055,15.2,11.379336561));
#227887=CARTESIAN_POINT('Ctrl Pts',(-0.656489306000055,11.6,11.379336561));
#227888=CARTESIAN_POINT('Ctrl Pts',(-0.658236473000056,15.2,11.382588344));
#227889=CARTESIAN_POINT('Ctrl Pts',(-0.658236473000056,11.6,11.382588344));
#227890=CARTESIAN_POINT('Ctrl Pts',(-0.659988281000056,15.2,11.385842773));
#227891=CARTESIAN_POINT('Ctrl Pts',(-0.659988281000056,11.6,11.385842773));
#227892=CARTESIAN_POINT('Ctrl Pts',(-0.661744730000056,15.2,11.389099835));
#227893=CARTESIAN_POINT('Ctrl Pts',(-0.661744730000056,11.6,11.389099835));
#227894=CARTESIAN_POINT('Ctrl Pts',(-0.663505825000056,15.2,11.392359523));
#227895=CARTESIAN_POINT('Ctrl Pts',(-0.663505825000056,11.6,11.392359523));
#227896=CARTESIAN_POINT('Ctrl Pts',(-0.665271567000056,15.2,11.395621828));
#227897=CARTESIAN_POINT('Ctrl Pts',(-0.665271567000056,11.6,11.395621828));
#227898=CARTESIAN_POINT('Ctrl Pts',(-0.667041956000055,15.2,11.398886739));
#227899=CARTESIAN_POINT('Ctrl Pts',(-0.667041956000055,11.6,11.398886739));
#227900=CARTESIAN_POINT('Ctrl Pts',(-0.668816993000056,15.2,11.402154251));
#227901=CARTESIAN_POINT('Ctrl Pts',(-0.668816993000056,11.6,11.402154251));
#227902=CARTESIAN_POINT('Ctrl Pts',(-0.670596683000056,15.2,11.405424351));
#227903=CARTESIAN_POINT('Ctrl Pts',(-0.670596683000056,11.6,11.405424351));
#227904=CARTESIAN_POINT('Ctrl Pts',(-0.672381024000056,15.2,11.408697033));
#227905=CARTESIAN_POINT('Ctrl Pts',(-0.672381024000056,11.6,11.408697033));
#227906=CARTESIAN_POINT('Ctrl Pts',(-0.674170019000057,15.2,11.411972284));
#227907=CARTESIAN_POINT('Ctrl Pts',(-0.674170019000057,11.6,11.411972284));
#227908=CARTESIAN_POINT('Ctrl Pts',(-0.675963671000056,15.2,11.415250096));
#227909=CARTESIAN_POINT('Ctrl Pts',(-0.675963671000056,11.6,11.415250096));
#227910=CARTESIAN_POINT('Ctrl Pts',(-0.677761979000057,15.2,11.418530461));
#227911=CARTESIAN_POINT('Ctrl Pts',(-0.677761979000057,11.6,11.418530461));
#227912=CARTESIAN_POINT('Ctrl Pts',(-0.679564947000056,15.2,11.421813369));
#227913=CARTESIAN_POINT('Ctrl Pts',(-0.679564947000056,11.6,11.421813369));
#227914=CARTESIAN_POINT('Ctrl Pts',(-0.681372573000055,15.2,11.425098812));
#227915=CARTESIAN_POINT('Ctrl Pts',(-0.681372573000055,11.6,11.425098812));
#227916=CARTESIAN_POINT('Ctrl Pts',(-0.683184863000056,15.2,11.428386781));
#227917=CARTESIAN_POINT('Ctrl Pts',(-0.683184863000056,11.6,11.428386781));
#227918=CARTESIAN_POINT('Ctrl Pts',(-0.685001814000056,15.2,11.431677269));
#227919=CARTESIAN_POINT('Ctrl Pts',(-0.685001814000056,11.6,11.431677269));
#227920=CARTESIAN_POINT('Ctrl Pts',(-0.686823430000055,15.2,11.434970269));
#227921=CARTESIAN_POINT('Ctrl Pts',(-0.686823430000055,11.6,11.434970269));
#227922=CARTESIAN_POINT('Ctrl Pts',(-0.688649711000057,15.2,11.438265769));
#227923=CARTESIAN_POINT('Ctrl Pts',(-0.688649711000057,11.6,11.438265769));
#227924=CARTESIAN_POINT('Ctrl Pts',(-0.690480660000056,15.2,11.441563763));
#227925=CARTESIAN_POINT('Ctrl Pts',(-0.690480660000056,11.6,11.441563763));
#227926=CARTESIAN_POINT('Ctrl Pts',(-0.692316277000057,15.2,11.444864239));
#227927=CARTESIAN_POINT('Ctrl Pts',(-0.692316277000057,11.6,11.444864239));
#227928=CARTESIAN_POINT('Ctrl Pts',(-0.694156564000057,15.2,11.448167187));
#227929=CARTESIAN_POINT('Ctrl Pts',(-0.694156564000057,11.6,11.448167187));
#227930=CARTESIAN_POINT('Ctrl Pts',(-0.696001525000056,15.2,11.451472594));
#227931=CARTESIAN_POINT('Ctrl Pts',(-0.696001525000056,11.6,11.451472594));
#227932=CARTESIAN_POINT('Ctrl Pts',(-0.697851160000056,15.2,11.454780452));
#227933=CARTESIAN_POINT('Ctrl Pts',(-0.697851160000056,11.6,11.454780452));
#227934=CARTESIAN_POINT('Ctrl Pts',(-0.699705469000056,15.2,11.458090751));
#227935=CARTESIAN_POINT('Ctrl Pts',(-0.699705469000056,11.6,11.458090751));
#227936=CARTESIAN_POINT('Ctrl Pts',(-0.701564456000057,15.2,11.461403481));
#227937=CARTESIAN_POINT('Ctrl Pts',(-0.701564456000057,11.6,11.461403481));
#227938=CARTESIAN_POINT('Ctrl Pts',(-0.703428121000057,15.2,11.464718637));
#227939=CARTESIAN_POINT('Ctrl Pts',(-0.703428121000057,11.6,11.464718637));
#227940=CARTESIAN_POINT('Ctrl Pts',(-0.705296465000057,15.2,11.468036216));
#227941=CARTESIAN_POINT('Ctrl Pts',(-0.705296465000057,11.6,11.468036216));
#227942=CARTESIAN_POINT('Ctrl Pts',(-0.707169486000057,15.2,11.471356215));
#227943=CARTESIAN_POINT('Ctrl Pts',(-0.707169486000057,11.6,11.471356215));
#227944=CARTESIAN_POINT('Ctrl Pts',(-0.708671646000055,15.2,11.474014149));
#227945=CARTESIAN_POINT('Ctrl Pts',(-0.708671646000055,11.6,11.474014149));
#227946=CARTESIAN_POINT('Ctrl Pts',(-0.709800371000057,15.2,11.476008688));
#227947=CARTESIAN_POINT('Ctrl Pts',(-0.709800371000057,11.6,11.476008688));
#227948=CARTESIAN_POINT('Ctrl Pts',(-0.710553791000056,15.2,11.477338864));
#227949=CARTESIAN_POINT('Ctrl Pts',(-0.710553791000056,11.6,11.477338864));
#227950=CARTESIAN_POINT('Ctrl Pts',(-0.710930735000056,15.2,11.478004073));
#227951=CARTESIAN_POINT('Ctrl Pts',(-0.710930735000056,11.6,11.478004073));
#227952=CARTESIAN_POINT('Ctrl Pts',(-0.292001930000056,15.2,10.370890024));
#227953=CARTESIAN_POINT('Ctrl Pts',(-0.29220549901488,15.2,10.372665048257));
#227954=CARTESIAN_POINT('Ctrl Pts',(-0.292420934152544,15.2,10.3744962450942));
#227955=CARTESIAN_POINT('Ctrl Pts',(-0.29264874396675,15.2,10.3763825865516));
#227956=CARTESIAN_POINT('Ctrl Pts',(-0.292877652395031,15.2,10.378278024901));
#227957=CARTESIAN_POINT('Ctrl Pts',(-0.293119060472346,15.2,10.3802291369147));
#227958=CARTESIAN_POINT('Ctrl Pts',(-0.293373491749677,15.2,10.3822349054607));
#227959=CARTESIAN_POINT('Ctrl Pts',(-0.293712733429673,15.2,10.3849092633399));
#227960=CARTESIAN_POINT('Ctrl Pts',(-0.294075124384088,15.2,10.3876807806492));
#227961=CARTESIAN_POINT('Ctrl Pts',(-0.294461852490938,15.2,10.3905471173926));
#227962=CARTESIAN_POINT('Ctrl Pts',(-0.294751898564489,15.2,10.3926968699013));
#227963=CARTESIAN_POINT('Ctrl Pts',(-0.295055632160027,15.2,10.3948999596624));
#227964=CARTESIAN_POINT('Ctrl Pts',(-0.295373532483221,15.2,10.3971554301739));
#227965=CARTESIAN_POINT('Ctrl Pts',(-0.295691432806416,15.2,10.3994109006854));
#227966=CARTESIAN_POINT('Ctrl Pts',(-0.296023501634165,15.2,10.4017187517486));
#227967=CARTESIAN_POINT('Ctrl Pts',(-0.296370202703911,15.2,10.4040780504928));
#227968=CARTESIAN_POINT('Ctrl Pts',(-0.29671690380515,15.2,10.4064373494512));
#227969=CARTESIAN_POINT('Ctrl Pts',(-0.297078237096281,15.2,10.4088480977447));
#227970=CARTESIAN_POINT('Ctrl Pts',(-0.297454650303147,15.2,10.4113093850048));
#227971=CARTESIAN_POINT('Ctrl Pts',(-0.297893798993205,15.2,10.4141808864729));
#227972=CARTESIAN_POINT('Ctrl Pts',(-0.298353477225178,15.2,10.4171211802824));
#227973=CARTESIAN_POINT('Ctrl Pts',(-0.298834369221771,15.2,10.4201288594939));
#227974=CARTESIAN_POINT('Ctrl Pts',(-0.299246562409847,15.2,10.4227068705477));
#227975=CARTESIAN_POINT('Ctrl Pts',(-0.299674342220718,15.2,10.4253343918266));
#227976=CARTESIAN_POINT('Ctrl Pts',(-0.300118128017998,15.2,10.4280105622756));
#227977=CARTESIAN_POINT('Ctrl Pts',(-0.300561913774966,15.2,10.4306867324815));
#227978=CARTESIAN_POINT('Ctrl Pts',(-0.301021703625674,15.2,10.4334115520424));
#227979=CARTESIAN_POINT('Ctrl Pts',(-0.301497903525024,15.2,10.4361841820249));
#227980=CARTESIAN_POINT('Ctrl Pts',(-0.301974103424374,15.2,10.4389568120074));
#227981=CARTESIAN_POINT('Ctrl Pts',(-0.302466713969813,15.2,10.4417772508279));
#227982=CARTESIAN_POINT('Ctrl Pts',(-0.30297612672579,15.2,10.4446446819476));
#227983=CARTESIAN_POINT('Ctrl Pts',(-0.30348553952804,15.2,10.4475121133278));
#227984=CARTESIAN_POINT('Ctrl Pts',(-0.304011754820135,15.2,10.4504265334164));
#227985=CARTESIAN_POINT('Ctrl Pts',(-0.304555152600927,15.2,10.453387143831));
#227986=CARTESIAN_POINT('Ctrl Pts',(-0.305189116604479,15.2,10.4568411889112));
#227987=CARTESIAN_POINT('Ctrl Pts',(-0.305846467136494,15.2,10.4603581000338));
#227988=CARTESIAN_POINT('Ctrl Pts',(-0.306527791710242,15.2,10.463936641445));
#227989=CARTESIAN_POINT('Ctrl Pts',(-0.307111784270228,15.2,10.4670039630128));
#227990=CARTESIAN_POINT('Ctrl Pts',(-0.307713387740921,15.2,10.4701165605774));
#227991=CARTESIAN_POINT('Ctrl Pts',(-0.308332958359225,15.2,10.4732736733357));
#227992=CARTESIAN_POINT('Ctrl Pts',(-0.308952528921253,15.2,10.4764307858073));
#227993=CARTESIAN_POINT('Ctrl Pts',(-0.309590066523853,15.2,10.4796324144928));
#227994=CARTESIAN_POINT('Ctrl Pts',(-0.310245916000022,15.2,10.4828778109582));
#227995=CARTESIAN_POINT('Ctrl Pts',(-0.310901765476191,15.2,10.4861232074236));
#227996=CARTESIAN_POINT('Ctrl Pts',(-0.311575927099688,15.2,10.4894123722348));
#227997=CARTESIAN_POINT('Ctrl Pts',(-0.312268733691382,15.2,10.4927445759443));
#227998=CARTESIAN_POINT('Ctrl Pts',(-0.312961540346006,15.2,10.4960767799566));
#227999=CARTESIAN_POINT('Ctrl Pts',(-0.313672994921877,15.2,10.4994520210167));
#228000=CARTESIAN_POINT('Ctrl Pts',(-0.31440341779631,15.2,10.5028695858724));
#228001=CARTESIAN_POINT('Ctrl Pts',(-0.315620789121003,15.2,10.5085655266779));
#228002=CARTESIAN_POINT('Ctrl Pts',(-0.316890865154458,15.2,10.5143790241343));
#228003=CARTESIAN_POINT('Ctrl Pts',(-0.318215080913419,15.2,10.5203068568622));
#228004=CARTESIAN_POINT('Ctrl Pts',(-0.319009610455399,15.2,10.5238635568866));
#228005=CARTESIAN_POINT('Ctrl Pts',(-0.31982363092424,15.2,10.5274614183316));
#228006=CARTESIAN_POINT('Ctrl Pts',(-0.320657440553881,15.2,10.5310997671984));
#228007=CARTESIAN_POINT('Ctrl Pts',(-0.321491250107784,15.2,10.5347381157346));
#228008=CARTESIAN_POINT('Ctrl Pts',(-0.322344850352457,15.2,10.5384169472249));
#228009=CARTESIAN_POINT('Ctrl Pts',(-0.323218530741291,15.2,10.5421356000232));
#228010=CARTESIAN_POINT('Ctrl Pts',(-0.324092211130125,15.2,10.5458542528215));
#228011=CARTESIAN_POINT('Ctrl Pts',(-0.324985972868309,15.2,10.549612724485));
#228012=CARTESIAN_POINT('Ctrl Pts',(-0.325900097167055,15.2,10.553410366261));
#228013=CARTESIAN_POINT('Ctrl Pts',(-0.326814221548833,15.2,10.557208008382));
#228014=CARTESIAN_POINT('Ctrl Pts',(-0.327748709641514,15.2,10.5610448175429));
#228015=CARTESIAN_POINT('Ctrl Pts',(-0.3287038350758,15.2,10.5649201568666));
#228016=CARTESIAN_POINT('Ctrl Pts',(-0.329499772894327,15.2,10.568149606127));
#228017=CARTESIAN_POINT('Ctrl Pts',(-0.330310042073378,15.2,10.5714058104271));
#228018=CARTESIAN_POINT('Ctrl Pts',(-0.331134798116238,15.2,10.5746884079293));
#228019=CARTESIAN_POINT('Ctrl Pts',(-0.331959554159098,15.2,10.5779710054315));
#228020=CARTESIAN_POINT('Ctrl Pts',(-0.332798795749401,15.2,10.5812799938229));
#228021=CARTESIAN_POINT('Ctrl Pts',(-0.333652674361709,15.2,10.5846150172278));
#228022=CARTESIAN_POINT('Ctrl Pts',(-0.334506552880944,15.2,10.5879500402692));
#228023=CARTESIAN_POINT('Ctrl Pts',(-0.335375070626419,15.2,10.5913110967615));
#228024=CARTESIAN_POINT('Ctrl Pts',(-0.336258370667821,15.2,10.5946978340986));
#228025=CARTESIAN_POINT('Ctrl Pts',(-0.337318330890808,15.2,10.5987619195676));
#228026=CARTESIAN_POINT('Ctrl Pts',(-0.338399582482505,15.2,10.6028629845068));
#228027=CARTESIAN_POINT('Ctrl Pts',(-0.339502371543545,15.2,10.6070004289839));
#228028=CARTESIAN_POINT('Ctrl Pts',(-0.340605160504416,15.2,10.6111378730852));
#228029=CARTESIAN_POINT('Ctrl Pts',(-0.341729486777676,15.2,10.6153116960487));
#228030=CARTESIAN_POINT('Ctrl Pts',(-0.3428755928245,15.2,10.619521308248));
#228031=CARTESIAN_POINT('Ctrl Pts',(-0.344021698871324,15.2,10.6237309204474));
#228032=CARTESIAN_POINT('Ctrl Pts',(-0.345189583431716,15.2,10.6279763233579));
#228033=CARTESIAN_POINT('Ctrl Pts',(-0.346379481553657,15.2,10.6322569345333));
#228034=CARTESIAN_POINT('Ctrl Pts',(-0.34756937978368,15.2,10.6365375460976));
#228035=CARTESIAN_POINT('Ctrl Pts',(-0.348781291647598,15.2,10.6408533677311));
#228036=CARTESIAN_POINT('Ctrl Pts',(-0.350015443861127,15.2,10.6452038266875));
#228037=CARTESIAN_POINT('Ctrl Pts',(-0.35145528794209,15.2,10.6502793615439));
#228038=CARTESIAN_POINT('Ctrl Pts',(-0.352925406743964,15.2,10.6554020458361));
#228039=CARTESIAN_POINT('Ctrl Pts',(-0.354426147343142,15.2,10.660570986192));
#228040=CARTESIAN_POINT('Ctrl Pts',(-0.355712496578379,15.2,10.6650015070145));
#228041=CARTESIAN_POINT('Ctrl Pts',(-0.357021345021807,15.2,10.6694660135717));
#228042=CARTESIAN_POINT('Ctrl Pts',(-0.358352906162216,15.2,10.6739639554601));
#228043=CARTESIAN_POINT('Ctrl Pts',(-0.359462540385416,15.2,10.6777122401629));
#228044=CARTESIAN_POINT('Ctrl Pts',(-0.360587946892452,15.2,10.6814837430611));
#228045=CARTESIAN_POINT('Ctrl Pts',(-0.361729247657636,15.2,10.6852781509796));
#228046=CARTESIAN_POINT('Ctrl Pts',(-0.36287054842282,15.2,10.6890725588981));
#228047=CARTESIAN_POINT('Ctrl Pts',(-0.364027741913281,15.2,10.6928898715004));
#228048=CARTESIAN_POINT('Ctrl Pts',(-0.365200947678475,15.2,10.6967297802522));
#228049=CARTESIAN_POINT('Ctrl Pts',(-0.36637415344367,15.2,10.700569689004));
#228050=CARTESIAN_POINT('Ctrl Pts',(-0.36756336964523,15.2,10.7044321930117));
#228051=CARTESIAN_POINT('Ctrl Pts',(-0.368768713674349,15.2,10.7083169859997));
#228052=CARTESIAN_POINT('Ctrl Pts',(-0.369974057572086,15.2,10.7122017785643));
#228053=CARTESIAN_POINT('Ctrl Pts',(-0.371195528302116,15.2,10.7161088606771));
#228054=CARTESIAN_POINT('Ctrl Pts',(-0.372433238096463,15.2,10.7200379299694));
#228055=CARTESIAN_POINT('Ctrl Pts',(-0.373670948025721,15.2,10.7239669996899));
#228056=CARTESIAN_POINT('Ctrl Pts',(-0.374924897418553,15.2,10.7279180584377));
#228057=CARTESIAN_POINT('Ctrl Pts',(-0.376195196375531,15.2,10.7318908049636));
#228058=CARTESIAN_POINT('Ctrl Pts',(-0.377211435596498,15.2,10.7350690023576));
#228059=CARTESIAN_POINT('Ctrl Pts',(-0.37823813745333,15.2,10.7382610825544));
#228060=CARTESIAN_POINT('Ctrl Pts',(-0.379275358792392,15.2,10.7414668912438));
#228061=CARTESIAN_POINT('Ctrl Pts',(-0.380312579990132,15.2,10.7446726994963));
#228062=CARTESIAN_POINT('Ctrl Pts',(-0.381360319825712,15.2,10.7478922394315));
#228063=CARTESIAN_POINT('Ctrl Pts',(-0.382418632293648,15.2,10.7511253597213));
#228064=CARTESIAN_POINT('Ctrl Pts',(-0.383476944905779,15.2,10.7543584804516));
#228065=CARTESIAN_POINT('Ctrl Pts',(-0.384545831121746,15.2,10.7576051824751));
#228066=CARTESIAN_POINT('Ctrl Pts',(-0.385625342458339,15.2,10.7608653170416));
#228067=CARTESIAN_POINT('Ctrl Pts',(-0.386704853794932,15.2,10.7641254516081));
#228068=CARTESIAN_POINT('Ctrl Pts',(-0.387794991685586,15.2,10.7673990188624));
#228069=CARTESIAN_POINT('Ctrl Pts',(-0.388895806413339,15.2,10.7706858728207));
#228070=CARTESIAN_POINT('Ctrl Pts',(-0.390271824598052,15.2,10.7747944395968));
#228071=CARTESIAN_POINT('Ctrl Pts',(-0.391664529609553,15.2,10.7789237657556));
#228072=CARTESIAN_POINT('Ctrl Pts',(-0.39307401681565,15.2,10.7830735691905));
#228073=CARTESIAN_POINT('Ctrl Pts',(-0.394201606764888,15.2,10.7863934124811));
#228074=CARTESIAN_POINT('Ctrl Pts',(-0.395339938962376,15.2,10.789726360612));
#228075=CARTESIAN_POINT('Ctrl Pts',(-0.396489063525012,15.2,10.7930722700166));
#228076=CARTESIAN_POINT('Ctrl Pts',(-0.397638188087647,15.2,10.7964181794212));
#228077=CARTESIAN_POINT('Ctrl Pts',(-0.398798103118186,15.2,10.7997770520689));
#228078=CARTESIAN_POINT('Ctrl Pts',(-0.399968859683108,15.2,10.8031487423096));
#228079=CARTESIAN_POINT('Ctrl Pts',(-0.401139616088514,15.2,10.8065204320908));
#228080=CARTESIAN_POINT('Ctrl Pts',(-0.402321214349639,15.2,10.8099049426655));
#228081=CARTESIAN_POINT('Ctrl Pts',(-0.403513700757539,15.2,10.8133021315143));
#228082=CARTESIAN_POINT('Ctrl Pts',(-0.404706187327917,15.2,10.816699320826));
#228083=CARTESIAN_POINT('Ctrl Pts',(-0.405909563539603,15.2,10.8201091892523));
#228084=CARTESIAN_POINT('Ctrl Pts',(-0.407123875440221,15.2,10.8235315960512));
#228085=CARTESIAN_POINT('Ctrl Pts',(-0.408338187175388,15.2,10.8269540023837));
#228086=CARTESIAN_POINT('Ctrl Pts',(-0.409563434453614,15.2,10.8303889480148));
#228087=CARTESIAN_POINT('Ctrl Pts',(-0.410799665407387,15.2,10.8338362950099));
#228088=CARTESIAN_POINT('Ctrl Pts',(-0.412654011922266,15.2,10.8390073157375));
#228089=CARTESIAN_POINT('Ctrl Pts',(-0.41453306750502,15.2,10.8442062380553));
#228090=CARTESIAN_POINT('Ctrl Pts',(-0.416436989017487,15.2,10.8494326006969));
#228091=CARTESIAN_POINT('Ctrl Pts',(-0.417706270141092,15.2,10.8529168427745));
#228092=CARTESIAN_POINT('Ctrl Pts',(-0.418986601168512,15.2,10.8564132814948));
#228093=CARTESIAN_POINT('Ctrl Pts',(-0.420278027016682,15.2,10.8599217797416));
#228094=CARTESIAN_POINT('Ctrl Pts',(-0.421892309238915,15.2,10.8643074023111));
#228095=CARTESIAN_POINT('Ctrl Pts',(-0.423523927621153,15.2,10.8687118704544));
#228096=CARTESIAN_POINT('Ctrl Pts',(-0.425172965684246,15.2,10.8731349220024));
#228097=CARTESIAN_POINT('Ctrl Pts',(-0.426492196026873,15.2,10.8766733629514));
#228098=CARTESIAN_POINT('Ctrl Pts',(-0.42782257640538,15.2,10.8802236975433));
#228099=CARTESIAN_POINT('Ctrl Pts',(-0.429164146239003,15.2,10.8837857919175));
#228100=CARTESIAN_POINT('Ctrl Pts',(-0.430505716255415,15.2,10.8873478867771));
#228101=CARTESIAN_POINT('Ctrl Pts',(-0.431858479650664,15.2,10.8909217432767));
#228102=CARTESIAN_POINT('Ctrl Pts',(-0.433222474225011,15.2,10.8945072282499));
#228103=CARTESIAN_POINT('Ctrl Pts',(-0.434586468799358,15.2,10.8980927132232));
#228104=CARTESIAN_POINT('Ctrl Pts',(-0.435961696255549,15.2,10.9016898279004));
#228105=CARTESIAN_POINT('Ctrl Pts',(-0.437348197443381,15.2,10.9052984425983));
#228106=CARTESIAN_POINT('Ctrl Pts',(-0.439081323644806,15.2,10.9098092102331));
#228107=CARTESIAN_POINT('Ctrl Pts',(-0.440832065601813,15.2,10.9143379434412));
#228108=CARTESIAN_POINT('Ctrl Pts',(-0.442600500060369,15.2,10.9188843921803));
#228109=CARTESIAN_POINT('Ctrl Pts',(-0.444015247858525,15.2,10.9225215517662));
#228110=CARTESIAN_POINT('Ctrl Pts',(-0.445441320160564,15.2,10.9261700500227));
#228111=CARTESIAN_POINT('Ctrl Pts',(-0.446878754016672,15.2,10.9298297569999));
#228112=CARTESIAN_POINT('Ctrl Pts',(-0.449034904604986,15.2,10.9353193169671));
#228113=CARTESIAN_POINT('Ctrl Pts',(-0.451216621466244,15.2,10.940834099765));
#228114=CARTESIAN_POINT('Ctrl Pts',(-0.4534240330782,15.2,10.9463736779224));
#228115=CARTESIAN_POINT('Ctrl Pts',(-0.454895640953175,15.2,10.9500667303629));
#228116=CARTESIAN_POINT('Ctrl Pts',(-0.456378668998441,15.2,10.9537708021451));
#228117=CARTESIAN_POINT('Ctrl Pts',(-0.457873153580622,15.2,10.9574857695704));
#228118=CARTESIAN_POINT('Ctrl Pts',(-0.460114880250268,15.2,10.9630582202023));
#228119=CARTESIAN_POINT('Ctrl Pts',(-0.462382385784579,15.2,10.968655181899));
#228120=CARTESIAN_POINT('Ctrl Pts',(-0.464675793116795,15.2,10.9742762396937));
#228121=CARTESIAN_POINT('Ctrl Pts',(-0.466969200657329,15.2,10.979897297999));
#228122=CARTESIAN_POINT('Ctrl Pts',(-0.469288508567733,15.2,10.9855424511073));
#228123=CARTESIAN_POINT('Ctrl Pts',(-0.471633837280656,15.2,10.9912112855845));
#228124=CARTESIAN_POINT('Ctrl Pts',(-0.473197389542904,15.2,10.9949905080544));
#228125=CARTESIAN_POINT('Ctrl Pts',(-0.474772506335361,15.2,10.9987802561602));
#228126=CARTESIAN_POINT('Ctrl Pts',(-0.476359222490603,15.2,11.0025804072557));
#228127=CARTESIAN_POINT('Ctrl Pts',(-0.477945938862034,15.2,11.0063805588689));
#228128=CARTESIAN_POINT('Ctrl Pts',(-0.479544253288192,15.2,11.0101911138653));
#228129=CARTESIAN_POINT('Ctrl Pts',(-0.481154200988244,15.2,11.014011953408));
#228130=CARTESIAN_POINT('Ctrl Pts',(-0.482764148468941,15.2,11.01783279243));
#228131=CARTESIAN_POINT('Ctrl Pts',(-0.484385728903638,15.2,11.0216639138201));
#228132=CARTESIAN_POINT('Ctrl Pts',(-0.486018975158269,15.2,11.0255052002277));
#228133=CARTESIAN_POINT('Ctrl Pts',(-0.487652221635429,15.2,11.0293464871587));
#228134=CARTESIAN_POINT('Ctrl Pts',(-0.48929713271086,15.2,11.0331979375784));
#228135=CARTESIAN_POINT('Ctrl Pts',(-0.490953743773792,15.2,11.0370594340937));
#228136=CARTESIAN_POINT('Ctrl Pts',(-0.493024507489601,15.2,11.0418863044747));
#228137=CARTESIAN_POINT('Ctrl Pts',(-0.49511354770195,15.2,11.0467288702119));
#228138=CARTESIAN_POINT('Ctrl Pts',(-0.497220930550665,15.2,11.0515869028521));
#228139=CARTESIAN_POINT('Ctrl Pts',(-0.498906836691815,15.2,11.0554733286465));
#228140=CARTESIAN_POINT('Ctrl Pts',(-0.500604480267564,15.2,11.0593696530007));
#228141=CARTESIAN_POINT('Ctrl Pts',(-0.502313893127041,15.2,11.0632757606807));
#228142=CARTESIAN_POINT('Ctrl Pts',(-0.504450659376066,15.2,11.0681583956799));
#228143=CARTESIAN_POINT('Ctrl Pts',(-0.506605814700106,15.2,11.0730563131416));
#228144=CARTESIAN_POINT('Ctrl Pts',(-0.508779417765496,15.2,11.0779692914973));
#228145=CARTESIAN_POINT('Ctrl Pts',(-0.510518300312577,15.2,11.081899674396));
#228146=CARTESIAN_POINT('Ctrl Pts',(-0.512268990654795,15.2,11.0858396936878));
#228147=CARTESIAN_POINT('Ctrl Pts',(-0.514031517029858,15.2,11.089789237404));
#228148=CARTESIAN_POINT('Ctrl Pts',(-0.515794043164776,15.2,11.0937387805822));
#228149=CARTESIAN_POINT('Ctrl Pts',(-0.517568405928673,15.2,11.0976978474562));
#228150=CARTESIAN_POINT('Ctrl Pts',(-0.519354634670766,15.2,11.101666323909));
#228151=CARTESIAN_POINT('Ctrl Pts',(-0.521587420780912,15.2,11.1066269198804));
#228152=CARTESIAN_POINT('Ctrl Pts',(-0.523838745549627,15.2,11.1116022162968));
#228153=CARTESIAN_POINT('Ctrl Pts',(-0.52610866674044,15.2,11.1165919972222));
#228154=CARTESIAN_POINT('Ctrl Pts',(-0.52792460379206,15.2,11.1205838221801));
#228155=CARTESIAN_POINT('Ctrl Pts',(-0.529752441729908,15.2,11.1245849154279));
#228156=CARTESIAN_POINT('Ctrl Pts',(-0.531592208775819,15.2,11.1285951651473));
#228157=CARTESIAN_POINT('Ctrl Pts',(-0.533891917457873,15.2,11.1336079770234));
#228158=CARTESIAN_POINT('Ctrl Pts',(-0.536210264054167,15.2,11.1386350964804));
#228159=CARTESIAN_POINT('Ctrl Pts',(-0.5385473028057,15.2,11.1436763073843));
#228160=CARTESIAN_POINT('Ctrl Pts',(-0.539949526005673,15.2,11.1467010338168));
#228161=CARTESIAN_POINT('Ctrl Pts',(-0.541358478453927,15.2,11.1497308329453));
#228162=CARTESIAN_POINT('Ctrl Pts',(-0.54277417076564,15.2,11.1527656581122));
#228163=CARTESIAN_POINT('Ctrl Pts',(-0.545133658037555,15.2,11.1578237002407));
#228164=CARTESIAN_POINT('Ctrl Pts',(-0.547511868750903,15.2,11.1628957042696));
#228165=CARTESIAN_POINT('Ctrl Pts',(-0.549908852363539,15.2,11.1679814562152));
#228166=CARTESIAN_POINT('Ctrl Pts',(-0.551347042478867,15.2,11.1710329072716));
#228167=CARTESIAN_POINT('Ctrl Pts',(-0.552791990943856,15.2,11.1740893077445));
#228168=CARTESIAN_POINT('Ctrl Pts',(-0.554243708183353,15.2,11.1771506118004));
#228169=CARTESIAN_POINT('Ctrl Pts',(-0.55569542542285,15.2,11.1802119158562));
#228170=CARTESIAN_POINT('Ctrl Pts',(-0.557153913097895,15.2,11.183278123767));
#228171=CARTESIAN_POINT('Ctrl Pts',(-0.558619179759674,15.2,11.1863491892944));
#228172=CARTESIAN_POINT('Ctrl Pts',(-0.560084446421453,15.2,11.1894202548218));
#228173=CARTESIAN_POINT('Ctrl Pts',(-0.561556491845709,15.2,11.1924961777451));
#228174=CARTESIAN_POINT('Ctrl Pts',(-0.56303532796533,15.2,11.1955769142305));
#228175=CARTESIAN_POINT('Ctrl Pts',(-0.564514164084952,15.2,11.1986576507159));
#228176=CARTESIAN_POINT('Ctrl Pts',(-0.565999790142274,15.2,11.2017431996759));
#228177=CARTESIAN_POINT('Ctrl Pts',(-0.567492216337446,15.2,11.2048335157299));
#228178=CARTESIAN_POINT('Ctrl Pts',(-0.569482118111756,15.2,11.2089539375094));
#228179=CARTESIAN_POINT('Ctrl Pts',(-0.571484110512555,15.2,11.2130828347872));
#228180=CARTESIAN_POINT('Ctrl Pts',(-0.57349821545644,15.2,11.2172201018466));
#228181=CARTESIAN_POINT('Ctrl Pts',(-0.575008794027143,15.2,11.2203230518592));
#228182=CARTESIAN_POINT('Ctrl Pts',(-0.576526185283166,15.2,11.2234307084851));
#228183=CARTESIAN_POINT('Ctrl Pts',(-0.578050400484732,15.2,11.2265430294695));
#228184=CARTESIAN_POINT('Ctrl Pts',(-0.579574615686298,15.2,11.2296553504539));
#228185=CARTESIAN_POINT('Ctrl Pts',(-0.581105655497523,15.2,11.2327723339964));
#228186=CARTESIAN_POINT('Ctrl Pts',(-0.582643527198618,15.2,11.2358939369805));
#228187=CARTESIAN_POINT('Ctrl Pts',(-0.584181398899714,15.2,11.2390155399646));
#228188=CARTESIAN_POINT('Ctrl Pts',(-0.585726104487975,15.2,11.2421417611063));
#228189=CARTESIAN_POINT('Ctrl Pts',(-0.587277652097671,15.2,11.2452725571588));
#228190=CARTESIAN_POINT('Ctrl Pts',(-0.589346382431842,15.2,11.2494469522746));
#228191=CARTESIAN_POINT('Ctrl Pts',(-0.591427277434147,15.2,11.2536294800221));
#228192=CARTESIAN_POINT('Ctrl Pts',(-0.59352035910457,15.2,11.2578200370843));
#228193=CARTESIAN_POINT('Ctrl Pts',(-0.595090170214797,15.2,11.2609629545955));
#228194=CARTESIAN_POINT('Ctrl Pts',(-0.596666836451787,15.2,11.2641103879864));
#228195=CARTESIAN_POINT('Ctrl Pts',(-0.598250366568114,15.2,11.2672622940528));
#228196=CARTESIAN_POINT('Ctrl Pts',(-0.599833896684441,15.2,11.2704142001192));
#228197=CARTESIAN_POINT('Ctrl Pts',(-0.601424291416032,15.2,11.2735705785976));
#228198=CARTESIAN_POINT('Ctrl Pts',(-0.60302155949023,15.2,11.2767313862471));
#228199=CARTESIAN_POINT('Ctrl Pts',(-0.60568367304395,15.2,11.2819993991877));
#228200=CARTESIAN_POINT('Ctrl Pts',(-0.608364877499989,15.2,11.2872797161888));
#228201=CARTESIAN_POINT('Ctrl Pts',(-0.611065215208339,15.2,11.2925721364666));
#228202=CARTESIAN_POINT('Ctrl Pts',(-0.612685417774481,15.2,11.2957475885179));
#228203=CARTESIAN_POINT('Ctrl Pts',(-0.614312507332004,15.2,11.2989273971024));
#228204=CARTESIAN_POINT('Ctrl Pts',(-0.615946494313679,15.2,11.3021115211113));
#228205=CARTESIAN_POINT('Ctrl Pts',(-0.617580481295354,15.2,11.3052956451202));
#228206=CARTESIAN_POINT('Ctrl Pts',(-0.619221363601611,15.2,11.3084840835705));
#228207=CARTESIAN_POINT('Ctrl Pts',(-0.620869151624126,15.2,11.3116767940789));
#228208=CARTESIAN_POINT('Ctrl Pts',(-0.622516939945989,15.2,11.3148695051673));
#228209=CARTESIAN_POINT('Ctrl Pts',(-0.62417163293648,15.2,11.318066487332));
#228210=CARTESIAN_POINT('Ctrl Pts',(-0.625833238387245,15.2,11.3212676994645));
#228211=CARTESIAN_POINT('Ctrl Pts',(-0.628048711818499,15.2,11.3255359813386));
#228212=CARTESIAN_POINT('Ctrl Pts',(-0.63027647683816,15.2,11.3298117829972));
#228213=CARTESIAN_POINT('Ctrl Pts',(-0.632516548998486,15.2,11.3340950030554));
#228214=CARTESIAN_POINT('Ctrl Pts',(-0.634196603195032,15.2,11.3373074182449));
#228215=CARTESIAN_POINT('Ctrl Pts',(-0.635883582144314,15.2,11.3405240072497));
#228216=CARTESIAN_POINT('Ctrl Pts',(-0.637577492290494,15.2,11.343744726924));
#228217=CARTESIAN_POINT('Ctrl Pts',(-0.639271402436673,15.2,11.3469654465983));
#228218=CARTESIAN_POINT('Ctrl Pts',(-0.640972244990714,15.2,11.3501902979473));
#228219=CARTESIAN_POINT('Ctrl Pts',(-0.642680026136049,15.2,11.3534192385794));
#228220=CARTESIAN_POINT('Ctrl Pts',(-0.64438780759163,15.2,11.3566481797981));
#228221=CARTESIAN_POINT('Ctrl Pts',(-0.646102529490854,15.2,11.359881210268));
#228222=CARTESIAN_POINT('Ctrl Pts',(-0.647824197908676,15.2,11.3631182894473));
#228223=CARTESIAN_POINT('Ctrl Pts',(-0.650119755277823,15.2,11.3674343940396));
#228224=CARTESIAN_POINT('Ctrl Pts',(-0.652427663408144,15.2,11.3717576959785));
#228225=CARTESIAN_POINT('Ctrl Pts',(-0.654747939506772,15.2,11.3760880952554));
#228226=CARTESIAN_POINT('Ctrl Pts',(-0.657068215921539,15.2,11.3804184951222));
#228227=CARTESIAN_POINT('Ctrl Pts',(-0.659400862054365,15.2,11.384755992845));
#228228=CARTESIAN_POINT('Ctrl Pts',(-0.6617458918501,15.2,11.3891004921936));
#228229=CARTESIAN_POINT('Ctrl Pts',(-0.663504664037145,15.2,11.3923588664091));
#228230=CARTESIAN_POINT('Ctrl Pts',(-0.665270405040484,15.2,11.3956211789077));
#228231=CARTESIAN_POINT('Ctrl Pts',(-0.667043118226683,15.2,11.3988873895394));
#228232=CARTESIAN_POINT('Ctrl Pts',(-0.669406735700934,15.2,11.4032423368505));
#228233=CARTESIAN_POINT('Ctrl Pts',(-0.671782751502728,15.2,11.4076042159778));
#228234=CARTESIAN_POINT('Ctrl Pts',(-0.674171182870168,15.2,11.4119729236161));
#228235=CARTESIAN_POINT('Ctrl Pts',(-0.675962506477103,15.2,11.4152494544936));
#228236=CARTESIAN_POINT('Ctrl Pts',(-0.677760814073012,15.2,11.4185298273539));
#228237=CARTESIAN_POINT('Ctrl Pts',(-0.679566111173121,15.2,11.4218140020257));
#228238=CARTESIAN_POINT('Ctrl Pts',(-0.681371408601192,15.2,11.4250981772941));
#228239=CARTESIAN_POINT('Ctrl Pts',(-0.683183696681263,15.2,11.4283861539887));
#228240=CARTESIAN_POINT('Ctrl Pts',(-0.685002980613288,15.2,11.4316778976759));
#228241=CARTESIAN_POINT('Ctrl Pts',(-0.687428691971815,15.2,11.4360668882622));
#228242=CARTESIAN_POINT('Ctrl Pts',(-0.689866841517626,15.2,11.4404625755866));
#228243=CARTESIAN_POINT('Ctrl Pts',(-0.692317444316457,15.2,11.4448648566151));
#228244=CARTESIAN_POINT('Ctrl Pts',(-0.694155396499053,15.2,11.4481665675365));
#228245=CARTESIAN_POINT('Ctrl Pts',(-0.696000355984013,15.2,11.4514719838984));
#228246=CARTESIAN_POINT('Ctrl Pts',(-0.697852328175099,15.2,11.4547810616098));
#228247=CARTESIAN_POINT('Ctrl Pts',(-0.699704300366184,15.2,11.4580901393211));
#228248=CARTESIAN_POINT('Ctrl Pts',(-0.701563285928658,15.2,11.461402874898));
#228249=CARTESIAN_POINT('Ctrl Pts',(-0.703429290318224,15.2,11.464719242027));
#228250=CARTESIAN_POINT('Ctrl Pts',(-0.705917296396971,15.2,11.4691410652673));
#228251=CARTESIAN_POINT('Ctrl Pts',(-0.708417774315274,15.2,11.4735693451248));
#228252=CARTESIAN_POINT('Ctrl Pts',(-0.710930735000056,15.2,11.478004073));
#228253=CARTESIAN_POINT('Ctrl Pts',(-0.292001930000056,12.2,10.370890024));
#228254=CARTESIAN_POINT('Ctrl Pts',(-0.29220549901488,12.2,10.372665048257));
#228255=CARTESIAN_POINT('Ctrl Pts',(-0.292420934152544,12.2,10.3744962450942));
#228256=CARTESIAN_POINT('Ctrl Pts',(-0.29264874396675,12.2,10.3763825865516));
#228257=CARTESIAN_POINT('Ctrl Pts',(-0.292877652395031,12.2,10.378278024901));
#228258=CARTESIAN_POINT('Ctrl Pts',(-0.293119060472346,12.2,10.3802291369147));
#228259=CARTESIAN_POINT('Ctrl Pts',(-0.293373491749677,12.2,10.3822349054607));
#228260=CARTESIAN_POINT('Ctrl Pts',(-0.293627923003897,12.2,10.3842406738245));
#228261=CARTESIAN_POINT('Ctrl Pts',(-0.29389537585191,12.2,10.3863010957184));
#228262=CARTESIAN_POINT('Ctrl Pts',(-0.294176351258366,12.2,10.3884151802249));
#228263=CARTESIAN_POINT('Ctrl Pts',(-0.294457326664821,12.2,10.3905292647314));
#228264=CARTESIAN_POINT('Ctrl Pts',(-0.294751826391833,12.2,10.3926970122247));
#228265=CARTESIAN_POINT('Ctrl Pts',(-0.295060336478553,12.2,10.3949174557519));
#228266=CARTESIAN_POINT('Ctrl Pts',(-0.295368846593297,12.2,10.3971378994807));
#228267=CARTESIAN_POINT('Ctrl Pts',(-0.295691365100748,12.2,10.3994110391898));
#228268=CARTESIAN_POINT('Ctrl Pts',(-0.296028362286767,12.2,10.4017359359867));
#228269=CARTESIAN_POINT('Ctrl Pts',(-0.29642152562454,12.2,10.4044483152663));
#228270=CARTESIAN_POINT('Ctrl Pts',(-0.296834399281608,12.2,10.407231138541));
#228271=CARTESIAN_POINT('Ctrl Pts',(-0.297267698205805,12.2,10.4100829567802));
#228272=CARTESIAN_POINT('Ctrl Pts',(-0.297639097327062,12.2,10.4125273726993));
#228273=CARTESIAN_POINT('Ctrl Pts',(-0.298025503737548,12.2,10.4150224780102));
#228274=CARTESIAN_POINT('Ctrl Pts',(-0.298427354760501,12.2,10.417567385069));
#228275=CARTESIAN_POINT('Ctrl Pts',(-0.298829205746953,12.2,10.4201122918966));
#228276=CARTESIAN_POINT('Ctrl Pts',(-0.2992465001973,12.2,10.4227069991351));
#228277=CARTESIAN_POINT('Ctrl Pts',(-0.299679662016898,12.2,10.4253506402178));
#228278=CARTESIAN_POINT('Ctrl Pts',(-0.300112823836495,12.2,10.4279942813005));
#228279=CARTESIAN_POINT('Ctrl Pts',(-0.300561853225689,12.2,10.4306868582274));
#228280=CARTESIAN_POINT('Ctrl Pts',(-0.301027158208068,12.2,10.4334275203757));
#228281=CARTESIAN_POINT('Ctrl Pts',(-0.301492463232712,12.2,10.4361681827729));
#228282=CARTESIAN_POINT('Ctrl Pts',(-0.301974044942714,12.2,10.4389569340179));
#228283=CARTESIAN_POINT('Ctrl Pts',(-0.30247229980434,12.2,10.4417929463424));
#228284=CARTESIAN_POINT('Ctrl Pts',(-0.303053597075016,12.2,10.4451016270012));
#228285=CARTESIAN_POINT('Ctrl Pts',(-0.303657588305184,12.2,10.4484746348393));
#228286=CARTESIAN_POINT('Ctrl Pts',(-0.304284883445796,12.2,10.4519106910813));
#228287=CARTESIAN_POINT('Ctrl Pts',(-0.304822565057686,12.2,10.4548558824898));
#228288=CARTESIAN_POINT('Ctrl Pts',(-0.305377366496697,12.2,10.4578473947873));
#228289=CARTESIAN_POINT('Ctrl Pts',(-0.305949657362403,12.2,10.4608844433726));
#228290=CARTESIAN_POINT('Ctrl Pts',(-0.306521948176124,12.2,10.463921491682));
#228291=CARTESIAN_POINT('Ctrl Pts',(-0.307111731829524,12.2,10.4670040761239));
#228292=CARTESIAN_POINT('Ctrl Pts',(-0.307719363558214,12.2,10.4701314274289));
#228293=CARTESIAN_POINT('Ctrl Pts',(-0.308326995286904,12.2,10.4732587787338));
#228294=CARTESIAN_POINT('Ctrl Pts',(-0.308952478339206,12.2,10.4764308968936));
#228295=CARTESIAN_POINT('Ctrl Pts',(-0.30959615798169,12.2,10.4796470312748));
#228296=CARTESIAN_POINT('Ctrl Pts',(-0.310239837682641,12.2,10.4828631659482));
#228297=CARTESIAN_POINT('Ctrl Pts',(-0.310901714877504,12.2,10.4861233166853));
#228298=CARTESIAN_POINT('Ctrl Pts',(-0.311582129332527,12.2,10.4894267466183));
#228299=CARTESIAN_POINT('Ctrl Pts',(-0.312262543725746,12.2,10.4927301762513));
#228300=CARTESIAN_POINT('Ctrl Pts',(-0.312961492072808,12.2,10.4960768859977));
#228301=CARTESIAN_POINT('Ctrl Pts',(-0.313679305464225,12.2,10.4994661554598));
#228302=CARTESIAN_POINT('Ctrl Pts',(-0.314397118855642,12.2,10.5028554249219));
#228303=CARTESIAN_POINT('Ctrl Pts',(-0.315133794903881,12.2,10.5062872556305));
#228304=CARTESIAN_POINT('Ctrl Pts',(-0.315889653208907,12.2,10.5097609375858));
#228305=CARTESIAN_POINT('Ctrl Pts',(-0.316645511513932,12.2,10.513234619541));
#228306=CARTESIAN_POINT('Ctrl Pts',(-0.317420551443608,12.2,10.5167501571609));
#228307=CARTESIAN_POINT('Ctrl Pts',(-0.318215080913418,12.2,10.5203068568622));
#228308=CARTESIAN_POINT('Ctrl Pts',(-0.319009610455398,12.2,10.5238635568866));
#228309=CARTESIAN_POINT('Ctrl Pts',(-0.319823630924239,12.2,10.5274614183316));
#228310=CARTESIAN_POINT('Ctrl Pts',(-0.320657440553881,12.2,10.5310997671984));
#228311=CARTESIAN_POINT('Ctrl Pts',(-0.321491250107784,12.2,10.5347381157346));
#228312=CARTESIAN_POINT('Ctrl Pts',(-0.322344850352457,12.2,10.5384169472249));
#228313=CARTESIAN_POINT('Ctrl Pts',(-0.323218530741291,12.2,10.5421356000232));
#228314=CARTESIAN_POINT('Ctrl Pts',(-0.324092211130125,12.2,10.5458542528215));
#228315=CARTESIAN_POINT('Ctrl Pts',(-0.324985972868309,12.2,10.549612724485));
#228316=CARTESIAN_POINT('Ctrl Pts',(-0.325900097167055,12.2,10.553410366261));
#228317=CARTESIAN_POINT('Ctrl Pts',(-0.326814221548832,12.2,10.557208008382));
#228318=CARTESIAN_POINT('Ctrl Pts',(-0.327748709641513,12.2,10.5610448175429));
#228319=CARTESIAN_POINT('Ctrl Pts',(-0.3287038350758,12.2,10.5649201568666));
#228320=CARTESIAN_POINT('Ctrl Pts',(-0.329499772894327,12.2,10.568149606127));
#228321=CARTESIAN_POINT('Ctrl Pts',(-0.330310042073378,12.2,10.5714058104271));
#228322=CARTESIAN_POINT('Ctrl Pts',(-0.331134798116238,12.2,10.5746884079293));
#228323=CARTESIAN_POINT('Ctrl Pts',(-0.331959554159098,12.2,10.5779710054315));
#228324=CARTESIAN_POINT('Ctrl Pts',(-0.332798795749401,12.2,10.5812799938229));
#228325=CARTESIAN_POINT('Ctrl Pts',(-0.333652674361709,12.2,10.5846150172278));
#228326=CARTESIAN_POINT('Ctrl Pts',(-0.334506552880944,12.2,10.5879500402692));
#228327=CARTESIAN_POINT('Ctrl Pts',(-0.335375070626421,12.2,10.5913110967615));
#228328=CARTESIAN_POINT('Ctrl Pts',(-0.336258370667824,12.2,10.5946978340986));
#228329=CARTESIAN_POINT('Ctrl Pts',(-0.33731833089081,12.2,10.5987619195676));
#228330=CARTESIAN_POINT('Ctrl Pts',(-0.338399582482504,12.2,10.6028629845068));
#228331=CARTESIAN_POINT('Ctrl Pts',(-0.339502371543545,12.2,10.6070004289839));
#228332=CARTESIAN_POINT('Ctrl Pts',(-0.34042136237766,12.2,10.6104482991936));
#228333=CARTESIAN_POINT('Ctrl Pts',(-0.34135530832287,12.2,10.6139214322795));
#228334=CARTESIAN_POINT('Ctrl Pts',(-0.342304353301911,12.2,10.6174194876644));
#228335=CARTESIAN_POINT('Ctrl Pts',(-0.343253398280953,12.2,10.6209175430493));
#228336=CARTESIAN_POINT('Ctrl Pts',(-0.344217538393549,12.2,10.6244405197508));
#228337=CARTESIAN_POINT('Ctrl Pts',(-0.345196912561453,12.2,10.6279880816973));
#228338=CARTESIAN_POINT('Ctrl Pts',(-0.346176286729357,12.2,10.6315356436437));
#228339=CARTESIAN_POINT('Ctrl Pts',(-0.347170893953096,12.2,10.6351077891795));
#228340=CARTESIAN_POINT('Ctrl Pts',(-0.348180867357127,12.2,10.638704188487));
#228341=CARTESIAN_POINT('Ctrl Pts',(-0.349190840651072,12.2,10.6423005874025));
#228342=CARTESIAN_POINT('Ctrl Pts',(-0.350216180523041,12.2,10.6459212354502));
#228343=CARTESIAN_POINT('Ctrl Pts',(-0.351257017838883,12.2,10.6495658110232));
#228344=CARTESIAN_POINT('Ctrl Pts',(-0.352297855268177,12.2,10.6532103869935));
#228345=CARTESIAN_POINT('Ctrl Pts',(-0.353354189705533,12.2,10.6568788857078));
#228346=CARTESIAN_POINT('Ctrl Pts',(-0.354426147343142,12.2,10.660570986192));
#228347=CARTESIAN_POINT('Ctrl Pts',(-0.355712496578379,12.2,10.6650015070145));
#228348=CARTESIAN_POINT('Ctrl Pts',(-0.357021345021807,12.2,10.6694660135717));
#228349=CARTESIAN_POINT('Ctrl Pts',(-0.358352906162216,12.2,10.6739639554601));
#228350=CARTESIAN_POINT('Ctrl Pts',(-0.359462540385416,12.2,10.6777122401629));
#228351=CARTESIAN_POINT('Ctrl Pts',(-0.360587946892449,12.2,10.681483743061));
#228352=CARTESIAN_POINT('Ctrl Pts',(-0.361729247657633,12.2,10.6852781509796));
#228353=CARTESIAN_POINT('Ctrl Pts',(-0.362870548422817,12.2,10.6890725588981));
#228354=CARTESIAN_POINT('Ctrl Pts',(-0.364027741913281,12.2,10.6928898715004));
#228355=CARTESIAN_POINT('Ctrl Pts',(-0.365200947678475,12.2,10.6967297802522));
#228356=CARTESIAN_POINT('Ctrl Pts',(-0.36637415344367,12.2,10.700569689004));
#228357=CARTESIAN_POINT('Ctrl Pts',(-0.36756336964523,12.2,10.7044321930117));
#228358=CARTESIAN_POINT('Ctrl Pts',(-0.368768713674349,12.2,10.7083169859997));
#228359=CARTESIAN_POINT('Ctrl Pts',(-0.369974057572086,12.2,10.7122017785643));
#228360=CARTESIAN_POINT('Ctrl Pts',(-0.371195528302116,12.2,10.7161088606771));
#228361=CARTESIAN_POINT('Ctrl Pts',(-0.372433238096463,12.2,10.7200379299694));
#228362=CARTESIAN_POINT('Ctrl Pts',(-0.37367094802572,12.2,10.7239669996899));
#228363=CARTESIAN_POINT('Ctrl Pts',(-0.374924897418553,12.2,10.7279180584377));
#228364=CARTESIAN_POINT('Ctrl Pts',(-0.376195196375531,12.2,10.7318908049636));
#228365=CARTESIAN_POINT('Ctrl Pts',(-0.377211435596498,12.2,10.7350690023576));
#228366=CARTESIAN_POINT('Ctrl Pts',(-0.37823813745333,12.2,10.7382610825544));
#228367=CARTESIAN_POINT('Ctrl Pts',(-0.379275358792392,12.2,10.7414668912438));
#228368=CARTESIAN_POINT('Ctrl Pts',(-0.380312579990132,12.2,10.7446726994963));
#228369=CARTESIAN_POINT('Ctrl Pts',(-0.381360319825717,12.2,10.7478922394315));
#228370=CARTESIAN_POINT('Ctrl Pts',(-0.382418632293654,12.2,10.7511253597213));
#228371=CARTESIAN_POINT('Ctrl Pts',(-0.383476944905785,12.2,10.7543584804516));
#228372=CARTESIAN_POINT('Ctrl Pts',(-0.384545831121746,12.2,10.7576051824751));
#228373=CARTESIAN_POINT('Ctrl Pts',(-0.385625342458339,12.2,10.7608653170416));
#228374=CARTESIAN_POINT('Ctrl Pts',(-0.386704853794931,12.2,10.7641254516081));
#228375=CARTESIAN_POINT('Ctrl Pts',(-0.387794991685585,12.2,10.7673990188624));
#228376=CARTESIAN_POINT('Ctrl Pts',(-0.388895806413339,12.2,10.7706858728207));
#228377=CARTESIAN_POINT('Ctrl Pts',(-0.389996620991107,12.2,10.7739727263311));
#228378=CARTESIAN_POINT('Ctrl Pts',(-0.391108115344244,12.2,10.7772728660313));
#228379=CARTESIAN_POINT('Ctrl Pts',(-0.392230337757589,12.2,10.7805861469977));
#228380=CARTESIAN_POINT('Ctrl Pts',(-0.393352560323837,12.2,10.7838994284156));
#228381=CARTESIAN_POINT('Ctrl Pts',(-0.394485511079143,12.2,10.7872258510848));
#228382=CARTESIAN_POINT('Ctrl Pts',(-0.395629242920353,12.2,10.7905652710459));
#228383=CARTESIAN_POINT('Ctrl Pts',(-0.396772974605729,12.2,10.793904690552));
#228384=CARTESIAN_POINT('Ctrl Pts',(-0.39792748563137,12.2,10.7972571073398));
#228385=CARTESIAN_POINT('Ctrl Pts',(-0.399092824146519,12.2,10.8006223795083));
#228386=CARTESIAN_POINT('Ctrl Pts',(-0.400258162820446,12.2,10.8039876521353));
#228387=CARTESIAN_POINT('Ctrl Pts',(-0.401434331622365,12.2,10.8073657787339));
#228388=CARTESIAN_POINT('Ctrl Pts',(-0.402621376913991,12.2,10.8107566197004));
#228389=CARTESIAN_POINT('Ctrl Pts',(-0.403808422043882,12.2,10.8141474602048));
#228390=CARTESIAN_POINT('Ctrl Pts',(-0.4050063439064,12.2,10.8175510144232));
#228391=CARTESIAN_POINT('Ctrl Pts',(-0.406215190917957,12.2,10.8209671432541));
#228392=CARTESIAN_POINT('Ctrl Pts',(-0.40742403809422,12.2,10.8243832725505));
#228393=CARTESIAN_POINT('Ctrl Pts',(-0.408643808321823,12.2,10.8278119736319));
#228394=CARTESIAN_POINT('Ctrl Pts',(-0.409874550834068,12.2,10.8312531122647));
#228395=CARTESIAN_POINT('Ctrl Pts',(-0.411105293178624,12.2,10.8346942504287));
#228396=CARTESIAN_POINT('Ctrl Pts',(-0.412347006228511,12.2,10.8381478235389));
#228397=CARTESIAN_POINT('Ctrl Pts',(-0.413599736576627,12.2,10.8416136947054));
#228398=CARTESIAN_POINT('Ctrl Pts',(-0.414852467095428,12.2,10.8450795663442));
#228399=CARTESIAN_POINT('Ctrl Pts',(-0.416116213753581,12.2,10.8485577360111));
#228400=CARTESIAN_POINT('Ctrl Pts',(-0.417391022879335,12.2,10.8520480675354));
#228401=CARTESIAN_POINT('Ctrl Pts',(-0.418665831831396,12.2,10.8555383985842));
#228402=CARTESIAN_POINT('Ctrl Pts',(-0.419951701303461,12.2,10.8590408918916));
#228403=CARTESIAN_POINT('Ctrl Pts',(-0.421248677029627,12.2,10.8625554121587));
#228404=CARTESIAN_POINT('Ctrl Pts',(-0.422545652932505,12.2,10.8660699329045));
#228405=CARTESIAN_POINT('Ctrl Pts',(-0.423853735161873,12.2,10.8695964805712));
#228406=CARTESIAN_POINT('Ctrl Pts',(-0.425172965684246,12.2,10.8731349220024));
#228407=CARTESIAN_POINT('Ctrl Pts',(-0.426492196026873,12.2,10.8766733629514));
#228408=CARTESIAN_POINT('Ctrl Pts',(-0.42782257640538,12.2,10.8802236975433));
#228409=CARTESIAN_POINT('Ctrl Pts',(-0.429164146239003,12.2,10.8837857919175));
#228410=CARTESIAN_POINT('Ctrl Pts',(-0.430505716255415,12.2,10.8873478867771));
#228411=CARTESIAN_POINT('Ctrl Pts',(-0.431858479650664,12.2,10.8909217432767));
#228412=CARTESIAN_POINT('Ctrl Pts',(-0.433222474225011,12.2,10.8945072282499));
#228413=CARTESIAN_POINT('Ctrl Pts',(-0.434586468799358,12.2,10.8980927132232));
#228414=CARTESIAN_POINT('Ctrl Pts',(-0.435961696255549,12.2,10.9016898279004));
#228415=CARTESIAN_POINT('Ctrl Pts',(-0.437348197443381,12.2,10.9052984425983));
#228416=CARTESIAN_POINT('Ctrl Pts',(-0.439081323644806,12.2,10.9098092102331));
#228417=CARTESIAN_POINT('Ctrl Pts',(-0.440832065601813,12.2,10.9143379434412));
#228418=CARTESIAN_POINT('Ctrl Pts',(-0.442600500060369,12.2,10.9188843921803));
#228419=CARTESIAN_POINT('Ctrl Pts',(-0.444015247858525,12.2,10.9225215517662));
#228420=CARTESIAN_POINT('Ctrl Pts',(-0.445441320160564,12.2,10.9261700500227));
#228421=CARTESIAN_POINT('Ctrl Pts',(-0.446878754016672,12.2,10.9298297569999));
#228422=CARTESIAN_POINT('Ctrl Pts',(-0.448316187872781,12.2,10.9334894639771));
#228423=CARTESIAN_POINT('Ctrl Pts',(-0.449764984749679,12.2,10.9371603810779));
#228424=CARTESIAN_POINT('Ctrl Pts',(-0.451225181997092,12.2,10.9408423818353));
#228425=CARTESIAN_POINT('Ctrl Pts',(-0.452685379045552,12.2,10.944524382091));
#228426=CARTESIAN_POINT('Ctrl Pts',(-0.454156977041318,12.2,10.9482174661418));
#228427=CARTESIAN_POINT('Ctrl Pts',(-0.455640014482341,12.2,10.9519215060224));
#228428=CARTESIAN_POINT('Ctrl Pts',(-0.457123052125427,12.2,10.9556255464078));
#228429=CARTESIAN_POINT('Ctrl Pts',(-0.45861752763244,12.2,10.9593405450272));
#228430=CARTESIAN_POINT('Ctrl Pts',(-0.460123478771237,12.2,10.9630663753424));
#228431=CARTESIAN_POINT('Ctrl Pts',(-0.461629429704847,12.2,10.9667922051501));
#228432=CARTESIAN_POINT('Ctrl Pts',(-0.463146854964757,12.2,10.9705288680007));
#228433=CARTESIAN_POINT('Ctrl Pts',(-0.464675793116795,12.2,10.9742762396937));
#228434=CARTESIAN_POINT('Ctrl Pts',(-0.466586965963081,12.2,10.9789604546928));
#228435=CARTESIAN_POINT('Ctrl Pts',(-0.468516124940402,12.2,10.9836614020813));
#228436=CARTESIAN_POINT('Ctrl Pts',(-0.470463340356108,12.2,10.9883788429832));
#228437=CARTESIAN_POINT('Ctrl Pts',(-0.472021112773571,12.2,10.9921527959104));
#228438=CARTESIAN_POINT('Ctrl Pts',(-0.473590441352209,12.2,10.9959373043395));
#228439=CARTESIAN_POINT('Ctrl Pts',(-0.475171359962806,12.2,10.9997322467923));
#228440=CARTESIAN_POINT('Ctrl Pts',(-0.476752278358003,12.2,11.0035271887281));
#228441=CARTESIAN_POINT('Ctrl Pts',(-0.478344787703661,12.2,11.0073325632174));
#228442=CARTESIAN_POINT('Ctrl Pts',(-0.479948920627313,12.2,11.0111482529048));
#228443=CARTESIAN_POINT('Ctrl Pts',(-0.481954086945801,12.2,11.0159178654039));
#228444=CARTESIAN_POINT('Ctrl Pts',(-0.483977417173082,12.2,11.0207035918257));
#228445=CARTESIAN_POINT('Ctrl Pts',(-0.486018975158267,12.2,11.0255052002277));
#228446=CARTESIAN_POINT('Ctrl Pts',(-0.487652221635427,12.2,11.0293464871587));
#228447=CARTESIAN_POINT('Ctrl Pts',(-0.489297132710859,12.2,11.0331979375784));
#228448=CARTESIAN_POINT('Ctrl Pts',(-0.490953743773791,12.2,11.0370594340937));
#228449=CARTESIAN_POINT('Ctrl Pts',(-0.49261035461101,12.2,11.0409209300828));
#228450=CARTESIAN_POINT('Ctrl Pts',(-0.494278662031432,12.2,11.0447924710896));
#228451=CARTESIAN_POINT('Ctrl Pts',(-0.495958700837779,12.2,11.0486739402161));
#228452=CARTESIAN_POINT('Ctrl Pts',(-0.497638739873032,12.2,11.0525554098714));
#228453=CARTESIAN_POINT('Ctrl Pts',(-0.499330509445771,12.2,11.0564468067085));
#228454=CARTESIAN_POINT('Ctrl Pts',(-0.501034039872722,12.2,11.0603480163106));
#228455=CARTESIAN_POINT('Ctrl Pts',(-0.502737570067566,12.2,11.0642492253813));
#228456=CARTESIAN_POINT('Ctrl Pts',(-0.504452861691518,12.2,11.0681602448955));
#228457=CARTESIAN_POINT('Ctrl Pts',(-0.50617994469113,12.2,11.0720809602144));
#228458=CARTESIAN_POINT('Ctrl Pts',(-0.50833879861713,12.2,11.0769818547637));
#228459=CARTESIAN_POINT('Ctrl Pts',(-0.510516078696392,12.2,11.0818978977839));
#228460=CARTESIAN_POINT('Ctrl Pts',(-0.512711840848184,12.2,11.0868288661859));
#228461=CARTESIAN_POINT('Ctrl Pts',(-0.514468450665353,12.2,11.0907736411224));
#228462=CARTESIAN_POINT('Ctrl Pts',(-0.51623688907285,12.2,11.0947279680324));
#228463=CARTESIAN_POINT('Ctrl Pts',(-0.518017187337333,12.2,11.0986917330824));
#228464=CARTESIAN_POINT('Ctrl Pts',(-0.519797485359249,12.2,11.1026554975924));
#228465=CARTESIAN_POINT('Ctrl Pts',(-0.521589640343912,12.2,11.1066286997412));
#228466=CARTESIAN_POINT('Ctrl Pts',(-0.523393683229959,12.2,11.1106112264471));
#228467=CARTESIAN_POINT('Ctrl Pts',(-0.525197726361805,12.2,11.1145937536956));
#228468=CARTESIAN_POINT('Ctrl Pts',(-0.527013656329686,12.2,11.1185856069529));
#228469=CARTESIAN_POINT('Ctrl Pts',(-0.528841501374546,12.2,11.1225866720605));
#228470=CARTESIAN_POINT('Ctrl Pts',(-0.5311263075561,12.2,11.1275880031724));
#228471=CARTESIAN_POINT('Ctrl Pts',(-0.533429730945455,12.2,11.1326037289227));
#228472=CARTESIAN_POINT('Ctrl Pts',(-0.535751824626986,12.2,11.1376336323957));
#228473=CARTESIAN_POINT('Ctrl Pts',(-0.537609499420346,12.2,11.1416575548451));
#228474=CARTESIAN_POINT('Ctrl Pts',(-0.539479124035124,12.2,11.1456905501205));
#228475=CARTESIAN_POINT('Ctrl Pts',(-0.541360724252043,12.2,11.1497325088802));
#228476=CARTESIAN_POINT('Ctrl Pts',(-0.542771924478824,12.2,11.1527639780875));
#228477=CARTESIAN_POINT('Ctrl Pts',(-0.544189861392124,12.2,11.1558004885981));
#228478=CARTESIAN_POINT('Ctrl Pts',(-0.545614545964432,12.2,11.1588419950702));
#228479=CARTESIAN_POINT('Ctrl Pts',(-0.547039230795557,12.2,11.1618835020949));
#228480=CARTESIAN_POINT('Ctrl Pts',(-0.54847066198694,12.2,11.1649300046044));
#228481=CARTESIAN_POINT('Ctrl Pts',(-0.549908852363539,12.2,11.1679814562152));
#228482=CARTESIAN_POINT('Ctrl Pts',(-0.551347042478867,12.2,11.1710329072716));
#228483=CARTESIAN_POINT('Ctrl Pts',(-0.552791990943856,12.2,11.1740893077445));
#228484=CARTESIAN_POINT('Ctrl Pts',(-0.554243708183353,12.2,11.1771506118004));
#228485=CARTESIAN_POINT('Ctrl Pts',(-0.55569542542285,12.2,11.1802119158562));
#228486=CARTESIAN_POINT('Ctrl Pts',(-0.557153913097895,12.2,11.183278123767));
#228487=CARTESIAN_POINT('Ctrl Pts',(-0.558619179759674,12.2,11.1863491892944));
#228488=CARTESIAN_POINT('Ctrl Pts',(-0.560084446421453,12.2,11.1894202548218));
#228489=CARTESIAN_POINT('Ctrl Pts',(-0.561556491845709,12.2,11.1924961777451));
#228490=CARTESIAN_POINT('Ctrl Pts',(-0.56303532796533,12.2,11.1955769142305));
#228491=CARTESIAN_POINT('Ctrl Pts',(-0.564514164084952,12.2,11.1986576507159));
#228492=CARTESIAN_POINT('Ctrl Pts',(-0.565999790142274,12.2,11.2017431996759));
#228493=CARTESIAN_POINT('Ctrl Pts',(-0.567492216337446,12.2,11.2048335157299));
#228494=CARTESIAN_POINT('Ctrl Pts',(-0.568984642532617,12.2,11.2079238317838));
#228495=CARTESIAN_POINT('Ctrl Pts',(-0.570483869960694,12.2,11.2110189150042));
#228496=CARTESIAN_POINT('Ctrl Pts',(-0.571989907113364,12.2,11.2141187215575));
#228497=CARTESIAN_POINT('Ctrl Pts',(-0.573495944539631,12.2,11.217218528674));
#228498=CARTESIAN_POINT('Ctrl Pts',(-0.575008792426188,12.2,11.2203230582253));
#228499=CARTESIAN_POINT('Ctrl Pts',(-0.576528459856301,12.2,11.2234322654278));
#228500=CARTESIAN_POINT('Ctrl Pts',(-0.57804812701034,12.2,11.2265414720654));
#228501=CARTESIAN_POINT('Ctrl Pts',(-0.579574615375054,12.2,11.2296553577437));
#228502=CARTESIAN_POINT('Ctrl Pts',(-0.581107933105065,12.2,11.2327738760784));
#228503=CARTESIAN_POINT('Ctrl Pts',(-0.583152356652229,12.2,11.2369319003357));
#228504=CARTESIAN_POINT('Ctrl Pts',(-0.585208922045364,12.2,11.2410981626117));
#228505=CARTESIAN_POINT('Ctrl Pts',(-0.58727765209767,12.2,11.2452725571588));
#228506=CARTESIAN_POINT('Ctrl Pts',(-0.588829199707366,12.2,11.2484033532113));
#228507=CARTESIAN_POINT('Ctrl Pts',(-0.590387590066615,12.2,11.2515387239635));
#228508=CARTESIAN_POINT('Ctrl Pts',(-0.591952832217119,12.2,11.2546786255571));
#228509=CARTESIAN_POINT('Ctrl Pts',(-0.593518074651977,12.2,11.2578185277211));
#228510=CARTESIAN_POINT('Ctrl Pts',(-0.59509016888047,12.2,11.2609629607615));
#228511=CARTESIAN_POINT('Ctrl Pts',(-0.596669124277563,12.2,11.2641118808864));
#228512=CARTESIAN_POINT('Ctrl Pts',(-0.598248079387812,12.2,11.2672608004393));
#228513=CARTESIAN_POINT('Ctrl Pts',(-0.599833895219053,12.2,11.2704142069174));
#228514=CARTESIAN_POINT('Ctrl Pts',(-0.601426582324892,12.2,11.2735720571276));
#228515=CARTESIAN_POINT('Ctrl Pts',(-0.603019269430731,12.2,11.2767299073379));
#228516=CARTESIAN_POINT('Ctrl Pts',(-0.60461882624966,12.2,11.2798922010599));
#228517=CARTESIAN_POINT('Ctrl Pts',(-0.606225261900224,12.2,11.2830588956119));
#228518=CARTESIAN_POINT('Ctrl Pts',(-0.607831697550787,12.2,11.2862255901638));
#228519=CARTESIAN_POINT('Ctrl Pts',(-0.609445012642199,12.2,11.2893966844153));
#228520=CARTESIAN_POINT('Ctrl Pts',(-0.611065215208341,12.2,11.2925721364666));
#228521=CARTESIAN_POINT('Ctrl Pts',(-0.612685417774483,12.2,11.2957475885179));
#228522=CARTESIAN_POINT('Ctrl Pts',(-0.614312507332006,12.2,11.2989273971024));
#228523=CARTESIAN_POINT('Ctrl Pts',(-0.615946494313681,12.2,11.3021115211113));
#228524=CARTESIAN_POINT('Ctrl Pts',(-0.617580481295356,12.2,11.3052956451202));
#228525=CARTESIAN_POINT('Ctrl Pts',(-0.619221363601612,12.2,11.3084840835705));
#228526=CARTESIAN_POINT('Ctrl Pts',(-0.620869151624128,12.2,11.3116767940789));
#228527=CARTESIAN_POINT('Ctrl Pts',(-0.622516939945991,12.2,11.3148695051673));
#228528=CARTESIAN_POINT('Ctrl Pts',(-0.624171632936478,12.2,11.318066487332));
#228529=CARTESIAN_POINT('Ctrl Pts',(-0.625833238387243,12.2,11.3212676994645));
#228530=CARTESIAN_POINT('Ctrl Pts',(-0.627494843536147,12.2,11.3244689110154));
#228531=CARTESIAN_POINT('Ctrl Pts',(-0.629163362900605,12.2,11.3276743514768));
#228532=CARTESIAN_POINT('Ctrl Pts',(-0.630838802590896,12.2,11.3308839806043));
#228533=CARTESIAN_POINT('Ctrl Pts',(-0.633072722076496,12.2,11.3351634859133));
#228534=CARTESIAN_POINT('Ctrl Pts',(-0.635318945531495,12.2,11.33945043422));
#228535=CARTESIAN_POINT('Ctrl Pts',(-0.637577492290492,12.2,11.343744726924));
#228536=CARTESIAN_POINT('Ctrl Pts',(-0.639271402436672,12.2,11.3469654465983));
#228537=CARTESIAN_POINT('Ctrl Pts',(-0.640972244990713,12.2,11.3501902979473));
#228538=CARTESIAN_POINT('Ctrl Pts',(-0.642680026136048,12.2,11.3534192385794));
#228539=CARTESIAN_POINT('Ctrl Pts',(-0.644387807591629,12.2,11.3566481797981));
#228540=CARTESIAN_POINT('Ctrl Pts',(-0.646102529490848,12.2,11.359881210268));
#228541=CARTESIAN_POINT('Ctrl Pts',(-0.64782419790867,12.2,11.3631182894473));
#228542=CARTESIAN_POINT('Ctrl Pts',(-0.649545866013722,12.2,11.3663553680386));
#228543=CARTESIAN_POINT('Ctrl Pts',(-0.65127448119475,12.2,11.3695964946665));
#228544=CARTESIAN_POINT('Ctrl Pts',(-0.653010051344197,12.2,11.3728416283778));
#228545=CARTESIAN_POINT('Ctrl Pts',(-0.654745621493644,12.2,11.3760867620892));
#228546=CARTESIAN_POINT('Ctrl Pts',(-0.656488146003774,12.2,11.3793359007058));
#228547=CARTESIAN_POINT('Ctrl Pts',(-0.658237633440817,12.2,11.3825890057963));
#228548=CARTESIAN_POINT('Ctrl Pts',(-0.660570283250933,12.2,11.3869264790533));
#228549=CARTESIAN_POINT('Ctrl Pts',(-0.662915307844703,12.2,11.3912710027505));
#228550=CARTESIAN_POINT('Ctrl Pts',(-0.665272728372901,12.2,11.3956224788385));
#228551=CARTESIAN_POINT('Ctrl Pts',(-0.667630149222297,12.2,11.3999739555193));
#228552=CARTESIAN_POINT('Ctrl Pts',(-0.669999963027594,12.2,11.4043323875368));
#228553=CARTESIAN_POINT('Ctrl Pts',(-0.672382187501631,12.2,11.4086976752946));
#228554=CARTESIAN_POINT('Ctrl Pts',(-0.674168855694871,12.2,11.4119716408156));
#228555=CARTESIAN_POINT('Ctrl Pts',(-0.675962505922318,12.2,11.415249461118));
#228556=CARTESIAN_POINT('Ctrl Pts',(-0.677763143948374,12.2,11.4185310967636));
#228557=CARTESIAN_POINT('Ctrl Pts',(-0.67956378197443,12.2,11.4218127324093));
#228558=CARTESIAN_POINT('Ctrl Pts',(-0.68137140763554,12.2,11.4250981825947));
#228559=CARTESIAN_POINT('Ctrl Pts',(-0.683186028110665,12.2,11.4283874103915));
#228560=CARTESIAN_POINT('Ctrl Pts',(-0.685000648585788,12.2,11.4316766381883));
#228561=CARTESIAN_POINT('Ctrl Pts',(-0.686822262518783,12.2,11.4349696456016));
#228562=CARTESIAN_POINT('Ctrl Pts',(-0.688650877576374,12.2,11.4382663917313));
#228563=CARTESIAN_POINT('Ctrl Pts',(-0.690479492966162,12.2,11.4415631384599));
#228564=CARTESIAN_POINT('Ctrl Pts',(-0.692315108432972,12.2,11.4448636254063));
#228565=CARTESIAN_POINT('Ctrl Pts',(-0.694157732868378,12.2,11.4481678025119));
#228566=CARTESIAN_POINT('Ctrl Pts',(-0.696000356969041,12.2,11.4514719790174));
#228567=CARTESIAN_POINT('Ctrl Pts',(-0.697849990633181,12.2,11.4547798455118));
#228568=CARTESIAN_POINT('Ctrl Pts',(-0.699706638825956,12.2,11.4580913594324));
#228569=CARTESIAN_POINT('Ctrl Pts',(-0.701563287018731,12.2,11.4614028733529));
#228570=CARTESIAN_POINT('Ctrl Pts',(-0.703426952058125,12.2,11.4647180326881));
#228571=CARTESIAN_POINT('Ctrl Pts',(-0.705297634486514,12.2,11.4680368213728));
#228572=CARTESIAN_POINT('Ctrl Pts',(-0.707168316914903,12.2,11.4713556100575));
#228573=CARTESIAN_POINT('Ctrl Pts',(-0.709046014657665,12.2,11.4746780273957));
#228574=CARTESIAN_POINT('Ctrl Pts',(-0.710930735000056,12.2,11.478004073));
#228575=CARTESIAN_POINT('Ctrl Pts',(-1.09337743000006,15.2,11.447904865));
#228576=CARTESIAN_POINT('Ctrl Pts',(-1.09337743000006,11.6,11.447904865));
#228577=CARTESIAN_POINT('Ctrl Pts',(-1.09364567100006,15.2,11.447188879));
#228578=CARTESIAN_POINT('Ctrl Pts',(-1.09364567100006,11.6,11.447188879));
#228579=CARTESIAN_POINT('Ctrl Pts',(-1.09418172900006,15.2,11.445757219));
#228580=CARTESIAN_POINT('Ctrl Pts',(-1.09418172900006,11.6,11.445757219));
#228581=CARTESIAN_POINT('Ctrl Pts',(-1.09498454400006,15.2,11.443610665));
#228582=CARTESIAN_POINT('Ctrl Pts',(-1.09498454400006,11.6,11.443610665));
#228583=CARTESIAN_POINT('Ctrl Pts',(-1.09605241700006,15.2,11.440750464));
#228584=CARTESIAN_POINT('Ctrl Pts',(-1.09605241700006,11.6,11.440750464));
#228585=CARTESIAN_POINT('Ctrl Pts',(-1.09738301600006,15.2,11.437178336));
#228586=CARTESIAN_POINT('Ctrl Pts',(-1.09738301600006,11.6,11.437178336));
#228587=CARTESIAN_POINT('Ctrl Pts',(-1.09870937300006,15.2,11.433609329));
#228588=CARTESIAN_POINT('Ctrl Pts',(-1.09870937300006,11.6,11.433609329));
#228589=CARTESIAN_POINT('Ctrl Pts',(-1.10003148900006,15.2,11.430043446));
#228590=CARTESIAN_POINT('Ctrl Pts',(-1.10003148900006,11.6,11.430043446));
#228591=CARTESIAN_POINT('Ctrl Pts',(-1.10134936300006,15.2,11.42648069));
#228592=CARTESIAN_POINT('Ctrl Pts',(-1.10134936300006,11.6,11.42648069));
#228593=CARTESIAN_POINT('Ctrl Pts',(-1.10266299900006,15.2,11.42292107));
#228594=CARTESIAN_POINT('Ctrl Pts',(-1.10266299900006,11.6,11.42292107));
#228595=CARTESIAN_POINT('Ctrl Pts',(-1.10397239800006,15.2,11.419364591));
#228596=CARTESIAN_POINT('Ctrl Pts',(-1.10397239800006,11.6,11.419364591));
#228597=CARTESIAN_POINT('Ctrl Pts',(-1.10527756400006,15.2,11.415811262));
#228598=CARTESIAN_POINT('Ctrl Pts',(-1.10527756400006,11.6,11.415811262));
#228599=CARTESIAN_POINT('Ctrl Pts',(-1.10657850100006,15.2,11.412261095));
#228600=CARTESIAN_POINT('Ctrl Pts',(-1.10657850100006,11.6,11.412261095));
#228601=CARTESIAN_POINT('Ctrl Pts',(-1.10787521000006,15.2,11.408714099));
#228602=CARTESIAN_POINT('Ctrl Pts',(-1.10787521000006,11.6,11.408714099));
#228603=CARTESIAN_POINT('Ctrl Pts',(-1.10916769700006,15.2,11.405170286));
#228604=CARTESIAN_POINT('Ctrl Pts',(-1.10916769700006,11.6,11.405170286));
#228605=CARTESIAN_POINT('Ctrl Pts',(-1.11045596300006,15.2,11.401629665));
#228606=CARTESIAN_POINT('Ctrl Pts',(-1.11045596300006,11.6,11.401629665));
#228607=CARTESIAN_POINT('Ctrl Pts',(-1.11174001400006,15.2,11.398092245));
#228608=CARTESIAN_POINT('Ctrl Pts',(-1.11174001400006,11.6,11.398092245));
#228609=CARTESIAN_POINT('Ctrl Pts',(-1.11301985000006,15.2,11.394558034));
#228610=CARTESIAN_POINT('Ctrl Pts',(-1.11301985000006,11.6,11.394558034));
#228611=CARTESIAN_POINT('Ctrl Pts',(-1.11429547500006,15.2,11.391027041));
#228612=CARTESIAN_POINT('Ctrl Pts',(-1.11429547500006,11.6,11.391027041));
#228613=CARTESIAN_POINT('Ctrl Pts',(-1.11556689100005,15.2,11.387499272));
#228614=CARTESIAN_POINT('Ctrl Pts',(-1.11556689100005,11.6,11.387499272));
#228615=CARTESIAN_POINT('Ctrl Pts',(-1.11683410000005,15.2,11.383974736));
#228616=CARTESIAN_POINT('Ctrl Pts',(-1.11683410000005,11.6,11.383974736));
#228617=CARTESIAN_POINT('Ctrl Pts',(-1.11809710700006,15.2,11.38045344));
#228618=CARTESIAN_POINT('Ctrl Pts',(-1.11809710700006,11.6,11.38045344));
#228619=CARTESIAN_POINT('Ctrl Pts',(-1.11935591200006,15.2,11.376935394));
#228620=CARTESIAN_POINT('Ctrl Pts',(-1.11935591200006,11.6,11.376935394));
#228621=CARTESIAN_POINT('Ctrl Pts',(-1.12061052000006,15.2,11.373420606));
#228622=CARTESIAN_POINT('Ctrl Pts',(-1.12061052000006,11.6,11.373420606));
#228623=CARTESIAN_POINT('Ctrl Pts',(-1.12186093300006,15.2,11.369909085));
#228624=CARTESIAN_POINT('Ctrl Pts',(-1.12186093300006,11.6,11.369909085));
#228625=CARTESIAN_POINT('Ctrl Pts',(-1.12310715500006,15.2,11.36640084));
#228626=CARTESIAN_POINT('Ctrl Pts',(-1.12310715500006,11.6,11.36640084));
#228627=CARTESIAN_POINT('Ctrl Pts',(-1.12434918700006,15.2,11.36289588));
#228628=CARTESIAN_POINT('Ctrl Pts',(-1.12434918700006,11.6,11.36289588));
#228629=CARTESIAN_POINT('Ctrl Pts',(-1.12558703500006,15.2,11.359394214));
#228630=CARTESIAN_POINT('Ctrl Pts',(-1.12558703500006,11.6,11.359394214));
#228631=CARTESIAN_POINT('Ctrl Pts',(-1.12682070000006,15.2,11.355895852));
#228632=CARTESIAN_POINT('Ctrl Pts',(-1.12682070000006,11.6,11.355895852));
#228633=CARTESIAN_POINT('Ctrl Pts',(-1.12805018600006,15.2,11.352400799));
#228634=CARTESIAN_POINT('Ctrl Pts',(-1.12805018600006,11.6,11.352400799));
#228635=CARTESIAN_POINT('Ctrl Pts',(-1.12927549500006,15.2,11.348909068));
#228636=CARTESIAN_POINT('Ctrl Pts',(-1.12927549500006,11.6,11.348909068));
#228637=CARTESIAN_POINT('Ctrl Pts',(-1.13049663000006,15.2,11.345420664));
#228638=CARTESIAN_POINT('Ctrl Pts',(-1.13049663000006,11.6,11.345420664));
#228639=CARTESIAN_POINT('Ctrl Pts',(-1.13171359400006,15.2,11.341935598));
#228640=CARTESIAN_POINT('Ctrl Pts',(-1.13171359400006,11.6,11.341935598));
#228641=CARTESIAN_POINT('Ctrl Pts',(-1.13292639100006,15.2,11.338453878));
#228642=CARTESIAN_POINT('Ctrl Pts',(-1.13292639100006,11.6,11.338453878));
#228643=CARTESIAN_POINT('Ctrl Pts',(-1.13413502300006,15.2,11.334975512));
#228644=CARTESIAN_POINT('Ctrl Pts',(-1.13413502300006,11.6,11.334975512));
#228645=CARTESIAN_POINT('Ctrl Pts',(-1.13533949400005,15.2,11.33150051));
#228646=CARTESIAN_POINT('Ctrl Pts',(-1.13533949400005,11.6,11.33150051));
#228647=CARTESIAN_POINT('Ctrl Pts',(-1.13653980600006,15.2,11.328028879));
#228648=CARTESIAN_POINT('Ctrl Pts',(-1.13653980600006,11.6,11.328028879));
#228649=CARTESIAN_POINT('Ctrl Pts',(-1.13773596300006,15.2,11.324560631));
#228650=CARTESIAN_POINT('Ctrl Pts',(-1.13773596300006,11.6,11.324560631));
#228651=CARTESIAN_POINT('Ctrl Pts',(-1.13892796700006,15.2,11.321095772));
#228652=CARTESIAN_POINT('Ctrl Pts',(-1.13892796700006,11.6,11.321095772));
#228653=CARTESIAN_POINT('Ctrl Pts',(-1.14011582300006,15.2,11.317634313));
#228654=CARTESIAN_POINT('Ctrl Pts',(-1.14011582300006,11.6,11.317634313));
#228655=CARTESIAN_POINT('Ctrl Pts',(-1.14129953300006,15.2,11.31417626));
#228656=CARTESIAN_POINT('Ctrl Pts',(-1.14129953300006,11.6,11.31417626));
#228657=CARTESIAN_POINT('Ctrl Pts',(-1.14247909900006,15.2,11.310721624));
#228658=CARTESIAN_POINT('Ctrl Pts',(-1.14247909900006,11.6,11.310721624));
#228659=CARTESIAN_POINT('Ctrl Pts',(-1.14365452600006,15.2,11.307270414));
#228660=CARTESIAN_POINT('Ctrl Pts',(-1.14365452600006,11.6,11.307270414));
#228661=CARTESIAN_POINT('Ctrl Pts',(-1.14482581600006,15.2,11.303822638));
#228662=CARTESIAN_POINT('Ctrl Pts',(-1.14482581600006,11.6,11.303822638));
#228663=CARTESIAN_POINT('Ctrl Pts',(-1.14599297300006,15.2,11.300378306));
#228664=CARTESIAN_POINT('Ctrl Pts',(-1.14599297300006,11.6,11.300378306));
#228665=CARTESIAN_POINT('Ctrl Pts',(-1.14715599900006,15.2,11.296937425));
#228666=CARTESIAN_POINT('Ctrl Pts',(-1.14715599900006,11.6,11.296937425));
#228667=CARTESIAN_POINT('Ctrl Pts',(-1.14831489900006,15.2,11.293500007));
#228668=CARTESIAN_POINT('Ctrl Pts',(-1.14831489900006,11.6,11.293500007));
#228669=CARTESIAN_POINT('Ctrl Pts',(-1.14946967500006,15.2,11.290066056));
#228670=CARTESIAN_POINT('Ctrl Pts',(-1.14946967500006,11.6,11.290066056));
#228671=CARTESIAN_POINT('Ctrl Pts',(-1.15062033100006,15.2,11.286635586));
#228672=CARTESIAN_POINT('Ctrl Pts',(-1.15062033100006,11.6,11.286635586));
#228673=CARTESIAN_POINT('Ctrl Pts',(-1.15176686800006,15.2,11.283208603));
#228674=CARTESIAN_POINT('Ctrl Pts',(-1.15176686800006,11.6,11.283208603));
#228675=CARTESIAN_POINT('Ctrl Pts',(-1.15290929200005,15.2,11.279785118));
#228676=CARTESIAN_POINT('Ctrl Pts',(-1.15290929200005,11.6,11.279785118));
#228677=CARTESIAN_POINT('Ctrl Pts',(-1.15404760400006,15.2,11.276365138));
#228678=CARTESIAN_POINT('Ctrl Pts',(-1.15404760400006,11.6,11.276365138));
#228679=CARTESIAN_POINT('Ctrl Pts',(-1.15518181000006,15.2,11.272948674));
#228680=CARTESIAN_POINT('Ctrl Pts',(-1.15518181000006,11.6,11.272948674));
#228681=CARTESIAN_POINT('Ctrl Pts',(-1.15631191200006,15.2,11.269535733));
#228682=CARTESIAN_POINT('Ctrl Pts',(-1.15631191200006,11.6,11.269535733));
#228683=CARTESIAN_POINT('Ctrl Pts',(-1.15743791100006,15.2,11.266126325));
#228684=CARTESIAN_POINT('Ctrl Pts',(-1.15743791100006,11.6,11.266126325));
#228685=CARTESIAN_POINT('Ctrl Pts',(-1.15855981400006,15.2,11.262720459));
#228686=CARTESIAN_POINT('Ctrl Pts',(-1.15855981400006,11.6,11.262720459));
#228687=CARTESIAN_POINT('Ctrl Pts',(-1.15967762200005,15.2,11.259318144));
#228688=CARTESIAN_POINT('Ctrl Pts',(-1.15967762200005,11.6,11.259318144));
#228689=CARTESIAN_POINT('Ctrl Pts',(-1.16079133800006,15.2,11.25591939));
#228690=CARTESIAN_POINT('Ctrl Pts',(-1.16079133800006,11.6,11.25591939));
#228691=CARTESIAN_POINT('Ctrl Pts',(-1.16190096800006,15.2,11.252524204));
#228692=CARTESIAN_POINT('Ctrl Pts',(-1.16190096800006,11.6,11.252524204));
#228693=CARTESIAN_POINT('Ctrl Pts',(-1.16300651300006,15.2,11.249132598));
#228694=CARTESIAN_POINT('Ctrl Pts',(-1.16300651300006,11.6,11.249132598));
#228695=CARTESIAN_POINT('Ctrl Pts',(-1.16410797800006,15.2,11.245744578));
#228696=CARTESIAN_POINT('Ctrl Pts',(-1.16410797800006,11.6,11.245744578));
#228697=CARTESIAN_POINT('Ctrl Pts',(-1.16520536400005,15.2,11.242360155));
#228698=CARTESIAN_POINT('Ctrl Pts',(-1.16520536400005,11.6,11.242360155));
#228699=CARTESIAN_POINT('Ctrl Pts',(-1.16629867800006,15.2,11.238979337));
#228700=CARTESIAN_POINT('Ctrl Pts',(-1.16629867800006,11.6,11.238979337));
#228701=CARTESIAN_POINT('Ctrl Pts',(-1.16738792000006,15.2,11.235602136));
#228702=CARTESIAN_POINT('Ctrl Pts',(-1.16738792000006,11.6,11.235602136));
#228703=CARTESIAN_POINT('Ctrl Pts',(-1.16847309500006,15.2,11.232228557));
#228704=CARTESIAN_POINT('Ctrl Pts',(-1.16847309500006,11.6,11.232228557));
#228705=CARTESIAN_POINT('Ctrl Pts',(-1.16955420600006,15.2,11.228858613));
#228706=CARTESIAN_POINT('Ctrl Pts',(-1.16955420600006,11.6,11.228858613));
#228707=CARTESIAN_POINT('Ctrl Pts',(-1.17063125700006,15.2,11.22549231));
#228708=CARTESIAN_POINT('Ctrl Pts',(-1.17063125700006,11.6,11.22549231));
#228709=CARTESIAN_POINT('Ctrl Pts',(-1.17170425100006,15.2,11.222129659));
#228710=CARTESIAN_POINT('Ctrl Pts',(-1.17170425100006,11.6,11.222129659));
#228711=CARTESIAN_POINT('Ctrl Pts',(-1.17277319200006,15.2,11.218770669));
#228712=CARTESIAN_POINT('Ctrl Pts',(-1.17277319200006,11.6,11.218770669));
#228713=CARTESIAN_POINT('Ctrl Pts',(-1.17383808200006,15.2,11.215415349));
#228714=CARTESIAN_POINT('Ctrl Pts',(-1.17383808200006,11.6,11.215415349));
#228715=CARTESIAN_POINT('Ctrl Pts',(-1.17489892800006,15.2,11.212063709));
#228716=CARTESIAN_POINT('Ctrl Pts',(-1.17489892800006,11.6,11.212063709));
#228717=CARTESIAN_POINT('Ctrl Pts',(-1.17595573000006,15.2,11.208715757));
#228718=CARTESIAN_POINT('Ctrl Pts',(-1.17595573000006,11.6,11.208715757));
#228719=CARTESIAN_POINT('Ctrl Pts',(-1.17700849300006,15.2,11.205371502));
#228720=CARTESIAN_POINT('Ctrl Pts',(-1.17700849300006,11.6,11.205371502));
#228721=CARTESIAN_POINT('Ctrl Pts',(-1.17805722000006,15.2,11.202030956));
#228722=CARTESIAN_POINT('Ctrl Pts',(-1.17805722000006,11.6,11.202030956));
#228723=CARTESIAN_POINT('Ctrl Pts',(-1.17910191400005,15.2,11.198694126));
#228724=CARTESIAN_POINT('Ctrl Pts',(-1.17910191400005,11.6,11.198694126));
#228725=CARTESIAN_POINT('Ctrl Pts',(-1.18014258100006,15.2,11.195361021));
#228726=CARTESIAN_POINT('Ctrl Pts',(-1.18014258100006,11.6,11.195361021));
#228727=CARTESIAN_POINT('Ctrl Pts',(-1.18117922300006,15.2,11.192031652));
#228728=CARTESIAN_POINT('Ctrl Pts',(-1.18117922300006,11.6,11.192031652));
#228729=CARTESIAN_POINT('Ctrl Pts',(-1.18221184300006,15.2,11.188706028));
#228730=CARTESIAN_POINT('Ctrl Pts',(-1.18221184300006,11.6,11.188706028));
#228731=CARTESIAN_POINT('Ctrl Pts',(-1.18324044700006,15.2,11.185384157));
#228732=CARTESIAN_POINT('Ctrl Pts',(-1.18324044700006,11.6,11.185384157));
#228733=CARTESIAN_POINT('Ctrl Pts',(-1.18426503600006,15.2,11.18206605));
#228734=CARTESIAN_POINT('Ctrl Pts',(-1.18426503600006,11.6,11.18206605));
#228735=CARTESIAN_POINT('Ctrl Pts',(-1.18528561400006,15.2,11.178751716));
#228736=CARTESIAN_POINT('Ctrl Pts',(-1.18528561400006,11.6,11.178751716));
#228737=CARTESIAN_POINT('Ctrl Pts',(-1.18630218600006,15.2,11.175441163));
#228738=CARTESIAN_POINT('Ctrl Pts',(-1.18630218600006,11.6,11.175441163));
#228739=CARTESIAN_POINT('Ctrl Pts',(-1.18731475500006,15.2,11.172134402));
#228740=CARTESIAN_POINT('Ctrl Pts',(-1.18731475500006,11.6,11.172134402));
#228741=CARTESIAN_POINT('Ctrl Pts',(-1.18832332500006,15.2,11.168831442));
#228742=CARTESIAN_POINT('Ctrl Pts',(-1.18832332500006,11.6,11.168831442));
#228743=CARTESIAN_POINT('Ctrl Pts',(-1.18932789900006,15.2,11.165532292));
#228744=CARTESIAN_POINT('Ctrl Pts',(-1.18932789900006,11.6,11.165532292));
#228745=CARTESIAN_POINT('Ctrl Pts',(-1.19032848200006,15.2,11.162236963));
#228746=CARTESIAN_POINT('Ctrl Pts',(-1.19032848200006,11.6,11.162236963));
#228747=CARTESIAN_POINT('Ctrl Pts',(-1.19132507600006,15.2,11.158945463));
#228748=CARTESIAN_POINT('Ctrl Pts',(-1.19132507600006,11.6,11.158945463));
#228749=CARTESIAN_POINT('Ctrl Pts',(-1.19231768600006,15.2,11.155657801));
#228750=CARTESIAN_POINT('Ctrl Pts',(-1.19231768600006,11.6,11.155657801));
#228751=CARTESIAN_POINT('Ctrl Pts',(-1.19330631700006,15.2,11.152373988));
#228752=CARTESIAN_POINT('Ctrl Pts',(-1.19330631700006,11.6,11.152373988));
#228753=CARTESIAN_POINT('Ctrl Pts',(-1.19429096900006,15.2,11.149094033));
#228754=CARTESIAN_POINT('Ctrl Pts',(-1.19429096900006,11.6,11.149094033));
#228755=CARTESIAN_POINT('Ctrl Pts',(-1.19527164900005,15.2,11.145817946));
#228756=CARTESIAN_POINT('Ctrl Pts',(-1.19527164900005,11.6,11.145817946));
#228757=CARTESIAN_POINT('Ctrl Pts',(-1.19624836000006,15.2,11.142545735));
#228758=CARTESIAN_POINT('Ctrl Pts',(-1.19624836000006,11.6,11.142545735));
#228759=CARTESIAN_POINT('Ctrl Pts',(-1.19722110600006,15.2,11.139277411));
#228760=CARTESIAN_POINT('Ctrl Pts',(-1.19722110600006,11.6,11.139277411));
#228761=CARTESIAN_POINT('Ctrl Pts',(-1.19818989100006,15.2,11.136012984));
#228762=CARTESIAN_POINT('Ctrl Pts',(-1.19818989100006,11.6,11.136012984));
#228763=CARTESIAN_POINT('Ctrl Pts',(-1.19915471800006,15.2,11.132752462));
#228764=CARTESIAN_POINT('Ctrl Pts',(-1.19915471800006,11.6,11.132752462));
#228765=CARTESIAN_POINT('Ctrl Pts',(-1.20011559100006,15.2,11.129495856));
#228766=CARTESIAN_POINT('Ctrl Pts',(-1.20011559100006,11.6,11.129495856));
#228767=CARTESIAN_POINT('Ctrl Pts',(-1.20107251500006,15.2,11.126243174));
#228768=CARTESIAN_POINT('Ctrl Pts',(-1.20107251500006,11.6,11.126243174));
#228769=CARTESIAN_POINT('Ctrl Pts',(-1.20202549300006,15.2,11.122994428));
#228770=CARTESIAN_POINT('Ctrl Pts',(-1.20202549300006,11.6,11.122994428));
#228771=CARTESIAN_POINT('Ctrl Pts',(-1.20297452900005,15.2,11.119749626));
#228772=CARTESIAN_POINT('Ctrl Pts',(-1.20297452900005,11.6,11.119749626));
#228773=CARTESIAN_POINT('Ctrl Pts',(-1.20391962700006,15.2,11.116508777));
#228774=CARTESIAN_POINT('Ctrl Pts',(-1.20391962700006,11.6,11.116508777));
#228775=CARTESIAN_POINT('Ctrl Pts',(-1.20486079100006,15.2,11.113271893));
#228776=CARTESIAN_POINT('Ctrl Pts',(-1.20486079100006,11.6,11.113271893));
#228777=CARTESIAN_POINT('Ctrl Pts',(-1.20579802500006,15.2,11.110038983));
#228778=CARTESIAN_POINT('Ctrl Pts',(-1.20579802500006,11.6,11.110038983));
#228779=CARTESIAN_POINT('Ctrl Pts',(-1.20673133300006,15.2,11.106810056));
#228780=CARTESIAN_POINT('Ctrl Pts',(-1.20673133300006,11.6,11.106810056));
#228781=CARTESIAN_POINT('Ctrl Pts',(-1.20766072000006,15.2,11.103585122));
#228782=CARTESIAN_POINT('Ctrl Pts',(-1.20766072000006,11.6,11.103585122));
#228783=CARTESIAN_POINT('Ctrl Pts',(-1.20858618900006,15.2,11.10036419));
#228784=CARTESIAN_POINT('Ctrl Pts',(-1.20858618900006,11.6,11.10036419));
#228785=CARTESIAN_POINT('Ctrl Pts',(-1.20950774300006,15.2,11.097147269));
#228786=CARTESIAN_POINT('Ctrl Pts',(-1.20950774300006,11.6,11.097147269));
#228787=CARTESIAN_POINT('Ctrl Pts',(-1.21042538700006,15.2,11.093934373));
#228788=CARTESIAN_POINT('Ctrl Pts',(-1.21042538700006,11.6,11.093934373));
#228789=CARTESIAN_POINT('Ctrl Pts',(-1.21133912600005,15.2,11.090725508));
#228790=CARTESIAN_POINT('Ctrl Pts',(-1.21133912600005,11.6,11.090725508));
#228791=CARTESIAN_POINT('Ctrl Pts',(-1.21224896300006,15.2,11.087520686));
#228792=CARTESIAN_POINT('Ctrl Pts',(-1.21224896300006,11.6,11.087520686));
#228793=CARTESIAN_POINT('Ctrl Pts',(-1.21315490300006,15.2,11.084319914));
#228794=CARTESIAN_POINT('Ctrl Pts',(-1.21315490300006,11.6,11.084319914));
#228795=CARTESIAN_POINT('Ctrl Pts',(-1.21405694800006,15.2,11.081123205));
#228796=CARTESIAN_POINT('Ctrl Pts',(-1.21405694800006,11.6,11.081123205));
#228797=CARTESIAN_POINT('Ctrl Pts',(-1.21495510500006,15.2,11.077930567));
#228798=CARTESIAN_POINT('Ctrl Pts',(-1.21495510500006,11.6,11.077930567));
#228799=CARTESIAN_POINT('Ctrl Pts',(-1.21584937600006,15.2,11.074742011));
#228800=CARTESIAN_POINT('Ctrl Pts',(-1.21584937600006,11.6,11.074742011));
#228801=CARTESIAN_POINT('Ctrl Pts',(-1.21673976600006,15.2,11.071557546));
#228802=CARTESIAN_POINT('Ctrl Pts',(-1.21673976600006,11.6,11.071557546));
#228803=CARTESIAN_POINT('Ctrl Pts',(-1.21762628000006,15.2,11.068377182));
#228804=CARTESIAN_POINT('Ctrl Pts',(-1.21762628000006,11.6,11.068377182));
#228805=CARTESIAN_POINT('Ctrl Pts',(-1.21850892000006,15.2,11.065200929));
#228806=CARTESIAN_POINT('Ctrl Pts',(-1.21850892000006,11.6,11.065200929));
#228807=CARTESIAN_POINT('Ctrl Pts',(-1.21938769300006,15.2,11.062028798));
#228808=CARTESIAN_POINT('Ctrl Pts',(-1.21938769300006,11.6,11.062028798));
#228809=CARTESIAN_POINT('Ctrl Pts',(-1.22026260100006,15.2,11.058860798));
#228810=CARTESIAN_POINT('Ctrl Pts',(-1.22026260100006,11.6,11.058860798));
#228811=CARTESIAN_POINT('Ctrl Pts',(-1.22113364900006,15.2,11.055696939));
#228812=CARTESIAN_POINT('Ctrl Pts',(-1.22113364900006,11.6,11.055696939));
#228813=CARTESIAN_POINT('Ctrl Pts',(-1.22200084200006,15.2,11.05253723));
#228814=CARTESIAN_POINT('Ctrl Pts',(-1.22200084200006,11.6,11.05253723));
#228815=CARTESIAN_POINT('Ctrl Pts',(-1.22286418200006,15.2,11.049381684));
#228816=CARTESIAN_POINT('Ctrl Pts',(-1.22286418200006,11.6,11.049381684));
#228817=CARTESIAN_POINT('Ctrl Pts',(-1.22372367600006,15.2,11.046230308));
#228818=CARTESIAN_POINT('Ctrl Pts',(-1.22372367600006,11.6,11.046230308));
#228819=CARTESIAN_POINT('Ctrl Pts',(-1.22457932700006,15.2,11.043083114));
#228820=CARTESIAN_POINT('Ctrl Pts',(-1.22457932700006,11.6,11.043083114));
#228821=CARTESIAN_POINT('Ctrl Pts',(-1.22543114100006,15.2,11.039940111));
#228822=CARTESIAN_POINT('Ctrl Pts',(-1.22543114100006,11.6,11.039940111));
#228823=CARTESIAN_POINT('Ctrl Pts',(-1.22627911900006,15.2,11.036801309));
#228824=CARTESIAN_POINT('Ctrl Pts',(-1.22627911900006,11.6,11.036801309));
#228825=CARTESIAN_POINT('Ctrl Pts',(-1.22712326800006,15.2,11.033666719));
#228826=CARTESIAN_POINT('Ctrl Pts',(-1.22712326800006,11.6,11.033666719));
#228827=CARTESIAN_POINT('Ctrl Pts',(-1.22796359200006,15.2,11.03053635));
#228828=CARTESIAN_POINT('Ctrl Pts',(-1.22796359200006,11.6,11.03053635));
#228829=CARTESIAN_POINT('Ctrl Pts',(-1.22880009300006,15.2,11.027410214));
#228830=CARTESIAN_POINT('Ctrl Pts',(-1.22880009300006,11.6,11.027410214));
#228831=CARTESIAN_POINT('Ctrl Pts',(-1.22963277900006,15.2,11.024288319));
#228832=CARTESIAN_POINT('Ctrl Pts',(-1.22963277900006,11.6,11.024288319));
#228833=CARTESIAN_POINT('Ctrl Pts',(-1.23046165300006,15.2,11.021170677));
#228834=CARTESIAN_POINT('Ctrl Pts',(-1.23046165300006,11.6,11.021170677));
#228835=CARTESIAN_POINT('Ctrl Pts',(-1.23128671900006,15.2,11.018057297));
#228836=CARTESIAN_POINT('Ctrl Pts',(-1.23128671900006,11.6,11.018057297));
#228837=CARTESIAN_POINT('Ctrl Pts',(-1.23210798200006,15.2,11.014948189));
#228838=CARTESIAN_POINT('Ctrl Pts',(-1.23210798200006,11.6,11.014948189));
#228839=CARTESIAN_POINT('Ctrl Pts',(-1.23292544600006,15.2,11.011843364));
#228840=CARTESIAN_POINT('Ctrl Pts',(-1.23292544600006,11.6,11.011843364));
#228841=CARTESIAN_POINT('Ctrl Pts',(-1.23373911600006,15.2,11.008742833));
#228842=CARTESIAN_POINT('Ctrl Pts',(-1.23373911600006,11.6,11.008742833));
#228843=CARTESIAN_POINT('Ctrl Pts',(-1.23454899600006,15.2,11.005646604));
#228844=CARTESIAN_POINT('Ctrl Pts',(-1.23454899600006,11.6,11.005646604));
#228845=CARTESIAN_POINT('Ctrl Pts',(-1.23535509200006,15.2,11.00255469));
#228846=CARTESIAN_POINT('Ctrl Pts',(-1.23535509200006,11.6,11.00255469));
#228847=CARTESIAN_POINT('Ctrl Pts',(-1.23615740600005,15.2,10.999467099));
#228848=CARTESIAN_POINT('Ctrl Pts',(-1.23615740600005,11.6,10.999467099));
#228849=CARTESIAN_POINT('Ctrl Pts',(-1.23695594400006,15.2,10.996383843));
#228850=CARTESIAN_POINT('Ctrl Pts',(-1.23695594400006,11.6,10.996383843));
#228851=CARTESIAN_POINT('Ctrl Pts',(-1.23775071100006,15.2,10.99330493));
#228852=CARTESIAN_POINT('Ctrl Pts',(-1.23775071100006,11.6,10.99330493));
#228853=CARTESIAN_POINT('Ctrl Pts',(-1.23854171100006,15.2,10.990230373));
#228854=CARTESIAN_POINT('Ctrl Pts',(-1.23854171100006,11.6,10.990230373));
#228855=CARTESIAN_POINT('Ctrl Pts',(-1.23932894900006,15.2,10.987160181));
#228856=CARTESIAN_POINT('Ctrl Pts',(-1.23932894900006,11.6,10.987160181));
#228857=CARTESIAN_POINT('Ctrl Pts',(-1.24011243000006,15.2,10.984094365));
#228858=CARTESIAN_POINT('Ctrl Pts',(-1.24011243000006,11.6,10.984094365));
#228859=CARTESIAN_POINT('Ctrl Pts',(-1.24089215700006,15.2,10.981032934));
#228860=CARTESIAN_POINT('Ctrl Pts',(-1.24089215700006,11.6,10.981032934));
#228861=CARTESIAN_POINT('Ctrl Pts',(-1.24166813600006,15.2,10.977975901));
#228862=CARTESIAN_POINT('Ctrl Pts',(-1.24166813600006,11.6,10.977975901));
#228863=CARTESIAN_POINT('Ctrl Pts',(-1.24244037200006,15.2,10.974923274));
#228864=CARTESIAN_POINT('Ctrl Pts',(-1.24244037200006,11.6,10.974923274));
#228865=CARTESIAN_POINT('Ctrl Pts',(-1.24320886800006,15.2,10.971875065));
#228866=CARTESIAN_POINT('Ctrl Pts',(-1.24320886800006,11.6,10.971875065));
#228867=CARTESIAN_POINT('Ctrl Pts',(-1.24397363200006,15.2,10.968831284));
#228868=CARTESIAN_POINT('Ctrl Pts',(-1.24397363200006,11.6,10.968831284));
#228869=CARTESIAN_POINT('Ctrl Pts',(-1.24473466500006,15.2,10.965791942));
#228870=CARTESIAN_POINT('Ctrl Pts',(-1.24473466500006,11.6,10.965791942));
#228871=CARTESIAN_POINT('Ctrl Pts',(-1.24549197400005,15.2,10.962757048));
#228872=CARTESIAN_POINT('Ctrl Pts',(-1.24549197400005,11.6,10.962757048));
#228873=CARTESIAN_POINT('Ctrl Pts',(-1.24624556200006,15.2,10.959726614));
#228874=CARTESIAN_POINT('Ctrl Pts',(-1.24624556200006,11.6,10.959726614));
#228875=CARTESIAN_POINT('Ctrl Pts',(-1.24699543600006,15.2,10.95670065));
#228876=CARTESIAN_POINT('Ctrl Pts',(-1.24699543600006,11.6,10.95670065));
#228877=CARTESIAN_POINT('Ctrl Pts',(-1.24774160000006,15.2,10.953679167));
#228878=CARTESIAN_POINT('Ctrl Pts',(-1.24774160000006,11.6,10.953679167));
#228879=CARTESIAN_POINT('Ctrl Pts',(-1.24848405900006,15.2,10.950662174));
#228880=CARTESIAN_POINT('Ctrl Pts',(-1.24848405900006,11.6,10.950662174));
#228881=CARTESIAN_POINT('Ctrl Pts',(-1.24922281700006,15.2,10.947649683));
#228882=CARTESIAN_POINT('Ctrl Pts',(-1.24922281700006,11.6,10.947649683));
#228883=CARTESIAN_POINT('Ctrl Pts',(-1.24995788000006,15.2,10.944641706));
#228884=CARTESIAN_POINT('Ctrl Pts',(-1.24995788000006,11.6,10.944641706));
#228885=CARTESIAN_POINT('Ctrl Pts',(-1.25068925200006,15.2,10.941638251));
#228886=CARTESIAN_POINT('Ctrl Pts',(-1.25068925200006,11.6,10.941638251));
#228887=CARTESIAN_POINT('Ctrl Pts',(-1.25141693800006,15.2,10.93863933));
#228888=CARTESIAN_POINT('Ctrl Pts',(-1.25141693800006,11.6,10.93863933));
#228889=CARTESIAN_POINT('Ctrl Pts',(-1.25214094400006,15.2,10.935644954));
#228890=CARTESIAN_POINT('Ctrl Pts',(-1.25214094400006,11.6,10.935644954));
#228891=CARTESIAN_POINT('Ctrl Pts',(-1.25286127400006,15.2,10.932655133));
#228892=CARTESIAN_POINT('Ctrl Pts',(-1.25286127400006,11.6,10.932655133));
#228893=CARTESIAN_POINT('Ctrl Pts',(-1.25357793200006,15.2,10.929669878));
#228894=CARTESIAN_POINT('Ctrl Pts',(-1.25357793200006,11.6,10.929669878));
#228895=CARTESIAN_POINT('Ctrl Pts',(-1.25429092600006,15.2,10.926689199));
#228896=CARTESIAN_POINT('Ctrl Pts',(-1.25429092600006,11.6,10.926689199));
#228897=CARTESIAN_POINT('Ctrl Pts',(-1.25500025800006,15.2,10.923713109));
#228898=CARTESIAN_POINT('Ctrl Pts',(-1.25500025800006,11.6,10.923713109));
#228899=CARTESIAN_POINT('Ctrl Pts',(-1.25570593400006,15.2,10.920741617));
#228900=CARTESIAN_POINT('Ctrl Pts',(-1.25570593400006,11.6,10.920741617));
#228901=CARTESIAN_POINT('Ctrl Pts',(-1.25640795900006,15.2,10.917774733));
#228902=CARTESIAN_POINT('Ctrl Pts',(-1.25640795900006,11.6,10.917774733));
#228903=CARTESIAN_POINT('Ctrl Pts',(-1.25710633900006,15.2,10.914812471));
#228904=CARTESIAN_POINT('Ctrl Pts',(-1.25710633900006,11.6,10.914812471));
#228905=CARTESIAN_POINT('Ctrl Pts',(-1.25780107900006,15.2,10.911854838));
#228906=CARTESIAN_POINT('Ctrl Pts',(-1.25780107900006,11.6,10.911854838));
#228907=CARTESIAN_POINT('Ctrl Pts',(-1.25849218300006,15.2,10.908901847));
#228908=CARTESIAN_POINT('Ctrl Pts',(-1.25849218300006,11.6,10.908901847));
#228909=CARTESIAN_POINT('Ctrl Pts',(-1.25917965600006,15.2,10.905953509));
#228910=CARTESIAN_POINT('Ctrl Pts',(-1.25917965600006,11.6,10.905953509));
#228911=CARTESIAN_POINT('Ctrl Pts',(-1.25986350500006,15.2,10.903009835));
#228912=CARTESIAN_POINT('Ctrl Pts',(-1.25986350500006,11.6,10.903009835));
#228913=CARTESIAN_POINT('Ctrl Pts',(-1.26054373300006,15.2,10.900070834));
#228914=CARTESIAN_POINT('Ctrl Pts',(-1.26054373300006,11.6,10.900070834));
#228915=CARTESIAN_POINT('Ctrl Pts',(-1.26122034700006,15.2,10.897136519));
#228916=CARTESIAN_POINT('Ctrl Pts',(-1.26122034700006,11.6,10.897136519));
#228917=CARTESIAN_POINT('Ctrl Pts',(-1.26189335100006,15.2,10.894206902));
#228918=CARTESIAN_POINT('Ctrl Pts',(-1.26189335100006,11.6,10.894206902));
#228919=CARTESIAN_POINT('Ctrl Pts',(-1.26256275000006,15.2,10.891281991));
#228920=CARTESIAN_POINT('Ctrl Pts',(-1.26256275000006,11.6,10.891281991));
#228921=CARTESIAN_POINT('Ctrl Pts',(-1.26322855100006,15.2,10.888361797));
#228922=CARTESIAN_POINT('Ctrl Pts',(-1.26322855100006,11.6,10.888361797));
#228923=CARTESIAN_POINT('Ctrl Pts',(-1.26389075800006,15.2,10.885446334));
#228924=CARTESIAN_POINT('Ctrl Pts',(-1.26389075800006,11.6,10.885446334));
#228925=CARTESIAN_POINT('Ctrl Pts',(-1.26454937500006,15.2,10.882535612));
#228926=CARTESIAN_POINT('Ctrl Pts',(-1.26454937500006,11.6,10.882535612));
#228927=CARTESIAN_POINT('Ctrl Pts',(-1.26520441000006,15.2,10.879629641));
#228928=CARTESIAN_POINT('Ctrl Pts',(-1.26520441000006,11.6,10.879629641));
#228929=CARTESIAN_POINT('Ctrl Pts',(-1.26585586800006,15.2,10.876728433));
#228930=CARTESIAN_POINT('Ctrl Pts',(-1.26585586800006,11.6,10.876728433));
#228931=CARTESIAN_POINT('Ctrl Pts',(-1.26650375300006,15.2,10.873831998));
#228932=CARTESIAN_POINT('Ctrl Pts',(-1.26650375300006,11.6,10.873831998));
#228933=CARTESIAN_POINT('Ctrl Pts',(-1.26714807000006,15.2,10.870940349));
#228934=CARTESIAN_POINT('Ctrl Pts',(-1.26714807000006,11.6,10.870940349));
#228935=CARTESIAN_POINT('Ctrl Pts',(-1.26778882500005,15.2,10.868053496));
#228936=CARTESIAN_POINT('Ctrl Pts',(-1.26778882500005,11.6,10.868053496));
#228937=CARTESIAN_POINT('Ctrl Pts',(-1.26842602500005,15.2,10.86517145));
#228938=CARTESIAN_POINT('Ctrl Pts',(-1.26842602500005,11.6,10.86517145));
#228939=CARTESIAN_POINT('Ctrl Pts',(-1.26905967300006,15.2,10.862294222));
#228940=CARTESIAN_POINT('Ctrl Pts',(-1.26905967300006,11.6,10.862294222));
#228941=CARTESIAN_POINT('Ctrl Pts',(-1.26968977600006,15.2,10.859421824));
#228942=CARTESIAN_POINT('Ctrl Pts',(-1.26968977600006,11.6,10.859421824));
#228943=CARTESIAN_POINT('Ctrl Pts',(-1.27031633900006,15.2,10.856554268));
#228944=CARTESIAN_POINT('Ctrl Pts',(-1.27031633900006,11.6,10.856554268));
#228945=CARTESIAN_POINT('Ctrl Pts',(-1.27093936800006,15.2,10.853691564));
#228946=CARTESIAN_POINT('Ctrl Pts',(-1.27093936800006,11.6,10.853691564));
#228947=CARTESIAN_POINT('Ctrl Pts',(-1.27155886700006,15.2,10.850833723));
#228948=CARTESIAN_POINT('Ctrl Pts',(-1.27155886700006,11.6,10.850833723));
#228949=CARTESIAN_POINT('Ctrl Pts',(-1.27217484300005,15.2,10.847980757));
#228950=CARTESIAN_POINT('Ctrl Pts',(-1.27217484300005,11.6,10.847980757));
#228951=CARTESIAN_POINT('Ctrl Pts',(-1.27278730200006,15.2,10.845132678));
#228952=CARTESIAN_POINT('Ctrl Pts',(-1.27278730200006,11.6,10.845132678));
#228953=CARTESIAN_POINT('Ctrl Pts',(-1.27339624900006,15.2,10.842289496));
#228954=CARTESIAN_POINT('Ctrl Pts',(-1.27339624900006,11.6,10.842289496));
#228955=CARTESIAN_POINT('Ctrl Pts',(-1.27400168800005,15.2,10.839451223));
#228956=CARTESIAN_POINT('Ctrl Pts',(-1.27400168800005,11.6,10.839451223));
#228957=CARTESIAN_POINT('Ctrl Pts',(-1.27460362700006,15.2,10.836617871));
#228958=CARTESIAN_POINT('Ctrl Pts',(-1.27460362700006,11.6,10.836617871));
#228959=CARTESIAN_POINT('Ctrl Pts',(-1.27520207000006,15.2,10.83378945));
#228960=CARTESIAN_POINT('Ctrl Pts',(-1.27520207000006,11.6,10.83378945));
#228961=CARTESIAN_POINT('Ctrl Pts',(-1.27579702400006,15.2,10.830965973));
#228962=CARTESIAN_POINT('Ctrl Pts',(-1.27579702400006,11.6,10.830965973));
#228963=CARTESIAN_POINT('Ctrl Pts',(-1.27638849400006,15.2,10.82814745));
#228964=CARTESIAN_POINT('Ctrl Pts',(-1.27638849400006,11.6,10.82814745));
#228965=CARTESIAN_POINT('Ctrl Pts',(-1.27697648500006,15.2,10.825333894));
#228966=CARTESIAN_POINT('Ctrl Pts',(-1.27697648500006,11.6,10.825333894));
#228967=CARTESIAN_POINT('Ctrl Pts',(-1.27756100500006,15.2,10.822525316));
#228968=CARTESIAN_POINT('Ctrl Pts',(-1.27756100500006,11.6,10.822525316));
#228969=CARTESIAN_POINT('Ctrl Pts',(-1.27814205700005,15.2,10.819721727));
#228970=CARTESIAN_POINT('Ctrl Pts',(-1.27814205700005,11.6,10.819721727));
#228971=CARTESIAN_POINT('Ctrl Pts',(-1.27871964800006,15.2,10.816923139));
#228972=CARTESIAN_POINT('Ctrl Pts',(-1.27871964800006,11.6,10.816923139));
#228973=CARTESIAN_POINT('Ctrl Pts',(-1.27929378500006,15.2,10.814129563));
#228974=CARTESIAN_POINT('Ctrl Pts',(-1.27929378500006,11.6,10.814129563));
#228975=CARTESIAN_POINT('Ctrl Pts',(-1.27986447300006,15.2,10.811341012));
#228976=CARTESIAN_POINT('Ctrl Pts',(-1.27986447300006,11.6,10.811341012));
#228977=CARTESIAN_POINT('Ctrl Pts',(-1.28043171600006,15.2,10.808557496));
#228978=CARTESIAN_POINT('Ctrl Pts',(-1.28043171600006,11.6,10.808557496));
#228979=CARTESIAN_POINT('Ctrl Pts',(-1.28099552200006,15.2,10.805779029));
#228980=CARTESIAN_POINT('Ctrl Pts',(-1.28099552200006,11.6,10.805779029));
#228981=CARTESIAN_POINT('Ctrl Pts',(-1.28155589700006,15.2,10.803005619));
#228982=CARTESIAN_POINT('Ctrl Pts',(-1.28155589700006,11.6,10.803005619));
#228983=CARTESIAN_POINT('Ctrl Pts',(-1.28211284600006,15.2,10.800237282));
#228984=CARTESIAN_POINT('Ctrl Pts',(-1.28211284600006,11.6,10.800237282));
#228985=CARTESIAN_POINT('Ctrl Pts',(-1.28266637500006,15.2,10.797474027));
#228986=CARTESIAN_POINT('Ctrl Pts',(-1.28266637500006,11.6,10.797474027));
#228987=CARTESIAN_POINT('Ctrl Pts',(-1.28321649000006,15.2,10.794715865));
#228988=CARTESIAN_POINT('Ctrl Pts',(-1.28321649000006,11.6,10.794715865));
#228989=CARTESIAN_POINT('Ctrl Pts',(-1.28376319800006,15.2,10.79196281));
#228990=CARTESIAN_POINT('Ctrl Pts',(-1.28376319800006,11.6,10.79196281));
#228991=CARTESIAN_POINT('Ctrl Pts',(-1.28430650400006,15.2,10.789214874));
#228992=CARTESIAN_POINT('Ctrl Pts',(-1.28430650400006,11.6,10.789214874));
#228993=CARTESIAN_POINT('Ctrl Pts',(-1.28484641400005,15.2,10.786472066));
#228994=CARTESIAN_POINT('Ctrl Pts',(-1.28484641400005,11.6,10.786472066));
#228995=CARTESIAN_POINT('Ctrl Pts',(-1.28538293400006,15.2,10.783734401));
#228996=CARTESIAN_POINT('Ctrl Pts',(-1.28538293400006,11.6,10.783734401));
#228997=CARTESIAN_POINT('Ctrl Pts',(-1.28591607100006,15.2,10.781001889));
#228998=CARTESIAN_POINT('Ctrl Pts',(-1.28591607100006,11.6,10.781001889));
#228999=CARTESIAN_POINT('Ctrl Pts',(-1.28644583000006,15.2,10.778274542));
#229000=CARTESIAN_POINT('Ctrl Pts',(-1.28644583000006,11.6,10.778274542));
#229001=CARTESIAN_POINT('Ctrl Pts',(-1.28697221900006,15.2,10.775552373));
#229002=CARTESIAN_POINT('Ctrl Pts',(-1.28697221900006,11.6,10.775552373));
#229003=CARTESIAN_POINT('Ctrl Pts',(-1.28749524100006,15.2,10.772835393));
#229004=CARTESIAN_POINT('Ctrl Pts',(-1.28749524100006,11.6,10.772835393));
#229005=CARTESIAN_POINT('Ctrl Pts',(-1.28801490600006,15.2,10.770123615));
#229006=CARTESIAN_POINT('Ctrl Pts',(-1.28801490600006,11.6,10.770123615));
#229007=CARTESIAN_POINT('Ctrl Pts',(-1.28853121600006,15.2,10.767417049));
#229008=CARTESIAN_POINT('Ctrl Pts',(-1.28853121600006,11.6,10.767417049));
#229009=CARTESIAN_POINT('Ctrl Pts',(-1.28904418100006,15.2,10.764715709));
#229010=CARTESIAN_POINT('Ctrl Pts',(-1.28904418100006,11.6,10.764715709));
#229011=CARTESIAN_POINT('Ctrl Pts',(-1.28955380600006,15.2,10.762019607));
#229012=CARTESIAN_POINT('Ctrl Pts',(-1.28955380600006,11.6,10.762019607));
#229013=CARTESIAN_POINT('Ctrl Pts',(-1.29006009600006,15.2,10.759328754));
#229014=CARTESIAN_POINT('Ctrl Pts',(-1.29006009600006,11.6,10.759328754));
#229015=CARTESIAN_POINT('Ctrl Pts',(-1.29056305900005,15.2,10.756643162));
#229016=CARTESIAN_POINT('Ctrl Pts',(-1.29056305900005,11.6,10.756643162));
#229017=CARTESIAN_POINT('Ctrl Pts',(-1.29106270000006,15.2,10.753962845));
#229018=CARTESIAN_POINT('Ctrl Pts',(-1.29106270000006,11.6,10.753962845));
#229019=CARTESIAN_POINT('Ctrl Pts',(-1.29155902700006,15.2,10.751287813));
#229020=CARTESIAN_POINT('Ctrl Pts',(-1.29155902700006,11.6,10.751287813));
#229021=CARTESIAN_POINT('Ctrl Pts',(-1.29205204400006,15.2,10.748618079));
#229022=CARTESIAN_POINT('Ctrl Pts',(-1.29205204400006,11.6,10.748618079));
#229023=CARTESIAN_POINT('Ctrl Pts',(-1.29254176000006,15.2,10.745953656));
#229024=CARTESIAN_POINT('Ctrl Pts',(-1.29254176000006,11.6,10.745953656));
#229025=CARTESIAN_POINT('Ctrl Pts',(-1.29302817900006,15.2,10.743294555));
#229026=CARTESIAN_POINT('Ctrl Pts',(-1.29302817900006,11.6,10.743294555));
#229027=CARTESIAN_POINT('Ctrl Pts',(-1.29351131000006,15.2,10.740640789));
#229028=CARTESIAN_POINT('Ctrl Pts',(-1.29351131000006,11.6,10.740640789));
#229029=CARTESIAN_POINT('Ctrl Pts',(-1.29399115800006,15.2,10.73799237));
#229030=CARTESIAN_POINT('Ctrl Pts',(-1.29399115800006,11.6,10.73799237));
#229031=CARTESIAN_POINT('Ctrl Pts',(-1.29446772900006,15.2,10.73534931));
#229032=CARTESIAN_POINT('Ctrl Pts',(-1.29446772900006,11.6,10.73534931));
#229033=CARTESIAN_POINT('Ctrl Pts',(-1.29494103100006,15.2,10.732711622));
#229034=CARTESIAN_POINT('Ctrl Pts',(-1.29494103100006,11.6,10.732711622));
#229035=CARTESIAN_POINT('Ctrl Pts',(-1.29541106900006,15.2,10.730079318));
#229036=CARTESIAN_POINT('Ctrl Pts',(-1.29541106900006,11.6,10.730079318));
#229037=CARTESIAN_POINT('Ctrl Pts',(-1.29587785100005,15.2,10.727452412));
#229038=CARTESIAN_POINT('Ctrl Pts',(-1.29587785100005,11.6,10.727452412));
#229039=CARTESIAN_POINT('Ctrl Pts',(-1.29634138200006,15.2,10.724830913));
#229040=CARTESIAN_POINT('Ctrl Pts',(-1.29634138200006,11.6,10.724830913));
#229041=CARTESIAN_POINT('Ctrl Pts',(-1.29680167100006,15.2,10.722214836));
#229042=CARTESIAN_POINT('Ctrl Pts',(-1.29680167100006,11.6,10.722214836));
#229043=CARTESIAN_POINT('Ctrl Pts',(-1.29725872200006,15.2,10.719604193));
#229044=CARTESIAN_POINT('Ctrl Pts',(-1.29725872200006,11.6,10.719604193));
#229045=CARTESIAN_POINT('Ctrl Pts',(-1.29771254400006,15.2,10.716998997));
#229046=CARTESIAN_POINT('Ctrl Pts',(-1.29771254400006,11.6,10.716998997));
#229047=CARTESIAN_POINT('Ctrl Pts',(-1.29816314300006,15.2,10.714399259));
#229048=CARTESIAN_POINT('Ctrl Pts',(-1.29816314300006,11.6,10.714399259));
#229049=CARTESIAN_POINT('Ctrl Pts',(-1.29861052400006,15.2,10.711804993));
#229050=CARTESIAN_POINT('Ctrl Pts',(-1.29861052400006,11.6,10.711804993));
#229051=CARTESIAN_POINT('Ctrl Pts',(-1.29905469700006,15.2,10.709216211));
#229052=CARTESIAN_POINT('Ctrl Pts',(-1.29905469700006,11.6,10.709216211));
#229053=CARTESIAN_POINT('Ctrl Pts',(-1.29949566600006,15.2,10.706632926));
#229054=CARTESIAN_POINT('Ctrl Pts',(-1.29949566600006,11.6,10.706632926));
#229055=CARTESIAN_POINT('Ctrl Pts',(-1.29993343800006,15.2,10.70405515));
#229056=CARTESIAN_POINT('Ctrl Pts',(-1.29993343800006,11.6,10.70405515));
#229057=CARTESIAN_POINT('Ctrl Pts',(-1.30036802200006,15.2,10.701482895));
#229058=CARTESIAN_POINT('Ctrl Pts',(-1.30036802200006,11.6,10.701482895));
#229059=CARTESIAN_POINT('Ctrl Pts',(-1.30079942300006,15.2,10.698916176));
#229060=CARTESIAN_POINT('Ctrl Pts',(-1.30079942300006,11.6,10.698916176));
#229061=CARTESIAN_POINT('Ctrl Pts',(-1.30122764900006,15.2,10.696355005));
#229062=CARTESIAN_POINT('Ctrl Pts',(-1.30122764900006,11.6,10.696355005));
#229063=CARTESIAN_POINT('Ctrl Pts',(-1.30165270600005,15.2,10.693799394));
#229064=CARTESIAN_POINT('Ctrl Pts',(-1.30165270600005,11.6,10.693799394));
#229065=CARTESIAN_POINT('Ctrl Pts',(-1.30207460100006,15.2,10.691249355));
#229066=CARTESIAN_POINT('Ctrl Pts',(-1.30207460100006,11.6,10.691249355));
#229067=CARTESIAN_POINT('Ctrl Pts',(-1.30249334300006,15.2,10.688704903));
#229068=CARTESIAN_POINT('Ctrl Pts',(-1.30249334300006,11.6,10.688704903));
#229069=CARTESIAN_POINT('Ctrl Pts',(-1.30290893600006,15.2,10.686166049));
#229070=CARTESIAN_POINT('Ctrl Pts',(-1.30290893600006,11.6,10.686166049));
#229071=CARTESIAN_POINT('Ctrl Pts',(-1.30332138800005,15.2,10.683632807));
#229072=CARTESIAN_POINT('Ctrl Pts',(-1.30332138800005,11.6,10.683632807));
#229073=CARTESIAN_POINT('Ctrl Pts',(-1.30373070700006,15.2,10.681105189));
#229074=CARTESIAN_POINT('Ctrl Pts',(-1.30373070700006,11.6,10.681105189));
#229075=CARTESIAN_POINT('Ctrl Pts',(-1.30413690000006,15.2,10.678583208));
#229076=CARTESIAN_POINT('Ctrl Pts',(-1.30413690000006,11.6,10.678583208));
#229077=CARTESIAN_POINT('Ctrl Pts',(-1.30453997400006,15.2,10.676066878));
#229078=CARTESIAN_POINT('Ctrl Pts',(-1.30453997400006,11.6,10.676066878));
#229079=CARTESIAN_POINT('Ctrl Pts',(-1.30493993500005,15.2,10.673556212));
#229080=CARTESIAN_POINT('Ctrl Pts',(-1.30493993500005,11.6,10.673556212));
#229081=CARTESIAN_POINT('Ctrl Pts',(-1.30533679100005,15.2,10.671051222));
#229082=CARTESIAN_POINT('Ctrl Pts',(-1.30533679100005,11.6,10.671051222));
#229083=CARTESIAN_POINT('Ctrl Pts',(-1.30573055000006,15.2,10.668551921));
#229084=CARTESIAN_POINT('Ctrl Pts',(-1.30573055000006,11.6,10.668551921));
#229085=CARTESIAN_POINT('Ctrl Pts',(-1.30612121800006,15.2,10.666058323));
#229086=CARTESIAN_POINT('Ctrl Pts',(-1.30612121800006,11.6,10.666058323));
#229087=CARTESIAN_POINT('Ctrl Pts',(-1.30650880400006,15.2,10.663570442));
#229088=CARTESIAN_POINT('Ctrl Pts',(-1.30650880400006,11.6,10.663570442));
#229089=CARTESIAN_POINT('Ctrl Pts',(-1.30689331300006,15.2,10.661088288));
#229090=CARTESIAN_POINT('Ctrl Pts',(-1.30689331300006,11.6,10.661088288));
#229091=CARTESIAN_POINT('Ctrl Pts',(-1.30727475400006,15.2,10.658611876));
#229092=CARTESIAN_POINT('Ctrl Pts',(-1.30727475400006,11.6,10.658611876));
#229093=CARTESIAN_POINT('Ctrl Pts',(-1.30765313300006,15.2,10.656141221));
#229094=CARTESIAN_POINT('Ctrl Pts',(-1.30765313300006,11.6,10.656141221));
#229095=CARTESIAN_POINT('Ctrl Pts',(-1.30802846000006,15.2,10.653676333));
#229096=CARTESIAN_POINT('Ctrl Pts',(-1.30802846000006,11.6,10.653676333));
#229097=CARTESIAN_POINT('Ctrl Pts',(-1.30840073900006,15.2,10.651217227));
#229098=CARTESIAN_POINT('Ctrl Pts',(-1.30840073900006,11.6,10.651217227));
#229099=CARTESIAN_POINT('Ctrl Pts',(-1.30876997900006,15.2,10.648763916));
#229100=CARTESIAN_POINT('Ctrl Pts',(-1.30876997900006,11.6,10.648763916));
#229101=CARTESIAN_POINT('Ctrl Pts',(-1.30913618800006,15.2,10.646316414));
#229102=CARTESIAN_POINT('Ctrl Pts',(-1.30913618800006,11.6,10.646316414));
#229103=CARTESIAN_POINT('Ctrl Pts',(-1.30949937300006,15.2,10.643874734));
#229104=CARTESIAN_POINT('Ctrl Pts',(-1.30949937300006,11.6,10.643874734));
#229105=CARTESIAN_POINT('Ctrl Pts',(-1.30985954300006,15.2,10.641438888));
#229106=CARTESIAN_POINT('Ctrl Pts',(-1.30985954300006,11.6,10.641438888));
#229107=CARTESIAN_POINT('Ctrl Pts',(-1.31021670300006,15.2,10.639008892));
#229108=CARTESIAN_POINT('Ctrl Pts',(-1.31021670300006,11.6,10.639008892));
#229109=CARTESIAN_POINT('Ctrl Pts',(-1.31057086200006,15.2,10.636584757));
#229110=CARTESIAN_POINT('Ctrl Pts',(-1.31057086200006,11.6,10.636584757));
#229111=CARTESIAN_POINT('Ctrl Pts',(-1.31092202700006,15.2,10.634166497));
#229112=CARTESIAN_POINT('Ctrl Pts',(-1.31092202700006,11.6,10.634166497));
#229113=CARTESIAN_POINT('Ctrl Pts',(-1.31127020600006,15.2,10.631754128));
#229114=CARTESIAN_POINT('Ctrl Pts',(-1.31127020600006,11.6,10.631754128));
#229115=CARTESIAN_POINT('Ctrl Pts',(-1.31161540800006,15.2,10.629347661));
#229116=CARTESIAN_POINT('Ctrl Pts',(-1.31161540800006,11.6,10.629347661));
#229117=CARTESIAN_POINT('Ctrl Pts',(-1.31195763900006,15.2,10.62694711));
#229118=CARTESIAN_POINT('Ctrl Pts',(-1.31195763900006,11.6,10.62694711));
#229119=CARTESIAN_POINT('Ctrl Pts',(-1.31229690700006,15.2,10.624552489));
#229120=CARTESIAN_POINT('Ctrl Pts',(-1.31229690700006,11.6,10.624552489));
#229121=CARTESIAN_POINT('Ctrl Pts',(-1.31263322100006,15.2,10.622163811));
#229122=CARTESIAN_POINT('Ctrl Pts',(-1.31263322100006,11.6,10.622163811));
#229123=CARTESIAN_POINT('Ctrl Pts',(-1.31296658700006,15.2,10.619781092));
#229124=CARTESIAN_POINT('Ctrl Pts',(-1.31296658700006,11.6,10.619781092));
#229125=CARTESIAN_POINT('Ctrl Pts',(-1.31329701400006,15.2,10.617404342));
#229126=CARTESIAN_POINT('Ctrl Pts',(-1.31329701400006,11.6,10.617404342));
#229127=CARTESIAN_POINT('Ctrl Pts',(-1.31362451000006,15.2,10.615033579));
#229128=CARTESIAN_POINT('Ctrl Pts',(-1.31362451000006,11.6,10.615033579));
#229129=CARTESIAN_POINT('Ctrl Pts',(-1.31394908200006,15.2,10.612668813));
#229130=CARTESIAN_POINT('Ctrl Pts',(-1.31394908200006,11.6,10.612668813));
#229131=CARTESIAN_POINT('Ctrl Pts',(-1.31427073800006,15.2,10.61031006));
#229132=CARTESIAN_POINT('Ctrl Pts',(-1.31427073800006,11.6,10.61031006));
#229133=CARTESIAN_POINT('Ctrl Pts',(-1.31458948800006,15.2,10.607957333));
#229134=CARTESIAN_POINT('Ctrl Pts',(-1.31458948800006,11.6,10.607957333));
#229135=CARTESIAN_POINT('Ctrl Pts',(-1.31490533800006,15.2,10.605610646));
#229136=CARTESIAN_POINT('Ctrl Pts',(-1.31490533800006,11.6,10.605610646));
#229137=CARTESIAN_POINT('Ctrl Pts',(-1.31521829600006,15.2,10.603270014));
#229138=CARTESIAN_POINT('Ctrl Pts',(-1.31521829600006,11.6,10.603270014));
#229139=CARTESIAN_POINT('Ctrl Pts',(-1.31552837100006,15.2,10.60093545));
#229140=CARTESIAN_POINT('Ctrl Pts',(-1.31552837100006,11.6,10.60093545));
#229141=CARTESIAN_POINT('Ctrl Pts',(-1.31583557200006,15.2,10.598606967));
#229142=CARTESIAN_POINT('Ctrl Pts',(-1.31583557200006,11.6,10.598606967));
#229143=CARTESIAN_POINT('Ctrl Pts',(-1.31613990500006,15.2,10.596284581));
#229144=CARTESIAN_POINT('Ctrl Pts',(-1.31613990500006,11.6,10.596284581));
#229145=CARTESIAN_POINT('Ctrl Pts',(-1.31644137900006,15.2,10.593968305));
#229146=CARTESIAN_POINT('Ctrl Pts',(-1.31644137900006,11.6,10.593968305));
#229147=CARTESIAN_POINT('Ctrl Pts',(-1.31674000300006,15.2,10.591658154));
#229148=CARTESIAN_POINT('Ctrl Pts',(-1.31674000300006,11.6,10.591658154));
#229149=CARTESIAN_POINT('Ctrl Pts',(-1.31703578300006,15.2,10.589354141));
#229150=CARTESIAN_POINT('Ctrl Pts',(-1.31703578300006,11.6,10.589354141));
#229151=CARTESIAN_POINT('Ctrl Pts',(-1.31732873000006,15.2,10.58705628));
#229152=CARTESIAN_POINT('Ctrl Pts',(-1.31732873000006,11.6,10.58705628));
#229153=CARTESIAN_POINT('Ctrl Pts',(-1.31761885100006,15.2,10.584764587));
#229154=CARTESIAN_POINT('Ctrl Pts',(-1.31761885100006,11.6,10.584764587));
#229155=CARTESIAN_POINT('Ctrl Pts',(-1.31790615400006,15.2,10.582479075));
#229156=CARTESIAN_POINT('Ctrl Pts',(-1.31790615400006,11.6,10.582479075));
#229157=CARTESIAN_POINT('Ctrl Pts',(-1.31819064900006,15.2,10.580199759));
#229158=CARTESIAN_POINT('Ctrl Pts',(-1.31819064900006,11.6,10.580199759));
#229159=CARTESIAN_POINT('Ctrl Pts',(-1.31847234300006,15.2,10.577926652));
#229160=CARTESIAN_POINT('Ctrl Pts',(-1.31847234300006,11.6,10.577926652));
#229161=CARTESIAN_POINT('Ctrl Pts',(-1.31875124500006,15.2,10.575659769));
#229162=CARTESIAN_POINT('Ctrl Pts',(-1.31875124500006,11.6,10.575659769));
#229163=CARTESIAN_POINT('Ctrl Pts',(-1.31902736400006,15.2,10.573399125));
#229164=CARTESIAN_POINT('Ctrl Pts',(-1.31902736400006,11.6,10.573399125));
#229165=CARTESIAN_POINT('Ctrl Pts',(-1.31930070600006,15.2,10.571144734));
#229166=CARTESIAN_POINT('Ctrl Pts',(-1.31930070600006,11.6,10.571144734));
#229167=CARTESIAN_POINT('Ctrl Pts',(-1.31957128300005,15.2,10.568896611));
#229168=CARTESIAN_POINT('Ctrl Pts',(-1.31957128300005,11.6,10.568896611));
#229169=CARTESIAN_POINT('Ctrl Pts',(-1.31983910100006,15.2,10.566654769));
#229170=CARTESIAN_POINT('Ctrl Pts',(-1.31983910100006,11.6,10.566654769));
#229171=CARTESIAN_POINT('Ctrl Pts',(-1.32010417000005,15.2,10.564419225));
#229172=CARTESIAN_POINT('Ctrl Pts',(-1.32010417000005,11.6,10.564419225));
#229173=CARTESIAN_POINT('Ctrl Pts',(-1.32036649900006,15.2,10.562189991));
#229174=CARTESIAN_POINT('Ctrl Pts',(-1.32036649900006,11.6,10.562189991));
#229175=CARTESIAN_POINT('Ctrl Pts',(-1.32062609500006,15.2,10.559967083));
#229176=CARTESIAN_POINT('Ctrl Pts',(-1.32062609500006,11.6,10.559967083));
#229177=CARTESIAN_POINT('Ctrl Pts',(-1.32088296800006,15.2,10.557750516));
#229178=CARTESIAN_POINT('Ctrl Pts',(-1.32088296800006,11.6,10.557750516));
#229179=CARTESIAN_POINT('Ctrl Pts',(-1.32113712700006,15.2,10.555540305));
#229180=CARTESIAN_POINT('Ctrl Pts',(-1.32113712700006,11.6,10.555540305));
#229181=CARTESIAN_POINT('Ctrl Pts',(-1.32138858000006,15.2,10.553336463));
#229182=CARTESIAN_POINT('Ctrl Pts',(-1.32138858000006,11.6,10.553336463));
#229183=CARTESIAN_POINT('Ctrl Pts',(-1.32163733600006,15.2,10.551139006));
#229184=CARTESIAN_POINT('Ctrl Pts',(-1.32163733600006,11.6,10.551139006));
#229185=CARTESIAN_POINT('Ctrl Pts',(-1.32188340500006,15.2,10.548947949));
#229186=CARTESIAN_POINT('Ctrl Pts',(-1.32188340500006,11.6,10.548947949));
#229187=CARTESIAN_POINT('Ctrl Pts',(-1.32212679500006,15.2,10.546763307));
#229188=CARTESIAN_POINT('Ctrl Pts',(-1.32212679500006,11.6,10.546763307));
#229189=CARTESIAN_POINT('Ctrl Pts',(-1.32236751400006,15.2,10.544585094));
#229190=CARTESIAN_POINT('Ctrl Pts',(-1.32236751400006,11.6,10.544585094));
#229191=CARTESIAN_POINT('Ctrl Pts',(-1.32260557300006,15.2,10.542413324));
#229192=CARTESIAN_POINT('Ctrl Pts',(-1.32260557300006,11.6,10.542413324));
#229193=CARTESIAN_POINT('Ctrl Pts',(-1.32284098000006,15.2,10.540248015));
#229194=CARTESIAN_POINT('Ctrl Pts',(-1.32284098000006,11.6,10.540248015));
#229195=CARTESIAN_POINT('Ctrl Pts',(-1.32307374400006,15.2,10.538089179));
#229196=CARTESIAN_POINT('Ctrl Pts',(-1.32307374400006,11.6,10.538089179));
#229197=CARTESIAN_POINT('Ctrl Pts',(-1.32330387400006,15.2,10.535936834));
#229198=CARTESIAN_POINT('Ctrl Pts',(-1.32330387400006,11.6,10.535936834));
#229199=CARTESIAN_POINT('Ctrl Pts',(-1.32353137900005,15.2,10.533790993));
#229200=CARTESIAN_POINT('Ctrl Pts',(-1.32353137900005,11.6,10.533790993));
#229201=CARTESIAN_POINT('Ctrl Pts',(-1.32375627000005,15.2,10.531651672));
#229202=CARTESIAN_POINT('Ctrl Pts',(-1.32375627000005,11.6,10.531651672));
#229203=CARTESIAN_POINT('Ctrl Pts',(-1.32397855300006,15.2,10.529518886));
#229204=CARTESIAN_POINT('Ctrl Pts',(-1.32397855300006,11.6,10.529518886));
#229205=CARTESIAN_POINT('Ctrl Pts',(-1.32419824100006,15.2,10.52739265));
#229206=CARTESIAN_POINT('Ctrl Pts',(-1.32419824100006,11.6,10.52739265));
#229207=CARTESIAN_POINT('Ctrl Pts',(-1.32441534000006,15.2,10.52527298));
#229208=CARTESIAN_POINT('Ctrl Pts',(-1.32441534000006,11.6,10.52527298));
#229209=CARTESIAN_POINT('Ctrl Pts',(-1.32462986200006,15.2,10.52315989));
#229210=CARTESIAN_POINT('Ctrl Pts',(-1.32462986200006,11.6,10.52315989));
#229211=CARTESIAN_POINT('Ctrl Pts',(-1.32484181500006,15.2,10.521053397));
#229212=CARTESIAN_POINT('Ctrl Pts',(-1.32484181500006,11.6,10.521053397));
#229213=CARTESIAN_POINT('Ctrl Pts',(-1.32505120800006,15.2,10.518953515));
#229214=CARTESIAN_POINT('Ctrl Pts',(-1.32505120800006,11.6,10.518953515));
#229215=CARTESIAN_POINT('Ctrl Pts',(-1.32525805200006,15.2,10.516860261));
#229216=CARTESIAN_POINT('Ctrl Pts',(-1.32525805200006,11.6,10.516860261));
#229217=CARTESIAN_POINT('Ctrl Pts',(-1.32546235400006,15.2,10.514773649));
#229218=CARTESIAN_POINT('Ctrl Pts',(-1.32546235400006,11.6,10.514773649));
#229219=CARTESIAN_POINT('Ctrl Pts',(-1.32566412700006,15.2,10.512693695));
#229220=CARTESIAN_POINT('Ctrl Pts',(-1.32566412700006,11.6,10.512693695));
#229221=CARTESIAN_POINT('Ctrl Pts',(-1.32586337700006,15.2,10.510620415));
#229222=CARTESIAN_POINT('Ctrl Pts',(-1.32586337700006,11.6,10.510620415));
#229223=CARTESIAN_POINT('Ctrl Pts',(-1.32606011800006,15.2,10.508553824));
#229224=CARTESIAN_POINT('Ctrl Pts',(-1.32606011800006,11.6,10.508553824));
#229225=CARTESIAN_POINT('Ctrl Pts',(-1.32625435500006,15.2,10.506493939));
#229226=CARTESIAN_POINT('Ctrl Pts',(-1.32625435500006,11.6,10.506493939));
#229227=CARTESIAN_POINT('Ctrl Pts',(-1.32644610000006,15.2,10.504440774));
#229228=CARTESIAN_POINT('Ctrl Pts',(-1.32644610000006,11.6,10.504440774));
#229229=CARTESIAN_POINT('Ctrl Pts',(-1.32663536400006,15.2,10.502394347));
#229230=CARTESIAN_POINT('Ctrl Pts',(-1.32663536400006,11.6,10.502394347));
#229231=CARTESIAN_POINT('Ctrl Pts',(-1.32682215400005,15.2,10.500354671));
#229232=CARTESIAN_POINT('Ctrl Pts',(-1.32682215400005,11.6,10.500354671));
#229233=CARTESIAN_POINT('Ctrl Pts',(-1.32700648100006,15.2,10.498321763));
#229234=CARTESIAN_POINT('Ctrl Pts',(-1.32700648100006,11.6,10.498321763));
#229235=CARTESIAN_POINT('Ctrl Pts',(-1.32718835600006,15.2,10.49629564));
#229236=CARTESIAN_POINT('Ctrl Pts',(-1.32718835600006,11.6,10.49629564));
#229237=CARTESIAN_POINT('Ctrl Pts',(-1.32736778800005,15.2,10.494276317));
#229238=CARTESIAN_POINT('Ctrl Pts',(-1.32736778800005,11.6,10.494276317));
#229239=CARTESIAN_POINT('Ctrl Pts',(-1.32754478700006,15.2,10.49226381));
#229240=CARTESIAN_POINT('Ctrl Pts',(-1.32754478700006,11.6,10.49226381));
#229241=CARTESIAN_POINT('Ctrl Pts',(-1.32771936300006,15.2,10.490258135));
#229242=CARTESIAN_POINT('Ctrl Pts',(-1.32771936300006,11.6,10.490258135));
#229243=CARTESIAN_POINT('Ctrl Pts',(-1.32789152600005,15.2,10.488259309));
#229244=CARTESIAN_POINT('Ctrl Pts',(-1.32789152600005,11.6,10.488259309));
#229245=CARTESIAN_POINT('Ctrl Pts',(-1.32806128600006,15.2,10.486267346));
#229246=CARTESIAN_POINT('Ctrl Pts',(-1.32806128600006,11.6,10.486267346));
#229247=CARTESIAN_POINT('Ctrl Pts',(-1.32822865400006,15.2,10.484282264));
#229248=CARTESIAN_POINT('Ctrl Pts',(-1.32822865400006,11.6,10.484282264));
#229249=CARTESIAN_POINT('Ctrl Pts',(-1.32839364000006,15.2,10.48230408));
#229250=CARTESIAN_POINT('Ctrl Pts',(-1.32839364000006,11.6,10.48230408));
#229251=CARTESIAN_POINT('Ctrl Pts',(-1.32855625300005,15.2,10.480332808));
#229252=CARTESIAN_POINT('Ctrl Pts',(-1.32855625300005,11.6,10.480332808));
#229253=CARTESIAN_POINT('Ctrl Pts',(-1.32871650400006,15.2,10.478368466));
#229254=CARTESIAN_POINT('Ctrl Pts',(-1.32871650400006,11.6,10.478368466));
#229255=CARTESIAN_POINT('Ctrl Pts',(-1.32887440300006,15.2,10.47641107));
#229256=CARTESIAN_POINT('Ctrl Pts',(-1.32887440300006,11.6,10.47641107));
#229257=CARTESIAN_POINT('Ctrl Pts',(-1.32902996200006,15.2,10.474460635));
#229258=CARTESIAN_POINT('Ctrl Pts',(-1.32902996200006,11.6,10.474460635));
#229259=CARTESIAN_POINT('Ctrl Pts',(-1.32918319000006,15.2,10.47251718));
#229260=CARTESIAN_POINT('Ctrl Pts',(-1.32918319000006,11.6,10.47251718));
#229261=CARTESIAN_POINT('Ctrl Pts',(-1.32933409700006,15.2,10.47058072));
#229262=CARTESIAN_POINT('Ctrl Pts',(-1.32933409700006,11.6,10.47058072));
#229263=CARTESIAN_POINT('Ctrl Pts',(-1.32948269500006,15.2,10.468651272));
#229264=CARTESIAN_POINT('Ctrl Pts',(-1.32948269500006,11.6,10.468651272));
#229265=CARTESIAN_POINT('Ctrl Pts',(-1.32962899400005,15.2,10.466728852));
#229266=CARTESIAN_POINT('Ctrl Pts',(-1.32962899400005,11.6,10.466728852));
#229267=CARTESIAN_POINT('Ctrl Pts',(-1.32977300300006,15.2,10.464813478));
#229268=CARTESIAN_POINT('Ctrl Pts',(-1.32977300300006,11.6,10.464813478));
#229269=CARTESIAN_POINT('Ctrl Pts',(-1.32991473600006,15.2,10.462905165));
#229270=CARTESIAN_POINT('Ctrl Pts',(-1.32991473600006,11.6,10.462905165));
#229271=CARTESIAN_POINT('Ctrl Pts',(-1.33005420100006,15.2,10.461003931));
#229272=CARTESIAN_POINT('Ctrl Pts',(-1.33005420100006,11.6,10.461003931));
#229273=CARTESIAN_POINT('Ctrl Pts',(-1.33019140900006,15.2,10.459109793));
#229274=CARTESIAN_POINT('Ctrl Pts',(-1.33019140900006,11.6,10.459109793));
#229275=CARTESIAN_POINT('Ctrl Pts',(-1.33032637200006,15.2,10.457222767));
#229276=CARTESIAN_POINT('Ctrl Pts',(-1.33032637200006,11.6,10.457222767));
#229277=CARTESIAN_POINT('Ctrl Pts',(-1.33045910000006,15.2,10.455342871));
#229278=CARTESIAN_POINT('Ctrl Pts',(-1.33045910000006,11.6,10.455342871));
#229279=CARTESIAN_POINT('Ctrl Pts',(-1.33058960300006,15.2,10.453470121));
#229280=CARTESIAN_POINT('Ctrl Pts',(-1.33058960300006,11.6,10.453470121));
#229281=CARTESIAN_POINT('Ctrl Pts',(-1.33071789300006,15.2,10.451604534));
#229282=CARTESIAN_POINT('Ctrl Pts',(-1.33071789300006,11.6,10.451604534));
#229283=CARTESIAN_POINT('Ctrl Pts',(-1.33084398200006,15.2,10.449746128));
#229284=CARTESIAN_POINT('Ctrl Pts',(-1.33084398200006,11.6,10.449746128));
#229285=CARTESIAN_POINT('Ctrl Pts',(-1.33096788000006,15.2,10.447894919));
#229286=CARTESIAN_POINT('Ctrl Pts',(-1.33096788000006,11.6,10.447894919));
#229287=CARTESIAN_POINT('Ctrl Pts',(-1.33108959800005,15.2,10.446050926));
#229288=CARTESIAN_POINT('Ctrl Pts',(-1.33108959800005,11.6,10.446050926));
#229289=CARTESIAN_POINT('Ctrl Pts',(-1.33120914700006,15.2,10.444214164));
#229290=CARTESIAN_POINT('Ctrl Pts',(-1.33120914700006,11.6,10.444214164));
#229291=CARTESIAN_POINT('Ctrl Pts',(-1.33132653900006,15.2,10.442384653));
#229292=CARTESIAN_POINT('Ctrl Pts',(-1.33132653900006,11.6,10.442384653));
#229293=CARTESIAN_POINT('Ctrl Pts',(-1.33144178500006,15.2,10.440562408));
#229294=CARTESIAN_POINT('Ctrl Pts',(-1.33144178500006,11.6,10.440562408));
#229295=CARTESIAN_POINT('Ctrl Pts',(-1.33155489500006,15.2,10.438747447));
#229296=CARTESIAN_POINT('Ctrl Pts',(-1.33155489500006,11.6,10.438747447));
#229297=CARTESIAN_POINT('Ctrl Pts',(-1.33166588100006,15.2,10.436939787));
#229298=CARTESIAN_POINT('Ctrl Pts',(-1.33166588100006,11.6,10.436939787));
#229299=CARTESIAN_POINT('Ctrl Pts',(-1.33177475500006,15.2,10.435139449));
#229300=CARTESIAN_POINT('Ctrl Pts',(-1.33177475500006,11.6,10.435139449));
#229301=CARTESIAN_POINT('Ctrl Pts',(-1.33188152900006,15.2,10.433346446));
#229302=CARTESIAN_POINT('Ctrl Pts',(-1.33188152900006,11.6,10.433346446));
#229303=CARTESIAN_POINT('Ctrl Pts',(-1.33198621300005,15.2,10.431560798));
#229304=CARTESIAN_POINT('Ctrl Pts',(-1.33198621300005,11.6,10.431560798));
#229305=CARTESIAN_POINT('Ctrl Pts',(-1.33208882000006,15.2,10.429782522));
#229306=CARTESIAN_POINT('Ctrl Pts',(-1.33208882000006,11.6,10.429782522));
#229307=CARTESIAN_POINT('Ctrl Pts',(-1.33218935900006,15.2,10.428011636));
#229308=CARTESIAN_POINT('Ctrl Pts',(-1.33218935900006,11.6,10.428011636));
#229309=CARTESIAN_POINT('Ctrl Pts',(-1.33228784600006,15.2,10.426248158));
#229310=CARTESIAN_POINT('Ctrl Pts',(-1.33228784600006,11.6,10.426248158));
#229311=CARTESIAN_POINT('Ctrl Pts',(-1.33238428800006,15.2,10.424492106));
#229312=CARTESIAN_POINT('Ctrl Pts',(-1.33238428800006,11.6,10.424492106));
#229313=CARTESIAN_POINT('Ctrl Pts',(-1.33247870000006,15.2,10.422743498));
#229314=CARTESIAN_POINT('Ctrl Pts',(-1.33247870000006,11.6,10.422743498));
#229315=CARTESIAN_POINT('Ctrl Pts',(-1.33257109300006,15.2,10.421002351));
#229316=CARTESIAN_POINT('Ctrl Pts',(-1.33257109300006,11.6,10.421002351));
#229317=CARTESIAN_POINT('Ctrl Pts',(-1.33266147800006,15.2,10.419268684));
#229318=CARTESIAN_POINT('Ctrl Pts',(-1.33266147800006,11.6,10.419268684));
#229319=CARTESIAN_POINT('Ctrl Pts',(-1.33274986800005,15.2,10.417542516));
#229320=CARTESIAN_POINT('Ctrl Pts',(-1.33274986800005,11.6,10.417542516));
#229321=CARTESIAN_POINT('Ctrl Pts',(-1.33283627400006,15.2,10.415823863));
#229322=CARTESIAN_POINT('Ctrl Pts',(-1.33283627400006,11.6,10.415823863));
#229323=CARTESIAN_POINT('Ctrl Pts',(-1.33292070900006,15.2,10.414112744));
#229324=CARTESIAN_POINT('Ctrl Pts',(-1.33292070900006,11.6,10.414112744));
#229325=CARTESIAN_POINT('Ctrl Pts',(-1.33300318500006,15.2,10.412409178));
#229326=CARTESIAN_POINT('Ctrl Pts',(-1.33300318500006,11.6,10.412409178));
#229327=CARTESIAN_POINT('Ctrl Pts',(-1.33308371300006,15.2,10.410713184));
#229328=CARTESIAN_POINT('Ctrl Pts',(-1.33308371300006,11.6,10.410713184));
#229329=CARTESIAN_POINT('Ctrl Pts',(-1.33316230700006,15.2,10.409024779));
#229330=CARTESIAN_POINT('Ctrl Pts',(-1.33316230700006,11.6,10.409024779));
#229331=CARTESIAN_POINT('Ctrl Pts',(-1.33323897800006,15.2,10.407343981));
#229332=CARTESIAN_POINT('Ctrl Pts',(-1.33323897800006,11.6,10.407343981));
#229333=CARTESIAN_POINT('Ctrl Pts',(-1.33331373800006,15.2,10.40567081));
#229334=CARTESIAN_POINT('Ctrl Pts',(-1.33331373800006,11.6,10.40567081));
#229335=CARTESIAN_POINT('Ctrl Pts',(-1.33338660000006,15.2,10.404005284));
#229336=CARTESIAN_POINT('Ctrl Pts',(-1.33338660000006,11.6,10.404005284));
#229337=CARTESIAN_POINT('Ctrl Pts',(-1.33345757800006,15.2,10.402347423));
#229338=CARTESIAN_POINT('Ctrl Pts',(-1.33345757800006,11.6,10.402347423));
#229339=CARTESIAN_POINT('Ctrl Pts',(-1.33352668100006,15.2,10.400697244));
#229340=CARTESIAN_POINT('Ctrl Pts',(-1.33352668100006,11.6,10.400697244));
#229341=CARTESIAN_POINT('Ctrl Pts',(-1.33359392500006,15.2,10.399054765));
#229342=CARTESIAN_POINT('Ctrl Pts',(-1.33359392500006,11.6,10.399054765));
#229343=CARTESIAN_POINT('Ctrl Pts',(-1.33365932000006,15.2,10.397420008));
#229344=CARTESIAN_POINT('Ctrl Pts',(-1.33365932000006,11.6,10.397420008));
#229345=CARTESIAN_POINT('Ctrl Pts',(-1.33372288000006,15.2,10.39579299));
#229346=CARTESIAN_POINT('Ctrl Pts',(-1.33372288000006,11.6,10.39579299));
#229347=CARTESIAN_POINT('Ctrl Pts',(-1.33378461800006,15.2,10.39417373));
#229348=CARTESIAN_POINT('Ctrl Pts',(-1.33378461800006,11.6,10.39417373));
#229349=CARTESIAN_POINT('Ctrl Pts',(-1.33384454600006,15.2,10.392562247));
#229350=CARTESIAN_POINT('Ctrl Pts',(-1.33384454600006,11.6,10.392562247));
#229351=CARTESIAN_POINT('Ctrl Pts',(-1.33390267700006,15.2,10.390958561));
#229352=CARTESIAN_POINT('Ctrl Pts',(-1.33390267700006,11.6,10.390958561));
#229353=CARTESIAN_POINT('Ctrl Pts',(-1.33395902400006,15.2,10.38936269));
#229354=CARTESIAN_POINT('Ctrl Pts',(-1.33395902400006,11.6,10.38936269));
#229355=CARTESIAN_POINT('Ctrl Pts',(-1.33401360000006,15.2,10.387774655));
#229356=CARTESIAN_POINT('Ctrl Pts',(-1.33401360000006,11.6,10.387774655));
#229357=CARTESIAN_POINT('Ctrl Pts',(-1.33406641900006,15.2,10.386194473));
#229358=CARTESIAN_POINT('Ctrl Pts',(-1.33406641900006,11.6,10.386194473));
#229359=CARTESIAN_POINT('Ctrl Pts',(-1.33411749200006,15.2,10.384622166));
#229360=CARTESIAN_POINT('Ctrl Pts',(-1.33411749200006,11.6,10.384622166));
#229361=CARTESIAN_POINT('Ctrl Pts',(-1.33416683400006,15.2,10.383057751));
#229362=CARTESIAN_POINT('Ctrl Pts',(-1.33416683400006,11.6,10.383057751));
#229363=CARTESIAN_POINT('Ctrl Pts',(-1.33421445700006,15.2,10.381501249));
#229364=CARTESIAN_POINT('Ctrl Pts',(-1.33421445700006,11.6,10.381501249));
#229365=CARTESIAN_POINT('Ctrl Pts',(-1.33426037600006,15.2,10.37995268));
#229366=CARTESIAN_POINT('Ctrl Pts',(-1.33426037600006,11.6,10.37995268));
#229367=CARTESIAN_POINT('Ctrl Pts',(-1.33430460300006,15.2,10.378412062));
#229368=CARTESIAN_POINT('Ctrl Pts',(-1.33430460300006,11.6,10.378412062));
#229369=CARTESIAN_POINT('Ctrl Pts',(-1.33434715000006,15.2,10.376879417));
#229370=CARTESIAN_POINT('Ctrl Pts',(-1.33434715000006,11.6,10.376879417));
#229371=CARTESIAN_POINT('Ctrl Pts',(-1.33438803300006,15.2,10.375354763));
#229372=CARTESIAN_POINT('Ctrl Pts',(-1.33438803300006,11.6,10.375354763));
#229373=CARTESIAN_POINT('Ctrl Pts',(-1.33442726500006,15.2,10.373838121));
#229374=CARTESIAN_POINT('Ctrl Pts',(-1.33442726500006,11.6,10.373838121));
#229375=CARTESIAN_POINT('Ctrl Pts',(-1.33446485900006,15.2,10.37232951));
#229376=CARTESIAN_POINT('Ctrl Pts',(-1.33446485900006,11.6,10.37232951));
#229377=CARTESIAN_POINT('Ctrl Pts',(-1.33450082900006,15.2,10.370828952));
#229378=CARTESIAN_POINT('Ctrl Pts',(-1.33450082900006,11.6,10.370828952));
#229379=CARTESIAN_POINT('Ctrl Pts',(-1.33453518800006,15.2,10.369336464));
#229380=CARTESIAN_POINT('Ctrl Pts',(-1.33453518800006,11.6,10.369336464));
#229381=CARTESIAN_POINT('Ctrl Pts',(-1.33456795200006,15.2,10.367852069));
#229382=CARTESIAN_POINT('Ctrl Pts',(-1.33456795200006,11.6,10.367852069));
#229383=CARTESIAN_POINT('Ctrl Pts',(-1.33459913200006,15.2,10.366375787));
#229384=CARTESIAN_POINT('Ctrl Pts',(-1.33459913200006,11.6,10.366375787));
#229385=CARTESIAN_POINT('Ctrl Pts',(-1.33462874400006,15.2,10.364907636));
#229386=CARTESIAN_POINT('Ctrl Pts',(-1.33462874400006,11.6,10.364907636));
#229387=CARTESIAN_POINT('Ctrl Pts',(-1.33465680200006,15.2,10.36344764));
#229388=CARTESIAN_POINT('Ctrl Pts',(-1.33465680200006,11.6,10.36344764));
#229389=CARTESIAN_POINT('Ctrl Pts',(-1.33468331800006,15.2,10.361995816));
#229390=CARTESIAN_POINT('Ctrl Pts',(-1.33468331800006,11.6,10.361995816));
#229391=CARTESIAN_POINT('Ctrl Pts',(-1.33470830800006,15.2,10.360552186));
#229392=CARTESIAN_POINT('Ctrl Pts',(-1.33470830800006,11.6,10.360552186));
#229393=CARTESIAN_POINT('Ctrl Pts',(-1.33473178600006,15.2,10.359116772));
#229394=CARTESIAN_POINT('Ctrl Pts',(-1.33473178600006,11.6,10.359116772));
#229395=CARTESIAN_POINT('Ctrl Pts',(-1.33475376600006,15.2,10.357689593));
#229396=CARTESIAN_POINT('Ctrl Pts',(-1.33475376600006,11.6,10.357689593));
#229397=CARTESIAN_POINT('Ctrl Pts',(-1.33477426300006,15.2,10.35627067));
#229398=CARTESIAN_POINT('Ctrl Pts',(-1.33477426300006,11.6,10.35627067));
#229399=CARTESIAN_POINT('Ctrl Pts',(-1.33479329000005,15.2,10.354860025));
#229400=CARTESIAN_POINT('Ctrl Pts',(-1.33479329000005,11.6,10.354860025));
#229401=CARTESIAN_POINT('Ctrl Pts',(-1.33481086200006,15.2,10.353457679));
#229402=CARTESIAN_POINT('Ctrl Pts',(-1.33481086200006,11.6,10.353457679));
#229403=CARTESIAN_POINT('Ctrl Pts',(-1.33482699600005,15.2,10.352063651));
#229404=CARTESIAN_POINT('Ctrl Pts',(-1.33482699600005,11.6,10.352063651));
#229405=CARTESIAN_POINT('Ctrl Pts',(-1.33484170300005,15.2,10.350677965));
#229406=CARTESIAN_POINT('Ctrl Pts',(-1.33484170300005,11.6,10.350677965));
#229407=CARTESIAN_POINT('Ctrl Pts',(-1.33485499900006,15.2,10.34930064));
#229408=CARTESIAN_POINT('Ctrl Pts',(-1.33485499900006,11.6,10.34930064));
#229409=CARTESIAN_POINT('Ctrl Pts',(-1.33486690000006,15.2,10.347931698));
#229410=CARTESIAN_POINT('Ctrl Pts',(-1.33486690000006,11.6,10.347931698));
#229411=CARTESIAN_POINT('Ctrl Pts',(-1.33487742000006,15.2,10.34657116));
#229412=CARTESIAN_POINT('Ctrl Pts',(-1.33487742000006,11.6,10.34657116));
#229413=CARTESIAN_POINT('Ctrl Pts',(-1.33488657400005,15.2,10.345219048));
#229414=CARTESIAN_POINT('Ctrl Pts',(-1.33488657400005,11.6,10.345219048));
#229415=CARTESIAN_POINT('Ctrl Pts',(-1.33489437700006,15.2,10.343875385));
#229416=CARTESIAN_POINT('Ctrl Pts',(-1.33489437700006,11.6,10.343875385));
#229417=CARTESIAN_POINT('Ctrl Pts',(-1.33490084400006,15.2,10.34254019));
#229418=CARTESIAN_POINT('Ctrl Pts',(-1.33490084400006,11.6,10.34254019));
#229419=CARTESIAN_POINT('Ctrl Pts',(-1.33490598900006,15.2,10.341213486));
#229420=CARTESIAN_POINT('Ctrl Pts',(-1.33490598900006,11.6,10.341213486));
#229421=CARTESIAN_POINT('Ctrl Pts',(-1.33490983000006,15.2,10.339895295));
#229422=CARTESIAN_POINT('Ctrl Pts',(-1.33490983000006,11.6,10.339895295));
#229423=CARTESIAN_POINT('Ctrl Pts',(-1.33491238100006,15.2,10.338585638));
#229424=CARTESIAN_POINT('Ctrl Pts',(-1.33491238100006,11.6,10.338585638));
#229425=CARTESIAN_POINT('Ctrl Pts',(-1.33491365600006,15.2,10.337284538));
#229426=CARTESIAN_POINT('Ctrl Pts',(-1.33491365600006,11.6,10.337284538));
#229427=CARTESIAN_POINT('Ctrl Pts',(-1.33491367300006,15.2,10.335992017));
#229428=CARTESIAN_POINT('Ctrl Pts',(-1.33491367300006,11.6,10.335992017));
#229429=CARTESIAN_POINT('Ctrl Pts',(-1.33491244700006,15.2,10.334708096));
#229430=CARTESIAN_POINT('Ctrl Pts',(-1.33491244700006,11.6,10.334708096));
#229431=CARTESIAN_POINT('Ctrl Pts',(-1.33490999100006,15.2,10.333432799));
#229432=CARTESIAN_POINT('Ctrl Pts',(-1.33490999100006,11.6,10.333432799));
#229433=CARTESIAN_POINT('Ctrl Pts',(-1.33490632300005,15.2,10.332166147));
#229434=CARTESIAN_POINT('Ctrl Pts',(-1.33490632300005,11.6,10.332166147));
#229435=CARTESIAN_POINT('Ctrl Pts',(-1.33490146100006,15.2,10.330908164));
#229436=CARTESIAN_POINT('Ctrl Pts',(-1.33490146100006,11.6,10.330908164));
#229437=CARTESIAN_POINT('Ctrl Pts',(-1.33489541600005,15.2,10.329658871));
#229438=CARTESIAN_POINT('Ctrl Pts',(-1.33489541600005,11.6,10.329658871));
#229439=CARTESIAN_POINT('Ctrl Pts',(-1.33488820600006,15.2,10.32841829));
#229440=CARTESIAN_POINT('Ctrl Pts',(-1.33488820600006,11.6,10.32841829));
#229441=CARTESIAN_POINT('Ctrl Pts',(-1.33487984900006,15.2,10.327186446));
#229442=CARTESIAN_POINT('Ctrl Pts',(-1.33487984900006,11.6,10.327186446));
#229443=CARTESIAN_POINT('Ctrl Pts',(-1.33487035900006,15.2,10.325963361));
#229444=CARTESIAN_POINT('Ctrl Pts',(-1.33487035900006,11.6,10.325963361));
#229445=CARTESIAN_POINT('Ctrl Pts',(-1.33485975300006,15.2,10.324749057));
#229446=CARTESIAN_POINT('Ctrl Pts',(-1.33485975300006,11.6,10.324749057));
#229447=CARTESIAN_POINT('Ctrl Pts',(-1.33484804700006,15.2,10.323543557));
#229448=CARTESIAN_POINT('Ctrl Pts',(-1.33484804700006,11.6,10.323543557));
#229449=CARTESIAN_POINT('Ctrl Pts',(-1.33483525700006,15.2,10.322346887));
#229450=CARTESIAN_POINT('Ctrl Pts',(-1.33483525700006,11.6,10.322346887));
#229451=CARTESIAN_POINT('Ctrl Pts',(-1.33482140000006,15.2,10.321159066));
#229452=CARTESIAN_POINT('Ctrl Pts',(-1.33482140000006,11.6,10.321159066));
#229453=CARTESIAN_POINT('Ctrl Pts',(-1.33480649300005,15.2,10.31998012));
#229454=CARTESIAN_POINT('Ctrl Pts',(-1.33480649300005,11.6,10.31998012));
#229455=CARTESIAN_POINT('Ctrl Pts',(-1.33479055200006,15.2,10.31881007));
#229456=CARTESIAN_POINT('Ctrl Pts',(-1.33479055200006,11.6,10.31881007));
#229457=CARTESIAN_POINT('Ctrl Pts',(-1.33477359500006,15.2,10.317648944));
#229458=CARTESIAN_POINT('Ctrl Pts',(-1.33477359500006,11.6,10.317648944));
#229459=CARTESIAN_POINT('Ctrl Pts',(-1.33475563700006,15.2,10.31649676));
#229460=CARTESIAN_POINT('Ctrl Pts',(-1.33475563700006,11.6,10.31649676));
#229461=CARTESIAN_POINT('Ctrl Pts',(-1.33473669500005,15.2,10.315353546));
#229462=CARTESIAN_POINT('Ctrl Pts',(-1.33473669500005,11.6,10.315353546));
#229463=CARTESIAN_POINT('Ctrl Pts',(-1.33471678800006,15.2,10.314219324));
#229464=CARTESIAN_POINT('Ctrl Pts',(-1.33471678800006,11.6,10.314219324));
#229465=CARTESIAN_POINT('Ctrl Pts',(-1.33469593100006,15.2,10.313094118));
#229466=CARTESIAN_POINT('Ctrl Pts',(-1.33469593100006,11.6,10.313094118));
#229467=CARTESIAN_POINT('Ctrl Pts',(-1.33467414200006,15.2,10.311977953));
#229468=CARTESIAN_POINT('Ctrl Pts',(-1.33467414200006,11.6,10.311977953));
#229469=CARTESIAN_POINT('Ctrl Pts',(-1.33465143900006,15.2,10.310870851));
#229470=CARTESIAN_POINT('Ctrl Pts',(-1.33465143900006,11.6,10.310870851));
#229471=CARTESIAN_POINT('Ctrl Pts',(-1.33462783800006,15.2,10.309772838));
#229472=CARTESIAN_POINT('Ctrl Pts',(-1.33462783800006,11.6,10.309772838));
#229473=CARTESIAN_POINT('Ctrl Pts',(-1.33460335700006,15.2,10.308683939));
#229474=CARTESIAN_POINT('Ctrl Pts',(-1.33460335700006,11.6,10.308683939));
#229475=CARTESIAN_POINT('Ctrl Pts',(-1.33457801400006,15.2,10.307604176));
#229476=CARTESIAN_POINT('Ctrl Pts',(-1.33457801400006,11.6,10.307604176));
#229477=CARTESIAN_POINT('Ctrl Pts',(-1.33455182600006,15.2,10.306533574));
#229478=CARTESIAN_POINT('Ctrl Pts',(-1.33455182600006,11.6,10.306533574));
#229479=CARTESIAN_POINT('Ctrl Pts',(-1.33452481200006,15.2,10.30547216));
#229480=CARTESIAN_POINT('Ctrl Pts',(-1.33452481200006,11.6,10.30547216));
#229481=CARTESIAN_POINT('Ctrl Pts',(-1.33449698900006,15.2,10.304419957));
#229482=CARTESIAN_POINT('Ctrl Pts',(-1.33449698900006,11.6,10.304419957));
#229483=CARTESIAN_POINT('Ctrl Pts',(-1.33446837400006,15.2,10.30337699));
#229484=CARTESIAN_POINT('Ctrl Pts',(-1.33446837400006,11.6,10.30337699));
#229485=CARTESIAN_POINT('Ctrl Pts',(-1.33443898700006,15.2,10.302343284));
#229486=CARTESIAN_POINT('Ctrl Pts',(-1.33443898700006,11.6,10.302343284));
#229487=CARTESIAN_POINT('Ctrl Pts',(-1.33440884500006,15.2,10.301318864));
#229488=CARTESIAN_POINT('Ctrl Pts',(-1.33440884500006,11.6,10.301318864));
#229489=CARTESIAN_POINT('Ctrl Pts',(-1.33437796600006,15.2,10.300303756));
#229490=CARTESIAN_POINT('Ctrl Pts',(-1.33437796600006,11.6,10.300303756));
#229491=CARTESIAN_POINT('Ctrl Pts',(-1.33434636900006,15.2,10.299297985));
#229492=CARTESIAN_POINT('Ctrl Pts',(-1.33434636900006,11.6,10.299297985));
#229493=CARTESIAN_POINT('Ctrl Pts',(-1.33431407200006,15.2,10.298301576));
#229494=CARTESIAN_POINT('Ctrl Pts',(-1.33431407200006,11.6,10.298301576));
#229495=CARTESIAN_POINT('Ctrl Pts',(-1.33428109400006,15.2,10.297314554));
#229496=CARTESIAN_POINT('Ctrl Pts',(-1.33428109400006,11.6,10.297314554));
#229497=CARTESIAN_POINT('Ctrl Pts',(-1.33424745300006,15.2,10.296336947));
#229498=CARTESIAN_POINT('Ctrl Pts',(-1.33424745300006,11.6,10.296336947));
#229499=CARTESIAN_POINT('Ctrl Pts',(-1.33421316800006,15.2,10.295368779));
#229500=CARTESIAN_POINT('Ctrl Pts',(-1.33421316800006,11.6,10.295368779));
#229501=CARTESIAN_POINT('Ctrl Pts',(-1.33417825800006,15.2,10.294410074));
#229502=CARTESIAN_POINT('Ctrl Pts',(-1.33417825800006,11.6,10.294410074));
#229503=CARTESIAN_POINT('Ctrl Pts',(-1.33414274300006,15.2,10.293460863));
#229504=CARTESIAN_POINT('Ctrl Pts',(-1.33414274300006,11.6,10.293460863));
#229505=CARTESIAN_POINT('Ctrl Pts',(-1.33410664000006,15.2,10.292521168));
#229506=CARTESIAN_POINT('Ctrl Pts',(-1.33410664000006,11.6,10.292521168));
#229507=CARTESIAN_POINT('Ctrl Pts',(-1.33406997000006,15.2,10.291591016));
#229508=CARTESIAN_POINT('Ctrl Pts',(-1.33406997000006,11.6,10.291591016));
#229509=CARTESIAN_POINT('Ctrl Pts',(-1.33403296600005,15.2,10.290675737));
#229510=CARTESIAN_POINT('Ctrl Pts',(-1.33403296600005,11.6,10.290675737));
#229511=CARTESIAN_POINT('Ctrl Pts',(-1.33400298800006,15.2,10.289952142));
#229512=CARTESIAN_POINT('Ctrl Pts',(-1.33400298800006,11.6,10.289952142));
#229513=CARTESIAN_POINT('Ctrl Pts',(-1.33398033300006,15.2,10.289415004));
#229514=CARTESIAN_POINT('Ctrl Pts',(-1.33398033300006,11.6,10.289415004));
#229515=CARTESIAN_POINT('Ctrl Pts',(-1.33396520800006,15.2,10.289060521));
#229516=CARTESIAN_POINT('Ctrl Pts',(-1.33396520800006,11.6,10.289060521));
#229517=CARTESIAN_POINT('Ctrl Pts',(-1.33395773200006,15.2,10.288886324));
#229518=CARTESIAN_POINT('Ctrl Pts',(-1.33395773200006,11.6,10.288886324));
#229519=CARTESIAN_POINT('',(-1.33395773266456,12.2,10.2888863233166));
#229520=CARTESIAN_POINT('',(-1.33395773266456,15.2,10.2888863233166));
#229521=CARTESIAN_POINT('',(-1.33395773300006,12.2,10.288886323));
#229522=CARTESIAN_POINT('Ctrl Pts',(-1.09337743000006,12.2,11.447904865));
#229523=CARTESIAN_POINT('Ctrl Pts',(-1.09471863524371,12.2,11.4443249343496));
#229524=CARTESIAN_POINT('Ctrl Pts',(-1.09605347736072,12.2,11.4407496840126));
#229525=CARTESIAN_POINT('Ctrl Pts',(-1.09738195536205,12.2,11.4371791166813));
#229526=CARTESIAN_POINT('Ctrl Pts',(-1.09871043336338,12.2,11.43360854935));
#229527=CARTESIAN_POINT('Ctrl Pts',(-1.10003254799348,12.2,11.4300426621214));
#229528=CARTESIAN_POINT('Ctrl Pts',(-1.10134830322047,12.2,11.4264814746557));
#229529=CARTESIAN_POINT('Ctrl Pts',(-1.10266405844746,12.2,11.42292028719));
#229530=CARTESIAN_POINT('Ctrl Pts',(-1.10397345477917,12.2,11.4193638002458));
#229531=CARTESIAN_POINT('Ctrl Pts',(-1.10527650644103,12.2,11.4158120532492));
#229532=CARTESIAN_POINT('Ctrl Pts',(-1.10657955833961,12.2,11.4122603056074));
#229533=CARTESIAN_POINT('Ctrl Pts',(-1.10787626509472,12.2,11.4087132999919));
#229534=CARTESIAN_POINT('Ctrl Pts',(-1.10916664207306,12.2,11.4051710832278));
#229535=CARTESIAN_POINT('Ctrl Pts',(-1.11088714432015,12.2,11.4004481286147));
#229536=CARTESIAN_POINT('Ctrl Pts',(-1.11259639519372,12.2,11.3957336875256));
#229537=CARTESIAN_POINT('Ctrl Pts',(-1.11429442261118,12.2,11.3910278474097));
#229538=CARTESIAN_POINT('Ctrl Pts',(-1.11556794323211,12.2,11.3874984671626));
#229539=CARTESIAN_POINT('Ctrl Pts',(-1.11683515007152,12.2,11.3839739234628));
#229540=CARTESIAN_POINT('Ctrl Pts',(-1.11809605629775,12.2,11.3804542531643));
#229541=CARTESIAN_POINT('Ctrl Pts',(-1.11935696252398,12.2,11.3769345828658));
#229542=CARTESIAN_POINT('Ctrl Pts',(-1.12061156728913,12.2,11.3734197868882));
#229543=CARTESIAN_POINT('Ctrl Pts',(-1.12185988495296,12.2,11.3699099047651));
#229544=CARTESIAN_POINT('Ctrl Pts',(-1.12310820284356,12.2,11.3664000220044));
#229545=CARTESIAN_POINT('Ctrl Pts',(-1.12435023265742,12.2,11.3628950530783));
#229546=CARTESIAN_POINT('Ctrl Pts',(-1.12558598954449,12.2,11.3593950391953));
#229547=CARTESIAN_POINT('Ctrl Pts',(-1.12682174620705,12.2,11.3558950259482));
#229548=CARTESIAN_POINT('Ctrl Pts',(-1.12805122942831,12.2,11.3523999661257));
#229549=CARTESIAN_POINT('Ctrl Pts',(-1.12927445163333,12.2,11.3489098994196));
#229550=CARTESIAN_POINT('Ctrl Pts',(-1.13049767383834,12.2,11.3454198327135));
#229551=CARTESIAN_POINT('Ctrl Pts',(-1.13171463505637,12.2,11.3419347586528));
#229552=CARTESIAN_POINT('Ctrl Pts',(-1.13292534976787,12.2,11.3384547165134));
#229553=CARTESIAN_POINT('Ctrl Pts',(-1.13413606447937,12.2,11.3349746743741));
#229554=CARTESIAN_POINT('Ctrl Pts',(-1.1353405325204,12.2,11.3314996633428));
#229555=CARTESIAN_POINT('Ctrl Pts',(-1.13653876723234,12.2,11.3280297247031));
#229556=CARTESIAN_POINT('Ctrl Pts',(-1.13773700194428,12.2,11.3245597860634));
#229557=CARTESIAN_POINT('Ctrl Pts',(-1.13892900324662,12.2,11.3210949200852));
#229558=CARTESIAN_POINT('Ctrl Pts',(-1.14011478637075,12.2,11.3176351649188));
#229559=CARTESIAN_POINT('Ctrl Pts',(-1.14130056949487,12.2,11.3141754097524));
#229560=CARTESIAN_POINT('Ctrl Pts',(-1.14248013280275,12.2,11.310720765394));
#229561=CARTESIAN_POINT('Ctrl Pts',(-1.14365349151097,12.2,11.3072712732686));
#229562=CARTESIAN_POINT('Ctrl Pts',(-1.14482685043236,12.2,11.3038217805165));
#229563=CARTESIAN_POINT('Ctrl Pts',(-1.14599400426863,12.2,11.300377439266));
#229564=CARTESIAN_POINT('Ctrl Pts',(-1.14715496772818,12.2,11.2969382899336));
#229565=CARTESIAN_POINT('Ctrl Pts',(-1.14831593097682,12.2,11.2934991412259));
#229566=CARTESIAN_POINT('Ctrl Pts',(-1.14947070470733,12.2,11.2900651829661));
#229567=CARTESIAN_POINT('Ctrl Pts',(-1.15061930151393,12.2,11.2866364571283));
#229568=CARTESIAN_POINT('Ctrl Pts',(-1.15176789832052,12.2,11.2832077312905));
#229569=CARTESIAN_POINT('Ctrl Pts',(-1.152910318299,12.2,11.2797842377195));
#229570=CARTESIAN_POINT('Ctrl Pts',(-1.15404657759052,12.2,11.2763660165941));
#229571=CARTESIAN_POINT('Ctrl Pts',(-1.15518283688203,12.2,11.2729477954687));
#229572=CARTESIAN_POINT('Ctrl Pts',(-1.15631293565759,12.2,11.2695348466262));
#229573=CARTESIAN_POINT('Ctrl Pts',(-1.1574368869501,12.2,11.2661272104999));
#229574=CARTESIAN_POINT('Ctrl Pts',(-1.15856083824261,12.2,11.2627195743737));
#229575=CARTESIAN_POINT('Ctrl Pts',(-1.15967864308535,12.2,11.2593172514973));
#229576=CARTESIAN_POINT('Ctrl Pts',(-1.16079031633716,12.2,11.255920282412));
#229577=CARTESIAN_POINT('Ctrl Pts',(-1.16190198958896,12.2,11.2525233133266));
#229578=CARTESIAN_POINT('Ctrl Pts',(-1.16300753226618,12.2,11.2491316985492));
#229579=CARTESIAN_POINT('Ctrl Pts',(-1.16410695806042,12.2,11.2457454779631));
#229580=CARTESIAN_POINT('Ctrl Pts',(-1.16520638405438,12.2,11.2423592567619));
#229581=CARTESIAN_POINT('Ctrl Pts',(-1.16629969447993,12.2,11.2389784305706));
#229582=CARTESIAN_POINT('Ctrl Pts',(-1.16738690347044,12.2,11.2356030408308));
#229583=CARTESIAN_POINT('Ctrl Pts',(-1.16847411226344,12.2,11.2322276517042));
#229584=CARTESIAN_POINT('Ctrl Pts',(-1.16955522016075,12.2,11.2288576985443));
#229585=CARTESIAN_POINT('Ctrl Pts',(-1.17063024296636,12.2,11.2254932223324));
#229586=CARTESIAN_POINT('Ctrl Pts',(-1.17170526577197,12.2,11.2221287461205));
#229587=CARTESIAN_POINT('Ctrl Pts',(-1.172774202805,12.2,11.2187697477455));
#229588=CARTESIAN_POINT('Ctrl Pts',(-1.17383707105751,12.2,11.2154162686179));
#229589=CARTESIAN_POINT('Ctrl Pts',(-1.17489993931003,12.2,11.2120627894902));
#229590=CARTESIAN_POINT('Ctrl Pts',(-1.17595673878829,12.2,11.2087148287951));
#229591=CARTESIAN_POINT('Ctrl Pts',(-1.1770074840001,12.2,11.2053724292083));
#229592=CARTESIAN_POINT('Ctrl Pts',(-1.17805822921191,12.2,11.2020300296214));
#229593=CARTESIAN_POINT('Ctrl Pts',(-1.17910291997399,12.2,11.1986931913926));
#229594=CARTESIAN_POINT('Ctrl Pts',(-1.18014157464512,12.2,11.1953619553465));
#229595=CARTESIAN_POINT('Ctrl Pts',(-1.18118022931625,12.2,11.1920307193003));
#229596=CARTESIAN_POINT('Ctrl Pts',(-1.18221284635339,12.2,11.1887050868382));
#229597=CARTESIAN_POINT('Ctrl Pts',(-1.18323944307642,12.2,11.1853850986257));
#229598=CARTESIAN_POINT('Ctrl Pts',(-1.18426603979944,12.2,11.1820651104131));
#229599=CARTESIAN_POINT('Ctrl Pts',(-1.18528661428163,12.2,11.1787507677518));
#229600=CARTESIAN_POINT('Ctrl Pts',(-1.18630118503725,12.2,11.1754421117046));
#229601=CARTESIAN_POINT('Ctrl Pts',(-1.18731575597719,12.2,11.1721334550563));
#229602=CARTESIAN_POINT('Ctrl Pts',(-1.18832432250709,12.2,11.1688304856929));
#229603=CARTESIAN_POINT('Ctrl Pts',(-1.18932690144366,12.2,11.1655332465062));
#229604=CARTESIAN_POINT('Ctrl Pts',(-1.19066367305552,12.2,11.1611369285888));
#229605=CARTESIAN_POINT('Ctrl Pts',(-1.19198979991875,12.2,11.1567507967868));
#229606=CARTESIAN_POINT('Ctrl Pts',(-1.19330532220079,12.2,11.1523749528661));
#229607=CARTESIAN_POINT('Ctrl Pts',(-1.19429196395713,12.2,11.1490930697765));
#229608=CARTESIAN_POINT('Ctrl Pts',(-1.19527263971414,12.2,11.1458169740446));
#229609=CARTESIAN_POINT('Ctrl Pts',(-1.19624736856145,12.2,11.1425467073744));
#229610=CARTESIAN_POINT('Ctrl Pts',(-1.19722209740877,12.2,11.1392764407041));
#229611=CARTESIAN_POINT('Ctrl Pts',(-1.1981908789577,12.2,11.136012004776));
#229612=CARTESIAN_POINT('Ctrl Pts',(-1.19915372929852,12.2,11.1327534416853));
#229613=CARTESIAN_POINT('Ctrl Pts',(-1.20011657981426,12.2,11.1294948780026));
#229614=CARTESIAN_POINT('Ctrl Pts',(-1.20107350023667,12.2,11.1262421870632));
#229615=CARTESIAN_POINT('Ctrl Pts',(-1.2020245077074,12.2,11.1229954133005));
#229616=CARTESIAN_POINT('Ctrl Pts',(-1.20297551500537,12.2,11.1197486401276));
#229617=CARTESIAN_POINT('Ctrl Pts',(-1.20392060930367,12.2,11.1165077822794));
#229618=CARTESIAN_POINT('Ctrl Pts',(-1.20485980860238,12.2,11.1132728861474));
#229619=CARTESIAN_POINT('Ctrl Pts',(-1.20579900790108,12.2,11.1100379900154));
#229620=CARTESIAN_POINT('Ctrl Pts',(-1.20673231228045,12.2,11.1068090546445));
#229621=CARTESIAN_POINT('Ctrl Pts',(-1.20765974050094,12.2,11.103586122497));
#229622=CARTESIAN_POINT('Ctrl Pts',(-1.20858716872143,12.2,11.1003631903495));
#229623=CARTESIAN_POINT('Ctrl Pts',(-1.20950871892835,12.2,11.0971462604508));
#229624=CARTESIAN_POINT('Ctrl Pts',(-1.2104244107326,12.2,11.0939353808029));
#229625=CARTESIAN_POINT('Ctrl Pts',(-1.21164533324916,12.2,11.0896542075501));
#229626=CARTESIAN_POINT('Ctrl Pts',(-1.21285584092362,12.2,11.0853837859207));
#229627=CARTESIAN_POINT('Ctrl Pts',(-1.21405597615465,12.2,11.0811242220785));
#229628=CARTESIAN_POINT('Ctrl Pts',(-1.21525611122216,12.2,11.0768646588167));
#229629=CARTESIAN_POINT('Ctrl Pts',(-1.21644587504099,12.2,11.0726159532591));
#229630=CARTESIAN_POINT('Ctrl Pts',(-1.21762531144525,12.2,11.0683782101048));
#229631=CARTESIAN_POINT('Ctrl Pts',(-1.2188047480102,12.2,11.0641404663731));
#229632=CARTESIAN_POINT('Ctrl Pts',(-1.21997385755081,12.2,11.0599136871388));
#229633=CARTESIAN_POINT('Ctrl Pts',(-1.22113268539319,12.2,11.0556979759216));
#229634=CARTESIAN_POINT('Ctrl Pts',(-1.22229151307767,12.2,11.0514822652789));
#229635=CARTESIAN_POINT('Ctrl Pts',(-1.22344005731877,12.2,11.0472776253702));
#229636=CARTESIAN_POINT('Ctrl Pts',(-1.22457836761528,12.2,11.0430841621012));
#229637=CARTESIAN_POINT('Ctrl Pts',(-1.22600125560224,12.2,11.0378423325863));
#229638=CARTESIAN_POINT('Ctrl Pts',(-1.22740814918597,12.2,11.032617965736));
#229639=CARTESIAN_POINT('Ctrl Pts',(-1.22879913911737,12.2,11.0274112746239));
#229640=CARTESIAN_POINT('Ctrl Pts',(-1.22991193112313,12.2,11.0232459215072));
#229641=CARTESIAN_POINT('Ctrl Pts',(-1.23101454713699,12.2,11.0190918803584));
#229642=CARTESIAN_POINT('Ctrl Pts',(-1.2321070324169,12.2,11.0149492591489));
#229643=CARTESIAN_POINT('Ctrl Pts',(-1.23319951754795,12.2,11.0108066385038));
#229644=CARTESIAN_POINT('Ctrl Pts',(-1.23428187275489,12.2,11.0066754396731));
#229645=CARTESIAN_POINT('Ctrl Pts',(-1.23535414644568,12.2,11.0025557711202));
#229646=CARTESIAN_POINT('Ctrl Pts',(-1.23669448866874,12.2,10.9974061850081));
#229647=CARTESIAN_POINT('Ctrl Pts',(-1.23801907659135,12.2,10.9922746139299));
#229648=CARTESIAN_POINT('Ctrl Pts',(-1.23932800964773,12.2,10.9871612753178));
#229649=CARTESIAN_POINT('Ctrl Pts',(-1.24063694270411,12.2,10.9820479367057));
#229650=CARTESIAN_POINT('Ctrl Pts',(-1.24193021764355,12.2,10.9769528289092));
#229651=CARTESIAN_POINT('Ctrl Pts',(-1.24320793494107,12.2,10.971876172011));
#229652=CARTESIAN_POINT('Ctrl Pts',(-1.24423010883479,12.2,10.9678148462712));
#229653=CARTESIAN_POINT('Ctrl Pts',(-1.24524232497424,12.2,10.963765328567));
#229654=CARTESIAN_POINT('Ctrl Pts',(-1.24624463363897,12.2,10.9597277308481));
#229655=CARTESIAN_POINT('Ctrl Pts',(-1.24724694216714,12.2,10.9556901336794));
#229656=CARTESIAN_POINT('Ctrl Pts',(-1.2482393453438,12.2,10.9516644556897));
#229657=CARTESIAN_POINT('Ctrl Pts',(-1.24922189315301,12.2,10.9476508117948));
#229658=CARTESIAN_POINT('Ctrl Pts',(-1.25020444109609,12.2,10.9436371673531));
#229659=CARTESIAN_POINT('Ctrl Pts',(-1.25117713392891,12.2,10.9396355560951));
#229660=CARTESIAN_POINT('Ctrl Pts',(-1.25214002513976,12.2,10.9356460921794));
#229661=CARTESIAN_POINT('Ctrl Pts',(-1.25334363908772,12.2,10.9306592625566));
#229662=CARTESIAN_POINT('Ctrl Pts',(-1.25453193648254,12.2,10.9256914133845));
#229663=CARTESIAN_POINT('Ctrl Pts',(-1.25570502141186,12.2,10.920742768386));
#229664=CARTESIAN_POINT('Ctrl Pts',(-1.25664348927859,12.2,10.9167838527109));
#229665=CARTESIAN_POINT('Ctrl Pts',(-1.25757222326605,12.2,10.9128372283619));
#229666=CARTESIAN_POINT('Ctrl Pts',(-1.25849127519153,12.2,10.9089030105717));
#229667=CARTESIAN_POINT('Ctrl Pts',(-1.25941032724225,12.2,10.9049687922454));
#229668=CARTESIAN_POINT('Ctrl Pts',(-1.26031969870015,12.2,10.9010469802483));
#229669=CARTESIAN_POINT('Ctrl Pts',(-1.26121944458189,12.2,10.8971376931471));
#229670=CARTESIAN_POINT('Ctrl Pts',(-1.26211919034104,12.2,10.8932284065787));
#229671=CARTESIAN_POINT('Ctrl Pts',(-1.26300931043274,12.2,10.8893316419135));
#229672=CARTESIAN_POINT('Ctrl Pts',(-1.2638898604056,12.2,10.8854475198136));
#229673=CARTESIAN_POINT('Ctrl Pts',(-1.26499054796166,12.2,10.8805923667918));
#229674=CARTESIAN_POINT('Ctrl Pts',(-1.26607628520143,12.2,10.8757569651993));
#229675=CARTESIAN_POINT('Ctrl Pts',(-1.2671471794383,12.2,10.8709415483233));
#229676=CARTESIAN_POINT('Ctrl Pts',(-1.26821807367517,12.2,10.8661261314473));
#229677=CARTESIAN_POINT('Ctrl Pts',(-1.26927412805335,12.2,10.8613306965301));
#229678=CARTESIAN_POINT('Ctrl Pts',(-1.27031545541524,12.2,10.8565554813207));
#229679=CARTESIAN_POINT('Ctrl Pts',(-1.27114851735014,12.2,10.852735308945));
#229680=CARTESIAN_POINT('Ctrl Pts',(-1.27197215285895,12.2,10.8489280748891));
#229681=CARTESIAN_POINT('Ctrl Pts',(-1.27278642410986,12.2,10.8451339017161));
#229682=CARTESIAN_POINT('Ctrl Pts',(-1.27360069524983,12.2,10.8413397290601));
#229683=CARTESIAN_POINT('Ctrl Pts',(-1.27440559906606,12.2,10.8375586166981));
#229684=CARTESIAN_POINT('Ctrl Pts',(-1.2752011976683,12.2,10.8337906862831));
#229685=CARTESIAN_POINT('Ctrl Pts',(-1.27599679637893,12.2,10.8300227553547));
#229686=CARTESIAN_POINT('Ctrl Pts',(-1.27678308949955,12.2,10.8262680065445));
#229687=CARTESIAN_POINT('Ctrl Pts',(-1.27756013809686,12.2,10.8225265629525));
#229688=CARTESIAN_POINT('Ctrl Pts',(-1.2783371865883,12.2,10.8187851198703));
#229689=CARTESIAN_POINT('Ctrl Pts',(-1.27910499036327,12.2,10.8150569812055));
#229690=CARTESIAN_POINT('Ctrl Pts',(-1.2798636116733,12.2,10.8113422713224));
#229691=CARTESIAN_POINT('Ctrl Pts',(-1.28062223308668,12.2,10.8076275609331));
#229692=CARTESIAN_POINT('Ctrl Pts',(-1.28137167168744,12.2,10.8039262793042));
#229693=CARTESIAN_POINT('Ctrl Pts',(-1.28211199106053,12.2,10.8002385522153));
#229694=CARTESIAN_POINT('Ctrl Pts',(-1.28285231033274,12.2,10.7965508256287));
#229695=CARTESIAN_POINT('Ctrl Pts',(-1.28358351027346,12.2,10.7928766510173));
#229696=CARTESIAN_POINT('Ctrl Pts',(-1.28430565488202,12.2,10.7892161566484));
#229697=CARTESIAN_POINT('Ctrl Pts',(-1.28502779958897,12.2,10.7855556617808));
#229698=CARTESIAN_POINT('Ctrl Pts',(-1.28574088813958,12.2,10.7819088460286));
#229699=CARTESIAN_POINT('Ctrl Pts',(-1.2864449874589,12.2,10.7782758364808));
#229700=CARTESIAN_POINT('Ctrl Pts',(-1.28714908668229,12.2,10.774642827428));
#229701=CARTESIAN_POINT('Ctrl Pts',(-1.28784419548474,12.2,10.7710236250016));
#229702=CARTESIAN_POINT('Ctrl Pts',(-1.28853037959623,12.2,10.7674183560727));
#229703=CARTESIAN_POINT('Ctrl Pts',(-1.28921656380121,12.2,10.7638130866526));
#229704=CARTESIAN_POINT('Ctrl Pts',(-1.28989382509978,12.2,10.7602217522449));
#229705=CARTESIAN_POINT('Ctrl Pts',(-1.29056222852509,12.2,10.7566444807166));
#229706=CARTESIAN_POINT('Ctrl Pts',(-1.29123063195041,12.2,10.7530672091883));
#229707=CARTESIAN_POINT('Ctrl Pts',(-1.29189017847469,12.2,10.749504000795));
#229708=CARTESIAN_POINT('Ctrl Pts',(-1.29254093589815,12.2,10.7459549859363));
#229709=CARTESIAN_POINT('Ctrl Pts',(-1.29319169323294,12.2,10.7424059715613));
#229710=CARTESIAN_POINT('Ctrl Pts',(-1.29383366238463,12.2,10.73887115));
#229711=CARTESIAN_POINT('Ctrl Pts',(-1.29446691172466,12.2,10.735350652994));
#229712=CARTESIAN_POINT('Ctrl Pts',(-1.29510016115096,12.2,10.7318301555083));
#229713=CARTESIAN_POINT('Ctrl Pts',(-1.29572469080421,12.2,10.7283239839262));
#229714=CARTESIAN_POINT('Ctrl Pts',(-1.29634057155912,12.2,10.724832267904));
#229715=CARTESIAN_POINT('Ctrl Pts',(-1.29695645223011,12.2,10.7213405523576));
#229716=CARTESIAN_POINT('Ctrl Pts',(-1.29756368437444,12.2,10.7178632948732));
#229717=CARTESIAN_POINT('Ctrl Pts',(-1.29816233849274,12.2,10.7144006272665));
#229718=CARTESIAN_POINT('Ctrl Pts',(-1.29876099269259,12.2,10.7109379591879));
#229719=CARTESIAN_POINT('Ctrl Pts',(-1.29935106954665,12.2,10.7074898826341));
#229720=CARTESIAN_POINT('Ctrl Pts',(-1.2999326410511,12.2,10.7040565297768));
#229721=CARTESIAN_POINT('Ctrl Pts',(-1.30051421247631,12.2,10.7006231773873));
#229722=CARTESIAN_POINT('Ctrl Pts',(-1.30108727996058,12.2,10.6972045521927));
#229723=CARTESIAN_POINT('Ctrl Pts',(-1.30165191547052,12.2,10.6938007873033));
#229724=CARTESIAN_POINT('Ctrl Pts',(-1.30235770991564,12.2,10.6895460808438));
#229725=CARTESIAN_POINT('Ctrl Pts',(-1.30305033114932,12.2,10.6853145958265));
#229726=CARTESIAN_POINT('Ctrl Pts',(-1.30372992545557,12.2,10.6811065985336));
#229727=CARTESIAN_POINT('Ctrl Pts',(-1.30440951976181,12.2,10.6768986012407));
#229728=CARTESIAN_POINT('Ctrl Pts',(-1.30507608706339,12.2,10.6727140939934));
#229729=CARTESIAN_POINT('Ctrl Pts',(-1.30572977727473,12.2,10.6685533467522));
#229730=CARTESIAN_POINT('Ctrl Pts',(-1.3062527294723,12.2,10.6652247487778));
#229731=CARTESIAN_POINT('Ctrl Pts',(-1.3067674410339,12.2,10.661911358125));
#229732=CARTESIAN_POINT('Ctrl Pts',(-1.30727398861624,12.2,10.658613314669));
#229733=CARTESIAN_POINT('Ctrl Pts',(-1.30790717305964,12.2,10.6544907605738));
#229734=CARTESIAN_POINT('Ctrl Pts',(-1.30852760265283,12.2,10.650392185554));
#229735=CARTESIAN_POINT('Ctrl Pts',(-1.30913543209625,12.2,10.6463178689587));
#229736=CARTESIAN_POINT('Ctrl Pts',(-1.30974326147342,12.2,10.6422435528075));
#229737=CARTESIAN_POINT('Ctrl Pts',(-1.31033849264746,12.2,10.6381934920898));
#229738=CARTESIAN_POINT('Ctrl Pts',(-1.31092128043219,12.2,10.6341679702348));
#229739=CARTESIAN_POINT('Ctrl Pts',(-1.31150406828044,12.2,10.630142447941));
#229740=CARTESIAN_POINT('Ctrl Pts',(-1.31207441624275,12.2,10.6261414635832));
#229741=CARTESIAN_POINT('Ctrl Pts',(-1.31263248395209,12.2,10.62216530122));
#229742=CARTESIAN_POINT('Ctrl Pts',(-1.31319055166142,12.2,10.6181891388569));
#229743=CARTESIAN_POINT('Ctrl Pts',(-1.31373633861817,12.2,10.6142377984822));
#229744=CARTESIAN_POINT('Ctrl Pts',(-1.31427001139695,12.2,10.6103115670218));
#229745=CARTESIAN_POINT('Ctrl Pts',(-1.31480368417572,12.2,10.6063853355614));
#229746=CARTESIAN_POINT('Ctrl Pts',(-1.31532524223126,12.2,10.6024842140231));
#229747=CARTESIAN_POINT('Ctrl Pts',(-1.31583485496588,12.2,10.5986084916749));
#229748=CARTESIAN_POINT('Ctrl Pts',(-1.31634446770052,12.2,10.5947327693267));
#229749=CARTESIAN_POINT('Ctrl Pts',(-1.31684213243429,12.2,10.590882448546));
#229750=CARTESIAN_POINT('Ctrl Pts',(-1.31732802347657,12.2,10.5870578222252));
#229751=CARTESIAN_POINT('Ctrl Pts',(-1.31781391451885,12.2,10.5832331959044));
#229752=CARTESIAN_POINT('Ctrl Pts',(-1.31828803065249,12.2,10.5794342661427));
#229753=CARTESIAN_POINT('Ctrl Pts',(-1.31875054919477,12.2,10.5756613289885));
#229754=CARTESIAN_POINT('Ctrl Pts',(-1.31939807516404,12.2,10.5703792168904));
#229755=CARTESIAN_POINT('Ctrl Pts',(-1.32002286524739,12.2,10.5651480526702));
#229756=CARTESIAN_POINT('Ctrl Pts',(-1.32062541426983,12.2,10.5599686680081));
#229757=CARTESIAN_POINT('Ctrl Pts',(-1.32105580642201,12.2,10.5562691075929));
#229758=CARTESIAN_POINT('Ctrl Pts',(-1.32147485166617,12.2,10.5525959663213));
#229759=CARTESIAN_POINT('Ctrl Pts',(-1.32188273527669,12.2,10.5489495525033));
#229760=CARTESIAN_POINT('Ctrl Pts',(-1.32229061888722,12.2,10.5453031386853));
#229761=CARTESIAN_POINT('Ctrl Pts',(-1.32268733927631,12.2,10.5416834501495));
#229762=CARTESIAN_POINT('Ctrl Pts',(-1.32307308554482,12.2,10.5380908012913));
#229763=CARTESIAN_POINT('Ctrl Pts',(-1.32345883181334,12.2,10.5344981524331));
#229764=CARTESIAN_POINT('Ctrl Pts',(-1.3238336034319,12.2,10.5309325439349));
#229765=CARTESIAN_POINT('Ctrl Pts',(-1.32419759384769,12.2,10.5273942910204));
#229766=CARTESIAN_POINT('Ctrl Pts',(-1.32463438233077,12.2,10.5231483876774));
#229767=CARTESIAN_POINT('Ctrl Pts',(-1.32505564512154,12.2,10.5189418766988));
#229768=CARTESIAN_POINT('Ctrl Pts',(-1.32546172169193,12.2,10.514775313498));
#229769=CARTESIAN_POINT('Ctrl Pts',(-1.32580011884622,12.2,10.5113031773712));
#229770=CARTESIAN_POINT('Ctrl Pts',(-1.32612797098799,12.2,10.5078587827475));
#229771=CARTESIAN_POINT('Ctrl Pts',(-1.32644547973745,12.2,10.504442458235));
#229772=CARTESIAN_POINT('Ctrl Pts',(-1.32676298848692,12.2,10.5010261337225));
#229773=CARTESIAN_POINT('Ctrl Pts',(-1.32707015254776,12.2,10.49763787689));
#229774=CARTESIAN_POINT('Ctrl Pts',(-1.32736717976944,12.2,10.4942780207804));
#229775=CARTESIAN_POINT('Ctrl Pts',(-1.32766420699113,12.2,10.4909181646708));
#229776=CARTESIAN_POINT('Ctrl Pts',(-1.3279510955246,12.2,10.4875867077685));
#229777=CARTESIAN_POINT('Ctrl Pts',(-1.32822805852386,12.2,10.4842839880916));
#229778=CARTESIAN_POINT('Ctrl Pts',(-1.3285604141109,12.2,10.4803207246233));
#229779=CARTESIAN_POINT('Ctrl Pts',(-1.32887847294447,12.2,10.4763988409589));
#229780=CARTESIAN_POINT('Ctrl Pts',(-1.32918260976675,12.2,10.4725189287666));
#229781=CARTESIAN_POINT('Ctrl Pts',(-1.32948674658902,12.2,10.4686390165743));
#229782=CARTESIAN_POINT('Ctrl Pts',(-1.32977696181039,12.2,10.464801074663));
#229783=CARTESIAN_POINT('Ctrl Pts',(-1.33005363673162,12.2,10.4610057053588));
#229784=CARTESIAN_POINT('Ctrl Pts',(-1.33033031167796,12.2,10.4572103357099));
#229785=CARTESIAN_POINT('Ctrl Pts',(-1.33059344552293,12.2,10.4534575391531));
#229786=CARTESIAN_POINT('Ctrl Pts',(-1.33084343428566,12.2,10.4497479268706));
#229787=CARTESIAN_POINT('Ctrl Pts',(-1.33109342302568,12.2,10.446038314925));
#229788=CARTESIAN_POINT('Ctrl Pts',(-1.33133026600734,12.2,10.4423718899996));
#229789=CARTESIAN_POINT('Ctrl Pts',(-1.33155436400018,12.2,10.4387492722816));
#229790=CARTESIAN_POINT('Ctrl Pts',(-1.33177846199302,12.2,10.4351266545636));
#229791=CARTESIAN_POINT('Ctrl Pts',(-1.33198981800421,12.2,10.4315478490662));
#229792=CARTESIAN_POINT('Ctrl Pts',(-1.33218884591418,12.2,10.4280134881927));
#229793=CARTESIAN_POINT('Ctrl Pts',(-1.33238787384223,12.2,10.4244791269982));
#229794=CARTESIAN_POINT('Ctrl Pts',(-1.33257457402707,12.2,10.4209892126675));
#229795=CARTESIAN_POINT('Ctrl Pts',(-1.33274937203579,12.2,10.4175443943994));
#229796=CARTESIAN_POINT('Ctrl Pts',(-1.33295330302215,12.2,10.4135254402227));
#229797=CARTESIAN_POINT('Ctrl Pts',(-1.33314103521879,12.2,10.4095678640141));
#229798=CARTESIAN_POINT('Ctrl Pts',(-1.33331326350032,12.2,10.4056727214487));
#229799=CARTESIAN_POINT('Ctrl Pts',(-1.33346088775886,12.2,10.4023340274313));
#229800=CARTESIAN_POINT('Ctrl Pts',(-1.33359712441598,12.2,10.3990412041531));
#229801=CARTESIAN_POINT('Ctrl Pts',(-1.3337224245054,12.2,10.3957949291461));
#229802=CARTESIAN_POINT('Ctrl Pts',(-1.33384772458343,12.2,10.3925486544339));
#229803=CARTESIAN_POINT('Ctrl Pts',(-1.33396208837012,12.2,10.3893489273564));
#229804=CARTESIAN_POINT('Ctrl Pts',(-1.33406598253345,12.2,10.3861964417068));
#229805=CARTESIAN_POINT('Ctrl Pts',(-1.33416987669679,12.2,10.3830439560572));
#229806=CARTESIAN_POINT('Ctrl Pts',(-1.33426330155641,12.2,10.3799387105827));
#229807=CARTESIAN_POINT('Ctrl Pts',(-1.33434673397048,12.2,10.3768814149417));
#229808=CARTESIAN_POINT('Ctrl Pts',(-1.33443016639213,12.2,10.373824119023));
#229809=CARTESIAN_POINT('Ctrl Pts',(-1.33450360979587,12.2,10.370814770902));
#229810=CARTESIAN_POINT('Ctrl Pts',(-1.33456755604871,12.2,10.3678540969105));
#229811=CARTESIAN_POINT('Ctrl Pts',(-1.33463150229574,12.2,10.364893423188));
#229812=CARTESIAN_POINT('Ctrl Pts',(-1.33468595109622,12.2,10.3619814201713));
#229813=CARTESIAN_POINT('Ctrl Pts',(-1.33473141151084,12.2,10.3591188306107));
#229814=CARTESIAN_POINT('Ctrl Pts',(-1.33477687192547,12.2,10.3562562410502));
#229815=CARTESIAN_POINT('Ctrl Pts',(-1.33481334458249,12.2,10.3534430629109));
#229816=CARTESIAN_POINT('Ctrl Pts',(-1.33484135024851,12.2,10.3506800554257));
#229817=CARTESIAN_POINT('Ctrl Pts',(-1.33486935591453,12.2,10.3479170479405));
#229818=CARTESIAN_POINT('Ctrl Pts',(-1.33488889886535,12.2,10.3452042081885));
#229819=CARTESIAN_POINT('Ctrl Pts',(-1.33490051353214,12.2,10.3425423130317));
#229820=CARTESIAN_POINT('Ctrl Pts',(-1.33491212819997,12.2,10.3398804176332));
#229821=CARTESIAN_POINT('Ctrl Pts',(-1.33491581895869,12.2,10.3372694662229));
#229822=CARTESIAN_POINT('Ctrl Pts',(-1.3349121395415,12.2,10.3347102518356));
#229823=CARTESIAN_POINT('Ctrl Pts',(-1.33490846012465,12.2,10.3321510376808));
#229824=CARTESIAN_POINT('Ctrl Pts',(-1.33489741019116,12.2,10.3296435610064));
#229825=CARTESIAN_POINT('Ctrl Pts',(-1.33487956577508,12.2,10.327188635751));
#229826=CARTESIAN_POINT('Ctrl Pts',(-1.33486172135899,12.2,10.3247337104956));
#229827=CARTESIAN_POINT('Ctrl Pts',(-1.33483707968522,12.2,10.3223313361492));
#229828=CARTESIAN_POINT('Ctrl Pts',(-1.33480623452009,12.2,10.3199823443143));
#229829=CARTESIAN_POINT('Ctrl Pts',(-1.33477538935217,12.2,10.317633352266));
#229830=CARTESIAN_POINT('Ctrl Pts',(-1.3347383410007,12.2,10.3153377453225));
#229831=CARTESIAN_POINT('Ctrl Pts',(-1.33469569799593,12.2,10.3130963780082));
#229832=CARTESIAN_POINT('Ctrl Pts',(-1.33465305499502,12.2,10.3108550108975));
#229833=CARTESIAN_POINT('Ctrl Pts',(-1.33460481848147,12.2,10.3086678827224));
#229834=CARTESIAN_POINT('Ctrl Pts',(-1.3345516194834,12.2,10.3065358709665));
#229835=CARTESIAN_POINT('Ctrl Pts',(-1.33449842048533,12.2,10.3044038592106));
#229836=CARTESIAN_POINT('Ctrl Pts',(-1.33444025941503,12.2,10.3023269653096));
#229837=CARTESIAN_POINT('Ctrl Pts',(-1.33437778649776,12.2,10.3003060904455));
#229838=CARTESIAN_POINT('Ctrl Pts',(-1.33431531357482,12.2,10.2982852153979));
#229839=CARTESIAN_POINT('Ctrl Pts',(-1.33424852863814,12.2,10.2963203589004));
#229840=CARTESIAN_POINT('Ctrl Pts',(-1.33417810671739,12.2,10.2944124472169));
#229841=CARTESIAN_POINT('Ctrl Pts',(-1.33410802277682,12.2,10.2925136922895));
#229842=CARTESIAN_POINT('Ctrl Pts',(-1.33403433934042,12.2,10.2906713385628));
#229843=CARTESIAN_POINT('Ctrl Pts',(-1.33395773200006,12.2,10.288886324));
#229844=CARTESIAN_POINT('Ctrl Pts',(-1.33395773200006,15.2,10.288886324));
#229845=CARTESIAN_POINT('Ctrl Pts',(-1.33403433934042,15.2,10.2906713385628));
#229846=CARTESIAN_POINT('Ctrl Pts',(-1.33410802277682,15.2,10.2925136922895));
#229847=CARTESIAN_POINT('Ctrl Pts',(-1.33417810671739,15.2,10.2944124472169));
#229848=CARTESIAN_POINT('Ctrl Pts',(-1.33424852863814,15.2,10.2963203589004));
#229849=CARTESIAN_POINT('Ctrl Pts',(-1.33431531357482,15.2,10.2982852153978));
#229850=CARTESIAN_POINT('Ctrl Pts',(-1.33437778649776,15.2,10.3003060904455));
#229851=CARTESIAN_POINT('Ctrl Pts',(-1.33444025941503,15.2,10.3023269653096));
#229852=CARTESIAN_POINT('Ctrl Pts',(-1.33449842048533,15.2,10.3044038592107));
#229853=CARTESIAN_POINT('Ctrl Pts',(-1.3345516194834,15.2,10.3065358709666));
#229854=CARTESIAN_POINT('Ctrl Pts',(-1.33460481848146,15.2,10.3086678827224));
#229855=CARTESIAN_POINT('Ctrl Pts',(-1.33465305499502,15.2,10.3108550108974));
#229856=CARTESIAN_POINT('Ctrl Pts',(-1.33469569799593,15.2,10.3130963780082));
#229857=CARTESIAN_POINT('Ctrl Pts',(-1.3347383410007,15.2,10.3153377453225));
#229858=CARTESIAN_POINT('Ctrl Pts',(-1.33477538935217,15.2,10.317633352266));
#229859=CARTESIAN_POINT('Ctrl Pts',(-1.33480623452009,15.2,10.3199823443143));
#229860=CARTESIAN_POINT('Ctrl Pts',(-1.33483707968522,15.2,10.3223313361492));
#229861=CARTESIAN_POINT('Ctrl Pts',(-1.33486172135899,15.2,10.3247337104956));
#229862=CARTESIAN_POINT('Ctrl Pts',(-1.33487956577508,15.2,10.327188635751));
#229863=CARTESIAN_POINT('Ctrl Pts',(-1.33489741019116,15.2,10.3296435610064));
#229864=CARTESIAN_POINT('Ctrl Pts',(-1.33490846012465,15.2,10.3321510376809));
#229865=CARTESIAN_POINT('Ctrl Pts',(-1.3349121395415,15.2,10.3347102518356));
#229866=CARTESIAN_POINT('Ctrl Pts',(-1.33491581895869,15.2,10.3372694662229));
#229867=CARTESIAN_POINT('Ctrl Pts',(-1.33491212819997,15.2,10.3398804176332));
#229868=CARTESIAN_POINT('Ctrl Pts',(-1.33490051353214,15.2,10.3425423130317));
#229869=CARTESIAN_POINT('Ctrl Pts',(-1.33488889886535,15.2,10.3452042081885));
#229870=CARTESIAN_POINT('Ctrl Pts',(-1.33486935591453,15.2,10.3479170479406));
#229871=CARTESIAN_POINT('Ctrl Pts',(-1.33484135024851,15.2,10.3506800554257));
#229872=CARTESIAN_POINT('Ctrl Pts',(-1.33481334458249,15.2,10.3534430629108));
#229873=CARTESIAN_POINT('Ctrl Pts',(-1.33477687192547,15.2,10.3562562410502));
#229874=CARTESIAN_POINT('Ctrl Pts',(-1.33473141151084,15.2,10.3591188306108));
#229875=CARTESIAN_POINT('Ctrl Pts',(-1.33468595109622,15.2,10.3619814201713));
#229876=CARTESIAN_POINT('Ctrl Pts',(-1.33463150229574,15.2,10.3648934231881));
#229877=CARTESIAN_POINT('Ctrl Pts',(-1.33456755604871,15.2,10.3678540969105));
#229878=CARTESIAN_POINT('Ctrl Pts',(-1.33448229437826,15.2,10.3718016622324));
#229879=CARTESIAN_POINT('Ctrl Pts',(-1.33438015033105,15.2,10.3758357563356));
#229880=CARTESIAN_POINT('Ctrl Pts',(-1.33425995299025,15.2,10.37995466812));
#229881=CARTESIAN_POINT('Ctrl Pts',(-1.33415478032932,15.2,10.3835587155104));
#229882=CARTESIAN_POINT('Ctrl Pts',(-1.33403579119185,15.2,10.3872277021273));
#229883=CARTESIAN_POINT('Ctrl Pts',(-1.33390223100627,15.2,10.3909605146007));
#229884=CARTESIAN_POINT('Ctrl Pts',(-1.33378775083383,15.2,10.3941600685231));
#229885=CARTESIAN_POINT('Ctrl Pts',(-1.33366256536007,15.2,10.3974065145429));
#229886=CARTESIAN_POINT('Ctrl Pts',(-1.33352621618521,15.2,10.4006991693921));
#229887=CARTESIAN_POINT('Ctrl Pts',(-1.33336714216645,15.2,10.404540599601));
#229888=CARTESIAN_POINT('Ctrl Pts',(-1.33319287180157,15.2,10.4084449208732));
#229889=CARTESIAN_POINT('Ctrl Pts',(-1.33300269804082,15.2,10.4124110706545));
#229890=CARTESIAN_POINT('Ctrl Pts',(-1.33283969194114,15.2,10.4158106280069));
#229891=CARTESIAN_POINT('Ctrl Pts',(-1.33266500207405,15.2,10.4192556114537));
#229892=CARTESIAN_POINT('Ctrl Pts',(-1.33247819522971,15.2,10.422745363647));
#229893=CARTESIAN_POINT('Ctrl Pts',(-1.33229138840234,15.2,10.4262351155232));
#229894=CARTESIAN_POINT('Ctrl Pts',(-1.33209246643496,15.2,10.4297696369234));
#229895=CARTESIAN_POINT('Ctrl Pts',(-1.33188100652498,15.2,10.4333482847265));
#229896=CARTESIAN_POINT('Ctrl Pts',(-1.33163430328387,15.2,10.4375233740468));
#229897=CARTESIAN_POINT('Ctrl Pts',(-1.3313705361403,15.2,10.4417585233586));
#229898=CARTESIAN_POINT('Ctrl Pts',(-1.33108905573211,15.2,10.4460527341928));
#229899=CARTESIAN_POINT('Ctrl Pts',(-1.33080757534583,15.2,10.4503469446927));
#229900=CARTESIAN_POINT('Ctrl Pts',(-1.3305083827271,15.2,10.4547002160138));
#229901=CARTESIAN_POINT('Ctrl Pts',(-1.33019084775971,15.2,10.4591115706509));
#229902=CARTESIAN_POINT('Ctrl Pts',(-1.32991867489873,15.2,10.46289273221));
#229903=CARTESIAN_POINT('Ctrl Pts',(-1.32963302655136,15.2,10.4667165679494));
#229904=CARTESIAN_POINT('Ctrl Pts',(-1.32933351970076,15.2,10.470582473413));
#229905=CARTESIAN_POINT('Ctrl Pts',(-1.32903401287737,15.2,10.4744483785254));
#229906=CARTESIAN_POINT('Ctrl Pts',(-1.32872064742288,15.2,10.4783563548272));
#229907=CARTESIAN_POINT('Ctrl Pts',(-1.3283930467666,15.2,10.4823058080351));
#229908=CARTESIAN_POINT('Ctrl Pts',(-1.32784704565295,15.2,10.4888882302873));
#229909=CARTESIAN_POINT('Ctrl Pts',(-1.32726150468059,15.2,10.4955858675033));
#229910=CARTESIAN_POINT('Ctrl Pts',(-1.32663474551286,15.2,10.5023960350061));
#229911=CARTESIAN_POINT('Ctrl Pts',(-1.32632136592899,15.2,10.5058011187576));
#229912=CARTESIAN_POINT('Ctrl Pts',(-1.32599768351757,15.2,10.509234337538));
#229913=CARTESIAN_POINT('Ctrl Pts',(-1.32566349627792,15.2,10.5126953638935));
#229914=CARTESIAN_POINT('Ctrl Pts',(-1.32519563417155,15.2,10.5175408004892));
#229915=CARTESIAN_POINT('Ctrl Pts',(-1.32470718039805,15.2,10.5224407372488));
#229916=CARTESIAN_POINT('Ctrl Pts',(-1.32419759384769,15.2,10.5273942910205));
#229917=CARTESIAN_POINT('Ctrl Pts',(-1.32383360343191,15.2,10.5309325439348));
#229918=CARTESIAN_POINT('Ctrl Pts',(-1.32345883181334,15.2,10.5344981524331));
#229919=CARTESIAN_POINT('Ctrl Pts',(-1.32307308554483,15.2,10.5380908012913));
#229920=CARTESIAN_POINT('Ctrl Pts',(-1.32268733927631,15.2,10.5416834501495));
#229921=CARTESIAN_POINT('Ctrl Pts',(-1.32229061888723,15.2,10.5453031386852));
#229922=CARTESIAN_POINT('Ctrl Pts',(-1.32188273527669,15.2,10.5489495525033));
#229923=CARTESIAN_POINT('Ctrl Pts',(-1.32147485166616,15.2,10.5525959663214));
#229924=CARTESIAN_POINT('Ctrl Pts',(-1.32105580642201,15.2,10.5562691075929));
#229925=CARTESIAN_POINT('Ctrl Pts',(-1.32062541426983,15.2,10.5599686680081));
#229926=CARTESIAN_POINT('Ctrl Pts',(-1.32002286524739,15.2,10.5651480526701));
#229927=CARTESIAN_POINT('Ctrl Pts',(-1.31939807516402,15.2,10.5703792168905));
#229928=CARTESIAN_POINT('Ctrl Pts',(-1.31875054919476,15.2,10.5756613289885));
#229929=CARTESIAN_POINT('Ctrl Pts',(-1.3182880306525,15.2,10.5794342661426));
#229930=CARTESIAN_POINT('Ctrl Pts',(-1.31781391451886,15.2,10.5832331959043));
#229931=CARTESIAN_POINT('Ctrl Pts',(-1.31732802347657,15.2,10.5870578222252));
#229932=CARTESIAN_POINT('Ctrl Pts',(-1.31684213243428,15.2,10.5908824485461));
#229933=CARTESIAN_POINT('Ctrl Pts',(-1.31634446770051,15.2,10.5947327693267));
#229934=CARTESIAN_POINT('Ctrl Pts',(-1.31583485496588,15.2,10.5986084916749));
#229935=CARTESIAN_POINT('Ctrl Pts',(-1.31532524223126,15.2,10.6024842140231));
#229936=CARTESIAN_POINT('Ctrl Pts',(-1.31480368417572,15.2,10.6063853355614));
#229937=CARTESIAN_POINT('Ctrl Pts',(-1.31427001139694,15.2,10.6103115670218));
#229938=CARTESIAN_POINT('Ctrl Pts',(-1.3135228695532,15.2,10.6158082907241));
#229939=CARTESIAN_POINT('Ctrl Pts',(-1.3127519821012,15.2,10.6213542276119));
#229940=CARTESIAN_POINT('Ctrl Pts',(-1.3119568983327,15.2,10.6269485919689));
#229941=CARTESIAN_POINT('Ctrl Pts',(-1.31127539788012,15.2,10.6317437619777));
#229942=CARTESIAN_POINT('Ctrl Pts',(-1.31057612170664,15.2,10.6365745106687));
#229943=CARTESIAN_POINT('Ctrl Pts',(-1.30985879046398,15.2,10.6414403509291));
#229944=CARTESIAN_POINT('Ctrl Pts',(-1.30926101446102,15.2,10.6454952175917));
#229945=CARTESIAN_POINT('Ctrl Pts',(-1.30865070386409,15.2,10.6495744526291));
#229946=CARTESIAN_POINT('Ctrl Pts',(-1.30802769796026,15.2,10.65367777902));
#229947=CARTESIAN_POINT('Ctrl Pts',(-1.30752929327794,15.2,10.6569604398644));
#229948=CARTESIAN_POINT('Ctrl Pts',(-1.30702276556058,15.2,10.660258518515));
#229949=CARTESIAN_POINT('Ctrl Pts',(-1.30650803482543,15.2,10.6635718735209));
#229950=CARTESIAN_POINT('Ctrl Pts',(-1.30599330402014,15.2,10.6668852289782));
#229951=CARTESIAN_POINT('Ctrl Pts',(-1.30547037095139,15.2,10.6702138618652));
#229952=CARTESIAN_POINT('Ctrl Pts',(-1.30493915867296,15.2,10.6735576314935));
#229953=CARTESIAN_POINT('Ctrl Pts',(-1.30400953729426,15.2,10.6794092276599));
#229954=CARTESIAN_POINT('Ctrl Pts',(-1.30305455716802,15.2,10.6853071812285));
#229955=CARTESIAN_POINT('Ctrl Pts',(-1.30207381280005,15.2,10.6912507511613));
#229956=CARTESIAN_POINT('Ctrl Pts',(-1.30123317467218,15.2,10.6963452402701));
#229957=CARTESIAN_POINT('Ctrl Pts',(-1.30037360910795,15.2,10.7014732442082));
#229958=CARTESIAN_POINT('Ctrl Pts',(-1.2994948666817,15.2,10.7066343037493));
#229959=CARTESIAN_POINT('Ctrl Pts',(-1.29890903847735,15.2,10.7100750096412));
#229960=CARTESIAN_POINT('Ctrl Pts',(-1.29831468618556,15.2,10.7135304069149));
#229961=CARTESIAN_POINT('Ctrl Pts',(-1.29771173829097,15.2,10.7170003612414));
#229962=CARTESIAN_POINT('Ctrl Pts',(-1.29665657937275,15.2,10.7230727819037));
#229963=CARTESIAN_POINT('Ctrl Pts',(-1.29557509817755,15.2,10.7291897826339));
#229964=CARTESIAN_POINT('Ctrl Pts',(-1.29446691172466,15.2,10.735350652994));
#229965=CARTESIAN_POINT('Ctrl Pts',(-1.29367534998492,15.2,10.7397512746113));
#229966=CARTESIAN_POINT('Ctrl Pts',(-1.29287016372494,15.2,10.7441742778563));
#229967=CARTESIAN_POINT('Ctrl Pts',(-1.29205121865479,15.2,10.7486194070241));
#229968=CARTESIAN_POINT('Ctrl Pts',(-1.29139606265222,15.2,10.7521755100676));
#229969=CARTESIAN_POINT('Ctrl Pts',(-1.29073210033475,15.2,10.7557457737527));
#229970=CARTESIAN_POINT('Ctrl Pts',(-1.2900592643351,15.2,10.7593300686806));
#229971=CARTESIAN_POINT('Ctrl Pts',(-1.28921821926677,15.2,10.7638104377067));
#229972=CARTESIAN_POINT('Ctrl Pts',(-1.28836330849334,15.2,10.7683127293226));
#229973=CARTESIAN_POINT('Ctrl Pts',(-1.28749440178425,15.2,10.7728366929498));
#229974=CARTESIAN_POINT('Ctrl Pts',(-1.28679927637909,15.2,10.7764558640489));
#229975=CARTESIAN_POINT('Ctrl Pts',(-1.28609519354783,15.2,10.7800889059208));
#229976=CARTESIAN_POINT('Ctrl Pts',(-1.28538208817504,15.2,10.7837356895648));
#229977=CARTESIAN_POINT('Ctrl Pts',(-1.28431243021302,15.2,10.7892058645341));
#229978=CARTESIAN_POINT('Ctrl Pts',(-1.28322247001929,15.2,10.7947069620842));
#229979=CARTESIAN_POINT('Ctrl Pts',(-1.28211199106053,15.2,10.8002385522152));
#229980=CARTESIAN_POINT('Ctrl Pts',(-1.28137167168744,15.2,10.8039262793042));
#229981=CARTESIAN_POINT('Ctrl Pts',(-1.28062223308668,15.2,10.8076275609331));
#229982=CARTESIAN_POINT('Ctrl Pts',(-1.27986361167329,15.2,10.8113422713224));
#229983=CARTESIAN_POINT('Ctrl Pts',(-1.2785360243549,15.2,10.8178430137444));
#229984=CARTESIAN_POINT('Ctrl Pts',(-1.27718031534707,15.2,10.8243848802251));
#229985=CARTESIAN_POINT('Ctrl Pts',(-1.27579615312941,15.2,10.83096721091));
#229986=CARTESIAN_POINT('Ctrl Pts',(-1.27500520319837,15.2,10.8347285431691));
#229987=CARTESIAN_POINT('Ctrl Pts',(-1.27420496341403,15.2,10.8385030876955));
#229988=CARTESIAN_POINT('Ctrl Pts',(-1.27339537203287,15.2,10.8422907232525));
#229989=CARTESIAN_POINT('Ctrl Pts',(-1.27258578076202,15.2,10.8460783582935));
#229990=CARTESIAN_POINT('Ctrl Pts',(-1.27176683820296,15.2,10.8498790840589));
#229991=CARTESIAN_POINT('Ctrl Pts',(-1.27093848566053,15.2,10.8536927791347));
#229992=CARTESIAN_POINT('Ctrl Pts',(-1.27011013300523,15.2,10.8575064747301));
#229993=CARTESIAN_POINT('Ctrl Pts',(-1.26927236963515,15.2,10.8613331395768));
#229994=CARTESIAN_POINT('Ctrl Pts',(-1.26842513703343,15.2,10.8651726545083));
#229995=CARTESIAN_POINT('Ctrl Pts',(-1.26757790443171,15.2,10.8690121694397));
#229996=CARTESIAN_POINT('Ctrl Pts',(-1.26672120383163,15.2,10.8728645326394));
#229997=CARTESIAN_POINT('Ctrl Pts',(-1.2658549746168,15.2,10.8767296269069));
#229998=CARTESIAN_POINT('Ctrl Pts',(-1.26477218827528,15.2,10.8815609939513));
#229999=CARTESIAN_POINT('Ctrl Pts',(-1.26367451792866,15.2,10.8864122510732));
#230000=CARTESIAN_POINT('Ctrl Pts',(-1.26256185062063,15.2,10.8912831696378));
#230001=CARTESIAN_POINT('Ctrl Pts',(-1.26144918319131,15.2,10.8961540887334));
#230002=CARTESIAN_POINT('Ctrl Pts',(-1.26032151914277,15.2,10.9010446657315));
#230003=CARTESIAN_POINT('Ctrl Pts',(-1.25917875011623,15.2,10.905954674341));
#230004=CARTESIAN_POINT('Ctrl Pts',(-1.25826453484518,15.2,10.9098826814427));
#230005=CARTESIAN_POINT('Ctrl Pts',(-1.2573406517371,15.2,10.9138231253928));
#230006=CARTESIAN_POINT('Ctrl Pts',(-1.25640704774176,15.2,10.9177758884416));
#230007=CARTESIAN_POINT('Ctrl Pts',(-1.25547344374643,15.2,10.9217286514904));
#230008=CARTESIAN_POINT('Ctrl Pts',(-1.25453011773608,15.2,10.9256937344017));
#230009=CARTESIAN_POINT('Ctrl Pts',(-1.25357701579425,15.2,10.9296710226752));
#230010=CARTESIAN_POINT('Ctrl Pts',(-1.25262391398229,15.2,10.9336483104068));
#230011=CARTESIAN_POINT('Ctrl Pts',(-1.2516610363784,15.2,10.9376378020757));
#230012=CARTESIAN_POINT('Ctrl Pts',(-1.25068833050909,15.2,10.9416393844889));
#230013=CARTESIAN_POINT('Ctrl Pts',(-1.24947244807305,15.2,10.9466413629143));
#230014=CARTESIAN_POINT('Ctrl Pts',(-1.24824120746676,15.2,10.9516622324555));
#230015=CARTESIAN_POINT('Ctrl Pts',(-1.24699450850843,15.2,10.9567017702333));
#230016=CARTESIAN_POINT('Ctrl Pts',(-1.24599714928742,15.2,10.9607334006752));
#230017=CARTESIAN_POINT('Ctrl Pts',(-1.24498989763467,15.2,10.9647769799519));
#230018=CARTESIAN_POINT('Ctrl Pts',(-1.24397269913378,15.2,10.9688323943963));
#230019=CARTESIAN_POINT('Ctrl Pts',(-1.24270120121554,15.2,10.9739016616231));
#230020=CARTESIAN_POINT('Ctrl Pts',(-1.24141416551056,15.2,10.9789894235345));
#230021=CARTESIAN_POINT('Ctrl Pts',(-1.24011149169548,15.2,10.9840954606154));
#230022=CARTESIAN_POINT('Ctrl Pts',(-1.23880881773842,15.2,10.9892014982528));
#230023=CARTESIAN_POINT('Ctrl Pts',(-1.23749050626219,15.2,10.9943258109343));
#230024=CARTESIAN_POINT('Ctrl Pts',(-1.23615646216625,15.2,10.999468182044));
#230025=CARTESIAN_POINT('Ctrl Pts',(-1.23482241807032,15.2,11.0046105531536));
#230026=CARTESIAN_POINT('Ctrl Pts',(-1.23347263894236,15.2,11.0097709829192));
#230027=CARTESIAN_POINT('Ctrl Pts',(-1.2321070324169,15.2,11.0149492591489));
#230028=CARTESIAN_POINT('Ctrl Pts',(-1.23101454713699,15.2,11.0190918803584));
#230029=CARTESIAN_POINT('Ctrl Pts',(-1.22991193112312,15.2,11.0232459215073));
#230030=CARTESIAN_POINT('Ctrl Pts',(-1.22879913911736,15.2,11.0274112746239));
#230031=CARTESIAN_POINT('Ctrl Pts',(-1.22768634726322,15.2,11.031576627173));
#230032=CARTESIAN_POINT('Ctrl Pts',(-1.22656337725278,15.2,11.0357532920838));
#230033=CARTESIAN_POINT('Ctrl Pts',(-1.22543018223537,15.2,11.0399411605736));
#230034=CARTESIAN_POINT('Ctrl Pts',(-1.22429698706356,15.2,11.0441290296339));
#230035=CARTESIAN_POINT('Ctrl Pts',(-1.2231535680258,15.2,11.0483281015653));
#230036=CARTESIAN_POINT('Ctrl Pts',(-1.22199987879097,15.2,11.0525382707028));
#230037=CARTESIAN_POINT('Ctrl Pts',(-1.22084618971334,15.2,11.0567484392667));
#230038=CARTESIAN_POINT('Ctrl Pts',(-1.2196822291367,15.2,11.0609697042495));
#230039=CARTESIAN_POINT('Ctrl Pts',(-1.21850795340042,15.2,11.0652019587913));
#230040=CARTESIAN_POINT('Ctrl Pts',(-1.216746539556,15.2,11.0715503414689));
#230041=CARTESIAN_POINT('Ctrl Pts',(-1.21496191504266,15.2,11.0779234504574));
#230042=CARTESIAN_POINT('Ctrl Pts',(-1.21315392919313,15.2,11.084320930057));
#230043=CARTESIAN_POINT('Ctrl Pts',(-1.21194860545767,15.2,11.0885859158757));
#230044=CARTESIAN_POINT('Ctrl Pts',(-1.21073289819365,15.2,11.0928617311429));
#230045=CARTESIAN_POINT('Ctrl Pts',(-1.20950676567796,15.2,11.0971482745613));
#230046=CARTESIAN_POINT('Ctrl Pts',(-1.20858716624943,15.2,11.1003631822712));
#230047=CARTESIAN_POINT('Ctrl Pts',(-1.20766170073515,15.2,11.1035841239479));
#230048=CARTESIAN_POINT('Ctrl Pts',(-1.20673035293646,15.2,11.1068110535381));
#230049=CARTESIAN_POINT('Ctrl Pts',(-1.20517810654891,15.2,11.1121892697173));
#230050=CARTESIAN_POINT('Ctrl Pts',(-1.20360951992828,15.2,11.1175841244824));
#230051=CARTESIAN_POINT('Ctrl Pts',(-1.20202450770741,15.2,11.1229954133005));
#230052=CARTESIAN_POINT('Ctrl Pts',(-1.2007564978616,15.2,11.1273244445909));
#230053=CARTESIAN_POINT('Ctrl Pts',(-1.19947797663925,15.2,11.1316639950766));
#230054=CARTESIAN_POINT('Ctrl Pts',(-1.19818890150755,15.2,11.1360139602779));
#230055=CARTESIAN_POINT('Ctrl Pts',(-1.19722209524659,15.2,11.1392764338826));
#230056=CARTESIAN_POINT('Ctrl Pts',(-1.19624935251984,15.2,11.1425447669178));
#230057=CARTESIAN_POINT('Ctrl Pts',(-1.19527065675932,15.2,11.145818915022));
#230058=CARTESIAN_POINT('Ctrl Pts',(-1.19396572896009,15.2,11.1501844462241));
#230059=CARTESIAN_POINT('Ctrl Pts',(-1.19265021641218,15.2,11.1545603161048));
#230060=CARTESIAN_POINT('Ctrl Pts',(-1.19132407978327,15.2,11.1589464232337));
#230061=CARTESIAN_POINT('Ctrl Pts',(-1.19032947740193,15.2,11.1622360032817));
#230062=CARTESIAN_POINT('Ctrl Pts',(-1.18932889820423,15.2,11.1655313408293));
#230063=CARTESIAN_POINT('Ctrl Pts',(-1.18832232590695,15.2,11.1688323948765));
#230064=CARTESIAN_POINT('Ctrl Pts',(-1.18698022957153,15.2,11.1732338000729));
#230065=CARTESIAN_POINT('Ctrl Pts',(-1.1856274785786,15.2,11.1776453663527));
#230066=CARTESIAN_POINT('Ctrl Pts',(-1.18426403345622,15.2,11.1820669926001));
#230067=CARTESIAN_POINT('Ctrl Pts',(-1.18324144956799,15.2,11.1853832124362));
#230068=CARTESIAN_POINT('Ctrl Pts',(-1.18221284908723,15.2,11.1887050918462));
#230069=CARTESIAN_POINT('Ctrl Pts',(-1.18117821775065,15.2,11.1920325875162));
#230070=CARTESIAN_POINT('Ctrl Pts',(-1.17979870917657,15.2,11.1964692488125));
#230071=CARTESIAN_POINT('Ctrl Pts',(-1.17840847774311,15.2,11.200915896021));
#230072=CARTESIAN_POINT('Ctrl Pts',(-1.17700748400011,15.2,11.2053724292083));
#230073=CARTESIAN_POINT('Ctrl Pts',(-1.1759567387883,15.2,11.2087148287951));
#230074=CARTESIAN_POINT('Ctrl Pts',(-1.17489993931003,15.2,11.2120627894902));
#230075=CARTESIAN_POINT('Ctrl Pts',(-1.17383707105752,15.2,11.2154162686178));
#230076=CARTESIAN_POINT('Ctrl Pts',(-1.172774202805,15.2,11.2187697477455));
#230077=CARTESIAN_POINT('Ctrl Pts',(-1.17170526577197,15.2,11.2221287461205));
#230078=CARTESIAN_POINT('Ctrl Pts',(-1.17063024296636,15.2,11.2254932223324));
#230079=CARTESIAN_POINT('Ctrl Pts',(-1.16955522016075,15.2,11.2288576985443));
#230080=CARTESIAN_POINT('Ctrl Pts',(-1.16847411226343,15.2,11.2322276517042));
#230081=CARTESIAN_POINT('Ctrl Pts',(-1.16738690347044,15.2,11.2356030408308));
#230082=CARTESIAN_POINT('Ctrl Pts',(-1.16629969447994,15.2,11.2389784305706));
#230083=CARTESIAN_POINT('Ctrl Pts',(-1.16520638405436,15.2,11.242359256762));
#230084=CARTESIAN_POINT('Ctrl Pts',(-1.16410695806042,15.2,11.2457454779632));
#230085=CARTESIAN_POINT('Ctrl Pts',(-1.1630075322662,15.2,11.2491316985492));
#230086=CARTESIAN_POINT('Ctrl Pts',(-1.16190198958896,15.2,11.2525233133266));
#230087=CARTESIAN_POINT('Ctrl Pts',(-1.16079031633715,15.2,11.255920282412));
#230088=CARTESIAN_POINT('Ctrl Pts',(-1.15930808540207,15.2,11.2604495743201));
#230089=CARTESIAN_POINT('Ctrl Pts',(-1.15781495419971,15.2,11.2649883842597));
#230090=CARTESIAN_POINT('Ctrl Pts',(-1.15631088654601,15.2,11.269536615498));
#230091=CARTESIAN_POINT('Ctrl Pts',(-1.15518283554958,15.2,11.2729477897013));
#230092=CARTESIAN_POINT('Ctrl Pts',(-1.15404863225139,15.2,11.2763642627813));
#230093=CARTESIAN_POINT('Ctrl Pts',(-1.15290826379315,15.2,11.2797859950292));
#230094=CARTESIAN_POINT('Ctrl Pts',(-1.15176789554209,15.2,11.2832077266556));
#230095=CARTESIAN_POINT('Ctrl Pts',(-1.15062136097677,15.2,11.2866347171334));
#230096=CARTESIAN_POINT('Ctrl Pts',(-1.14946864475202,15.2,11.2900669268474));
#230097=CARTESIAN_POINT('Ctrl Pts',(-1.1475474509743,15.2,11.2957872765786));
#230098=CARTESIAN_POINT('Ctrl Pts',(-1.14560908942906,15.2,11.3015221195174));
#230099=CARTESIAN_POINT('Ctrl Pts',(-1.14365349151096,15.2,11.3072712732686));
#230100=CARTESIAN_POINT('Ctrl Pts',(-1.14248013280273,15.2,11.310720765394));
#230101=CARTESIAN_POINT('Ctrl Pts',(-1.14130056949487,15.2,11.3141754097524));
#230102=CARTESIAN_POINT('Ctrl Pts',(-1.14011478637074,15.2,11.3176351649188));
#230103=CARTESIAN_POINT('Ctrl Pts',(-1.13853374227705,15.2,11.3222481715979));
#230104=CARTESIAN_POINT('Ctrl Pts',(-1.13694164344741,15.2,11.3268702646566));
#230105=CARTESIAN_POINT('Ctrl Pts',(-1.13533845449933,15.2,11.3315013521197));
#230106=CARTESIAN_POINT('Ctrl Pts',(-1.13413606273367,15.2,11.3349746678748));
#230107=CARTESIAN_POINT('Ctrl Pts',(-1.13292743320328,15.2,11.3384530415345));
#230108=CARTESIAN_POINT('Ctrl Pts',(-1.13171255249827,15.2,11.3419364337406));
#230109=CARTESIAN_POINT('Ctrl Pts',(-1.1296877512497,15.2,11.3477420876283));
#230110=CARTESIAN_POINT('Ctrl Pts',(-1.12764558405698,15.2,11.3535616835713));
#230111=CARTESIAN_POINT('Ctrl Pts',(-1.12558598954449,15.2,11.3593950391953));
#230112=CARTESIAN_POINT('Ctrl Pts',(-1.1243502326574,15.2,11.3628950530783));
#230113=CARTESIAN_POINT('Ctrl Pts',(-1.12310820284356,15.2,11.3664000220044));
#230114=CARTESIAN_POINT('Ctrl Pts',(-1.12185988495296,15.2,11.3699099047651));
#230115=CARTESIAN_POINT('Ctrl Pts',(-1.11977935566443,15.2,11.3757597078786));
#230116=CARTESIAN_POINT('Ctrl Pts',(-1.11768136063922,15.2,11.381623160384));
#230117=CARTESIAN_POINT('Ctrl Pts',(-1.11556583955181,15.2,11.3875000794646));
#230118=CARTESIAN_POINT('Ctrl Pts',(-1.11429652657653,15.2,11.3910262318097));
#230119=CARTESIAN_POINT('Ctrl Pts',(-1.1130209038578,15.2,11.3945572327229));
#230120=CARTESIAN_POINT('Ctrl Pts',(-1.11173896000396,15.2,11.3980930480291));
#230121=CARTESIAN_POINT('Ctrl Pts',(-1.110457016383,15.2,11.401628862693));
#230122=CARTESIAN_POINT('Ctrl Pts',(-1.10916875256239,15.2,11.4051694916149));
#230123=CARTESIAN_POINT('Ctrl Pts',(-1.10787415431722,15.2,11.4087148951115));
#230124=CARTESIAN_POINT('Ctrl Pts',(-1.10657955607204,15.2,11.4122602986081));
#230125=CARTESIAN_POINT('Ctrl Pts',(-1.10527862254071,15.2,11.4158104755162));
#230126=CARTESIAN_POINT('Ctrl Pts',(-1.10397133974891,15.2,11.4193653785282));
#230127=CARTESIAN_POINT('Ctrl Pts',(-1.10179253501675,15.2,11.4252902170968));
#230128=CARTESIAN_POINT('Ctrl Pts',(-1.09959608544472,15.2,11.431228170913));
#230129=CARTESIAN_POINT('Ctrl Pts',(-1.09738195536205,15.2,11.4371791166813));
#230130=CARTESIAN_POINT('Ctrl Pts',(-1.09605347736072,15.2,11.4407496840126));
#230131=CARTESIAN_POINT('Ctrl Pts',(-1.09471863524371,15.2,11.4443249343496));
#230132=CARTESIAN_POINT('Ctrl Pts',(-1.09337743000006,15.2,11.447904865));
#230133=CARTESIAN_POINT('Origin',(-5.66257110645729E-14,15.2,-1.77635683940025E-14));
#230134=CARTESIAN_POINT('',(-1.76496130700006,15.2,10.223773109));
#230135=CARTESIAN_POINT('',(-1.76496130700006,12.2,10.223773109));
#230136=CARTESIAN_POINT('',(-1.76496130700006,15.2,10.223773109));
#230137=CARTESIAN_POINT('Origin',(-5.66257110645729E-14,12.2,-1.77635683940025E-14));
#230138=CARTESIAN_POINT('Origin',(-5.66257110645729E-14,15.2,-1.77635683940025E-14));
#230139=CARTESIAN_POINT('Origin',(-5.66257110645729E-14,15.2,-1.77635683940025E-14));
#230140=CARTESIAN_POINT('',(-2.33718477800006,15.2,11.259998549));
#230141=CARTESIAN_POINT('',(-2.71145515300006,15.2,11.175777868));
#230142=CARTESIAN_POINT('Origin',(-5.66257110645729E-14,15.2,-1.77635683940025E-14));
#230143=CARTESIAN_POINT('',(-2.71145515300006,12.2,11.175777868));
#230144=CARTESIAN_POINT('',(-2.71145515300006,15.2,11.175777868));
#230145=CARTESIAN_POINT('',(-2.33718477800006,12.2,11.259998549));
#230146=CARTESIAN_POINT('Origin',(-5.66257110645729E-14,12.2,-1.77635683940025E-14));
#230147=CARTESIAN_POINT('',(-2.33718477800006,15.2,11.259998549));
#230148=CARTESIAN_POINT('Ctrl Pts',(-2.71145515300006,15.2,11.175777868));
#230149=CARTESIAN_POINT('Ctrl Pts',(-2.71145515300006,11.6,11.175777868));
#230150=CARTESIAN_POINT('Ctrl Pts',(-2.71161876900006,15.2,11.175030994));
#230151=CARTESIAN_POINT('Ctrl Pts',(-2.71161876900006,11.6,11.175030994));
#230152=CARTESIAN_POINT('Ctrl Pts',(-2.71194562400006,15.2,11.173537618));
#230153=CARTESIAN_POINT('Ctrl Pts',(-2.71194562400006,11.6,11.173537618));
#230154=CARTESIAN_POINT('Ctrl Pts',(-2.71243478100006,15.2,11.17129866));
#230155=CARTESIAN_POINT('Ctrl Pts',(-2.71243478100006,11.6,11.17129866));
#230156=CARTESIAN_POINT('Ctrl Pts',(-2.71308473600006,15.2,11.168315598));
#230157=CARTESIAN_POINT('Ctrl Pts',(-2.71308473600006,11.6,11.168315598));
#230158=CARTESIAN_POINT('Ctrl Pts',(-2.71389342500005,15.2,11.164590464));
#230159=CARTESIAN_POINT('Ctrl Pts',(-2.71389342500005,11.6,11.164590464));
#230160=CARTESIAN_POINT('Ctrl Pts',(-2.71469835900006,15.2,11.160869024));
#230161=CARTESIAN_POINT('Ctrl Pts',(-2.71469835900006,11.6,11.160869024));
#230162=CARTESIAN_POINT('Ctrl Pts',(-2.71549953800006,15.2,11.15715128));
#230163=CARTESIAN_POINT('Ctrl Pts',(-2.71549953800006,11.6,11.15715128));
#230164=CARTESIAN_POINT('Ctrl Pts',(-2.71629696700006,15.2,11.153437237));
#230165=CARTESIAN_POINT('Ctrl Pts',(-2.71629696700006,11.6,11.153437237));
#230166=CARTESIAN_POINT('Ctrl Pts',(-2.71709064500006,15.2,11.149726898));
#230167=CARTESIAN_POINT('Ctrl Pts',(-2.71709064500006,11.6,11.149726898));
#230168=CARTESIAN_POINT('Ctrl Pts',(-2.71788057600005,15.2,11.146020271));
#230169=CARTESIAN_POINT('Ctrl Pts',(-2.71788057600005,11.6,11.146020271));
#230170=CARTESIAN_POINT('Ctrl Pts',(-2.71866676600005,15.2,11.142317366));
#230171=CARTESIAN_POINT('Ctrl Pts',(-2.71866676600005,11.6,11.142317366));
#230172=CARTESIAN_POINT('Ctrl Pts',(-2.71944921900006,15.2,11.138618192));
#230173=CARTESIAN_POINT('Ctrl Pts',(-2.71944921900006,11.6,11.138618192));
#230174=CARTESIAN_POINT('Ctrl Pts',(-2.72022794000006,15.2,11.134922759));
#230175=CARTESIAN_POINT('Ctrl Pts',(-2.72022794000006,11.6,11.134922759));
#230176=CARTESIAN_POINT('Ctrl Pts',(-2.72100293300006,15.2,11.131231076));
#230177=CARTESIAN_POINT('Ctrl Pts',(-2.72100293300006,11.6,11.131231076));
#230178=CARTESIAN_POINT('Ctrl Pts',(-2.72177420400005,15.2,11.127543154));
#230179=CARTESIAN_POINT('Ctrl Pts',(-2.72177420400005,11.6,11.127543154));
#230180=CARTESIAN_POINT('Ctrl Pts',(-2.72254175800006,15.2,11.123859));
#230181=CARTESIAN_POINT('Ctrl Pts',(-2.72254175800006,11.6,11.123859));
#230182=CARTESIAN_POINT('Ctrl Pts',(-2.72330559700006,15.2,11.120178623));
#230183=CARTESIAN_POINT('Ctrl Pts',(-2.72330559700006,11.6,11.120178623));
#230184=CARTESIAN_POINT('Ctrl Pts',(-2.72406572400006,15.2,11.116502029));
#230185=CARTESIAN_POINT('Ctrl Pts',(-2.72406572400006,11.6,11.116502029));
#230186=CARTESIAN_POINT('Ctrl Pts',(-2.72482214500006,15.2,11.112829227));
#230187=CARTESIAN_POINT('Ctrl Pts',(-2.72482214500006,11.6,11.112829227));
#230188=CARTESIAN_POINT('Ctrl Pts',(-2.72557486200005,15.2,11.109160223));
#230189=CARTESIAN_POINT('Ctrl Pts',(-2.72557486200005,11.6,11.109160223));
#230190=CARTESIAN_POINT('Ctrl Pts',(-2.72632388100006,15.2,11.105495025));
#230191=CARTESIAN_POINT('Ctrl Pts',(-2.72632388100006,11.6,11.105495025));
#230192=CARTESIAN_POINT('Ctrl Pts',(-2.72706920300006,15.2,11.10183364));
#230193=CARTESIAN_POINT('Ctrl Pts',(-2.72706920300006,11.6,11.10183364));
#230194=CARTESIAN_POINT('Ctrl Pts',(-2.72781083400006,15.2,11.098176078));
#230195=CARTESIAN_POINT('Ctrl Pts',(-2.72781083400006,11.6,11.098176078));
#230196=CARTESIAN_POINT('Ctrl Pts',(-2.72854877900006,15.2,11.094522347));
#230197=CARTESIAN_POINT('Ctrl Pts',(-2.72854877900006,11.6,11.094522347));
#230198=CARTESIAN_POINT('Ctrl Pts',(-2.72928304000006,15.2,11.090872455));
#230199=CARTESIAN_POINT('Ctrl Pts',(-2.72928304000006,11.6,11.090872455));
#230200=CARTESIAN_POINT('Ctrl Pts',(-2.73001362300006,15.2,11.087226411));
#230201=CARTESIAN_POINT('Ctrl Pts',(-2.73001362300006,11.6,11.087226411));
#230202=CARTESIAN_POINT('Ctrl Pts',(-2.73074053200005,15.2,11.083584223));
#230203=CARTESIAN_POINT('Ctrl Pts',(-2.73074053200005,11.6,11.083584223));
#230204=CARTESIAN_POINT('Ctrl Pts',(-2.73146377200006,15.2,11.0799459));
#230205=CARTESIAN_POINT('Ctrl Pts',(-2.73146377200006,11.6,11.0799459));
#230206=CARTESIAN_POINT('Ctrl Pts',(-2.73218334500006,15.2,11.076311449));
#230207=CARTESIAN_POINT('Ctrl Pts',(-2.73218334500006,11.6,11.076311449));
#230208=CARTESIAN_POINT('Ctrl Pts',(-2.73289925700006,15.2,11.072680878));
#230209=CARTESIAN_POINT('Ctrl Pts',(-2.73289925700006,11.6,11.072680878));
#230210=CARTESIAN_POINT('Ctrl Pts',(-2.73361151100006,15.2,11.069054196));
#230211=CARTESIAN_POINT('Ctrl Pts',(-2.73361151100006,11.6,11.069054196));
#230212=CARTESIAN_POINT('Ctrl Pts',(-2.73432011200006,15.2,11.065431411));
#230213=CARTESIAN_POINT('Ctrl Pts',(-2.73432011200006,11.6,11.065431411));
#230214=CARTESIAN_POINT('Ctrl Pts',(-2.73502506400006,15.2,11.06181253));
#230215=CARTESIAN_POINT('Ctrl Pts',(-2.73502506400006,11.6,11.06181253));
#230216=CARTESIAN_POINT('Ctrl Pts',(-2.73572637100005,15.2,11.058197563));
#230217=CARTESIAN_POINT('Ctrl Pts',(-2.73572637100005,11.6,11.058197563));
#230218=CARTESIAN_POINT('Ctrl Pts',(-2.73642403700005,15.2,11.054586517));
#230219=CARTESIAN_POINT('Ctrl Pts',(-2.73642403700005,11.6,11.054586517));
#230220=CARTESIAN_POINT('Ctrl Pts',(-2.73711806800006,15.2,11.050979401));
#230221=CARTESIAN_POINT('Ctrl Pts',(-2.73711806800006,11.6,11.050979401));
#230222=CARTESIAN_POINT('Ctrl Pts',(-2.73780846600005,15.2,11.047376223));
#230223=CARTESIAN_POINT('Ctrl Pts',(-2.73780846600005,11.6,11.047376223));
#230224=CARTESIAN_POINT('Ctrl Pts',(-2.73849523700005,15.2,11.043776991));
#230225=CARTESIAN_POINT('Ctrl Pts',(-2.73849523700005,11.6,11.043776991));
#230226=CARTESIAN_POINT('Ctrl Pts',(-2.73917838500005,15.2,11.040181715));
#230227=CARTESIAN_POINT('Ctrl Pts',(-2.73917838500005,11.6,11.040181715));
#230228=CARTESIAN_POINT('Ctrl Pts',(-2.73985791300006,15.2,11.036590401));
#230229=CARTESIAN_POINT('Ctrl Pts',(-2.73985791300006,11.6,11.036590401));
#230230=CARTESIAN_POINT('Ctrl Pts',(-2.74053382800005,15.2,11.033003059));
#230231=CARTESIAN_POINT('Ctrl Pts',(-2.74053382800005,11.6,11.033003059));
#230232=CARTESIAN_POINT('Ctrl Pts',(-2.74120613200005,15.2,11.029419696));
#230233=CARTESIAN_POINT('Ctrl Pts',(-2.74120613200005,11.6,11.029419696));
#230234=CARTESIAN_POINT('Ctrl Pts',(-2.74187483100006,15.2,11.025840322));
#230235=CARTESIAN_POINT('Ctrl Pts',(-2.74187483100006,11.6,11.025840322));
#230236=CARTESIAN_POINT('Ctrl Pts',(-2.74253992800006,15.2,11.022264944));
#230237=CARTESIAN_POINT('Ctrl Pts',(-2.74253992800006,11.6,11.022264944));
#230238=CARTESIAN_POINT('Ctrl Pts',(-2.74320142800006,15.2,11.01869357));
#230239=CARTESIAN_POINT('Ctrl Pts',(-2.74320142800006,11.6,11.01869357));
#230240=CARTESIAN_POINT('Ctrl Pts',(-2.74385933600006,15.2,11.015126211));
#230241=CARTESIAN_POINT('Ctrl Pts',(-2.74385933600006,11.6,11.015126211));
#230242=CARTESIAN_POINT('Ctrl Pts',(-2.74451365600005,15.2,11.011562872));
#230243=CARTESIAN_POINT('Ctrl Pts',(-2.74451365600005,11.6,11.011562872));
#230244=CARTESIAN_POINT('Ctrl Pts',(-2.74516439300006,15.2,11.008003564));
#230245=CARTESIAN_POINT('Ctrl Pts',(-2.74516439300006,11.6,11.008003564));
#230246=CARTESIAN_POINT('Ctrl Pts',(-2.74581155000006,15.2,11.004448294));
#230247=CARTESIAN_POINT('Ctrl Pts',(-2.74581155000006,11.6,11.004448294));
#230248=CARTESIAN_POINT('Ctrl Pts',(-2.74645513200006,15.2,11.00089707));
#230249=CARTESIAN_POINT('Ctrl Pts',(-2.74645513200006,11.6,11.00089707));
#230250=CARTESIAN_POINT('Ctrl Pts',(-2.74709514500006,15.2,10.997349902));
#230251=CARTESIAN_POINT('Ctrl Pts',(-2.74709514500006,11.6,10.997349902));
#230252=CARTESIAN_POINT('Ctrl Pts',(-2.74773159200006,15.2,10.993806798));
#230253=CARTESIAN_POINT('Ctrl Pts',(-2.74773159200006,11.6,10.993806798));
#230254=CARTESIAN_POINT('Ctrl Pts',(-2.74836447800006,15.2,10.990267766));
#230255=CARTESIAN_POINT('Ctrl Pts',(-2.74836447800006,11.6,10.990267766));
#230256=CARTESIAN_POINT('Ctrl Pts',(-2.74899380800006,15.2,10.986732814));
#230257=CARTESIAN_POINT('Ctrl Pts',(-2.74899380800006,11.6,10.986732814));
#230258=CARTESIAN_POINT('Ctrl Pts',(-2.74961958600006,15.2,10.983201952));
#230259=CARTESIAN_POINT('Ctrl Pts',(-2.74961958600006,11.6,10.983201952));
#230260=CARTESIAN_POINT('Ctrl Pts',(-2.75024181600006,15.2,10.979675187));
#230261=CARTESIAN_POINT('Ctrl Pts',(-2.75024181600006,11.6,10.979675187));
#230262=CARTESIAN_POINT('Ctrl Pts',(-2.75086050500006,15.2,10.976152528));
#230263=CARTESIAN_POINT('Ctrl Pts',(-2.75086050500006,11.6,10.976152528));
#230264=CARTESIAN_POINT('Ctrl Pts',(-2.75147565400006,15.2,10.972633985));
#230265=CARTESIAN_POINT('Ctrl Pts',(-2.75147565400006,11.6,10.972633985));
#230266=CARTESIAN_POINT('Ctrl Pts',(-2.75208727000006,15.2,10.969119564));
#230267=CARTESIAN_POINT('Ctrl Pts',(-2.75208727000006,11.6,10.969119564));
#230268=CARTESIAN_POINT('Ctrl Pts',(-2.75269535800006,15.2,10.965609275));
#230269=CARTESIAN_POINT('Ctrl Pts',(-2.75269535800006,11.6,10.965609275));
#230270=CARTESIAN_POINT('Ctrl Pts',(-2.75329992200006,15.2,10.962103126));
#230271=CARTESIAN_POINT('Ctrl Pts',(-2.75329992200006,11.6,10.962103126));
#230272=CARTESIAN_POINT('Ctrl Pts',(-2.75390096500006,15.2,10.958601125));
#230273=CARTESIAN_POINT('Ctrl Pts',(-2.75390096500006,11.6,10.958601125));
#230274=CARTESIAN_POINT('Ctrl Pts',(-2.75449849500006,15.2,10.955103284));
#230275=CARTESIAN_POINT('Ctrl Pts',(-2.75449849500006,11.6,10.955103284));
#230276=CARTESIAN_POINT('Ctrl Pts',(-2.75509251400006,15.2,10.951609606));
#230277=CARTESIAN_POINT('Ctrl Pts',(-2.75509251400006,11.6,10.951609606));
#230278=CARTESIAN_POINT('Ctrl Pts',(-2.75568302800006,15.2,10.948120105));
#230279=CARTESIAN_POINT('Ctrl Pts',(-2.75568302800006,11.6,10.948120105));
#230280=CARTESIAN_POINT('Ctrl Pts',(-2.75627004200006,15.2,10.944634786));
#230281=CARTESIAN_POINT('Ctrl Pts',(-2.75627004200006,11.6,10.944634786));
#230282=CARTESIAN_POINT('Ctrl Pts',(-2.75685355900006,15.2,10.941153659));
#230283=CARTESIAN_POINT('Ctrl Pts',(-2.75685355900006,11.6,10.941153659));
#230284=CARTESIAN_POINT('Ctrl Pts',(-2.75743358600006,15.2,10.937676733));
#230285=CARTESIAN_POINT('Ctrl Pts',(-2.75743358600006,11.6,10.937676733));
#230286=CARTESIAN_POINT('Ctrl Pts',(-2.75801012600006,15.2,10.934204015));
#230287=CARTESIAN_POINT('Ctrl Pts',(-2.75801012600006,11.6,10.934204015));
#230288=CARTESIAN_POINT('Ctrl Pts',(-2.75858318400005,15.2,10.930735515));
#230289=CARTESIAN_POINT('Ctrl Pts',(-2.75858318400005,11.6,10.930735515));
#230290=CARTESIAN_POINT('Ctrl Pts',(-2.75915276600006,15.2,10.927271243));
#230291=CARTESIAN_POINT('Ctrl Pts',(-2.75915276600006,11.6,10.927271243));
#230292=CARTESIAN_POINT('Ctrl Pts',(-2.75971887700006,15.2,10.923811204));
#230293=CARTESIAN_POINT('Ctrl Pts',(-2.75971887700006,11.6,10.923811204));
#230294=CARTESIAN_POINT('Ctrl Pts',(-2.76028152000006,15.2,10.92035541));
#230295=CARTESIAN_POINT('Ctrl Pts',(-2.76028152000006,11.6,10.92035541));
#230296=CARTESIAN_POINT('Ctrl Pts',(-2.76084070100006,15.2,10.916903869));
#230297=CARTESIAN_POINT('Ctrl Pts',(-2.76084070100006,11.6,10.916903869));
#230298=CARTESIAN_POINT('Ctrl Pts',(-2.76139642500006,15.2,10.913456588));
#230299=CARTESIAN_POINT('Ctrl Pts',(-2.76139642500006,11.6,10.913456588));
#230300=CARTESIAN_POINT('Ctrl Pts',(-2.76194869600006,15.2,10.910013578));
#230301=CARTESIAN_POINT('Ctrl Pts',(-2.76194869600006,11.6,10.910013578));
#230302=CARTESIAN_POINT('Ctrl Pts',(-2.76249752100005,15.2,10.906574846));
#230303=CARTESIAN_POINT('Ctrl Pts',(-2.76249752100005,11.6,10.906574846));
#230304=CARTESIAN_POINT('Ctrl Pts',(-2.76304290200006,15.2,10.903140402));
#230305=CARTESIAN_POINT('Ctrl Pts',(-2.76304290200006,11.6,10.903140402));
#230306=CARTESIAN_POINT('Ctrl Pts',(-2.76358484700005,15.2,10.899710254));
#230307=CARTESIAN_POINT('Ctrl Pts',(-2.76358484700005,11.6,10.899710254));
#230308=CARTESIAN_POINT('Ctrl Pts',(-2.76412335700006,15.2,10.896284411));
#230309=CARTESIAN_POINT('Ctrl Pts',(-2.76412335700006,11.6,10.896284411));
#230310=CARTESIAN_POINT('Ctrl Pts',(-2.76465844200006,15.2,10.892862881));
#230311=CARTESIAN_POINT('Ctrl Pts',(-2.76465844200006,11.6,10.892862881));
#230312=CARTESIAN_POINT('Ctrl Pts',(-2.76519010400006,15.2,10.889445675));
#230313=CARTESIAN_POINT('Ctrl Pts',(-2.76519010400006,11.6,10.889445675));
#230314=CARTESIAN_POINT('Ctrl Pts',(-2.76571834700006,15.2,10.8860328));
#230315=CARTESIAN_POINT('Ctrl Pts',(-2.76571834700006,11.6,10.8860328));
#230316=CARTESIAN_POINT('Ctrl Pts',(-2.76624317800006,15.2,10.882624266));
#230317=CARTESIAN_POINT('Ctrl Pts',(-2.76624317800006,11.6,10.882624266));
#230318=CARTESIAN_POINT('Ctrl Pts',(-2.76676460200005,15.2,10.87922008));
#230319=CARTESIAN_POINT('Ctrl Pts',(-2.76676460200005,11.6,10.87922008));
#230320=CARTESIAN_POINT('Ctrl Pts',(-2.76728262300006,15.2,10.875820252));
#230321=CARTESIAN_POINT('Ctrl Pts',(-2.76728262300006,11.6,10.875820252));
#230322=CARTESIAN_POINT('Ctrl Pts',(-2.76779724800006,15.2,10.872424791));
#230323=CARTESIAN_POINT('Ctrl Pts',(-2.76779724800006,11.6,10.872424791));
#230324=CARTESIAN_POINT('Ctrl Pts',(-2.76830847900006,15.2,10.869033706));
#230325=CARTESIAN_POINT('Ctrl Pts',(-2.76830847900006,11.6,10.869033706));
#230326=CARTESIAN_POINT('Ctrl Pts',(-2.76881632300006,15.2,10.865647005));
#230327=CARTESIAN_POINT('Ctrl Pts',(-2.76881632300006,11.6,10.865647005));
#230328=CARTESIAN_POINT('Ctrl Pts',(-2.76932078600006,15.2,10.862264699));
#230329=CARTESIAN_POINT('Ctrl Pts',(-2.76932078600006,11.6,10.862264699));
#230330=CARTESIAN_POINT('Ctrl Pts',(-2.76982187200006,15.2,10.858886794));
#230331=CARTESIAN_POINT('Ctrl Pts',(-2.76982187200006,11.6,10.858886794));
#230332=CARTESIAN_POINT('Ctrl Pts',(-2.77031958500006,15.2,10.855513301));
#230333=CARTESIAN_POINT('Ctrl Pts',(-2.77031958500006,11.6,10.855513301));
#230334=CARTESIAN_POINT('Ctrl Pts',(-2.77081393200006,15.2,10.852144229));
#230335=CARTESIAN_POINT('Ctrl Pts',(-2.77081393200006,11.6,10.852144229));
#230336=CARTESIAN_POINT('Ctrl Pts',(-2.77130491800006,15.2,10.848779585));
#230337=CARTESIAN_POINT('Ctrl Pts',(-2.77130491800006,11.6,10.848779585));
#230338=CARTESIAN_POINT('Ctrl Pts',(-2.77179254800005,15.2,10.845419379));
#230339=CARTESIAN_POINT('Ctrl Pts',(-2.77179254800005,11.6,10.845419379));
#230340=CARTESIAN_POINT('Ctrl Pts',(-2.77227682700006,15.2,10.842063621));
#230341=CARTESIAN_POINT('Ctrl Pts',(-2.77227682700006,11.6,10.842063621));
#230342=CARTESIAN_POINT('Ctrl Pts',(-2.77275776000006,15.2,10.838712319));
#230343=CARTESIAN_POINT('Ctrl Pts',(-2.77275776000006,11.6,10.838712319));
#230344=CARTESIAN_POINT('Ctrl Pts',(-2.77323535300006,15.2,10.835365483));
#230345=CARTESIAN_POINT('Ctrl Pts',(-2.77323535300006,11.6,10.835365483));
#230346=CARTESIAN_POINT('Ctrl Pts',(-2.77370961000006,15.2,10.83202312));
#230347=CARTESIAN_POINT('Ctrl Pts',(-2.77370961000006,11.6,10.83202312));
#230348=CARTESIAN_POINT('Ctrl Pts',(-2.77418053800006,15.2,10.828685241));
#230349=CARTESIAN_POINT('Ctrl Pts',(-2.77418053800006,11.6,10.828685241));
#230350=CARTESIAN_POINT('Ctrl Pts',(-2.77464814200005,15.2,10.825351855));
#230351=CARTESIAN_POINT('Ctrl Pts',(-2.77464814200005,11.6,10.825351855));
#230352=CARTESIAN_POINT('Ctrl Pts',(-2.77511242500006,15.2,10.822022969));
#230353=CARTESIAN_POINT('Ctrl Pts',(-2.77511242500006,11.6,10.822022969));
#230354=CARTESIAN_POINT('Ctrl Pts',(-2.77557339600006,15.2,10.818698594));
#230355=CARTESIAN_POINT('Ctrl Pts',(-2.77557339600006,11.6,10.818698594));
#230356=CARTESIAN_POINT('Ctrl Pts',(-2.77603105800006,15.2,10.815378739));
#230357=CARTESIAN_POINT('Ctrl Pts',(-2.77603105800006,11.6,10.815378739));
#230358=CARTESIAN_POINT('Ctrl Pts',(-2.77648541700006,15.2,10.812063413));
#230359=CARTESIAN_POINT('Ctrl Pts',(-2.77648541700006,11.6,10.812063413));
#230360=CARTESIAN_POINT('Ctrl Pts',(-2.77693647800006,15.2,10.808752625));
#230361=CARTESIAN_POINT('Ctrl Pts',(-2.77693647800006,11.6,10.808752625));
#230362=CARTESIAN_POINT('Ctrl Pts',(-2.77738424800006,15.2,10.805446383));
#230363=CARTESIAN_POINT('Ctrl Pts',(-2.77738424800006,11.6,10.805446383));
#230364=CARTESIAN_POINT('Ctrl Pts',(-2.77782872900006,15.2,10.802144697));
#230365=CARTESIAN_POINT('Ctrl Pts',(-2.77782872900006,11.6,10.802144697));
#230366=CARTESIAN_POINT('Ctrl Pts',(-2.77826993000006,15.2,10.798847577));
#230367=CARTESIAN_POINT('Ctrl Pts',(-2.77826993000006,11.6,10.798847577));
#230368=CARTESIAN_POINT('Ctrl Pts',(-2.77870785500005,15.2,10.795555031));
#230369=CARTESIAN_POINT('Ctrl Pts',(-2.77870785500005,11.6,10.795555031));
#230370=CARTESIAN_POINT('Ctrl Pts',(-2.77914251100006,15.2,10.792267068));
#230371=CARTESIAN_POINT('Ctrl Pts',(-2.77914251100006,11.6,10.792267068));
#230372=CARTESIAN_POINT('Ctrl Pts',(-2.77957390000005,15.2,10.788983699));
#230373=CARTESIAN_POINT('Ctrl Pts',(-2.77957390000005,11.6,10.788983699));
#230374=CARTESIAN_POINT('Ctrl Pts',(-2.78000203100006,15.2,10.785704931));
#230375=CARTESIAN_POINT('Ctrl Pts',(-2.78000203100006,11.6,10.785704931));
#230376=CARTESIAN_POINT('Ctrl Pts',(-2.78042690800006,15.2,10.782430774));
#230377=CARTESIAN_POINT('Ctrl Pts',(-2.78042690800006,11.6,10.782430774));
#230378=CARTESIAN_POINT('Ctrl Pts',(-2.78084853700005,15.2,10.779161239));
#230379=CARTESIAN_POINT('Ctrl Pts',(-2.78084853700005,11.6,10.779161239));
#230380=CARTESIAN_POINT('Ctrl Pts',(-2.78126692300006,15.2,10.775896333));
#230381=CARTESIAN_POINT('Ctrl Pts',(-2.78126692300006,11.6,10.775896333));
#230382=CARTESIAN_POINT('Ctrl Pts',(-2.78168207300005,15.2,10.772636066));
#230383=CARTESIAN_POINT('Ctrl Pts',(-2.78168207300005,11.6,10.772636066));
#230384=CARTESIAN_POINT('Ctrl Pts',(-2.78209399200006,15.2,10.769380447));
#230385=CARTESIAN_POINT('Ctrl Pts',(-2.78209399200006,11.6,10.769380447));
#230386=CARTESIAN_POINT('Ctrl Pts',(-2.78250268400006,15.2,10.766129486));
#230387=CARTESIAN_POINT('Ctrl Pts',(-2.78250268400006,11.6,10.766129486));
#230388=CARTESIAN_POINT('Ctrl Pts',(-2.78290815600006,15.2,10.762883192));
#230389=CARTESIAN_POINT('Ctrl Pts',(-2.78290815600006,11.6,10.762883192));
#230390=CARTESIAN_POINT('Ctrl Pts',(-2.78331041400006,15.2,10.759641574));
#230391=CARTESIAN_POINT('Ctrl Pts',(-2.78331041400006,11.6,10.759641574));
#230392=CARTESIAN_POINT('Ctrl Pts',(-2.78370946300006,15.2,10.756404641));
#230393=CARTESIAN_POINT('Ctrl Pts',(-2.78370946300006,11.6,10.756404641));
#230394=CARTESIAN_POINT('Ctrl Pts',(-2.78410531000006,15.2,10.753172404));
#230395=CARTESIAN_POINT('Ctrl Pts',(-2.78410531000006,11.6,10.753172404));
#230396=CARTESIAN_POINT('Ctrl Pts',(-2.78449795900006,15.2,10.749944871));
#230397=CARTESIAN_POINT('Ctrl Pts',(-2.78449795900006,11.6,10.749944871));
#230398=CARTESIAN_POINT('Ctrl Pts',(-2.78488741700006,15.2,10.746722052));
#230399=CARTESIAN_POINT('Ctrl Pts',(-2.78488741700006,11.6,10.746722052));
#230400=CARTESIAN_POINT('Ctrl Pts',(-2.78527368900006,15.2,10.743503955));
#230401=CARTESIAN_POINT('Ctrl Pts',(-2.78527368900006,11.6,10.743503955));
#230402=CARTESIAN_POINT('Ctrl Pts',(-2.78565678100006,15.2,10.740290591));
#230403=CARTESIAN_POINT('Ctrl Pts',(-2.78565678100006,11.6,10.740290591));
#230404=CARTESIAN_POINT('Ctrl Pts',(-2.78603670000006,15.2,10.73708197));
#230405=CARTESIAN_POINT('Ctrl Pts',(-2.78603670000006,11.6,10.73708197));
#230406=CARTESIAN_POINT('Ctrl Pts',(-2.78641345100006,15.2,10.7338781));
#230407=CARTESIAN_POINT('Ctrl Pts',(-2.78641345100006,11.6,10.7338781));
#230408=CARTESIAN_POINT('Ctrl Pts',(-2.78678703800006,15.2,10.73067899));
#230409=CARTESIAN_POINT('Ctrl Pts',(-2.78678703800006,11.6,10.73067899));
#230410=CARTESIAN_POINT('Ctrl Pts',(-2.78715746900006,15.2,10.727484651));
#230411=CARTESIAN_POINT('Ctrl Pts',(-2.78715746900006,11.6,10.727484651));
#230412=CARTESIAN_POINT('Ctrl Pts',(-2.78752475100006,15.2,10.724295092));
#230413=CARTESIAN_POINT('Ctrl Pts',(-2.78752475100006,11.6,10.724295092));
#230414=CARTESIAN_POINT('Ctrl Pts',(-2.78788888700006,15.2,10.721110321));
#230415=CARTESIAN_POINT('Ctrl Pts',(-2.78788888700006,11.6,10.721110321));
#230416=CARTESIAN_POINT('Ctrl Pts',(-2.78824988500005,15.2,10.71793035));
#230417=CARTESIAN_POINT('Ctrl Pts',(-2.78824988500005,11.6,10.71793035));
#230418=CARTESIAN_POINT('Ctrl Pts',(-2.78860774900005,15.2,10.714755188));
#230419=CARTESIAN_POINT('Ctrl Pts',(-2.78860774900005,11.6,10.714755188));
#230420=CARTESIAN_POINT('Ctrl Pts',(-2.78896248700006,15.2,10.711584842));
#230421=CARTESIAN_POINT('Ctrl Pts',(-2.78896248700006,11.6,10.711584842));
#230422=CARTESIAN_POINT('Ctrl Pts',(-2.78931410500005,15.2,10.708419325));
#230423=CARTESIAN_POINT('Ctrl Pts',(-2.78931410500005,11.6,10.708419325));
#230424=CARTESIAN_POINT('Ctrl Pts',(-2.78966260700006,15.2,10.705258645));
#230425=CARTESIAN_POINT('Ctrl Pts',(-2.78966260700006,11.6,10.705258645));
#230426=CARTESIAN_POINT('Ctrl Pts',(-2.79000800100006,15.2,10.702102811));
#230427=CARTESIAN_POINT('Ctrl Pts',(-2.79000800100006,11.6,10.702102811));
#230428=CARTESIAN_POINT('Ctrl Pts',(-2.79035029200006,15.2,10.698951833));
#230429=CARTESIAN_POINT('Ctrl Pts',(-2.79035029200006,11.6,10.698951833));
#230430=CARTESIAN_POINT('Ctrl Pts',(-2.79068948600006,15.2,10.695805722));
#230431=CARTESIAN_POINT('Ctrl Pts',(-2.79068948600006,11.6,10.695805722));
#230432=CARTESIAN_POINT('Ctrl Pts',(-2.79102559000005,15.2,10.692664486));
#230433=CARTESIAN_POINT('Ctrl Pts',(-2.79102559000005,11.6,10.692664486));
#230434=CARTESIAN_POINT('Ctrl Pts',(-2.79135860900006,15.2,10.689528136));
#230435=CARTESIAN_POINT('Ctrl Pts',(-2.79135860900006,11.6,10.689528136));
#230436=CARTESIAN_POINT('Ctrl Pts',(-2.79168855100006,15.2,10.68639668));
#230437=CARTESIAN_POINT('Ctrl Pts',(-2.79168855100006,11.6,10.68639668));
#230438=CARTESIAN_POINT('Ctrl Pts',(-2.79201542000005,15.2,10.683270128));
#230439=CARTESIAN_POINT('Ctrl Pts',(-2.79201542000005,11.6,10.683270128));
#230440=CARTESIAN_POINT('Ctrl Pts',(-2.79233922300006,15.2,10.680148491));
#230441=CARTESIAN_POINT('Ctrl Pts',(-2.79233922300006,11.6,10.680148491));
#230442=CARTESIAN_POINT('Ctrl Pts',(-2.79265996700006,15.2,10.677031779));
#230443=CARTESIAN_POINT('Ctrl Pts',(-2.79265996700006,11.6,10.677031779));
#230444=CARTESIAN_POINT('Ctrl Pts',(-2.79297765700006,15.2,10.67392));
#230445=CARTESIAN_POINT('Ctrl Pts',(-2.79297765700006,11.6,10.67392));
#230446=CARTESIAN_POINT('Ctrl Pts',(-2.79329230000006,15.2,10.670813164));
#230447=CARTESIAN_POINT('Ctrl Pts',(-2.79329230000006,11.6,10.670813164));
#230448=CARTESIAN_POINT('Ctrl Pts',(-2.79360390200006,15.2,10.667711281));
#230449=CARTESIAN_POINT('Ctrl Pts',(-2.79360390200006,11.6,10.667711281));
#230450=CARTESIAN_POINT('Ctrl Pts',(-2.79391246900006,15.2,10.664614362));
#230451=CARTESIAN_POINT('Ctrl Pts',(-2.79391246900006,11.6,10.664614362));
#230452=CARTESIAN_POINT('Ctrl Pts',(-2.79421800800006,15.2,10.661522415));
#230453=CARTESIAN_POINT('Ctrl Pts',(-2.79421800800006,11.6,10.661522415));
#230454=CARTESIAN_POINT('Ctrl Pts',(-2.79452052500006,15.2,10.658435452));
#230455=CARTESIAN_POINT('Ctrl Pts',(-2.79452052500006,11.6,10.658435452));
#230456=CARTESIAN_POINT('Ctrl Pts',(-2.79482002600006,15.2,10.655353481));
#230457=CARTESIAN_POINT('Ctrl Pts',(-2.79482002600006,11.6,10.655353481));
#230458=CARTESIAN_POINT('Ctrl Pts',(-2.79511651700005,15.2,10.652276512));
#230459=CARTESIAN_POINT('Ctrl Pts',(-2.79511651700005,11.6,10.652276512));
#230460=CARTESIAN_POINT('Ctrl Pts',(-2.79541000600006,15.2,10.649204555));
#230461=CARTESIAN_POINT('Ctrl Pts',(-2.79541000600006,11.6,10.649204555));
#230462=CARTESIAN_POINT('Ctrl Pts',(-2.79570049800005,15.2,10.64613762));
#230463=CARTESIAN_POINT('Ctrl Pts',(-2.79570049800005,11.6,10.64613762));
#230464=CARTESIAN_POINT('Ctrl Pts',(-2.79598799900006,15.2,10.643075718));
#230465=CARTESIAN_POINT('Ctrl Pts',(-2.79598799900006,11.6,10.643075718));
#230466=CARTESIAN_POINT('Ctrl Pts',(-2.79627251800005,15.2,10.640018857));
#230467=CARTESIAN_POINT('Ctrl Pts',(-2.79627251800005,11.6,10.640018857));
#230468=CARTESIAN_POINT('Ctrl Pts',(-2.79655405900006,15.2,10.636967049));
#230469=CARTESIAN_POINT('Ctrl Pts',(-2.79655405900006,11.6,10.636967049));
#230470=CARTESIAN_POINT('Ctrl Pts',(-2.79683262900006,15.2,10.633920302));
#230471=CARTESIAN_POINT('Ctrl Pts',(-2.79683262900006,11.6,10.633920302));
#230472=CARTESIAN_POINT('Ctrl Pts',(-2.79710823600006,15.2,10.630878627));
#230473=CARTESIAN_POINT('Ctrl Pts',(-2.79710823600006,11.6,10.630878627));
#230474=CARTESIAN_POINT('Ctrl Pts',(-2.79738088300005,15.2,10.627842034));
#230475=CARTESIAN_POINT('Ctrl Pts',(-2.79738088300005,11.6,10.627842034));
#230476=CARTESIAN_POINT('Ctrl Pts',(-2.79765058100006,15.2,10.624810531));
#230477=CARTESIAN_POINT('Ctrl Pts',(-2.79765058100006,11.6,10.624810531));
#230478=CARTESIAN_POINT('Ctrl Pts',(-2.79791733400006,15.2,10.621784132));
#230479=CARTESIAN_POINT('Ctrl Pts',(-2.79791733400006,11.6,10.621784132));
#230480=CARTESIAN_POINT('Ctrl Pts',(-2.79818114900006,15.2,10.618762845));
#230481=CARTESIAN_POINT('Ctrl Pts',(-2.79818114900006,11.6,10.618762845));
#230482=CARTESIAN_POINT('Ctrl Pts',(-2.79844203300006,15.2,10.615746678));
#230483=CARTESIAN_POINT('Ctrl Pts',(-2.79844203300006,11.6,10.615746678));
#230484=CARTESIAN_POINT('Ctrl Pts',(-2.79869999200006,15.2,10.612735644));
#230485=CARTESIAN_POINT('Ctrl Pts',(-2.79869999200006,11.6,10.612735644));
#230486=CARTESIAN_POINT('Ctrl Pts',(-2.79895503300006,15.2,10.609729752));
#230487=CARTESIAN_POINT('Ctrl Pts',(-2.79895503300006,11.6,10.609729752));
#230488=CARTESIAN_POINT('Ctrl Pts',(-2.79920716400006,15.2,10.606729013));
#230489=CARTESIAN_POINT('Ctrl Pts',(-2.79920716400006,11.6,10.606729013));
#230490=CARTESIAN_POINT('Ctrl Pts',(-2.79945638900006,15.2,10.603733435));
#230491=CARTESIAN_POINT('Ctrl Pts',(-2.79945638900006,11.6,10.603733435));
#230492=CARTESIAN_POINT('Ctrl Pts',(-2.79970271700006,15.2,10.60074303));
#230493=CARTESIAN_POINT('Ctrl Pts',(-2.79970271700006,11.6,10.60074303));
#230494=CARTESIAN_POINT('Ctrl Pts',(-2.79994615400006,15.2,10.597757808));
#230495=CARTESIAN_POINT('Ctrl Pts',(-2.79994615400006,11.6,10.597757808));
#230496=CARTESIAN_POINT('Ctrl Pts',(-2.80018670700006,15.2,10.594777778));
#230497=CARTESIAN_POINT('Ctrl Pts',(-2.80018670700006,11.6,10.594777778));
#230498=CARTESIAN_POINT('Ctrl Pts',(-2.80042438200006,15.2,10.591802951));
#230499=CARTESIAN_POINT('Ctrl Pts',(-2.80042438200006,11.6,10.591802951));
#230500=CARTESIAN_POINT('Ctrl Pts',(-2.80065918600005,15.2,10.588833338));
#230501=CARTESIAN_POINT('Ctrl Pts',(-2.80065918600005,11.6,10.588833338));
#230502=CARTESIAN_POINT('Ctrl Pts',(-2.80089112800006,15.2,10.585868947));
#230503=CARTESIAN_POINT('Ctrl Pts',(-2.80089112800006,11.6,10.585868947));
#230504=CARTESIAN_POINT('Ctrl Pts',(-2.80112021200006,15.2,10.582909791));
#230505=CARTESIAN_POINT('Ctrl Pts',(-2.80112021200006,11.6,10.582909791));
#230506=CARTESIAN_POINT('Ctrl Pts',(-2.80134644700006,15.2,10.579955878));
#230507=CARTESIAN_POINT('Ctrl Pts',(-2.80134644700006,11.6,10.579955878));
#230508=CARTESIAN_POINT('Ctrl Pts',(-2.80156983900006,15.2,10.57700722));
#230509=CARTESIAN_POINT('Ctrl Pts',(-2.80156983900006,11.6,10.57700722));
#230510=CARTESIAN_POINT('Ctrl Pts',(-2.80179039400006,15.2,10.574063826));
#230511=CARTESIAN_POINT('Ctrl Pts',(-2.80179039400006,11.6,10.574063826));
#230512=CARTESIAN_POINT('Ctrl Pts',(-2.80200812100006,15.2,10.571125707));
#230513=CARTESIAN_POINT('Ctrl Pts',(-2.80200812100006,11.6,10.571125707));
#230514=CARTESIAN_POINT('Ctrl Pts',(-2.80222302600006,15.2,10.568192874));
#230515=CARTESIAN_POINT('Ctrl Pts',(-2.80222302600006,11.6,10.568192874));
#230516=CARTESIAN_POINT('Ctrl Pts',(-2.80243511500006,15.2,10.565265335));
#230517=CARTESIAN_POINT('Ctrl Pts',(-2.80243511500006,11.6,10.565265335));
#230518=CARTESIAN_POINT('Ctrl Pts',(-2.80264439700006,15.2,10.562343103));
#230519=CARTESIAN_POINT('Ctrl Pts',(-2.80264439700006,11.6,10.562343103));
#230520=CARTESIAN_POINT('Ctrl Pts',(-2.80285087800006,15.2,10.559426187));
#230521=CARTESIAN_POINT('Ctrl Pts',(-2.80285087800006,11.6,10.559426187));
#230522=CARTESIAN_POINT('Ctrl Pts',(-2.80305456500006,15.2,10.556514597));
#230523=CARTESIAN_POINT('Ctrl Pts',(-2.80305456500006,11.6,10.556514597));
#230524=CARTESIAN_POINT('Ctrl Pts',(-2.80325546600006,15.2,10.553608346));
#230525=CARTESIAN_POINT('Ctrl Pts',(-2.80325546600006,11.6,10.553608346));
#230526=CARTESIAN_POINT('Ctrl Pts',(-2.80345358700006,15.2,10.550707441));
#230527=CARTESIAN_POINT('Ctrl Pts',(-2.80345358700006,11.6,10.550707441));
#230528=CARTESIAN_POINT('Ctrl Pts',(-2.80364893600006,15.2,10.547811894));
#230529=CARTESIAN_POINT('Ctrl Pts',(-2.80364893600006,11.6,10.547811894));
#230530=CARTESIAN_POINT('Ctrl Pts',(-2.80384152000006,15.2,10.544921717));
#230531=CARTESIAN_POINT('Ctrl Pts',(-2.80384152000006,11.6,10.544921717));
#230532=CARTESIAN_POINT('Ctrl Pts',(-2.80403134500005,15.2,10.542036918));
#230533=CARTESIAN_POINT('Ctrl Pts',(-2.80403134500005,11.6,10.542036918));
#230534=CARTESIAN_POINT('Ctrl Pts',(-2.80421842000006,15.2,10.539157509));
#230535=CARTESIAN_POINT('Ctrl Pts',(-2.80421842000006,11.6,10.539157509));
#230536=CARTESIAN_POINT('Ctrl Pts',(-2.80440275200006,15.2,10.5362835));
#230537=CARTESIAN_POINT('Ctrl Pts',(-2.80440275200006,11.6,10.5362835));
#230538=CARTESIAN_POINT('Ctrl Pts',(-2.80458434800006,15.2,10.533414902));
#230539=CARTESIAN_POINT('Ctrl Pts',(-2.80458434800006,11.6,10.533414902));
#230540=CARTESIAN_POINT('Ctrl Pts',(-2.80476321500006,15.2,10.530551726));
#230541=CARTESIAN_POINT('Ctrl Pts',(-2.80476321500006,11.6,10.530551726));
#230542=CARTESIAN_POINT('Ctrl Pts',(-2.80493936200005,15.2,10.52769398));
#230543=CARTESIAN_POINT('Ctrl Pts',(-2.80493936200005,11.6,10.52769398));
#230544=CARTESIAN_POINT('Ctrl Pts',(-2.80511279300006,15.2,10.524841678));
#230545=CARTESIAN_POINT('Ctrl Pts',(-2.80511279300006,11.6,10.524841678));
#230546=CARTESIAN_POINT('Ctrl Pts',(-2.80528351900006,15.2,10.52199483));
#230547=CARTESIAN_POINT('Ctrl Pts',(-2.80528351900006,11.6,10.52199483));
#230548=CARTESIAN_POINT('Ctrl Pts',(-2.80545154500006,15.2,10.519153444));
#230549=CARTESIAN_POINT('Ctrl Pts',(-2.80545154500006,11.6,10.519153444));
#230550=CARTESIAN_POINT('Ctrl Pts',(-2.80561687900006,15.2,10.516317534));
#230551=CARTESIAN_POINT('Ctrl Pts',(-2.80561687900006,11.6,10.516317534));
#230552=CARTESIAN_POINT('Ctrl Pts',(-2.80577953000006,15.2,10.513487108));
#230553=CARTESIAN_POINT('Ctrl Pts',(-2.80577953000006,11.6,10.513487108));
#230554=CARTESIAN_POINT('Ctrl Pts',(-2.80593950400006,15.2,10.510662179));
#230555=CARTESIAN_POINT('Ctrl Pts',(-2.80593950400006,11.6,10.510662179));
#230556=CARTESIAN_POINT('Ctrl Pts',(-2.80609680800006,15.2,10.507842757));
#230557=CARTESIAN_POINT('Ctrl Pts',(-2.80609680800006,11.6,10.507842757));
#230558=CARTESIAN_POINT('Ctrl Pts',(-2.80625145000006,15.2,10.505028852));
#230559=CARTESIAN_POINT('Ctrl Pts',(-2.80625145000006,11.6,10.505028852));
#230560=CARTESIAN_POINT('Ctrl Pts',(-2.80640343900005,15.2,10.502220475));
#230561=CARTESIAN_POINT('Ctrl Pts',(-2.80640343900005,11.6,10.502220475));
#230562=CARTESIAN_POINT('Ctrl Pts',(-2.80655278100005,15.2,10.499417638));
#230563=CARTESIAN_POINT('Ctrl Pts',(-2.80655278100005,11.6,10.499417638));
#230564=CARTESIAN_POINT('Ctrl Pts',(-2.80669948500006,15.2,10.49662035));
#230565=CARTESIAN_POINT('Ctrl Pts',(-2.80669948500006,11.6,10.49662035));
#230566=CARTESIAN_POINT('Ctrl Pts',(-2.80684355800005,15.2,10.493828624));
#230567=CARTESIAN_POINT('Ctrl Pts',(-2.80684355800005,11.6,10.493828624));
#230568=CARTESIAN_POINT('Ctrl Pts',(-2.80698500600006,15.2,10.491042469));
#230569=CARTESIAN_POINT('Ctrl Pts',(-2.80698500600006,11.6,10.491042469));
#230570=CARTESIAN_POINT('Ctrl Pts',(-2.80712383900006,15.2,10.488261897));
#230571=CARTESIAN_POINT('Ctrl Pts',(-2.80712383900006,11.6,10.488261897));
#230572=CARTESIAN_POINT('Ctrl Pts',(-2.80726006500006,15.2,10.485486918));
#230573=CARTESIAN_POINT('Ctrl Pts',(-2.80726006500006,11.6,10.485486918));
#230574=CARTESIAN_POINT('Ctrl Pts',(-2.80739369000006,15.2,10.482717543));
#230575=CARTESIAN_POINT('Ctrl Pts',(-2.80739369000006,11.6,10.482717543));
#230576=CARTESIAN_POINT('Ctrl Pts',(-2.80752472300006,15.2,10.479953784));
#230577=CARTESIAN_POINT('Ctrl Pts',(-2.80752472300006,11.6,10.479953784));
#230578=CARTESIAN_POINT('Ctrl Pts',(-2.80765317100005,15.2,10.477195653));
#230579=CARTESIAN_POINT('Ctrl Pts',(-2.80765317100005,11.6,10.477195653));
#230580=CARTESIAN_POINT('Ctrl Pts',(-2.80777904200006,15.2,10.474443157));
#230581=CARTESIAN_POINT('Ctrl Pts',(-2.80777904200006,11.6,10.474443157));
#230582=CARTESIAN_POINT('Ctrl Pts',(-2.80790234500006,15.2,10.47169631));
#230583=CARTESIAN_POINT('Ctrl Pts',(-2.80790234500006,11.6,10.47169631));
#230584=CARTESIAN_POINT('Ctrl Pts',(-2.80802308700005,15.2,10.468955123));
#230585=CARTESIAN_POINT('Ctrl Pts',(-2.80802308700005,11.6,10.468955123));
#230586=CARTESIAN_POINT('Ctrl Pts',(-2.80814127600005,15.2,10.466219607));
#230587=CARTESIAN_POINT('Ctrl Pts',(-2.80814127600005,11.6,10.466219607));
#230588=CARTESIAN_POINT('Ctrl Pts',(-2.80825692000006,15.2,10.463489772));
#230589=CARTESIAN_POINT('Ctrl Pts',(-2.80825692000006,11.6,10.463489772));
#230590=CARTESIAN_POINT('Ctrl Pts',(-2.80837002600005,15.2,10.460765629));
#230591=CARTESIAN_POINT('Ctrl Pts',(-2.80837002600005,11.6,10.460765629));
#230592=CARTESIAN_POINT('Ctrl Pts',(-2.80848060400006,15.2,10.458047191));
#230593=CARTESIAN_POINT('Ctrl Pts',(-2.80848060400006,11.6,10.458047191));
#230594=CARTESIAN_POINT('Ctrl Pts',(-2.80858866100006,15.2,10.455334468));
#230595=CARTESIAN_POINT('Ctrl Pts',(-2.80858866100006,11.6,10.455334468));
#230596=CARTESIAN_POINT('Ctrl Pts',(-2.80869420500005,15.2,10.45262747));
#230597=CARTESIAN_POINT('Ctrl Pts',(-2.80869420500005,11.6,10.45262747));
#230598=CARTESIAN_POINT('Ctrl Pts',(-2.80879724400006,15.2,10.44992621));
#230599=CARTESIAN_POINT('Ctrl Pts',(-2.80879724400006,11.6,10.44992621));
#230600=CARTESIAN_POINT('Ctrl Pts',(-2.80889778700006,15.2,10.447230699));
#230601=CARTESIAN_POINT('Ctrl Pts',(-2.80889778700006,11.6,10.447230699));
#230602=CARTESIAN_POINT('Ctrl Pts',(-2.80899584100006,15.2,10.444540948));
#230603=CARTESIAN_POINT('Ctrl Pts',(-2.80899584100006,11.6,10.444540948));
#230604=CARTESIAN_POINT('Ctrl Pts',(-2.80909141500006,15.2,10.441856968));
#230605=CARTESIAN_POINT('Ctrl Pts',(-2.80909141500006,11.6,10.441856968));
#230606=CARTESIAN_POINT('Ctrl Pts',(-2.80918451700006,15.2,10.43917877));
#230607=CARTESIAN_POINT('Ctrl Pts',(-2.80918451700006,11.6,10.43917877));
#230608=CARTESIAN_POINT('Ctrl Pts',(-2.80927515500006,15.2,10.436506365));
#230609=CARTESIAN_POINT('Ctrl Pts',(-2.80927515500006,11.6,10.436506365));
#230610=CARTESIAN_POINT('Ctrl Pts',(-2.80936333800006,15.2,10.433839767));
#230611=CARTESIAN_POINT('Ctrl Pts',(-2.80936333800006,11.6,10.433839767));
#230612=CARTESIAN_POINT('Ctrl Pts',(-2.80944907400006,15.2,10.431178984));
#230613=CARTESIAN_POINT('Ctrl Pts',(-2.80944907400006,11.6,10.431178984));
#230614=CARTESIAN_POINT('Ctrl Pts',(-2.80953237000006,15.2,10.428524029));
#230615=CARTESIAN_POINT('Ctrl Pts',(-2.80953237000006,11.6,10.428524029));
#230616=CARTESIAN_POINT('Ctrl Pts',(-2.80961323600006,15.2,10.425874914));
#230617=CARTESIAN_POINT('Ctrl Pts',(-2.80961323600006,11.6,10.425874914));
#230618=CARTESIAN_POINT('Ctrl Pts',(-2.80969168100006,15.2,10.423231649));
#230619=CARTESIAN_POINT('Ctrl Pts',(-2.80969168100006,11.6,10.423231649));
#230620=CARTESIAN_POINT('Ctrl Pts',(-2.80976771100006,15.2,10.420594246));
#230621=CARTESIAN_POINT('Ctrl Pts',(-2.80976771100006,11.6,10.420594246));
#230622=CARTESIAN_POINT('Ctrl Pts',(-2.80984133800006,15.2,10.417962717));
#230623=CARTESIAN_POINT('Ctrl Pts',(-2.80984133800006,11.6,10.417962717));
#230624=CARTESIAN_POINT('Ctrl Pts',(-2.80991256600006,15.2,10.415337072));
#230625=CARTESIAN_POINT('Ctrl Pts',(-2.80991256600006,11.6,10.415337072));
#230626=CARTESIAN_POINT('Ctrl Pts',(-2.80998140700006,15.2,10.412717324));
#230627=CARTESIAN_POINT('Ctrl Pts',(-2.80998140700006,11.6,10.412717324));
#230628=CARTESIAN_POINT('Ctrl Pts',(-2.81004786900006,15.2,10.410103485));
#230629=CARTESIAN_POINT('Ctrl Pts',(-2.81004786900006,11.6,10.410103485));
#230630=CARTESIAN_POINT('Ctrl Pts',(-2.81011195900006,15.2,10.407495565));
#230631=CARTESIAN_POINT('Ctrl Pts',(-2.81011195900006,11.6,10.407495565));
#230632=CARTESIAN_POINT('Ctrl Pts',(-2.81017368600006,15.2,10.404893577));
#230633=CARTESIAN_POINT('Ctrl Pts',(-2.81017368600006,11.6,10.404893577));
#230634=CARTESIAN_POINT('Ctrl Pts',(-2.81023306000006,15.2,10.402297531));
#230635=CARTESIAN_POINT('Ctrl Pts',(-2.81023306000006,11.6,10.402297531));
#230636=CARTESIAN_POINT('Ctrl Pts',(-2.81029009000005,15.2,10.399707441));
#230637=CARTESIAN_POINT('Ctrl Pts',(-2.81029009000005,11.6,10.399707441));
#230638=CARTESIAN_POINT('Ctrl Pts',(-2.81034478200006,15.2,10.397123316));
#230639=CARTESIAN_POINT('Ctrl Pts',(-2.81034478200006,11.6,10.397123316));
#230640=CARTESIAN_POINT('Ctrl Pts',(-2.81039714700006,15.2,10.39454517));
#230641=CARTESIAN_POINT('Ctrl Pts',(-2.81039714700006,11.6,10.39454517));
#230642=CARTESIAN_POINT('Ctrl Pts',(-2.81044719400006,15.2,10.391973013));
#230643=CARTESIAN_POINT('Ctrl Pts',(-2.81044719400006,11.6,10.391973013));
#230644=CARTESIAN_POINT('Ctrl Pts',(-2.81049493100006,15.2,10.389406857));
#230645=CARTESIAN_POINT('Ctrl Pts',(-2.81049493100006,11.6,10.389406857));
#230646=CARTESIAN_POINT('Ctrl Pts',(-2.81054036600006,15.2,10.386846714));
#230647=CARTESIAN_POINT('Ctrl Pts',(-2.81054036600006,11.6,10.386846714));
#230648=CARTESIAN_POINT('Ctrl Pts',(-2.81058350900006,15.2,10.384292596));
#230649=CARTESIAN_POINT('Ctrl Pts',(-2.81058350900006,11.6,10.384292596));
#230650=CARTESIAN_POINT('Ctrl Pts',(-2.81062436900006,15.2,10.381744516));
#230651=CARTESIAN_POINT('Ctrl Pts',(-2.81062436900006,11.6,10.381744516));
#230652=CARTESIAN_POINT('Ctrl Pts',(-2.81066295400006,15.2,10.379202484));
#230653=CARTESIAN_POINT('Ctrl Pts',(-2.81066295400006,11.6,10.379202484));
#230654=CARTESIAN_POINT('Ctrl Pts',(-2.81069927400006,15.2,10.376666512));
#230655=CARTESIAN_POINT('Ctrl Pts',(-2.81069927400006,11.6,10.376666512));
#230656=CARTESIAN_POINT('Ctrl Pts',(-2.81073333700005,15.2,10.374136614));
#230657=CARTESIAN_POINT('Ctrl Pts',(-2.81073333700005,11.6,10.374136614));
#230658=CARTESIAN_POINT('Ctrl Pts',(-2.81076515300006,15.2,10.371612799));
#230659=CARTESIAN_POINT('Ctrl Pts',(-2.81076515300006,11.6,10.371612799));
#230660=CARTESIAN_POINT('Ctrl Pts',(-2.81079473100006,15.2,10.369095081));
#230661=CARTESIAN_POINT('Ctrl Pts',(-2.81079473100006,11.6,10.369095081));
#230662=CARTESIAN_POINT('Ctrl Pts',(-2.81082207900006,15.2,10.366583471));
#230663=CARTESIAN_POINT('Ctrl Pts',(-2.81082207900006,11.6,10.366583471));
#230664=CARTESIAN_POINT('Ctrl Pts',(-2.81084720700005,15.2,10.364077981));
#230665=CARTESIAN_POINT('Ctrl Pts',(-2.81084720700005,11.6,10.364077981));
#230666=CARTESIAN_POINT('Ctrl Pts',(-2.81087012500006,15.2,10.361578624));
#230667=CARTESIAN_POINT('Ctrl Pts',(-2.81087012500006,11.6,10.361578624));
#230668=CARTESIAN_POINT('Ctrl Pts',(-2.81089084000006,15.2,10.359085411));
#230669=CARTESIAN_POINT('Ctrl Pts',(-2.81089084000006,11.6,10.359085411));
#230670=CARTESIAN_POINT('Ctrl Pts',(-2.81090936200005,15.2,10.356598354));
#230671=CARTESIAN_POINT('Ctrl Pts',(-2.81090936200005,11.6,10.356598354));
#230672=CARTESIAN_POINT('Ctrl Pts',(-2.81092570200005,15.2,10.354117466));
#230673=CARTESIAN_POINT('Ctrl Pts',(-2.81092570200005,11.6,10.354117466));
#230674=CARTESIAN_POINT('Ctrl Pts',(-2.81093986900005,15.2,10.351642759));
#230675=CARTESIAN_POINT('Ctrl Pts',(-2.81093986900005,11.6,10.351642759));
#230676=CARTESIAN_POINT('Ctrl Pts',(-2.81095187000005,15.2,10.349174244));
#230677=CARTESIAN_POINT('Ctrl Pts',(-2.81095187000005,11.6,10.349174244));
#230678=CARTESIAN_POINT('Ctrl Pts',(-2.81096171500006,15.2,10.346711935));
#230679=CARTESIAN_POINT('Ctrl Pts',(-2.81096171500006,11.6,10.346711935));
#230680=CARTESIAN_POINT('Ctrl Pts',(-2.81096941600006,15.2,10.344255843));
#230681=CARTESIAN_POINT('Ctrl Pts',(-2.81096941600006,11.6,10.344255843));
#230682=CARTESIAN_POINT('Ctrl Pts',(-2.81097498000006,15.2,10.34180598));
#230683=CARTESIAN_POINT('Ctrl Pts',(-2.81097498000006,11.6,10.34180598));
#230684=CARTESIAN_POINT('Ctrl Pts',(-2.81097841700006,15.2,10.33936236));
#230685=CARTESIAN_POINT('Ctrl Pts',(-2.81097841700006,11.6,10.33936236));
#230686=CARTESIAN_POINT('Ctrl Pts',(-2.81097973600006,15.2,10.336924994));
#230687=CARTESIAN_POINT('Ctrl Pts',(-2.81097973600006,11.6,10.336924994));
#230688=CARTESIAN_POINT('Ctrl Pts',(-2.81097894800005,15.2,10.334493893));
#230689=CARTESIAN_POINT('Ctrl Pts',(-2.81097894800005,11.6,10.334493893));
#230690=CARTESIAN_POINT('Ctrl Pts',(-2.81097606100006,15.2,10.332069072));
#230691=CARTESIAN_POINT('Ctrl Pts',(-2.81097606100006,11.6,10.332069072));
#230692=CARTESIAN_POINT('Ctrl Pts',(-2.81097108600005,15.2,10.329650542));
#230693=CARTESIAN_POINT('Ctrl Pts',(-2.81097108600005,11.6,10.329650542));
#230694=CARTESIAN_POINT('Ctrl Pts',(-2.81096403200006,15.2,10.327238316));
#230695=CARTESIAN_POINT('Ctrl Pts',(-2.81096403200006,11.6,10.327238316));
#230696=CARTESIAN_POINT('Ctrl Pts',(-2.81095490900006,15.2,10.324832405));
#230697=CARTESIAN_POINT('Ctrl Pts',(-2.81095490900006,11.6,10.324832405));
#230698=CARTESIAN_POINT('Ctrl Pts',(-2.81094372600006,15.2,10.322432823));
#230699=CARTESIAN_POINT('Ctrl Pts',(-2.81094372600006,11.6,10.322432823));
#230700=CARTESIAN_POINT('Ctrl Pts',(-2.81093049400006,15.2,10.320039583));
#230701=CARTESIAN_POINT('Ctrl Pts',(-2.81093049400006,11.6,10.320039583));
#230702=CARTESIAN_POINT('Ctrl Pts',(-2.81091522100006,15.2,10.317652695));
#230703=CARTESIAN_POINT('Ctrl Pts',(-2.81091522100006,11.6,10.317652695));
#230704=CARTESIAN_POINT('Ctrl Pts',(-2.81089791700006,15.2,10.315272175));
#230705=CARTESIAN_POINT('Ctrl Pts',(-2.81089791700006,11.6,10.315272175));
#230706=CARTESIAN_POINT('Ctrl Pts',(-2.81087859400006,15.2,10.312898032));
#230707=CARTESIAN_POINT('Ctrl Pts',(-2.81087859400006,11.6,10.312898032));
#230708=CARTESIAN_POINT('Ctrl Pts',(-2.81085726200006,15.2,10.310530282));
#230709=CARTESIAN_POINT('Ctrl Pts',(-2.81085726200006,11.6,10.310530282));
#230710=CARTESIAN_POINT('Ctrl Pts',(-2.81083392800006,15.2,10.308168934));
#230711=CARTESIAN_POINT('Ctrl Pts',(-2.81083392800006,11.6,10.308168934));
#230712=CARTESIAN_POINT('Ctrl Pts',(-2.81080860300006,15.2,10.305814004));
#230713=CARTESIAN_POINT('Ctrl Pts',(-2.81080860300006,11.6,10.305814004));
#230714=CARTESIAN_POINT('Ctrl Pts',(-2.81078129900005,15.2,10.303465504));
#230715=CARTESIAN_POINT('Ctrl Pts',(-2.81078129900005,11.6,10.303465504));
#230716=CARTESIAN_POINT('Ctrl Pts',(-2.81075202400006,15.2,10.301123445));
#230717=CARTESIAN_POINT('Ctrl Pts',(-2.81075202400006,11.6,10.301123445));
#230718=CARTESIAN_POINT('Ctrl Pts',(-2.81072078900006,15.2,10.298787841));
#230719=CARTESIAN_POINT('Ctrl Pts',(-2.81072078900006,11.6,10.298787841));
#230720=CARTESIAN_POINT('Ctrl Pts',(-2.81068760400006,15.2,10.296458705));
#230721=CARTESIAN_POINT('Ctrl Pts',(-2.81068760400006,11.6,10.296458705));
#230722=CARTESIAN_POINT('Ctrl Pts',(-2.81065248000006,15.2,10.29413605));
#230723=CARTESIAN_POINT('Ctrl Pts',(-2.81065248000006,11.6,10.29413605));
#230724=CARTESIAN_POINT('Ctrl Pts',(-2.81061542500006,15.2,10.291819888));
#230725=CARTESIAN_POINT('Ctrl Pts',(-2.81061542500006,11.6,10.291819888));
#230726=CARTESIAN_POINT('Ctrl Pts',(-2.81057645100006,15.2,10.289510232));
#230727=CARTESIAN_POINT('Ctrl Pts',(-2.81057645100006,11.6,10.289510232));
#230728=CARTESIAN_POINT('Ctrl Pts',(-2.81053556900006,15.2,10.287207096));
#230729=CARTESIAN_POINT('Ctrl Pts',(-2.81053556900006,11.6,10.287207096));
#230730=CARTESIAN_POINT('Ctrl Pts',(-2.81049278700006,15.2,10.284910491));
#230731=CARTESIAN_POINT('Ctrl Pts',(-2.81049278700006,11.6,10.284910491));
#230732=CARTESIAN_POINT('Ctrl Pts',(-2.81044811600006,15.2,10.282620433));
#230733=CARTESIAN_POINT('Ctrl Pts',(-2.81044811600006,11.6,10.282620433));
#230734=CARTESIAN_POINT('Ctrl Pts',(-2.81040156900006,15.2,10.280336931));
#230735=CARTESIAN_POINT('Ctrl Pts',(-2.81040156900006,11.6,10.280336931));
#230736=CARTESIAN_POINT('Ctrl Pts',(-2.81035315300006,15.2,10.278060001));
#230737=CARTESIAN_POINT('Ctrl Pts',(-2.81035315300006,11.6,10.278060001));
#230738=CARTESIAN_POINT('Ctrl Pts',(-2.81030288100005,15.2,10.275789656));
#230739=CARTESIAN_POINT('Ctrl Pts',(-2.81030288100005,11.6,10.275789656));
#230740=CARTESIAN_POINT('Ctrl Pts',(-2.81025076100006,15.2,10.273525909));
#230741=CARTESIAN_POINT('Ctrl Pts',(-2.81025076100006,11.6,10.273525909));
#230742=CARTESIAN_POINT('Ctrl Pts',(-2.81019680700005,15.2,10.271268772));
#230743=CARTESIAN_POINT('Ctrl Pts',(-2.81019680700005,11.6,10.271268772));
#230744=CARTESIAN_POINT('Ctrl Pts',(-2.81014102700006,15.2,10.269018258));
#230745=CARTESIAN_POINT('Ctrl Pts',(-2.81014102700006,11.6,10.269018258));
#230746=CARTESIAN_POINT('Ctrl Pts',(-2.81008343200006,15.2,10.266774382));
#230747=CARTESIAN_POINT('Ctrl Pts',(-2.81008343200006,11.6,10.266774382));
#230748=CARTESIAN_POINT('Ctrl Pts',(-2.81002403300006,15.2,10.264537156));
#230749=CARTESIAN_POINT('Ctrl Pts',(-2.81002403300006,11.6,10.264537156));
#230750=CARTESIAN_POINT('Ctrl Pts',(-2.80996284200006,15.2,10.262306594));
#230751=CARTESIAN_POINT('Ctrl Pts',(-2.80996284200006,11.6,10.262306594));
#230752=CARTESIAN_POINT('Ctrl Pts',(-2.80989986700006,15.2,10.260082708));
#230753=CARTESIAN_POINT('Ctrl Pts',(-2.80989986700006,11.6,10.260082708));
#230754=CARTESIAN_POINT('Ctrl Pts',(-2.80983512200006,15.2,10.257865513));
#230755=CARTESIAN_POINT('Ctrl Pts',(-2.80983512200006,11.6,10.257865513));
#230756=CARTESIAN_POINT('Ctrl Pts',(-2.80976861600006,15.2,10.255655021));
#230757=CARTESIAN_POINT('Ctrl Pts',(-2.80976861600006,11.6,10.255655021));
#230758=CARTESIAN_POINT('Ctrl Pts',(-2.80970036000005,15.2,10.253451246));
#230759=CARTESIAN_POINT('Ctrl Pts',(-2.80970036000005,11.6,10.253451246));
#230760=CARTESIAN_POINT('Ctrl Pts',(-2.80963036400005,15.2,10.251254202));
#230761=CARTESIAN_POINT('Ctrl Pts',(-2.80963036400005,11.6,10.251254202));
#230762=CARTESIAN_POINT('Ctrl Pts',(-2.80955864200005,15.2,10.249063902));
#230763=CARTESIAN_POINT('Ctrl Pts',(-2.80955864200005,11.6,10.249063902));
#230764=CARTESIAN_POINT('Ctrl Pts',(-2.80948520300006,15.2,10.246880359));
#230765=CARTESIAN_POINT('Ctrl Pts',(-2.80948520300006,11.6,10.246880359));
#230766=CARTESIAN_POINT('Ctrl Pts',(-2.80941005800006,15.2,10.244703588));
#230767=CARTESIAN_POINT('Ctrl Pts',(-2.80941005800006,11.6,10.244703588));
#230768=CARTESIAN_POINT('Ctrl Pts',(-2.80933321800005,15.2,10.242533601));
#230769=CARTESIAN_POINT('Ctrl Pts',(-2.80933321800005,11.6,10.242533601));
#230770=CARTESIAN_POINT('Ctrl Pts',(-2.80925469500006,15.2,10.240370412));
#230771=CARTESIAN_POINT('Ctrl Pts',(-2.80925469500006,11.6,10.240370412));
#230772=CARTESIAN_POINT('Ctrl Pts',(-2.80917450000006,15.2,10.238214036));
#230773=CARTESIAN_POINT('Ctrl Pts',(-2.80917450000006,11.6,10.238214036));
#230774=CARTESIAN_POINT('Ctrl Pts',(-2.80909264400006,15.2,10.236064484));
#230775=CARTESIAN_POINT('Ctrl Pts',(-2.80909264400006,11.6,10.236064484));
#230776=CARTESIAN_POINT('Ctrl Pts',(-2.80900913900005,15.2,10.233921772));
#230777=CARTESIAN_POINT('Ctrl Pts',(-2.80900913900005,11.6,10.233921772));
#230778=CARTESIAN_POINT('Ctrl Pts',(-2.80892399400006,15.2,10.231785914));
#230779=CARTESIAN_POINT('Ctrl Pts',(-2.80892399400006,11.6,10.231785914));
#230780=CARTESIAN_POINT('Ctrl Pts',(-2.80883722400006,15.2,10.229656922));
#230781=CARTESIAN_POINT('Ctrl Pts',(-2.80883722400006,11.6,10.229656922));
#230782=CARTESIAN_POINT('Ctrl Pts',(-2.80874883800006,15.2,10.227534811));
#230783=CARTESIAN_POINT('Ctrl Pts',(-2.80874883800006,11.6,10.227534811));
#230784=CARTESIAN_POINT('Ctrl Pts',(-2.80865884800006,15.2,10.225419595));
#230785=CARTESIAN_POINT('Ctrl Pts',(-2.80865884800006,11.6,10.225419595));
#230786=CARTESIAN_POINT('Ctrl Pts',(-2.80856726600006,15.2,10.223311287));
#230787=CARTESIAN_POINT('Ctrl Pts',(-2.80856726600006,11.6,10.223311287));
#230788=CARTESIAN_POINT('Ctrl Pts',(-2.80847410200006,15.2,10.221209902));
#230789=CARTESIAN_POINT('Ctrl Pts',(-2.80847410200006,11.6,10.221209902));
#230790=CARTESIAN_POINT('Ctrl Pts',(-2.80837937000005,15.2,10.219115454));
#230791=CARTESIAN_POINT('Ctrl Pts',(-2.80837937000005,11.6,10.219115454));
#230792=CARTESIAN_POINT('Ctrl Pts',(-2.80828308100005,15.2,10.217027956));
#230793=CARTESIAN_POINT('Ctrl Pts',(-2.80828308100005,11.6,10.217027956));
#230794=CARTESIAN_POINT('Ctrl Pts',(-2.80818524500006,15.2,10.214947422));
#230795=CARTESIAN_POINT('Ctrl Pts',(-2.80818524500006,11.6,10.214947422));
#230796=CARTESIAN_POINT('Ctrl Pts',(-2.80808587600006,15.2,10.212873868));
#230797=CARTESIAN_POINT('Ctrl Pts',(-2.80808587600006,11.6,10.212873868));
#230798=CARTESIAN_POINT('Ctrl Pts',(-2.80798498400006,15.2,10.210807306));
#230799=CARTESIAN_POINT('Ctrl Pts',(-2.80798498400006,11.6,10.210807306));
#230800=CARTESIAN_POINT('Ctrl Pts',(-2.80788258200006,15.2,10.208747751));
#230801=CARTESIAN_POINT('Ctrl Pts',(-2.80788258200006,11.6,10.208747751));
#230802=CARTESIAN_POINT('Ctrl Pts',(-2.80777868100006,15.2,10.206695219));
#230803=CARTESIAN_POINT('Ctrl Pts',(-2.80777868100006,11.6,10.206695219));
#230804=CARTESIAN_POINT('Ctrl Pts',(-2.80767329400006,15.2,10.20464972));
#230805=CARTESIAN_POINT('Ctrl Pts',(-2.80767329400006,11.6,10.20464972));
#230806=CARTESIAN_POINT('Ctrl Pts',(-2.80756643200006,15.2,10.202611273));
#230807=CARTESIAN_POINT('Ctrl Pts',(-2.80756643200006,11.6,10.202611273));
#230808=CARTESIAN_POINT('Ctrl Pts',(-2.80745810900005,15.2,10.200579889));
#230809=CARTESIAN_POINT('Ctrl Pts',(-2.80745810900005,11.6,10.200579889));
#230810=CARTESIAN_POINT('Ctrl Pts',(-2.80734833500006,15.2,10.198555584));
#230811=CARTESIAN_POINT('Ctrl Pts',(-2.80734833500006,11.6,10.198555584));
#230812=CARTESIAN_POINT('Ctrl Pts',(-2.80723712200006,15.2,10.196538372));
#230813=CARTESIAN_POINT('Ctrl Pts',(-2.80723712200006,11.6,10.196538372));
#230814=CARTESIAN_POINT('Ctrl Pts',(-2.80712448400006,15.2,10.194528266));
#230815=CARTESIAN_POINT('Ctrl Pts',(-2.80712448400006,11.6,10.194528266));
#230816=CARTESIAN_POINT('Ctrl Pts',(-2.80701043200006,15.2,10.192525284));
#230817=CARTESIAN_POINT('Ctrl Pts',(-2.80701043200006,11.6,10.192525284));
#230818=CARTESIAN_POINT('Ctrl Pts',(-2.80689497900006,15.2,10.190529438));
#230819=CARTESIAN_POINT('Ctrl Pts',(-2.80689497900006,11.6,10.190529438));
#230820=CARTESIAN_POINT('Ctrl Pts',(-2.80677813600006,15.2,10.188540742));
#230821=CARTESIAN_POINT('Ctrl Pts',(-2.80677813600006,11.6,10.188540742));
#230822=CARTESIAN_POINT('Ctrl Pts',(-2.80665991800006,15.2,10.186559212));
#230823=CARTESIAN_POINT('Ctrl Pts',(-2.80665991800006,11.6,10.186559212));
#230824=CARTESIAN_POINT('Ctrl Pts',(-2.80654033400006,15.2,10.184584864));
#230825=CARTESIAN_POINT('Ctrl Pts',(-2.80654033400006,11.6,10.184584864));
#230826=CARTESIAN_POINT('Ctrl Pts',(-2.80641939900006,15.2,10.182617709));
#230827=CARTESIAN_POINT('Ctrl Pts',(-2.80641939900006,11.6,10.182617709));
#230828=CARTESIAN_POINT('Ctrl Pts',(-2.80629712500006,15.2,10.180657765));
#230829=CARTESIAN_POINT('Ctrl Pts',(-2.80629712500006,11.6,10.180657765));
#230830=CARTESIAN_POINT('Ctrl Pts',(-2.80617352500005,15.2,10.178705045));
#230831=CARTESIAN_POINT('Ctrl Pts',(-2.80617352500005,11.6,10.178705045));
#230832=CARTESIAN_POINT('Ctrl Pts',(-2.80604861100006,15.2,10.176759565));
#230833=CARTESIAN_POINT('Ctrl Pts',(-2.80604861100006,11.6,10.176759565));
#230834=CARTESIAN_POINT('Ctrl Pts',(-2.80592239500006,15.2,10.174821339));
#230835=CARTESIAN_POINT('Ctrl Pts',(-2.80592239500006,11.6,10.174821339));
#230836=CARTESIAN_POINT('Ctrl Pts',(-2.80579489100006,15.2,10.172890382));
#230837=CARTESIAN_POINT('Ctrl Pts',(-2.80579489100006,11.6,10.172890382));
#230838=CARTESIAN_POINT('Ctrl Pts',(-2.80566611200006,15.2,10.170966709));
#230839=CARTESIAN_POINT('Ctrl Pts',(-2.80566611200006,11.6,10.170966709));
#230840=CARTESIAN_POINT('Ctrl Pts',(-2.80553607000006,15.2,10.169050336));
#230841=CARTESIAN_POINT('Ctrl Pts',(-2.80553607000006,11.6,10.169050336));
#230842=CARTESIAN_POINT('Ctrl Pts',(-2.80540477700006,15.2,10.167141276));
#230843=CARTESIAN_POINT('Ctrl Pts',(-2.80540477700006,11.6,10.167141276));
#230844=CARTESIAN_POINT('Ctrl Pts',(-2.80527224900006,15.2,10.165239546));
#230845=CARTESIAN_POINT('Ctrl Pts',(-2.80527224900006,11.6,10.165239546));
#230846=CARTESIAN_POINT('Ctrl Pts',(-2.80513849700006,15.2,10.16334516));
#230847=CARTESIAN_POINT('Ctrl Pts',(-2.80513849700006,11.6,10.16334516));
#230848=CARTESIAN_POINT('Ctrl Pts',(-2.80500353400006,15.2,10.161458135));
#230849=CARTESIAN_POINT('Ctrl Pts',(-2.80500353400006,11.6,10.161458135));
#230850=CARTESIAN_POINT('Ctrl Pts',(-2.80486737300006,15.2,10.159578484));
#230851=CARTESIAN_POINT('Ctrl Pts',(-2.80486737300006,11.6,10.159578484));
#230852=CARTESIAN_POINT('Ctrl Pts',(-2.80473002900006,15.2,10.157706223));
#230853=CARTESIAN_POINT('Ctrl Pts',(-2.80473002900006,11.6,10.157706223));
#230854=CARTESIAN_POINT('Ctrl Pts',(-2.80459151300006,15.2,10.155841368));
#230855=CARTESIAN_POINT('Ctrl Pts',(-2.80459151300006,11.6,10.155841368));
#230856=CARTESIAN_POINT('Ctrl Pts',(-2.80445184000006,15.2,10.153983933));
#230857=CARTESIAN_POINT('Ctrl Pts',(-2.80445184000006,11.6,10.153983933));
#230858=CARTESIAN_POINT('Ctrl Pts',(-2.80431102200006,15.2,10.152133935));
#230859=CARTESIAN_POINT('Ctrl Pts',(-2.80431102200006,11.6,10.152133935));
#230860=CARTESIAN_POINT('Ctrl Pts',(-2.80416907300005,15.2,10.150291389));
#230861=CARTESIAN_POINT('Ctrl Pts',(-2.80416907300005,11.6,10.150291389));
#230862=CARTESIAN_POINT('Ctrl Pts',(-2.80402600700006,15.2,10.14845631));
#230863=CARTESIAN_POINT('Ctrl Pts',(-2.80402600700006,11.6,10.14845631));
#230864=CARTESIAN_POINT('Ctrl Pts',(-2.80388183800006,15.2,10.146628712));
#230865=CARTESIAN_POINT('Ctrl Pts',(-2.80388183800006,11.6,10.146628712));
#230866=CARTESIAN_POINT('Ctrl Pts',(-2.80373657700005,15.2,10.144808615));
#230867=CARTESIAN_POINT('Ctrl Pts',(-2.80373657700005,11.6,10.144808615));
#230868=CARTESIAN_POINT('Ctrl Pts',(-2.80359024100005,15.2,10.142996029));
#230869=CARTESIAN_POINT('Ctrl Pts',(-2.80359024100005,11.6,10.142996029));
#230870=CARTESIAN_POINT('Ctrl Pts',(-2.80344284000006,15.2,10.141190975));
#230871=CARTESIAN_POINT('Ctrl Pts',(-2.80344284000006,11.6,10.141190975));
#230872=CARTESIAN_POINT('Ctrl Pts',(-2.80329439200006,15.2,10.139393467));
#230873=CARTESIAN_POINT('Ctrl Pts',(-2.80329439200006,11.6,10.139393467));
#230874=CARTESIAN_POINT('Ctrl Pts',(-2.80314490700006,15.2,10.137603518));
#230875=CARTESIAN_POINT('Ctrl Pts',(-2.80314490700006,11.6,10.137603518));
#230876=CARTESIAN_POINT('Ctrl Pts',(-2.80299440200006,15.2,10.135821147));
#230877=CARTESIAN_POINT('Ctrl Pts',(-2.80299440200006,11.6,10.135821147));
#230878=CARTESIAN_POINT('Ctrl Pts',(-2.80284288900006,15.2,10.134046369));
#230879=CARTESIAN_POINT('Ctrl Pts',(-2.80284288900006,11.6,10.134046369));
#230880=CARTESIAN_POINT('Ctrl Pts',(-2.80269038200006,15.2,10.1322792));
#230881=CARTESIAN_POINT('Ctrl Pts',(-2.80269038200006,11.6,10.1322792));
#230882=CARTESIAN_POINT('Ctrl Pts',(-2.80253689600006,15.2,10.130519656));
#230883=CARTESIAN_POINT('Ctrl Pts',(-2.80253689600006,11.6,10.130519656));
#230884=CARTESIAN_POINT('Ctrl Pts',(-2.80238244500006,15.2,10.128767753));
#230885=CARTESIAN_POINT('Ctrl Pts',(-2.80238244500006,11.6,10.128767753));
#230886=CARTESIAN_POINT('Ctrl Pts',(-2.80222704300006,15.2,10.127023506));
#230887=CARTESIAN_POINT('Ctrl Pts',(-2.80222704300006,11.6,10.127023506));
#230888=CARTESIAN_POINT('Ctrl Pts',(-2.80207070500006,15.2,10.125286933));
#230889=CARTESIAN_POINT('Ctrl Pts',(-2.80207070500006,11.6,10.125286933));
#230890=CARTESIAN_POINT('Ctrl Pts',(-2.80191344400006,15.2,10.123558049));
#230891=CARTESIAN_POINT('Ctrl Pts',(-2.80191344400006,11.6,10.123558049));
#230892=CARTESIAN_POINT('Ctrl Pts',(-2.80175527400006,15.2,10.121836872));
#230893=CARTESIAN_POINT('Ctrl Pts',(-2.80175527400006,11.6,10.121836872));
#230894=CARTESIAN_POINT('Ctrl Pts',(-2.80159621100006,15.2,10.120123415));
#230895=CARTESIAN_POINT('Ctrl Pts',(-2.80159621100006,11.6,10.120123415));
#230896=CARTESIAN_POINT('Ctrl Pts',(-2.80143627000006,15.2,10.118417697));
#230897=CARTESIAN_POINT('Ctrl Pts',(-2.80143627000006,11.6,10.118417697));
#230898=CARTESIAN_POINT('Ctrl Pts',(-2.80127546300006,15.2,10.116719734));
#230899=CARTESIAN_POINT('Ctrl Pts',(-2.80127546300006,11.6,10.116719734));
#230900=CARTESIAN_POINT('Ctrl Pts',(-2.80111380600006,15.2,10.115029541));
#230901=CARTESIAN_POINT('Ctrl Pts',(-2.80111380600006,11.6,10.115029541));
#230902=CARTESIAN_POINT('Ctrl Pts',(-2.80095131400006,15.2,10.113347136));
#230903=CARTESIAN_POINT('Ctrl Pts',(-2.80095131400006,11.6,10.113347136));
#230904=CARTESIAN_POINT('Ctrl Pts',(-2.80078800200006,15.2,10.111672537));
#230905=CARTESIAN_POINT('Ctrl Pts',(-2.80078800200006,11.6,10.111672537));
#230906=CARTESIAN_POINT('Ctrl Pts',(-2.80062388500005,15.2,10.110005756));
#230907=CARTESIAN_POINT('Ctrl Pts',(-2.80062388500005,11.6,10.110005756));
#230908=CARTESIAN_POINT('Ctrl Pts',(-2.80045897700006,15.2,10.108346814));
#230909=CARTESIAN_POINT('Ctrl Pts',(-2.80045897700006,11.6,10.108346814));
#230910=CARTESIAN_POINT('Ctrl Pts',(-2.80029329300006,15.2,10.106695726));
#230911=CARTESIAN_POINT('Ctrl Pts',(-2.80029329300006,11.6,10.106695726));
#230912=CARTESIAN_POINT('Ctrl Pts',(-2.80012684900006,15.2,10.105052508));
#230913=CARTESIAN_POINT('Ctrl Pts',(-2.80012684900006,11.6,10.105052508));
#230914=CARTESIAN_POINT('Ctrl Pts',(-2.79995965900006,15.2,10.103417179));
#230915=CARTESIAN_POINT('Ctrl Pts',(-2.79995965900006,11.6,10.103417179));
#230916=CARTESIAN_POINT('Ctrl Pts',(-2.79979173800006,15.2,10.101789754));
#230917=CARTESIAN_POINT('Ctrl Pts',(-2.79979173800006,11.6,10.101789754));
#230918=CARTESIAN_POINT('Ctrl Pts',(-2.79962310200006,15.2,10.100170251));
#230919=CARTESIAN_POINT('Ctrl Pts',(-2.79962310200006,11.6,10.100170251));
#230920=CARTESIAN_POINT('Ctrl Pts',(-2.79945376700006,15.2,10.098558686));
#230921=CARTESIAN_POINT('Ctrl Pts',(-2.79945376700006,11.6,10.098558686));
#230922=CARTESIAN_POINT('Ctrl Pts',(-2.79928374700006,15.2,10.096955078));
#230923=CARTESIAN_POINT('Ctrl Pts',(-2.79928374700006,11.6,10.096955078));
#230924=CARTESIAN_POINT('Ctrl Pts',(-2.79911305800006,15.2,10.095359441));
#230925=CARTESIAN_POINT('Ctrl Pts',(-2.79911305800006,11.6,10.095359441));
#230926=CARTESIAN_POINT('Ctrl Pts',(-2.79894171600006,15.2,10.093771795));
#230927=CARTESIAN_POINT('Ctrl Pts',(-2.79894171600006,11.6,10.093771795));
#230928=CARTESIAN_POINT('Ctrl Pts',(-2.79876973600006,15.2,10.092192157));
#230929=CARTESIAN_POINT('Ctrl Pts',(-2.79876973600006,11.6,10.092192157));
#230930=CARTESIAN_POINT('Ctrl Pts',(-2.79859713300006,15.2,10.090620543));
#230931=CARTESIAN_POINT('Ctrl Pts',(-2.79859713300006,11.6,10.090620543));
#230932=CARTESIAN_POINT('Ctrl Pts',(-2.79842392400006,15.2,10.08905697));
#230933=CARTESIAN_POINT('Ctrl Pts',(-2.79842392400006,11.6,10.08905697));
#230934=CARTESIAN_POINT('Ctrl Pts',(-2.79825012400006,15.2,10.087501457));
#230935=CARTESIAN_POINT('Ctrl Pts',(-2.79825012400006,11.6,10.087501457));
#230936=CARTESIAN_POINT('Ctrl Pts',(-2.79807575000006,15.2,10.08595402));
#230937=CARTESIAN_POINT('Ctrl Pts',(-2.79807575000006,11.6,10.08595402));
#230938=CARTESIAN_POINT('Ctrl Pts',(-2.79790081600006,15.2,10.084414678));
#230939=CARTESIAN_POINT('Ctrl Pts',(-2.79790081600006,11.6,10.084414678));
#230940=CARTESIAN_POINT('Ctrl Pts',(-2.79772533900006,15.2,10.082883449));
#230941=CARTESIAN_POINT('Ctrl Pts',(-2.79772533900006,11.6,10.082883449));
#230942=CARTESIAN_POINT('Ctrl Pts',(-2.79754933700006,15.2,10.081360348));
#230943=CARTESIAN_POINT('Ctrl Pts',(-2.79754933700006,11.6,10.081360348));
#230944=CARTESIAN_POINT('Ctrl Pts',(-2.79737282200006,15.2,10.079845395));
#230945=CARTESIAN_POINT('Ctrl Pts',(-2.79737282200006,11.6,10.079845395));
#230946=CARTESIAN_POINT('Ctrl Pts',(-2.79719581400005,15.2,10.078338606));
#230947=CARTESIAN_POINT('Ctrl Pts',(-2.79719581400005,11.6,10.078338606));
#230948=CARTESIAN_POINT('Ctrl Pts',(-2.79701832900006,15.2,10.076840001));
#230949=CARTESIAN_POINT('Ctrl Pts',(-2.79701832900006,11.6,10.076840001));
#230950=CARTESIAN_POINT('Ctrl Pts',(-2.79684038000005,15.2,10.075349597));
#230951=CARTESIAN_POINT('Ctrl Pts',(-2.79684038000005,11.6,10.075349597));
#230952=CARTESIAN_POINT('Ctrl Pts',(-2.79666198700005,15.2,10.073867411));
#230953=CARTESIAN_POINT('Ctrl Pts',(-2.79666198700005,11.6,10.073867411));
#230954=CARTESIAN_POINT('Ctrl Pts',(-2.79648316500006,15.2,10.072393463));
#230955=CARTESIAN_POINT('Ctrl Pts',(-2.79648316500006,11.6,10.072393463));
#230956=CARTESIAN_POINT('Ctrl Pts',(-2.79630393100006,15.2,10.070927768));
#230957=CARTESIAN_POINT('Ctrl Pts',(-2.79630393100006,11.6,10.070927768));
#230958=CARTESIAN_POINT('Ctrl Pts',(-2.79612430200006,15.2,10.069470348));
#230959=CARTESIAN_POINT('Ctrl Pts',(-2.79612430200006,11.6,10.069470348));
#230960=CARTESIAN_POINT('Ctrl Pts',(-2.79594429400006,15.2,10.068021219));
#230961=CARTESIAN_POINT('Ctrl Pts',(-2.79594429400006,11.6,10.068021219));
#230962=CARTESIAN_POINT('Ctrl Pts',(-2.79576392500006,15.2,10.066580399));
#230963=CARTESIAN_POINT('Ctrl Pts',(-2.79576392500006,11.6,10.066580399));
#230964=CARTESIAN_POINT('Ctrl Pts',(-2.79558321100006,15.2,10.065147907));
#230965=CARTESIAN_POINT('Ctrl Pts',(-2.79558321100006,11.6,10.065147907));
#230966=CARTESIAN_POINT('Ctrl Pts',(-2.79540216900006,15.2,10.063723762));
#230967=CARTESIAN_POINT('Ctrl Pts',(-2.79540216900006,11.6,10.063723762));
#230968=CARTESIAN_POINT('Ctrl Pts',(-2.79522081700006,15.2,10.062307981));
#230969=CARTESIAN_POINT('Ctrl Pts',(-2.79522081700006,11.6,10.062307981));
#230970=CARTESIAN_POINT('Ctrl Pts',(-2.79503917100006,15.2,10.060900584));
#230971=CARTESIAN_POINT('Ctrl Pts',(-2.79503917100006,11.6,10.060900584));
#230972=CARTESIAN_POINT('Ctrl Pts',(-2.79485724900006,15.2,10.05950159));
#230973=CARTESIAN_POINT('Ctrl Pts',(-2.79485724900006,11.6,10.05950159));
#230974=CARTESIAN_POINT('Ctrl Pts',(-2.79467506800006,15.2,10.058111017));
#230975=CARTESIAN_POINT('Ctrl Pts',(-2.79467506800006,11.6,10.058111017));
#230976=CARTESIAN_POINT('Ctrl Pts',(-2.79449264500006,15.2,10.056728882));
#230977=CARTESIAN_POINT('Ctrl Pts',(-2.79449264500006,11.6,10.056728882));
#230978=CARTESIAN_POINT('Ctrl Pts',(-2.79431000000006,15.2,10.055355206));
#230979=CARTESIAN_POINT('Ctrl Pts',(-2.79431000000006,11.6,10.055355206));
#230980=CARTESIAN_POINT('Ctrl Pts',(-2.79412714700006,15.2,10.053990008));
#230981=CARTESIAN_POINT('Ctrl Pts',(-2.79412714700006,11.6,10.053990008));
#230982=CARTESIAN_POINT('Ctrl Pts',(-2.79394410600006,15.2,10.052633307));
#230983=CARTESIAN_POINT('Ctrl Pts',(-2.79394410600006,11.6,10.052633307));
#230984=CARTESIAN_POINT('Ctrl Pts',(-2.79376089400006,15.2,10.05128512));
#230985=CARTESIAN_POINT('Ctrl Pts',(-2.79376089400006,11.6,10.05128512));
#230986=CARTESIAN_POINT('Ctrl Pts',(-2.79357752900005,15.2,10.049945468));
#230987=CARTESIAN_POINT('Ctrl Pts',(-2.79357752900005,11.6,10.049945468));
#230988=CARTESIAN_POINT('Ctrl Pts',(-2.79339402900006,15.2,10.048614371));
#230989=CARTESIAN_POINT('Ctrl Pts',(-2.79339402900006,11.6,10.048614371));
#230990=CARTESIAN_POINT('Ctrl Pts',(-2.79321041200005,15.2,10.047291846));
#230991=CARTESIAN_POINT('Ctrl Pts',(-2.79321041200005,11.6,10.047291846));
#230992=CARTESIAN_POINT('Ctrl Pts',(-2.79302669600006,15.2,10.045977913));
#230993=CARTESIAN_POINT('Ctrl Pts',(-2.79302669600006,11.6,10.045977913));
#230994=CARTESIAN_POINT('Ctrl Pts',(-2.79284290000006,15.2,10.044672593));
#230995=CARTESIAN_POINT('Ctrl Pts',(-2.79284290000006,11.6,10.044672593));
#230996=CARTESIAN_POINT('Ctrl Pts',(-2.79265904100006,15.2,10.043375903));
#230997=CARTESIAN_POINT('Ctrl Pts',(-2.79265904100006,11.6,10.043375903));
#230998=CARTESIAN_POINT('Ctrl Pts',(-2.79247513800006,15.2,10.042087865));
#230999=CARTESIAN_POINT('Ctrl Pts',(-2.79247513800006,11.6,10.042087865));
#231000=CARTESIAN_POINT('Ctrl Pts',(-2.79229120900006,15.2,10.040808498));
#231001=CARTESIAN_POINT('Ctrl Pts',(-2.79229120900006,11.6,10.040808498));
#231002=CARTESIAN_POINT('Ctrl Pts',(-2.79210727300006,15.2,10.03953782));
#231003=CARTESIAN_POINT('Ctrl Pts',(-2.79210727300006,11.6,10.03953782));
#231004=CARTESIAN_POINT('Ctrl Pts',(-2.79192335000006,15.2,10.038275854));
#231005=CARTESIAN_POINT('Ctrl Pts',(-2.79192335000006,11.6,10.038275854));
#231006=CARTESIAN_POINT('Ctrl Pts',(-2.79173945700005,15.2,10.037022616));
#231007=CARTESIAN_POINT('Ctrl Pts',(-2.79173945700005,11.6,10.037022616));
#231008=CARTESIAN_POINT('Ctrl Pts',(-2.79155561200006,15.2,10.035778129));
#231009=CARTESIAN_POINT('Ctrl Pts',(-2.79155561200006,11.6,10.035778129));
#231010=CARTESIAN_POINT('Ctrl Pts',(-2.79137183700006,15.2,10.034542412));
#231011=CARTESIAN_POINT('Ctrl Pts',(-2.79137183700006,11.6,10.034542412));
#231012=CARTESIAN_POINT('Ctrl Pts',(-2.79118814900006,15.2,10.033315486));
#231013=CARTESIAN_POINT('Ctrl Pts',(-2.79118814900006,11.6,10.033315486));
#231014=CARTESIAN_POINT('Ctrl Pts',(-2.79100456600006,15.2,10.032097369));
#231015=CARTESIAN_POINT('Ctrl Pts',(-2.79100456600006,11.6,10.032097369));
#231016=CARTESIAN_POINT('Ctrl Pts',(-2.79082110900006,15.2,10.030888083));
#231017=CARTESIAN_POINT('Ctrl Pts',(-2.79082110900006,11.6,10.030888083));
#231018=CARTESIAN_POINT('Ctrl Pts',(-2.79063779700006,15.2,10.029687649));
#231019=CARTESIAN_POINT('Ctrl Pts',(-2.79063779700006,11.6,10.029687649));
#231020=CARTESIAN_POINT('Ctrl Pts',(-2.79045465000006,15.2,10.028496085));
#231021=CARTESIAN_POINT('Ctrl Pts',(-2.79045465000006,11.6,10.028496085));
#231022=CARTESIAN_POINT('Ctrl Pts',(-2.79027168600006,15.2,10.027313415));
#231023=CARTESIAN_POINT('Ctrl Pts',(-2.79027168600006,11.6,10.027313415));
#231024=CARTESIAN_POINT('Ctrl Pts',(-2.79008892600006,15.2,10.026139656));
#231025=CARTESIAN_POINT('Ctrl Pts',(-2.79008892600006,11.6,10.026139656));
#231026=CARTESIAN_POINT('Ctrl Pts',(-2.78990639000006,15.2,10.024974832));
#231027=CARTESIAN_POINT('Ctrl Pts',(-2.78990639000006,11.6,10.024974832));
#231028=CARTESIAN_POINT('Ctrl Pts',(-2.78972409600006,15.2,10.023818962));
#231029=CARTESIAN_POINT('Ctrl Pts',(-2.78972409600006,11.6,10.023818962));
#231030=CARTESIAN_POINT('Ctrl Pts',(-2.78954206500006,15.2,10.022672066));
#231031=CARTESIAN_POINT('Ctrl Pts',(-2.78954206500006,11.6,10.022672066));
#231032=CARTESIAN_POINT('Ctrl Pts',(-2.78936031700006,15.2,10.021534166));
#231033=CARTESIAN_POINT('Ctrl Pts',(-2.78936031700006,11.6,10.021534166));
#231034=CARTESIAN_POINT('Ctrl Pts',(-2.78917887200006,15.2,10.020405283));
#231035=CARTESIAN_POINT('Ctrl Pts',(-2.78917887200006,11.6,10.020405283));
#231036=CARTESIAN_POINT('Ctrl Pts',(-2.78899775000006,15.2,10.01928544));
#231037=CARTESIAN_POINT('Ctrl Pts',(-2.78899775000006,11.6,10.01928544));
#231038=CARTESIAN_POINT('Ctrl Pts',(-2.78881697200006,15.2,10.018174655));
#231039=CARTESIAN_POINT('Ctrl Pts',(-2.78881697200006,11.6,10.018174655));
#231040=CARTESIAN_POINT('Ctrl Pts',(-2.78863655900006,15.2,10.017072951));
#231041=CARTESIAN_POINT('Ctrl Pts',(-2.78863655900006,11.6,10.017072951));
#231042=CARTESIAN_POINT('Ctrl Pts',(-2.78845652900006,15.2,10.015980349));
#231043=CARTESIAN_POINT('Ctrl Pts',(-2.78845652900006,11.6,10.015980349));
#231044=CARTESIAN_POINT('Ctrl Pts',(-2.78827690500006,15.2,10.014896871));
#231045=CARTESIAN_POINT('Ctrl Pts',(-2.78827690500006,11.6,10.014896871));
#231046=CARTESIAN_POINT('Ctrl Pts',(-2.78809770700006,15.2,10.013822538));
#231047=CARTESIAN_POINT('Ctrl Pts',(-2.78809770700006,11.6,10.013822538));
#231048=CARTESIAN_POINT('Ctrl Pts',(-2.78791895500006,15.2,10.012757373));
#231049=CARTESIAN_POINT('Ctrl Pts',(-2.78791895500006,11.6,10.012757373));
#231050=CARTESIAN_POINT('Ctrl Pts',(-2.78774067200006,15.2,10.011701396));
#231051=CARTESIAN_POINT('Ctrl Pts',(-2.78774067200006,11.6,10.011701396));
#231052=CARTESIAN_POINT('Ctrl Pts',(-2.78756287800006,15.2,10.01065463));
#231053=CARTESIAN_POINT('Ctrl Pts',(-2.78756287800006,11.6,10.01065463));
#231054=CARTESIAN_POINT('Ctrl Pts',(-2.78738559300006,15.2,10.009617096));
#231055=CARTESIAN_POINT('Ctrl Pts',(-2.78738559300006,11.6,10.009617096));
#231056=CARTESIAN_POINT('Ctrl Pts',(-2.78720884000006,15.2,10.008588818));
#231057=CARTESIAN_POINT('Ctrl Pts',(-2.78720884000006,11.6,10.008588818));
#231058=CARTESIAN_POINT('Ctrl Pts',(-2.78703264000006,15.2,10.007569816));
#231059=CARTESIAN_POINT('Ctrl Pts',(-2.78703264000006,11.6,10.007569816));
#231060=CARTESIAN_POINT('Ctrl Pts',(-2.78685701500006,15.2,10.006560113));
#231061=CARTESIAN_POINT('Ctrl Pts',(-2.78685701500006,11.6,10.006560113));
#231062=CARTESIAN_POINT('Ctrl Pts',(-2.78668198600006,15.2,10.005559731));
#231063=CARTESIAN_POINT('Ctrl Pts',(-2.78668198600006,11.6,10.005559731));
#231064=CARTESIAN_POINT('Ctrl Pts',(-2.78650757400006,15.2,10.004568694));
#231065=CARTESIAN_POINT('Ctrl Pts',(-2.78650757400006,11.6,10.004568694));
#231066=CARTESIAN_POINT('Ctrl Pts',(-2.78633380200006,15.2,10.003587023));
#231067=CARTESIAN_POINT('Ctrl Pts',(-2.78633380200006,11.6,10.003587023));
#231068=CARTESIAN_POINT('Ctrl Pts',(-2.78616069100006,15.2,10.002614742));
#231069=CARTESIAN_POINT('Ctrl Pts',(-2.78616069100006,11.6,10.002614742));
#231070=CARTESIAN_POINT('Ctrl Pts',(-2.78598826500006,15.2,10.001651872));
#231071=CARTESIAN_POINT('Ctrl Pts',(-2.78598826500006,11.6,10.001651872));
#231072=CARTESIAN_POINT('Ctrl Pts',(-2.78581654500006,15.2,10.000698438));
#231073=CARTESIAN_POINT('Ctrl Pts',(-2.78581654500006,11.6,10.000698438));
#231074=CARTESIAN_POINT('Ctrl Pts',(-2.78564555300005,15.2,9.99975446099998));
#231075=CARTESIAN_POINT('Ctrl Pts',(-2.78564555300005,11.6,9.99975446099998));
#231076=CARTESIAN_POINT('Ctrl Pts',(-2.78547531100005,15.2,9.99881996499998));
#231077=CARTESIAN_POINT('Ctrl Pts',(-2.78547531100005,11.6,9.99881996499998));
#231078=CARTESIAN_POINT('Ctrl Pts',(-2.78530584400006,15.2,9.99789497199998));
#231079=CARTESIAN_POINT('Ctrl Pts',(-2.78530584400006,11.6,9.99789497199998));
#231080=CARTESIAN_POINT('Ctrl Pts',(-2.78513717300005,15.2,9.99697950799998));
#231081=CARTESIAN_POINT('Ctrl Pts',(-2.78513717300005,11.6,9.99697950799998));
#231082=CARTESIAN_POINT('Ctrl Pts',(-2.78497028700006,15.2,9.99607881099998));
#231083=CARTESIAN_POINT('Ctrl Pts',(-2.78497028700006,11.6,9.99607881099998));
#231084=CARTESIAN_POINT('Ctrl Pts',(-2.78483763600006,15.2,9.99536684699999));
#231085=CARTESIAN_POINT('Ctrl Pts',(-2.78483763600006,11.6,9.99536684699999));
#231086=CARTESIAN_POINT('Ctrl Pts',(-2.78473877000006,15.2,9.99483839999998));
#231087=CARTESIAN_POINT('Ctrl Pts',(-2.78473877000006,11.6,9.99483839999998));
#231088=CARTESIAN_POINT('Ctrl Pts',(-2.78467335000005,15.2,9.99448967799999));
#231089=CARTESIAN_POINT('Ctrl Pts',(-2.78467335000005,11.6,9.99448967799999));
#231090=CARTESIAN_POINT('Ctrl Pts',(-2.78464115900006,15.2,9.99431831799999));
#231091=CARTESIAN_POINT('Ctrl Pts',(-2.78464115900006,11.6,9.99431831799999));
#231092=CARTESIAN_POINT('',(-2.78464115900006,12.2,9.99431831699999));
#231093=CARTESIAN_POINT('',(-2.78464115900006,15.2,9.99431831699999));
#231094=CARTESIAN_POINT('',(-2.78464115900006,12.2,9.99431831699999));
#231095=CARTESIAN_POINT('Ctrl Pts',(-2.71145515300006,12.2,11.175777868));
#231096=CARTESIAN_POINT('Ctrl Pts',(-2.71281861996396,12.2,11.1695539166432));
#231097=CARTESIAN_POINT('Ctrl Pts',(-2.7141664268337,12.2,11.1633453605358));
#231098=CARTESIAN_POINT('Ctrl Pts',(-2.71549860045082,12.2,11.1571522052299));
#231099=CARTESIAN_POINT('Ctrl Pts',(-2.71629790459205,12.2,11.1534363121814));
#231100=CARTESIAN_POINT('Ctrl Pts',(-2.71709157984107,12.2,11.1497259665856));
#231101=CARTESIAN_POINT('Ctrl Pts',(-2.71787964073271,12.2,11.146021201495));
#231102=CARTESIAN_POINT('Ctrl Pts',(-2.71866770162435,12.2,11.1423164364044));
#231103=CARTESIAN_POINT('Ctrl Pts',(-2.71945015054306,12.2,11.1386172539523));
#231104=CARTESIAN_POINT('Ctrl Pts',(-2.72022700793199,12.2,11.1349236969193));
#231105=CARTESIAN_POINT('Ctrl Pts',(-2.72100386532092,12.2,11.1312301398863));
#231106=CARTESIAN_POINT('Ctrl Pts',(-2.72177513241023,12.2,11.1275422097697));
#231107=CARTESIAN_POINT('Ctrl Pts',(-2.7225408290915,12.2,11.1238599450277));
#231108=CARTESIAN_POINT('Ctrl Pts',(-2.72381699027332,12.2,11.1177228369014));
#231109=CARTESIAN_POINT('Ctrl Pts',(-2.72507767193107,12.2,11.1116014639427));
#231110=CARTESIAN_POINT('Ctrl Pts',(-2.72632295664715,12.2,11.1054959789837));
#231111=CARTESIAN_POINT('Ctrl Pts',(-2.72707012744965,12.2,11.1018326881415));
#231112=CARTESIAN_POINT('Ctrl Pts',(-2.72781175456561,12.2,11.0981751182142));
#231113=CARTESIAN_POINT('Ctrl Pts',(-2.72854785787295,12.2,11.0945233075544));
#231114=CARTESIAN_POINT('Ctrl Pts',(-2.72928396131402,12.2,11.0908714962312));
#231115=CARTESIAN_POINT('Ctrl Pts',(-2.73001453998686,12.2,11.0872254438013));
#231116=CARTESIAN_POINT('Ctrl Pts',(-2.73073961488315,12.2,11.0835851884397));
#231117=CARTESIAN_POINT('Ctrl Pts',(-2.73146468964772,12.2,11.0799449337394));
#231118=CARTESIAN_POINT('Ctrl Pts',(-2.73218425928759,12.2,11.0763104755055));
#231119=CARTESIAN_POINT('Ctrl Pts',(-2.7328983425945,12.2,11.0726818498462));
#231120=CARTESIAN_POINT('Ctrl Pts',(-2.73361242590142,12.2,11.0690532241869));
#231121=CARTESIAN_POINT('Ctrl Pts',(-2.73432102293977,12.2,11.0654304316483));
#231122=CARTESIAN_POINT('Ctrl Pts',(-2.73502415275073,12.2,11.0618135084717));
#231123=CARTESIAN_POINT('Ctrl Pts',(-2.73572728256168,12.2,11.058196585295));
#231124=CARTESIAN_POINT('Ctrl Pts',(-2.73642494497144,12.2,11.054585531722));
#231125=CARTESIAN_POINT('Ctrl Pts',(-2.73711715978279,12.2,11.0509803855032));
#231126=CARTESIAN_POINT('Ctrl Pts',(-2.73780937459415,12.2,11.0473752392845));
#231127=CARTESIAN_POINT('Ctrl Pts',(-2.73849614156669,12.2,11.0437760001283));
#231128=CARTESIAN_POINT('Ctrl Pts',(-2.73917747995907,12.2,11.040182705925));
#231129=CARTESIAN_POINT('Ctrl Pts',(-2.73985881835145,12.2,11.0365894117218));
#231130=CARTESIAN_POINT('Ctrl Pts',(-2.74053472872754,12.2,11.033002061668));
#231131=CARTESIAN_POINT('Ctrl Pts',(-2.74120523057892,12.2,11.0294206940057));
#231132=CARTESIAN_POINT('Ctrl Pts',(-2.7418757325521,12.2,11.0258393256927));
#231133=CARTESIAN_POINT('Ctrl Pts',(-2.74254082566543,12.2,11.0222639392731));
#231134=CARTESIAN_POINT('Ctrl Pts',(-2.74320053013557,12.2,11.0186945729218));
#231135=CARTESIAN_POINT('Ctrl Pts',(-2.74386023448586,12.2,11.0151252072191));
#231136=CARTESIAN_POINT('Ctrl Pts',(-2.74451455080071,12.2,11.0115618612429));
#231137=CARTESIAN_POINT('Ctrl Pts',(-2.74516349814226,12.2,11.0080045728201));
#231138=CARTESIAN_POINT('Ctrl Pts',(-2.74581244548382,12.2,11.0044472843973));
#231139=CARTESIAN_POINT('Ctrl Pts',(-2.74645602327657,12.2,11.0008960528176));
#231140=CARTESIAN_POINT('Ctrl Pts',(-2.74709425358624,12.2,10.9973509176136));
#231141=CARTESIAN_POINT('Ctrl Pts',(-2.74773248389591,12.2,10.9938057824097));
#231142=CARTESIAN_POINT('Ctrl Pts',(-2.74836536568956,12.2,10.9902667426383));
#231143=CARTESIAN_POINT('Ctrl Pts',(-2.7489929200001,12.2,10.9867338364749));
#231144=CARTESIAN_POINT('Ctrl Pts',(-2.74962047431063,12.2,10.9832009303116));
#231145=CARTESIAN_POINT('Ctrl Pts',(-2.75024270067137,12.2,10.9796741575564));
#231146=CARTESIAN_POINT('Ctrl Pts',(-2.75085961998276,12.2,10.9761535573505));
#231147=CARTESIAN_POINT('Ctrl Pts',(-2.75147653929415,12.2,10.9726329571445));
#231148=CARTESIAN_POINT('Ctrl Pts',(-2.75208815058921,12.2,10.9691185289715));
#231149=CARTESIAN_POINT('Ctrl Pts',(-2.75269447685958,12.2,10.9656103107647));
#231150=CARTESIAN_POINT('Ctrl Pts',(-2.75330080324009,12.2,10.9621020919207));
#231151=CARTESIAN_POINT('Ctrl Pts',(-2.7539018424941,12.2,10.9586000833784));
#231152=CARTESIAN_POINT('Ctrl Pts',(-2.7544976174133,12.2,10.9551043240796));
#231153=CARTESIAN_POINT('Ctrl Pts',(-2.75509339222427,12.2,10.9516085654158));
#231154=CARTESIAN_POINT('Ctrl Pts',(-2.75568390197257,12.2,10.9481190555728));
#231155=CARTESIAN_POINT('Ctrl Pts',(-2.75626916789661,12.2,10.9446358333177));
#231156=CARTESIAN_POINT('Ctrl Pts',(-2.75685443382064,12.2,10.9411526110627));
#231157=CARTESIAN_POINT('Ctrl Pts',(-2.757434456134,12.2,10.9376756771618));
#231158=CARTESIAN_POINT('Ctrl Pts',(-2.75800925557099,12.2,10.9342050691218));
#231159=CARTESIAN_POINT('Ctrl Pts',(-2.75858405500798,12.2,10.9307344610817));
#231160=CARTESIAN_POINT('Ctrl Pts',(-2.7591536326706,12.2,10.9272701807576));
#231161=CARTESIAN_POINT('Ctrl Pts',(-2.7597180100251,12.2,10.9238122652166));
#231162=CARTESIAN_POINT('Ctrl Pts',(-2.76028238737959,12.2,10.9203543496756));
#231163=CARTESIAN_POINT('Ctrl Pts',(-2.76084156377596,12.2,10.9169028007176));
#231164=CARTESIAN_POINT('Ctrl Pts',(-2.76139556171462,12.2,10.9134576560922));
#231165=CARTESIAN_POINT('Ctrl Pts',(-2.76194955965328,12.2,10.9100125114668));
#231166=CARTESIAN_POINT('Ctrl Pts',(-2.76249837945352,12.2,10.9065737720116));
#231167=CARTESIAN_POINT('Ctrl Pts',(-2.76304204283652,12.2,10.9031414766724));
#231168=CARTESIAN_POINT('Ctrl Pts',(-2.76358570621952,12.2,10.8997091813332));
#231169=CARTESIAN_POINT('Ctrl Pts',(-2.76412421241916,12.2,10.8962833298386));
#231170=CARTESIAN_POINT('Ctrl Pts',(-2.76465758615048,12.2,10.892863962712));
#231171=CARTESIAN_POINT('Ctrl Pts',(-2.76519095997869,12.2,10.8894445949642));
#231172=CARTESIAN_POINT('Ctrl Pts',(-2.76571919840546,12.2,10.8860317120682));
#231173=CARTESIAN_POINT('Ctrl Pts',(-2.76624232635579,12.2,10.8826253522824));
#231174=CARTESIAN_POINT('Ctrl Pts',(-2.7667654542111,12.2,10.8792189931153));
#231175=CARTESIAN_POINT('Ctrl Pts',(-2.76728347124166,12.2,10.8758191567896));
#231176=CARTESIAN_POINT('Ctrl Pts',(-2.76779639959758,12.2,10.8724258846218));
#231177=CARTESIAN_POINT('Ctrl Pts',(-2.7683093279535,12.2,10.8690326124541));
#231178=CARTESIAN_POINT('Ctrl Pts',(-2.76881716693322,12.2,10.8656459039727));
#231179=CARTESIAN_POINT('Ctrl Pts',(-2.76931994175055,12.2,10.8622657992885));
#231180=CARTESIAN_POINT('Ctrl Pts',(-2.76982271656787,12.2,10.8588856946044));
#231181=CARTESIAN_POINT('Ctrl Pts',(-2.77032042484861,12.2,10.8555121932127));
#231182=CARTESIAN_POINT('Ctrl Pts',(-2.77081309174964,12.2,10.852145336028));
#231183=CARTESIAN_POINT('Ctrl Pts',(-2.77130575865067,12.2,10.8487784788433));
#231184=CARTESIAN_POINT('Ctrl Pts',(-2.7717933840145,12.2,10.845418264511));
#231185=CARTESIAN_POINT('Ctrl Pts',(-2.77227599045574,12.2,10.8420647353823));
#231186=CARTESIAN_POINT('Ctrl Pts',(-2.77275859689697,12.2,10.8387112062535));
#231187=CARTESIAN_POINT('Ctrl Pts',(-2.77323618464688,12.2,10.8353643617576));
#231188=CARTESIAN_POINT('Ctrl Pts',(-2.77370877763039,12.2,10.8320242417114));
#231189=CARTESIAN_POINT('Ctrl Pts',(-2.77433890166564,12.2,10.8275707479119));
#231190=CARTESIAN_POINT('Ctrl Pts',(-2.77496014623938,12.2,10.8231292099251));
#231191=CARTESIAN_POINT('Ctrl Pts',(-2.77557256877551,12.2,10.8186997239969));
#231192=CARTESIAN_POINT('Ctrl Pts',(-2.77603188563588,12.2,10.8153776098526));
#231193=CARTESIAN_POINT('Ctrl Pts',(-2.77648623934728,12.2,10.8120622756645));
#231194=CARTESIAN_POINT('Ctrl Pts',(-2.77693565520801,12.2,10.8087537615196));
#231195=CARTESIAN_POINT('Ctrl Pts',(-2.77753487641009,12.2,10.8043424089258));
#231196=CARTESIAN_POINT('Ctrl Pts',(-2.77812531660605,12.2,10.7999431811761));
#231197=CARTESIAN_POINT('Ctrl Pts',(-2.77870703780353,12.2,10.7955561760493));
#231198=CARTESIAN_POINT('Ctrl Pts',(-2.77928875892175,12.2,10.7911691715203));
#231199=CARTESIAN_POINT('Ctrl Pts',(-2.77986175804667,12.2,10.7867943898008));
#231200=CARTESIAN_POINT('Ctrl Pts',(-2.78042609594554,12.2,10.7824319298234));
#231201=CARTESIAN_POINT('Ctrl Pts',(-2.7809904339213,12.2,10.7780694692515));
#231202=CARTESIAN_POINT('Ctrl Pts',(-2.78154611068692,12.2,10.7737193302587));
#231203=CARTESIAN_POINT('Ctrl Pts',(-2.78209318535443,12.2,10.7693816108623));
#231204=CARTESIAN_POINT('Ctrl Pts',(-2.7826402599474,12.2,10.7650438920568));
#231205=CARTESIAN_POINT('Ctrl Pts',(-2.78317873119667,12.2,10.7607185939203));
#231206=CARTESIAN_POINT('Ctrl Pts',(-2.78370866243169,12.2,10.7564058153276));
#231207=CARTESIAN_POINT('Ctrl Pts',(-2.78423859373891,12.2,10.7520930361473));
#231208=CARTESIAN_POINT('Ctrl Pts',(-2.78475998396732,12.2,10.747792777624));
#231209=CARTESIAN_POINT('Ctrl Pts',(-2.78527289405027,12.2,10.7435051378912));
#231210=CARTESIAN_POINT('Ctrl Pts',(-2.78578580406334,12.2,10.7392174987426));
#231211=CARTESIAN_POINT('Ctrl Pts',(-2.78629023610144,12.2,10.7349424814397));
#231212=CARTESIAN_POINT('Ctrl Pts',(-2.78678624891974,12.2,10.7306801833518));
#231213=CARTESIAN_POINT('Ctrl Pts',(-2.78728226180562,12.2,10.7264178846832));
#231214=CARTESIAN_POINT('Ctrl Pts',(-2.78776985954695,12.2,10.7221683065615));
#231215=CARTESIAN_POINT('Ctrl Pts',(-2.78824910157252,12.2,10.717931551887));
#231216=CARTESIAN_POINT('Ctrl Pts',(-2.7887283435328,12.2,10.7136947977898));
#231217=CARTESIAN_POINT('Ctrl Pts',(-2.78919923188086,12.2,10.7094708651316));
#231218=CARTESIAN_POINT('Ctrl Pts',(-2.78966182989945,12.2,10.7052598571968));
#231219=CARTESIAN_POINT('Ctrl Pts',(-2.79012442798107,12.2,10.7010488486882));
#231220=CARTESIAN_POINT('Ctrl Pts',(-2.79057873602685,12.2,10.696850763997));
#231221=CARTESIAN_POINT('Ctrl Pts',(-2.79102481877539,12.2,10.6926657074721));
#231222=CARTESIAN_POINT('Ctrl Pts',(-2.79147090146315,12.2,10.6884806515174));
#231223=CARTESIAN_POINT('Ctrl Pts',(-2.79190875953079,12.2,10.6843086209079));
#231224=CARTESIAN_POINT('Ctrl Pts',(-2.79233845816316,12.2,10.6801497229133));
#231225=CARTESIAN_POINT('Ctrl Pts',(-2.79276815685408,12.2,10.6759908243519));
#231226=CARTESIAN_POINT('Ctrl Pts',(-2.79318969651368,12.2,10.6718450558112));
#231227=CARTESIAN_POINT('Ctrl Pts',(-2.79360314325842,12.2,10.6677125219749));
#231228=CARTESIAN_POINT('Ctrl Pts',(-2.79401659000317,12.2,10.6635799881386));
#231229=CARTESIAN_POINT('Ctrl Pts',(-2.7944219447831,12.2,10.6594606899399));
#231230=CARTESIAN_POINT('Ctrl Pts',(-2.79481927358171,12.2,10.6553547308286));
#231231=CARTESIAN_POINT('Ctrl Pts',(-2.79531593449877,12.2,10.6502222827787));
#231232=CARTESIAN_POINT('Ctrl Pts',(-2.79580005608323,12.2,10.6451106764404));
#231233=CARTESIAN_POINT('Ctrl Pts',(-2.79627177346338,12.2,10.6400201208825));
#231234=CARTESIAN_POINT('Ctrl Pts',(-2.7966491474292,12.2,10.6359476757703));
#231235=CARTESIAN_POINT('Ctrl Pts',(-2.79701858150538,12.2,10.6318887028815));
#231236=CARTESIAN_POINT('Ctrl Pts',(-2.79738014569176,12.2,10.6278433065499));
#231237=CARTESIAN_POINT('Ctrl Pts',(-2.79774170987813,12.2,10.6237979102183));
#231238=CARTESIAN_POINT('Ctrl Pts',(-2.79809540574137,12.2,10.6197660935549));
#231239=CARTESIAN_POINT('Ctrl Pts',(-2.79844130181497,12.2,10.6157479605596));
#231240=CARTESIAN_POINT('Ctrl Pts',(-2.79878719784145,12.2,10.6117298281118));
#231241=CARTESIAN_POINT('Ctrl Pts',(-2.79912529522451,12.2,10.6077253823454));
#231242=CARTESIAN_POINT('Ctrl Pts',(-2.799455664698,12.2,10.6037347285596));
#231243=CARTESIAN_POINT('Ctrl Pts',(-2.79978603421651,12.2,10.5997440742302));
#231244=CARTESIAN_POINT('Ctrl Pts',(-2.80010867739129,12.2,10.5957672132572));
#231245=CARTESIAN_POINT('Ctrl Pts',(-2.80042366431242,12.2,10.5918042539));
#231246=CARTESIAN_POINT('Ctrl Pts',(-2.80073865119063,12.2,10.5878412950827));
#231247=CARTESIAN_POINT('Ctrl Pts',(-2.80104598424952,12.2,10.5838922378927));
#231248=CARTESIAN_POINT('Ctrl Pts',(-2.80134573622551,12.2,10.5799571920467));
#231249=CARTESIAN_POINT('Ctrl Pts',(-2.80172042622613,12.2,10.5750383843372));
#231250=CARTESIAN_POINT('Ctrl Pts',(-2.80208326965978,12.2,10.5701414696755));
#231251=CARTESIAN_POINT('Ctrl Pts',(-2.80243441320205,12.2,10.5652666620355));
#231252=CARTESIAN_POINT('Ctrl Pts',(-2.80271532805118,12.2,10.561366815711));
#231253=CARTESIAN_POINT('Ctrl Pts',(-2.80298875558372,12.2,10.5574811186609));
#231254=CARTESIAN_POINT('Ctrl Pts',(-2.80325477105531,12.2,10.5536096819799));
#231255=CARTESIAN_POINT('Ctrl Pts',(-2.80352078649065,12.2,10.5497382458264));
#231256=CARTESIAN_POINT('Ctrl Pts',(-2.80377938992731,12.2,10.5458810695954));
#231257=CARTESIAN_POINT('Ctrl Pts',(-2.80403065746281,12.2,10.5420382657976));
#231258=CARTESIAN_POINT('Ctrl Pts',(-2.80428192503253,12.2,10.5381954614761));
#231259=CARTESIAN_POINT('Ctrl Pts',(-2.80452585824305,12.2,10.534367030223));
#231260=CARTESIAN_POINT('Ctrl Pts',(-2.8047625349777,12.2,10.5305530832383));
#231261=CARTESIAN_POINT('Ctrl Pts',(-2.8049992116801,12.2,10.5267391367732));
#231262=CARTESIAN_POINT('Ctrl Pts',(-2.80522863103812,12.2,10.522939676158));
#231263=CARTESIAN_POINT('Ctrl Pts',(-2.80545087197613,12.2,10.5191548134992));
#231264=CARTESIAN_POINT('Ctrl Pts',(-2.80572867317135,12.2,10.514423734789));
#231265=CARTESIAN_POINT('Ctrl Pts',(-2.80599525983273,12.2,10.5097154677188));
#231266=CARTESIAN_POINT('Ctrl Pts',(-2.80625078670831,12.2,10.5050302343148));
#231267=CARTESIAN_POINT('Ctrl Pts',(-2.80645520821991,12.2,10.5012820473874));
#231268=CARTESIAN_POINT('Ctrl Pts',(-2.80665255356677,12.2,10.4975486028395));
#231269=CARTESIAN_POINT('Ctrl Pts',(-2.80684290179891,12.2,10.4938300164711));
#231270=CARTESIAN_POINT('Ctrl Pts',(-2.80703325000512,12.2,10.4901114306093));
#231271=CARTESIAN_POINT('Ctrl Pts',(-2.80721660240723,12.2,10.486407702086));
#231272=CARTESIAN_POINT('Ctrl Pts',(-2.80739304195778,12.2,10.4827189475353));
#231273=CARTESIAN_POINT('Ctrl Pts',(-2.80756948153236,12.2,10.479030192482));
#231274=CARTESIAN_POINT('Ctrl Pts',(-2.80773900726324,12.2,10.4753564130104));
#231275=CARTESIAN_POINT('Ctrl Pts',(-2.80790170477165,12.2,10.471697724701));
#231276=CARTESIAN_POINT('Ctrl Pts',(-2.8080644022579,12.2,10.46803903689));
#231277=CARTESIAN_POINT('Ctrl Pts',(-2.80822027035108,12.2,10.4643954415787));
#231278=CARTESIAN_POINT('Ctrl Pts',(-2.8083693939507,12.2,10.4607670558182));
#231279=CARTESIAN_POINT('Ctrl Pts',(-2.80851851757063,12.2,10.4571386695633));
#231280=CARTESIAN_POINT('Ctrl Pts',(-2.80866089775329,12.2,10.4535254935709));
#231281=CARTESIAN_POINT('Ctrl Pts',(-2.80879661998351,12.2,10.4499276472475));
#231282=CARTESIAN_POINT('Ctrl Pts',(-2.80893234219523,12.2,10.4463298014142));
#231283=CARTESIAN_POINT('Ctrl Pts',(-2.80906140671995,12.2,10.4427472858459));
#231284=CARTESIAN_POINT('Ctrl Pts',(-2.80918390098838,12.2,10.4391802188581));
#231285=CARTESIAN_POINT('Ctrl Pts',(-2.80930639527351,12.2,10.4356131513843));
#231286=CARTESIAN_POINT('Ctrl Pts',(-2.8094223200969,12.2,10.4320615346203));
#231287=CARTESIAN_POINT('Ctrl Pts',(-2.80953176249175,12.2,10.4285254889833));
#231288=CARTESIAN_POINT('Ctrl Pts',(-2.8096412048866,12.2,10.4249894433462));
#231289=CARTESIAN_POINT('Ctrl Pts',(-2.80974416743904,12.2,10.4214689690302));
#231290=CARTESIAN_POINT('Ctrl Pts',(-2.80984073833253,12.2,10.4179641874519));
#231291=CARTESIAN_POINT('Ctrl Pts',(-2.80996145192967,12.2,10.4135832111954));
#231292=CARTESIAN_POINT('Ctrl Pts',(-2.81007217891929,12.2,10.4092267559631));
#231293=CARTESIAN_POINT('Ctrl Pts',(-2.81017309772854,12.2,10.4048950630998));
#231294=CARTESIAN_POINT('Ctrl Pts',(-2.8102740165488,12.2,10.4005633697644));
#231295=CARTESIAN_POINT('Ctrl Pts',(-2.81036512871086,12.2,10.3962564396454));
#231296=CARTESIAN_POINT('Ctrl Pts',(-2.81044661648942,12.2,10.39197451381));
#231297=CARTESIAN_POINT('Ctrl Pts',(-2.81051180671583,12.2,10.388548972955));
#231298=CARTESIAN_POINT('Ctrl Pts',(-2.81057083593034,12.2,10.3851394349924));
#231299=CARTESIAN_POINT('Ctrl Pts',(-2.81062380026678,12.2,10.3817460280143));
#231300=CARTESIAN_POINT('Ctrl Pts',(-2.810676764596,12.2,10.3783526214986));
#231301=CARTESIAN_POINT('Ctrl Pts',(-2.81072366321001,12.2,10.3749753441125));
#231302=CARTESIAN_POINT('Ctrl Pts',(-2.81076459348505,12.2,10.3716143237745));
#231303=CARTESIAN_POINT('Ctrl Pts',(-2.81080552376568,12.2,10.3682533029785));
#231304=CARTESIAN_POINT('Ctrl Pts',(-2.81084048466238,12.2,10.3649085389119));
#231305=CARTESIAN_POINT('Ctrl Pts',(-2.81086957427508,12.2,10.3615801600082));
#231306=CARTESIAN_POINT('Ctrl Pts',(-2.81090593628897,12.2,10.3574196866054));
#231307=CARTESIAN_POINT('Ctrl Pts',(-2.81093312448892,12.2,10.3532848137552));
#231308=CARTESIAN_POINT('Ctrl Pts',(-2.81095133101675,12.2,10.3491757954727));
#231309=CARTESIAN_POINT('Ctrl Pts',(-2.81097317884937,12.2,10.3442449737128));
#231310=CARTESIAN_POINT('Ctrl Pts',(-2.81098209669121,12.2,10.3393513828899));
#231311=CARTESIAN_POINT('Ctrl Pts',(-2.81097842327522,12.2,10.3344954632314));
#231312=CARTESIAN_POINT('Ctrl Pts',(-2.81097536209512,12.2,10.3304488633689));
#231313=CARTESIAN_POINT('Ctrl Pts',(-2.8109635582398,12.2,10.3264284254738));
#231314=CARTESIAN_POINT('Ctrl Pts',(-2.81094321372636,12.2,10.3224344087363));
#231315=CARTESIAN_POINT('Ctrl Pts',(-2.81092286921291,12.2,10.3184403919987));
#231316=CARTESIAN_POINT('Ctrl Pts',(-2.81089398195202,12.2,10.3144727960815));
#231317=CARTESIAN_POINT('Ctrl Pts',(-2.81085676153579,12.2,10.3105318828162));
#231318=CARTESIAN_POINT('Ctrl Pts',(-2.81081954111956,12.2,10.3065909695509));
#231319=CARTESIAN_POINT('Ctrl Pts',(-2.81077398338366,12.2,10.3026767395475));
#231320=CARTESIAN_POINT('Ctrl Pts',(-2.81072030150844,12.2,10.298789458002));
#231321=CARTESIAN_POINT('Ctrl Pts',(-2.81066661963322,12.2,10.2949021764566));
#231322=CARTESIAN_POINT('Ctrl Pts',(-2.81060481270563,12.2,10.2910418444166));
#231323=CARTESIAN_POINT('Ctrl Pts',(-2.81053509402508,12.2,10.2872087287916));
#231324=CARTESIAN_POINT('Ctrl Pts',(-2.81046537534452,12.2,10.2833756131666));
#231325=CARTESIAN_POINT('Ctrl Pts',(-2.81038774418933,12.2,10.2795697137705));
#231326=CARTESIAN_POINT('Ctrl Pts',(-2.81030241905003,12.2,10.2757913054895));
#231327=CARTESIAN_POINT('Ctrl Pts',(-2.81021709391073,12.2,10.2720128972086));
#231328=CARTESIAN_POINT('Ctrl Pts',(-2.81012407523829,12.2,10.2682619765996));
#231329=CARTESIAN_POINT('Ctrl Pts',(-2.81002358496012,12.2,10.2645388217399));
#231330=CARTESIAN_POINT('Ctrl Pts',(-2.80992309468195,12.2,10.2608156668803));
#231331=CARTESIAN_POINT('Ctrl Pts',(-2.80981513335954,12.2,10.2571202757921));
#231332=CARTESIAN_POINT('Ctrl Pts',(-2.80969992502583,12.2,10.2534529285019));
#231333=CARTESIAN_POINT('Ctrl Pts',(-2.80958471669212,12.2,10.2497855812117));
#231334=CARTESIAN_POINT('Ctrl Pts',(-2.80946226480308,12.2,10.2461462782537));
#231335=CARTESIAN_POINT('Ctrl Pts',(-2.80933279722669,12.2,10.2425353000892));
#231336=CARTESIAN_POINT('Ctrl Pts',(-2.80920332965029,12.2,10.2389243219246));
#231337=CARTESIAN_POINT('Ctrl Pts',(-2.80906684851522,12.2,10.2353416698494));
#231338=CARTESIAN_POINT('Ctrl Pts',(-2.80892358768133,12.2,10.23178763006));
#231339=CARTESIAN_POINT('Ctrl Pts',(-2.80875167468692,12.2,10.2275227824678));
#231340=CARTESIAN_POINT('Ctrl Pts',(-2.8085699999856,12.2,10.2232991351234));
#231341=CARTESIAN_POINT('Ctrl Pts',(-2.80837898074165,12.2,10.2191171915063));
#231342=CARTESIAN_POINT('Ctrl Pts',(-2.80821979803257,12.2,10.2156322383655));
#231343=CARTESIAN_POINT('Ctrl Pts',(-2.80805412475578,12.2,10.2121762438355));
#231344=CARTESIAN_POINT('Ctrl Pts',(-2.80788220725546,12.2,10.208749506476));
#231345=CARTESIAN_POINT('Ctrl Pts',(-2.80771028975513,12.2,10.2053227691164));
#231346=CARTESIAN_POINT('Ctrl Pts',(-2.80753212928275,12.2,10.2019252859783));
#231347=CARTESIAN_POINT('Ctrl Pts',(-2.80734797525466,12.2,10.1985573570215));
#231348=CARTESIAN_POINT('Ctrl Pts',(-2.80709015963139,12.2,10.1938422567757));
#231349=CARTESIAN_POINT('Ctrl Pts',(-2.80682059910816,12.2,10.1891850798021));
#231350=CARTESIAN_POINT('Ctrl Pts',(-2.80653999625128,12.2,10.1845866627379));
#231351=CARTESIAN_POINT('Ctrl Pts',(-2.80629947948873,12.2,10.1806451619368));
#231352=CARTESIAN_POINT('Ctrl Pts',(-2.8060508531587,12.2,10.1767468304232));
#231353=CARTESIAN_POINT('Ctrl Pts',(-2.80579457222774,12.2,10.1728922027983));
#231354=CARTESIAN_POINT('Ctrl Pts',(-2.80553829132005,12.2,10.1690375755236));
#231355=CARTESIAN_POINT('Ctrl Pts',(-2.80527435617489,12.2,10.1652266519903));
#231356=CARTESIAN_POINT('Ctrl Pts',(-2.80500323451686,12.2,10.1614599785266));
#231357=CARTESIAN_POINT('Ctrl Pts',(-2.80473211285883,12.2,10.1576933050629));
#231358=CARTESIAN_POINT('Ctrl Pts',(-2.80445380643698,12.2,10.1539708785952));
#231359=CARTESIAN_POINT('Ctrl Pts',(-2.80416879378113,12.2,10.1502932561424));
#231360=CARTESIAN_POINT('Ctrl Pts',(-2.80388378109939,12.2,10.1466156333556));
#231361=CARTESIAN_POINT('Ctrl Pts',(-2.80359206356105,12.2,10.1429828111584));
#231362=CARTESIAN_POINT('Ctrl Pts',(-2.80329413277956,12.2,10.139395356453));
#231363=CARTESIAN_POINT('Ctrl Pts',(-2.80299620202515,12.2,10.1358079020734));
#231364=CARTESIAN_POINT('Ctrl Pts',(-2.80269205783048,12.2,10.1322658141479));
#231365=CARTESIAN_POINT('Ctrl Pts',(-2.8023822072584,12.2,10.1287696670249));
#231366=CARTESIAN_POINT('Ctrl Pts',(-2.80207235668633,12.2,10.1252735199019));
#231367=CARTESIAN_POINT('Ctrl Pts',(-2.80175679923515,12.2,10.1218233145367));
#231368=CARTESIAN_POINT('Ctrl Pts',(-2.80143605356441,12.2,10.1184196360709));
#231369=CARTESIAN_POINT('Ctrl Pts',(-2.80111530786454,12.2,10.1150159572961));
#231370=CARTESIAN_POINT('Ctrl Pts',(-2.80078937240736,12.2,10.1116588047413));
#231371=CARTESIAN_POINT('Ctrl Pts',(-2.80045878297236,12.2,10.1083487771475));
#231372=CARTESIAN_POINT('Ctrl Pts',(-2.80007309534324,12.2,10.104487078739));
#231373=CARTESIAN_POINT('Ctrl Pts',(-2.79968107048435,12.2,10.1006895201144));
#231374=CARTESIAN_POINT('Ctrl Pts',(-2.7992835797872,12.2,10.0969570711486));
#231375=CARTESIAN_POINT('Ctrl Pts',(-2.79894287343557,12.2,10.0937578288044));
#231376=CARTESIAN_POINT('Ctrl Pts',(-2.79859815189461,12.2,10.0906064231295));
#231377=CARTESIAN_POINT('Ctrl Pts',(-2.79824998044137,12.2,10.0875034757249));
#231378=CARTESIAN_POINT('Ctrl Pts',(-2.79790180901977,12.2,10.0844005286021));
#231379=CARTESIAN_POINT('Ctrl Pts',(-2.79755018529552,12.2,10.0813460427824));
#231380=CARTESIAN_POINT('Ctrl Pts',(-2.79719569472506,12.2,10.0783406519749));
#231381=CARTESIAN_POINT('Ctrl Pts',(-2.7968412041546,12.2,10.0753352611674));
#231382=CARTESIAN_POINT('Ctrl Pts',(-2.79648384147295,12.2,10.072378967257));
#231383=CARTESIAN_POINT('Ctrl Pts',(-2.79612420730151,12.2,10.0694724210479));
#231384=CARTESIAN_POINT('Ctrl Pts',(-2.79576457309741,12.2,10.0665658745747));
#231385=CARTESIAN_POINT('Ctrl Pts',(-2.79540266705536,12.2,10.0637090725018));
#231386=CARTESIAN_POINT('Ctrl Pts',(-2.7950391019521,12.2,10.0609026844357));
#231387=CARTESIAN_POINT('Ctrl Pts',(-2.79467553688187,12.2,10.0580962966244));
#231388=CARTESIAN_POINT('Ctrl Pts',(-2.79431031332991,12.2,10.0553403202792));
#231389=CARTESIAN_POINT('Ctrl Pts',(-2.79394406325822,12.2,10.052635435532));
#231390=CARTESIAN_POINT('Ctrl Pts',(-2.79357781318653,12.2,10.0499305507847));
#231391=CARTESIAN_POINT('Ctrl Pts',(-2.79321053627339,12.2,10.0472767573413));
#231392=CARTESIAN_POINT('Ctrl Pts',(-2.79284288428676,12.2,10.0446747506836));
#231393=CARTESIAN_POINT('Ctrl Pts',(-2.79247523226674,12.2,10.0420727437895));
#231394=CARTESIAN_POINT('Ctrl Pts',(-2.79210720367999,12.2,10.0395225250769));
#231395=CARTESIAN_POINT('Ctrl Pts',(-2.7917394689933,12.2,10.0370248034443));
#231396=CARTESIAN_POINT('Ctrl Pts',(-2.79137173434002,12.2,10.0345270820386));
#231397=CARTESIAN_POINT('Ctrl Pts',(-2.79100429403339,12.2,10.0320818608305));
#231398=CARTESIAN_POINT('Ctrl Pts',(-2.79063783821342,12.2,10.0296898664198));
#231399=CARTESIAN_POINT('Ctrl Pts',(-2.79027138239345,12.2,10.027297872009));
#231400=CARTESIAN_POINT('Ctrl Pts',(-2.78990591142341,12.2,10.0249591074523));
#231401=CARTESIAN_POINT('Ctrl Pts',(-2.78954213576989,12.2,10.0226743151163));
#231402=CARTESIAN_POINT('Ctrl Pts',(-2.78917836011637,12.2,10.0203895227803));
#231403=CARTESIAN_POINT('Ctrl Pts',(-2.78881628091801,12.2,10.0181587065701));
#231404=CARTESIAN_POINT('Ctrl Pts',(-2.78845663051425,12.2,10.0159826302288));
#231405=CARTESIAN_POINT('Ctrl Pts',(-2.78809698007782,12.2,10.0138065536898));
#231406=CARTESIAN_POINT('Ctrl Pts',(-2.7877397603166,12.2,10.0116852182978));
#231407=CARTESIAN_POINT('Ctrl Pts',(-2.7873857259641,12.2,10.0096194098542));
#231408=CARTESIAN_POINT('Ctrl Pts',(-2.78703169164377,12.2,10.0075536015983));
#231409=CARTESIAN_POINT('Ctrl Pts',(-2.78668084651418,12.2,10.0055433186638));
#231410=CARTESIAN_POINT('Ctrl Pts',(-2.7863339672752,12.2,10.0035893704758));
#231411=CARTESIAN_POINT('Ctrl Pts',(-2.7857574999564,12.2,10.0003421675693));
#231412=CARTESIAN_POINT('Ctrl Pts',(-2.78519199058759,12.2,9.99725051957323));
#231413=CARTESIAN_POINT('Ctrl Pts',(-2.78464115900006,12.2,9.99431831799999));
#231414=CARTESIAN_POINT('Ctrl Pts',(-2.78464115900006,15.2,9.99431831799999));
#231415=CARTESIAN_POINT('Ctrl Pts',(-2.78497102164681,15.2,9.9960742517439));
#231416=CARTESIAN_POINT('Ctrl Pts',(-2.7853061480725,15.2,9.99788737721449));
#231417=CARTESIAN_POINT('Ctrl Pts',(-2.78564574048785,15.2,9.99975683102847));
#231418=CARTESIAN_POINT('Ctrl Pts',(-2.78598697058949,15.2,10.0016353002937));
#231419=CARTESIAN_POINT('Ctrl Pts',(-2.78633270293049,15.2,10.0035706519564));
#231420=CARTESIAN_POINT('Ctrl Pts',(-2.78668214030053,15.2,10.0055620674177));
#231421=CARTESIAN_POINT('Ctrl Pts',(-2.78703157763883,15.2,10.007553482698));
#231422=CARTESIAN_POINT('Ctrl Pts',(-2.78738472059632,15.2,10.0096009594763));
#231423=CARTESIAN_POINT('Ctrl Pts',(-2.78774079425005,15.2,10.0117036987332));
#231424=CARTESIAN_POINT('Ctrl Pts',(-2.78809686790378,15.2,10.0138064379902));
#231425=CARTESIAN_POINT('Ctrl Pts',(-2.78845587543532,15.2,10.015964439659));
#231426=CARTESIAN_POINT('Ctrl Pts',(-2.78881706319012,15.2,10.0181769250193));
#231427=CARTESIAN_POINT('Ctrl Pts',(-2.78917825097771,15.2,10.0203894105806));
#231428=CARTESIAN_POINT('Ctrl Pts',(-2.78954162379485,15.2,10.0226563798811));
#231429=CARTESIAN_POINT('Ctrl Pts',(-2.78990645056482,15.2,10.0249770707612));
#231430=CARTESIAN_POINT('Ctrl Pts',(-2.79027127730165,15.2,10.0272977614305));
#231431=CARTESIAN_POINT('Ctrl Pts',(-2.79063756082855,15.2,10.0296721774031));
#231432=CARTESIAN_POINT('Ctrl Pts',(-2.79100459748355,15.2,10.0320995767427));
#231433=CARTESIAN_POINT('Ctrl Pts',(-2.79137163413856,15.2,10.0345269760823));
#231434=CARTESIAN_POINT('Ctrl Pts',(-2.79173942030171,15.2,10.0370073571481));
#231435=CARTESIAN_POINT('Ctrl Pts',(-2.79210727620501,15.2,10.0395399978038));
#231436=CARTESIAN_POINT('Ctrl Pts',(-2.79247513214172,15.2,10.0420726386895));
#231437=CARTESIAN_POINT('Ctrl Pts',(-2.79284305736179,15.2,10.0446575395651));
#231438=CARTESIAN_POINT('Ctrl Pts',(-2.79321038729843,15.2,10.0472939942956));
#231439=CARTESIAN_POINT('Ctrl Pts',(-2.7935777172017,15.2,10.0499304487866));
#231440=CARTESIAN_POINT('Ctrl Pts',(-2.79394445291664,15.2,10.0526184549133));
#231441=CARTESIAN_POINT('Ctrl Pts',(-2.79430994806997,15.2,10.0553573256494));
#231442=CARTESIAN_POINT('Ctrl Pts',(-2.79467544322331,15.2,10.0580961963854));
#231443=CARTESIAN_POINT('Ctrl Pts',(-2.79503970031006,15.2,10.060885930059));
#231444=CARTESIAN_POINT('Ctrl Pts',(-2.79540209146363,15.2,10.0637258528703));
#231445=CARTESIAN_POINT('Ctrl Pts',(-2.79576448261721,15.2,10.0665657756816));
#231446=CARTESIAN_POINT('Ctrl Pts',(-2.79612500880721,15.2,10.0694558861813));
#231447=CARTESIAN_POINT('Ctrl Pts',(-2.79648306196103,15.2,10.0723955259878));
#231448=CARTESIAN_POINT('Ctrl Pts',(-2.79684111514738,15.2,10.0753351660613));
#231449=CARTESIAN_POINT('Ctrl Pts',(-2.79719669448351,15.2,10.0783243339647));
#231450=CARTESIAN_POINT('Ctrl Pts',(-2.79754920883593,15.2,10.0813623851324));
#231451=CARTESIAN_POINT('Ctrl Pts',(-2.79790172315632,15.2,10.0844004360241));
#231452=CARTESIAN_POINT('Ctrl Pts',(-2.79825117216088,15.2,10.0874873693649));
#231453=CARTESIAN_POINT('Ctrl Pts',(-2.79859698148324,15.2,10.0906225532652));
#231454=CARTESIAN_POINT('Ctrl Pts',(-2.79900042571359,15.2,10.0942802680053));
#231455=CARTESIAN_POINT('Ctrl Pts',(-2.79939891254026,15.2,10.0980036552378));
#231456=CARTESIAN_POINT('Ctrl Pts',(-2.79979155926839,15.2,10.1017917346604));
#231457=CARTESIAN_POINT('Ctrl Pts',(-2.80012811358931,15.2,10.1050386597112));
#231458=CARTESIAN_POINT('Ctrl Pts',(-2.80046037415222,15.2,10.1083331142665));
#231459=CARTESIAN_POINT('Ctrl Pts',(-2.80078780072386,15.2,10.111674491393));
#231460=CARTESIAN_POINT('Ctrl Pts',(-2.80111522729551,15.2,10.1150158685195));
#231461=CARTESIAN_POINT('Ctrl Pts',(-2.80143782030164,15.2,10.1184041704702));
#231462=CARTESIAN_POINT('Ctrl Pts',(-2.80175505070715,15.2,10.1218388016755));
#231463=CARTESIAN_POINT('Ctrl Pts',(-2.80207228114147,15.2,10.1252734331929));
#231464=CARTESIAN_POINT('Ctrl Pts',(-2.80238414665863,15.2,10.1287543959148));
#231465=CARTESIAN_POINT('Ctrl Pts',(-2.80269013725838,15.2,10.1322811064423));
#231466=CARTESIAN_POINT('Ctrl Pts',(-2.80299612783034,15.2,10.1358078166494));
#231467=CARTESIAN_POINT('Ctrl Pts',(-2.80329624015926,15.2,10.1393802749717));
#231468=CARTESIAN_POINT('Ctrl Pts',(-2.8035899748166,15.2,10.1429979119399));
#231469=CARTESIAN_POINT('Ctrl Pts',(-2.80388370947394,15.2,10.1466155489081));
#231470=CARTESIAN_POINT('Ctrl Pts',(-2.80417106491254,15.2,10.1502783616335));
#231471=CARTESIAN_POINT('Ctrl Pts',(-2.80445155373616,15.2,10.1539857918291));
#231472=CARTESIAN_POINT('Ctrl Pts',(-2.80477879071402,15.2,10.1583111272819));
#231473=CARTESIAN_POINT('Ctrl Pts',(-2.8050966796604,15.2,10.1626971897311));
#231474=CARTESIAN_POINT('Ctrl Pts',(-2.80540446820828,15.2,10.1671431084732));
#231475=CARTESIAN_POINT('Ctrl Pts',(-2.80571225675616,15.2,10.1715890272153));
#231476=CARTESIAN_POINT('Ctrl Pts',(-2.8060099429316,15.2,10.1760947993178));
#231477=CARTESIAN_POINT('Ctrl Pts',(-2.8062967935051,15.2,10.1806595712383));
#231478=CARTESIAN_POINT('Ctrl Pts',(-2.80658364405628,15.2,10.1852243428035));
#231479=CARTESIAN_POINT('Ctrl Pts',(-2.8068596611745,15.2,10.1898481137241));
#231480=CARTESIAN_POINT('Ctrl Pts',(-2.80712413049203,15.2,10.1945300465125));
#231481=CARTESIAN_POINT('Ctrl Pts',(-2.80731303715918,15.2,10.1978742844268));
#231482=CARTESIAN_POINT('Ctrl Pts',(-2.80749605282088,15.2,10.2012481962405));
#231483=CARTESIAN_POINT('Ctrl Pts',(-2.80767292525193,15.2,10.2046514824881));
#231484=CARTESIAN_POINT('Ctrl Pts',(-2.80788517218078,15.2,10.2087354262079));
#231485=CARTESIAN_POINT('Ctrl Pts',(-2.80808857128242,15.2,10.2128616674821));
#231486=CARTESIAN_POINT('Ctrl Pts',(-2.80828269430216,15.2,10.2170296974199));
#231487=CARTESIAN_POINT('Ctrl Pts',(-2.80844446347646,15.2,10.2205030555121));
#231488=CARTESIAN_POINT('Ctrl Pts',(-2.80859979202005,15.2,10.2240054312428));
#231489=CARTESIAN_POINT('Ctrl Pts',(-2.80874843701951,15.2,10.2275365352035));
#231490=CARTESIAN_POINT('Ctrl Pts',(-2.80889708201897,15.2,10.2310676391641));
#231491=CARTESIAN_POINT('Ctrl Pts',(-2.80903904387386,15.2,10.2346274710503));
#231492=CARTESIAN_POINT('Ctrl Pts',(-2.80917408477607,15.2,10.2382157425109));
#231493=CARTESIAN_POINT('Ctrl Pts',(-2.80930912566356,15.2,10.2418040135805));
#231494=CARTESIAN_POINT('Ctrl Pts',(-2.80943724665241,15.2,10.2454207239672));
#231495=CARTESIAN_POINT('Ctrl Pts',(-2.80955821275092,15.2,10.2490655907898));
#231496=CARTESIAN_POINT('Ctrl Pts',(-2.80972756530992,15.2,10.2541684049772));
#231497=CARTESIAN_POINT('Ctrl Pts',(-2.80988289856849,15.2,10.2593264048552));
#231498=CARTESIAN_POINT('Ctrl Pts',(-2.81002358496012,15.2,10.2645388217399));
#231499=CARTESIAN_POINT('Ctrl Pts',(-2.81012407523829,15.2,10.2682619765996));
#231500=CARTESIAN_POINT('Ctrl Pts',(-2.81021709391073,15.2,10.2720128972086));
#231501=CARTESIAN_POINT('Ctrl Pts',(-2.81030241905003,15.2,10.2757913054895));
#231502=CARTESIAN_POINT('Ctrl Pts',(-2.81038774418933,15.2,10.2795697137705));
#231503=CARTESIAN_POINT('Ctrl Pts',(-2.81046537534452,15.2,10.2833756131666));
#231504=CARTESIAN_POINT('Ctrl Pts',(-2.81053509402508,15.2,10.2872087287916));
#231505=CARTESIAN_POINT('Ctrl Pts',(-2.81060481270563,15.2,10.2910418444166));
#231506=CARTESIAN_POINT('Ctrl Pts',(-2.81066661963322,15.2,10.2949021764565));
#231507=CARTESIAN_POINT('Ctrl Pts',(-2.81072030150844,15.2,10.298789458002));
#231508=CARTESIAN_POINT('Ctrl Pts',(-2.81077398338366,15.2,10.3026767395475));
#231509=CARTESIAN_POINT('Ctrl Pts',(-2.81081954111956,15.2,10.3065909695509));
#231510=CARTESIAN_POINT('Ctrl Pts',(-2.81085676153579,15.2,10.3105318828162));
#231511=CARTESIAN_POINT('Ctrl Pts',(-2.81090142603365,15.2,10.3152609785627));
#231512=CARTESIAN_POINT('Ctrl Pts',(-2.81093408968245,15.2,10.3200284964061));
#231513=CARTESIAN_POINT('Ctrl Pts',(-2.81095439401559,15.2,10.3248339869798));
#231514=CARTESIAN_POINT('Ctrl Pts',(-2.81097808240547,15.2,10.3304403929402));
#231515=CARTESIAN_POINT('Ctrl Pts',(-2.81098495125587,15.2,10.3360984795428));
#231516=CARTESIAN_POINT('Ctrl Pts',(-2.81097444824174,15.2,10.3418075407271));
#231517=CARTESIAN_POINT('Ctrl Pts',(-2.8109669460889,15.2,10.3458854415096));
#231518=CARTESIAN_POINT('Ctrl Pts',(-2.81095058234328,15.2,10.3499893506076));
#231519=CARTESIAN_POINT('Ctrl Pts',(-2.81092515873169,15.2,10.3541190115118));
#231520=CARTESIAN_POINT('Ctrl Pts',(-2.81089973512011,15.2,10.3582486724161));
#231521=CARTESIAN_POINT('Ctrl Pts',(-2.81086525538654,15.2,10.36240408635));
#231522=CARTESIAN_POINT('Ctrl Pts',(-2.81082152399716,15.2,10.3665850012818));
#231523=CARTESIAN_POINT('Ctrl Pts',(-2.81078653888852,15.2,10.3699297329539));
#231524=CARTESIAN_POINT('Ctrl Pts',(-2.8107456327715,15.2,10.3732907846882));
#231525=CARTESIAN_POINT('Ctrl Pts',(-2.81069870977352,15.2,10.3766680299683));
#231526=CARTESIAN_POINT('Ctrl Pts',(-2.81065178676915,15.2,10.3800452757085));
#231527=CARTESIAN_POINT('Ctrl Pts',(-2.81059884604604,15.2,10.3834387144058));
#231528=CARTESIAN_POINT('Ctrl Pts',(-2.81053979298686,15.2,10.3868482205371));
#231529=CARTESIAN_POINT('Ctrl Pts',(-2.81048073993573,15.2,10.3902577262039));
#231530=CARTESIAN_POINT('Ctrl Pts',(-2.81041557268305,15.2,10.3936832977703));
#231531=CARTESIAN_POINT('Ctrl Pts',(-2.81034420024508,15.2,10.3971248101539));
#231532=CARTESIAN_POINT('Ctrl Pts',(-2.81025498469032,15.2,10.4014267009851));
#231533=CARTESIAN_POINT('Ctrl Pts',(-2.81015607047853,15.2,10.4057534998181));
#231534=CARTESIAN_POINT('Ctrl Pts',(-2.81004727602934,15.2,10.4101049642699));
#231535=CARTESIAN_POINT('Ctrl Pts',(-2.80996024046524,15.2,10.413586136021));
#231536=CARTESIAN_POINT('Ctrl Pts',(-2.80986688240328,15.2,10.417083094467));
#231537=CARTESIAN_POINT('Ctrl Pts',(-2.8097671101752,15.2,10.4205957147706));
#231538=CARTESIAN_POINT('Ctrl Pts',(-2.8096423948969,15.2,10.4249864899107));
#231539=CARTESIAN_POINT('Ctrl Pts',(-2.80950765977441,15.2,10.4294017383725));
#231540=CARTESIAN_POINT('Ctrl Pts',(-2.80936272623221,15.2,10.4338412210821));
#231541=CARTESIAN_POINT('Ctrl Pts',(-2.80924677940793,15.2,10.4373928069594));
#231542=CARTESIAN_POINT('Ctrl Pts',(-2.80912430728355,15.2,10.4409599042343));
#231543=CARTESIAN_POINT('Ctrl Pts',(-2.80899522101044,15.2,10.4445423902302));
#231544=CARTESIAN_POINT('Ctrl Pts',(-2.80883386315588,15.2,10.4490204980911));
#231545=CARTESIAN_POINT('Ctrl Pts',(-2.80866217064472,15.2,10.4535226533442));
#231546=CARTESIAN_POINT('Ctrl Pts',(-2.80847997377027,15.2,10.4580486194541));
#231547=CARTESIAN_POINT('Ctrl Pts',(-2.80833421626276,15.2,10.4616693925393));
#231548=CARTESIAN_POINT('Ctrl Pts',(-2.80818173696834,15.2,10.4653054066736));
#231549=CARTESIAN_POINT('Ctrl Pts',(-2.808022448737,15.2,10.4689565410402));
#231550=CARTESIAN_POINT('Ctrl Pts',(-2.80786316052735,15.2,10.4726076749094));
#231551=CARTESIAN_POINT('Ctrl Pts',(-2.80769706494405,15.2,10.476273931598));
#231552=CARTESIAN_POINT('Ctrl Pts',(-2.80752407678348,15.2,10.4799551904242));
#231553=CARTESIAN_POINT('Ctrl Pts',(-2.8073078415651,15.2,10.484556764333));
#231554=CARTESIAN_POINT('Ctrl Pts',(-2.80708083707612,15.2,10.489181783764));
#231555=CARTESIAN_POINT('Ctrl Pts',(-2.80684290179891,15.2,10.4938300164711));
#231556=CARTESIAN_POINT('Ctrl Pts',(-2.8065573794507,15.2,10.4994078960236));
#231557=CARTESIAN_POINT('Ctrl Pts',(-2.80625611574221,15.2,10.505019206722));
#231558=CARTESIAN_POINT('Ctrl Pts',(-2.80593883647383,15.2,10.5106635563652));
#231559=CARTESIAN_POINT('Ctrl Pts',(-2.80567443712674,15.2,10.5153671802988));
#231560=CARTESIAN_POINT('Ctrl Pts',(-2.80539891531652,15.2,10.520093750965));
#231561=CARTESIAN_POINT('Ctrl Pts',(-2.8051121167376,15.2,10.5248430408621));
#231562=CARTESIAN_POINT('Ctrl Pts',(-2.80482531812741,15.2,10.5295923312768));
#231563=CARTESIAN_POINT('Ctrl Pts',(-2.80452724109519,15.2,10.5343643448414));
#231564=CARTESIAN_POINT('Ctrl Pts',(-2.80421773429056,15.2,10.5391588583812));
#231565=CARTESIAN_POINT('Ctrl Pts',(-2.80390822748595,15.2,10.543953371921));
#231566=CARTESIAN_POINT('Ctrl Pts',(-2.80358729037667,15.2,10.5487703863925));
#231567=CARTESIAN_POINT('Ctrl Pts',(-2.80325477105531,15.2,10.5536096819799));
#231568=CARTESIAN_POINT('Ctrl Pts',(-2.80298875558372,15.2,10.5574811186608));
#231569=CARTESIAN_POINT('Ctrl Pts',(-2.80271532805118,15.2,10.561366815711));
#231570=CARTESIAN_POINT('Ctrl Pts',(-2.80243441320205,15.2,10.5652666620355));
#231571=CARTESIAN_POINT('Ctrl Pts',(-2.80215349839119,15.2,10.5691665078288));
#231572=CARTESIAN_POINT('Ctrl Pts',(-2.80186509529851,15.2,10.5730805021414));
#231573=CARTESIAN_POINT('Ctrl Pts',(-2.80156912982347,15.2,10.5770085353744));
#231574=CARTESIAN_POINT('Ctrl Pts',(-2.80127316430811,15.2,10.5809365691426));
#231575=CARTESIAN_POINT('Ctrl Pts',(-2.80096963519882,15.2,10.5848786418107));
#231576=CARTESIAN_POINT('Ctrl Pts',(-2.80065847045821,15.2,10.5888346435443));
#231577=CARTESIAN_POINT('Ctrl Pts',(-2.80034730575999,15.2,10.5927906447388));
#231578=CARTESIAN_POINT('Ctrl Pts',(-2.80002850500653,15.2,10.5967605751396));
#231579=CARTESIAN_POINT('Ctrl Pts',(-2.7997019943118,15.2,10.6007443250903));
#231580=CARTESIAN_POINT('Ctrl Pts',(-2.79937548357257,15.2,10.6047280755837));
#231581=CARTESIAN_POINT('Ctrl Pts',(-2.7990412633604,15.2,10.6087256464091));
#231582=CARTESIAN_POINT('Ctrl Pts',(-2.79869926250842,15.2,10.6127369295166));
#231583=CARTESIAN_POINT('Ctrl Pts',(-2.79818626127706,15.2,10.6187538536314));
#231584=CARTESIAN_POINT('Ctrl Pts',(-2.79765575127205,15.2,10.6248016305437));
#231585=CARTESIAN_POINT('Ctrl Pts',(-2.79710749612651,15.2,10.6308798968207));
#231586=CARTESIAN_POINT('Ctrl Pts',(-2.79665061682196,15.2,10.6359451189023));
#231587=CARTESIAN_POINT('Ctrl Pts',(-2.79618141222916,15.2,10.6410315145312));
#231588=CARTESIAN_POINT('Ctrl Pts',(-2.79569975033096,15.2,10.6461388776321));
#231589=CARTESIAN_POINT('Ctrl Pts',(-2.7953144207914,15.2,10.6502247683355));
#231590=CARTESIAN_POINT('Ctrl Pts',(-2.79492111698961,15.2,10.6543240784612));
#231591=CARTESIAN_POINT('Ctrl Pts',(-2.7945197709672,15.2,10.6584367003529));
#231592=CARTESIAN_POINT('Ctrl Pts',(-2.79391775198827,15.2,10.6646056326302));
#231593=CARTESIAN_POINT('Ctrl Pts',(-2.79329763852748,15.2,10.6708045226549));
#231594=CARTESIAN_POINT('Ctrl Pts',(-2.79265920355147,15.2,10.6770330119273));
#231595=CARTESIAN_POINT('Ctrl Pts',(-2.79212717438547,15.2,10.6822234198429));
#231596=CARTESIAN_POINT('Ctrl Pts',(-2.79158242218066,15.2,10.6874343871012));
#231597=CARTESIAN_POINT('Ctrl Pts',(-2.79102481877539,15.2,10.6926657074721));
#231598=CARTESIAN_POINT('Ctrl Pts',(-2.79057873602686,15.2,10.6968507639969));
#231599=CARTESIAN_POINT('Ctrl Pts',(-2.79012442798107,15.2,10.7010488486882));
#231600=CARTESIAN_POINT('Ctrl Pts',(-2.78966182989945,15.2,10.7052598571968));
#231601=CARTESIAN_POINT('Ctrl Pts',(-2.78896793284005,15.2,10.7115763693859));
#231602=CARTESIAN_POINT('Ctrl Pts',(-2.78825538343487,15.2,10.7179219609055));
#231603=CARTESIAN_POINT('Ctrl Pts',(-2.78752396454142,15.2,10.7242962890362));
#231604=CARTESIAN_POINT('Ctrl Pts',(-2.78703635196794,15.2,10.7285458409303));
#231605=CARTESIAN_POINT('Ctrl Pts',(-2.7865403551988,15.2,10.7328081643545));
#231606=CARTESIAN_POINT('Ctrl Pts',(-2.78603590807423,15.2,10.7370831570593));
#231607=CARTESIAN_POINT('Ctrl Pts',(-2.78553146088093,15.2,10.7413581503466));
#231608=CARTESIAN_POINT('Ctrl Pts',(-2.78501856659518,15.2,10.7456458155822));
#231609=CARTESIAN_POINT('Ctrl Pts',(-2.78449716123343,15.2,10.7499460494833));
#231610=CARTESIAN_POINT('Ctrl Pts',(-2.78397575587167,15.2,10.7542462833843));
#231611=CARTESIAN_POINT('Ctrl Pts',(-2.78344583971171,15.2,10.7585590878035));
#231612=CARTESIAN_POINT('Ctrl Pts',(-2.78290735240371,15.2,10.7628843617071));
#231613=CARTESIAN_POINT('Ctrl Pts',(-2.78223424337876,15.2,10.7682909532027));
#231614=CARTESIAN_POINT('Ctrl Pts',(-2.78154773961424,15.2,10.7737170298384));
#231615=CARTESIAN_POINT('Ctrl Pts',(-2.78084772635831,15.2,10.7791623955627));
#231616=CARTESIAN_POINT('Ctrl Pts',(-2.78014771302609,15.2,10.7846077618805));
#231617=CARTESIAN_POINT('Ctrl Pts',(-2.77943418926074,15.2,10.7900724199398));
#231618=CARTESIAN_POINT('Ctrl Pts',(-2.77870703780353,15.2,10.7955561760493));
#231619=CARTESIAN_POINT('Ctrl Pts',(-2.77812531660606,15.2,10.799943181176));
#231620=CARTESIAN_POINT('Ctrl Pts',(-2.77753487641009,15.2,10.8043424089258));
#231621=CARTESIAN_POINT('Ctrl Pts',(-2.77693565520801,15.2,10.8087537615196));
#231622=CARTESIAN_POINT('Ctrl Pts',(-2.77618662874624,15.2,10.8142679519614));
#231623=CARTESIAN_POINT('Ctrl Pts',(-2.77542388508326,15.2,10.8198010883122));
#231624=CARTESIAN_POINT('Ctrl Pts',(-2.77464731174922,15.2,10.8253529803965));
#231625=CARTESIAN_POINT('Ctrl Pts',(-2.77402605313277,15.2,10.8297944937008));
#231626=CARTESIAN_POINT('Ctrl Pts',(-2.77339594292364,15.2,10.8342480107222));
#231627=CARTESIAN_POINT('Ctrl Pts',(-2.7727569250879,15.2,10.8387134347448));
#231628=CARTESIAN_POINT('Ctrl Pts',(-2.77227766160226,15.2,10.8420625035223));
#231629=CARTESIAN_POINT('Ctrl Pts',(-2.77179338738188,15.2,10.8454182705767));
#231630=CARTESIAN_POINT('Ctrl Pts',(-2.77130407889342,15.2,10.8487806952329));
#231631=CARTESIAN_POINT('Ctrl Pts',(-2.77081477049385,15.2,10.8521431192783));
#231632=CARTESIAN_POINT('Ctrl Pts',(-2.77032042864414,15.2,10.8555121994231));
#231633=CARTESIAN_POINT('Ctrl Pts',(-2.76982102867842,15.2,10.8588878976365));
#231634=CARTESIAN_POINT('Ctrl Pts',(-2.7693216287127,15.2,10.8622635958499));
#231635=CARTESIAN_POINT('Ctrl Pts',(-2.76881717020973,15.2,10.8656459103087));
#231636=CARTESIAN_POINT('Ctrl Pts',(-2.76830763218613,15.2,10.8690348023944));
#231637=CARTESIAN_POINT('Ctrl Pts',(-2.76762824818553,15.2,10.8735533249703));
#231638=CARTESIAN_POINT('Ctrl Pts',(-2.76693983013118,15.2,10.878083540266));
#231639=CARTESIAN_POINT('Ctrl Pts',(-2.7662423263558,15.2,10.8826253522824));
#231640=CARTESIAN_POINT('Ctrl Pts',(-2.7653704465653,15.2,10.8883026177669));
#231641=CARTESIAN_POINT('Ctrl Pts',(-2.76448436840411,15.2,10.8939980046414));
#231642=CARTESIAN_POINT('Ctrl Pts',(-2.76358398842956,15.2,10.8997113295784));
#231643=CARTESIAN_POINT('Ctrl Pts',(-2.76304376046446,15.2,10.9031393244161));
#231644=CARTESIAN_POINT('Ctrl Pts',(-2.76249838293274,15.2,10.906573776609));
#231645=CARTESIAN_POINT('Ctrl Pts',(-2.76194783457844,15.2,10.9100146467748));
#231646=CARTESIAN_POINT('Ctrl Pts',(-2.76139728612413,15.2,10.9134555175657));
#231647=CARTESIAN_POINT('Ctrl Pts',(-2.76084156691003,15.2,10.9169028066167));
#231648=CARTESIAN_POINT('Ctrl Pts',(-2.76028065436947,15.2,10.9203564739945));
#231649=CARTESIAN_POINT('Ctrl Pts',(-2.75953277115189,15.2,10.9249613627859));
#231650=CARTESIAN_POINT('Ctrl Pts',(-2.7587756547855,15.2,10.9295775919452));
#231651=CARTESIAN_POINT('Ctrl Pts',(-2.75800925557099,15.2,10.9342050691217));
#231652=CARTESIAN_POINT('Ctrl Pts',(-2.75705125647454,15.2,10.9399894160652));
#231653=CARTESIAN_POINT('Ctrl Pts',(-2.75607874934396,15.2,10.9457913356315));
#231654=CARTESIAN_POINT('Ctrl Pts',(-2.7550916377423,15.2,10.9516106501718));
#231655=CARTESIAN_POINT('Ctrl Pts',(-2.75430194841792,15.2,10.9562661020577));
#231656=CARTESIAN_POINT('Ctrl Pts',(-2.75350291196016,15.2,10.9609326860642));
#231657=CARTESIAN_POINT('Ctrl Pts',(-2.75269447685957,15.2,10.9656103107648));
#231658=CARTESIAN_POINT('Ctrl Pts',(-2.75208815058921,15.2,10.9691185289715));
#231659=CARTESIAN_POINT('Ctrl Pts',(-2.75147653929414,15.2,10.9726329571445));
#231660=CARTESIAN_POINT('Ctrl Pts',(-2.75085961998276,15.2,10.9761535573505));
#231661=CARTESIAN_POINT('Ctrl Pts',(-2.75003706093827,15.2,10.9808476907452));
#231662=CARTESIAN_POINT('Ctrl Pts',(-2.74920506689291,15.2,10.9855527972988));
#231663=CARTESIAN_POINT('Ctrl Pts',(-2.74836358912933,15.2,10.9902687852456));
#231664=CARTESIAN_POINT('Ctrl Pts',(-2.74752211125111,15.2,10.9949847738348));
#231665=CARTESIAN_POINT('Ctrl Pts',(-2.74667114958644,15.2,10.9997116435735));
#231666=CARTESIAN_POINT('Ctrl Pts',(-2.74581065625784,15.2,11.0044493055198));
#231667=CARTESIAN_POINT('Ctrl Pts',(-2.74516528632001,15.2,11.0080025516568));
#231668=CARTESIAN_POINT('Ctrl Pts',(-2.74451455336314,15.2,11.0115618678267));
#231669=CARTESIAN_POINT('Ctrl Pts',(-2.74385843900902,15.2,11.0151272160467));
#231670=CARTESIAN_POINT('Ctrl Pts',(-2.74320232465491,15.2,11.0186925642667));
#231671=CARTESIAN_POINT('Ctrl Pts',(-2.74254082889799,15.2,11.0222639453739));
#231672=CARTESIAN_POINT('Ctrl Pts',(-2.74187393058936,15.2,11.0258413206185));
#231673=CARTESIAN_POINT('Ctrl Pts',(-2.74120703228073,15.2,11.029418695863));
#231674=CARTESIAN_POINT('Ctrl Pts',(-2.74053473170581,15.2,11.033002066032));
#231675=CARTESIAN_POINT('Ctrl Pts',(-2.73985700985617,15.2,11.0365913931925));
#231676=CARTESIAN_POINT('Ctrl Pts',(-2.73917928788341,15.2,11.040180721005));
#231677=CARTESIAN_POINT('Ctrl Pts',(-2.73849614410079,15.2,11.0437760055275));
#231678=CARTESIAN_POINT('Ctrl Pts',(-2.73780755908331,15.2,11.0473772103017));
#231679=CARTESIAN_POINT('Ctrl Pts',(-2.73665991767939,15.2,11.0533792167321));
#231680=CARTESIAN_POINT('Ctrl Pts',(-2.73549716116342,15.2,11.0593976664086));
#231681=CARTESIAN_POINT('Ctrl Pts',(-2.73431919990417,15.2,11.0654323862356));
#231682=CARTESIAN_POINT('Ctrl Pts',(-2.73314123851652,15.2,11.0714671067204));
#231683=CARTESIAN_POINT('Ctrl Pts',(-2.73194807286801,15.2,11.0775180970522));
#231684=CARTESIAN_POINT('Ctrl Pts',(-2.73073961488316,15.2,11.0835851884397));
#231685=CARTESIAN_POINT('Ctrl Pts',(-2.73001453998687,15.2,11.0872254438013));
#231686=CARTESIAN_POINT('Ctrl Pts',(-2.72928396131402,15.2,11.0908714962312));
#231687=CARTESIAN_POINT('Ctrl Pts',(-2.72854785787295,15.2,11.0945233075544));
#231688=CARTESIAN_POINT('Ctrl Pts',(-2.72732101911654,15.2,11.1006096582117));
#231689=CARTESIAN_POINT('Ctrl Pts',(-2.72607883461512,15.2,11.1067120056901));
#231690=CARTESIAN_POINT('Ctrl Pts',(-2.72482121919792,15.2,11.1128301757163));
#231691=CARTESIAN_POINT('Ctrl Pts',(-2.72406664975569,15.2,11.1165010786657));
#231692=CARTESIAN_POINT('Ctrl Pts',(-2.72330652591187,15.2,11.1201776796168));
#231693=CARTESIAN_POINT('Ctrl Pts',(-2.7225408290915,15.2,11.1238599450277));
#231694=CARTESIAN_POINT('Ctrl Pts',(-2.72177513241023,15.2,11.1275422097697));
#231695=CARTESIAN_POINT('Ctrl Pts',(-2.72100386532091,15.2,11.1312301398864));
#231696=CARTESIAN_POINT('Ctrl Pts',(-2.72022700793199,15.2,11.1349236969193));
#231697=CARTESIAN_POINT('Ctrl Pts',(-2.71945015054306,15.2,11.1386172539523));
#231698=CARTESIAN_POINT('Ctrl Pts',(-2.71866770162434,15.2,11.1423164364044));
#231699=CARTESIAN_POINT('Ctrl Pts',(-2.71787964073271,15.2,11.146021201495));
#231700=CARTESIAN_POINT('Ctrl Pts',(-2.71709157984108,15.2,11.1497259665855));
#231701=CARTESIAN_POINT('Ctrl Pts',(-2.71629790459204,15.2,11.1534363121814));
#231702=CARTESIAN_POINT('Ctrl Pts',(-2.71549860045082,15.2,11.1571522052299));
#231703=CARTESIAN_POINT('Ctrl Pts',(-2.71416642683371,15.2,11.1633453605357));
#231704=CARTESIAN_POINT('Ctrl Pts',(-2.71281861996396,15.2,11.1695539166432));
#231705=CARTESIAN_POINT('Ctrl Pts',(-2.71145515300006,15.2,11.175777868));
#231706=CARTESIAN_POINT('Ctrl Pts',(-1.76496130700006,15.2,10.22377311));
#231707=CARTESIAN_POINT('Ctrl Pts',(-1.76496130700006,11.6,10.22377311));
#231708=CARTESIAN_POINT('Ctrl Pts',(-1.76500562500005,15.2,10.223941742));
#231709=CARTESIAN_POINT('Ctrl Pts',(-1.76500562500005,11.6,10.223941742));
#231710=CARTESIAN_POINT('Ctrl Pts',(-1.76509588900006,15.2,10.224284874));
#231711=CARTESIAN_POINT('Ctrl Pts',(-1.76509588900006,11.6,10.224284874));
#231712=CARTESIAN_POINT('Ctrl Pts',(-1.76523291900006,15.2,10.224804732));
#231713=CARTESIAN_POINT('Ctrl Pts',(-1.76523291900006,11.6,10.224804732));
#231714=CARTESIAN_POINT('Ctrl Pts',(-1.76541803300006,15.2,10.22550489));
#231715=CARTESIAN_POINT('Ctrl Pts',(-1.76541803300006,11.6,10.22550489));
#231716=CARTESIAN_POINT('Ctrl Pts',(-1.76565305800006,15.2,10.226390254));
#231717=CARTESIAN_POINT('Ctrl Pts',(-1.76565305800006,11.6,10.226390254));
#231718=CARTESIAN_POINT('Ctrl Pts',(-1.76589279600006,15.2,10.227289726));
#231719=CARTESIAN_POINT('Ctrl Pts',(-1.76589279600006,11.6,10.227289726));
#231720=CARTESIAN_POINT('Ctrl Pts',(-1.76613589400006,15.2,10.22819815));
#231721=CARTESIAN_POINT('Ctrl Pts',(-1.76613589400006,11.6,10.22819815));
#231722=CARTESIAN_POINT('Ctrl Pts',(-1.76638236600006,15.2,10.229115492));
#231723=CARTESIAN_POINT('Ctrl Pts',(-1.76638236600006,11.6,10.229115492));
#231724=CARTESIAN_POINT('Ctrl Pts',(-1.76663222000006,15.2,10.230041723));
#231725=CARTESIAN_POINT('Ctrl Pts',(-1.76663222000006,11.6,10.230041723));
#231726=CARTESIAN_POINT('Ctrl Pts',(-1.76688546700006,15.2,10.230976812));
#231727=CARTESIAN_POINT('Ctrl Pts',(-1.76688546700006,11.6,10.230976812));
#231728=CARTESIAN_POINT('Ctrl Pts',(-1.76714211800005,15.2,10.231920729));
#231729=CARTESIAN_POINT('Ctrl Pts',(-1.76714211800005,11.6,10.231920729));
#231730=CARTESIAN_POINT('Ctrl Pts',(-1.76740218300006,15.2,10.232873444));
#231731=CARTESIAN_POINT('Ctrl Pts',(-1.76740218300006,11.6,10.232873444));
#231732=CARTESIAN_POINT('Ctrl Pts',(-1.76766567100006,15.2,10.233834926));
#231733=CARTESIAN_POINT('Ctrl Pts',(-1.76766567100006,11.6,10.233834926));
#231734=CARTESIAN_POINT('Ctrl Pts',(-1.76793259300006,15.2,10.234805146));
#231735=CARTESIAN_POINT('Ctrl Pts',(-1.76793259300006,11.6,10.234805146));
#231736=CARTESIAN_POINT('Ctrl Pts',(-1.76820296100006,15.2,10.235784074));
#231737=CARTESIAN_POINT('Ctrl Pts',(-1.76820296100006,11.6,10.235784074));
#231738=CARTESIAN_POINT('Ctrl Pts',(-1.76847678200006,15.2,10.23677168));
#231739=CARTESIAN_POINT('Ctrl Pts',(-1.76847678200006,11.6,10.23677168));
#231740=CARTESIAN_POINT('Ctrl Pts',(-1.76875406800006,15.2,10.237767935));
#231741=CARTESIAN_POINT('Ctrl Pts',(-1.76875406800006,11.6,10.237767935));
#231742=CARTESIAN_POINT('Ctrl Pts',(-1.76903482800005,15.2,10.23877281));
#231743=CARTESIAN_POINT('Ctrl Pts',(-1.76903482800005,11.6,10.23877281));
#231744=CARTESIAN_POINT('Ctrl Pts',(-1.76931907200006,15.2,10.239786274));
#231745=CARTESIAN_POINT('Ctrl Pts',(-1.76931907200006,11.6,10.239786274));
#231746=CARTESIAN_POINT('Ctrl Pts',(-1.76960681100006,15.2,10.2408083));
#231747=CARTESIAN_POINT('Ctrl Pts',(-1.76960681100006,11.6,10.2408083));
#231748=CARTESIAN_POINT('Ctrl Pts',(-1.76989805200006,15.2,10.241838858));
#231749=CARTESIAN_POINT('Ctrl Pts',(-1.76989805200006,11.6,10.241838858));
#231750=CARTESIAN_POINT('Ctrl Pts',(-1.77019280700006,15.2,10.24287792));
#231751=CARTESIAN_POINT('Ctrl Pts',(-1.77019280700006,11.6,10.24287792));
#231752=CARTESIAN_POINT('Ctrl Pts',(-1.77049108600006,15.2,10.243925457));
#231753=CARTESIAN_POINT('Ctrl Pts',(-1.77049108600006,11.6,10.243925457));
#231754=CARTESIAN_POINT('Ctrl Pts',(-1.77079289700006,15.2,10.244981439));
#231755=CARTESIAN_POINT('Ctrl Pts',(-1.77079289700006,11.6,10.244981439));
#231756=CARTESIAN_POINT('Ctrl Pts',(-1.77109824900006,15.2,10.246045839));
#231757=CARTESIAN_POINT('Ctrl Pts',(-1.77109824900006,11.6,10.246045839));
#231758=CARTESIAN_POINT('Ctrl Pts',(-1.77140715400005,15.2,10.24711863));
#231759=CARTESIAN_POINT('Ctrl Pts',(-1.77140715400005,11.6,10.24711863));
#231760=CARTESIAN_POINT('Ctrl Pts',(-1.77171961900006,15.2,10.248199782));
#231761=CARTESIAN_POINT('Ctrl Pts',(-1.77171961900006,11.6,10.248199782));
#231762=CARTESIAN_POINT('Ctrl Pts',(-1.77203565500006,15.2,10.249289266));
#231763=CARTESIAN_POINT('Ctrl Pts',(-1.77203565500006,11.6,10.249289266));
#231764=CARTESIAN_POINT('Ctrl Pts',(-1.77235527000006,15.2,10.250387056));
#231765=CARTESIAN_POINT('Ctrl Pts',(-1.77235527000006,11.6,10.250387056));
#231766=CARTESIAN_POINT('Ctrl Pts',(-1.77267847400006,15.2,10.251493125));
#231767=CARTESIAN_POINT('Ctrl Pts',(-1.77267847400006,11.6,10.251493125));
#231768=CARTESIAN_POINT('Ctrl Pts',(-1.77300527500006,15.2,10.252607443));
#231769=CARTESIAN_POINT('Ctrl Pts',(-1.77300527500006,11.6,10.252607443));
#231770=CARTESIAN_POINT('Ctrl Pts',(-1.77333568300006,15.2,10.253729984));
#231771=CARTESIAN_POINT('Ctrl Pts',(-1.77333568300006,11.6,10.253729984));
#231772=CARTESIAN_POINT('Ctrl Pts',(-1.77366970800006,15.2,10.254860721));
#231773=CARTESIAN_POINT('Ctrl Pts',(-1.77366970800006,11.6,10.254860721));
#231774=CARTESIAN_POINT('Ctrl Pts',(-1.77400735800005,15.2,10.255999624));
#231775=CARTESIAN_POINT('Ctrl Pts',(-1.77400735800005,11.6,10.255999624));
#231776=CARTESIAN_POINT('Ctrl Pts',(-1.77434864200006,15.2,10.257146669));
#231777=CARTESIAN_POINT('Ctrl Pts',(-1.77434864200006,11.6,10.257146669));
#231778=CARTESIAN_POINT('Ctrl Pts',(-1.77469356900006,15.2,10.258301828));
#231779=CARTESIAN_POINT('Ctrl Pts',(-1.77469356900006,11.6,10.258301828));
#231780=CARTESIAN_POINT('Ctrl Pts',(-1.77504214700006,15.2,10.259465072));
#231781=CARTESIAN_POINT('Ctrl Pts',(-1.77504214700006,11.6,10.259465072));
#231782=CARTESIAN_POINT('Ctrl Pts',(-1.77539438600005,15.2,10.260636378));
#231783=CARTESIAN_POINT('Ctrl Pts',(-1.77539438600005,11.6,10.260636378));
#231784=CARTESIAN_POINT('Ctrl Pts',(-1.77575029400006,15.2,10.261815716));
#231785=CARTESIAN_POINT('Ctrl Pts',(-1.77575029400006,11.6,10.261815716));
#231786=CARTESIAN_POINT('Ctrl Pts',(-1.77610988000006,15.2,10.263003062));
#231787=CARTESIAN_POINT('Ctrl Pts',(-1.77610988000006,11.6,10.263003062));
#231788=CARTESIAN_POINT('Ctrl Pts',(-1.77647315400006,15.2,10.264198387));
#231789=CARTESIAN_POINT('Ctrl Pts',(-1.77647315400006,11.6,10.264198387));
#231790=CARTESIAN_POINT('Ctrl Pts',(-1.77684012100006,15.2,10.265401667));
#231791=CARTESIAN_POINT('Ctrl Pts',(-1.77684012100006,11.6,10.265401667));
#231792=CARTESIAN_POINT('Ctrl Pts',(-1.77721079300006,15.2,10.266612873));
#231793=CARTESIAN_POINT('Ctrl Pts',(-1.77721079300006,11.6,10.266612873));
#231794=CARTESIAN_POINT('Ctrl Pts',(-1.77758517500005,15.2,10.267831982));
#231795=CARTESIAN_POINT('Ctrl Pts',(-1.77758517500005,11.6,10.267831982));
#231796=CARTESIAN_POINT('Ctrl Pts',(-1.77796328000006,15.2,10.269058967));
#231797=CARTESIAN_POINT('Ctrl Pts',(-1.77796328000006,11.6,10.269058967));
#231798=CARTESIAN_POINT('Ctrl Pts',(-1.77834511300006,15.2,10.2702938));
#231799=CARTESIAN_POINT('Ctrl Pts',(-1.77834511300006,11.6,10.2702938));
#231800=CARTESIAN_POINT('Ctrl Pts',(-1.77873068400005,15.2,10.271536458));
#231801=CARTESIAN_POINT('Ctrl Pts',(-1.77873068400005,11.6,10.271536458));
#231802=CARTESIAN_POINT('Ctrl Pts',(-1.77911999900006,15.2,10.272786914));
#231803=CARTESIAN_POINT('Ctrl Pts',(-1.77911999900006,11.6,10.272786914));
#231804=CARTESIAN_POINT('Ctrl Pts',(-1.77951306900006,15.2,10.274045143));
#231805=CARTESIAN_POINT('Ctrl Pts',(-1.77951306900006,11.6,10.274045143));
#231806=CARTESIAN_POINT('Ctrl Pts',(-1.77990990000006,15.2,10.275311119));
#231807=CARTESIAN_POINT('Ctrl Pts',(-1.77990990000006,11.6,10.275311119));
#231808=CARTESIAN_POINT('Ctrl Pts',(-1.78031050100006,15.2,10.276584816));
#231809=CARTESIAN_POINT('Ctrl Pts',(-1.78031050100006,11.6,10.276584816));
#231810=CARTESIAN_POINT('Ctrl Pts',(-1.78071488100006,15.2,10.277866211));
#231811=CARTESIAN_POINT('Ctrl Pts',(-1.78071488100006,11.6,10.277866211));
#231812=CARTESIAN_POINT('Ctrl Pts',(-1.78112304700006,15.2,10.279155276));
#231813=CARTESIAN_POINT('Ctrl Pts',(-1.78112304700006,11.6,10.279155276));
#231814=CARTESIAN_POINT('Ctrl Pts',(-1.78153500600006,15.2,10.280451988));
#231815=CARTESIAN_POINT('Ctrl Pts',(-1.78153500600006,11.6,10.280451988));
#231816=CARTESIAN_POINT('Ctrl Pts',(-1.78195076800006,15.2,10.281756322));
#231817=CARTESIAN_POINT('Ctrl Pts',(-1.78195076800006,11.6,10.281756322));
#231818=CARTESIAN_POINT('Ctrl Pts',(-1.78237034000006,15.2,10.283068252));
#231819=CARTESIAN_POINT('Ctrl Pts',(-1.78237034000006,11.6,10.283068252));
#231820=CARTESIAN_POINT('Ctrl Pts',(-1.78279372900006,15.2,10.284387754));
#231821=CARTESIAN_POINT('Ctrl Pts',(-1.78279372900006,11.6,10.284387754));
#231822=CARTESIAN_POINT('Ctrl Pts',(-1.78322094500006,15.2,10.285714803));
#231823=CARTESIAN_POINT('Ctrl Pts',(-1.78322094500006,11.6,10.285714803));
#231824=CARTESIAN_POINT('Ctrl Pts',(-1.78365199300006,15.2,10.287049375));
#231825=CARTESIAN_POINT('Ctrl Pts',(-1.78365199300006,11.6,10.287049375));
#231826=CARTESIAN_POINT('Ctrl Pts',(-1.78408688300005,15.2,10.288391445));
#231827=CARTESIAN_POINT('Ctrl Pts',(-1.78408688300005,11.6,10.288391445));
#231828=CARTESIAN_POINT('Ctrl Pts',(-1.78452562100006,15.2,10.28974099));
#231829=CARTESIAN_POINT('Ctrl Pts',(-1.78452562100006,11.6,10.28974099));
#231830=CARTESIAN_POINT('Ctrl Pts',(-1.78496821700006,15.2,10.291097984));
#231831=CARTESIAN_POINT('Ctrl Pts',(-1.78496821700006,11.6,10.291097984));
#231832=CARTESIAN_POINT('Ctrl Pts',(-1.78541467400006,15.2,10.292462403));
#231833=CARTESIAN_POINT('Ctrl Pts',(-1.78541467400006,11.6,10.292462403));
#231834=CARTESIAN_POINT('Ctrl Pts',(-1.78586500500006,15.2,10.293834224));
#231835=CARTESIAN_POINT('Ctrl Pts',(-1.78586500500006,11.6,10.293834224));
#231836=CARTESIAN_POINT('Ctrl Pts',(-1.78631921400006,15.2,10.295213423));
#231837=CARTESIAN_POINT('Ctrl Pts',(-1.78631921400006,11.6,10.295213423));
#231838=CARTESIAN_POINT('Ctrl Pts',(-1.78677730900006,15.2,10.296599975));
#231839=CARTESIAN_POINT('Ctrl Pts',(-1.78677730900006,11.6,10.296599975));
#231840=CARTESIAN_POINT('Ctrl Pts',(-1.78723929800006,15.2,10.297993857));
#231841=CARTESIAN_POINT('Ctrl Pts',(-1.78723929800006,11.6,10.297993857));
#231842=CARTESIAN_POINT('Ctrl Pts',(-1.78770518700006,15.2,10.299395046));
#231843=CARTESIAN_POINT('Ctrl Pts',(-1.78770518700006,11.6,10.299395046));
#231844=CARTESIAN_POINT('Ctrl Pts',(-1.78817498600006,15.2,10.300803517));
#231845=CARTESIAN_POINT('Ctrl Pts',(-1.78817498600006,11.6,10.300803517));
#231846=CARTESIAN_POINT('Ctrl Pts',(-1.78864870100006,15.2,10.302219248));
#231847=CARTESIAN_POINT('Ctrl Pts',(-1.78864870100006,11.6,10.302219248));
#231848=CARTESIAN_POINT('Ctrl Pts',(-1.78912633700006,15.2,10.303642214));
#231849=CARTESIAN_POINT('Ctrl Pts',(-1.78912633700006,11.6,10.303642214));
#231850=CARTESIAN_POINT('Ctrl Pts',(-1.78960790600006,15.2,10.305072394));
#231851=CARTESIAN_POINT('Ctrl Pts',(-1.78960790600006,11.6,10.305072394));
#231852=CARTESIAN_POINT('Ctrl Pts',(-1.79009341000006,15.2,10.306509761));
#231853=CARTESIAN_POINT('Ctrl Pts',(-1.79009341000006,11.6,10.306509761));
#231854=CARTESIAN_POINT('Ctrl Pts',(-1.79058285800005,15.2,10.307954296));
#231855=CARTESIAN_POINT('Ctrl Pts',(-1.79058285800005,11.6,10.307954296));
#231856=CARTESIAN_POINT('Ctrl Pts',(-1.79107625800006,15.2,10.309405975));
#231857=CARTESIAN_POINT('Ctrl Pts',(-1.79107625800006,11.6,10.309405975));
#231858=CARTESIAN_POINT('Ctrl Pts',(-1.79157361700006,15.2,10.310864773));
#231859=CARTESIAN_POINT('Ctrl Pts',(-1.79157361700006,11.6,10.310864773));
#231860=CARTESIAN_POINT('Ctrl Pts',(-1.79207494100006,15.2,10.312330668));
#231861=CARTESIAN_POINT('Ctrl Pts',(-1.79207494100006,11.6,10.312330668));
#231862=CARTESIAN_POINT('Ctrl Pts',(-1.79258023800006,15.2,10.313803638));
#231863=CARTESIAN_POINT('Ctrl Pts',(-1.79258023800006,11.6,10.313803638));
#231864=CARTESIAN_POINT('Ctrl Pts',(-1.79308951300006,15.2,10.315283661));
#231865=CARTESIAN_POINT('Ctrl Pts',(-1.79308951300006,11.6,10.315283661));
#231866=CARTESIAN_POINT('Ctrl Pts',(-1.79360277400006,15.2,10.316770712));
#231867=CARTESIAN_POINT('Ctrl Pts',(-1.79360277400006,11.6,10.316770712));
#231868=CARTESIAN_POINT('Ctrl Pts',(-1.79412002900006,15.2,10.31826477));
#231869=CARTESIAN_POINT('Ctrl Pts',(-1.79412002900006,11.6,10.31826477));
#231870=CARTESIAN_POINT('Ctrl Pts',(-1.79464128300005,15.2,10.319765814));
#231871=CARTESIAN_POINT('Ctrl Pts',(-1.79464128300005,11.6,10.319765814));
#231872=CARTESIAN_POINT('Ctrl Pts',(-1.79516654300006,15.2,10.321273819));
#231873=CARTESIAN_POINT('Ctrl Pts',(-1.79516654300006,11.6,10.321273819));
#231874=CARTESIAN_POINT('Ctrl Pts',(-1.79569581700005,15.2,10.322788764));
#231875=CARTESIAN_POINT('Ctrl Pts',(-1.79569581700005,11.6,10.322788764));
#231876=CARTESIAN_POINT('Ctrl Pts',(-1.79622911000005,15.2,10.324310627));
#231877=CARTESIAN_POINT('Ctrl Pts',(-1.79622911000005,11.6,10.324310627));
#231878=CARTESIAN_POINT('Ctrl Pts',(-1.79676643100006,15.2,10.325839385));
#231879=CARTESIAN_POINT('Ctrl Pts',(-1.79676643100006,11.6,10.325839385));
#231880=CARTESIAN_POINT('Ctrl Pts',(-1.79730778400006,15.2,10.327375017));
#231881=CARTESIAN_POINT('Ctrl Pts',(-1.79730778400006,11.6,10.327375017));
#231882=CARTESIAN_POINT('Ctrl Pts',(-1.79785317600006,15.2,10.328917501));
#231883=CARTESIAN_POINT('Ctrl Pts',(-1.79785317600006,11.6,10.328917501));
#231884=CARTESIAN_POINT('Ctrl Pts',(-1.79840261400006,15.2,10.330466814));
#231885=CARTESIAN_POINT('Ctrl Pts',(-1.79840261400006,11.6,10.330466814));
#231886=CARTESIAN_POINT('Ctrl Pts',(-1.79895610500005,15.2,10.332022936));
#231887=CARTESIAN_POINT('Ctrl Pts',(-1.79895610500005,11.6,10.332022936));
#231888=CARTESIAN_POINT('Ctrl Pts',(-1.79951365500005,15.2,10.333585844));
#231889=CARTESIAN_POINT('Ctrl Pts',(-1.79951365500005,11.6,10.333585844));
#231890=CARTESIAN_POINT('Ctrl Pts',(-1.80007527000006,15.2,10.335155517));
#231891=CARTESIAN_POINT('Ctrl Pts',(-1.80007527000006,11.6,10.335155517));
#231892=CARTESIAN_POINT('Ctrl Pts',(-1.80064095700006,15.2,10.336731933));
#231893=CARTESIAN_POINT('Ctrl Pts',(-1.80064095700006,11.6,10.336731933));
#231894=CARTESIAN_POINT('Ctrl Pts',(-1.80121072300006,15.2,10.338315071));
#231895=CARTESIAN_POINT('Ctrl Pts',(-1.80121072300006,11.6,10.338315071));
#231896=CARTESIAN_POINT('Ctrl Pts',(-1.80178457200005,15.2,10.339904909));
#231897=CARTESIAN_POINT('Ctrl Pts',(-1.80178457200005,11.6,10.339904909));
#231898=CARTESIAN_POINT('Ctrl Pts',(-1.80236251100005,15.2,10.341501427));
#231899=CARTESIAN_POINT('Ctrl Pts',(-1.80236251100005,11.6,10.341501427));
#231900=CARTESIAN_POINT('Ctrl Pts',(-1.80294454800005,15.2,10.343104602));
#231901=CARTESIAN_POINT('Ctrl Pts',(-1.80294454800005,11.6,10.343104602));
#231902=CARTESIAN_POINT('Ctrl Pts',(-1.80353068700006,15.2,10.344714415));
#231903=CARTESIAN_POINT('Ctrl Pts',(-1.80353068700006,11.6,10.344714415));
#231904=CARTESIAN_POINT('Ctrl Pts',(-1.80412093600005,15.2,10.346330843));
#231905=CARTESIAN_POINT('Ctrl Pts',(-1.80412093600005,11.6,10.346330843));
#231906=CARTESIAN_POINT('Ctrl Pts',(-1.80471530000006,15.2,10.347953866));
#231907=CARTESIAN_POINT('Ctrl Pts',(-1.80471530000006,11.6,10.347953866));
#231908=CARTESIAN_POINT('Ctrl Pts',(-1.80531378500006,15.2,10.349583462));
#231909=CARTESIAN_POINT('Ctrl Pts',(-1.80531378500006,11.6,10.349583462));
#231910=CARTESIAN_POINT('Ctrl Pts',(-1.80591639800005,15.2,10.351219613));
#231911=CARTESIAN_POINT('Ctrl Pts',(-1.80591639800005,11.6,10.351219613));
#231912=CARTESIAN_POINT('Ctrl Pts',(-1.80652314300006,15.2,10.352862294));
#231913=CARTESIAN_POINT('Ctrl Pts',(-1.80652314300006,11.6,10.352862294));
#231914=CARTESIAN_POINT('Ctrl Pts',(-1.80713402800006,15.2,10.354511488));
#231915=CARTESIAN_POINT('Ctrl Pts',(-1.80713402800006,11.6,10.354511488));
#231916=CARTESIAN_POINT('Ctrl Pts',(-1.80774906000006,15.2,10.356167173));
#231917=CARTESIAN_POINT('Ctrl Pts',(-1.80774906000006,11.6,10.356167173));
#231918=CARTESIAN_POINT('Ctrl Pts',(-1.80836824100005,15.2,10.357829328));
#231919=CARTESIAN_POINT('Ctrl Pts',(-1.80836824100005,11.6,10.357829328));
#231920=CARTESIAN_POINT('Ctrl Pts',(-1.80899158000006,15.2,10.359497932));
#231921=CARTESIAN_POINT('Ctrl Pts',(-1.80899158000006,11.6,10.359497932));
#231922=CARTESIAN_POINT('Ctrl Pts',(-1.80961908100006,15.2,10.361172966));
#231923=CARTESIAN_POINT('Ctrl Pts',(-1.80961908100006,11.6,10.361172966));
#231924=CARTESIAN_POINT('Ctrl Pts',(-1.81025075100006,15.2,10.36285441));
#231925=CARTESIAN_POINT('Ctrl Pts',(-1.81025075100006,11.6,10.36285441));
#231926=CARTESIAN_POINT('Ctrl Pts',(-1.81088659600006,15.2,10.364542243));
#231927=CARTESIAN_POINT('Ctrl Pts',(-1.81088659600006,11.6,10.364542243));
#231928=CARTESIAN_POINT('Ctrl Pts',(-1.81152662100006,15.2,10.366236443));
#231929=CARTESIAN_POINT('Ctrl Pts',(-1.81152662100006,11.6,10.366236443));
#231930=CARTESIAN_POINT('Ctrl Pts',(-1.81217083200006,15.2,10.367936993));
#231931=CARTESIAN_POINT('Ctrl Pts',(-1.81217083200006,11.6,10.367936993));
#231932=CARTESIAN_POINT('Ctrl Pts',(-1.81281923400005,15.2,10.36964387));
#231933=CARTESIAN_POINT('Ctrl Pts',(-1.81281923400005,11.6,10.36964387));
#231934=CARTESIAN_POINT('Ctrl Pts',(-1.81347183300006,15.2,10.371357057));
#231935=CARTESIAN_POINT('Ctrl Pts',(-1.81347183300006,11.6,10.371357057));
#231936=CARTESIAN_POINT('Ctrl Pts',(-1.81412863500006,15.2,10.373076533));
#231937=CARTESIAN_POINT('Ctrl Pts',(-1.81412863500006,11.6,10.373076533));
#231938=CARTESIAN_POINT('Ctrl Pts',(-1.81478964600006,15.2,10.374802277));
#231939=CARTESIAN_POINT('Ctrl Pts',(-1.81478964600006,11.6,10.374802277));
#231940=CARTESIAN_POINT('Ctrl Pts',(-1.81545487000006,15.2,10.37653427));
#231941=CARTESIAN_POINT('Ctrl Pts',(-1.81545487000006,11.6,10.37653427));
#231942=CARTESIAN_POINT('Ctrl Pts',(-1.81612431400006,15.2,10.378272492));
#231943=CARTESIAN_POINT('Ctrl Pts',(-1.81612431400006,11.6,10.378272492));
#231944=CARTESIAN_POINT('Ctrl Pts',(-1.81679798300005,15.2,10.380016924));
#231945=CARTESIAN_POINT('Ctrl Pts',(-1.81679798300005,11.6,10.380016924));
#231946=CARTESIAN_POINT('Ctrl Pts',(-1.81747588200006,15.2,10.381767546));
#231947=CARTESIAN_POINT('Ctrl Pts',(-1.81747588200006,11.6,10.381767546));
#231948=CARTESIAN_POINT('Ctrl Pts',(-1.81815801700006,15.2,10.383524338));
#231949=CARTESIAN_POINT('Ctrl Pts',(-1.81815801700006,11.6,10.383524338));
#231950=CARTESIAN_POINT('Ctrl Pts',(-1.81884439400006,15.2,10.385287281));
#231951=CARTESIAN_POINT('Ctrl Pts',(-1.81884439400006,11.6,10.385287281));
#231952=CARTESIAN_POINT('Ctrl Pts',(-1.81953501600006,15.2,10.387056356));
#231953=CARTESIAN_POINT('Ctrl Pts',(-1.81953501600006,11.6,10.387056356));
#231954=CARTESIAN_POINT('Ctrl Pts',(-1.82022989100005,15.2,10.388831544));
#231955=CARTESIAN_POINT('Ctrl Pts',(-1.82022989100005,11.6,10.388831544));
#231956=CARTESIAN_POINT('Ctrl Pts',(-1.82092902200006,15.2,10.390612824));
#231957=CARTESIAN_POINT('Ctrl Pts',(-1.82092902200006,11.6,10.390612824));
#231958=CARTESIAN_POINT('Ctrl Pts',(-1.82163241600006,15.2,10.392400178));
#231959=CARTESIAN_POINT('Ctrl Pts',(-1.82163241600006,11.6,10.392400178));
#231960=CARTESIAN_POINT('Ctrl Pts',(-1.82234007900006,15.2,10.394193587));
#231961=CARTESIAN_POINT('Ctrl Pts',(-1.82234007900006,11.6,10.394193587));
#231962=CARTESIAN_POINT('Ctrl Pts',(-1.82305201300006,15.2,10.395993032));
#231963=CARTESIAN_POINT('Ctrl Pts',(-1.82305201300006,11.6,10.395993032));
#231964=CARTESIAN_POINT('Ctrl Pts',(-1.82376822600005,15.2,10.397798493));
#231965=CARTESIAN_POINT('Ctrl Pts',(-1.82376822600005,11.6,10.397798493));
#231966=CARTESIAN_POINT('Ctrl Pts',(-1.82448872100006,15.2,10.399609951));
#231967=CARTESIAN_POINT('Ctrl Pts',(-1.82448872100006,11.6,10.399609951));
#231968=CARTESIAN_POINT('Ctrl Pts',(-1.82521350600006,15.2,10.40142739));
#231969=CARTESIAN_POINT('Ctrl Pts',(-1.82521350600006,11.6,10.40142739));
#231970=CARTESIAN_POINT('Ctrl Pts',(-1.82594258300006,15.2,10.403250787));
#231971=CARTESIAN_POINT('Ctrl Pts',(-1.82594258300006,11.6,10.403250787));
#231972=CARTESIAN_POINT('Ctrl Pts',(-1.82667595900006,15.2,10.405080126));
#231973=CARTESIAN_POINT('Ctrl Pts',(-1.82667595900006,11.6,10.405080126));
#231974=CARTESIAN_POINT('Ctrl Pts',(-1.82741363900006,15.2,10.406915388));
#231975=CARTESIAN_POINT('Ctrl Pts',(-1.82741363900006,11.6,10.406915388));
#231976=CARTESIAN_POINT('Ctrl Pts',(-1.82815562700006,15.2,10.408756553));
#231977=CARTESIAN_POINT('Ctrl Pts',(-1.82815562700006,11.6,10.408756553));
#231978=CARTESIAN_POINT('Ctrl Pts',(-1.82890192700006,15.2,10.410603602));
#231979=CARTESIAN_POINT('Ctrl Pts',(-1.82890192700006,11.6,10.410603602));
#231980=CARTESIAN_POINT('Ctrl Pts',(-1.82965254700005,15.2,10.41245652));
#231981=CARTESIAN_POINT('Ctrl Pts',(-1.82965254700005,11.6,10.41245652));
#231982=CARTESIAN_POINT('Ctrl Pts',(-1.83040749000006,15.2,10.414315285));
#231983=CARTESIAN_POINT('Ctrl Pts',(-1.83040749000006,11.6,10.414315285));
#231984=CARTESIAN_POINT('Ctrl Pts',(-1.83116676100005,15.2,10.416179881));
#231985=CARTESIAN_POINT('Ctrl Pts',(-1.83116676100005,11.6,10.416179881));
#231986=CARTESIAN_POINT('Ctrl Pts',(-1.83193036600006,15.2,10.418050288));
#231987=CARTESIAN_POINT('Ctrl Pts',(-1.83193036600006,11.6,10.418050288));
#231988=CARTESIAN_POINT('Ctrl Pts',(-1.83269830800006,15.2,10.419926488));
#231989=CARTESIAN_POINT('Ctrl Pts',(-1.83269830800006,11.6,10.419926488));
#231990=CARTESIAN_POINT('Ctrl Pts',(-1.83347059200006,15.2,10.421808463));
#231991=CARTESIAN_POINT('Ctrl Pts',(-1.83347059200006,11.6,10.421808463));
#231992=CARTESIAN_POINT('Ctrl Pts',(-1.83424722500006,15.2,10.423696195));
#231993=CARTESIAN_POINT('Ctrl Pts',(-1.83424722500006,11.6,10.423696195));
#231994=CARTESIAN_POINT('Ctrl Pts',(-1.83502821000005,15.2,10.425589666));
#231995=CARTESIAN_POINT('Ctrl Pts',(-1.83502821000005,11.6,10.425589666));
#231996=CARTESIAN_POINT('Ctrl Pts',(-1.83581355100006,15.2,10.427488856));
#231997=CARTESIAN_POINT('Ctrl Pts',(-1.83581355100006,11.6,10.427488856));
#231998=CARTESIAN_POINT('Ctrl Pts',(-1.83660325400006,15.2,10.42939375));
#231999=CARTESIAN_POINT('Ctrl Pts',(-1.83660325400006,11.6,10.42939375));
#232000=CARTESIAN_POINT('Ctrl Pts',(-1.83739732400006,15.2,10.431304328));
#232001=CARTESIAN_POINT('Ctrl Pts',(-1.83739732400006,11.6,10.431304328));
#232002=CARTESIAN_POINT('Ctrl Pts',(-1.83819576400006,15.2,10.433220574));
#232003=CARTESIAN_POINT('Ctrl Pts',(-1.83819576400006,11.6,10.433220574));
#232004=CARTESIAN_POINT('Ctrl Pts',(-1.83899858000005,15.2,10.435142469));
#232005=CARTESIAN_POINT('Ctrl Pts',(-1.83899858000005,11.6,10.435142469));
#232006=CARTESIAN_POINT('Ctrl Pts',(-1.83980577600006,15.2,10.437069993));
#232007=CARTESIAN_POINT('Ctrl Pts',(-1.83980577600006,11.6,10.437069993));
#232008=CARTESIAN_POINT('Ctrl Pts',(-1.84061735700006,15.2,10.439003133));
#232009=CARTESIAN_POINT('Ctrl Pts',(-1.84061735700006,11.6,10.439003133));
#232010=CARTESIAN_POINT('Ctrl Pts',(-1.84143332700006,15.2,10.440941867));
#232011=CARTESIAN_POINT('Ctrl Pts',(-1.84143332700006,11.6,10.440941867));
#232012=CARTESIAN_POINT('Ctrl Pts',(-1.84225369100006,15.2,10.442886179));
#232013=CARTESIAN_POINT('Ctrl Pts',(-1.84225369100006,11.6,10.442886179));
#232014=CARTESIAN_POINT('Ctrl Pts',(-1.84307845300005,15.2,10.444836052));
#232015=CARTESIAN_POINT('Ctrl Pts',(-1.84307845300005,11.6,10.444836052));
#232016=CARTESIAN_POINT('Ctrl Pts',(-1.84390761700006,15.2,10.446791469));
#232017=CARTESIAN_POINT('Ctrl Pts',(-1.84390761700006,11.6,10.446791469));
#232018=CARTESIAN_POINT('Ctrl Pts',(-1.84474118900006,15.2,10.44875241));
#232019=CARTESIAN_POINT('Ctrl Pts',(-1.84474118900006,11.6,10.44875241));
#232020=CARTESIAN_POINT('Ctrl Pts',(-1.84557917400005,15.2,10.45071886));
#232021=CARTESIAN_POINT('Ctrl Pts',(-1.84557917400005,11.6,10.45071886));
#232022=CARTESIAN_POINT('Ctrl Pts',(-1.84642157300006,15.2,10.4526908));
#232023=CARTESIAN_POINT('Ctrl Pts',(-1.84642157300006,11.6,10.4526908));
#232024=CARTESIAN_POINT('Ctrl Pts',(-1.84726839200006,15.2,10.454668215));
#232025=CARTESIAN_POINT('Ctrl Pts',(-1.84726839200006,11.6,10.454668215));
#232026=CARTESIAN_POINT('Ctrl Pts',(-1.84811963700006,15.2,10.456651086));
#232027=CARTESIAN_POINT('Ctrl Pts',(-1.84811963700006,11.6,10.456651086));
#232028=CARTESIAN_POINT('Ctrl Pts',(-1.84897531000005,15.2,10.458639395));
#232029=CARTESIAN_POINT('Ctrl Pts',(-1.84897531000005,11.6,10.458639395));
#232030=CARTESIAN_POINT('Ctrl Pts',(-1.84983541700006,15.2,10.460633126));
#232031=CARTESIAN_POINT('Ctrl Pts',(-1.84983541700006,11.6,10.460633126));
#232032=CARTESIAN_POINT('Ctrl Pts',(-1.85069996000006,15.2,10.462632262));
#232033=CARTESIAN_POINT('Ctrl Pts',(-1.85069996000006,11.6,10.462632262));
#232034=CARTESIAN_POINT('Ctrl Pts',(-1.85156894600006,15.2,10.464636786));
#232035=CARTESIAN_POINT('Ctrl Pts',(-1.85156894600006,11.6,10.464636786));
#232036=CARTESIAN_POINT('Ctrl Pts',(-1.85244237800006,15.2,10.46664668));
#232037=CARTESIAN_POINT('Ctrl Pts',(-1.85244237800006,11.6,10.46664668));
#232038=CARTESIAN_POINT('Ctrl Pts',(-1.85332026000005,15.2,10.468661929));
#232039=CARTESIAN_POINT('Ctrl Pts',(-1.85332026000005,11.6,10.468661929));
#232040=CARTESIAN_POINT('Ctrl Pts',(-1.85420259600006,15.2,10.470682514));
#232041=CARTESIAN_POINT('Ctrl Pts',(-1.85420259600006,11.6,10.470682514));
#232042=CARTESIAN_POINT('Ctrl Pts',(-1.85508939000006,15.2,10.472708419));
#232043=CARTESIAN_POINT('Ctrl Pts',(-1.85508939000006,11.6,10.472708419));
#232044=CARTESIAN_POINT('Ctrl Pts',(-1.85598064800006,15.2,10.474739628));
#232045=CARTESIAN_POINT('Ctrl Pts',(-1.85598064800006,11.6,10.474739628));
#232046=CARTESIAN_POINT('Ctrl Pts',(-1.85687637100005,15.2,10.476776124));
#232047=CARTESIAN_POINT('Ctrl Pts',(-1.85687637100005,11.6,10.476776124));
#232048=CARTESIAN_POINT('Ctrl Pts',(-1.85777656600006,15.2,10.478817888));
#232049=CARTESIAN_POINT('Ctrl Pts',(-1.85777656600006,11.6,10.478817888));
#232050=CARTESIAN_POINT('Ctrl Pts',(-1.85868123400006,15.2,10.480864906));
#232051=CARTESIAN_POINT('Ctrl Pts',(-1.85868123400006,11.6,10.480864906));
#232052=CARTESIAN_POINT('Ctrl Pts',(-1.85959038200005,15.2,10.48291716));
#232053=CARTESIAN_POINT('Ctrl Pts',(-1.85959038200005,11.6,10.48291716));
#232054=CARTESIAN_POINT('Ctrl Pts',(-1.86050401200006,15.2,10.484974635));
#232055=CARTESIAN_POINT('Ctrl Pts',(-1.86050401200006,11.6,10.484974635));
#232056=CARTESIAN_POINT('Ctrl Pts',(-1.86142213000006,15.2,10.487037313));
#232057=CARTESIAN_POINT('Ctrl Pts',(-1.86142213000006,11.6,10.487037313));
#232058=CARTESIAN_POINT('Ctrl Pts',(-1.86234473700006,15.2,10.489105177));
#232059=CARTESIAN_POINT('Ctrl Pts',(-1.86234473700006,11.6,10.489105177));
#232060=CARTESIAN_POINT('Ctrl Pts',(-1.86327183900006,15.2,10.491178213));
#232061=CARTESIAN_POINT('Ctrl Pts',(-1.86327183900006,11.6,10.491178213));
#232062=CARTESIAN_POINT('Ctrl Pts',(-1.86420344100006,15.2,10.493256403));
#232063=CARTESIAN_POINT('Ctrl Pts',(-1.86420344100006,11.6,10.493256403));
#232064=CARTESIAN_POINT('Ctrl Pts',(-1.86513954500006,15.2,10.49533973));
#232065=CARTESIAN_POINT('Ctrl Pts',(-1.86513954500006,11.6,10.49533973));
#232066=CARTESIAN_POINT('Ctrl Pts',(-1.86608015400005,15.2,10.497428179));
#232067=CARTESIAN_POINT('Ctrl Pts',(-1.86608015400005,11.6,10.497428179));
#232068=CARTESIAN_POINT('Ctrl Pts',(-1.86702527300006,15.2,10.499521734));
#232069=CARTESIAN_POINT('Ctrl Pts',(-1.86702527300006,11.6,10.499521734));
#232070=CARTESIAN_POINT('Ctrl Pts',(-1.86797490700006,15.2,10.501620378));
#232071=CARTESIAN_POINT('Ctrl Pts',(-1.86797490700006,11.6,10.501620378));
#232072=CARTESIAN_POINT('Ctrl Pts',(-1.86892905800006,15.2,10.503724094));
#232073=CARTESIAN_POINT('Ctrl Pts',(-1.86892905800006,11.6,10.503724094));
#232074=CARTESIAN_POINT('Ctrl Pts',(-1.86988773000006,15.2,10.505832868));
#232075=CARTESIAN_POINT('Ctrl Pts',(-1.86988773000006,11.6,10.505832868));
#232076=CARTESIAN_POINT('Ctrl Pts',(-1.87085092800006,15.2,10.507946682));
#232077=CARTESIAN_POINT('Ctrl Pts',(-1.87085092800006,11.6,10.507946682));
#232078=CARTESIAN_POINT('Ctrl Pts',(-1.87181865400006,15.2,10.510065522));
#232079=CARTESIAN_POINT('Ctrl Pts',(-1.87181865400006,11.6,10.510065522));
#232080=CARTESIAN_POINT('Ctrl Pts',(-1.87279091300006,15.2,10.512189371));
#232081=CARTESIAN_POINT('Ctrl Pts',(-1.87279091300006,11.6,10.512189371));
#232082=CARTESIAN_POINT('Ctrl Pts',(-1.87376770900005,15.2,10.514318212));
#232083=CARTESIAN_POINT('Ctrl Pts',(-1.87376770900005,11.6,10.514318212));
#232084=CARTESIAN_POINT('Ctrl Pts',(-1.87474904500006,15.2,10.516452031));
#232085=CARTESIAN_POINT('Ctrl Pts',(-1.87474904500006,11.6,10.516452031));
#232086=CARTESIAN_POINT('Ctrl Pts',(-1.87573492300006,15.2,10.518590811));
#232087=CARTESIAN_POINT('Ctrl Pts',(-1.87573492300006,11.6,10.518590811));
#232088=CARTESIAN_POINT('Ctrl Pts',(-1.87672535000006,15.2,10.520734537));
#232089=CARTESIAN_POINT('Ctrl Pts',(-1.87672535000006,11.6,10.520734537));
#232090=CARTESIAN_POINT('Ctrl Pts',(-1.87772032700006,15.2,10.522883192));
#232091=CARTESIAN_POINT('Ctrl Pts',(-1.87772032700006,11.6,10.522883192));
#232092=CARTESIAN_POINT('Ctrl Pts',(-1.87871985800005,15.2,10.525036762));
#232093=CARTESIAN_POINT('Ctrl Pts',(-1.87871985800005,11.6,10.525036762));
#232094=CARTESIAN_POINT('Ctrl Pts',(-1.87972394600005,15.2,10.52719523));
#232095=CARTESIAN_POINT('Ctrl Pts',(-1.87972394600005,11.6,10.52719523));
#232096=CARTESIAN_POINT('Ctrl Pts',(-1.88073259700006,15.2,10.529358581));
#232097=CARTESIAN_POINT('Ctrl Pts',(-1.88073259700006,11.6,10.529358581));
#232098=CARTESIAN_POINT('Ctrl Pts',(-1.88174581300005,15.2,10.531526799));
#232099=CARTESIAN_POINT('Ctrl Pts',(-1.88174581300005,11.6,10.531526799));
#232100=CARTESIAN_POINT('Ctrl Pts',(-1.88276359700006,15.2,10.533699869));
#232101=CARTESIAN_POINT('Ctrl Pts',(-1.88276359700006,11.6,10.533699869));
#232102=CARTESIAN_POINT('Ctrl Pts',(-1.88378595300006,15.2,10.535877775));
#232103=CARTESIAN_POINT('Ctrl Pts',(-1.88378595300006,11.6,10.535877775));
#232104=CARTESIAN_POINT('Ctrl Pts',(-1.88481288500005,15.2,10.538060502));
#232105=CARTESIAN_POINT('Ctrl Pts',(-1.88481288500005,11.6,10.538060502));
#232106=CARTESIAN_POINT('Ctrl Pts',(-1.88584439500006,15.2,10.540248036));
#232107=CARTESIAN_POINT('Ctrl Pts',(-1.88584439500006,11.6,10.540248036));
#232108=CARTESIAN_POINT('Ctrl Pts',(-1.88688048700006,15.2,10.542440358));
#232109=CARTESIAN_POINT('Ctrl Pts',(-1.88688048700006,11.6,10.542440358));
#232110=CARTESIAN_POINT('Ctrl Pts',(-1.88792116500006,15.2,10.544637456));
#232111=CARTESIAN_POINT('Ctrl Pts',(-1.88792116500006,11.6,10.544637456));
#232112=CARTESIAN_POINT('Ctrl Pts',(-1.88896643100006,15.2,10.546839313));
#232113=CARTESIAN_POINT('Ctrl Pts',(-1.88896643100006,11.6,10.546839313));
#232114=CARTESIAN_POINT('Ctrl Pts',(-1.89001629100006,15.2,10.549045914));
#232115=CARTESIAN_POINT('Ctrl Pts',(-1.89001629100006,11.6,10.549045914));
#232116=CARTESIAN_POINT('Ctrl Pts',(-1.89107074600006,15.2,10.551257245));
#232117=CARTESIAN_POINT('Ctrl Pts',(-1.89107074600006,11.6,10.551257245));
#232118=CARTESIAN_POINT('Ctrl Pts',(-1.89212979900006,15.2,10.553473289));
#232119=CARTESIAN_POINT('Ctrl Pts',(-1.89212979900006,11.6,10.553473289));
#232120=CARTESIAN_POINT('Ctrl Pts',(-1.89319345500006,15.2,10.555694031));
#232121=CARTESIAN_POINT('Ctrl Pts',(-1.89319345500006,11.6,10.555694031));
#232122=CARTESIAN_POINT('Ctrl Pts',(-1.89426171700006,15.2,10.557919459));
#232123=CARTESIAN_POINT('Ctrl Pts',(-1.89426171700006,11.6,10.557919459));
#232124=CARTESIAN_POINT('Ctrl Pts',(-1.89533458700006,15.2,10.560149554));
#232125=CARTESIAN_POINT('Ctrl Pts',(-1.89533458700006,11.6,10.560149554));
#232126=CARTESIAN_POINT('Ctrl Pts',(-1.89641206900005,15.2,10.562384303));
#232127=CARTESIAN_POINT('Ctrl Pts',(-1.89641206900005,11.6,10.562384303));
#232128=CARTESIAN_POINT('Ctrl Pts',(-1.89749416700006,15.2,10.564623692));
#232129=CARTESIAN_POINT('Ctrl Pts',(-1.89749416700006,11.6,10.564623692));
#232130=CARTESIAN_POINT('Ctrl Pts',(-1.89858088300006,15.2,10.566867704));
#232131=CARTESIAN_POINT('Ctrl Pts',(-1.89858088300006,11.6,10.566867704));
#232132=CARTESIAN_POINT('Ctrl Pts',(-1.89967222000006,15.2,10.569116324));
#232133=CARTESIAN_POINT('Ctrl Pts',(-1.89967222000006,11.6,10.569116324));
#232134=CARTESIAN_POINT('Ctrl Pts',(-1.90076818200006,15.2,10.571369539));
#232135=CARTESIAN_POINT('Ctrl Pts',(-1.90076818200006,11.6,10.571369539));
#232136=CARTESIAN_POINT('Ctrl Pts',(-1.90186877100006,15.2,10.573627333));
#232137=CARTESIAN_POINT('Ctrl Pts',(-1.90186877100006,11.6,10.573627333));
#232138=CARTESIAN_POINT('Ctrl Pts',(-1.90297399300006,15.2,10.575889692));
#232139=CARTESIAN_POINT('Ctrl Pts',(-1.90297399300006,11.6,10.575889692));
#232140=CARTESIAN_POINT('Ctrl Pts',(-1.90408384600006,15.2,10.578156601));
#232141=CARTESIAN_POINT('Ctrl Pts',(-1.90408384600006,11.6,10.578156601));
#232142=CARTESIAN_POINT('Ctrl Pts',(-1.90519833900006,15.2,10.580428045));
#232143=CARTESIAN_POINT('Ctrl Pts',(-1.90519833900006,11.6,10.580428045));
#232144=CARTESIAN_POINT('Ctrl Pts',(-1.90631747000006,15.2,10.582704009));
#232145=CARTESIAN_POINT('Ctrl Pts',(-1.90631747000006,11.6,10.582704009));
#232146=CARTESIAN_POINT('Ctrl Pts',(-1.90744124500006,15.2,10.584984479));
#232147=CARTESIAN_POINT('Ctrl Pts',(-1.90744124500006,11.6,10.584984479));
#232148=CARTESIAN_POINT('Ctrl Pts',(-1.90856966700006,15.2,10.587269441));
#232149=CARTESIAN_POINT('Ctrl Pts',(-1.90856966700006,11.6,10.587269441));
#232150=CARTESIAN_POINT('Ctrl Pts',(-1.90970273800006,15.2,10.589558879));
#232151=CARTESIAN_POINT('Ctrl Pts',(-1.90970273800006,11.6,10.589558879));
#232152=CARTESIAN_POINT('Ctrl Pts',(-1.91084046000006,15.2,10.591852781));
#232153=CARTESIAN_POINT('Ctrl Pts',(-1.91084046000006,11.6,10.591852781));
#232154=CARTESIAN_POINT('Ctrl Pts',(-1.91198283900006,15.2,10.594151129));
#232155=CARTESIAN_POINT('Ctrl Pts',(-1.91198283900006,11.6,10.594151129));
#232156=CARTESIAN_POINT('Ctrl Pts',(-1.91312987400006,15.2,10.596453911));
#232157=CARTESIAN_POINT('Ctrl Pts',(-1.91312987400006,11.6,10.596453911));
#232158=CARTESIAN_POINT('Ctrl Pts',(-1.91428157100006,15.2,10.598761112));
#232159=CARTESIAN_POINT('Ctrl Pts',(-1.91428157100006,11.6,10.598761112));
#232160=CARTESIAN_POINT('Ctrl Pts',(-1.91543793200006,15.2,10.601072718));
#232161=CARTESIAN_POINT('Ctrl Pts',(-1.91543793200006,11.6,10.601072718));
#232162=CARTESIAN_POINT('Ctrl Pts',(-1.91659896000006,15.2,10.603388714));
#232163=CARTESIAN_POINT('Ctrl Pts',(-1.91659896000006,11.6,10.603388714));
#232164=CARTESIAN_POINT('Ctrl Pts',(-1.91776465700006,15.2,10.605709086));
#232165=CARTESIAN_POINT('Ctrl Pts',(-1.91776465700006,11.6,10.605709086));
#232166=CARTESIAN_POINT('Ctrl Pts',(-1.91893502800006,15.2,10.608033819));
#232167=CARTESIAN_POINT('Ctrl Pts',(-1.91893502800006,11.6,10.608033819));
#232168=CARTESIAN_POINT('Ctrl Pts',(-1.92011007300006,15.2,10.610362901));
#232169=CARTESIAN_POINT('Ctrl Pts',(-1.92011007300006,11.6,10.610362901));
#232170=CARTESIAN_POINT('Ctrl Pts',(-1.92128979700006,15.2,10.612696316));
#232171=CARTESIAN_POINT('Ctrl Pts',(-1.92128979700006,11.6,10.612696316));
#232172=CARTESIAN_POINT('Ctrl Pts',(-1.92247420100006,15.2,10.615034051));
#232173=CARTESIAN_POINT('Ctrl Pts',(-1.92247420100006,11.6,10.615034051));
#232174=CARTESIAN_POINT('Ctrl Pts',(-1.92366329000006,15.2,10.617376091));
#232175=CARTESIAN_POINT('Ctrl Pts',(-1.92366329000006,11.6,10.617376091));
#232176=CARTESIAN_POINT('Ctrl Pts',(-1.92485706500006,15.2,10.619722422));
#232177=CARTESIAN_POINT('Ctrl Pts',(-1.92485706500006,11.6,10.619722422));
#232178=CARTESIAN_POINT('Ctrl Pts',(-1.92605552900006,15.2,10.62207303));
#232179=CARTESIAN_POINT('Ctrl Pts',(-1.92605552900006,11.6,10.62207303));
#232180=CARTESIAN_POINT('Ctrl Pts',(-1.92725868600006,15.2,10.624427901));
#232181=CARTESIAN_POINT('Ctrl Pts',(-1.92725868600006,11.6,10.624427901));
#232182=CARTESIAN_POINT('Ctrl Pts',(-1.92846653700005,15.2,10.626787021));
#232183=CARTESIAN_POINT('Ctrl Pts',(-1.92846653700005,11.6,10.626787021));
#232184=CARTESIAN_POINT('Ctrl Pts',(-1.92967908600005,15.2,10.629150376));
#232185=CARTESIAN_POINT('Ctrl Pts',(-1.92967908600005,11.6,10.629150376));
#232186=CARTESIAN_POINT('Ctrl Pts',(-1.93089633400006,15.2,10.631517953));
#232187=CARTESIAN_POINT('Ctrl Pts',(-1.93089633400006,11.6,10.631517953));
#232188=CARTESIAN_POINT('Ctrl Pts',(-1.93211828500006,15.2,10.633889738));
#232189=CARTESIAN_POINT('Ctrl Pts',(-1.93211828500006,11.6,10.633889738));
#232190=CARTESIAN_POINT('Ctrl Pts',(-1.93334494300006,15.2,10.636265716));
#232191=CARTESIAN_POINT('Ctrl Pts',(-1.93334494300006,11.6,10.636265716));
#232192=CARTESIAN_POINT('Ctrl Pts',(-1.93457630800005,15.2,10.638645874));
#232193=CARTESIAN_POINT('Ctrl Pts',(-1.93457630800005,11.6,10.638645874));
#232194=CARTESIAN_POINT('Ctrl Pts',(-1.93581238400005,15.2,10.641030198));
#232195=CARTESIAN_POINT('Ctrl Pts',(-1.93581238400005,11.6,10.641030198));
#232196=CARTESIAN_POINT('Ctrl Pts',(-1.93705317300006,15.2,10.643418674));
#232197=CARTESIAN_POINT('Ctrl Pts',(-1.93705317300006,11.6,10.643418674));
#232198=CARTESIAN_POINT('Ctrl Pts',(-1.93829867700006,15.2,10.645811289));
#232199=CARTESIAN_POINT('Ctrl Pts',(-1.93829867700006,11.6,10.645811289));
#232200=CARTESIAN_POINT('Ctrl Pts',(-1.93954890100006,15.2,10.648208029));
#232201=CARTESIAN_POINT('Ctrl Pts',(-1.93954890100006,11.6,10.648208029));
#232202=CARTESIAN_POINT('Ctrl Pts',(-1.94080384500006,15.2,10.650608881));
#232203=CARTESIAN_POINT('Ctrl Pts',(-1.94080384500006,11.6,10.650608881));
#232204=CARTESIAN_POINT('Ctrl Pts',(-1.94206351300006,15.2,10.65301383));
#232205=CARTESIAN_POINT('Ctrl Pts',(-1.94206351300006,11.6,10.65301383));
#232206=CARTESIAN_POINT('Ctrl Pts',(-1.94332790700006,15.2,10.655422863));
#232207=CARTESIAN_POINT('Ctrl Pts',(-1.94332790700006,11.6,10.655422863));
#232208=CARTESIAN_POINT('Ctrl Pts',(-1.94459703000006,15.2,10.657835968));
#232209=CARTESIAN_POINT('Ctrl Pts',(-1.94459703000006,11.6,10.657835968));
#232210=CARTESIAN_POINT('Ctrl Pts',(-1.94587088300006,15.2,10.66025313));
#232211=CARTESIAN_POINT('Ctrl Pts',(-1.94587088300006,11.6,10.66025313));
#232212=CARTESIAN_POINT('Ctrl Pts',(-1.94714947000006,15.2,10.662674335));
#232213=CARTESIAN_POINT('Ctrl Pts',(-1.94714947000006,11.6,10.662674335));
#232214=CARTESIAN_POINT('Ctrl Pts',(-1.94843279200006,15.2,10.665099571));
#232215=CARTESIAN_POINT('Ctrl Pts',(-1.94843279200006,11.6,10.665099571));
#232216=CARTESIAN_POINT('Ctrl Pts',(-1.94972085400006,15.2,10.667528824));
#232217=CARTESIAN_POINT('Ctrl Pts',(-1.94972085400006,11.6,10.667528824));
#232218=CARTESIAN_POINT('Ctrl Pts',(-1.95101365600005,15.2,10.669962079));
#232219=CARTESIAN_POINT('Ctrl Pts',(-1.95101365600005,11.6,10.669962079));
#232220=CARTESIAN_POINT('Ctrl Pts',(-1.95231120100006,15.2,10.672399326));
#232221=CARTESIAN_POINT('Ctrl Pts',(-1.95231120100006,11.6,10.672399326));
#232222=CARTESIAN_POINT('Ctrl Pts',(-1.95361349100006,15.2,10.674840549));
#232223=CARTESIAN_POINT('Ctrl Pts',(-1.95361349100006,11.6,10.674840549));
#232224=CARTESIAN_POINT('Ctrl Pts',(-1.95492053000006,15.2,10.677285737));
#232225=CARTESIAN_POINT('Ctrl Pts',(-1.95492053000006,11.6,10.677285737));
#232226=CARTESIAN_POINT('Ctrl Pts',(-1.95623231900006,15.2,10.679734874));
#232227=CARTESIAN_POINT('Ctrl Pts',(-1.95623231900006,11.6,10.679734874));
#232228=CARTESIAN_POINT('Ctrl Pts',(-1.95754886100006,15.2,10.682187949));
#232229=CARTESIAN_POINT('Ctrl Pts',(-1.95754886100006,11.6,10.682187949));
#232230=CARTESIAN_POINT('Ctrl Pts',(-1.95887015700006,15.2,10.684644947));
#232231=CARTESIAN_POINT('Ctrl Pts',(-1.95887015700006,11.6,10.684644947));
#232232=CARTESIAN_POINT('Ctrl Pts',(-1.96019621100006,15.2,10.687105857));
#232233=CARTESIAN_POINT('Ctrl Pts',(-1.96019621100006,11.6,10.687105857));
#232234=CARTESIAN_POINT('Ctrl Pts',(-1.96152702400005,15.2,10.689570664));
#232235=CARTESIAN_POINT('Ctrl Pts',(-1.96152702400005,11.6,10.689570664));
#232236=CARTESIAN_POINT('Ctrl Pts',(-1.96286259900006,15.2,10.692039356));
#232237=CARTESIAN_POINT('Ctrl Pts',(-1.96286259900006,11.6,10.692039356));
#232238=CARTESIAN_POINT('Ctrl Pts',(-1.96420293800006,15.2,10.69451192));
#232239=CARTESIAN_POINT('Ctrl Pts',(-1.96420293800006,11.6,10.69451192));
#232240=CARTESIAN_POINT('Ctrl Pts',(-1.96554804400006,15.2,10.696988341));
#232241=CARTESIAN_POINT('Ctrl Pts',(-1.96554804400006,11.6,10.696988341));
#232242=CARTESIAN_POINT('Ctrl Pts',(-1.96689791800006,15.2,10.699468609));
#232243=CARTESIAN_POINT('Ctrl Pts',(-1.96689791800006,11.6,10.699468609));
#232244=CARTESIAN_POINT('Ctrl Pts',(-1.96825256200006,15.2,10.701952709));
#232245=CARTESIAN_POINT('Ctrl Pts',(-1.96825256200006,11.6,10.701952709));
#232246=CARTESIAN_POINT('Ctrl Pts',(-1.96961198100006,15.2,10.704440629));
#232247=CARTESIAN_POINT('Ctrl Pts',(-1.96961198100006,11.6,10.704440629));
#232248=CARTESIAN_POINT('Ctrl Pts',(-1.97097617400006,15.2,10.706932356));
#232249=CARTESIAN_POINT('Ctrl Pts',(-1.97097617400006,11.6,10.706932356));
#232250=CARTESIAN_POINT('Ctrl Pts',(-1.97234514400006,15.2,10.709427877));
#232251=CARTESIAN_POINT('Ctrl Pts',(-1.97234514400006,11.6,10.709427877));
#232252=CARTESIAN_POINT('Ctrl Pts',(-1.97371889400005,15.2,10.711927178));
#232253=CARTESIAN_POINT('Ctrl Pts',(-1.97371889400005,11.6,10.711927178));
#232254=CARTESIAN_POINT('Ctrl Pts',(-1.97509742500006,15.2,10.714430247));
#232255=CARTESIAN_POINT('Ctrl Pts',(-1.97509742500006,11.6,10.714430247));
#232256=CARTESIAN_POINT('Ctrl Pts',(-1.97648074000006,15.2,10.716937072));
#232257=CARTESIAN_POINT('Ctrl Pts',(-1.97648074000006,11.6,10.716937072));
#232258=CARTESIAN_POINT('Ctrl Pts',(-1.97786884200006,15.2,10.719447641));
#232259=CARTESIAN_POINT('Ctrl Pts',(-1.97786884200006,11.6,10.719447641));
#232260=CARTESIAN_POINT('Ctrl Pts',(-1.97926173100006,15.2,10.721961938));
#232261=CARTESIAN_POINT('Ctrl Pts',(-1.97926173100006,11.6,10.721961938));
#232262=CARTESIAN_POINT('Ctrl Pts',(-1.98065941000006,15.2,10.724479953));
#232263=CARTESIAN_POINT('Ctrl Pts',(-1.98065941000006,11.6,10.724479953));
#232264=CARTESIAN_POINT('Ctrl Pts',(-1.98206188100006,15.2,10.727001672));
#232265=CARTESIAN_POINT('Ctrl Pts',(-1.98206188100006,11.6,10.727001672));
#232266=CARTESIAN_POINT('Ctrl Pts',(-1.98346914700006,15.2,10.729527083));
#232267=CARTESIAN_POINT('Ctrl Pts',(-1.98346914700006,11.6,10.729527083));
#232268=CARTESIAN_POINT('Ctrl Pts',(-1.98488120800006,15.2,10.732056173));
#232269=CARTESIAN_POINT('Ctrl Pts',(-1.98488120800006,11.6,10.732056173));
#232270=CARTESIAN_POINT('Ctrl Pts',(-1.98629806800006,15.2,10.73458893));
#232271=CARTESIAN_POINT('Ctrl Pts',(-1.98629806800006,11.6,10.73458893));
#232272=CARTESIAN_POINT('Ctrl Pts',(-1.98771972900006,15.2,10.737125342));
#232273=CARTESIAN_POINT('Ctrl Pts',(-1.98771972900006,11.6,10.737125342));
#232274=CARTESIAN_POINT('Ctrl Pts',(-1.98914619100006,15.2,10.739665394));
#232275=CARTESIAN_POINT('Ctrl Pts',(-1.98914619100006,11.6,10.739665394));
#232276=CARTESIAN_POINT('Ctrl Pts',(-1.99057745700005,15.2,10.742209076));
#232277=CARTESIAN_POINT('Ctrl Pts',(-1.99057745700005,11.6,10.742209076));
#232278=CARTESIAN_POINT('Ctrl Pts',(-1.99201353000006,15.2,10.744756373));
#232279=CARTESIAN_POINT('Ctrl Pts',(-1.99201353000006,11.6,10.744756373));
#232280=CARTESIAN_POINT('Ctrl Pts',(-1.99345441100006,15.2,10.747307276));
#232281=CARTESIAN_POINT('Ctrl Pts',(-1.99345441100006,11.6,10.747307276));
#232282=CARTESIAN_POINT('Ctrl Pts',(-1.99490010200006,15.2,10.74986177));
#232283=CARTESIAN_POINT('Ctrl Pts',(-1.99490010200006,11.6,10.74986177));
#232284=CARTESIAN_POINT('Ctrl Pts',(-1.99635060500006,15.2,10.752419843));
#232285=CARTESIAN_POINT('Ctrl Pts',(-1.99635060500006,11.6,10.752419843));
#232286=CARTESIAN_POINT('Ctrl Pts',(-1.99780592300006,15.2,10.754981483));
#232287=CARTESIAN_POINT('Ctrl Pts',(-1.99780592300006,11.6,10.754981483));
#232288=CARTESIAN_POINT('Ctrl Pts',(-1.99926605600006,15.2,10.757546678));
#232289=CARTESIAN_POINT('Ctrl Pts',(-1.99926605600006,11.6,10.757546678));
#232290=CARTESIAN_POINT('Ctrl Pts',(-2.00073100600005,15.2,10.760115415));
#232291=CARTESIAN_POINT('Ctrl Pts',(-2.00073100600005,11.6,10.760115415));
#232292=CARTESIAN_POINT('Ctrl Pts',(-2.00220077600005,15.2,10.762687682));
#232293=CARTESIAN_POINT('Ctrl Pts',(-2.00220077600005,11.6,10.762687682));
#232294=CARTESIAN_POINT('Ctrl Pts',(-2.00367536800006,15.2,10.765263466));
#232295=CARTESIAN_POINT('Ctrl Pts',(-2.00367536800006,11.6,10.765263466));
#232296=CARTESIAN_POINT('Ctrl Pts',(-2.00515478300006,15.2,10.767842757));
#232297=CARTESIAN_POINT('Ctrl Pts',(-2.00515478300006,11.6,10.767842757));
#232298=CARTESIAN_POINT('Ctrl Pts',(-2.00663902300006,15.2,10.770425539));
#232299=CARTESIAN_POINT('Ctrl Pts',(-2.00663902300006,11.6,10.770425539));
#232300=CARTESIAN_POINT('Ctrl Pts',(-2.00812809100006,15.2,10.773011804));
#232301=CARTESIAN_POINT('Ctrl Pts',(-2.00812809100006,11.6,10.773011804));
#232302=CARTESIAN_POINT('Ctrl Pts',(-2.00962198600006,15.2,10.775601537));
#232303=CARTESIAN_POINT('Ctrl Pts',(-2.00962198600006,11.6,10.775601537));
#232304=CARTESIAN_POINT('Ctrl Pts',(-2.01112071300006,15.2,10.778194727));
#232305=CARTESIAN_POINT('Ctrl Pts',(-2.01112071300006,11.6,10.778194727));
#232306=CARTESIAN_POINT('Ctrl Pts',(-2.01262427200006,15.2,10.780791361));
#232307=CARTESIAN_POINT('Ctrl Pts',(-2.01262427200006,11.6,10.780791361));
#232308=CARTESIAN_POINT('Ctrl Pts',(-2.01413266500006,15.2,10.783391429));
#232309=CARTESIAN_POINT('Ctrl Pts',(-2.01413266500006,11.6,10.783391429));
#232310=CARTESIAN_POINT('Ctrl Pts',(-2.01564589300005,15.2,10.785994916));
#232311=CARTESIAN_POINT('Ctrl Pts',(-2.01564589300005,11.6,10.785994916));
#232312=CARTESIAN_POINT('Ctrl Pts',(-2.01716396000006,15.2,10.788601812));
#232313=CARTESIAN_POINT('Ctrl Pts',(-2.01716396000006,11.6,10.788601812));
#232314=CARTESIAN_POINT('Ctrl Pts',(-2.01868686500006,15.2,10.791212105));
#232315=CARTESIAN_POINT('Ctrl Pts',(-2.01868686500006,11.6,10.791212105));
#232316=CARTESIAN_POINT('Ctrl Pts',(-2.02021461200005,15.2,10.793825782));
#232317=CARTESIAN_POINT('Ctrl Pts',(-2.02021461200005,11.6,10.793825782));
#232318=CARTESIAN_POINT('Ctrl Pts',(-2.02174720100006,15.2,10.796442831));
#232319=CARTESIAN_POINT('Ctrl Pts',(-2.02174720100006,11.6,10.796442831));
#232320=CARTESIAN_POINT('Ctrl Pts',(-2.02328463500006,15.2,10.799063242));
#232321=CARTESIAN_POINT('Ctrl Pts',(-2.02328463500006,11.6,10.799063242));
#232322=CARTESIAN_POINT('Ctrl Pts',(-2.02482691500005,15.2,10.801687001));
#232323=CARTESIAN_POINT('Ctrl Pts',(-2.02482691500005,11.6,10.801687001));
#232324=CARTESIAN_POINT('Ctrl Pts',(-2.02637404300006,15.2,10.804314096));
#232325=CARTESIAN_POINT('Ctrl Pts',(-2.02637404300006,11.6,10.804314096));
#232326=CARTESIAN_POINT('Ctrl Pts',(-2.02792601900006,15.2,10.806944517));
#232327=CARTESIAN_POINT('Ctrl Pts',(-2.02792601900006,11.6,10.806944517));
#232328=CARTESIAN_POINT('Ctrl Pts',(-2.02948284700006,15.2,10.809578251));
#232329=CARTESIAN_POINT('Ctrl Pts',(-2.02948284700006,11.6,10.809578251));
#232330=CARTESIAN_POINT('Ctrl Pts',(-2.03104452800006,15.2,10.812215286));
#232331=CARTESIAN_POINT('Ctrl Pts',(-2.03104452800006,11.6,10.812215286));
#232332=CARTESIAN_POINT('Ctrl Pts',(-2.03261106300006,15.2,10.814855612));
#232333=CARTESIAN_POINT('Ctrl Pts',(-2.03261106300006,11.6,10.814855612));
#232334=CARTESIAN_POINT('Ctrl Pts',(-2.03418245300006,15.2,10.817499214));
#232335=CARTESIAN_POINT('Ctrl Pts',(-2.03418245300006,11.6,10.817499214));
#232336=CARTESIAN_POINT('Ctrl Pts',(-2.03575870100006,15.2,10.820146084));
#232337=CARTESIAN_POINT('Ctrl Pts',(-2.03575870100006,11.6,10.820146084));
#232338=CARTESIAN_POINT('Ctrl Pts',(-2.03733980800005,15.2,10.822796206));
#232339=CARTESIAN_POINT('Ctrl Pts',(-2.03733980800005,11.6,10.822796206));
#232340=CARTESIAN_POINT('Ctrl Pts',(-2.03892577600006,15.2,10.825449573));
#232341=CARTESIAN_POINT('Ctrl Pts',(-2.03892577600006,11.6,10.825449573));
#232342=CARTESIAN_POINT('Ctrl Pts',(-2.04051660600005,15.2,10.828106169));
#232343=CARTESIAN_POINT('Ctrl Pts',(-2.04051660600005,11.6,10.828106169));
#232344=CARTESIAN_POINT('Ctrl Pts',(-2.04211229900006,15.2,10.830765987));
#232345=CARTESIAN_POINT('Ctrl Pts',(-2.04211229900006,11.6,10.830765987));
#232346=CARTESIAN_POINT('Ctrl Pts',(-2.04371285800006,15.2,10.83342901));
#232347=CARTESIAN_POINT('Ctrl Pts',(-2.04371285800006,11.6,10.83342901));
#232348=CARTESIAN_POINT('Ctrl Pts',(-2.04531828300006,15.2,10.836095231));
#232349=CARTESIAN_POINT('Ctrl Pts',(-2.04531828300006,11.6,10.836095231));
#232350=CARTESIAN_POINT('Ctrl Pts',(-2.04692857600006,15.2,10.838764637));
#232351=CARTESIAN_POINT('Ctrl Pts',(-2.04692857600006,11.6,10.838764637));
#232352=CARTESIAN_POINT('Ctrl Pts',(-2.04854373900006,15.2,10.841437215));
#232353=CARTESIAN_POINT('Ctrl Pts',(-2.04854373900006,11.6,10.841437215));
#232354=CARTESIAN_POINT('Ctrl Pts',(-2.05016377400006,15.2,10.844112956));
#232355=CARTESIAN_POINT('Ctrl Pts',(-2.05016377400006,11.6,10.844112956));
#232356=CARTESIAN_POINT('Ctrl Pts',(-2.05178868100006,15.2,10.846791846));
#232357=CARTESIAN_POINT('Ctrl Pts',(-2.05178868100006,11.6,10.846791846));
#232358=CARTESIAN_POINT('Ctrl Pts',(-2.05341846200006,15.2,10.849473875));
#232359=CARTESIAN_POINT('Ctrl Pts',(-2.05341846200006,11.6,10.849473875));
#232360=CARTESIAN_POINT('Ctrl Pts',(-2.05505311800006,15.2,10.852159031));
#232361=CARTESIAN_POINT('Ctrl Pts',(-2.05505311800006,11.6,10.852159031));
#232362=CARTESIAN_POINT('Ctrl Pts',(-2.05669265100005,15.2,10.854847304));
#232363=CARTESIAN_POINT('Ctrl Pts',(-2.05669265100005,11.6,10.854847304));
#232364=CARTESIAN_POINT('Ctrl Pts',(-2.05833706300006,15.2,10.857538681));
#232365=CARTESIAN_POINT('Ctrl Pts',(-2.05833706300006,11.6,10.857538681));
#232366=CARTESIAN_POINT('Ctrl Pts',(-2.05998635400006,15.2,10.86023315));
#232367=CARTESIAN_POINT('Ctrl Pts',(-2.05998635400006,11.6,10.86023315));
#232368=CARTESIAN_POINT('Ctrl Pts',(-2.06164052600006,15.2,10.862930701));
#232369=CARTESIAN_POINT('Ctrl Pts',(-2.06164052600006,11.6,10.862930701));
#232370=CARTESIAN_POINT('Ctrl Pts',(-2.06329958100006,15.2,10.865631324));
#232371=CARTESIAN_POINT('Ctrl Pts',(-2.06329958100006,11.6,10.865631324));
#232372=CARTESIAN_POINT('Ctrl Pts',(-2.06496352000006,15.2,10.868335004));
#232373=CARTESIAN_POINT('Ctrl Pts',(-2.06496352000006,11.6,10.868335004));
#232374=CARTESIAN_POINT('Ctrl Pts',(-2.06663234400006,15.2,10.871041733));
#232375=CARTESIAN_POINT('Ctrl Pts',(-2.06663234400006,11.6,10.871041733));
#232376=CARTESIAN_POINT('Ctrl Pts',(-2.06830605500006,15.2,10.873751498));
#232377=CARTESIAN_POINT('Ctrl Pts',(-2.06830605500006,11.6,10.873751498));
#232378=CARTESIAN_POINT('Ctrl Pts',(-2.06998465300006,15.2,10.876464289));
#232379=CARTESIAN_POINT('Ctrl Pts',(-2.06998465300006,11.6,10.876464289));
#232380=CARTESIAN_POINT('Ctrl Pts',(-2.07166814000006,15.2,10.879180095));
#232381=CARTESIAN_POINT('Ctrl Pts',(-2.07166814000006,11.6,10.879180095));
#232382=CARTESIAN_POINT('Ctrl Pts',(-2.07335651800005,15.2,10.881898902));
#232383=CARTESIAN_POINT('Ctrl Pts',(-2.07335651800005,11.6,10.881898902));
#232384=CARTESIAN_POINT('Ctrl Pts',(-2.07504978800006,15.2,10.884620702));
#232385=CARTESIAN_POINT('Ctrl Pts',(-2.07504978800006,11.6,10.884620702));
#232386=CARTESIAN_POINT('Ctrl Pts',(-2.07674795100006,15.2,10.887345482));
#232387=CARTESIAN_POINT('Ctrl Pts',(-2.07674795100006,11.6,10.887345482));
#232388=CARTESIAN_POINT('Ctrl Pts',(-2.07845100800006,15.2,10.890073232));
#232389=CARTESIAN_POINT('Ctrl Pts',(-2.07845100800006,11.6,10.890073232));
#232390=CARTESIAN_POINT('Ctrl Pts',(-2.08015896100005,15.2,10.892803939));
#232391=CARTESIAN_POINT('Ctrl Pts',(-2.08015896100005,11.6,10.892803939));
#232392=CARTESIAN_POINT('Ctrl Pts',(-2.08187181100006,15.2,10.895537595));
#232393=CARTESIAN_POINT('Ctrl Pts',(-2.08187181100006,11.6,10.895537595));
#232394=CARTESIAN_POINT('Ctrl Pts',(-2.08358955800006,15.2,10.898274187));
#232395=CARTESIAN_POINT('Ctrl Pts',(-2.08358955800006,11.6,10.898274187));
#232396=CARTESIAN_POINT('Ctrl Pts',(-2.08531220600006,15.2,10.901013704));
#232397=CARTESIAN_POINT('Ctrl Pts',(-2.08531220600006,11.6,10.901013704));
#232398=CARTESIAN_POINT('Ctrl Pts',(-2.08703975300006,15.2,10.903756135));
#232399=CARTESIAN_POINT('Ctrl Pts',(-2.08703975300006,11.6,10.903756135));
#232400=CARTESIAN_POINT('Ctrl Pts',(-2.08877220300006,15.2,10.906501469));
#232401=CARTESIAN_POINT('Ctrl Pts',(-2.08877220300006,11.6,10.906501469));
#232402=CARTESIAN_POINT('Ctrl Pts',(-2.09050955500006,15.2,10.909249696));
#232403=CARTESIAN_POINT('Ctrl Pts',(-2.09050955500006,11.6,10.909249696));
#232404=CARTESIAN_POINT('Ctrl Pts',(-2.09225181300006,15.2,10.912000804));
#232405=CARTESIAN_POINT('Ctrl Pts',(-2.09225181300006,11.6,10.912000804));
#232406=CARTESIAN_POINT('Ctrl Pts',(-2.09399897400006,15.2,10.914754782));
#232407=CARTESIAN_POINT('Ctrl Pts',(-2.09399897400006,11.6,10.914754782));
#232408=CARTESIAN_POINT('Ctrl Pts',(-2.09575104200006,15.2,10.91751162));
#232409=CARTESIAN_POINT('Ctrl Pts',(-2.09575104200006,11.6,10.91751162));
#232410=CARTESIAN_POINT('Ctrl Pts',(-2.09750801800006,15.2,10.920271306));
#232411=CARTESIAN_POINT('Ctrl Pts',(-2.09750801800006,11.6,10.920271306));
#232412=CARTESIAN_POINT('Ctrl Pts',(-2.09926990300006,15.2,10.923033831));
#232413=CARTESIAN_POINT('Ctrl Pts',(-2.09926990300006,11.6,10.923033831));
#232414=CARTESIAN_POINT('Ctrl Pts',(-2.10103669800006,15.2,10.925799181));
#232415=CARTESIAN_POINT('Ctrl Pts',(-2.10103669800006,11.6,10.925799181));
#232416=CARTESIAN_POINT('Ctrl Pts',(-2.10280840300006,15.2,10.928567349));
#232417=CARTESIAN_POINT('Ctrl Pts',(-2.10280840300006,11.6,10.928567349));
#232418=CARTESIAN_POINT('Ctrl Pts',(-2.10458502100006,15.2,10.931338321));
#232419=CARTESIAN_POINT('Ctrl Pts',(-2.10458502100006,11.6,10.931338321));
#232420=CARTESIAN_POINT('Ctrl Pts',(-2.10636655200005,15.2,10.934112088));
#232421=CARTESIAN_POINT('Ctrl Pts',(-2.10636655200005,11.6,10.934112088));
#232422=CARTESIAN_POINT('Ctrl Pts',(-2.10815299700006,15.2,10.936888639));
#232423=CARTESIAN_POINT('Ctrl Pts',(-2.10815299700006,11.6,10.936888639));
#232424=CARTESIAN_POINT('Ctrl Pts',(-2.10994435800006,15.2,10.939667962));
#232425=CARTESIAN_POINT('Ctrl Pts',(-2.10994435800006,11.6,10.939667962));
#232426=CARTESIAN_POINT('Ctrl Pts',(-2.11174063500006,15.2,10.942450048));
#232427=CARTESIAN_POINT('Ctrl Pts',(-2.11174063500006,11.6,10.942450048));
#232428=CARTESIAN_POINT('Ctrl Pts',(-2.11354183000006,15.2,10.945234886));
#232429=CARTESIAN_POINT('Ctrl Pts',(-2.11354183000006,11.6,10.945234886));
#232430=CARTESIAN_POINT('Ctrl Pts',(-2.11534794300006,15.2,10.948022464));
#232431=CARTESIAN_POINT('Ctrl Pts',(-2.11534794300006,11.6,10.948022464));
#232432=CARTESIAN_POINT('Ctrl Pts',(-2.11715897500006,15.2,10.950812773));
#232433=CARTESIAN_POINT('Ctrl Pts',(-2.11715897500006,11.6,10.950812773));
#232434=CARTESIAN_POINT('Ctrl Pts',(-2.11897492800006,15.2,10.953605801));
#232435=CARTESIAN_POINT('Ctrl Pts',(-2.11897492800006,11.6,10.953605801));
#232436=CARTESIAN_POINT('Ctrl Pts',(-2.12079580400005,15.2,10.956401538));
#232437=CARTESIAN_POINT('Ctrl Pts',(-2.12079580400005,11.6,10.956401538));
#232438=CARTESIAN_POINT('Ctrl Pts',(-2.12262160100006,15.2,10.959199973));
#232439=CARTESIAN_POINT('Ctrl Pts',(-2.12262160100006,11.6,10.959199973));
#232440=CARTESIAN_POINT('Ctrl Pts',(-2.12445232200006,15.2,10.962001097));
#232441=CARTESIAN_POINT('Ctrl Pts',(-2.12445232200006,11.6,10.962001097));
#232442=CARTESIAN_POINT('Ctrl Pts',(-2.12628796700006,15.2,10.964804897));
#232443=CARTESIAN_POINT('Ctrl Pts',(-2.12628796700006,11.6,10.964804897));
#232444=CARTESIAN_POINT('Ctrl Pts',(-2.12812853900005,15.2,10.967611364));
#232445=CARTESIAN_POINT('Ctrl Pts',(-2.12812853900005,11.6,10.967611364));
#232446=CARTESIAN_POINT('Ctrl Pts',(-2.12997403700005,15.2,10.970420488));
#232447=CARTESIAN_POINT('Ctrl Pts',(-2.12997403700005,11.6,10.970420488));
#232448=CARTESIAN_POINT('Ctrl Pts',(-2.13182446200006,15.2,10.973232257));
#232449=CARTESIAN_POINT('Ctrl Pts',(-2.13182446200006,11.6,10.973232257));
#232450=CARTESIAN_POINT('Ctrl Pts',(-2.13367981500005,15.2,10.976046662));
#232451=CARTESIAN_POINT('Ctrl Pts',(-2.13367981500005,11.6,10.976046662));
#232452=CARTESIAN_POINT('Ctrl Pts',(-2.13554009800006,15.2,10.978863691));
#232453=CARTESIAN_POINT('Ctrl Pts',(-2.13554009800006,11.6,10.978863691));
#232454=CARTESIAN_POINT('Ctrl Pts',(-2.13740531100005,15.2,10.981683335));
#232455=CARTESIAN_POINT('Ctrl Pts',(-2.13740531100005,11.6,10.981683335));
#232456=CARTESIAN_POINT('Ctrl Pts',(-2.13927545500006,15.2,10.984505582));
#232457=CARTESIAN_POINT('Ctrl Pts',(-2.13927545500006,11.6,10.984505582));
#232458=CARTESIAN_POINT('Ctrl Pts',(-2.14115053100006,15.2,10.987330423));
#232459=CARTESIAN_POINT('Ctrl Pts',(-2.14115053100006,11.6,10.987330423));
#232460=CARTESIAN_POINT('Ctrl Pts',(-2.14303054100006,15.2,10.990157848));
#232461=CARTESIAN_POINT('Ctrl Pts',(-2.14303054100006,11.6,10.990157848));
#232462=CARTESIAN_POINT('Ctrl Pts',(-2.14491548400006,15.2,10.992987845));
#232463=CARTESIAN_POINT('Ctrl Pts',(-2.14491548400006,11.6,10.992987845));
#232464=CARTESIAN_POINT('Ctrl Pts',(-2.14680536100006,15.2,10.995820404));
#232465=CARTESIAN_POINT('Ctrl Pts',(-2.14680536100006,11.6,10.995820404));
#232466=CARTESIAN_POINT('Ctrl Pts',(-2.14870017400006,15.2,10.998655516));
#232467=CARTESIAN_POINT('Ctrl Pts',(-2.14870017400006,11.6,10.998655516));
#232468=CARTESIAN_POINT('Ctrl Pts',(-2.15059992400006,15.2,11.00149317));
#232469=CARTESIAN_POINT('Ctrl Pts',(-2.15059992400006,11.6,11.00149317));
#232470=CARTESIAN_POINT('Ctrl Pts',(-2.15250461100006,15.2,11.004333354));
#232471=CARTESIAN_POINT('Ctrl Pts',(-2.15250461100006,11.6,11.004333354));
#232472=CARTESIAN_POINT('Ctrl Pts',(-2.15441423500006,15.2,11.007176061));
#232473=CARTESIAN_POINT('Ctrl Pts',(-2.15441423500006,11.6,11.007176061));
#232474=CARTESIAN_POINT('Ctrl Pts',(-2.15632879900005,15.2,11.010021279));
#232475=CARTESIAN_POINT('Ctrl Pts',(-2.15632879900005,11.6,11.010021279));
#232476=CARTESIAN_POINT('Ctrl Pts',(-2.15824830200006,15.2,11.012868997));
#232477=CARTESIAN_POINT('Ctrl Pts',(-2.15824830200006,11.6,11.012868997));
#232478=CARTESIAN_POINT('Ctrl Pts',(-2.16017274700006,15.2,11.015719206));
#232479=CARTESIAN_POINT('Ctrl Pts',(-2.16017274700006,11.6,11.015719206));
#232480=CARTESIAN_POINT('Ctrl Pts',(-2.16210213200006,15.2,11.018571894));
#232481=CARTESIAN_POINT('Ctrl Pts',(-2.16210213200006,11.6,11.018571894));
#232482=CARTESIAN_POINT('Ctrl Pts',(-2.16403645900006,15.2,11.021427054));
#232483=CARTESIAN_POINT('Ctrl Pts',(-2.16403645900006,11.6,11.021427054));
#232484=CARTESIAN_POINT('Ctrl Pts',(-2.16597572900006,15.2,11.024284674));
#232485=CARTESIAN_POINT('Ctrl Pts',(-2.16597572900006,11.6,11.024284674));
#232486=CARTESIAN_POINT('Ctrl Pts',(-2.16791994200006,15.2,11.027144743));
#232487=CARTESIAN_POINT('Ctrl Pts',(-2.16791994200006,11.6,11.027144743));
#232488=CARTESIAN_POINT('Ctrl Pts',(-2.16986910100006,15.2,11.030007253));
#232489=CARTESIAN_POINT('Ctrl Pts',(-2.16986910100006,11.6,11.030007253));
#232490=CARTESIAN_POINT('Ctrl Pts',(-2.17182320400005,15.2,11.032872191));
#232491=CARTESIAN_POINT('Ctrl Pts',(-2.17182320400005,11.6,11.032872191));
#232492=CARTESIAN_POINT('Ctrl Pts',(-2.17378225200005,15.2,11.03573955));
#232493=CARTESIAN_POINT('Ctrl Pts',(-2.17378225200005,11.6,11.03573955));
#232494=CARTESIAN_POINT('Ctrl Pts',(-2.17574624800006,15.2,11.038609318));
#232495=CARTESIAN_POINT('Ctrl Pts',(-2.17574624800006,11.6,11.038609318));
#232496=CARTESIAN_POINT('Ctrl Pts',(-2.17771519000005,15.2,11.041481486));
#232497=CARTESIAN_POINT('Ctrl Pts',(-2.17771519000005,11.6,11.041481486));
#232498=CARTESIAN_POINT('Ctrl Pts',(-2.17968908100006,15.2,11.044356044));
#232499=CARTESIAN_POINT('Ctrl Pts',(-2.17968908100006,11.6,11.044356044));
#232500=CARTESIAN_POINT('Ctrl Pts',(-2.18166792000006,15.2,11.047232981));
#232501=CARTESIAN_POINT('Ctrl Pts',(-2.18166792000006,11.6,11.047232981));
#232502=CARTESIAN_POINT('Ctrl Pts',(-2.18365170900006,15.2,11.050112287));
#232503=CARTESIAN_POINT('Ctrl Pts',(-2.18365170900006,11.6,11.050112287));
#232504=CARTESIAN_POINT('Ctrl Pts',(-2.18564044700006,15.2,11.052993953));
#232505=CARTESIAN_POINT('Ctrl Pts',(-2.18564044700006,11.6,11.052993953));
#232506=CARTESIAN_POINT('Ctrl Pts',(-2.18763413600006,15.2,11.05587797));
#232507=CARTESIAN_POINT('Ctrl Pts',(-2.18763413600006,11.6,11.05587797));
#232508=CARTESIAN_POINT('Ctrl Pts',(-2.18963277800006,15.2,11.058764325));
#232509=CARTESIAN_POINT('Ctrl Pts',(-2.18963277800006,11.6,11.058764325));
#232510=CARTESIAN_POINT('Ctrl Pts',(-2.19163637000006,15.2,11.06165301));
#232511=CARTESIAN_POINT('Ctrl Pts',(-2.19163637000006,11.6,11.06165301));
#232512=CARTESIAN_POINT('Ctrl Pts',(-2.19364491500006,15.2,11.064544015));
#232513=CARTESIAN_POINT('Ctrl Pts',(-2.19364491500006,11.6,11.064544015));
#232514=CARTESIAN_POINT('Ctrl Pts',(-2.19565841400006,15.2,11.06743733));
#232515=CARTESIAN_POINT('Ctrl Pts',(-2.19565841400006,11.6,11.06743733));
#232516=CARTESIAN_POINT('Ctrl Pts',(-2.19767686600005,15.2,11.070332946));
#232517=CARTESIAN_POINT('Ctrl Pts',(-2.19767686600005,11.6,11.070332946));
#232518=CARTESIAN_POINT('Ctrl Pts',(-2.19970027200006,15.2,11.073230851));
#232519=CARTESIAN_POINT('Ctrl Pts',(-2.19970027200006,11.6,11.073230851));
#232520=CARTESIAN_POINT('Ctrl Pts',(-2.20172863400005,15.2,11.076131037));
#232521=CARTESIAN_POINT('Ctrl Pts',(-2.20172863400005,11.6,11.076131037));
#232522=CARTESIAN_POINT('Ctrl Pts',(-2.20376195100005,15.2,11.079033494));
#232523=CARTESIAN_POINT('Ctrl Pts',(-2.20376195100005,11.6,11.079033494));
#232524=CARTESIAN_POINT('Ctrl Pts',(-2.20580022500006,15.2,11.081938211));
#232525=CARTESIAN_POINT('Ctrl Pts',(-2.20580022500006,11.6,11.081938211));
#232526=CARTESIAN_POINT('Ctrl Pts',(-2.20784345600006,15.2,11.08484518));
#232527=CARTESIAN_POINT('Ctrl Pts',(-2.20784345600006,11.6,11.08484518));
#232528=CARTESIAN_POINT('Ctrl Pts',(-2.20989164400006,15.2,11.08775439));
#232529=CARTESIAN_POINT('Ctrl Pts',(-2.20989164400006,11.6,11.08775439));
#232530=CARTESIAN_POINT('Ctrl Pts',(-2.21194479000005,15.2,11.090665832));
#232531=CARTESIAN_POINT('Ctrl Pts',(-2.21194479000005,11.6,11.090665832));
#232532=CARTESIAN_POINT('Ctrl Pts',(-2.21400289400006,15.2,11.093579495));
#232533=CARTESIAN_POINT('Ctrl Pts',(-2.21400289400006,11.6,11.093579495));
#232534=CARTESIAN_POINT('Ctrl Pts',(-2.21606595800006,15.2,11.09649537));
#232535=CARTESIAN_POINT('Ctrl Pts',(-2.21606595800006,11.6,11.09649537));
#232536=CARTESIAN_POINT('Ctrl Pts',(-2.21813398100006,15.2,11.099413448));
#232537=CARTESIAN_POINT('Ctrl Pts',(-2.21813398100006,11.6,11.099413448));
#232538=CARTESIAN_POINT('Ctrl Pts',(-2.22020696400006,15.2,11.102333719));
#232539=CARTESIAN_POINT('Ctrl Pts',(-2.22020696400006,11.6,11.102333719));
#232540=CARTESIAN_POINT('Ctrl Pts',(-2.22228490800005,15.2,11.105256173));
#232541=CARTESIAN_POINT('Ctrl Pts',(-2.22228490800005,11.6,11.105256173));
#232542=CARTESIAN_POINT('Ctrl Pts',(-2.22436781300006,15.2,11.1081808));
#232543=CARTESIAN_POINT('Ctrl Pts',(-2.22436781300006,11.6,11.1081808));
#232544=CARTESIAN_POINT('Ctrl Pts',(-2.22645567900006,15.2,11.111107592));
#232545=CARTESIAN_POINT('Ctrl Pts',(-2.22645567900006,11.6,11.111107592));
#232546=CARTESIAN_POINT('Ctrl Pts',(-2.22854850800006,15.2,11.114036538));
#232547=CARTESIAN_POINT('Ctrl Pts',(-2.22854850800006,11.6,11.114036538));
#232548=CARTESIAN_POINT('Ctrl Pts',(-2.23064629900006,15.2,11.116967628));
#232549=CARTESIAN_POINT('Ctrl Pts',(-2.23064629900006,11.6,11.116967628));
#232550=CARTESIAN_POINT('Ctrl Pts',(-2.23274905300006,15.2,11.119900853));
#232551=CARTESIAN_POINT('Ctrl Pts',(-2.23274905300006,11.6,11.119900853));
#232552=CARTESIAN_POINT('Ctrl Pts',(-2.23485677000005,15.2,11.122836203));
#232553=CARTESIAN_POINT('Ctrl Pts',(-2.23485677000005,11.6,11.122836203));
#232554=CARTESIAN_POINT('Ctrl Pts',(-2.23696945300006,15.2,11.12577367));
#232555=CARTESIAN_POINT('Ctrl Pts',(-2.23696945300006,11.6,11.12577367));
#232556=CARTESIAN_POINT('Ctrl Pts',(-2.23908709900006,15.2,11.128713244));
#232557=CARTESIAN_POINT('Ctrl Pts',(-2.23908709900006,11.6,11.128713244));
#232558=CARTESIAN_POINT('Ctrl Pts',(-2.24120971000006,15.2,11.131654913));
#232559=CARTESIAN_POINT('Ctrl Pts',(-2.24120971000006,11.6,11.131654913));
#232560=CARTESIAN_POINT('Ctrl Pts',(-2.24333728600006,15.2,11.134598672));
#232561=CARTESIAN_POINT('Ctrl Pts',(-2.24333728600006,11.6,11.134598672));
#232562=CARTESIAN_POINT('Ctrl Pts',(-2.24546982700006,15.2,11.137544507));
#232563=CARTESIAN_POINT('Ctrl Pts',(-2.24546982700006,11.6,11.137544507));
#232564=CARTESIAN_POINT('Ctrl Pts',(-2.24760733500006,15.2,11.140492411));
#232565=CARTESIAN_POINT('Ctrl Pts',(-2.24760733500006,11.6,11.140492411));
#232566=CARTESIAN_POINT('Ctrl Pts',(-2.24974981000006,15.2,11.143442374));
#232567=CARTESIAN_POINT('Ctrl Pts',(-2.24974981000006,11.6,11.143442374));
#232568=CARTESIAN_POINT('Ctrl Pts',(-2.25189725100006,15.2,11.146394387));
#232569=CARTESIAN_POINT('Ctrl Pts',(-2.25189725100006,11.6,11.146394387));
#232570=CARTESIAN_POINT('Ctrl Pts',(-2.25404966000006,15.2,11.14934844));
#232571=CARTESIAN_POINT('Ctrl Pts',(-2.25404966000006,11.6,11.14934844));
#232572=CARTESIAN_POINT('Ctrl Pts',(-2.25620703600006,15.2,11.152304525));
#232573=CARTESIAN_POINT('Ctrl Pts',(-2.25620703600006,11.6,11.152304525));
#232574=CARTESIAN_POINT('Ctrl Pts',(-2.25836938000006,15.2,11.15526263));
#232575=CARTESIAN_POINT('Ctrl Pts',(-2.25836938000006,11.6,11.15526263));
#232576=CARTESIAN_POINT('Ctrl Pts',(-2.26053669300006,15.2,11.158222748));
#232577=CARTESIAN_POINT('Ctrl Pts',(-2.26053669300006,11.6,11.158222748));
#232578=CARTESIAN_POINT('Ctrl Pts',(-2.26270897400005,15.2,11.161184868));
#232579=CARTESIAN_POINT('Ctrl Pts',(-2.26270897400005,11.6,11.161184868));
#232580=CARTESIAN_POINT('Ctrl Pts',(-2.26488622500006,15.2,11.164148983));
#232581=CARTESIAN_POINT('Ctrl Pts',(-2.26488622500006,11.6,11.164148983));
#232582=CARTESIAN_POINT('Ctrl Pts',(-2.26706844500006,15.2,11.16711508));
#232583=CARTESIAN_POINT('Ctrl Pts',(-2.26706844500006,11.6,11.16711508));
#232584=CARTESIAN_POINT('Ctrl Pts',(-2.26925563400005,15.2,11.170083153));
#232585=CARTESIAN_POINT('Ctrl Pts',(-2.26925563400005,11.6,11.170083153));
#232586=CARTESIAN_POINT('Ctrl Pts',(-2.27144779400006,15.2,11.173053191));
#232587=CARTESIAN_POINT('Ctrl Pts',(-2.27144779400006,11.6,11.173053191));
#232588=CARTESIAN_POINT('Ctrl Pts',(-2.27364492400006,15.2,11.176025185));
#232589=CARTESIAN_POINT('Ctrl Pts',(-2.27364492400006,11.6,11.176025185));
#232590=CARTESIAN_POINT('Ctrl Pts',(-2.27584702400006,15.2,11.178999126));
#232591=CARTESIAN_POINT('Ctrl Pts',(-2.27584702400006,11.6,11.178999126));
#232592=CARTESIAN_POINT('Ctrl Pts',(-2.27805409600006,15.2,11.181975005));
#232593=CARTESIAN_POINT('Ctrl Pts',(-2.27805409600006,11.6,11.181975005));
#232594=CARTESIAN_POINT('Ctrl Pts',(-2.28026613900006,15.2,11.184952813));
#232595=CARTESIAN_POINT('Ctrl Pts',(-2.28026613900006,11.6,11.184952813));
#232596=CARTESIAN_POINT('Ctrl Pts',(-2.28248315300006,15.2,11.187932541));
#232597=CARTESIAN_POINT('Ctrl Pts',(-2.28248315300006,11.6,11.187932541));
#232598=CARTESIAN_POINT('Ctrl Pts',(-2.28470513900006,15.2,11.19091418));
#232599=CARTESIAN_POINT('Ctrl Pts',(-2.28470513900006,11.6,11.19091418));
#232600=CARTESIAN_POINT('Ctrl Pts',(-2.28693209700006,15.2,11.193897718));
#232601=CARTESIAN_POINT('Ctrl Pts',(-2.28693209700006,11.6,11.193897718));
#232602=CARTESIAN_POINT('Ctrl Pts',(-2.28916402800006,15.2,11.19688315));
#232603=CARTESIAN_POINT('Ctrl Pts',(-2.28916402800006,11.6,11.19688315));
#232604=CARTESIAN_POINT('Ctrl Pts',(-2.29140093100006,15.2,11.199870463));
#232605=CARTESIAN_POINT('Ctrl Pts',(-2.29140093100006,11.6,11.199870463));
#232606=CARTESIAN_POINT('Ctrl Pts',(-2.29364280600006,15.2,11.202859649));
#232607=CARTESIAN_POINT('Ctrl Pts',(-2.29364280600006,11.6,11.202859649));
#232608=CARTESIAN_POINT('Ctrl Pts',(-2.29588965500006,15.2,11.205850699));
#232609=CARTESIAN_POINT('Ctrl Pts',(-2.29588965500006,11.6,11.205850699));
#232610=CARTESIAN_POINT('Ctrl Pts',(-2.29814147700006,15.2,11.208843603));
#232611=CARTESIAN_POINT('Ctrl Pts',(-2.29814147700006,11.6,11.208843603));
#232612=CARTESIAN_POINT('Ctrl Pts',(-2.30039827300006,15.2,11.211838352));
#232613=CARTESIAN_POINT('Ctrl Pts',(-2.30039827300006,11.6,11.211838352));
#232614=CARTESIAN_POINT('Ctrl Pts',(-2.30266004300006,15.2,11.214834939));
#232615=CARTESIAN_POINT('Ctrl Pts',(-2.30266004300006,11.6,11.214834939));
#232616=CARTESIAN_POINT('Ctrl Pts',(-2.30492678500006,15.2,11.217833355));
#232617=CARTESIAN_POINT('Ctrl Pts',(-2.30492678500006,11.6,11.217833355));
#232618=CARTESIAN_POINT('Ctrl Pts',(-2.30719850200006,15.2,11.220833594));
#232619=CARTESIAN_POINT('Ctrl Pts',(-2.30719850200006,11.6,11.220833594));
#232620=CARTESIAN_POINT('Ctrl Pts',(-2.30947519300006,15.2,11.223835644));
#232621=CARTESIAN_POINT('Ctrl Pts',(-2.30947519300006,11.6,11.223835644));
#232622=CARTESIAN_POINT('Ctrl Pts',(-2.31175685900006,15.2,11.226839497));
#232623=CARTESIAN_POINT('Ctrl Pts',(-2.31175685900006,11.6,11.226839497));
#232624=CARTESIAN_POINT('Ctrl Pts',(-2.31404349900005,15.2,11.229845144));
#232625=CARTESIAN_POINT('Ctrl Pts',(-2.31404349900005,11.6,11.229845144));
#232626=CARTESIAN_POINT('Ctrl Pts',(-2.31633511400006,15.2,11.232852573));
#232627=CARTESIAN_POINT('Ctrl Pts',(-2.31633511400006,11.6,11.232852573));
#232628=CARTESIAN_POINT('Ctrl Pts',(-2.31863170400006,15.2,11.23586177));
#232629=CARTESIAN_POINT('Ctrl Pts',(-2.31863170400006,11.6,11.23586177));
#232630=CARTESIAN_POINT('Ctrl Pts',(-2.32093326800006,15.2,11.238872729));
#232631=CARTESIAN_POINT('Ctrl Pts',(-2.32093326800006,11.6,11.238872729));
#232632=CARTESIAN_POINT('Ctrl Pts',(-2.32323980900006,15.2,11.241885437));
#232633=CARTESIAN_POINT('Ctrl Pts',(-2.32323980900006,11.6,11.241885437));
#232634=CARTESIAN_POINT('Ctrl Pts',(-2.32555132500006,15.2,11.244899888));
#232635=CARTESIAN_POINT('Ctrl Pts',(-2.32555132500006,11.6,11.244899888));
#232636=CARTESIAN_POINT('Ctrl Pts',(-2.32786781600006,15.2,11.247916073));
#232637=CARTESIAN_POINT('Ctrl Pts',(-2.32786781600006,11.6,11.247916073));
#232638=CARTESIAN_POINT('Ctrl Pts',(-2.33018928300006,15.2,11.250933991));
#232639=CARTESIAN_POINT('Ctrl Pts',(-2.33018928300006,11.6,11.250933991));
#232640=CARTESIAN_POINT('Ctrl Pts',(-2.33251572500006,15.2,11.253953638));
#232641=CARTESIAN_POINT('Ctrl Pts',(-2.33251572500006,11.6,11.253953638));
#232642=CARTESIAN_POINT('Ctrl Pts',(-2.33438085900006,15.2,11.256370738));
#232643=CARTESIAN_POINT('Ctrl Pts',(-2.33438085900006,11.6,11.256370738));
#232644=CARTESIAN_POINT('Ctrl Pts',(-2.33578194800006,15.2,11.258184341));
#232645=CARTESIAN_POINT('Ctrl Pts',(-2.33578194800006,11.6,11.258184341));
#232646=CARTESIAN_POINT('Ctrl Pts',(-2.33671700200006,15.2,11.259393755));
#232647=CARTESIAN_POINT('Ctrl Pts',(-2.33671700200006,11.6,11.259393755));
#232648=CARTESIAN_POINT('Ctrl Pts',(-2.33718477800006,15.2,11.259998549));
#232649=CARTESIAN_POINT('Ctrl Pts',(-2.33718477800006,11.6,11.259998549));
#232650=CARTESIAN_POINT('Ctrl Pts',(-1.76496130700006,15.2,10.22377311));
#232651=CARTESIAN_POINT('Ctrl Pts',(-1.76541543493207,15.2,10.2255010873779));
#232652=CARTESIAN_POINT('Ctrl Pts',(-1.76588926591707,15.2,10.2272829938834));
#232653=CARTESIAN_POINT('Ctrl Pts',(-1.76638321147092,15.2,10.2291177140323));
#232654=CARTESIAN_POINT('Ctrl Pts',(-1.76687953907992,15.2,10.2309612821291));
#232655=CARTESIAN_POINT('Ctrl Pts',(-1.76739616286972,15.2,10.2328581799819));
#232656=CARTESIAN_POINT('Ctrl Pts',(-1.76793345451038,15.2,10.2348073231886));
#232657=CARTESIAN_POINT('Ctrl Pts',(-1.76847074610224,15.2,10.2367564662182));
#232658=CARTESIAN_POINT('Ctrl Pts',(-1.76902870497939,15.2,10.2387578539245));
#232659=CARTESIAN_POINT('Ctrl Pts',(-1.76960768654168,15.2,10.2408104330166));
#232660=CARTESIAN_POINT('Ctrl Pts',(-1.77018666810398,15.2,10.2428630121086));
#232661=CARTESIAN_POINT('Ctrl Pts',(-1.77078667246607,15.2,10.2449667819402));
#232662=CARTESIAN_POINT('Ctrl Pts',(-1.77140804397329,15.2,10.24712072005));
#232663=CARTESIAN_POINT('Ctrl Pts',(-1.77202941553697,15.2,10.2492746583554));
#232664=CARTESIAN_POINT('Ctrl Pts',(-1.77267215276809,15.2,10.2514787598444));
#232665=CARTESIAN_POINT('Ctrl Pts',(-1.77333658730578,15.2,10.2537320332205));
#232666=CARTESIAN_POINT('Ctrl Pts',(-1.77400102178312,15.2,10.255985306392));
#232667=CARTESIAN_POINT('Ctrl Pts',(-1.77468715486446,15.2,10.2582877466256));
#232668=CARTESIAN_POINT('Ctrl Pts',(-1.77539530325867,15.2,10.260638386051));
#232669=CARTESIAN_POINT('Ctrl Pts',(-1.77610345165288,15.2,10.2629890254764));
#232670=CARTESIAN_POINT('Ctrl Pts',(-1.77683361717075,15.2,10.2653878615328));
#232671=CARTESIAN_POINT('Ctrl Pts',(-1.77758610564243,15.2,10.2678339508585));
#232672=CARTESIAN_POINT('Ctrl Pts',(-1.77833859418247,15.2,10.2702800404063));
#232673=CARTESIAN_POINT('Ctrl Pts',(-1.77911340904196,15.2,10.2727733804935));
#232674=CARTESIAN_POINT('Ctrl Pts',(-1.77991084258694,15.2,10.2753130495517));
#232675=CARTESIAN_POINT('Ctrl Pts',(-1.7807082760595,15.2,10.2778527183792));
#232676=CARTESIAN_POINT('Ctrl Pts',(-1.78152833193401,15.2,10.2804387173121));
#232677=CARTESIAN_POINT('Ctrl Pts',(-1.78237129432105,15.2,10.2830701451352));
#232678=CARTESIAN_POINT('Ctrl Pts',(-1.7832142567081,15.2,10.2857015729583));
#232679=CARTESIAN_POINT('Ctrl Pts',(-1.78408012798497,15.2,10.2883784311276));
#232680=CARTESIAN_POINT('Ctrl Pts',(-1.78496918228499,15.2,10.2910998401101));
#232681=CARTESIAN_POINT('Ctrl Pts',(-1.78585823658502,15.2,10.2938212490926));
#232682=CARTESIAN_POINT('Ctrl Pts',(-1.78677047506695,15.2,10.2965872102404));
#232683=CARTESIAN_POINT('Ctrl Pts',(-1.7877061643647,15.2,10.2993968662187));
#232684=CARTESIAN_POINT('Ctrl Pts',(-1.7887978019354,15.2,10.3026747983635));
#232685=CARTESIAN_POINT('Ctrl Pts',(-1.78992136090724,15.2,10.3060122026356));
#232686=CARTESIAN_POINT('Ctrl Pts',(-1.79107724768775,15.2,10.3094077546164));
#232687=CARTESIAN_POINT('Ctrl Pts',(-1.79223313446825,15.2,10.3128033065971));
#232688=CARTESIAN_POINT('Ctrl Pts',(-1.79342135008691,15.2,10.3162570016962));
#232689=CARTESIAN_POINT('Ctrl Pts',(-1.79464228456548,15.2,10.3197675544474));
#232690=CARTESIAN_POINT('Ctrl Pts',(-1.79568879977852,15.2,10.3227765995066));
#232691=CARTESIAN_POINT('Ctrl Pts',(-1.79675935631462,15.2,10.325827414804));
#232692=CARTESIAN_POINT('Ctrl Pts',(-1.79785418744045,15.2,10.3289192081066));
#232693=CARTESIAN_POINT('Ctrl Pts',(-1.79913149048688,15.2,10.3325263004801));
#232694=CARTESIAN_POINT('Ctrl Pts',(-1.80044184035678,15.2,10.3361891677487));
#232695=CARTESIAN_POINT('Ctrl Pts',(-1.80178559450887,15.2,10.3399065789764));
#232696=CARTESIAN_POINT('Ctrl Pts',(-1.8029373837223,15.2,10.3430929312918));
#232697=CARTESIAN_POINT('Ctrl Pts',(-1.80411371803772,15.2,10.3463193572175));
#232698=CARTESIAN_POINT('Ctrl Pts',(-1.80531481690965,15.2,10.3495851005138));
#232699=CARTESIAN_POINT('Ctrl Pts',(-1.80651591589069,15.2,10.3528508441067));
#232700=CARTESIAN_POINT('Ctrl Pts',(-1.80774177967481,15.2,10.3561559049212));
#232701=CARTESIAN_POINT('Ctrl Pts',(-1.80899262066136,15.2,10.359499539856));
#232702=CARTESIAN_POINT('Ctrl Pts',(-1.81045193497523,15.2,10.3634004468245));
#232703=CARTESIAN_POINT('Ctrl Pts',(-1.81194524810849,15.2,10.3673538598976));
#232704=CARTESIAN_POINT('Ctrl Pts',(-1.81347288367876,15.2,10.371358629063));
#232705=CARTESIAN_POINT('Ctrl Pts',(-1.81478228574905,15.2,10.3747912887485));
#232706=CARTESIAN_POINT('Ctrl Pts',(-1.81611690607242,15.2,10.3782616779469));
#232707=CARTESIAN_POINT('Ctrl Pts',(-1.81747694114826,15.2,10.3817690888906));
#232708=CARTESIAN_POINT('Ctrl Pts',(-1.81883697610056,15.2,10.3852764995156));
#232709=CARTESIAN_POINT('Ctrl Pts',(-1.82022242567718,15.2,10.3888209322404));
#232710=CARTESIAN_POINT('Ctrl Pts',(-1.82163348329369,15.2,10.3924016919452));
#232711=CARTESIAN_POINT('Ctrl Pts',(-1.82327971726508,15.2,10.396579245151));
#232712=CARTESIAN_POINT('Ctrl Pts',(-1.82496080224826,15.2,10.40080624303));
#232713=CARTESIAN_POINT('Ctrl Pts',(-1.82667703515203,15.2,10.405081607141));
#232714=CARTESIAN_POINT('Ctrl Pts',(-1.82814809185033,15.2,10.4087462047603));
#232715=CARTESIAN_POINT('Ctrl Pts',(-1.82964496786233,15.2,10.4124463342712));
#232716=CARTESIAN_POINT('Ctrl Pts',(-1.83116784455811,15.2,10.4161813339703));
#232717=CARTESIAN_POINT('Ctrl Pts',(-1.83243690851737,15.2,10.4192938338326));
#232718=CARTESIAN_POINT('Ctrl Pts',(-1.83372402674008,15.2,10.4224305475944));
#232719=CARTESIAN_POINT('Ctrl Pts',(-1.83502929910215,15.2,10.4255910959984));
#232720=CARTESIAN_POINT('Ctrl Pts',(-1.83633457146423,15.2,10.4287516444025));
#232721=CARTESIAN_POINT('Ctrl Pts',(-1.8376579978042,15.2,10.4319360296438));
#232722=CARTESIAN_POINT('Ctrl Pts',(-1.83899967516415,15.2,10.4351438766807));
#232723=CARTESIAN_POINT('Ctrl Pts',(-1.8406096879376,15.2,10.4389932929851));
#232724=CARTESIAN_POINT('Ctrl Pts',(-1.84224598213541,15.2,10.4428764951005));
#232725=CARTESIAN_POINT('Ctrl Pts',(-1.84390871899168,15.2,10.4467928500416));
#232726=CARTESIAN_POINT('Ctrl Pts',(-1.84529433308891,15.2,10.4500564792777));
#232727=CARTESIAN_POINT('Ctrl Pts',(-1.84669831180539,15.2,10.4533431311977));
#232728=CARTESIAN_POINT('Ctrl Pts',(-1.84812074403412,15.2,10.4566524455184));
#232729=CARTESIAN_POINT('Ctrl Pts',(-1.84954317626286,15.2,10.4599617598391));
#232730=CARTESIAN_POINT('Ctrl Pts',(-1.85098406170572,15.2,10.4632937354628));
#232731=CARTESIAN_POINT('Ctrl Pts',(-1.85244349059557,15.2,10.4666480189361));
#232732=CARTESIAN_POINT('Ctrl Pts',(-1.8539029194854,15.2,10.4700023024094));
#232733=CARTESIAN_POINT('Ctrl Pts',(-1.85538089015814,15.2,10.4733788935545));
#232734=CARTESIAN_POINT('Ctrl Pts',(-1.856877489048,15.2,10.476777441264));
#232735=CARTESIAN_POINT('Ctrl Pts',(-1.85837408793786,15.2,10.4801759889735));
#232736=CARTESIAN_POINT('Ctrl Pts',(-1.8598893144058,15.2,10.4835964935706));
#232737=CARTESIAN_POINT('Ctrl Pts',(-1.86142325246981,15.2,10.4870386099246));
#232738=CARTESIAN_POINT('Ctrl Pts',(-1.86357076562567,15.2,10.49185757252));
#232739=CARTESIAN_POINT('Ctrl Pts',(-1.86575495311634,15.2,10.4967188955553));
#232740=CARTESIAN_POINT('Ctrl Pts',(-1.86797603605917,15.2,10.5016216455669));
#232741=CARTESIAN_POINT('Ctrl Pts',(-1.86956252397429,15.2,10.505123610079));
#232742=CARTESIAN_POINT('Ctrl Pts',(-1.87116783398727,15.2,10.5086467122575));
#232743=CARTESIAN_POINT('Ctrl Pts',(-1.87279204705319,15.2,10.5121906186136));
#232744=CARTESIAN_POINT('Ctrl Pts',(-1.87441626011912,15.2,10.5157345249697));
#232745=CARTESIAN_POINT('Ctrl Pts',(-1.87605937489797,15.2,10.5192992351444));
#232746=CARTESIAN_POINT('Ctrl Pts',(-1.87772146538309,15.2,10.5228844204906));
#232747=CARTESIAN_POINT('Ctrl Pts',(-1.87938355586821,15.2,10.5264696058367));
#232748=CARTESIAN_POINT('Ctrl Pts',(-1.8810646226677,15.2,10.5300752665917));
#232749=CARTESIAN_POINT('Ctrl Pts',(-1.88276473988894,15.2,10.5337010777713));
#232750=CARTESIAN_POINT('Ctrl Pts',(-1.88446485711018,15.2,10.5373268889508));
#232751=CARTESIAN_POINT('Ctrl Pts',(-1.88618402469853,15.2,10.5409728519169));
#232752=CARTESIAN_POINT('Ctrl Pts',(-1.88792231191978,15.2,10.544638645527));
#232753=CARTESIAN_POINT('Ctrl Pts',(-1.88966059914102,15.2,10.5483044391371));
#232754=CARTESIAN_POINT('Ctrl Pts',(-1.89141800780214,15.2,10.5519900629089));
#232755=CARTESIAN_POINT('Ctrl Pts',(-1.89319460649071,15.2,10.5556952024396));
#232756=CARTESIAN_POINT('Ctrl Pts',(-1.89497120517928,15.2,10.5594003419703));
#232757=CARTESIAN_POINT('Ctrl Pts',(-1.89676699360556,15.2,10.5631249979611));
#232758=CARTESIAN_POINT('Ctrl Pts',(-1.89858203825834,15.2,10.5668688560166));
#232759=CARTESIAN_POINT('Ctrl Pts',(-1.9000340740597,15.2,10.5698639426243));
#232760=CARTESIAN_POINT('Ctrl Pts',(-1.90149843394584,15.2,10.5728713194945));
#232761=CARTESIAN_POINT('Ctrl Pts',(-1.90297515108312,15.2,10.5758908299936));
#232762=CARTESIAN_POINT('Ctrl Pts',(-1.90445186801919,15.2,10.5789103400813));
#232763=CARTESIAN_POINT('Ctrl Pts',(-1.90594094191218,15.2,10.5819419825496));
#232764=CARTESIAN_POINT('Ctrl Pts',(-1.90744240674066,15.2,10.5849856019812));
#232765=CARTESIAN_POINT('Ctrl Pts',(-1.90894387177371,15.2,10.5880292218275));
#232766=CARTESIAN_POINT('Ctrl Pts',(-1.91045772694566,15.2,10.5910848193081));
#232767=CARTESIAN_POINT('Ctrl Pts',(-1.9119840033079,15.2,10.5941522379765));
#232768=CARTESIAN_POINT('Ctrl Pts',(-1.91351027946217,15.2,10.5972196562269));
#232769=CARTESIAN_POINT('Ctrl Pts',(-1.91504897688702,15.2,10.6002988976035));
#232770=CARTESIAN_POINT('Ctrl Pts',(-1.91660012714832,15.2,10.603389807739));
#232771=CARTESIAN_POINT('Ctrl Pts',(-1.91815127762096,15.2,10.6064807182957));
#232772=CARTESIAN_POINT('Ctrl Pts',(-1.91971488142971,15.2,10.6095832976644));
#232773=CARTESIAN_POINT('Ctrl Pts',(-1.92129096726211,15.2,10.6126973964352));
#232774=CARTESIAN_POINT('Ctrl Pts',(-1.92326107444525,15.2,10.6165900196865));
#232775=CARTESIAN_POINT('Ctrl Pts',(-1.92525068610564,15.2,10.6205006398734));
#232776=CARTESIAN_POINT('Ctrl Pts',(-1.92725985978782,15.2,10.6244289637638));
#232777=CARTESIAN_POINT('Ctrl Pts',(-1.92926903347,15.2,10.6283572876542));
#232778=CARTESIAN_POINT('Ctrl Pts',(-1.93129776727192,15.2,10.632303316717));
#232779=CARTESIAN_POINT('Ctrl Pts',(-1.93334612005127,15.2,10.63626676151));
#232780=CARTESIAN_POINT('Ctrl Pts',(-1.93498480214079,15.2,10.6394375170853));
#232781=CARTESIAN_POINT('Ctrl Pts',(-1.93663603814127,15.2,10.6426194186693));
#232782=CARTESIAN_POINT('Ctrl Pts',(-1.93829985695721,15.2,10.6458123202561));
#232783=CARTESIAN_POINT('Ctrl Pts',(-1.93996367599985,15.2,10.6490052222779));
#232784=CARTESIAN_POINT('Ctrl Pts',(-1.9416400778606,15.2,10.6522091241576));
#232785=CARTESIAN_POINT('Ctrl Pts',(-1.9433290895095,15.2,10.6554238815006));
#232786=CARTESIAN_POINT('Ctrl Pts',(-1.94501810092827,15.2,10.6586386384055));
#232787=CARTESIAN_POINT('Ctrl Pts',(-1.94671972068151,15.2,10.6618642508535));
#232788=CARTESIAN_POINT('Ctrl Pts',(-1.94843397681832,15.2,10.6651005749771));
#232789=CARTESIAN_POINT('Ctrl Pts',(-1.95014823318869,15.2,10.6683368995417));
#232790=CARTESIAN_POINT('Ctrl Pts',(-1.95187512535022,15.2,10.6715839345065));
#232791=CARTESIAN_POINT('Ctrl Pts',(-1.9536146784775,15.2,10.674841540681));
#232792=CARTESIAN_POINT('Ctrl Pts',(-1.95578911976809,15.2,10.6789135481773));
#232793=CARTESIAN_POINT('Ctrl Pts',(-1.95798334494354,15.2,10.6830020695188));
#232794=CARTESIAN_POINT('Ctrl Pts',(-1.96019740105628,15.2,10.6871068318119));
#232795=CARTESIAN_POINT('Ctrl Pts',(-1.96196864580168,15.2,10.6903906413778));
#232796=CARTESIAN_POINT('Ctrl Pts',(-1.96375258250929,15.2,10.6936848447646));
#232797=CARTESIAN_POINT('Ctrl Pts',(-1.96554923586158,15.2,10.6969893024382));
#232798=CARTESIAN_POINT('Ctrl Pts',(-1.96734588945867,15.2,10.7002937605621));
#232799=CARTESIAN_POINT('Ctrl Pts',(-1.96915525932304,15.2,10.7036084741259));
#232800=CARTESIAN_POINT('Ctrl Pts',(-1.97097736851447,15.2,10.7069333049741));
#232801=CARTESIAN_POINT('Ctrl Pts',(-1.97279947745765,15.2,10.7102581353693));
#232802=CARTESIAN_POINT('Ctrl Pts',(-1.97463432522597,15.2,10.7135930801896));
#232803=CARTESIAN_POINT('Ctrl Pts',(-1.97648193657408,15.2,10.7169380076933));
#232804=CARTESIAN_POINT('Ctrl Pts',(-1.97832954817392,15.2,10.7202829356526));
#232805=CARTESIAN_POINT('Ctrl Pts',(-1.98018992160868,15.2,10.7236378431383));
#232806=CARTESIAN_POINT('Ctrl Pts',(-1.98206307987825,15.2,10.7270025952668));
#232807=CARTESIAN_POINT('Ctrl Pts',(-1.98534110646718,15.2,10.7328909108039));
#232808=CARTESIAN_POINT('Ctrl Pts',(-1.98865828528117,15.2,10.7388093765999));
#232809=CARTESIAN_POINT('Ctrl Pts',(-1.99201473169475,15.2,10.7447572738942));
#232810=CARTESIAN_POINT('Ctrl Pts',(-1.99441219356806,15.2,10.7490057722262));
#232811=CARTESIAN_POINT('Ctrl Pts',(-1.99682969042726,15.2,10.7532692880193));
#232812=CARTESIAN_POINT('Ctrl Pts',(-1.99926725993951,15.2,10.7575475629487));
#232813=CARTESIAN_POINT('Ctrl Pts',(-2.00121731565559,15.2,10.7609701830787));
#232814=CARTESIAN_POINT('Ctrl Pts',(-2.00318021886519,15.2,10.7644022489491));
#232815=CARTESIAN_POINT('Ctrl Pts',(-2.00515598925969,15.2,10.767843629819));
#232816=CARTESIAN_POINT('Ctrl Pts',(-2.00762570211822,15.2,10.7721453556719));
#232817=CARTESIAN_POINT('Ctrl Pts',(-2.01011552044656,15.2,10.776461636477));
#232818=CARTESIAN_POINT('Ctrl Pts',(-2.01262548065595,15.2,10.7807922197416));
#232819=CARTESIAN_POINT('Ctrl Pts',(-2.01513544086535,15.2,10.7851228030062));
#232820=CARTESIAN_POINT('Ctrl Pts',(-2.01766554248254,15.2,10.7894676884955));
#232821=CARTESIAN_POINT('Ctrl Pts',(-2.02021582269191,15.2,10.7938266253018));
#232822=CARTESIAN_POINT('Ctrl Pts',(-2.02327615883198,15.2,10.7990573492793));
#232823=CARTESIAN_POINT('Ctrl Pts',(-2.02636555102808,15.2,10.8043083090051));
#232824=CARTESIAN_POINT('Ctrl Pts',(-2.02948406008016,15.2,10.8095790759794));
#232825=CARTESIAN_POINT('Ctrl Pts',(-2.03208281771799,15.2,10.8139713819509));
#232826=CARTESIAN_POINT('Ctrl Pts',(-2.0347017938533,15.2,10.8183774445831));
#232827=CARTESIAN_POINT('Ctrl Pts',(-2.03734102324024,15.2,10.8227970171725));
#232828=CARTESIAN_POINT('Ctrl Pts',(-2.03945240686485,15.2,10.8263326754368));
#232829=CARTESIAN_POINT('Ctrl Pts',(-2.04157675197055,15.2,10.8298769816141));
#232830=CARTESIAN_POINT('Ctrl Pts',(-2.04371407486613,15.2,10.8334298100308));
#232831=CARTESIAN_POINT('Ctrl Pts',(-2.04638572833999,15.2,10.8378708453097));
#232832=CARTESIAN_POINT('Ctrl Pts',(-2.04907765963643,15.2,10.8423252003443));
#232833=CARTESIAN_POINT('Ctrl Pts',(-2.05178989984644,15.2,10.8467926313176));
#232834=CARTESIAN_POINT('Ctrl Pts',(-2.05395969183708,15.2,10.8503665758041));
#232835=CARTESIAN_POINT('Ctrl Pts',(-2.05614248082365,15.2,10.8539488915136));
#232836=CARTESIAN_POINT('Ctrl Pts',(-2.05833828276517,15.2,10.8575394540142));
#232837=CARTESIAN_POINT('Ctrl Pts',(-2.06053408500586,15.2,10.8611300170039));
#232838=CARTESIAN_POINT('Ctrl Pts',(-2.0627428993325,15.2,10.8647288284339));
#232839=CARTESIAN_POINT('Ctrl Pts',(-2.06496474162162,15.2,10.868335766798));
#232840=CARTESIAN_POINT('Ctrl Pts',(-2.06718658360801,15.2,10.8719427046707));
#232841=CARTESIAN_POINT('Ctrl Pts',(-2.069421452576,15.2,10.8755577711895));
#232842=CARTESIAN_POINT('Ctrl Pts',(-2.07166936255802,15.2,10.8791808450038));
#232843=CARTESIAN_POINT('Ctrl Pts',(-2.07391727284633,15.2,10.8828039193119));
#232844=CARTESIAN_POINT('Ctrl Pts',(-2.07617822524971,15.2,10.8864350012722));
#232845=CARTESIAN_POINT('Ctrl Pts',(-2.07845223232172,15.2,10.8900739718197));
#232846=CARTESIAN_POINT('Ctrl Pts',(-2.08129474100681,15.2,10.8946226847561));
#232847=CARTESIAN_POINT('Ctrl Pts',(-2.08415764804215,15.2,10.8991837253138));
#232848=CARTESIAN_POINT('Ctrl Pts',(-2.08704097908548,15.2,10.9037568613565));
#232849=CARTESIAN_POINT('Ctrl Pts',(-2.08934764373158,15.2,10.9074153698915));
#232850=CARTESIAN_POINT('Ctrl Pts',(-2.09166738111486,15.2,10.9110816208727));
#232851=CARTESIAN_POINT('Ctrl Pts',(-2.09400020053442,15.2,10.914755496683));
#232852=CARTESIAN_POINT('Ctrl Pts',(-2.09633302027183,15.2,10.9184293729939));
#232853=CARTESIAN_POINT('Ctrl Pts',(-2.09867892545317,15.2,10.9221108747576));
#232854=CARTESIAN_POINT('Ctrl Pts',(-2.10103792586738,15.2,10.925799885977));
#232855=CARTESIAN_POINT('Ctrl Pts',(-2.10339692596018,15.2,10.9294888966937));
#232856=CARTESIAN_POINT('Ctrl Pts',(-2.1057690218732,15.2,10.9331854171922));
#232857=CARTESIAN_POINT('Ctrl Pts',(-2.10815422578847,15.2,10.9368893317222));
#232858=CARTESIAN_POINT('Ctrl Pts',(-2.11053943002873,15.2,10.940593246757));
#232859=CARTESIAN_POINT('Ctrl Pts',(-2.11293774265664,15.2,10.9443045566592));
#232860=CARTESIAN_POINT('Ctrl Pts',(-2.1153491729556,15.2,10.948023147029));
#232861=CARTESIAN_POINT('Ctrl Pts',(-2.11836346066501,15.2,10.952671384738));
#232862=CARTESIAN_POINT('Ctrl Pts',(-2.12139824801735,15.2,10.9573309978692));
#232863=CARTESIAN_POINT('Ctrl Pts',(-2.12445355337975,15.2,10.9620017665755));
#232864=CARTESIAN_POINT('Ctrl Pts',(-2.12689779746986,15.2,10.9657383812351));
#232865=CARTESIAN_POINT('Ctrl Pts',(-2.12935517517598,15.2,10.9694821344755));
#232866=CARTESIAN_POINT('Ctrl Pts',(-2.1318256938065,15.2,10.9732329156684));
#232867=CARTESIAN_POINT('Ctrl Pts',(-2.13367858286354,15.2,10.9760460016909));
#232868=CARTESIAN_POINT('Ctrl Pts',(-2.13553886482839,15.2,10.978863040638));
#232869=CARTESIAN_POINT('Ctrl Pts',(-2.13740654334285,15.2,10.98168398516));
#232870=CARTESIAN_POINT('Ctrl Pts',(-2.13927422219661,15.2,10.9845049301944));
#232871=CARTESIAN_POINT('Ctrl Pts',(-2.14114929790246,15.2,10.9873297811383));
#232872=CARTESIAN_POINT('Ctrl Pts',(-2.14303177467706,15.2,10.9901584916333));
#232873=CARTESIAN_POINT('Ctrl Pts',(-2.14554174313989,15.2,10.9939301047701));
#232874=CARTESIAN_POINT('Ctrl Pts',(-2.14806486711083,15.2,10.9977085785536));
#232875=CARTESIAN_POINT('Ctrl Pts',(-2.15060115824828,15.2,11.0014938025391));
#232876=CARTESIAN_POINT('Ctrl Pts',(-2.15250337668776,15.2,11.0043327206571));
#232877=CARTESIAN_POINT('Ctrl Pts',(-2.15441300006148,15.2,11.0071754366435));
#232878=CARTESIAN_POINT('Ctrl Pts',(-2.15633003357451,15.2,11.0100219037064));
#232879=CARTESIAN_POINT('Ctrl Pts',(-2.15888607849072,15.2,11.0138171934684));
#232880=CARTESIAN_POINT('Ctrl Pts',(-2.16145529675576,15.2,11.0176191503895));
#232881=CARTESIAN_POINT('Ctrl Pts',(-2.16403769495292,15.2,11.0214276693197));
#232882=CARTESIAN_POINT('Ctrl Pts',(-2.16597449342487,15.2,11.0242840582579));
#232883=CARTESIAN_POINT('Ctrl Pts',(-2.16791870613044,15.2,11.0271441369769));
#232884=CARTESIAN_POINT('Ctrl Pts',(-2.16987033702679,15.2,11.0300078600526));
#232885=CARTESIAN_POINT('Ctrl Pts',(-2.17182196792315,15.2,11.0328715831283));
#232886=CARTESIAN_POINT('Ctrl Pts',(-2.17378101556077,15.2,11.035738950872));
#232887=CARTESIAN_POINT('Ctrl Pts',(-2.17574748453989,15.2,11.038609917989));
#232888=CARTESIAN_POINT('Ctrl Pts',(-2.17771395351902,15.2,11.0414808851061));
#232889=CARTESIAN_POINT('Ctrl Pts',(-2.17968784329013,15.2,11.0443554523412));
#232890=CARTESIAN_POINT('Ctrl Pts',(-2.18166915725917,15.2,11.0472335729446));
#232891=CARTESIAN_POINT('Ctrl Pts',(-2.18365047122821,15.2,11.0501116935481));
#232892=CARTESIAN_POINT('Ctrl Pts',(-2.1856392083884,15.2,11.052993368893));
#232893=CARTESIAN_POINT('Ctrl Pts',(-2.18763537377317,15.2,11.0558785539126));
#232894=CARTESIAN_POINT('Ctrl Pts',(-2.18963153952058,15.2,11.0587637394565));
#232895=CARTESIAN_POINT('Ctrl Pts',(-2.19163513162849,15.2,11.0616524335097));
#232896=CARTESIAN_POINT('Ctrl Pts',(-2.19364615392175,15.2,11.0645445931388));
#232897=CARTESIAN_POINT('Ctrl Pts',(-2.19565717584967,15.2,11.0674367522425));
#232898=CARTESIAN_POINT('Ctrl Pts',(-2.1976756272969,15.2,11.0703323770043));
#232899=CARTESIAN_POINT('Ctrl Pts',(-2.19970151136704,15.2,11.0732314217942));
#232900=CARTESIAN_POINT('Ctrl Pts',(-2.20240269000454,15.2,11.0770968146719));
#232901=CARTESIAN_POINT('Ctrl Pts',(-2.20511708253712,15.2,11.0809682887116));
#232902=CARTESIAN_POINT('Ctrl Pts',(-2.20784469503548,15.2,11.0848457399497));
#232903=CARTESIAN_POINT('Ctrl Pts',(-2.20989040450217,15.2,11.0877538285104));
#232904=CARTESIAN_POINT('Ctrl Pts',(-2.21194354956001,15.2,11.0906652792209));
#232905=CARTESIAN_POINT('Ctrl Pts',(-2.21400413352581,15.2,11.0935800473646));
#232906=CARTESIAN_POINT('Ctrl Pts',(-2.21675157906309,15.2,11.0974664052425));
#232907=CARTESIAN_POINT('Ctrl Pts',(-2.21951224876549,15.2,11.1013586630542));
#232908=CARTESIAN_POINT('Ctrl Pts',(-2.22228614825,15.2,11.1052567162666));
#232909=CARTESIAN_POINT('Ctrl Pts',(-2.22436657267441,15.2,11.1081802559104));
#232910=CARTESIAN_POINT('Ctrl Pts',(-2.22645443836519,15.2,11.1111070565874));
#232911=CARTESIAN_POINT('Ctrl Pts',(-2.22854974828841,15.2,11.114037073689));
#232912=CARTESIAN_POINT('Ctrl Pts',(-2.23064505821163,15.2,11.1169670907906));
#232913=CARTESIAN_POINT('Ctrl Pts',(-2.23274781101391,15.2,11.1199003238756));
#232914=CARTESIAN_POINT('Ctrl Pts',(-2.23485801104179,15.2,11.1228367316652));
#232915=CARTESIAN_POINT('Ctrl Pts',(-2.23696821106968,15.2,11.1257731394548));
#232916=CARTESIAN_POINT('Ctrl Pts',(-2.23908585736497,15.2,11.1287127216825));
#232917=CARTESIAN_POINT('Ctrl Pts',(-2.24121095078674,15.2,11.1316554347835));
#232918=CARTESIAN_POINT('Ctrl Pts',(-2.2440444089398,15.2,11.1355790526078));
#232919=CARTESIAN_POINT('Ctrl Pts',(-2.24689110731358,15.2,11.1395082366661));
#232920=CARTESIAN_POINT('Ctrl Pts',(-2.249751051525,15.2,11.1434428864916));
#232921=CARTESIAN_POINT('Ctrl Pts',(-2.25189600948873,15.2,11.1463938735927));
#232922=CARTESIAN_POINT('Ctrl Pts',(-2.2540484177605,15.2,11.1493479356187));
#232923=CARTESIAN_POINT('Ctrl Pts',(-2.2562082777647,15.2,11.1523050297194));
#232924=CARTESIAN_POINT('Ctrl Pts',(-2.25836813776891,15.2,11.15526212382));
#232925=CARTESIAN_POINT('Ctrl Pts',(-2.2605354499839,15.2,11.15822224942));
#232926=CARTESIAN_POINT('Ctrl Pts',(-2.26271021605431,15.2,11.1611853661267));
#232927=CARTESIAN_POINT('Ctrl Pts',(-2.26633482630336,15.2,11.1661238941506));
#232928=CARTESIAN_POINT('Ctrl Pts',(-2.26998014113926,15.2,11.1710707268431));
#232929=CARTESIAN_POINT('Ctrl Pts',(-2.27364616627703,15.2,11.176025671426));
#232930=CARTESIAN_POINT('Ctrl Pts',(-2.27657898654709,15.2,11.1799896273083));
#232931=CARTESIAN_POINT('Ctrl Pts',(-2.2795250626827,15.2,11.183958775333));
#232932=CARTESIAN_POINT('Ctrl Pts',(-2.28248439623372,15.2,11.1879330190499));
#232933=CARTESIAN_POINT('Ctrl Pts',(-2.28470389619538,15.2,11.1909137015668));
#232934=CARTESIAN_POINT('Ctrl Pts',(-2.28693085412303,15.2,11.1938972487643));
#232935=CARTESIAN_POINT('Ctrl Pts',(-2.28916527101038,15.2,11.1968836202944));
#232936=CARTESIAN_POINT('Ctrl Pts',(-2.29139968789772,15.2,11.1998699918244));
#232937=CARTESIAN_POINT('Ctrl Pts',(-2.29364156283617,15.2,11.2028591863924));
#232938=CARTESIAN_POINT('Ctrl Pts',(-2.29589089826463,15.2,11.2058511625056));
#232939=CARTESIAN_POINT('Ctrl Pts',(-2.29889001244167,15.2,11.2098404643522));
#232940=CARTESIAN_POINT('Ctrl Pts',(-2.30190238960067,15.2,11.213834708802));
#232941=CARTESIAN_POINT('Ctrl Pts',(-2.30492802921138,15.2,11.2178338113538));
#232942=CARTESIAN_POINT('Ctrl Pts',(-2.30719725871329,15.2,11.2208331379952));
#232943=CARTESIAN_POINT('Ctrl Pts',(-2.30947394984811,15.2,11.2238351967865));
#232944=CARTESIAN_POINT('Ctrl Pts',(-2.31175810276576,15.2,11.2268399458025));
#232945=CARTESIAN_POINT('Ctrl Pts',(-2.31404225568342,15.2,11.2298446948186));
#232946=CARTESIAN_POINT('Ctrl Pts',(-2.31633387052517,15.2,11.2328521333317));
#232947=CARTESIAN_POINT('Ctrl Pts',(-2.31863294753543,15.2,11.2358622104444));
#232948=CARTESIAN_POINT('Ctrl Pts',(-2.3209320245457,15.2,11.238872287557));
#232949=CARTESIAN_POINT('Ctrl Pts',(-2.32323856528819,15.2,11.2418850040765));
#232950=CARTESIAN_POINT('Ctrl Pts',(-2.32555256875624,15.2,11.2449003215639));
#232951=CARTESIAN_POINT('Ctrl Pts',(-2.32940924134313,15.2,11.2499258508922));
#232952=CARTESIAN_POINT('Ctrl Pts',(-2.33328664381693,15.2,11.2549585979013));
#232953=CARTESIAN_POINT('Ctrl Pts',(-2.33718477800005,15.2,11.259998549));
#232954=CARTESIAN_POINT('Ctrl Pts',(-1.76496130700006,12.2,10.22377311));
#232955=CARTESIAN_POINT('Ctrl Pts',(-1.76541543493207,12.2,10.2255010873779));
#232956=CARTESIAN_POINT('Ctrl Pts',(-1.76588926591707,12.2,10.2272829938834));
#232957=CARTESIAN_POINT('Ctrl Pts',(-1.76638321147092,12.2,10.2291177140323));
#232958=CARTESIAN_POINT('Ctrl Pts',(-1.76687953907992,12.2,10.2309612821291));
#232959=CARTESIAN_POINT('Ctrl Pts',(-1.76739616286972,12.2,10.2328581799819));
#232960=CARTESIAN_POINT('Ctrl Pts',(-1.76793345451038,12.2,10.2348073231886));
#232961=CARTESIAN_POINT('Ctrl Pts',(-1.76847074610224,12.2,10.2367564662182));
#232962=CARTESIAN_POINT('Ctrl Pts',(-1.76902870497939,12.2,10.2387578539245));
#232963=CARTESIAN_POINT('Ctrl Pts',(-1.76960768654168,12.2,10.2408104330166));
#232964=CARTESIAN_POINT('Ctrl Pts',(-1.77018666810398,12.2,10.2428630121086));
#232965=CARTESIAN_POINT('Ctrl Pts',(-1.77078667246607,12.2,10.2449667819402));
#232966=CARTESIAN_POINT('Ctrl Pts',(-1.77140804397329,12.2,10.24712072005));
#232967=CARTESIAN_POINT('Ctrl Pts',(-1.77202941553697,12.2,10.2492746583554));
#232968=CARTESIAN_POINT('Ctrl Pts',(-1.77267215276809,12.2,10.2514787598444));
#232969=CARTESIAN_POINT('Ctrl Pts',(-1.77333658730578,12.2,10.2537320332205));
#232970=CARTESIAN_POINT('Ctrl Pts',(-1.77400102178312,12.2,10.255985306392));
#232971=CARTESIAN_POINT('Ctrl Pts',(-1.77468715486446,12.2,10.2582877466256));
#232972=CARTESIAN_POINT('Ctrl Pts',(-1.77539530325867,12.2,10.260638386051));
#232973=CARTESIAN_POINT('Ctrl Pts',(-1.77610345165288,12.2,10.2629890254764));
#232974=CARTESIAN_POINT('Ctrl Pts',(-1.77683361717075,12.2,10.2653878615328));
#232975=CARTESIAN_POINT('Ctrl Pts',(-1.77758610564243,12.2,10.2678339508585));
#232976=CARTESIAN_POINT('Ctrl Pts',(-1.77833859418247,12.2,10.2702800404063));
#232977=CARTESIAN_POINT('Ctrl Pts',(-1.77911340904195,12.2,10.2727733804935));
#232978=CARTESIAN_POINT('Ctrl Pts',(-1.77991084258694,12.2,10.2753130495517));
#232979=CARTESIAN_POINT('Ctrl Pts',(-1.7807082760595,12.2,10.2778527183792));
#232980=CARTESIAN_POINT('Ctrl Pts',(-1.78152833193401,12.2,10.2804387173121));
#232981=CARTESIAN_POINT('Ctrl Pts',(-1.78237129432105,12.2,10.2830701451352));
#232982=CARTESIAN_POINT('Ctrl Pts',(-1.7832142567081,12.2,10.2857015729583));
#232983=CARTESIAN_POINT('Ctrl Pts',(-1.78408012798497,12.2,10.2883784311276));
#232984=CARTESIAN_POINT('Ctrl Pts',(-1.78496918228499,12.2,10.2910998401101));
#232985=CARTESIAN_POINT('Ctrl Pts',(-1.78585823658502,12.2,10.2938212490926));
#232986=CARTESIAN_POINT('Ctrl Pts',(-1.78677047506695,12.2,10.2965872102404));
#232987=CARTESIAN_POINT('Ctrl Pts',(-1.7877061643647,12.2,10.2993968662187));
#232988=CARTESIAN_POINT('Ctrl Pts',(-1.7887978019354,12.2,10.3026747983635));
#232989=CARTESIAN_POINT('Ctrl Pts',(-1.78992136090724,12.2,10.3060122026356));
#232990=CARTESIAN_POINT('Ctrl Pts',(-1.79107724768775,12.2,10.3094077546164));
#232991=CARTESIAN_POINT('Ctrl Pts',(-1.79223313446825,12.2,10.3128033065971));
#232992=CARTESIAN_POINT('Ctrl Pts',(-1.79342135008691,12.2,10.3162570016962));
#232993=CARTESIAN_POINT('Ctrl Pts',(-1.79464228456549,12.2,10.3197675544474));
#232994=CARTESIAN_POINT('Ctrl Pts',(-1.79568879977852,12.2,10.3227765995066));
#232995=CARTESIAN_POINT('Ctrl Pts',(-1.79675935631462,12.2,10.325827414804));
#232996=CARTESIAN_POINT('Ctrl Pts',(-1.79785418744044,12.2,10.3289192081066));
#232997=CARTESIAN_POINT('Ctrl Pts',(-1.79894901866572,12.2,10.3320110016899));
#232998=CARTESIAN_POINT('Ctrl Pts',(-1.80006812791901,12.2,10.3351437736868));
#232999=CARTESIAN_POINT('Ctrl Pts',(-1.80121174389967,12.2,10.3383167463624));
#233000=CARTESIAN_POINT('Ctrl Pts',(-1.80235535977646,12.2,10.3414897187499));
#233001=CARTESIAN_POINT('Ctrl Pts',(-1.80352348028237,12.2,10.3447028939104));
#233002=CARTESIAN_POINT('Ctrl Pts',(-1.80471633032346,12.2,10.3479555094607));
#233003=CARTESIAN_POINT('Ctrl Pts',(-1.80590918036456,12.2,10.351208125011));
#233004=CARTESIAN_POINT('Ctrl Pts',(-1.80712675935363,12.2,10.3545001845413));
#233005=CARTESIAN_POINT('Ctrl Pts',(-1.80836928039073,12.2,10.3578309400852));
#233006=CARTESIAN_POINT('Ctrl Pts',(-1.80961180142783,12.2,10.3611616956292));
#233007=CARTESIAN_POINT('Ctrl Pts',(-1.81087926574946,12.2,10.3645311508882));
#233008=CARTESIAN_POINT('Ctrl Pts',(-1.81217187961746,12.2,10.3679385744285));
#233009=CARTESIAN_POINT('Ctrl Pts',(-1.81346449360286,12.2,10.3713459982783));
#233010=CARTESIAN_POINT('Ctrl Pts',(-1.81478225641568,12.2,10.3747913937401));
#233011=CARTESIAN_POINT('Ctrl Pts',(-1.81612537032332,12.2,10.3782740446815));
#233012=CARTESIAN_POINT('Ctrl Pts',(-1.81746848410895,12.2,10.3817566953066));
#233013=CARTESIAN_POINT('Ctrl Pts',(-1.81883694824376,12.2,10.3852766023865));
#233014=CARTESIAN_POINT('Ctrl Pts',(-1.82023095503271,12.2,10.3888330670233));
#233015=CARTESIAN_POINT('Ctrl Pts',(-1.82162496182165,12.2,10.3923895316601));
#233016=CARTESIAN_POINT('Ctrl Pts',(-1.8230445125134,12.2,10.3959825521803));
#233017=CARTESIAN_POINT('Ctrl Pts',(-1.82448979329248,12.2,10.3996114457961));
#233018=CARTESIAN_POINT('Ctrl Pts',(-1.82593507420284,12.2,10.4032403397414));
#233019=CARTESIAN_POINT('Ctrl Pts',(-1.82740608602869,12.2,10.4069051052444));
#233020=CARTESIAN_POINT('Ctrl Pts',(-1.82890300710321,12.2,10.4106050695496));
#233021=CARTESIAN_POINT('Ctrl Pts',(-1.83015044126398,12.2,10.4136883729692));
#233022=CARTESIAN_POINT('Ctrl Pts',(-1.83141587118312,12.2,10.4167961221577));
#233023=CARTESIAN_POINT('Ctrl Pts',(-1.83269939368457,12.2,10.4199279321596));
#233024=CARTESIAN_POINT('Ctrl Pts',(-1.83398291618601,12.2,10.4230597421614));
#233025=CARTESIAN_POINT('Ctrl Pts',(-1.83528453451561,12.2,10.4262156139472));
#233026=CARTESIAN_POINT('Ctrl Pts',(-1.83660434590599,12.2,10.4293951714492));
#233027=CARTESIAN_POINT('Ctrl Pts',(-1.83792415715251,12.2,10.4325747286046));
#233028=CARTESIAN_POINT('Ctrl Pts',(-1.83926216110527,12.2,10.4357779724537));
#233029=CARTESIAN_POINT('Ctrl Pts',(-1.84061845408095,12.2,10.4390045311279));
#233030=CARTESIAN_POINT('Ctrl Pts',(-1.84197474720446,12.2,10.4422310901538));
#233031=CARTESIAN_POINT('Ctrl Pts',(-1.84334932745266,12.2,10.4454809633182));
#233032=CARTESIAN_POINT('Ctrl Pts',(-1.84474229203447,12.2,10.4487537867885));
#233033=CARTESIAN_POINT('Ctrl Pts',(-1.84613525661629,12.2,10.4520266102588));
#233034=CARTESIAN_POINT('Ctrl Pts',(-1.8475466010084,12.2,10.4553223855673));
#233035=CARTESIAN_POINT('Ctrl Pts',(-1.84897641830076,12.2,10.4586407501065));
#233036=CARTESIAN_POINT('Ctrl Pts',(-1.85069219914511,12.2,10.4626227877705));
#233037=CARTESIAN_POINT('Ctrl Pts',(-1.85243457977794,12.2,10.466637356885));
#233038=CARTESIAN_POINT('Ctrl Pts',(-1.85420371070952,12.2,10.470683844441));
#233039=CARTESIAN_POINT('Ctrl Pts',(-1.85567798640548,12.2,10.4740559172206));
#233040=CARTESIAN_POINT('Ctrl Pts',(-1.85717084019619,12.2,10.4774501577616));
#233041=CARTESIAN_POINT('Ctrl Pts',(-1.85868235415605,12.2,10.4808662154718));
#233042=CARTESIAN_POINT('Ctrl Pts',(-1.86019386795117,12.2,10.4842822728095));
#233043=CARTESIAN_POINT('Ctrl Pts',(-1.86172404345668,12.2,10.4877201488652));
#233044=CARTESIAN_POINT('Ctrl Pts',(-1.86327296377242,12.2,10.4911795010558));
#233045=CARTESIAN_POINT('Ctrl Pts',(-1.86482188425699,12.2,10.4946388536235));
#233046=CARTESIAN_POINT('Ctrl Pts',(-1.86638954814405,12.2,10.4981196810547));
#233047=CARTESIAN_POINT('Ctrl Pts',(-1.86797603605917,12.2,10.5016216455669));
#233048=CARTESIAN_POINT('Ctrl Pts',(-1.86956252397429,12.2,10.505123610079));
#233049=CARTESIAN_POINT('Ctrl Pts',(-1.87116783398727,12.2,10.5086467122575));
#233050=CARTESIAN_POINT('Ctrl Pts',(-1.87279204705319,12.2,10.5121906186136));
#233051=CARTESIAN_POINT('Ctrl Pts',(-1.87441626011912,12.2,10.5157345249697));
#233052=CARTESIAN_POINT('Ctrl Pts',(-1.87605937489797,12.2,10.5192992351444));
#233053=CARTESIAN_POINT('Ctrl Pts',(-1.87772146538309,12.2,10.5228844204906));
#233054=CARTESIAN_POINT('Ctrl Pts',(-1.87938355586821,12.2,10.5264696058367));
#233055=CARTESIAN_POINT('Ctrl Pts',(-1.8810646226677,12.2,10.5300752665917));
#233056=CARTESIAN_POINT('Ctrl Pts',(-1.88276473988894,12.2,10.5337010777713));
#233057=CARTESIAN_POINT('Ctrl Pts',(-1.88446485711018,12.2,10.5373268889508));
#233058=CARTESIAN_POINT('Ctrl Pts',(-1.88618402469853,12.2,10.5409728519169));
#233059=CARTESIAN_POINT('Ctrl Pts',(-1.88792231191978,12.2,10.544638645527));
#233060=CARTESIAN_POINT('Ctrl Pts',(-1.88966059914102,12.2,10.5483044391371));
#233061=CARTESIAN_POINT('Ctrl Pts',(-1.89141800780214,12.2,10.5519900629089));
#233062=CARTESIAN_POINT('Ctrl Pts',(-1.89319460649071,12.2,10.5556952024396));
#233063=CARTESIAN_POINT('Ctrl Pts',(-1.89497120517928,12.2,10.5594003419703));
#233064=CARTESIAN_POINT('Ctrl Pts',(-1.89676699360556,12.2,10.5631249979611));
#233065=CARTESIAN_POINT('Ctrl Pts',(-1.89858203825834,12.2,10.5668688560166));
#233066=CARTESIAN_POINT('Ctrl Pts',(-1.9000340740597,12.2,10.5698639426243));
#233067=CARTESIAN_POINT('Ctrl Pts',(-1.90149843394584,12.2,10.5728713194945));
#233068=CARTESIAN_POINT('Ctrl Pts',(-1.90297515108312,12.2,10.5758908299936));
#233069=CARTESIAN_POINT('Ctrl Pts',(-1.90445186801919,12.2,10.5789103400813));
#233070=CARTESIAN_POINT('Ctrl Pts',(-1.90594094191218,12.2,10.5819419825496));
#233071=CARTESIAN_POINT('Ctrl Pts',(-1.90744240674066,12.2,10.5849856019812));
#233072=CARTESIAN_POINT('Ctrl Pts',(-1.90894387177371,12.2,10.5880292218275));
#233073=CARTESIAN_POINT('Ctrl Pts',(-1.91045772694566,12.2,10.5910848193081));
#233074=CARTESIAN_POINT('Ctrl Pts',(-1.9119840033079,12.2,10.5941522379765));
#233075=CARTESIAN_POINT('Ctrl Pts',(-1.91351027946217,12.2,10.5972196562269));
#233076=CARTESIAN_POINT('Ctrl Pts',(-1.91504897688702,12.2,10.6002988976035));
#233077=CARTESIAN_POINT('Ctrl Pts',(-1.91660012714832,12.2,10.603389807739));
#233078=CARTESIAN_POINT('Ctrl Pts',(-1.91815127762096,12.2,10.6064807182957));
#233079=CARTESIAN_POINT('Ctrl Pts',(-1.91971488142971,12.2,10.6095832976644));
#233080=CARTESIAN_POINT('Ctrl Pts',(-1.92129096726211,12.2,10.6126973964352));
#233081=CARTESIAN_POINT('Ctrl Pts',(-1.92286705287978,12.2,10.6158114947817));
#233082=CARTESIAN_POINT('Ctrl Pts',(-1.9244556212815,12.2,10.6189371113063));
#233083=CARTESIAN_POINT('Ctrl Pts',(-1.92605670209424,12.2,10.6220740954936));
#233084=CARTESIAN_POINT('Ctrl Pts',(-1.92765778312512,12.2,10.6252110801083));
#233085=CARTESIAN_POINT('Ctrl Pts',(-1.92927137668249,12.2,10.6283594320215));
#233086=CARTESIAN_POINT('Ctrl Pts',(-1.93089750988305,12.2,10.63151900525));
#233087=CARTESIAN_POINT('Ctrl Pts',(-1.93252364286205,12.2,10.634678578048));
#233088=CARTESIAN_POINT('Ctrl Pts',(-1.93416231850852,12.2,10.6378493704821));
#233089=CARTESIAN_POINT('Ctrl Pts',(-1.93581356201047,12.2,10.6410312355466));
#233090=CARTESIAN_POINT('Ctrl Pts',(-1.93829042760087,12.2,10.6458040337937));
#233091=CARTESIAN_POINT('Ctrl Pts',(-1.94079557203615,12.2,10.6506017454861));
#233092=CARTESIAN_POINT('Ctrl Pts',(-1.9433290895095,12.2,10.6554238815006));
#233093=CARTESIAN_POINT('Ctrl Pts',(-1.94501810092827,12.2,10.6586386384055));
#233094=CARTESIAN_POINT('Ctrl Pts',(-1.94671972068151,12.2,10.6618642508535));
#233095=CARTESIAN_POINT('Ctrl Pts',(-1.94843397681832,12.2,10.6651005749771));
#233096=CARTESIAN_POINT('Ctrl Pts',(-1.95014823318869,12.2,10.6683368995417));
#233097=CARTESIAN_POINT('Ctrl Pts',(-1.95187512535022,12.2,10.6715839345065));
#233098=CARTESIAN_POINT('Ctrl Pts',(-1.9536146784775,12.2,10.674841540681));
#233099=CARTESIAN_POINT('Ctrl Pts',(-1.95535423136776,12.2,10.6780991464118));
#233100=CARTESIAN_POINT('Ctrl Pts',(-1.95710644619818,12.2,10.6813673210785));
#233101=CARTESIAN_POINT('Ctrl Pts',(-1.95887134633085,12.2,10.6846459246987));
#233102=CARTESIAN_POINT('Ctrl Pts',(-1.96107747167705,12.2,10.688744179559));
#233103=CARTESIAN_POINT('Ctrl Pts',(-1.96330341898762,12.2,10.6928587300085));
#233104=CARTESIAN_POINT('Ctrl Pts',(-1.96554923586158,12.2,10.6969893024382));
#233105=CARTESIAN_POINT('Ctrl Pts',(-1.96734588945867,12.2,10.7002937605621));
#233106=CARTESIAN_POINT('Ctrl Pts',(-1.96915525932304,12.2,10.7036084741259));
#233107=CARTESIAN_POINT('Ctrl Pts',(-1.97097736851447,12.2,10.7069333049741));
#233108=CARTESIAN_POINT('Ctrl Pts',(-1.97279947745765,12.2,10.7102581353693));
#233109=CARTESIAN_POINT('Ctrl Pts',(-1.97463432522597,12.2,10.7135930801896));
#233110=CARTESIAN_POINT('Ctrl Pts',(-1.97648193657408,12.2,10.7169380076933));
#233111=CARTESIAN_POINT('Ctrl Pts',(-1.97832954817392,12.2,10.7202829356526));
#233112=CARTESIAN_POINT('Ctrl Pts',(-1.98018992160868,12.2,10.7236378431383));
#233113=CARTESIAN_POINT('Ctrl Pts',(-1.98206307987825,12.2,10.7270025952668));
#233114=CARTESIAN_POINT('Ctrl Pts',(-1.98393623789261,12.2,10.7303673469368));
#233115=CARTESIAN_POINT('Ctrl Pts',(-1.9858221802277,12.2,10.7337419437146));
#233116=CARTESIAN_POINT('Ctrl Pts',(-1.98772092899955,12.2,10.7371262515506));
#233117=CARTESIAN_POINT('Ctrl Pts',(-1.98961967803012,12.2,10.7405105598477));
#233118=CARTESIAN_POINT('Ctrl Pts',(-1.99153123199617,12.2,10.7439045773672));
#233119=CARTESIAN_POINT('Ctrl Pts',(-1.99345561365745,12.2,10.7473081740533));
#233120=CARTESIAN_POINT('Ctrl Pts',(-1.99537999505653,12.2,10.7507117702757));
#233121=CARTESIAN_POINT('Ctrl Pts',(-1.99731720448912,12.2,10.754124943285));
#233122=CARTESIAN_POINT('Ctrl Pts',(-1.99926725993951,12.2,10.7575475629487));
#233123=CARTESIAN_POINT('Ctrl Pts',(-2.00121731565559,12.2,10.7609701830787));
#233124=CARTESIAN_POINT('Ctrl Pts',(-2.0031802188652,12.2,10.7644022489491));
#233125=CARTESIAN_POINT('Ctrl Pts',(-2.00515598925969,12.2,10.767843629819));
#233126=CARTESIAN_POINT('Ctrl Pts',(-2.00713175938499,12.2,10.77128501022));
#233127=CARTESIAN_POINT('Ctrl Pts',(-2.00912039674324,12.2,10.7747357063541));
#233128=CARTESIAN_POINT('Ctrl Pts',(-2.01112192068943,12.2,10.7781955874593));
#233129=CARTESIAN_POINT('Ctrl Pts',(-2.01312344490833,12.2,10.7816554690358));
#233130=CARTESIAN_POINT('Ctrl Pts',(-2.01513785459787,12.2,10.785124536441));
#233131=CARTESIAN_POINT('Ctrl Pts',(-2.01716516954166,12.2,10.7886026612416));
#233132=CARTESIAN_POINT('Ctrl Pts',(-2.01919248448546,12.2,10.7920807860422));
#233133=CARTESIAN_POINT('Ctrl Pts',(-2.0212327038975,12.2,10.7955679675079));
#233134=CARTESIAN_POINT('Ctrl Pts',(-2.02328584684403,12.2,10.7990640795882));
#233135=CARTESIAN_POINT('Ctrl Pts',(-2.02533898951083,12.2,10.8025601911922));
#233136=CARTESIAN_POINT('Ctrl Pts',(-2.02740505413986,12.2,10.8060652314895));
#233137=CARTESIAN_POINT('Ctrl Pts',(-2.02948406008016,12.2,10.8095790759794));
#233138=CARTESIAN_POINT('Ctrl Pts',(-2.03156306630373,12.2,10.8130929209481));
#233139=CARTESIAN_POINT('Ctrl Pts',(-2.03365501234282,12.2,10.8166155704955));
#233140=CARTESIAN_POINT('Ctrl Pts',(-2.03575991606385,12.2,10.8201468975874));
#233141=CARTESIAN_POINT('Ctrl Pts',(-2.03786481949808,12.2,10.8236782241982));
#233142=CARTESIAN_POINT('Ctrl Pts',(-2.03998268064264,12.2,10.8272182290006));
#233143=CARTESIAN_POINT('Ctrl Pts',(-2.04211351530094,12.2,10.8307667880433));
#233144=CARTESIAN_POINT('Ctrl Pts',(-2.04424435024956,12.2,10.8343153475695));
#233145=CARTESIAN_POINT('Ctrl Pts',(-2.04638815826361,12.2,10.8378724610828));
#233146=CARTESIAN_POINT('Ctrl Pts',(-2.04854495715978,12.2,10.8414380059998));
#233147=CARTESIAN_POINT('Ctrl Pts',(-2.05070175576209,12.2,10.8450035504311));
#233148=CARTESIAN_POINT('Ctrl Pts',(-2.05287154411498,12.2,10.8485775250976));
#233149=CARTESIAN_POINT('Ctrl Pts',(-2.05505433693334,12.2,10.8521598097052));
#233150=CARTESIAN_POINT('Ctrl Pts',(-2.05723713004911,12.2,10.8557420948009));
#233151=CARTESIAN_POINT('Ctrl Pts',(-2.05943292863447,12.2,10.8593326877781));
#233152=CARTESIAN_POINT('Ctrl Pts',(-2.06164174692237,12.2,10.8629314692526));
#233153=CARTESIAN_POINT('Ctrl Pts',(-2.06385056490931,12.2,10.8665302502367));
#233154=CARTESIAN_POINT('Ctrl Pts',(-2.06607240380753,12.2,10.8701372180303));
#233155=CARTESIAN_POINT('Ctrl Pts',(-2.06830727640128,12.2,10.8737522539006));
#233156=CARTESIAN_POINT('Ctrl Pts',(-2.07054214929953,12.2,10.8773672902634));
#233157=CARTESIAN_POINT('Ctrl Pts',(-2.07279005567357,12.2,10.8809903947575));
#233158=CARTESIAN_POINT('Ctrl Pts',(-2.07505101125155,12.2,10.8846214470274));
#233159=CARTESIAN_POINT('Ctrl Pts',(-2.07787720556999,12.2,10.8891602621175));
#233160=CARTESIAN_POINT('Ctrl Pts',(-2.08072378741435,12.2,10.893711495909));
#233161=CARTESIAN_POINT('Ctrl Pts',(-2.08359078338763,12.2,10.8982749185485));
#233162=CARTESIAN_POINT('Ctrl Pts',(-2.08588437997875,12.2,10.9019256563616));
#233163=CARTESIAN_POINT('Ctrl Pts',(-2.0881910411978,12.2,10.9055841939038));
#233164=CARTESIAN_POINT('Ctrl Pts',(-2.0905107810624,12.2,10.9092504156589));
#233165=CARTESIAN_POINT('Ctrl Pts',(-2.09283052124306,12.2,10.9129166379135));
#233166=CARTESIAN_POINT('Ctrl Pts',(-2.09516333766861,12.2,10.9165905427712));
#233167=CARTESIAN_POINT('Ctrl Pts',(-2.09750924525161,12.2,10.9202720157108));
#233168=CARTESIAN_POINT('Ctrl Pts',(-2.09985515251497,12.2,10.9239534881488));
#233169=CARTESIAN_POINT('Ctrl Pts',(-2.10221414967688,12.2,10.9276425278763));
#233170=CARTESIAN_POINT('Ctrl Pts',(-2.1045862488705,12.2,10.9313390191289));
#233171=CARTESIAN_POINT('Ctrl Pts',(-2.10695834838733,12.2,10.9350355108852));
#233172=CARTESIAN_POINT('Ctrl Pts',(-2.10934354957487,12.2,10.9387394544005));
#233173=CARTESIAN_POINT('Ctrl Pts',(-2.11174186448333,12.2,10.9424507359916));
#233174=CARTESIAN_POINT('Ctrl Pts',(-2.11414017939179,12.2,10.9461620175827));
#233175=CARTESIAN_POINT('Ctrl Pts',(-2.11655160631296,12.2,10.9498806364804));
#233176=CARTESIAN_POINT('Ctrl Pts',(-2.11897615911309,12.2,10.9536064788508));
#233177=CARTESIAN_POINT('Ctrl Pts',(-2.12079457354802,12.2,10.9564008603748));
#233178=CARTESIAN_POINT('Ctrl Pts',(-2.12262037022891,12.2,10.9591993054536));
#233179=CARTESIAN_POINT('Ctrl Pts',(-2.12445355337975,12.2,10.9620017665755));
#233180=CARTESIAN_POINT('Ctrl Pts',(-2.12689779746986,12.2,10.9657383812351));
#233181=CARTESIAN_POINT('Ctrl Pts',(-2.12935517517598,12.2,10.9694821344755));
#233182=CARTESIAN_POINT('Ctrl Pts',(-2.1318256938065,12.2,10.9732329156684));
#233183=CARTESIAN_POINT('Ctrl Pts',(-2.13367858286354,12.2,10.9760460016909));
#233184=CARTESIAN_POINT('Ctrl Pts',(-2.13553886482839,12.2,10.978863040638));
#233185=CARTESIAN_POINT('Ctrl Pts',(-2.13740654334285,12.2,10.98168398516));
#233186=CARTESIAN_POINT('Ctrl Pts',(-2.13927422219661,12.2,10.9845049301944));
#233187=CARTESIAN_POINT('Ctrl Pts',(-2.14114929790246,12.2,10.9873297811383));
#233188=CARTESIAN_POINT('Ctrl Pts',(-2.14303177467706,12.2,10.9901584916333));
#233189=CARTESIAN_POINT('Ctrl Pts',(-2.14554174313989,12.2,10.9939301047701));
#233190=CARTESIAN_POINT('Ctrl Pts',(-2.14806486711083,12.2,10.9977085785536));
#233191=CARTESIAN_POINT('Ctrl Pts',(-2.15060115824828,12.2,11.0014938025391));
#233192=CARTESIAN_POINT('Ctrl Pts',(-2.15250337668776,12.2,11.0043327206571));
#233193=CARTESIAN_POINT('Ctrl Pts',(-2.15441300006148,12.2,11.0071754366435));
#233194=CARTESIAN_POINT('Ctrl Pts',(-2.1563300335745,12.2,11.0100219037064));
#233195=CARTESIAN_POINT('Ctrl Pts',(-2.15824706708753,12.2,11.0128683707693));
#233196=CARTESIAN_POINT('Ctrl Pts',(-2.16017151101673,12.2,11.015718588232));
#233197=CARTESIAN_POINT('Ctrl Pts',(-2.16210336707053,12.2,11.0185725113361));
#233198=CARTESIAN_POINT('Ctrl Pts',(-2.16403522347529,12.2,11.0214264349587));
#233199=CARTESIAN_POINT('Ctrl Pts',(-2.16597449255711,12.2,11.0242840647907));
#233200=CARTESIAN_POINT('Ctrl Pts',(-2.16792117888273,12.2,11.0271453538321));
#233201=CARTESIAN_POINT('Ctrl Pts',(-2.16986786485471,12.2,11.0300066423537));
#233202=CARTESIAN_POINT('Ctrl Pts',(-2.17182196726869,12.2,11.0328715901655));
#233203=CARTESIAN_POINT('Ctrl Pts',(-2.17378348933792,12.2,11.03574015283));
#233204=CARTESIAN_POINT('Ctrl Pts',(-2.17639885197811,12.2,11.0395649028756));
#233205=CARTESIAN_POINT('Ctrl Pts',(-2.17902740542042,12.2,11.043396078981));
#233206=CARTESIAN_POINT('Ctrl Pts',(-2.18166915725917,12.2,11.0472335729446));
#233207=CARTESIAN_POINT('Ctrl Pts',(-2.18365047122821,12.2,11.0501116935481));
#233208=CARTESIAN_POINT('Ctrl Pts',(-2.18563920838841,12.2,11.052993368893));
#233209=CARTESIAN_POINT('Ctrl Pts',(-2.18763537377318,12.2,11.0558785539127));
#233210=CARTESIAN_POINT('Ctrl Pts',(-2.18963153952059,12.2,11.0587637394565));
#233211=CARTESIAN_POINT('Ctrl Pts',(-2.19163513162849,12.2,11.0616524335097));
#233212=CARTESIAN_POINT('Ctrl Pts',(-2.19364615392175,12.2,11.0645445931388));
#233213=CARTESIAN_POINT('Ctrl Pts',(-2.19565717584967,12.2,11.0674367522425));
#233214=CARTESIAN_POINT('Ctrl Pts',(-2.1976756272969,12.2,11.0703323770043));
#233215=CARTESIAN_POINT('Ctrl Pts',(-2.19970151136704,12.2,11.0732314217942));
#233216=CARTESIAN_POINT('Ctrl Pts',(-2.20240269000454,12.2,11.0770968146719));
#233217=CARTESIAN_POINT('Ctrl Pts',(-2.20511708253712,12.2,11.0809682887116));
#233218=CARTESIAN_POINT('Ctrl Pts',(-2.20784469503548,12.2,11.0848457399497));
#233219=CARTESIAN_POINT('Ctrl Pts',(-2.20989040450216,12.2,11.0877538285104));
#233220=CARTESIAN_POINT('Ctrl Pts',(-2.21194354956001,12.2,11.0906652792209));
#233221=CARTESIAN_POINT('Ctrl Pts',(-2.21400413352581,12.2,11.0935800473646));
#233222=CARTESIAN_POINT('Ctrl Pts',(-2.21606471786595,12.2,11.0964948160377));
#233223=CARTESIAN_POINT('Ctrl Pts',(-2.21813274084982,12.2,11.0994129032952));
#233224=CARTESIAN_POINT('Ctrl Pts',(-2.22020820469413,12.2,11.1023342653868));
#233225=CARTESIAN_POINT('Ctrl Pts',(-2.22228366816139,12.2,11.1052556269478));
#233226=CARTESIAN_POINT('Ctrl Pts',(-2.2243665724866,12.2,11.1081802628086));
#233227=CARTESIAN_POINT('Ctrl Pts',(-2.22645691995298,12.2,11.1111081308275));
#233228=CARTESIAN_POINT('Ctrl Pts',(-2.22854726741935,12.2,11.1140359988464));
#233229=CARTESIAN_POINT('Ctrl Pts',(-2.23064505821883,12.2,11.1169670976126));
#233230=CARTESIAN_POINT('Ctrl Pts',(-2.23275029377692,12.2,11.1199013842693));
#233231=CARTESIAN_POINT('Ctrl Pts',(-2.23555727439356,12.2,11.1238137663006));
#233232=CARTESIAN_POINT('Ctrl Pts',(-2.23837749301974,12.2,11.1277318174937));
#233233=CARTESIAN_POINT('Ctrl Pts',(-2.24121095078674,12.2,11.1316554347835));
#233234=CARTESIAN_POINT('Ctrl Pts',(-2.24333604459456,12.2,11.134598148419));
#233235=CARTESIAN_POINT('Ctrl Pts',(-2.24546858543782,12.2,11.1375439932638));
#233236=CARTESIAN_POINT('Ctrl Pts',(-2.2476085772082,12.2,11.1404929264012));
#233237=CARTESIAN_POINT('Ctrl Pts',(-2.25046189892076,12.2,11.1444248363581));
#233238=CARTESIAN_POINT('Ctrl Pts',(-2.25332846455655,12.2,11.1483622377643));
#233239=CARTESIAN_POINT('Ctrl Pts',(-2.25620827776471,12.2,11.1523050297194));
#233240=CARTESIAN_POINT('Ctrl Pts',(-2.25836813776891,12.2,11.15526212382));
#233241=CARTESIAN_POINT('Ctrl Pts',(-2.2605354499839,12.2,11.15822224942));
#233242=CARTESIAN_POINT('Ctrl Pts',(-2.26271021605431,12.2,11.1611853661267));
#233243=CARTESIAN_POINT('Ctrl Pts',(-2.26488498212472,12.2,11.1641484828334));
#233244=CARTESIAN_POINT('Ctrl Pts',(-2.26706720178658,12.2,11.167114589061));
#233245=CARTESIAN_POINT('Ctrl Pts',(-2.26925687624766,12.2,11.1700836436194));
#233246=CARTESIAN_POINT('Ctrl Pts',(-2.27144655110652,12.2,11.1730526987171));
#233247=CARTESIAN_POINT('Ctrl Pts',(-2.27364368109253,12.2,11.1760247014658));
#233248=CARTESIAN_POINT('Ctrl Pts',(-2.27584826745561,12.2,11.1789996111485));
#233249=CARTESIAN_POINT('Ctrl Pts',(-2.27805285341819,12.2,11.1819745202908));
#233250=CARTESIAN_POINT('Ctrl Pts',(-2.28026489627206,12.2,11.184952336533));
#233251=CARTESIAN_POINT('Ctrl Pts',(-2.28248439623372,12.2,11.1879330190499));
#233252=CARTESIAN_POINT('Ctrl Pts',(-2.28470389619538,12.2,11.1909137015668));
#233253=CARTESIAN_POINT('Ctrl Pts',(-2.28693085412303,12.2,11.1938972487643));
#233254=CARTESIAN_POINT('Ctrl Pts',(-2.28916527101038,12.2,11.1968836202944));
#233255=CARTESIAN_POINT('Ctrl Pts',(-2.29139968789772,12.2,11.1998699918244));
#233256=CARTESIAN_POINT('Ctrl Pts',(-2.29364156283617,12.2,11.2028591863924));
#233257=CARTESIAN_POINT('Ctrl Pts',(-2.29589089826463,12.2,11.2058511625056));
#233258=CARTESIAN_POINT('Ctrl Pts',(-2.2981402336931,12.2,11.2088431386188));
#233259=CARTESIAN_POINT('Ctrl Pts',(-2.30039702983625,12.2,11.2118378951825));
#233260=CARTESIAN_POINT('Ctrl Pts',(-2.30266128579499,12.2,11.2148353959483));
#233261=CARTESIAN_POINT('Ctrl Pts',(-2.30492554175372,12.2,11.2178328967141));
#233262=CARTESIAN_POINT('Ctrl Pts',(-2.3071972578203,12.2,11.2208331434048));
#233263=CARTESIAN_POINT('Ctrl Pts',(-2.30947643623649,12.2,11.223836094087));
#233264=CARTESIAN_POINT('Ctrl Pts',(-2.31175561506672,12.2,11.2268390453147));
#233265=CARTESIAN_POINT('Ctrl Pts',(-2.31404225544904,12.2,11.2298447031182));
#233266=CARTESIAN_POINT('Ctrl Pts',(-2.31633635824179,12.2,11.2328530157224));
#233267=CARTESIAN_POINT('Ctrl Pts',(-2.31939516127085,12.2,11.2368640982839));
#233268=CARTESIAN_POINT('Ctrl Pts',(-2.32246723093896,12.2,11.2408798984299));
#233269=CARTESIAN_POINT('Ctrl Pts',(-2.32555256875624,12.2,11.2449003215639));
#233270=CARTESIAN_POINT('Ctrl Pts',(-2.32940924134313,12.2,11.2499258508922));
#233271=CARTESIAN_POINT('Ctrl Pts',(-2.33328664381693,12.2,11.2549585979013));
#233272=CARTESIAN_POINT('Ctrl Pts',(-2.33718477800005,12.2,11.259998549));
#233273=CARTESIAN_POINT('Origin',(-5.66257110645729E-14,15.2,-1.77635683940025E-14));
#233274=CARTESIAN_POINT('',(-3.20199116200006,15.2,9.86852965799999));
#233275=CARTESIAN_POINT('',(-3.20199116200006,12.2,9.86852965799999));
#233276=CARTESIAN_POINT('',(-3.20199116200006,15.2,9.86852965799999));
#233277=CARTESIAN_POINT('Origin',(-5.66257110645729E-14,12.2,-1.77635683940025E-14));
#233278=CARTESIAN_POINT('Origin',(-5.66257110645729E-14,15.2,-1.77635683940025E-14));
#233279=CARTESIAN_POINT('Origin',(-5.66257110645729E-14,15.2,-1.77635683940025E-14));
#233280=CARTESIAN_POINT('',(-3.91586047956408,15.2,10.8127719253567));
#233281=CARTESIAN_POINT('',(-4.27433547000006,15.2,10.676144262));
#233282=CARTESIAN_POINT('Origin',(-5.66257110645729E-14,15.2,-1.77635683940025E-14));
#233283=CARTESIAN_POINT('',(-4.27433547000006,12.2,10.676144262));
#233284=CARTESIAN_POINT('',(-4.27433547000006,15.2,10.676144262));
#233285=CARTESIAN_POINT('',(-3.91586047956408,12.2,10.8127719253567));
#233286=CARTESIAN_POINT('Origin',(-5.66257110645729E-14,12.2,-1.77635683940025E-14));
#233287=CARTESIAN_POINT('',(-3.91586048000006,15.2,10.812771926));
#233288=CARTESIAN_POINT('Ctrl Pts',(-3.20199116200006,15.2,9.86852965799999));
#233289=CARTESIAN_POINT('Ctrl Pts',(-3.20199116200006,11.6,9.86852965799999));
#233290=CARTESIAN_POINT('Ctrl Pts',(-3.20205902800006,15.2,9.86869026699999));
#233291=CARTESIAN_POINT('Ctrl Pts',(-3.20205902800006,11.6,9.86869026699999));
#233292=CARTESIAN_POINT('Ctrl Pts',(-3.20219720700006,15.2,9.86901705999998));
#233293=CARTESIAN_POINT('Ctrl Pts',(-3.20219720700006,11.6,9.86901705999998));
#233294=CARTESIAN_POINT('Ctrl Pts',(-3.20240682500006,15.2,9.86951212499999));
#233295=CARTESIAN_POINT('Ctrl Pts',(-3.20240682500006,11.6,9.86951212499999));
#233296=CARTESIAN_POINT('Ctrl Pts',(-3.20268969700006,15.2,9.87017881299998));
#233297=CARTESIAN_POINT('Ctrl Pts',(-3.20268969700006,11.6,9.87017881299998));
#233298=CARTESIAN_POINT('Ctrl Pts',(-3.20304833100006,15.2,9.87102171699998));
#233299=CARTESIAN_POINT('Ctrl Pts',(-3.20304833100006,11.6,9.87102171699998));
#233300=CARTESIAN_POINT('Ctrl Pts',(-3.20341363700006,15.2,9.87187791599998));
#233301=CARTESIAN_POINT('Ctrl Pts',(-3.20341363700006,11.6,9.87187791599998));
#233302=CARTESIAN_POINT('Ctrl Pts',(-3.20378354400006,15.2,9.87274249599999));
#233303=CARTESIAN_POINT('Ctrl Pts',(-3.20378354400006,11.6,9.87274249599999));
#233304=CARTESIAN_POINT('Ctrl Pts',(-3.20415805700006,15.2,9.87361542499999));
#233305=CARTESIAN_POINT('Ctrl Pts',(-3.20415805700006,11.6,9.87361542499999));
#233306=CARTESIAN_POINT('Ctrl Pts',(-3.20453718500006,15.2,9.87449666999998));
#233307=CARTESIAN_POINT('Ctrl Pts',(-3.20453718500006,11.6,9.87449666999998));
#233308=CARTESIAN_POINT('Ctrl Pts',(-3.20492093100006,15.2,9.87538620099999));
#233309=CARTESIAN_POINT('Ctrl Pts',(-3.20492093100006,11.6,9.87538620099999));
#233310=CARTESIAN_POINT('Ctrl Pts',(-3.20530930300006,15.2,9.87628398499999));
#233311=CARTESIAN_POINT('Ctrl Pts',(-3.20530930300006,11.6,9.87628398499999));
#233312=CARTESIAN_POINT('Ctrl Pts',(-3.20570230600006,15.2,9.87718999099998));
#233313=CARTESIAN_POINT('Ctrl Pts',(-3.20570230600006,11.6,9.87718999099998));
#233314=CARTESIAN_POINT('Ctrl Pts',(-3.20609994600006,15.2,9.87810418899999));
#233315=CARTESIAN_POINT('Ctrl Pts',(-3.20609994600006,11.6,9.87810418899999));
#233316=CARTESIAN_POINT('Ctrl Pts',(-3.20650222800006,15.2,9.87902654599999));
#233317=CARTESIAN_POINT('Ctrl Pts',(-3.20650222800006,11.6,9.87902654599999));
#233318=CARTESIAN_POINT('Ctrl Pts',(-3.20690915900005,15.2,9.87995703299998));
#233319=CARTESIAN_POINT('Ctrl Pts',(-3.20690915900005,11.6,9.87995703299998));
#233320=CARTESIAN_POINT('Ctrl Pts',(-3.20732074500006,15.2,9.88089561799999));
#233321=CARTESIAN_POINT('Ctrl Pts',(-3.20732074500006,11.6,9.88089561799999));
#233322=CARTESIAN_POINT('Ctrl Pts',(-3.20773698900005,15.2,9.88184226999999));
#233323=CARTESIAN_POINT('Ctrl Pts',(-3.20773698900005,11.6,9.88184226999999));
#233324=CARTESIAN_POINT('Ctrl Pts',(-3.20815790100006,15.2,9.88279695899998));
#233325=CARTESIAN_POINT('Ctrl Pts',(-3.20815790100006,11.6,9.88279695899998));
#233326=CARTESIAN_POINT('Ctrl Pts',(-3.20858348200006,15.2,9.88375965699999));
#233327=CARTESIAN_POINT('Ctrl Pts',(-3.20858348200006,11.6,9.88375965699999));
#233328=CARTESIAN_POINT('Ctrl Pts',(-3.20901374100006,15.2,9.88473032999998));
#233329=CARTESIAN_POINT('Ctrl Pts',(-3.20901374100006,11.6,9.88473032999998));
#233330=CARTESIAN_POINT('Ctrl Pts',(-3.20944868300006,15.2,9.88570895099999));
#233331=CARTESIAN_POINT('Ctrl Pts',(-3.20944868300006,11.6,9.88570895099999));
#233332=CARTESIAN_POINT('Ctrl Pts',(-3.20988831200005,15.2,9.88669548899999));
#233333=CARTESIAN_POINT('Ctrl Pts',(-3.20988831200005,11.6,9.88669548899999));
#233334=CARTESIAN_POINT('Ctrl Pts',(-3.21033263400006,15.2,9.88768991299998));
#233335=CARTESIAN_POINT('Ctrl Pts',(-3.21033263400006,11.6,9.88768991299998));
#233336=CARTESIAN_POINT('Ctrl Pts',(-3.21078165500006,15.2,9.88869219599999));
#233337=CARTESIAN_POINT('Ctrl Pts',(-3.21078165500006,11.6,9.88869219599999));
#233338=CARTESIAN_POINT('Ctrl Pts',(-3.21123538000006,15.2,9.88970230599998));
#233339=CARTESIAN_POINT('Ctrl Pts',(-3.21123538000006,11.6,9.88970230599998));
#233340=CARTESIAN_POINT('Ctrl Pts',(-3.21169381300006,15.2,9.89072021499998));
#233341=CARTESIAN_POINT('Ctrl Pts',(-3.21169381300006,11.6,9.89072021499998));
#233342=CARTESIAN_POINT('Ctrl Pts',(-3.21215696200006,15.2,9.89174589399998));
#233343=CARTESIAN_POINT('Ctrl Pts',(-3.21215696200006,11.6,9.89174589399998));
#233344=CARTESIAN_POINT('Ctrl Pts',(-3.21262483100006,15.2,9.89277931299998));
#233345=CARTESIAN_POINT('Ctrl Pts',(-3.21262483100006,11.6,9.89277931299998));
#233346=CARTESIAN_POINT('Ctrl Pts',(-3.21309742500006,15.2,9.89382044299998));
#233347=CARTESIAN_POINT('Ctrl Pts',(-3.21309742500006,11.6,9.89382044299998));
#233348=CARTESIAN_POINT('Ctrl Pts',(-3.21357474800006,15.2,9.89486925699998));
#233349=CARTESIAN_POINT('Ctrl Pts',(-3.21357474800006,11.6,9.89486925699998));
#233350=CARTESIAN_POINT('Ctrl Pts',(-3.21405680800006,15.2,9.89592572399999));
#233351=CARTESIAN_POINT('Ctrl Pts',(-3.21405680800006,11.6,9.89592572399999));
#233352=CARTESIAN_POINT('Ctrl Pts',(-3.21454360800006,15.2,9.89698981699998));
#233353=CARTESIAN_POINT('Ctrl Pts',(-3.21454360800006,11.6,9.89698981699998));
#233354=CARTESIAN_POINT('Ctrl Pts',(-3.21503515400006,15.2,9.89806150699999));
#233355=CARTESIAN_POINT('Ctrl Pts',(-3.21503515400006,11.6,9.89806150699999));
#233356=CARTESIAN_POINT('Ctrl Pts',(-3.21553144900005,15.2,9.89914076599998));
#233357=CARTESIAN_POINT('Ctrl Pts',(-3.21553144900005,11.6,9.89914076599998));
#233358=CARTESIAN_POINT('Ctrl Pts',(-3.21603250100006,15.2,9.90022756599998));
#233359=CARTESIAN_POINT('Ctrl Pts',(-3.21603250100006,11.6,9.90022756599998));
#233360=CARTESIAN_POINT('Ctrl Pts',(-3.21653831300006,15.2,9.90132187799999));
#233361=CARTESIAN_POINT('Ctrl Pts',(-3.21653831300006,11.6,9.90132187799999));
#233362=CARTESIAN_POINT('Ctrl Pts',(-3.21704889000006,15.2,9.90242367599999));
#233363=CARTESIAN_POINT('Ctrl Pts',(-3.21704889000006,11.6,9.90242367599999));
#233364=CARTESIAN_POINT('Ctrl Pts',(-3.21756423800006,15.2,9.90353292999998));
#233365=CARTESIAN_POINT('Ctrl Pts',(-3.21756423800006,11.6,9.90353292999998));
#233366=CARTESIAN_POINT('Ctrl Pts',(-3.21808436100006,15.2,9.90464961299999));
#233367=CARTESIAN_POINT('Ctrl Pts',(-3.21808436100006,11.6,9.90464961299999));
#233368=CARTESIAN_POINT('Ctrl Pts',(-3.21860926400006,15.2,9.90577369899999));
#233369=CARTESIAN_POINT('Ctrl Pts',(-3.21860926400006,11.6,9.90577369899999));
#233370=CARTESIAN_POINT('Ctrl Pts',(-3.21913895200006,15.2,9.90690515799999));
#233371=CARTESIAN_POINT('Ctrl Pts',(-3.21913895200006,11.6,9.90690515799999));
#233372=CARTESIAN_POINT('Ctrl Pts',(-3.21967342800006,15.2,9.90804396499998));
#233373=CARTESIAN_POINT('Ctrl Pts',(-3.21967342800006,11.6,9.90804396499998));
#233374=CARTESIAN_POINT('Ctrl Pts',(-3.22021270000006,15.2,9.90919009099999));
#233375=CARTESIAN_POINT('Ctrl Pts',(-3.22021270000006,11.6,9.90919009099999));
#233376=CARTESIAN_POINT('Ctrl Pts',(-3.22075677000006,15.2,9.91034351099999));
#233377=CARTESIAN_POINT('Ctrl Pts',(-3.22075677000006,11.6,9.91034351099999));
#233378=CARTESIAN_POINT('Ctrl Pts',(-3.22130564400006,15.2,9.91150419699999));
#233379=CARTESIAN_POINT('Ctrl Pts',(-3.22130564400006,11.6,9.91150419699999));
#233380=CARTESIAN_POINT('Ctrl Pts',(-3.22185932500005,15.2,9.91267212099999));
#233381=CARTESIAN_POINT('Ctrl Pts',(-3.22185932500005,11.6,9.91267212099999));
#233382=CARTESIAN_POINT('Ctrl Pts',(-3.22241782000006,15.2,9.91384725799998));
#233383=CARTESIAN_POINT('Ctrl Pts',(-3.22241782000006,11.6,9.91384725799998));
#233384=CARTESIAN_POINT('Ctrl Pts',(-3.22298113100006,15.2,9.91502958099998));
#233385=CARTESIAN_POINT('Ctrl Pts',(-3.22298113100006,11.6,9.91502958099998));
#233386=CARTESIAN_POINT('Ctrl Pts',(-3.22354926400005,15.2,9.91621906299999));
#233387=CARTESIAN_POINT('Ctrl Pts',(-3.22354926400005,11.6,9.91621906299999));
#233388=CARTESIAN_POINT('Ctrl Pts',(-3.22412222300006,15.2,9.91741567799998));
#233389=CARTESIAN_POINT('Ctrl Pts',(-3.22412222300006,11.6,9.91741567799998));
#233390=CARTESIAN_POINT('Ctrl Pts',(-3.22470001300006,15.2,9.91861939899999));
#233391=CARTESIAN_POINT('Ctrl Pts',(-3.22470001300006,11.6,9.91861939899999));
#233392=CARTESIAN_POINT('Ctrl Pts',(-3.22528263900006,15.2,9.91983020199999));
#233393=CARTESIAN_POINT('Ctrl Pts',(-3.22528263900006,11.6,9.91983020199999));
#233394=CARTESIAN_POINT('Ctrl Pts',(-3.22587010200006,15.2,9.92104805799999));
#233395=CARTESIAN_POINT('Ctrl Pts',(-3.22587010200006,11.6,9.92104805799999));
#233396=CARTESIAN_POINT('Ctrl Pts',(-3.22646241000006,15.2,9.92227294299998));
#233397=CARTESIAN_POINT('Ctrl Pts',(-3.22646241000006,11.6,9.92227294299998));
#233398=CARTESIAN_POINT('Ctrl Pts',(-3.22705956700006,15.2,9.92350483199999));
#233399=CARTESIAN_POINT('Ctrl Pts',(-3.22705956700006,11.6,9.92350483199999));
#233400=CARTESIAN_POINT('Ctrl Pts',(-3.22766157600006,15.2,9.92474369799999));
#233401=CARTESIAN_POINT('Ctrl Pts',(-3.22766157600006,11.6,9.92474369799999));
#233402=CARTESIAN_POINT('Ctrl Pts',(-3.22826843900006,15.2,9.92598951399999));
#233403=CARTESIAN_POINT('Ctrl Pts',(-3.22826843900006,11.6,9.92598951399999));
#233404=CARTESIAN_POINT('Ctrl Pts',(-3.22888016500006,15.2,9.92724225699998));
#233405=CARTESIAN_POINT('Ctrl Pts',(-3.22888016500006,11.6,9.92724225699998));
#233406=CARTESIAN_POINT('Ctrl Pts',(-3.22949675600006,15.2,9.92850189999999));
#233407=CARTESIAN_POINT('Ctrl Pts',(-3.22949675600006,11.6,9.92850189999999));
#233408=CARTESIAN_POINT('Ctrl Pts',(-3.23011821600006,15.2,9.92976841899999));
#233409=CARTESIAN_POINT('Ctrl Pts',(-3.23011821600006,11.6,9.92976841899999));
#233410=CARTESIAN_POINT('Ctrl Pts',(-3.23074454800006,15.2,9.93104178799998));
#233411=CARTESIAN_POINT('Ctrl Pts',(-3.23074454800006,11.6,9.93104178799998));
#233412=CARTESIAN_POINT('Ctrl Pts',(-3.23137575800006,15.2,9.93232198199999));
#233413=CARTESIAN_POINT('Ctrl Pts',(-3.23137575800006,11.6,9.93232198199999));
#233414=CARTESIAN_POINT('Ctrl Pts',(-3.23201185000006,15.2,9.93360897599998));
#233415=CARTESIAN_POINT('Ctrl Pts',(-3.23201185000006,11.6,9.93360897599998));
#233416=CARTESIAN_POINT('Ctrl Pts',(-3.23265282700006,15.2,9.93490274499998));
#233417=CARTESIAN_POINT('Ctrl Pts',(-3.23265282700006,11.6,9.93490274499998));
#233418=CARTESIAN_POINT('Ctrl Pts',(-3.23329869300006,15.2,9.93620326399999));
#233419=CARTESIAN_POINT('Ctrl Pts',(-3.23329869300006,11.6,9.93620326399999));
#233420=CARTESIAN_POINT('Ctrl Pts',(-3.23394945200006,15.2,9.93751050999998));
#233421=CARTESIAN_POINT('Ctrl Pts',(-3.23394945200006,11.6,9.93751050999998));
#233422=CARTESIAN_POINT('Ctrl Pts',(-3.23460510900006,15.2,9.93882445699998));
#233423=CARTESIAN_POINT('Ctrl Pts',(-3.23460510900006,11.6,9.93882445699998));
#233424=CARTESIAN_POINT('Ctrl Pts',(-3.23526566700005,15.2,9.94014507999999));
#233425=CARTESIAN_POINT('Ctrl Pts',(-3.23526566700005,11.6,9.94014507999999));
#233426=CARTESIAN_POINT('Ctrl Pts',(-3.23593113000006,15.2,9.94147235599998));
#233427=CARTESIAN_POINT('Ctrl Pts',(-3.23593113000006,11.6,9.94147235599998));
#233428=CARTESIAN_POINT('Ctrl Pts',(-3.23660150200006,15.2,9.94280625999998));
#233429=CARTESIAN_POINT('Ctrl Pts',(-3.23660150200006,11.6,9.94280625999998));
#233430=CARTESIAN_POINT('Ctrl Pts',(-3.23727678700005,15.2,9.94414676799998));
#233431=CARTESIAN_POINT('Ctrl Pts',(-3.23727678700005,11.6,9.94414676799998));
#233432=CARTESIAN_POINT('Ctrl Pts',(-3.23795698800006,15.2,9.94549385599999));
#233433=CARTESIAN_POINT('Ctrl Pts',(-3.23795698800006,11.6,9.94549385599999));
#233434=CARTESIAN_POINT('Ctrl Pts',(-3.23864211000005,15.2,9.94684749899999));
#233435=CARTESIAN_POINT('Ctrl Pts',(-3.23864211000005,11.6,9.94684749899999));
#233436=CARTESIAN_POINT('Ctrl Pts',(-3.23933215600006,15.2,9.94820767499998));
#233437=CARTESIAN_POINT('Ctrl Pts',(-3.23933215600006,11.6,9.94820767499998));
#233438=CARTESIAN_POINT('Ctrl Pts',(-3.24002712900006,15.2,9.94957435799999));
#233439=CARTESIAN_POINT('Ctrl Pts',(-3.24002712900006,11.6,9.94957435799999));
#233440=CARTESIAN_POINT('Ctrl Pts',(-3.24072703400006,15.2,9.95094752699998));
#233441=CARTESIAN_POINT('Ctrl Pts',(-3.24072703400006,11.6,9.95094752699998));
#233442=CARTESIAN_POINT('Ctrl Pts',(-3.24143187300006,15.2,9.95232715499998));
#233443=CARTESIAN_POINT('Ctrl Pts',(-3.24143187300006,11.6,9.95232715499998));
#233444=CARTESIAN_POINT('Ctrl Pts',(-3.24214165200006,15.2,9.95371322199999));
#233445=CARTESIAN_POINT('Ctrl Pts',(-3.24214165200006,11.6,9.95371322199999));
#233446=CARTESIAN_POINT('Ctrl Pts',(-3.24285637300005,15.2,9.95510570299999));
#233447=CARTESIAN_POINT('Ctrl Pts',(-3.24285637300005,11.6,9.95510570299999));
#233448=CARTESIAN_POINT('Ctrl Pts',(-3.24357604000005,15.2,9.95650457299998));
#233449=CARTESIAN_POINT('Ctrl Pts',(-3.24357604000005,11.6,9.95650457299998));
#233450=CARTESIAN_POINT('Ctrl Pts',(-3.24430065600006,15.2,9.95790981099999));
#233451=CARTESIAN_POINT('Ctrl Pts',(-3.24430065600006,11.6,9.95790981099999));
#233452=CARTESIAN_POINT('Ctrl Pts',(-3.24503022600005,15.2,9.95932139299999));
#233453=CARTESIAN_POINT('Ctrl Pts',(-3.24503022600005,11.6,9.95932139299999));
#233454=CARTESIAN_POINT('Ctrl Pts',(-3.24576475100006,15.2,9.96073929699998));
#233455=CARTESIAN_POINT('Ctrl Pts',(-3.24576475100006,11.6,9.96073929699998));
#233456=CARTESIAN_POINT('Ctrl Pts',(-3.24650423700006,15.2,9.96216349899999));
#233457=CARTESIAN_POINT('Ctrl Pts',(-3.24650423700006,11.6,9.96216349899999));
#233458=CARTESIAN_POINT('Ctrl Pts',(-3.24724868600006,15.2,9.96359397599999));
#233459=CARTESIAN_POINT('Ctrl Pts',(-3.24724868600006,11.6,9.96359397599999));
#233460=CARTESIAN_POINT('Ctrl Pts',(-3.24799810100005,15.2,9.96503070499998));
#233461=CARTESIAN_POINT('Ctrl Pts',(-3.24799810100005,11.6,9.96503070499998));
#233462=CARTESIAN_POINT('Ctrl Pts',(-3.24875248700006,15.2,9.96647366399999));
#233463=CARTESIAN_POINT('Ctrl Pts',(-3.24875248700006,11.6,9.96647366399999));
#233464=CARTESIAN_POINT('Ctrl Pts',(-3.24951184600006,15.2,9.96792282999999));
#233465=CARTESIAN_POINT('Ctrl Pts',(-3.24951184600006,11.6,9.96792282999999));
#233466=CARTESIAN_POINT('Ctrl Pts',(-3.25027618200005,15.2,9.96937817999999));
#233467=CARTESIAN_POINT('Ctrl Pts',(-3.25027618200005,11.6,9.96937817999999));
#233468=CARTESIAN_POINT('Ctrl Pts',(-3.25104550000006,15.2,9.97083969299998));
#233469=CARTESIAN_POINT('Ctrl Pts',(-3.25104550000006,11.6,9.97083969299998));
#233470=CARTESIAN_POINT('Ctrl Pts',(-3.25181979900006,15.2,9.97230734499999));
#233471=CARTESIAN_POINT('Ctrl Pts',(-3.25181979900006,11.6,9.97230734499999));
#233472=CARTESIAN_POINT('Ctrl Pts',(-3.25259908600006,15.2,9.97378111499999));
#233473=CARTESIAN_POINT('Ctrl Pts',(-3.25259908600006,11.6,9.97378111499999));
#233474=CARTESIAN_POINT('Ctrl Pts',(-3.25338336200006,15.2,9.97526097899998));
#233475=CARTESIAN_POINT('Ctrl Pts',(-3.25338336200006,11.6,9.97526097899998));
#233476=CARTESIAN_POINT('Ctrl Pts',(-3.25417263200006,15.2,9.97674691699999));
#233477=CARTESIAN_POINT('Ctrl Pts',(-3.25417263200006,11.6,9.97674691699999));
#233478=CARTESIAN_POINT('Ctrl Pts',(-3.25496689700006,15.2,9.97823890599999));
#233479=CARTESIAN_POINT('Ctrl Pts',(-3.25496689700006,11.6,9.97823890599999));
#233480=CARTESIAN_POINT('Ctrl Pts',(-3.25576616300005,15.2,9.97973692499999));
#233481=CARTESIAN_POINT('Ctrl Pts',(-3.25576616300005,11.6,9.97973692499999));
#233482=CARTESIAN_POINT('Ctrl Pts',(-3.25657043100006,15.2,9.98124094999999));
#233483=CARTESIAN_POINT('Ctrl Pts',(-3.25657043100006,11.6,9.98124094999999));
#233484=CARTESIAN_POINT('Ctrl Pts',(-3.25737970400006,15.2,9.98275095999999));
#233485=CARTESIAN_POINT('Ctrl Pts',(-3.25737970400006,11.6,9.98275095999999));
#233486=CARTESIAN_POINT('Ctrl Pts',(-3.25819398700005,15.2,9.98426693399999));
#233487=CARTESIAN_POINT('Ctrl Pts',(-3.25819398700005,11.6,9.98426693399999));
#233488=CARTESIAN_POINT('Ctrl Pts',(-3.25901328200006,15.2,9.98578885099998));
#233489=CARTESIAN_POINT('Ctrl Pts',(-3.25901328200006,11.6,9.98578885099998));
#233490=CARTESIAN_POINT('Ctrl Pts',(-3.25983759100006,15.2,9.98731668699998));
#233491=CARTESIAN_POINT('Ctrl Pts',(-3.25983759100006,11.6,9.98731668699998));
#233492=CARTESIAN_POINT('Ctrl Pts',(-3.26066691700006,15.2,9.98885042199999));
#233493=CARTESIAN_POINT('Ctrl Pts',(-3.26066691700006,11.6,9.98885042199999));
#233494=CARTESIAN_POINT('Ctrl Pts',(-3.26150126600006,15.2,9.99039003499998));
#233495=CARTESIAN_POINT('Ctrl Pts',(-3.26150126600006,11.6,9.99039003499998));
#233496=CARTESIAN_POINT('Ctrl Pts',(-3.26234063800006,15.2,9.99193550399998));
#233497=CARTESIAN_POINT('Ctrl Pts',(-3.26234063800006,11.6,9.99193550399998));
#233498=CARTESIAN_POINT('Ctrl Pts',(-3.26318503700006,15.2,9.99348680799999));
#233499=CARTESIAN_POINT('Ctrl Pts',(-3.26318503700006,11.6,9.99348680799999));
#233500=CARTESIAN_POINT('Ctrl Pts',(-3.26403446500006,15.2,9.99504392599999));
#233501=CARTESIAN_POINT('Ctrl Pts',(-3.26403446500006,11.6,9.99504392599999));
#233502=CARTESIAN_POINT('Ctrl Pts',(-3.26488892700006,15.2,9.99660683599998));
#233503=CARTESIAN_POINT('Ctrl Pts',(-3.26488892700006,11.6,9.99660683599998));
#233504=CARTESIAN_POINT('Ctrl Pts',(-3.26574842300006,15.2,9.99817551799998));
#233505=CARTESIAN_POINT('Ctrl Pts',(-3.26574842300006,11.6,9.99817551799998));
#233506=CARTESIAN_POINT('Ctrl Pts',(-3.26661295800006,15.2,9.99974995199998));
#233507=CARTESIAN_POINT('Ctrl Pts',(-3.26661295800006,11.6,9.99974995199998));
#233508=CARTESIAN_POINT('Ctrl Pts',(-3.26748253400006,15.2,10.001330114));
#233509=CARTESIAN_POINT('Ctrl Pts',(-3.26748253400006,11.6,10.001330114));
#233510=CARTESIAN_POINT('Ctrl Pts',(-3.26835715400006,15.2,10.002915986));
#233511=CARTESIAN_POINT('Ctrl Pts',(-3.26835715400006,11.6,10.002915986));
#233512=CARTESIAN_POINT('Ctrl Pts',(-3.26923682100006,15.2,10.004507545));
#233513=CARTESIAN_POINT('Ctrl Pts',(-3.26923682100006,11.6,10.004507545));
#233514=CARTESIAN_POINT('Ctrl Pts',(-3.27012153800006,15.2,10.006104772));
#233515=CARTESIAN_POINT('Ctrl Pts',(-3.27012153800006,11.6,10.006104772));
#233516=CARTESIAN_POINT('Ctrl Pts',(-3.27101130700005,15.2,10.007707647));
#233517=CARTESIAN_POINT('Ctrl Pts',(-3.27101130700005,11.6,10.007707647));
#233518=CARTESIAN_POINT('Ctrl Pts',(-3.27190613100006,15.2,10.009316147));
#233519=CARTESIAN_POINT('Ctrl Pts',(-3.27190613100006,11.6,10.009316147));
#233520=CARTESIAN_POINT('Ctrl Pts',(-3.27280601300005,15.2,10.010930254));
#233521=CARTESIAN_POINT('Ctrl Pts',(-3.27280601300005,11.6,10.010930254));
#233522=CARTESIAN_POINT('Ctrl Pts',(-3.27371095400005,15.2,10.012549946));
#233523=CARTESIAN_POINT('Ctrl Pts',(-3.27371095400005,11.6,10.012549946));
#233524=CARTESIAN_POINT('Ctrl Pts',(-3.27462095900006,15.2,10.014175204));
#233525=CARTESIAN_POINT('Ctrl Pts',(-3.27462095900006,11.6,10.014175204));
#233526=CARTESIAN_POINT('Ctrl Pts',(-3.27553603000006,15.2,10.015806007));
#233527=CARTESIAN_POINT('Ctrl Pts',(-3.27553603000006,11.6,10.015806007));
#233528=CARTESIAN_POINT('Ctrl Pts',(-3.27645616800006,15.2,10.017442335));
#233529=CARTESIAN_POINT('Ctrl Pts',(-3.27645616800006,11.6,10.017442335));
#233530=CARTESIAN_POINT('Ctrl Pts',(-3.27738137700006,15.2,10.019084167));
#233531=CARTESIAN_POINT('Ctrl Pts',(-3.27738137700006,11.6,10.019084167));
#233532=CARTESIAN_POINT('Ctrl Pts',(-3.27831166000006,15.2,10.020731485));
#233533=CARTESIAN_POINT('Ctrl Pts',(-3.27831166000006,11.6,10.020731485));
#233534=CARTESIAN_POINT('Ctrl Pts',(-3.27924701900006,15.2,10.022384268));
#233535=CARTESIAN_POINT('Ctrl Pts',(-3.27924701900006,11.6,10.022384268));
#233536=CARTESIAN_POINT('Ctrl Pts',(-3.28018745600006,15.2,10.024042496));
#233537=CARTESIAN_POINT('Ctrl Pts',(-3.28018745600006,11.6,10.024042496));
#233538=CARTESIAN_POINT('Ctrl Pts',(-3.28113297400006,15.2,10.025706148));
#233539=CARTESIAN_POINT('Ctrl Pts',(-3.28113297400006,11.6,10.025706148));
#233540=CARTESIAN_POINT('Ctrl Pts',(-3.28208357600006,15.2,10.027375206));
#233541=CARTESIAN_POINT('Ctrl Pts',(-3.28208357600006,11.6,10.027375206));
#233542=CARTESIAN_POINT('Ctrl Pts',(-3.28303926400006,15.2,10.02904965));
#233543=CARTESIAN_POINT('Ctrl Pts',(-3.28303926400006,11.6,10.02904965));
#233544=CARTESIAN_POINT('Ctrl Pts',(-3.28400003900006,15.2,10.03072946));
#233545=CARTESIAN_POINT('Ctrl Pts',(-3.28400003900006,11.6,10.03072946));
#233546=CARTESIAN_POINT('Ctrl Pts',(-3.28496590600006,15.2,10.032414616));
#233547=CARTESIAN_POINT('Ctrl Pts',(-3.28496590600006,11.6,10.032414616));
#233548=CARTESIAN_POINT('Ctrl Pts',(-3.28593686500006,15.2,10.0341051));
#233549=CARTESIAN_POINT('Ctrl Pts',(-3.28593686500006,11.6,10.0341051));
#233550=CARTESIAN_POINT('Ctrl Pts',(-3.28691292000005,15.2,10.035800891));
#233551=CARTESIAN_POINT('Ctrl Pts',(-3.28691292000005,11.6,10.035800891));
#233552=CARTESIAN_POINT('Ctrl Pts',(-3.28789407300006,15.2,10.037501971));
#233553=CARTESIAN_POINT('Ctrl Pts',(-3.28789407300006,11.6,10.037501971));
#233554=CARTESIAN_POINT('Ctrl Pts',(-3.28888032700006,15.2,10.03920832));
#233555=CARTESIAN_POINT('Ctrl Pts',(-3.28888032700006,11.6,10.03920832));
#233556=CARTESIAN_POINT('Ctrl Pts',(-3.28987168300006,15.2,10.040919918));
#233557=CARTESIAN_POINT('Ctrl Pts',(-3.28987168300006,11.6,10.040919918));
#233558=CARTESIAN_POINT('Ctrl Pts',(-3.29086814400006,15.2,10.042636747));
#233559=CARTESIAN_POINT('Ctrl Pts',(-3.29086814400006,11.6,10.042636747));
#233560=CARTESIAN_POINT('Ctrl Pts',(-3.29186971100006,15.2,10.044358787));
#233561=CARTESIAN_POINT('Ctrl Pts',(-3.29186971100006,11.6,10.044358787));
#233562=CARTESIAN_POINT('Ctrl Pts',(-3.29287638800006,15.2,10.046086019));
#233563=CARTESIAN_POINT('Ctrl Pts',(-3.29287638800006,11.6,10.046086019));
#233564=CARTESIAN_POINT('Ctrl Pts',(-3.29388817700006,15.2,10.047818426));
#233565=CARTESIAN_POINT('Ctrl Pts',(-3.29388817700006,11.6,10.047818426));
#233566=CARTESIAN_POINT('Ctrl Pts',(-3.29490507900006,15.2,10.049555987));
#233567=CARTESIAN_POINT('Ctrl Pts',(-3.29490507900006,11.6,10.049555987));
#233568=CARTESIAN_POINT('Ctrl Pts',(-3.29592709800006,15.2,10.051298683));
#233569=CARTESIAN_POINT('Ctrl Pts',(-3.29592709800006,11.6,10.051298683));
#233570=CARTESIAN_POINT('Ctrl Pts',(-3.29695423400006,15.2,10.053046497));
#233571=CARTESIAN_POINT('Ctrl Pts',(-3.29695423400006,11.6,10.053046497));
#233572=CARTESIAN_POINT('Ctrl Pts',(-3.29798649200006,15.2,10.054799409));
#233573=CARTESIAN_POINT('Ctrl Pts',(-3.29798649200006,11.6,10.054799409));
#233574=CARTESIAN_POINT('Ctrl Pts',(-3.29902387100006,15.2,10.0565574));
#233575=CARTESIAN_POINT('Ctrl Pts',(-3.29902387100006,11.6,10.0565574));
#233576=CARTESIAN_POINT('Ctrl Pts',(-3.30006637500006,15.2,10.058320453));
#233577=CARTESIAN_POINT('Ctrl Pts',(-3.30006637500006,11.6,10.058320453));
#233578=CARTESIAN_POINT('Ctrl Pts',(-3.30111400600006,15.2,10.060088547));
#233579=CARTESIAN_POINT('Ctrl Pts',(-3.30111400600006,11.6,10.060088547));
#233580=CARTESIAN_POINT('Ctrl Pts',(-3.30216676600006,15.2,10.061861665));
#233581=CARTESIAN_POINT('Ctrl Pts',(-3.30216676600006,11.6,10.061861665));
#233582=CARTESIAN_POINT('Ctrl Pts',(-3.30322465700006,15.2,10.063639789));
#233583=CARTESIAN_POINT('Ctrl Pts',(-3.30322465700006,11.6,10.063639789));
#233584=CARTESIAN_POINT('Ctrl Pts',(-3.30428768000006,15.2,10.065422899));
#233585=CARTESIAN_POINT('Ctrl Pts',(-3.30428768000006,11.6,10.065422899));
#233586=CARTESIAN_POINT('Ctrl Pts',(-3.30535583900006,15.2,10.067210979));
#233587=CARTESIAN_POINT('Ctrl Pts',(-3.30535583900006,11.6,10.067210979));
#233588=CARTESIAN_POINT('Ctrl Pts',(-3.30642913400006,15.2,10.069004009));
#233589=CARTESIAN_POINT('Ctrl Pts',(-3.30642913400006,11.6,10.069004009));
#233590=CARTESIAN_POINT('Ctrl Pts',(-3.30750756900006,15.2,10.070801971));
#233591=CARTESIAN_POINT('Ctrl Pts',(-3.30750756900006,11.6,10.070801971));
#233592=CARTESIAN_POINT('Ctrl Pts',(-3.30859114400006,15.2,10.072604847));
#233593=CARTESIAN_POINT('Ctrl Pts',(-3.30859114400006,11.6,10.072604847));
#233594=CARTESIAN_POINT('Ctrl Pts',(-3.30967986300006,15.2,10.07441262));
#233595=CARTESIAN_POINT('Ctrl Pts',(-3.30967986300006,11.6,10.07441262));
#233596=CARTESIAN_POINT('Ctrl Pts',(-3.31077372600005,15.2,10.07622527));
#233597=CARTESIAN_POINT('Ctrl Pts',(-3.31077372600005,11.6,10.07622527));
#233598=CARTESIAN_POINT('Ctrl Pts',(-3.31187273500006,15.2,10.078042781));
#233599=CARTESIAN_POINT('Ctrl Pts',(-3.31187273500006,11.6,10.078042781));
#233600=CARTESIAN_POINT('Ctrl Pts',(-3.31297689300006,15.2,10.079865133));
#233601=CARTESIAN_POINT('Ctrl Pts',(-3.31297689300006,11.6,10.079865133));
#233602=CARTESIAN_POINT('Ctrl Pts',(-3.31408620300006,15.2,10.081692309));
#233603=CARTESIAN_POINT('Ctrl Pts',(-3.31408620300006,11.6,10.081692309));
#233604=CARTESIAN_POINT('Ctrl Pts',(-3.31520066400006,15.2,10.083524292));
#233605=CARTESIAN_POINT('Ctrl Pts',(-3.31520066400006,11.6,10.083524292));
#233606=CARTESIAN_POINT('Ctrl Pts',(-3.31632027900006,15.2,10.085361064));
#233607=CARTESIAN_POINT('Ctrl Pts',(-3.31632027900006,11.6,10.085361064));
#233608=CARTESIAN_POINT('Ctrl Pts',(-3.31744505100006,15.2,10.087202607));
#233609=CARTESIAN_POINT('Ctrl Pts',(-3.31744505100006,11.6,10.087202607));
#233610=CARTESIAN_POINT('Ctrl Pts',(-3.31857498100006,15.2,10.089048904));
#233611=CARTESIAN_POINT('Ctrl Pts',(-3.31857498100006,11.6,10.089048904));
#233612=CARTESIAN_POINT('Ctrl Pts',(-3.31971007100006,15.2,10.090899936));
#233613=CARTESIAN_POINT('Ctrl Pts',(-3.31971007100006,11.6,10.090899936));
#233614=CARTESIAN_POINT('Ctrl Pts',(-3.32085032200006,15.2,10.092755686));
#233615=CARTESIAN_POINT('Ctrl Pts',(-3.32085032200006,11.6,10.092755686));
#233616=CARTESIAN_POINT('Ctrl Pts',(-3.32199573600006,15.2,10.094616137));
#233617=CARTESIAN_POINT('Ctrl Pts',(-3.32199573600006,11.6,10.094616137));
#233618=CARTESIAN_POINT('Ctrl Pts',(-3.32314631600005,15.2,10.096481272));
#233619=CARTESIAN_POINT('Ctrl Pts',(-3.32314631600005,11.6,10.096481272));
#233620=CARTESIAN_POINT('Ctrl Pts',(-3.32430206100006,15.2,10.098351073));
#233621=CARTESIAN_POINT('Ctrl Pts',(-3.32430206100006,11.6,10.098351073));
#233622=CARTESIAN_POINT('Ctrl Pts',(-3.32546297600006,15.2,10.100225521));
#233623=CARTESIAN_POINT('Ctrl Pts',(-3.32546297600006,11.6,10.100225521));
#233624=CARTESIAN_POINT('Ctrl Pts',(-3.32662906000006,15.2,10.102104602));
#233625=CARTESIAN_POINT('Ctrl Pts',(-3.32662906000006,11.6,10.102104602));
#233626=CARTESIAN_POINT('Ctrl Pts',(-3.32780031700006,15.2,10.103988296));
#233627=CARTESIAN_POINT('Ctrl Pts',(-3.32780031700006,11.6,10.103988296));
#233628=CARTESIAN_POINT('Ctrl Pts',(-3.32897674600006,15.2,10.105876588));
#233629=CARTESIAN_POINT('Ctrl Pts',(-3.32897674600006,11.6,10.105876588));
#233630=CARTESIAN_POINT('Ctrl Pts',(-3.33015835200006,15.2,10.107769459));
#233631=CARTESIAN_POINT('Ctrl Pts',(-3.33015835200006,11.6,10.107769459));
#233632=CARTESIAN_POINT('Ctrl Pts',(-3.33134513300006,15.2,10.109666894));
#233633=CARTESIAN_POINT('Ctrl Pts',(-3.33134513300006,11.6,10.109666894));
#233634=CARTESIAN_POINT('Ctrl Pts',(-3.33253709400006,15.2,10.111568874));
#233635=CARTESIAN_POINT('Ctrl Pts',(-3.33253709400006,11.6,10.111568874));
#233636=CARTESIAN_POINT('Ctrl Pts',(-3.33373423400006,15.2,10.113475383));
#233637=CARTESIAN_POINT('Ctrl Pts',(-3.33373423400006,11.6,10.113475383));
#233638=CARTESIAN_POINT('Ctrl Pts',(-3.33493655500006,15.2,10.115386405));
#233639=CARTESIAN_POINT('Ctrl Pts',(-3.33493655500006,11.6,10.115386405));
#233640=CARTESIAN_POINT('Ctrl Pts',(-3.33614406000006,15.2,10.11730192));
#233641=CARTESIAN_POINT('Ctrl Pts',(-3.33614406000006,11.6,10.11730192));
#233642=CARTESIAN_POINT('Ctrl Pts',(-3.33735675000006,15.2,10.119221915));
#233643=CARTESIAN_POINT('Ctrl Pts',(-3.33735675000006,11.6,10.119221915));
#233644=CARTESIAN_POINT('Ctrl Pts',(-3.33857462500006,15.2,10.121146371));
#233645=CARTESIAN_POINT('Ctrl Pts',(-3.33857462500006,11.6,10.121146371));
#233646=CARTESIAN_POINT('Ctrl Pts',(-3.33979768900006,15.2,10.123075272));
#233647=CARTESIAN_POINT('Ctrl Pts',(-3.33979768900006,11.6,10.123075272));
#233648=CARTESIAN_POINT('Ctrl Pts',(-3.34102594100006,15.2,10.125008601));
#233649=CARTESIAN_POINT('Ctrl Pts',(-3.34102594100006,11.6,10.125008601));
#233650=CARTESIAN_POINT('Ctrl Pts',(-3.34225938500006,15.2,10.126946342));
#233651=CARTESIAN_POINT('Ctrl Pts',(-3.34225938500006,11.6,10.126946342));
#233652=CARTESIAN_POINT('Ctrl Pts',(-3.34349802100005,15.2,10.128888478));
#233653=CARTESIAN_POINT('Ctrl Pts',(-3.34349802100005,11.6,10.128888478));
#233654=CARTESIAN_POINT('Ctrl Pts',(-3.34474185000006,15.2,10.130834991));
#233655=CARTESIAN_POINT('Ctrl Pts',(-3.34474185000006,11.6,10.130834991));
#233656=CARTESIAN_POINT('Ctrl Pts',(-3.34599087400006,15.2,10.132785868));
#233657=CARTESIAN_POINT('Ctrl Pts',(-3.34599087400006,11.6,10.132785868));
#233658=CARTESIAN_POINT('Ctrl Pts',(-3.34724509500006,15.2,10.134741089));
#233659=CARTESIAN_POINT('Ctrl Pts',(-3.34724509500006,11.6,10.134741089));
#233660=CARTESIAN_POINT('Ctrl Pts',(-3.34850451400006,15.2,10.13670064));
#233661=CARTESIAN_POINT('Ctrl Pts',(-3.34850451400006,11.6,10.13670064));
#233662=CARTESIAN_POINT('Ctrl Pts',(-3.34976913200005,15.2,10.138664505));
#233663=CARTESIAN_POINT('Ctrl Pts',(-3.34976913200005,11.6,10.138664505));
#233664=CARTESIAN_POINT('Ctrl Pts',(-3.35103895100006,15.2,10.140632665));
#233665=CARTESIAN_POINT('Ctrl Pts',(-3.35103895100006,11.6,10.140632665));
#233666=CARTESIAN_POINT('Ctrl Pts',(-3.35231397200006,15.2,10.142605106));
#233667=CARTESIAN_POINT('Ctrl Pts',(-3.35231397200006,11.6,10.142605106));
#233668=CARTESIAN_POINT('Ctrl Pts',(-3.35359419600006,15.2,10.144581811));
#233669=CARTESIAN_POINT('Ctrl Pts',(-3.35359419600006,11.6,10.144581811));
#233670=CARTESIAN_POINT('Ctrl Pts',(-3.35487962600005,15.2,10.146562764));
#233671=CARTESIAN_POINT('Ctrl Pts',(-3.35487962600005,11.6,10.146562764));
#233672=CARTESIAN_POINT('Ctrl Pts',(-3.35617026000006,15.2,10.14854795));
#233673=CARTESIAN_POINT('Ctrl Pts',(-3.35617026000006,11.6,10.14854795));
#233674=CARTESIAN_POINT('Ctrl Pts',(-3.35746610300005,15.2,10.150537351));
#233675=CARTESIAN_POINT('Ctrl Pts',(-3.35746610300005,11.6,10.150537351));
#233676=CARTESIAN_POINT('Ctrl Pts',(-3.35876715400006,15.2,10.152530952));
#233677=CARTESIAN_POINT('Ctrl Pts',(-3.35876715400006,11.6,10.152530952));
#233678=CARTESIAN_POINT('Ctrl Pts',(-3.36007341500005,15.2,10.154528737));
#233679=CARTESIAN_POINT('Ctrl Pts',(-3.36007341500005,11.6,10.154528737));
#233680=CARTESIAN_POINT('Ctrl Pts',(-3.36138488700006,15.2,10.156530691));
#233681=CARTESIAN_POINT('Ctrl Pts',(-3.36138488700006,11.6,10.156530691));
#233682=CARTESIAN_POINT('Ctrl Pts',(-3.36270157200006,15.2,10.158536796));
#233683=CARTESIAN_POINT('Ctrl Pts',(-3.36270157200006,11.6,10.158536796));
#233684=CARTESIAN_POINT('Ctrl Pts',(-3.36402347000006,15.2,10.160547038));
#233685=CARTESIAN_POINT('Ctrl Pts',(-3.36402347000006,11.6,10.160547038));
#233686=CARTESIAN_POINT('Ctrl Pts',(-3.36535058300006,15.2,10.162561401));
#233687=CARTESIAN_POINT('Ctrl Pts',(-3.36535058300006,11.6,10.162561401));
#233688=CARTESIAN_POINT('Ctrl Pts',(-3.36668291200006,15.2,10.164579868));
#233689=CARTESIAN_POINT('Ctrl Pts',(-3.36668291200006,11.6,10.164579868));
#233690=CARTESIAN_POINT('Ctrl Pts',(-3.36802045900006,15.2,10.166602425));
#233691=CARTESIAN_POINT('Ctrl Pts',(-3.36802045900006,11.6,10.166602425));
#233692=CARTESIAN_POINT('Ctrl Pts',(-3.36936322400006,15.2,10.168629055));
#233693=CARTESIAN_POINT('Ctrl Pts',(-3.36936322400006,11.6,10.168629055));
#233694=CARTESIAN_POINT('Ctrl Pts',(-3.37071120800006,15.2,10.170659744));
#233695=CARTESIAN_POINT('Ctrl Pts',(-3.37071120800006,11.6,10.170659744));
#233696=CARTESIAN_POINT('Ctrl Pts',(-3.37206441300005,15.2,10.172694474));
#233697=CARTESIAN_POINT('Ctrl Pts',(-3.37206441300005,11.6,10.172694474));
#233698=CARTESIAN_POINT('Ctrl Pts',(-3.37342284100006,15.2,10.174733231));
#233699=CARTESIAN_POINT('Ctrl Pts',(-3.37342284100006,11.6,10.174733231));
#233700=CARTESIAN_POINT('Ctrl Pts',(-3.37478649100006,15.2,10.176776001));
#233701=CARTESIAN_POINT('Ctrl Pts',(-3.37478649100006,11.6,10.176776001));
#233702=CARTESIAN_POINT('Ctrl Pts',(-3.37615536500006,15.2,10.178822766));
#233703=CARTESIAN_POINT('Ctrl Pts',(-3.37615536500006,11.6,10.178822766));
#233704=CARTESIAN_POINT('Ctrl Pts',(-3.37752946400005,15.2,10.180873512));
#233705=CARTESIAN_POINT('Ctrl Pts',(-3.37752946400005,11.6,10.180873512));
#233706=CARTESIAN_POINT('Ctrl Pts',(-3.37890879000006,15.2,10.182928223));
#233707=CARTESIAN_POINT('Ctrl Pts',(-3.37890879000006,11.6,10.182928223));
#233708=CARTESIAN_POINT('Ctrl Pts',(-3.38029334200006,15.2,10.184986884));
#233709=CARTESIAN_POINT('Ctrl Pts',(-3.38029334200006,11.6,10.184986884));
#233710=CARTESIAN_POINT('Ctrl Pts',(-3.38168312400006,15.2,10.18704948));
#233711=CARTESIAN_POINT('Ctrl Pts',(-3.38168312400006,11.6,10.18704948));
#233712=CARTESIAN_POINT('Ctrl Pts',(-3.38307813500006,15.2,10.189115995));
#233713=CARTESIAN_POINT('Ctrl Pts',(-3.38307813500006,11.6,10.189115995));
#233714=CARTESIAN_POINT('Ctrl Pts',(-3.38447837600006,15.2,10.191186415));
#233715=CARTESIAN_POINT('Ctrl Pts',(-3.38447837600006,11.6,10.191186415));
#233716=CARTESIAN_POINT('Ctrl Pts',(-3.38588384900006,15.2,10.193260723));
#233717=CARTESIAN_POINT('Ctrl Pts',(-3.38588384900006,11.6,10.193260723));
#233718=CARTESIAN_POINT('Ctrl Pts',(-3.38729455300005,15.2,10.195338907));
#233719=CARTESIAN_POINT('Ctrl Pts',(-3.38729455300005,11.6,10.195338907));
#233720=CARTESIAN_POINT('Ctrl Pts',(-3.38871049200006,15.2,10.197420948));
#233721=CARTESIAN_POINT('Ctrl Pts',(-3.38871049200006,11.6,10.197420948));
#233722=CARTESIAN_POINT('Ctrl Pts',(-3.39013166400006,15.2,10.199506834));
#233723=CARTESIAN_POINT('Ctrl Pts',(-3.39013166400006,11.6,10.199506834));
#233724=CARTESIAN_POINT('Ctrl Pts',(-3.39155807300005,15.2,10.20159655));
#233725=CARTESIAN_POINT('Ctrl Pts',(-3.39155807300005,11.6,10.20159655));
#233726=CARTESIAN_POINT('Ctrl Pts',(-3.39298971700006,15.2,10.203690079));
#233727=CARTESIAN_POINT('Ctrl Pts',(-3.39298971700006,11.6,10.203690079));
#233728=CARTESIAN_POINT('Ctrl Pts',(-3.39442659800006,15.2,10.205787407));
#233729=CARTESIAN_POINT('Ctrl Pts',(-3.39442659800006,11.6,10.205787407));
#233730=CARTESIAN_POINT('Ctrl Pts',(-3.39586871900006,15.2,10.207888521));
#233731=CARTESIAN_POINT('Ctrl Pts',(-3.39586871900006,11.6,10.207888521));
#233732=CARTESIAN_POINT('Ctrl Pts',(-3.39731607700006,15.2,10.209993403));
#233733=CARTESIAN_POINT('Ctrl Pts',(-3.39731607700006,11.6,10.209993403));
#233734=CARTESIAN_POINT('Ctrl Pts',(-3.39876867500006,15.2,10.21210204));
#233735=CARTESIAN_POINT('Ctrl Pts',(-3.39876867500006,11.6,10.21210204));
#233736=CARTESIAN_POINT('Ctrl Pts',(-3.40022651400006,15.2,10.214214418));
#233737=CARTESIAN_POINT('Ctrl Pts',(-3.40022651400006,11.6,10.214214418));
#233738=CARTESIAN_POINT('Ctrl Pts',(-3.40168959500006,15.2,10.21633052));
#233739=CARTESIAN_POINT('Ctrl Pts',(-3.40168959500006,11.6,10.21633052));
#233740=CARTESIAN_POINT('Ctrl Pts',(-3.40315791900006,15.2,10.218450334));
#233741=CARTESIAN_POINT('Ctrl Pts',(-3.40315791900006,11.6,10.218450334));
#233742=CARTESIAN_POINT('Ctrl Pts',(-3.40463148500006,15.2,10.220573844));
#233743=CARTESIAN_POINT('Ctrl Pts',(-3.40463148500006,11.6,10.220573844));
#233744=CARTESIAN_POINT('Ctrl Pts',(-3.40611029600006,15.2,10.222701035));
#233745=CARTESIAN_POINT('Ctrl Pts',(-3.40611029600006,11.6,10.222701035));
#233746=CARTESIAN_POINT('Ctrl Pts',(-3.40759435200006,15.2,10.224831892));
#233747=CARTESIAN_POINT('Ctrl Pts',(-3.40759435200006,11.6,10.224831892));
#233748=CARTESIAN_POINT('Ctrl Pts',(-3.40908365400006,15.2,10.226966403));
#233749=CARTESIAN_POINT('Ctrl Pts',(-3.40908365400006,11.6,10.226966403));
#233750=CARTESIAN_POINT('Ctrl Pts',(-3.41057820200006,15.2,10.229104551));
#233751=CARTESIAN_POINT('Ctrl Pts',(-3.41057820200006,11.6,10.229104551));
#233752=CARTESIAN_POINT('Ctrl Pts',(-3.41207799700005,15.2,10.231246324));
#233753=CARTESIAN_POINT('Ctrl Pts',(-3.41207799700005,11.6,10.231246324));
#233754=CARTESIAN_POINT('Ctrl Pts',(-3.41358304100006,15.2,10.233391705));
#233755=CARTESIAN_POINT('Ctrl Pts',(-3.41358304100006,11.6,10.233391705));
#233756=CARTESIAN_POINT('Ctrl Pts',(-3.41509333200006,15.2,10.235540681));
#233757=CARTESIAN_POINT('Ctrl Pts',(-3.41509333200006,11.6,10.235540681));
#233758=CARTESIAN_POINT('Ctrl Pts',(-3.41660887500006,15.2,10.237693238));
#233759=CARTESIAN_POINT('Ctrl Pts',(-3.41660887500006,11.6,10.237693238));
#233760=CARTESIAN_POINT('Ctrl Pts',(-3.41812966600005,15.2,10.239849361));
#233761=CARTESIAN_POINT('Ctrl Pts',(-3.41812966600005,11.6,10.239849361));
#233762=CARTESIAN_POINT('Ctrl Pts',(-3.41965570900005,15.2,10.242009036));
#233763=CARTESIAN_POINT('Ctrl Pts',(-3.41965570900005,11.6,10.242009036));
#233764=CARTESIAN_POINT('Ctrl Pts',(-3.42118700500006,15.2,10.244172248));
#233765=CARTESIAN_POINT('Ctrl Pts',(-3.42118700500006,11.6,10.244172248));
#233766=CARTESIAN_POINT('Ctrl Pts',(-3.42272355100006,15.2,10.246338985));
#233767=CARTESIAN_POINT('Ctrl Pts',(-3.42272355100006,11.6,10.246338985));
#233768=CARTESIAN_POINT('Ctrl Pts',(-3.42426535200006,15.2,10.24850923));
#233769=CARTESIAN_POINT('Ctrl Pts',(-3.42426535200006,11.6,10.24850923));
#233770=CARTESIAN_POINT('Ctrl Pts',(-3.42581240600006,15.2,10.250682971));
#233771=CARTESIAN_POINT('Ctrl Pts',(-3.42581240600006,11.6,10.250682971));
#233772=CARTESIAN_POINT('Ctrl Pts',(-3.42736471300006,15.2,10.252860194));
#233773=CARTESIAN_POINT('Ctrl Pts',(-3.42736471300006,11.6,10.252860194));
#233774=CARTESIAN_POINT('Ctrl Pts',(-3.42892227700006,15.2,10.255040884));
#233775=CARTESIAN_POINT('Ctrl Pts',(-3.42892227700006,11.6,10.255040884));
#233776=CARTESIAN_POINT('Ctrl Pts',(-3.43048509600006,15.2,10.257225026));
#233777=CARTESIAN_POINT('Ctrl Pts',(-3.43048509600006,11.6,10.257225026));
#233778=CARTESIAN_POINT('Ctrl Pts',(-3.43205317100006,15.2,10.25941261));
#233779=CARTESIAN_POINT('Ctrl Pts',(-3.43205317100006,11.6,10.25941261));
#233780=CARTESIAN_POINT('Ctrl Pts',(-3.43362650400006,15.2,10.261603617));
#233781=CARTESIAN_POINT('Ctrl Pts',(-3.43362650400006,11.6,10.261603617));
#233782=CARTESIAN_POINT('Ctrl Pts',(-3.43520509300005,15.2,10.263798037));
#233783=CARTESIAN_POINT('Ctrl Pts',(-3.43520509300005,11.6,10.263798037));
#233784=CARTESIAN_POINT('Ctrl Pts',(-3.43678894100006,15.2,10.265995854));
#233785=CARTESIAN_POINT('Ctrl Pts',(-3.43678894100006,11.6,10.265995854));
#233786=CARTESIAN_POINT('Ctrl Pts',(-3.43837804700006,15.2,10.268197055));
#233787=CARTESIAN_POINT('Ctrl Pts',(-3.43837804700006,11.6,10.268197055));
#233788=CARTESIAN_POINT('Ctrl Pts',(-3.43997241300006,15.2,10.270401626));
#233789=CARTESIAN_POINT('Ctrl Pts',(-3.43997241300006,11.6,10.270401626));
#233790=CARTESIAN_POINT('Ctrl Pts',(-3.44157203800005,15.2,10.272609554));
#233791=CARTESIAN_POINT('Ctrl Pts',(-3.44157203800005,11.6,10.272609554));
#233792=CARTESIAN_POINT('Ctrl Pts',(-3.44317692300006,15.2,10.274820823));
#233793=CARTESIAN_POINT('Ctrl Pts',(-3.44317692300006,11.6,10.274820823));
#233794=CARTESIAN_POINT('Ctrl Pts',(-3.44478706900006,15.2,10.277035423));
#233795=CARTESIAN_POINT('Ctrl Pts',(-3.44478706900006,11.6,10.277035423));
#233796=CARTESIAN_POINT('Ctrl Pts',(-3.44640247700006,15.2,10.279253337));
#233797=CARTESIAN_POINT('Ctrl Pts',(-3.44640247700006,11.6,10.279253337));
#233798=CARTESIAN_POINT('Ctrl Pts',(-3.44802314600006,15.2,10.281474554));
#233799=CARTESIAN_POINT('Ctrl Pts',(-3.44802314600006,11.6,10.281474554));
#233800=CARTESIAN_POINT('Ctrl Pts',(-3.44964907800006,15.2,10.283699057));
#233801=CARTESIAN_POINT('Ctrl Pts',(-3.44964907800006,11.6,10.283699057));
#233802=CARTESIAN_POINT('Ctrl Pts',(-3.45128027200006,15.2,10.285926836));
#233803=CARTESIAN_POINT('Ctrl Pts',(-3.45128027200006,11.6,10.285926836));
#233804=CARTESIAN_POINT('Ctrl Pts',(-3.45291672900006,15.2,10.288157876));
#233805=CARTESIAN_POINT('Ctrl Pts',(-3.45291672900006,11.6,10.288157876));
#233806=CARTESIAN_POINT('Ctrl Pts',(-3.45455845100005,15.2,10.290392165));
#233807=CARTESIAN_POINT('Ctrl Pts',(-3.45455845100005,11.6,10.290392165));
#233808=CARTESIAN_POINT('Ctrl Pts',(-3.45620543600006,15.2,10.292629685));
#233809=CARTESIAN_POINT('Ctrl Pts',(-3.45620543600006,11.6,10.292629685));
#233810=CARTESIAN_POINT('Ctrl Pts',(-3.45785768600006,15.2,10.294870428));
#233811=CARTESIAN_POINT('Ctrl Pts',(-3.45785768600006,11.6,10.294870428));
#233812=CARTESIAN_POINT('Ctrl Pts',(-3.45951520100006,15.2,10.297114378));
#233813=CARTESIAN_POINT('Ctrl Pts',(-3.45951520100006,11.6,10.297114378));
#233814=CARTESIAN_POINT('Ctrl Pts',(-3.46117798100006,15.2,10.299361522));
#233815=CARTESIAN_POINT('Ctrl Pts',(-3.46117798100006,11.6,10.299361522));
#233816=CARTESIAN_POINT('Ctrl Pts',(-3.46284602800006,15.2,10.301611847));
#233817=CARTESIAN_POINT('Ctrl Pts',(-3.46284602800006,11.6,10.301611847));
#233818=CARTESIAN_POINT('Ctrl Pts',(-3.46451934000005,15.2,10.303865339));
#233819=CARTESIAN_POINT('Ctrl Pts',(-3.46451934000005,11.6,10.303865339));
#233820=CARTESIAN_POINT('Ctrl Pts',(-3.46619791900005,15.2,10.306121985));
#233821=CARTESIAN_POINT('Ctrl Pts',(-3.46619791900005,11.6,10.306121985));
#233822=CARTESIAN_POINT('Ctrl Pts',(-3.46788176500006,15.2,10.308381772));
#233823=CARTESIAN_POINT('Ctrl Pts',(-3.46788176500006,11.6,10.308381772));
#233824=CARTESIAN_POINT('Ctrl Pts',(-3.46957087800006,15.2,10.310644686));
#233825=CARTESIAN_POINT('Ctrl Pts',(-3.46957087800006,11.6,10.310644686));
#233826=CARTESIAN_POINT('Ctrl Pts',(-3.47126525900006,15.2,10.312910717));
#233827=CARTESIAN_POINT('Ctrl Pts',(-3.47126525900006,11.6,10.312910717));
#233828=CARTESIAN_POINT('Ctrl Pts',(-3.47296490800006,15.2,10.315179848));
#233829=CARTESIAN_POINT('Ctrl Pts',(-3.47296490800006,11.6,10.315179848));
#233830=CARTESIAN_POINT('Ctrl Pts',(-3.47466982500006,15.2,10.317452067));
#233831=CARTESIAN_POINT('Ctrl Pts',(-3.47466982500006,11.6,10.317452067));
#233832=CARTESIAN_POINT('Ctrl Pts',(-3.47638001000006,15.2,10.319727363));
#233833=CARTESIAN_POINT('Ctrl Pts',(-3.47638001000006,11.6,10.319727363));
#233834=CARTESIAN_POINT('Ctrl Pts',(-3.47809546500006,15.2,10.322005719));
#233835=CARTESIAN_POINT('Ctrl Pts',(-3.47809546500006,11.6,10.322005719));
#233836=CARTESIAN_POINT('Ctrl Pts',(-3.47981618900006,15.2,10.324287126));
#233837=CARTESIAN_POINT('Ctrl Pts',(-3.47981618900006,11.6,10.324287126));
#233838=CARTESIAN_POINT('Ctrl Pts',(-3.48154218300006,15.2,10.326571569));
#233839=CARTESIAN_POINT('Ctrl Pts',(-3.48154218300006,11.6,10.326571569));
#233840=CARTESIAN_POINT('Ctrl Pts',(-3.48327344600006,15.2,10.328859035));
#233841=CARTESIAN_POINT('Ctrl Pts',(-3.48327344600006,11.6,10.328859035));
#233842=CARTESIAN_POINT('Ctrl Pts',(-3.48500997900006,15.2,10.331149512));
#233843=CARTESIAN_POINT('Ctrl Pts',(-3.48500997900006,11.6,10.331149512));
#233844=CARTESIAN_POINT('Ctrl Pts',(-3.48675178200006,15.2,10.333442987));
#233845=CARTESIAN_POINT('Ctrl Pts',(-3.48675178200006,11.6,10.333442987));
#233846=CARTESIAN_POINT('Ctrl Pts',(-3.48849885700006,15.2,10.335739446));
#233847=CARTESIAN_POINT('Ctrl Pts',(-3.48849885700006,11.6,10.335739446));
#233848=CARTESIAN_POINT('Ctrl Pts',(-3.49025120200006,15.2,10.338038877));
#233849=CARTESIAN_POINT('Ctrl Pts',(-3.49025120200006,11.6,10.338038877));
#233850=CARTESIAN_POINT('Ctrl Pts',(-3.49200881900006,15.2,10.340341268));
#233851=CARTESIAN_POINT('Ctrl Pts',(-3.49200881900006,11.6,10.340341268));
#233852=CARTESIAN_POINT('Ctrl Pts',(-3.49377170500006,15.2,10.342646605));
#233853=CARTESIAN_POINT('Ctrl Pts',(-3.49377170500006,11.6,10.342646605));
#233854=CARTESIAN_POINT('Ctrl Pts',(-3.49553986400006,15.2,10.344954876));
#233855=CARTESIAN_POINT('Ctrl Pts',(-3.49553986400006,11.6,10.344954876));
#233856=CARTESIAN_POINT('Ctrl Pts',(-3.49731329400006,15.2,10.347266067));
#233857=CARTESIAN_POINT('Ctrl Pts',(-3.49731329400006,11.6,10.347266067));
#233858=CARTESIAN_POINT('Ctrl Pts',(-3.49909199600006,15.2,10.349580167));
#233859=CARTESIAN_POINT('Ctrl Pts',(-3.49909199600006,11.6,10.349580167));
#233860=CARTESIAN_POINT('Ctrl Pts',(-3.50087597000006,15.2,10.351897163));
#233861=CARTESIAN_POINT('Ctrl Pts',(-3.50087597000006,11.6,10.351897163));
#233862=CARTESIAN_POINT('Ctrl Pts',(-3.50266521700005,15.2,10.354217043));
#233863=CARTESIAN_POINT('Ctrl Pts',(-3.50266521700005,11.6,10.354217043));
#233864=CARTESIAN_POINT('Ctrl Pts',(-3.50445973500006,15.2,10.356539792));
#233865=CARTESIAN_POINT('Ctrl Pts',(-3.50445973500006,11.6,10.356539792));
#233866=CARTESIAN_POINT('Ctrl Pts',(-3.50625952600006,15.2,10.3588654));
#233867=CARTESIAN_POINT('Ctrl Pts',(-3.50625952600006,11.6,10.3588654));
#233868=CARTESIAN_POINT('Ctrl Pts',(-3.50806458900006,15.2,10.361193853));
#233869=CARTESIAN_POINT('Ctrl Pts',(-3.50806458900006,11.6,10.361193853));
#233870=CARTESIAN_POINT('Ctrl Pts',(-3.50987492600006,15.2,10.363525139));
#233871=CARTESIAN_POINT('Ctrl Pts',(-3.50987492600006,11.6,10.363525139));
#233872=CARTESIAN_POINT('Ctrl Pts',(-3.51169053400006,15.2,10.365859245));
#233873=CARTESIAN_POINT('Ctrl Pts',(-3.51169053400006,11.6,10.365859245));
#233874=CARTESIAN_POINT('Ctrl Pts',(-3.51351141600006,15.2,10.36819616));
#233875=CARTESIAN_POINT('Ctrl Pts',(-3.51351141600006,11.6,10.36819616));
#233876=CARTESIAN_POINT('Ctrl Pts',(-3.51533757100006,15.2,10.370535871));
#233877=CARTESIAN_POINT('Ctrl Pts',(-3.51533757100006,11.6,10.370535871));
#233878=CARTESIAN_POINT('Ctrl Pts',(-3.51716899900006,15.2,10.372878364));
#233879=CARTESIAN_POINT('Ctrl Pts',(-3.51716899900006,11.6,10.372878364));
#233880=CARTESIAN_POINT('Ctrl Pts',(-3.51900570000006,15.2,10.375223629));
#233881=CARTESIAN_POINT('Ctrl Pts',(-3.51900570000006,11.6,10.375223629));
#233882=CARTESIAN_POINT('Ctrl Pts',(-3.52084767500005,15.2,10.377571653));
#233883=CARTESIAN_POINT('Ctrl Pts',(-3.52084767500005,11.6,10.377571653));
#233884=CARTESIAN_POINT('Ctrl Pts',(-3.52269492200006,15.2,10.379922423));
#233885=CARTESIAN_POINT('Ctrl Pts',(-3.52269492200006,11.6,10.379922423));
#233886=CARTESIAN_POINT('Ctrl Pts',(-3.52454744400006,15.2,10.382275926));
#233887=CARTESIAN_POINT('Ctrl Pts',(-3.52454744400006,11.6,10.382275926));
#233888=CARTESIAN_POINT('Ctrl Pts',(-3.52640523800006,15.2,10.384632152));
#233889=CARTESIAN_POINT('Ctrl Pts',(-3.52640523800006,11.6,10.384632152));
#233890=CARTESIAN_POINT('Ctrl Pts',(-3.52826830500006,15.2,10.386991087));
#233891=CARTESIAN_POINT('Ctrl Pts',(-3.52826830500006,11.6,10.386991087));
#233892=CARTESIAN_POINT('Ctrl Pts',(-3.53013664600006,15.2,10.389352721));
#233893=CARTESIAN_POINT('Ctrl Pts',(-3.53013664600006,11.6,10.389352721));
#233894=CARTESIAN_POINT('Ctrl Pts',(-3.53201026100006,15.2,10.391717039));
#233895=CARTESIAN_POINT('Ctrl Pts',(-3.53201026100006,11.6,10.391717039));
#233896=CARTESIAN_POINT('Ctrl Pts',(-3.53388914900005,15.2,10.39408403));
#233897=CARTESIAN_POINT('Ctrl Pts',(-3.53388914900005,11.6,10.39408403));
#233898=CARTESIAN_POINT('Ctrl Pts',(-3.53577331100006,15.2,10.396453683));
#233899=CARTESIAN_POINT('Ctrl Pts',(-3.53577331100006,11.6,10.396453683));
#233900=CARTESIAN_POINT('Ctrl Pts',(-3.53766274500006,15.2,10.398825984));
#233901=CARTESIAN_POINT('Ctrl Pts',(-3.53766274500006,11.6,10.398825984));
#233902=CARTESIAN_POINT('Ctrl Pts',(-3.53955745300006,15.2,10.401200923));
#233903=CARTESIAN_POINT('Ctrl Pts',(-3.53955745300006,11.6,10.401200923));
#233904=CARTESIAN_POINT('Ctrl Pts',(-3.54145743500006,15.2,10.403578487));
#233905=CARTESIAN_POINT('Ctrl Pts',(-3.54145743500006,11.6,10.403578487));
#233906=CARTESIAN_POINT('Ctrl Pts',(-3.54336269000005,15.2,10.405958664));
#233907=CARTESIAN_POINT('Ctrl Pts',(-3.54336269000005,11.6,10.405958664));
#233908=CARTESIAN_POINT('Ctrl Pts',(-3.54527321800005,15.2,10.408341441));
#233909=CARTESIAN_POINT('Ctrl Pts',(-3.54527321800005,11.6,10.408341441));
#233910=CARTESIAN_POINT('Ctrl Pts',(-3.54718901800006,15.2,10.410726808));
#233911=CARTESIAN_POINT('Ctrl Pts',(-3.54718901800006,11.6,10.410726808));
#233912=CARTESIAN_POINT('Ctrl Pts',(-3.54911009300006,15.2,10.413114752));
#233913=CARTESIAN_POINT('Ctrl Pts',(-3.54911009300006,11.6,10.413114752));
#233914=CARTESIAN_POINT('Ctrl Pts',(-3.55103644000006,15.2,10.415505261));
#233915=CARTESIAN_POINT('Ctrl Pts',(-3.55103644000006,11.6,10.415505261));
#233916=CARTESIAN_POINT('Ctrl Pts',(-3.55296806000006,15.2,10.417898323));
#233917=CARTESIAN_POINT('Ctrl Pts',(-3.55296806000006,11.6,10.417898323));
#233918=CARTESIAN_POINT('Ctrl Pts',(-3.55490495300006,15.2,10.420293927));
#233919=CARTESIAN_POINT('Ctrl Pts',(-3.55490495300006,11.6,10.420293927));
#233920=CARTESIAN_POINT('Ctrl Pts',(-3.55684711800006,15.2,10.422692061));
#233921=CARTESIAN_POINT('Ctrl Pts',(-3.55684711800006,11.6,10.422692061));
#233922=CARTESIAN_POINT('Ctrl Pts',(-3.55879455700006,15.2,10.425092713));
#233923=CARTESIAN_POINT('Ctrl Pts',(-3.55879455700006,11.6,10.425092713));
#233924=CARTESIAN_POINT('Ctrl Pts',(-3.56074726700006,15.2,10.427495872));
#233925=CARTESIAN_POINT('Ctrl Pts',(-3.56074726700006,11.6,10.427495872));
#233926=CARTESIAN_POINT('Ctrl Pts',(-3.56270525100006,15.2,10.429901523));
#233927=CARTESIAN_POINT('Ctrl Pts',(-3.56270525100006,11.6,10.429901523));
#233928=CARTESIAN_POINT('Ctrl Pts',(-3.56466850500006,15.2,10.432309659));
#233929=CARTESIAN_POINT('Ctrl Pts',(-3.56466850500006,11.6,10.432309659));
#233930=CARTESIAN_POINT('Ctrl Pts',(-3.56663703300006,15.2,10.434720265));
#233931=CARTESIAN_POINT('Ctrl Pts',(-3.56663703300006,11.6,10.434720265));
#233932=CARTESIAN_POINT('Ctrl Pts',(-3.56861083200006,15.2,10.437133332));
#233933=CARTESIAN_POINT('Ctrl Pts',(-3.56861083200006,11.6,10.437133332));
#233934=CARTESIAN_POINT('Ctrl Pts',(-3.57058990200006,15.2,10.439548846));
#233935=CARTESIAN_POINT('Ctrl Pts',(-3.57058990200006,11.6,10.439548846));
#233936=CARTESIAN_POINT('Ctrl Pts',(-3.57257424400006,15.2,10.441966796));
#233937=CARTESIAN_POINT('Ctrl Pts',(-3.57257424400006,11.6,10.441966796));
#233938=CARTESIAN_POINT('Ctrl Pts',(-3.57456385800006,15.2,10.44438717));
#233939=CARTESIAN_POINT('Ctrl Pts',(-3.57456385800006,11.6,10.44438717));
#233940=CARTESIAN_POINT('Ctrl Pts',(-3.57655874300006,15.2,10.446809958));
#233941=CARTESIAN_POINT('Ctrl Pts',(-3.57655874300006,11.6,10.446809958));
#233942=CARTESIAN_POINT('Ctrl Pts',(-3.57855889700006,15.2,10.449235148));
#233943=CARTESIAN_POINT('Ctrl Pts',(-3.57855889700006,11.6,10.449235148));
#233944=CARTESIAN_POINT('Ctrl Pts',(-3.58056432400006,15.2,10.451662728));
#233945=CARTESIAN_POINT('Ctrl Pts',(-3.58056432400006,11.6,10.451662728));
#233946=CARTESIAN_POINT('Ctrl Pts',(-3.58257502000006,15.2,10.454092686));
#233947=CARTESIAN_POINT('Ctrl Pts',(-3.58257502000006,11.6,10.454092686));
#233948=CARTESIAN_POINT('Ctrl Pts',(-3.58459098700005,15.2,10.456525011));
#233949=CARTESIAN_POINT('Ctrl Pts',(-3.58459098700005,11.6,10.456525011));
#233950=CARTESIAN_POINT('Ctrl Pts',(-3.58661222400006,15.2,10.458959692));
#233951=CARTESIAN_POINT('Ctrl Pts',(-3.58661222400006,11.6,10.458959692));
#233952=CARTESIAN_POINT('Ctrl Pts',(-3.58863873100006,15.2,10.461396717));
#233953=CARTESIAN_POINT('Ctrl Pts',(-3.58863873100006,11.6,10.461396717));
#233954=CARTESIAN_POINT('Ctrl Pts',(-3.59067050700006,15.2,10.463836075));
#233955=CARTESIAN_POINT('Ctrl Pts',(-3.59067050700006,11.6,10.463836075));
#233956=CARTESIAN_POINT('Ctrl Pts',(-3.59270755300006,15.2,10.466277755));
#233957=CARTESIAN_POINT('Ctrl Pts',(-3.59270755300006,11.6,10.466277755));
#233958=CARTESIAN_POINT('Ctrl Pts',(-3.59474986600006,15.2,10.468721746));
#233959=CARTESIAN_POINT('Ctrl Pts',(-3.59474986600006,11.6,10.468721746));
#233960=CARTESIAN_POINT('Ctrl Pts',(-3.59679745000006,15.2,10.471168035));
#233961=CARTESIAN_POINT('Ctrl Pts',(-3.59679745000006,11.6,10.471168035));
#233962=CARTESIAN_POINT('Ctrl Pts',(-3.59885030100005,15.2,10.473616611));
#233963=CARTESIAN_POINT('Ctrl Pts',(-3.59885030100005,11.6,10.473616611));
#233964=CARTESIAN_POINT('Ctrl Pts',(-3.60090842000006,15.2,10.476067465));
#233965=CARTESIAN_POINT('Ctrl Pts',(-3.60090842000006,11.6,10.476067465));
#233966=CARTESIAN_POINT('Ctrl Pts',(-3.60297180800006,15.2,10.478520583));
#233967=CARTESIAN_POINT('Ctrl Pts',(-3.60297180800006,11.6,10.478520583));
#233968=CARTESIAN_POINT('Ctrl Pts',(-3.60504046200006,15.2,10.480975954));
#233969=CARTESIAN_POINT('Ctrl Pts',(-3.60504046200006,11.6,10.480975954));
#233970=CARTESIAN_POINT('Ctrl Pts',(-3.60711438400006,15.2,10.48343357));
#233971=CARTESIAN_POINT('Ctrl Pts',(-3.60711438400006,11.6,10.48343357));
#233972=CARTESIAN_POINT('Ctrl Pts',(-3.60919357400006,15.2,10.485893416));
#233973=CARTESIAN_POINT('Ctrl Pts',(-3.60919357400006,11.6,10.485893416));
#233974=CARTESIAN_POINT('Ctrl Pts',(-3.61127802800006,15.2,10.488355482));
#233975=CARTESIAN_POINT('Ctrl Pts',(-3.61127802800006,11.6,10.488355482));
#233976=CARTESIAN_POINT('Ctrl Pts',(-3.61336775000006,15.2,10.490819758));
#233977=CARTESIAN_POINT('Ctrl Pts',(-3.61336775000006,11.6,10.490819758));
#233978=CARTESIAN_POINT('Ctrl Pts',(-3.61546273700006,15.2,10.493286233));
#233979=CARTESIAN_POINT('Ctrl Pts',(-3.61546273700006,11.6,10.493286233));
#233980=CARTESIAN_POINT('Ctrl Pts',(-3.61756298900006,15.2,10.495754894));
#233981=CARTESIAN_POINT('Ctrl Pts',(-3.61756298900006,11.6,10.495754894));
#233982=CARTESIAN_POINT('Ctrl Pts',(-3.61966850700006,15.2,10.498225732));
#233983=CARTESIAN_POINT('Ctrl Pts',(-3.61966850700006,11.6,10.498225732));
#233984=CARTESIAN_POINT('Ctrl Pts',(-3.62177928800006,15.2,10.500698735));
#233985=CARTESIAN_POINT('Ctrl Pts',(-3.62177928800006,11.6,10.500698735));
#233986=CARTESIAN_POINT('Ctrl Pts',(-3.62389533500005,15.2,10.503173891));
#233987=CARTESIAN_POINT('Ctrl Pts',(-3.62389533500005,11.6,10.503173891));
#233988=CARTESIAN_POINT('Ctrl Pts',(-3.62601664500006,15.2,10.505651191));
#233989=CARTESIAN_POINT('Ctrl Pts',(-3.62601664500006,11.6,10.505651191));
#233990=CARTESIAN_POINT('Ctrl Pts',(-3.62814321900006,15.2,10.508130623));
#233991=CARTESIAN_POINT('Ctrl Pts',(-3.62814321900006,11.6,10.508130623));
#233992=CARTESIAN_POINT('Ctrl Pts',(-3.63027505500006,15.2,10.510612176));
#233993=CARTESIAN_POINT('Ctrl Pts',(-3.63027505500006,11.6,10.510612176));
#233994=CARTESIAN_POINT('Ctrl Pts',(-3.63241215500006,15.2,10.513095839));
#233995=CARTESIAN_POINT('Ctrl Pts',(-3.63241215500006,11.6,10.513095839));
#233996=CARTESIAN_POINT('Ctrl Pts',(-3.63455451700006,15.2,10.515581602));
#233997=CARTESIAN_POINT('Ctrl Pts',(-3.63455451700006,11.6,10.515581602));
#233998=CARTESIAN_POINT('Ctrl Pts',(-3.63670214100006,15.2,10.518069453));
#233999=CARTESIAN_POINT('Ctrl Pts',(-3.63670214100006,11.6,10.518069453));
#234000=CARTESIAN_POINT('Ctrl Pts',(-3.63885502600006,15.2,10.520559382));
#234001=CARTESIAN_POINT('Ctrl Pts',(-3.63885502600006,11.6,10.520559382));
#234002=CARTESIAN_POINT('Ctrl Pts',(-3.64101317200006,15.2,10.523051378));
#234003=CARTESIAN_POINT('Ctrl Pts',(-3.64101317200006,11.6,10.523051378));
#234004=CARTESIAN_POINT('Ctrl Pts',(-3.64317657800005,15.2,10.525545429));
#234005=CARTESIAN_POINT('Ctrl Pts',(-3.64317657800005,11.6,10.525545429));
#234006=CARTESIAN_POINT('Ctrl Pts',(-3.64534524400006,15.2,10.528041525));
#234007=CARTESIAN_POINT('Ctrl Pts',(-3.64534524400006,11.6,10.528041525));
#234008=CARTESIAN_POINT('Ctrl Pts',(-3.64751916900006,15.2,10.530539657));
#234009=CARTESIAN_POINT('Ctrl Pts',(-3.64751916900006,11.6,10.530539657));
#234010=CARTESIAN_POINT('Ctrl Pts',(-3.64969835400006,15.2,10.533039813));
#234011=CARTESIAN_POINT('Ctrl Pts',(-3.64969835400006,11.6,10.533039813));
#234012=CARTESIAN_POINT('Ctrl Pts',(-3.65188279700006,15.2,10.53554198));
#234013=CARTESIAN_POINT('Ctrl Pts',(-3.65188279700006,11.6,10.53554198));
#234014=CARTESIAN_POINT('Ctrl Pts',(-3.65407249900006,15.2,10.538046151));
#234015=CARTESIAN_POINT('Ctrl Pts',(-3.65407249900006,11.6,10.538046151));
#234016=CARTESIAN_POINT('Ctrl Pts',(-3.65626745700006,15.2,10.540552313));
#234017=CARTESIAN_POINT('Ctrl Pts',(-3.65626745700006,11.6,10.540552313));
#234018=CARTESIAN_POINT('Ctrl Pts',(-3.65846767300006,15.2,10.543060457));
#234019=CARTESIAN_POINT('Ctrl Pts',(-3.65846767300006,11.6,10.543060457));
#234020=CARTESIAN_POINT('Ctrl Pts',(-3.66067314500006,15.2,10.54557057));
#234021=CARTESIAN_POINT('Ctrl Pts',(-3.66067314500006,11.6,10.54557057));
#234022=CARTESIAN_POINT('Ctrl Pts',(-3.66288387400005,15.2,10.548082643));
#234023=CARTESIAN_POINT('Ctrl Pts',(-3.66288387400005,11.6,10.548082643));
#234024=CARTESIAN_POINT('Ctrl Pts',(-3.66509985800006,15.2,10.550596665));
#234025=CARTESIAN_POINT('Ctrl Pts',(-3.66509985800006,11.6,10.550596665));
#234026=CARTESIAN_POINT('Ctrl Pts',(-3.66732109600005,15.2,10.553112627));
#234027=CARTESIAN_POINT('Ctrl Pts',(-3.66732109600005,11.6,10.553112627));
#234028=CARTESIAN_POINT('Ctrl Pts',(-3.66954759000006,15.2,10.555630515));
#234029=CARTESIAN_POINT('Ctrl Pts',(-3.66954759000006,11.6,10.555630515));
#234030=CARTESIAN_POINT('Ctrl Pts',(-3.67177933600006,15.2,10.558150322));
#234031=CARTESIAN_POINT('Ctrl Pts',(-3.67177933600006,11.6,10.558150322));
#234032=CARTESIAN_POINT('Ctrl Pts',(-3.67401633700006,15.2,10.560672036));
#234033=CARTESIAN_POINT('Ctrl Pts',(-3.67401633700006,11.6,10.560672036));
#234034=CARTESIAN_POINT('Ctrl Pts',(-3.67625858900006,15.2,10.563195645));
#234035=CARTESIAN_POINT('Ctrl Pts',(-3.67625858900006,11.6,10.563195645));
#234036=CARTESIAN_POINT('Ctrl Pts',(-3.67850609400006,15.2,10.565721141));
#234037=CARTESIAN_POINT('Ctrl Pts',(-3.67850609400006,11.6,10.565721141));
#234038=CARTESIAN_POINT('Ctrl Pts',(-3.68075885100006,15.2,10.568248513));
#234039=CARTESIAN_POINT('Ctrl Pts',(-3.68075885100006,11.6,10.568248513));
#234040=CARTESIAN_POINT('Ctrl Pts',(-3.68301685900006,15.2,10.570777751));
#234041=CARTESIAN_POINT('Ctrl Pts',(-3.68301685900006,11.6,10.570777751));
#234042=CARTESIAN_POINT('Ctrl Pts',(-3.68528011600006,15.2,10.573308843));
#234043=CARTESIAN_POINT('Ctrl Pts',(-3.68528011600006,11.6,10.573308843));
#234044=CARTESIAN_POINT('Ctrl Pts',(-3.68754862400006,15.2,10.575841779));
#234045=CARTESIAN_POINT('Ctrl Pts',(-3.68754862400006,11.6,10.575841779));
#234046=CARTESIAN_POINT('Ctrl Pts',(-3.68982238000005,15.2,10.57837655));
#234047=CARTESIAN_POINT('Ctrl Pts',(-3.68982238000005,11.6,10.57837655));
#234048=CARTESIAN_POINT('Ctrl Pts',(-3.69210138500006,15.2,10.580913144));
#234049=CARTESIAN_POINT('Ctrl Pts',(-3.69210138500006,11.6,10.580913144));
#234050=CARTESIAN_POINT('Ctrl Pts',(-3.69438563800006,15.2,10.583451552));
#234051=CARTESIAN_POINT('Ctrl Pts',(-3.69438563800006,11.6,10.583451552));
#234052=CARTESIAN_POINT('Ctrl Pts',(-3.69667513900006,15.2,10.585991762));
#234053=CARTESIAN_POINT('Ctrl Pts',(-3.69667513900006,11.6,10.585991762));
#234054=CARTESIAN_POINT('Ctrl Pts',(-3.69896988600006,15.2,10.588533766));
#234055=CARTESIAN_POINT('Ctrl Pts',(-3.69896988600006,11.6,10.588533766));
#234056=CARTESIAN_POINT('Ctrl Pts',(-3.70126987900006,15.2,10.591077552));
#234057=CARTESIAN_POINT('Ctrl Pts',(-3.70126987900006,11.6,10.591077552));
#234058=CARTESIAN_POINT('Ctrl Pts',(-3.70357511700006,15.2,10.593623111));
#234059=CARTESIAN_POINT('Ctrl Pts',(-3.70357511700006,11.6,10.593623111));
#234060=CARTESIAN_POINT('Ctrl Pts',(-3.70588560000006,15.2,10.596170432));
#234061=CARTESIAN_POINT('Ctrl Pts',(-3.70588560000006,11.6,10.596170432));
#234062=CARTESIAN_POINT('Ctrl Pts',(-3.70820132700006,15.2,10.598719505));
#234063=CARTESIAN_POINT('Ctrl Pts',(-3.70820132700006,11.6,10.598719505));
#234064=CARTESIAN_POINT('Ctrl Pts',(-3.71052229700005,15.2,10.60127032));
#234065=CARTESIAN_POINT('Ctrl Pts',(-3.71052229700005,11.6,10.60127032));
#234066=CARTESIAN_POINT('Ctrl Pts',(-3.71284850900006,15.2,10.603822866));
#234067=CARTESIAN_POINT('Ctrl Pts',(-3.71284850900006,11.6,10.603822866));
#234068=CARTESIAN_POINT('Ctrl Pts',(-3.71517996400006,15.2,10.606377133));
#234069=CARTESIAN_POINT('Ctrl Pts',(-3.71517996400006,11.6,10.606377133));
#234070=CARTESIAN_POINT('Ctrl Pts',(-3.71751666100006,15.2,10.608933113));
#234071=CARTESIAN_POINT('Ctrl Pts',(-3.71751666100006,11.6,10.608933113));
#234072=CARTESIAN_POINT('Ctrl Pts',(-3.71985859700006,15.2,10.611490792));
#234073=CARTESIAN_POINT('Ctrl Pts',(-3.71985859700006,11.6,10.611490792));
#234074=CARTESIAN_POINT('Ctrl Pts',(-3.72220577200006,15.2,10.614050164));
#234075=CARTESIAN_POINT('Ctrl Pts',(-3.72220577200006,11.6,10.614050164));
#234076=CARTESIAN_POINT('Ctrl Pts',(-3.72455818800006,15.2,10.616611217));
#234077=CARTESIAN_POINT('Ctrl Pts',(-3.72455818800006,11.6,10.616611217));
#234078=CARTESIAN_POINT('Ctrl Pts',(-3.72691584200005,15.2,10.619173941));
#234079=CARTESIAN_POINT('Ctrl Pts',(-3.72691584200005,11.6,10.619173941));
#234080=CARTESIAN_POINT('Ctrl Pts',(-3.72927873300006,15.2,10.621738325));
#234081=CARTESIAN_POINT('Ctrl Pts',(-3.72927873300006,11.6,10.621738325));
#234082=CARTESIAN_POINT('Ctrl Pts',(-3.73164686200006,15.2,10.624304361));
#234083=CARTESIAN_POINT('Ctrl Pts',(-3.73164686200006,11.6,10.624304361));
#234084=CARTESIAN_POINT('Ctrl Pts',(-3.73402022600006,15.2,10.626872037));
#234085=CARTESIAN_POINT('Ctrl Pts',(-3.73402022600006,11.6,10.626872037));
#234086=CARTESIAN_POINT('Ctrl Pts',(-3.73639882600005,15.2,10.629441345));
#234087=CARTESIAN_POINT('Ctrl Pts',(-3.73639882600005,11.6,10.629441345));
#234088=CARTESIAN_POINT('Ctrl Pts',(-3.73878266100006,15.2,10.632012275));
#234089=CARTESIAN_POINT('Ctrl Pts',(-3.73878266100006,11.6,10.632012275));
#234090=CARTESIAN_POINT('Ctrl Pts',(-3.74117172900006,15.2,10.634584815));
#234091=CARTESIAN_POINT('Ctrl Pts',(-3.74117172900006,11.6,10.634584815));
#234092=CARTESIAN_POINT('Ctrl Pts',(-3.74356603100006,15.2,10.637158957));
#234093=CARTESIAN_POINT('Ctrl Pts',(-3.74356603100006,11.6,10.637158957));
#234094=CARTESIAN_POINT('Ctrl Pts',(-3.74596556400006,15.2,10.63973469));
#234095=CARTESIAN_POINT('Ctrl Pts',(-3.74596556400006,11.6,10.63973469));
#234096=CARTESIAN_POINT('Ctrl Pts',(-3.74837033000006,15.2,10.642312005));
#234097=CARTESIAN_POINT('Ctrl Pts',(-3.74837033000006,11.6,10.642312005));
#234098=CARTESIAN_POINT('Ctrl Pts',(-3.75078032700006,15.2,10.644890891));
#234099=CARTESIAN_POINT('Ctrl Pts',(-3.75078032700006,11.6,10.644890891));
#234100=CARTESIAN_POINT('Ctrl Pts',(-3.75319555300006,15.2,10.647471339));
#234101=CARTESIAN_POINT('Ctrl Pts',(-3.75319555300006,11.6,10.647471339));
#234102=CARTESIAN_POINT('Ctrl Pts',(-3.75561600800006,15.2,10.650053339));
#234103=CARTESIAN_POINT('Ctrl Pts',(-3.75561600800006,11.6,10.650053339));
#234104=CARTESIAN_POINT('Ctrl Pts',(-3.75804169300006,15.2,10.652636882));
#234105=CARTESIAN_POINT('Ctrl Pts',(-3.75804169300006,11.6,10.652636882));
#234106=CARTESIAN_POINT('Ctrl Pts',(-3.76047260500005,15.2,10.655221957));
#234107=CARTESIAN_POINT('Ctrl Pts',(-3.76047260500005,11.6,10.655221957));
#234108=CARTESIAN_POINT('Ctrl Pts',(-3.76290874200006,15.2,10.657808555));
#234109=CARTESIAN_POINT('Ctrl Pts',(-3.76290874200006,11.6,10.657808555));
#234110=CARTESIAN_POINT('Ctrl Pts',(-3.76535010600006,15.2,10.660396666));
#234111=CARTESIAN_POINT('Ctrl Pts',(-3.76535010600006,11.6,10.660396666));
#234112=CARTESIAN_POINT('Ctrl Pts',(-3.76779669600006,15.2,10.66298628));
#234113=CARTESIAN_POINT('Ctrl Pts',(-3.76779669600006,11.6,10.66298628));
#234114=CARTESIAN_POINT('Ctrl Pts',(-3.77024850900006,15.2,10.665577388));
#234115=CARTESIAN_POINT('Ctrl Pts',(-3.77024850900006,11.6,10.665577388));
#234116=CARTESIAN_POINT('Ctrl Pts',(-3.77270554500006,15.2,10.66816998));
#234117=CARTESIAN_POINT('Ctrl Pts',(-3.77270554500006,11.6,10.66816998));
#234118=CARTESIAN_POINT('Ctrl Pts',(-3.77516780600006,15.2,10.670764045));
#234119=CARTESIAN_POINT('Ctrl Pts',(-3.77516780600006,11.6,10.670764045));
#234120=CARTESIAN_POINT('Ctrl Pts',(-3.77763528700005,15.2,10.673359576));
#234121=CARTESIAN_POINT('Ctrl Pts',(-3.77763528700005,11.6,10.673359576));
#234122=CARTESIAN_POINT('Ctrl Pts',(-3.78010798800006,15.2,10.67595656));
#234123=CARTESIAN_POINT('Ctrl Pts',(-3.78010798800006,11.6,10.67595656));
#234124=CARTESIAN_POINT('Ctrl Pts',(-3.78258591000006,15.2,10.678554992));
#234125=CARTESIAN_POINT('Ctrl Pts',(-3.78258591000006,11.6,10.678554992));
#234126=CARTESIAN_POINT('Ctrl Pts',(-3.78506905100005,15.2,10.681154858));
#234127=CARTESIAN_POINT('Ctrl Pts',(-3.78506905100005,11.6,10.681154858));
#234128=CARTESIAN_POINT('Ctrl Pts',(-3.78755741000006,15.2,10.68375615));
#234129=CARTESIAN_POINT('Ctrl Pts',(-3.78755741000006,11.6,10.68375615));
#234130=CARTESIAN_POINT('Ctrl Pts',(-3.79005098600006,15.2,10.686358859));
#234131=CARTESIAN_POINT('Ctrl Pts',(-3.79005098600006,11.6,10.686358859));
#234132=CARTESIAN_POINT('Ctrl Pts',(-3.79254977900006,15.2,10.688962975));
#234133=CARTESIAN_POINT('Ctrl Pts',(-3.79254977900006,11.6,10.688962975));
#234134=CARTESIAN_POINT('Ctrl Pts',(-3.79505378700006,15.2,10.691568489));
#234135=CARTESIAN_POINT('Ctrl Pts',(-3.79505378700006,11.6,10.691568489));
#234136=CARTESIAN_POINT('Ctrl Pts',(-3.79756300900006,15.2,10.69417539));
#234137=CARTESIAN_POINT('Ctrl Pts',(-3.79756300900006,11.6,10.69417539));
#234138=CARTESIAN_POINT('Ctrl Pts',(-3.80007744600006,15.2,10.696783671));
#234139=CARTESIAN_POINT('Ctrl Pts',(-3.80007744600006,11.6,10.696783671));
#234140=CARTESIAN_POINT('Ctrl Pts',(-3.80259709500006,15.2,10.69939332));
#234141=CARTESIAN_POINT('Ctrl Pts',(-3.80259709500006,11.6,10.69939332));
#234142=CARTESIAN_POINT('Ctrl Pts',(-3.80512195600006,15.2,10.702004329));
#234143=CARTESIAN_POINT('Ctrl Pts',(-3.80512195600006,11.6,10.702004329));
#234144=CARTESIAN_POINT('Ctrl Pts',(-3.80765202800006,15.2,10.704616688));
#234145=CARTESIAN_POINT('Ctrl Pts',(-3.80765202800006,11.6,10.704616688));
#234146=CARTESIAN_POINT('Ctrl Pts',(-3.81018731000006,15.2,10.707230387));
#234147=CARTESIAN_POINT('Ctrl Pts',(-3.81018731000006,11.6,10.707230387));
#234148=CARTESIAN_POINT('Ctrl Pts',(-3.81272780000006,15.2,10.709845418));
#234149=CARTESIAN_POINT('Ctrl Pts',(-3.81272780000006,11.6,10.709845418));
#234150=CARTESIAN_POINT('Ctrl Pts',(-3.81527349900006,15.2,10.712461771));
#234151=CARTESIAN_POINT('Ctrl Pts',(-3.81527349900006,11.6,10.712461771));
#234152=CARTESIAN_POINT('Ctrl Pts',(-3.81782440500006,15.2,10.715079436));
#234153=CARTESIAN_POINT('Ctrl Pts',(-3.81782440500006,11.6,10.715079436));
#234154=CARTESIAN_POINT('Ctrl Pts',(-3.82038051600006,15.2,10.717698406));
#234155=CARTESIAN_POINT('Ctrl Pts',(-3.82038051600006,11.6,10.717698406));
#234156=CARTESIAN_POINT('Ctrl Pts',(-3.82294183300006,15.2,10.720318668));
#234157=CARTESIAN_POINT('Ctrl Pts',(-3.82294183300006,11.6,10.720318668));
#234158=CARTESIAN_POINT('Ctrl Pts',(-3.82550835500005,15.2,10.722940216));
#234159=CARTESIAN_POINT('Ctrl Pts',(-3.82550835500005,11.6,10.722940216));
#234160=CARTESIAN_POINT('Ctrl Pts',(-3.82808007900006,15.2,10.725563037));
#234161=CARTESIAN_POINT('Ctrl Pts',(-3.82808007900006,11.6,10.725563037));
#234162=CARTESIAN_POINT('Ctrl Pts',(-3.83065700500006,15.2,10.728187127));
#234163=CARTESIAN_POINT('Ctrl Pts',(-3.83065700500006,11.6,10.728187127));
#234164=CARTESIAN_POINT('Ctrl Pts',(-3.83323913400006,15.2,10.730812472));
#234165=CARTESIAN_POINT('Ctrl Pts',(-3.83323913400006,11.6,10.730812472));
#234166=CARTESIAN_POINT('Ctrl Pts',(-3.83582646100006,15.2,10.733439064));
#234167=CARTESIAN_POINT('Ctrl Pts',(-3.83582646100006,11.6,10.733439064));
#234168=CARTESIAN_POINT('Ctrl Pts',(-3.83841898900006,15.2,10.736066894));
#234169=CARTESIAN_POINT('Ctrl Pts',(-3.83841898900006,11.6,10.736066894));
#234170=CARTESIAN_POINT('Ctrl Pts',(-3.84101671400006,15.2,10.738695954));
#234171=CARTESIAN_POINT('Ctrl Pts',(-3.84101671400006,11.6,10.738695954));
#234172=CARTESIAN_POINT('Ctrl Pts',(-3.84361963500006,15.2,10.741326232));
#234173=CARTESIAN_POINT('Ctrl Pts',(-3.84361963500006,11.6,10.741326232));
#234174=CARTESIAN_POINT('Ctrl Pts',(-3.84622775400006,15.2,10.743957722));
#234175=CARTESIAN_POINT('Ctrl Pts',(-3.84622775400006,11.6,10.743957722));
#234176=CARTESIAN_POINT('Ctrl Pts',(-3.84884106800006,15.2,10.746590414));
#234177=CARTESIAN_POINT('Ctrl Pts',(-3.84884106800006,11.6,10.746590414));
#234178=CARTESIAN_POINT('Ctrl Pts',(-3.85145957500006,15.2,10.749224298));
#234179=CARTESIAN_POINT('Ctrl Pts',(-3.85145957500006,11.6,10.749224298));
#234180=CARTESIAN_POINT('Ctrl Pts',(-3.85408327600006,15.2,10.751859366));
#234181=CARTESIAN_POINT('Ctrl Pts',(-3.85408327600006,11.6,10.751859366));
#234182=CARTESIAN_POINT('Ctrl Pts',(-3.85671217000006,15.2,10.754495608));
#234183=CARTESIAN_POINT('Ctrl Pts',(-3.85671217000006,11.6,10.754495608));
#234184=CARTESIAN_POINT('Ctrl Pts',(-3.85934625300006,15.2,10.757133016));
#234185=CARTESIAN_POINT('Ctrl Pts',(-3.85934625300006,11.6,10.757133016));
#234186=CARTESIAN_POINT('Ctrl Pts',(-3.86198552700006,15.2,10.759771578));
#234187=CARTESIAN_POINT('Ctrl Pts',(-3.86198552700006,11.6,10.759771578));
#234188=CARTESIAN_POINT('Ctrl Pts',(-3.86462998900006,15.2,10.762411286));
#234189=CARTESIAN_POINT('Ctrl Pts',(-3.86462998900006,11.6,10.762411286));
#234190=CARTESIAN_POINT('Ctrl Pts',(-3.86727963900006,15.2,10.765052131));
#234191=CARTESIAN_POINT('Ctrl Pts',(-3.86727963900006,11.6,10.765052131));
#234192=CARTESIAN_POINT('Ctrl Pts',(-3.86993447500006,15.2,10.767694103));
#234193=CARTESIAN_POINT('Ctrl Pts',(-3.86993447500006,11.6,10.767694103));
#234194=CARTESIAN_POINT('Ctrl Pts',(-3.87259449700006,15.2,10.770337195));
#234195=CARTESIAN_POINT('Ctrl Pts',(-3.87259449700006,11.6,10.770337195));
#234196=CARTESIAN_POINT('Ctrl Pts',(-3.87525970400006,15.2,10.772981399));
#234197=CARTESIAN_POINT('Ctrl Pts',(-3.87525970400006,11.6,10.772981399));
#234198=CARTESIAN_POINT('Ctrl Pts',(-3.87793009300006,15.2,10.775626704));
#234199=CARTESIAN_POINT('Ctrl Pts',(-3.87793009300006,11.6,10.775626704));
#234200=CARTESIAN_POINT('Ctrl Pts',(-3.88060566700006,15.2,10.778273105));
#234201=CARTESIAN_POINT('Ctrl Pts',(-3.88060566700006,11.6,10.778273105));
#234202=CARTESIAN_POINT('Ctrl Pts',(-3.88328642000006,15.2,10.780920592));
#234203=CARTESIAN_POINT('Ctrl Pts',(-3.88328642000006,11.6,10.780920592));
#234204=CARTESIAN_POINT('Ctrl Pts',(-3.88597235500006,15.2,10.783569156));
#234205=CARTESIAN_POINT('Ctrl Pts',(-3.88597235500006,11.6,10.783569156));
#234206=CARTESIAN_POINT('Ctrl Pts',(-3.88866346800006,15.2,10.786218787));
#234207=CARTESIAN_POINT('Ctrl Pts',(-3.88866346800006,11.6,10.786218787));
#234208=CARTESIAN_POINT('Ctrl Pts',(-3.89135975900006,15.2,10.788869473));
#234209=CARTESIAN_POINT('Ctrl Pts',(-3.89135975900006,11.6,10.788869473));
#234210=CARTESIAN_POINT('Ctrl Pts',(-3.89406122700006,15.2,10.791521203));
#234211=CARTESIAN_POINT('Ctrl Pts',(-3.89406122700006,11.6,10.791521203));
#234212=CARTESIAN_POINT('Ctrl Pts',(-3.89676786900006,15.2,10.794173967));
#234213=CARTESIAN_POINT('Ctrl Pts',(-3.89676786900006,11.6,10.794173967));
#234214=CARTESIAN_POINT('Ctrl Pts',(-3.89947968600006,15.2,10.796827755));
#234215=CARTESIAN_POINT('Ctrl Pts',(-3.89947968600006,11.6,10.796827755));
#234216=CARTESIAN_POINT('Ctrl Pts',(-3.90219667500006,15.2,10.79948256));
#234217=CARTESIAN_POINT('Ctrl Pts',(-3.90219667500006,11.6,10.79948256));
#234218=CARTESIAN_POINT('Ctrl Pts',(-3.90491883500006,15.2,10.802138374));
#234219=CARTESIAN_POINT('Ctrl Pts',(-3.90491883500006,11.6,10.802138374));
#234220=CARTESIAN_POINT('Ctrl Pts',(-3.90764616700006,15.2,10.804795194));
#234221=CARTESIAN_POINT('Ctrl Pts',(-3.90764616700006,11.6,10.804795194));
#234222=CARTESIAN_POINT('Ctrl Pts',(-3.91037867000006,15.2,10.807453019));
#234223=CARTESIAN_POINT('Ctrl Pts',(-3.91037867000006,11.6,10.807453019));
#234224=CARTESIAN_POINT('Ctrl Pts',(-3.91256880800006,15.2,10.80958008));
#234225=CARTESIAN_POINT('Ctrl Pts',(-3.91256880800006,11.6,10.80958008));
#234226=CARTESIAN_POINT('Ctrl Pts',(-3.91421373900006,15.2,10.811175828));
#234227=CARTESIAN_POINT('Ctrl Pts',(-3.91421373900006,11.6,10.811175828));
#234228=CARTESIAN_POINT('Ctrl Pts',(-3.91531139400006,15.2,10.81223986));
#234229=CARTESIAN_POINT('Ctrl Pts',(-3.91531139400006,11.6,10.81223986));
#234230=CARTESIAN_POINT('Ctrl Pts',(-3.91586047900006,15.2,10.812771925));
#234231=CARTESIAN_POINT('Ctrl Pts',(-3.91586047900006,11.6,10.812771925));
#234232=CARTESIAN_POINT('Ctrl Pts',(-3.20199116200006,15.2,9.86852965799999));
#234233=CARTESIAN_POINT('Ctrl Pts',(-3.20268658144428,15.2,9.87017541023993));
#234234=CARTESIAN_POINT('Ctrl Pts',(-3.20340918557853,15.2,9.8718717538802));
#234235=CARTESIAN_POINT('Ctrl Pts',(-3.20415921061787,15.2,9.87361750383371));
#234236=CARTESIAN_POINT('Ctrl Pts',(-3.20491285265707,15.2,9.87537167267594));
#234237=CARTESIAN_POINT('Ctrl Pts',(-3.20569417615054,15.2,9.87717573954122));
#234238=CARTESIAN_POINT('Ctrl Pts',(-3.20650339032002,15.2,9.87902857865426));
#234239=CARTESIAN_POINT('Ctrl Pts',(-3.207312604416,15.2,9.880881417599));
#234240=CARTESIAN_POINT('Ctrl Pts',(-3.20814971002311,15.2,9.88278302787072));
#234241=CARTESIAN_POINT('Ctrl Pts',(-3.20901491174167,15.2,9.88473231696656));
#234242=CARTESIAN_POINT('Ctrl Pts',(-3.20988011346024,15.2,9.88668160606242));
#234243=CARTESIAN_POINT('Ctrl Pts',(-3.21077340886668,15.2,9.88867857418553));
#234244=CARTESIAN_POINT('Ctrl Pts',(-3.21169499187759,15.2,9.89072215729398));
#234245=CARTESIAN_POINT('Ctrl Pts',(-3.2126165749722,15.2,9.89276574058806));
#234246=CARTESIAN_POINT('Ctrl Pts',(-3.21356644777639,15.2,9.89485593812154));
#234247=CARTESIAN_POINT('Ctrl Pts',(-3.21454479458166,15.2,9.89699171649106));
#234248=CARTESIAN_POINT('Ctrl Pts',(-3.21552314129806,15.2,9.89912749466659));
#234249=CARTESIAN_POINT('Ctrl Pts',(-3.21652996004167,15.2,9.9013088547466));
#234250=CARTESIAN_POINT('Ctrl Pts',(-3.21756543175881,15.2,9.90353478725925));
#234251=CARTESIAN_POINT('Ctrl Pts',(-3.21860090347595,15.2,9.9057607197719));
#234252=CARTESIAN_POINT('Ctrl Pts',(-3.21966502620654,15.2,9.90803122612666));
#234253=CARTESIAN_POINT('Ctrl Pts',(-3.22075797091556,15.2,9.91034532737397));
#234254=CARTESIAN_POINT('Ctrl Pts',(-3.22185091572386,15.2,9.91265942883149));
#234255=CARTESIAN_POINT('Ctrl Pts',(-3.22297268097742,15.2,9.91501712290282));
#234256=CARTESIAN_POINT('Ctrl Pts',(-3.22412343087545,15.2,9.91741745478656));
#234257=CARTESIAN_POINT('Ctrl Pts',(-3.22527418066896,15.2,9.91981778645227));
#234258=CARTESIAN_POINT('Ctrl Pts',(-3.22645391675033,15.2,9.92226075792395));
#234259=CARTESIAN_POINT('Ctrl Pts',(-3.22766278962435,15.2,9.92474543566884));
#234260=CARTESIAN_POINT('Ctrl Pts',(-3.22887166249837,15.2,9.92723011341373));
#234261=CARTESIAN_POINT('Ctrl Pts',(-3.23010967588672,15.2,9.9297564981219));
#234262=CARTESIAN_POINT('Ctrl Pts',(-3.23137697842272,15.2,9.93232368186017));
#234263=CARTESIAN_POINT('Ctrl Pts',(-3.23264428095873,15.2,9.93489086559843));
#234264=CARTESIAN_POINT('Ctrl Pts',(-3.23394087148897,15.2,9.93749884804353));
#234265=CARTESIAN_POINT('Ctrl Pts',(-3.23526689310548,15.2,9.94014674294464));
#234266=CARTESIAN_POINT('Ctrl Pts',(-3.23659291484242,15.2,9.94279463808627));
#234267=CARTESIAN_POINT('Ctrl Pts',(-3.23794836809883,15.2,9.94548244670671));
#234268=CARTESIAN_POINT('Ctrl Pts',(-3.23933338784228,15.2,9.94820930194036));
#234269=CARTESIAN_POINT('Ctrl Pts',(-3.24071840745992,15.2,9.95093615692632));
#234270=CARTESIAN_POINT('Ctrl Pts',(-3.24213299364533,15.2,9.95370206081286));
#234271=CARTESIAN_POINT('Ctrl Pts',(-3.24357727726601,15.2,9.95650616497364));
#234272=CARTESIAN_POINT('Ctrl Pts',(-3.2450215608867,15.2,9.95931026913442));
#234273=CARTESIAN_POINT('Ctrl Pts',(-3.24649554203443,15.2,9.96215257803488));
#234274=CARTESIAN_POINT('Ctrl Pts',(-3.2479993435611,15.2,9.96503226217771));
#234275=CARTESIAN_POINT('Ctrl Pts',(-3.24950314522436,15.2,9.96791194658211));
#234276=CARTESIAN_POINT('Ctrl Pts',(-3.25103676978215,15.2,9.97082900819847));
#234277=CARTESIAN_POINT('Ctrl Pts',(-3.25260033336868,15.2,9.97378263869438));
#234278=CARTESIAN_POINT('Ctrl Pts',(-3.25416389681318,15.2,9.97673626892201));
#234279=CARTESIAN_POINT('Ctrl Pts',(-3.25575739994263,15.2,9.97972647059485));
#234280=CARTESIAN_POINT('Ctrl Pts',(-3.25738095647427,15.2,9.98275245099855));
#234281=CARTESIAN_POINT('Ctrl Pts',(-3.2592751058595,15.2,9.98628276165277));
#234282=CARTESIAN_POINT('Ctrl Pts',(-3.26121016215456,15.2,9.98986177345009));
#234283=CARTESIAN_POINT('Ctrl Pts',(-3.26318629436744,15.2,9.99348826166115));
#234284=CARTESIAN_POINT('Ctrl Pts',(-3.26488012189057,15.2,9.99659667996642));
#234285=CARTESIAN_POINT('Ctrl Pts',(-3.26660412830504,15.2,9.99973998038289));
#234286=CARTESIAN_POINT('Ctrl Pts',(-3.26835841574921,15.2,10.0029174077818));
#234287=CARTESIAN_POINT('Ctrl Pts',(-3.27011270319338,15.2,10.0060948351807));
#234288=CARTESIAN_POINT('Ctrl Pts',(-3.27189727326186,15.2,10.0093063905831));
#234289=CARTESIAN_POINT('Ctrl Pts',(-3.27371221977718,15.2,10.0125513371296));
#234290=CARTESIAN_POINT('Ctrl Pts',(-3.27552716645736,15.2,10.0157962839708));
#234291=CARTESIAN_POINT('Ctrl Pts',(-3.27737249207549,15.2,10.0190746216309));
#234292=CARTESIAN_POINT('Ctrl Pts',(-3.27924828868987,15.2,10.022385629562));
#234293=CARTESIAN_POINT('Ctrl Pts',(-3.28112408513387,15.2,10.0256966371923));
#234294=CARTESIAN_POINT('Ctrl Pts',(-3.28303035277037,15.2,10.0290403113476));
#234295=CARTESIAN_POINT('Ctrl Pts',(-3.28496717903333,15.2,10.0324159479749));
#234296=CARTESIAN_POINT('Ctrl Pts',(-3.28690400529629,15.2,10.0357915846023));
#234297=CARTESIAN_POINT('Ctrl Pts',(-3.28887139188969,15.2,10.0391991836307));
#234298=CARTESIAN_POINT('Ctrl Pts',(-3.29086942033179,15.2,10.0426380494257));
#234299=CARTESIAN_POINT('Ctrl Pts',(-3.29253444409405,15.2,10.0455037710257));
#234300=CARTESIAN_POINT('Ctrl Pts',(-3.29422074766736,15.2,10.0483912065221));
#234301=CARTESIAN_POINT('Ctrl Pts',(-3.29592837718012,15.2,10.0512999622848));
#234302=CARTESIAN_POINT('Ctrl Pts',(-3.29763600669288,15.2,10.0542087180476));
#234303=CARTESIAN_POINT('Ctrl Pts',(-3.29936496202567,15.2,10.0571387952304));
#234304=CARTESIAN_POINT('Ctrl Pts',(-3.30111528813566,15.2,10.0600898027987));
#234305=CARTESIAN_POINT('Ctrl Pts',(-3.30286561424566,15.2,10.0630408103671));
#234306=CARTESIAN_POINT('Ctrl Pts',(-3.3046373103465,15.2,10.0660127511514));
#234307=CARTESIAN_POINT('Ctrl Pts',(-3.3064304189657,15.2,10.0690052419983));
#234308=CARTESIAN_POINT('Ctrl Pts',(-3.3082235275849,15.2,10.0719977328452));
#234309=CARTESIAN_POINT('Ctrl Pts',(-3.31003804933333,15.2,10.0750107746777));
#234310=CARTESIAN_POINT('Ctrl Pts',(-3.31187402225,15.2,10.0780439912749));
#234311=CARTESIAN_POINT('Ctrl Pts',(-3.31370999516666,15.2,10.0810772078721));
#234312=CARTESIAN_POINT('Ctrl Pts',(-3.31556742195911,15.2,10.0841305979709));
#234313=CARTESIAN_POINT('Ctrl Pts',(-3.31744634050936,15.2,10.0872037954849));
#234314=CARTESIAN_POINT('Ctrl Pts',(-3.31932525905961,15.2,10.0902769929989));
#234315=CARTESIAN_POINT('Ctrl Pts',(-3.32122566964693,15.2,10.0933699945971));
#234316=CARTESIAN_POINT('Ctrl Pts',(-3.32314760742583,15.2,10.0964824386953));
#234317=CARTESIAN_POINT('Ctrl Pts',(-3.32506954520472,15.2,10.0995948827935));
#234318=CARTESIAN_POINT('Ctrl Pts',(-3.3270130109442,15.2,10.1027267661829));
#234319=CARTESIAN_POINT('Ctrl Pts',(-3.32897804032031,15.2,10.1058777329895));
#234320=CARTESIAN_POINT('Ctrl Pts',(-3.33094306969641,15.2,10.109028699796));
#234321=CARTESIAN_POINT('Ctrl Pts',(-3.33292966250359,15.2,10.1121987499762));
#234322=CARTESIAN_POINT('Ctrl Pts',(-3.33493785121653,15.2,10.1153875286785));
#234323=CARTESIAN_POINT('Ctrl Pts',(-3.33694603992947,15.2,10.1185763073808));
#234324=CARTESIAN_POINT('Ctrl Pts',(-3.33897582562212,15.2,10.1217838150371));
#234325=CARTESIAN_POINT('Ctrl Pts',(-3.341027239235,15.2,10.1250097044136));
#234326=CARTESIAN_POINT('Ctrl Pts',(-3.34307865284788,15.2,10.12823559379));
#234327=CARTESIAN_POINT('Ctrl Pts',(-3.34515169463332,15.2,10.1314798639918));
#234328=CARTESIAN_POINT('Ctrl Pts',(-3.347246394774,15.2,10.13474217191));
#234329=CARTESIAN_POINT('Ctrl Pts',(-3.34934109468635,15.2,10.1380044794726));
#234330=CARTESIAN_POINT('Ctrl Pts',(-3.35145745234407,15.2,10.1412848267573));
#234331=CARTESIAN_POINT('Ctrl Pts',(-3.35359549717868,15.2,10.1445828725769));
#234332=CARTESIAN_POINT('Ctrl Pts',(-3.35573354224635,15.2,10.147880918756));
#234333=CARTESIAN_POINT('Ctrl Pts',(-3.35789327309978,15.2,10.1511966652487));
#234334=CARTESIAN_POINT('Ctrl Pts',(-3.36007471747301,15.2,10.154529778789));
#234335=CARTESIAN_POINT('Ctrl Pts',(-3.36225616184624,15.2,10.1578628923292));
#234336=CARTESIAN_POINT('Ctrl Pts',(-3.36445931938858,15.2,10.1612133721887));
#234337=CARTESIAN_POINT('Ctrl Pts',(-3.36668421619232,15.2,10.1645808900345));
#234338=CARTESIAN_POINT('Ctrl Pts',(-3.36890911299606,15.2,10.1679484078802));
#234339=CARTESIAN_POINT('Ctrl Pts',(-3.37115574774714,15.2,10.1713329633753));
#234340=CARTESIAN_POINT('Ctrl Pts',(-3.37342414626175,15.2,10.1747342338218));
#234341=CARTESIAN_POINT('Ctrl Pts',(-3.37569254477636,15.2,10.1781355042684));
#234342=CARTESIAN_POINT('Ctrl Pts',(-3.37798270410007,15.2,10.1815534888374));
#234343=CARTESIAN_POINT('Ctrl Pts',(-3.38029464930727,15.2,10.1849878675171));
#234344=CARTESIAN_POINT('Ctrl Pts',(-3.38260659451446,15.2,10.1884222461968));
#234345=CARTESIAN_POINT('Ctrl Pts',(-3.38494032557501,15.2,10.1918730190686));
#234346=CARTESIAN_POINT('Ctrl Pts',(-3.38729586154608,15.2,10.1953398710816));
#234347=CARTESIAN_POINT('Ctrl Pts',(-3.38918029042563,15.2,10.1981133528432));
#234348=CARTESIAN_POINT('Ctrl Pts',(-3.39107867605716,15.2,10.2008971257044));
#234349=CARTESIAN_POINT('Ctrl Pts',(-3.39299102653591,15.2,10.2036910291637));
#234350=CARTESIAN_POINT('Ctrl Pts',(-3.39538146450407,15.2,10.2071834082976));
#234351=CARTESIAN_POINT('Ctrl Pts',(-3.39779372467773,15.2,10.2106916181818));
#234352=CARTESIAN_POINT('Ctrl Pts',(-3.40022782481839,15.2,10.2142153495025));
#234353=CARTESIAN_POINT('Ctrl Pts',(-3.40217510477173,15.2,10.2170343343286));
#234354=CARTESIAN_POINT('Ctrl Pts',(-3.40413636253717,15.2,10.219863254359));
#234355=CARTESIAN_POINT('Ctrl Pts',(-3.40611160709699,15.2,10.222701951293));
#234356=CARTESIAN_POINT('Ctrl Pts',(-3.40808685192593,15.2,10.2255406486137));
#234357=CARTESIAN_POINT('Ctrl Pts',(-3.41007608329694,15.2,10.2283891251486));
#234358=CARTESIAN_POINT('Ctrl Pts',(-3.41207930950743,15.2,10.2312472264481));
#234359=CARTESIAN_POINT('Ctrl Pts',(-3.41408253544497,15.2,10.234105327358));
#234360=CARTESIAN_POINT('Ctrl Pts',(-3.41609975603161,15.2,10.2369730519368));
#234361=CARTESIAN_POINT('Ctrl Pts',(-3.41813097880908,15.2,10.2398502487565));
#234362=CARTESIAN_POINT('Ctrl Pts',(-3.42016220186329,15.2,10.2427274459682));
#234363=CARTESIAN_POINT('Ctrl Pts',(-3.42220742876644,15.2,10.2456141148395));
#234364=CARTESIAN_POINT('Ctrl Pts',(-3.42426666543514,15.2,10.2485101042201));
#234365=CARTESIAN_POINT('Ctrl Pts',(-3.42632590182327,15.2,10.2514060932062));
#234366=CARTESIAN_POINT('Ctrl Pts',(-3.42839914693979,15.2,10.2543114037067));
#234367=CARTESIAN_POINT('Ctrl Pts',(-3.43048640970553,15.2,10.2572258860021));
#234368=CARTESIAN_POINT('Ctrl Pts',(-3.43257367275567,15.2,10.2601403686946));
#234369=CARTESIAN_POINT('Ctrl Pts',(-3.43467495285964,15.2,10.2630640229044));
#234370=CARTESIAN_POINT('Ctrl Pts',(-3.43679025569806,15.2,10.2659967002314));
#234371=CARTESIAN_POINT('Ctrl Pts',(-3.43890555824827,15.2,10.268929377159));
#234372=CARTESIAN_POINT('Ctrl Pts',(-3.44103488396512,15.2,10.271871077618));
#234373=CARTESIAN_POINT('Ctrl Pts',(-3.44317823789957,15.2,10.2748216552092));
#234374=CARTESIAN_POINT('Ctrl Pts',(-3.44532159212606,15.2,10.2777722332024));
#234375=CARTESIAN_POINT('Ctrl Pts',(-3.44747897605656,15.2,10.2807316891739));
#234376=CARTESIAN_POINT('Ctrl Pts',(-3.44965039351815,15.2,10.2836998759603));
#234377=CARTESIAN_POINT('Ctrl Pts',(-3.45345037392799,15.2,10.2888942026342));
#234378=CARTESIAN_POINT('Ctrl Pts',(-3.45729333318342,15.2,10.294115273107));
#234379=CARTESIAN_POINT('Ctrl Pts',(-3.46117929807973,15.2,10.2993623177318));
#234380=CARTESIAN_POINT('Ctrl Pts',(-3.46339984923295,15.2,10.3023606286542));
#234381=CARTESIAN_POINT('Ctrl Pts',(-3.4656344423705,15.2,10.3053674211172));
#234382=CARTESIAN_POINT('Ctrl Pts',(-3.46788308157464,15.2,10.3083825535369));
#234383=CARTESIAN_POINT('Ctrl Pts',(-3.47181820056487,15.2,10.3136590357848));
#234384=CARTESIAN_POINT('Ctrl Pts',(-3.47579633560707,15.2,10.3189610629039));
#234385=CARTESIAN_POINT('Ctrl Pts',(-3.47981750667132,15.2,10.3242878852655));
#234386=CARTESIAN_POINT('Ctrl Pts',(-3.4821153184844,15.2,10.3273317834617));
#234387=CARTESIAN_POINT('Ctrl Pts',(-3.4844271811113,15.2,10.3303837782117));
#234388=CARTESIAN_POINT('Ctrl Pts',(-3.48675309958638,15.2,10.3334437325163));
#234389=CARTESIAN_POINT('Ctrl Pts',(-3.48907901837838,15.2,10.3365036872378));
#234390=CARTESIAN_POINT('Ctrl Pts',(-3.49141899295146,15.2,10.3395716010815));
#234391=CARTESIAN_POINT('Ctrl Pts',(-3.49377302320161,15.2,10.3426473384854));
#234392=CARTESIAN_POINT('Ctrl Pts',(-3.49671556085393,15.2,10.3464920100307));
#234393=CARTESIAN_POINT('Ctrl Pts',(-3.49968006414432,15.2,10.3503489047802));
#234394=CARTESIAN_POINT('Ctrl Pts',(-3.50266653497879,15.2,10.3542177605447));
#234395=CARTESIAN_POINT('Ctrl Pts',(-3.50505571145104,15.2,10.3573128449033));
#234396=CARTESIAN_POINT('Ctrl Pts',(-3.50745894693715,15.2,10.3604155837631));
#234397=CARTESIAN_POINT('Ctrl Pts',(-3.50987624340478,15.2,10.3635258435081));
#234398=CARTESIAN_POINT('Ctrl Pts',(-3.51229354020176,15.2,10.3666361036768));
#234399=CARTESIAN_POINT('Ctrl Pts',(-3.51472489772667,15.2,10.3697538860703));
#234400=CARTESIAN_POINT('Ctrl Pts',(-3.51717031726001,15.2,10.3728790569771));
#234401=CARTESIAN_POINT('Ctrl Pts',(-3.51961573646016,15.2,10.3760042274581));
#234402=CARTESIAN_POINT('Ctrl Pts',(-3.52207521794367,15.2,10.3791367884607));
#234403=CARTESIAN_POINT('Ctrl Pts',(-3.52454876162892,15.2,10.3822766062033));
#234404=CARTESIAN_POINT('Ctrl Pts',(-3.52764069148824,15.2,10.3862013787023));
#234405=CARTESIAN_POINT('Ctrl Pts',(-3.5307545921361,15.2,10.3901374933624));
#234406=CARTESIAN_POINT('Ctrl Pts',(-3.53389046706483,15.2,10.3940846949587));
#234407=CARTESIAN_POINT('Ctrl Pts',(-3.53702634199355,15.2,10.3980318965549));
#234408=CARTESIAN_POINT('Ctrl Pts',(-3.54018418873035,15.2,10.4019901867706));
#234409=CARTESIAN_POINT('Ctrl Pts',(-3.54336400782575,15.2,10.4059593135058));
#234410=CARTESIAN_POINT('Ctrl Pts',(-3.54654382692116,15.2,10.409928440241));
#234411=CARTESIAN_POINT('Ctrl Pts',(-3.54974561694407,15.2,10.413908404427));
#234412=CARTESIAN_POINT('Ctrl Pts',(-3.55296937786751,15.2,10.4178989580284));
#234413=CARTESIAN_POINT('Ctrl Pts',(-3.55619313879095,15.2,10.4218895116298));
#234414=CARTESIAN_POINT('Ctrl Pts',(-3.55943887002089,15.2,10.4258906562826));
#234415=CARTESIAN_POINT('Ctrl Pts',(-3.5627065683531,15.2,10.429902143921));
#234416=CARTESIAN_POINT('Ctrl Pts',(-3.56532072716133,15.2,10.4331113342066));
#234417=CARTESIAN_POINT('Ctrl Pts',(-3.56794894534067,15.2,10.4363271470235));
#234418=CARTESIAN_POINT('Ctrl Pts',(-3.5705912202078,15.2,10.4395494552551));
#234419=CARTESIAN_POINT('Ctrl Pts',(-3.57323349471492,15.2,10.4427717630476));
#234420=CARTESIAN_POINT('Ctrl Pts',(-3.57588982754871,15.2,10.4460005664673));
#234421=CARTESIAN_POINT('Ctrl Pts',(-3.57856021479592,15.2,10.4492357450305));
#234422=CARTESIAN_POINT('Ctrl Pts',(-3.58123060240697,15.2,10.4524709240346));
#234423=CARTESIAN_POINT('Ctrl Pts',(-3.58391504561995,15.2,10.4557124753742));
#234424=CARTESIAN_POINT('Ctrl Pts',(-3.58661354171241,15.2,10.4589602782739));
#234425=CARTESIAN_POINT('Ctrl Pts',(-3.58931203743721,15.2,10.462208080731));
#234426=CARTESIAN_POINT('Ctrl Pts',(-3.59202458546188,15.2,10.4654621349174));
#234427=CARTESIAN_POINT('Ctrl Pts',(-3.59475118323754,15.2,10.4687223199836));
#234428=CARTESIAN_POINT('Ctrl Pts',(-3.5974777813847,15.2,10.471982505494));
#234429=CARTESIAN_POINT('Ctrl Pts',(-3.60021842976976,15.2,10.4752488211395));
#234430=CARTESIAN_POINT('Ctrl Pts',(-3.60297312454355,15.2,10.4785211462772));
#234431=CARTESIAN_POINT('Ctrl Pts',(-3.60572781894201,15.2,10.481793470969));
#234432=CARTESIAN_POINT('Ctrl Pts',(-3.6084965606601,15.2,10.4850718073905));
#234433=CARTESIAN_POINT('Ctrl Pts',(-3.61127934448668,15.2,10.4883560339547));
#234434=CARTESIAN_POINT('Ctrl Pts',(-3.61475782455427,15.2,10.4924613174955));
#234435=CARTESIAN_POINT('Ctrl Pts',(-3.61825824732444,15.2,10.4965758083614));
#234436=CARTESIAN_POINT('Ctrl Pts',(-3.62178060398928,15.2,10.5006992727356));
#234437=CARTESIAN_POINT('Ctrl Pts',(-3.62459848947474,15.2,10.5039980444148));
#234438=CARTESIAN_POINT('Ctrl Pts',(-3.62743041346721,15.2,10.5073025604818));
#234439=CARTESIAN_POINT('Ctrl Pts',(-3.63027637096861,15.2,10.5106127035106));
#234440=CARTESIAN_POINT('Ctrl Pts',(-3.63383381765147,15.2,10.514750382071));
#234441=CARTESIAN_POINT('Ctrl Pts',(-3.63741319397896,15.2,10.5188968543991));
#234442=CARTESIAN_POINT('Ctrl Pts',(-3.641014487244,15.2,10.5230518920384));
#234443=CARTESIAN_POINT('Ctrl Pts',(-3.6438955216205,15.2,10.5263759218782));
#234444=CARTESIAN_POINT('Ctrl Pts',(-3.64679058301087,15.2,10.529705434639));
#234445=CARTESIAN_POINT('Ctrl Pts',(-3.64969966804937,15.2,10.5330403152547));
#234446=CARTESIAN_POINT('Ctrl Pts',(-3.65406329620166,15.2,10.5380426368598));
#234447=CARTESIAN_POINT('Ctrl Pts',(-3.65845847497241,15.2,10.5430570368939));
#234448=CARTESIAN_POINT('Ctrl Pts',(-3.66288518818665,15.2,10.5480831307529));
#234449=CARTESIAN_POINT('Ctrl Pts',(-3.66509854459271,15.2,10.5505961774541));
#234450=CARTESIAN_POINT('Ctrl Pts',(-3.66731978342341,15.2,10.5531121483658));
#234451=CARTESIAN_POINT('Ctrl Pts',(-3.66954890330144,15.2,10.5556309949829));
#234452=CARTESIAN_POINT('Ctrl Pts',(-3.67177802317947,15.2,10.5581498416));
#234453=CARTESIAN_POINT('Ctrl Pts',(-3.67401502376491,15.2,10.5606715651084));
#234454=CARTESIAN_POINT('Ctrl Pts',(-3.676259902225,15.2,10.563196116725));
#234455=CARTESIAN_POINT('Ctrl Pts',(-3.6785047806851,15.2,10.5657206683416));
#234456=CARTESIAN_POINT('Ctrl Pts',(-3.6807575386199,15.2,10.5682480502498));
#234457=CARTESIAN_POINT('Ctrl Pts',(-3.68301817103705,15.2,10.5707782142409));
#234458=CARTESIAN_POINT('Ctrl Pts',(-3.6852788034542,15.2,10.573308378232));
#234459=CARTESIAN_POINT('Ctrl Pts',(-3.6875473112629,15.2,10.5758413236252));
#234460=CARTESIAN_POINT('Ctrl Pts',(-3.68982369179299,15.2,10.5783770052844));
#234461=CARTESIAN_POINT('Ctrl Pts',(-3.69210007232306,15.2,10.5809126869436));
#234462=CARTESIAN_POINT('Ctrl Pts',(-3.6943843261847,15.2,10.5834511038387));
#234463=CARTESIAN_POINT('Ctrl Pts',(-3.69667645001699,15.2,10.5859922099127));
#234464=CARTESIAN_POINT('Ctrl Pts',(-3.69896857426568,15.2,10.5885333164482));
#234465=CARTESIAN_POINT('Ctrl Pts',(-3.70126856794999,15.2,10.591077112568));
#234466=CARTESIAN_POINT('Ctrl Pts',(-3.70357642874479,15.2,10.5936235520634));
#234467=CARTESIAN_POINT('Ctrl Pts',(-3.70588428912032,15.2,10.5961699910962));
#234468=CARTESIAN_POINT('Ctrl Pts',(-3.70820001685382,15.2,10.598719073504));
#234469=CARTESIAN_POINT('Ctrl Pts',(-3.71052360777007,15.2,10.6012707530365));
#234470=CARTESIAN_POINT('Ctrl Pts',(-3.71284719868632,15.2,10.603822432569));
#234471=CARTESIAN_POINT('Ctrl Pts',(-3.71517865447647,15.2,10.6063767092336));
#234472=CARTESIAN_POINT('Ctrl Pts',(-3.71751797077713,15.2,10.608933537819));
#234473=CARTESIAN_POINT('Ctrl Pts',(-3.7214168314199,15.2,10.6131949189494));
#234474=CARTESIAN_POINT('Ctrl Pts',(-3.72533752619572,15.2,10.6174633896348));
#234475=CARTESIAN_POINT('Ctrl Pts',(-3.72928004272464,15.2,10.6217387382463));
#234476=CARTESIAN_POINT('Ctrl Pts',(-3.73164555255604,15.2,10.62430394732));
#234477=CARTESIAN_POINT('Ctrl Pts',(-3.73401891745318,15.2,10.6268716324934));
#234478=CARTESIAN_POINT('Ctrl Pts',(-3.73640013474166,15.2,10.6294417504833));
#234479=CARTESIAN_POINT('Ctrl Pts',(-3.73878135203014,15.2,10.6320118684733));
#234480=CARTESIAN_POINT('Ctrl Pts',(-3.74117042115997,15.2,10.6345844179131));
#234481=CARTESIAN_POINT('Ctrl Pts',(-3.74356733853053,15.2,10.637159354486));
#234482=CARTESIAN_POINT('Ctrl Pts',(-3.74596425590109,15.2,10.6397342910589));
#234483=CARTESIAN_POINT('Ctrl Pts',(-3.74836902235136,15.2,10.6423116147494));
#234484=CARTESIAN_POINT('Ctrl Pts',(-3.75078163379996,15.2,10.6448912809926));
#234485=CARTESIAN_POINT('Ctrl Pts',(-3.75319424524857,15.2,10.6474709472357));
#234486=CARTESIAN_POINT('Ctrl Pts',(-3.7556147010266,15.2,10.6500529563808));
#234487=CARTESIAN_POINT('Ctrl Pts',(-3.75804299922897,15.2,10.6526372644532));
#234488=CARTESIAN_POINT('Ctrl Pts',(-3.76128073045955,15.2,10.6560830088629));
#234489=CARTESIAN_POINT('Ctrl Pts',(-3.76453239976366,15.2,10.6595328396923));
#234490=CARTESIAN_POINT('Ctrl Pts',(-3.767798001775,15.2,10.6629866534916));
#234491=CARTESIAN_POINT('Ctrl Pts',(-3.77024720306104,15.2,10.6655770136059));
#234492=CARTESIAN_POINT('Ctrl Pts',(-3.7727042400717,15.2,10.668169614095));
#234493=CARTESIAN_POINT('Ctrl Pts',(-3.77516911077313,15.2,10.6707644111672));
#234494=CARTESIAN_POINT('Ctrl Pts',(-3.77845560534022,15.2,10.674224140911));
#234495=CARTESIAN_POINT('Ctrl Pts',(-3.78175602236732,15.2,10.6776877768637));
#234496=CARTESIAN_POINT('Ctrl Pts',(-3.78507035577107,15.2,10.6811552147751));
#234497=CARTESIAN_POINT('Ctrl Pts',(-3.7875561055981,15.2,10.6837557929725));
#234498=CARTESIAN_POINT('Ctrl Pts',(-3.7900496824651,15.2,10.6863585104018));
#234499=CARTESIAN_POINT('Ctrl Pts',(-3.79255108276061,15.2,10.6889633244857));
#234500=CARTESIAN_POINT('Ctrl Pts',(-3.79672008340459,15.2,10.6933046814498));
#234501=CARTESIAN_POINT('Ctrl Pts',(-3.80091081499673,15.2,10.6976518615066));
#234502=CARTESIAN_POINT('Ctrl Pts',(-3.80512325902562,15.2,10.7020046667847));
#234503=CARTESIAN_POINT('Ctrl Pts',(-3.80765072535113,15.2,10.7046163498566));
#234504=CARTESIAN_POINT('Ctrl Pts',(-3.81018600785905,15.2,10.7072300574283));
#234505=CARTESIAN_POINT('Ctrl Pts',(-3.81272910222501,15.2,10.7098457485));
#234506=CARTESIAN_POINT('Ctrl Pts',(-3.81527219659096,15.2,10.7124614395716));
#234507=CARTESIAN_POINT('Ctrl Pts',(-3.81782310329824,15.2,10.7150791136598));
#234508=CARTESIAN_POINT('Ctrl Pts',(-3.82038181720456,15.2,10.7176987287728));
#234509=CARTESIAN_POINT('Ctrl Pts',(-3.82294053111088,15.2,10.7203183438857));
#234510=CARTESIAN_POINT('Ctrl Pts',(-3.8255070539345,15.2,10.7229398988736));
#234511=CARTESIAN_POINT('Ctrl Pts',(-3.82808137901035,15.2,10.7255633536591));
#234512=CARTESIAN_POINT('Ctrl Pts',(-3.83065570408619,15.2,10.7281868084446));
#234513=CARTESIAN_POINT('Ctrl Pts',(-3.8332378332639,15.2,10.7308121627396));
#234514=CARTESIAN_POINT('Ctrl Pts',(-3.83582776062707,15.2,10.7334393729356));
#234515=CARTESIAN_POINT('Ctrl Pts',(-3.83841768846073,15.2,10.7360665836088));
#234516=CARTESIAN_POINT('Ctrl Pts',(-3.8410154146883,15.2,10.7386956518243));
#234517=CARTESIAN_POINT('Ctrl Pts',(-3.84362093502635,15.2,10.7413265355402));
#234518=CARTESIAN_POINT('Ctrl Pts',(-3.84622645489106,15.2,10.7439574187782));
#234519=CARTESIAN_POINT('Ctrl Pts',(-3.84883976986375,15.2,10.7465901191161));
#234520=CARTESIAN_POINT('Ctrl Pts',(-3.85146087376917,15.2,10.7492245942705));
#234521=CARTESIAN_POINT('Ctrl Pts',(-3.85408197767459,15.2,10.7518590694249));
#234522=CARTESIAN_POINT('Ctrl Pts',(-3.85671087233616,15.2,10.7544953204529));
#234523=CARTESIAN_POINT('Ctrl Pts',(-3.85934755071074,15.2,10.7571333045357));
#234524=CARTESIAN_POINT('Ctrl Pts',(-3.86286312171717,15.2,10.7606506164864));
#234525=CARTESIAN_POINT('Ctrl Pts',(-3.86639253259233,15.2,10.7641710075372));
#234526=CARTESIAN_POINT('Ctrl Pts',(-3.86993577091234,15.2,10.7676943824156));
#234527=CARTESIAN_POINT('Ctrl Pts',(-3.87259320025582,15.2,10.7703369141744));
#234528=CARTESIAN_POINT('Ctrl Pts',(-3.87525840799319,15.2,10.7729811257754));
#234529=CARTESIAN_POINT('Ctrl Pts',(-3.87793138975772,15.2,10.7756269785351));
#234530=CARTESIAN_POINT('Ctrl Pts',(-3.88060437103665,15.2,10.7782728308142));
#234531=CARTESIAN_POINT('Ctrl Pts',(-3.88328512609018,15.2,10.7809203265349));
#234532=CARTESIAN_POINT('Ctrl Pts',(-3.88597364982652,15.2,10.7835694230221));
#234533=CARTESIAN_POINT('Ctrl Pts',(-3.89045452288323,15.2,10.7879845839946));
#234534=CARTESIAN_POINT('Ctrl Pts',(-3.89495697459219,15.2,10.7924041830756));
#234535=CARTESIAN_POINT('Ctrl Pts',(-3.89948097954192,15.2,10.7968280097552));
#234536=CARTESIAN_POINT('Ctrl Pts',(-3.90219538241314,15.2,10.7994823056665));
#234537=CARTESIAN_POINT('Ctrl Pts',(-3.90491754275119,15.2,10.8021381233159));
#234538=CARTESIAN_POINT('Ctrl Pts',(-3.90764746004228,15.2,10.8047954455155));
#234539=CARTESIAN_POINT('Ctrl Pts',(-3.91037737733337,15.2,10.8074527677151));
#234540=CARTESIAN_POINT('Ctrl Pts',(-3.91311505247005,15.2,10.8101115985174));
#234541=CARTESIAN_POINT('Ctrl Pts',(-3.91586047900006,15.2,10.812771925));
#234542=CARTESIAN_POINT('Ctrl Pts',(-3.20199116200006,12.2,9.86852965799999));
#234543=CARTESIAN_POINT('Ctrl Pts',(-3.20268658144428,12.2,9.87017541023993));
#234544=CARTESIAN_POINT('Ctrl Pts',(-3.20340918557853,12.2,9.8718717538802));
#234545=CARTESIAN_POINT('Ctrl Pts',(-3.20415921061787,12.2,9.87361750383371));
#234546=CARTESIAN_POINT('Ctrl Pts',(-3.20491285265707,12.2,9.87537167267594));
#234547=CARTESIAN_POINT('Ctrl Pts',(-3.20569417615054,12.2,9.87717573954122));
#234548=CARTESIAN_POINT('Ctrl Pts',(-3.20650339032002,12.2,9.87902857865426));
#234549=CARTESIAN_POINT('Ctrl Pts',(-3.207312604416,12.2,9.880881417599));
#234550=CARTESIAN_POINT('Ctrl Pts',(-3.20814971002311,12.2,9.88278302787072));
#234551=CARTESIAN_POINT('Ctrl Pts',(-3.20901491174167,12.2,9.88473231696656));
#234552=CARTESIAN_POINT('Ctrl Pts',(-3.20988011346024,12.2,9.88668160606242));
#234553=CARTESIAN_POINT('Ctrl Pts',(-3.21077340886668,12.2,9.88867857418553));
#234554=CARTESIAN_POINT('Ctrl Pts',(-3.21169499187759,12.2,9.89072215729398));
#234555=CARTESIAN_POINT('Ctrl Pts',(-3.2126165749722,12.2,9.89276574058806));
#234556=CARTESIAN_POINT('Ctrl Pts',(-3.21356644777639,12.2,9.89485593812154));
#234557=CARTESIAN_POINT('Ctrl Pts',(-3.21454479458166,12.2,9.89699171649106));
#234558=CARTESIAN_POINT('Ctrl Pts',(-3.21552314129806,12.2,9.89912749466659));
#234559=CARTESIAN_POINT('Ctrl Pts',(-3.21652996004167,12.2,9.9013088547466));
#234560=CARTESIAN_POINT('Ctrl Pts',(-3.21756543175881,12.2,9.90353478725925));
#234561=CARTESIAN_POINT('Ctrl Pts',(-3.21860090347595,12.2,9.9057607197719));
#234562=CARTESIAN_POINT('Ctrl Pts',(-3.21966502620654,12.2,9.90803122612666));
#234563=CARTESIAN_POINT('Ctrl Pts',(-3.22075797091556,12.2,9.91034532737397));
#234564=CARTESIAN_POINT('Ctrl Pts',(-3.22185091572386,12.2,9.91265942883149));
#234565=CARTESIAN_POINT('Ctrl Pts',(-3.22297268097742,12.2,9.91501712290282));
#234566=CARTESIAN_POINT('Ctrl Pts',(-3.22412343087545,12.2,9.91741745478656));
#234567=CARTESIAN_POINT('Ctrl Pts',(-3.22527418066896,12.2,9.91981778645227));
#234568=CARTESIAN_POINT('Ctrl Pts',(-3.22645391675033,12.2,9.92226075792395));
#234569=CARTESIAN_POINT('Ctrl Pts',(-3.22766278962434,12.2,9.92474543566884));
#234570=CARTESIAN_POINT('Ctrl Pts',(-3.22887166249836,12.2,9.92723011341373));
#234571=CARTESIAN_POINT('Ctrl Pts',(-3.23010967588672,12.2,9.9297564981219));
#234572=CARTESIAN_POINT('Ctrl Pts',(-3.23137697842272,12.2,9.93232368186017));
#234573=CARTESIAN_POINT('Ctrl Pts',(-3.23264428095873,12.2,9.93489086559843));
#234574=CARTESIAN_POINT('Ctrl Pts',(-3.23394087148897,12.2,9.93749884804353));
#234575=CARTESIAN_POINT('Ctrl Pts',(-3.23526689310548,12.2,9.94014674294464));
#234576=CARTESIAN_POINT('Ctrl Pts',(-3.23659291484242,12.2,9.94279463808627));
#234577=CARTESIAN_POINT('Ctrl Pts',(-3.23794836809883,12.2,9.94548244670671));
#234578=CARTESIAN_POINT('Ctrl Pts',(-3.23933338784228,12.2,9.94820930194037));
#234579=CARTESIAN_POINT('Ctrl Pts',(-3.24071840745992,12.2,9.95093615692632));
#234580=CARTESIAN_POINT('Ctrl Pts',(-3.24213299364532,12.2,9.95370206081285));
#234581=CARTESIAN_POINT('Ctrl Pts',(-3.243577277266,12.2,9.95650616497363));
#234582=CARTESIAN_POINT('Ctrl Pts',(-3.24502156088669,12.2,9.9593102691344));
#234583=CARTESIAN_POINT('Ctrl Pts',(-3.24649554203443,12.2,9.96215257803488));
#234584=CARTESIAN_POINT('Ctrl Pts',(-3.2479993435611,12.2,9.96503226217771));
#234585=CARTESIAN_POINT('Ctrl Pts',(-3.24950314522436,12.2,9.96791194658211));
#234586=CARTESIAN_POINT('Ctrl Pts',(-3.25103676978215,12.2,9.97082900819847));
#234587=CARTESIAN_POINT('Ctrl Pts',(-3.25260033336868,12.2,9.97378263869438));
#234588=CARTESIAN_POINT('Ctrl Pts',(-3.25416389681318,12.2,9.97673626892201));
#234589=CARTESIAN_POINT('Ctrl Pts',(-3.25575739994263,12.2,9.97972647059485));
#234590=CARTESIAN_POINT('Ctrl Pts',(-3.25738095647427,12.2,9.98275245099855));
#234591=CARTESIAN_POINT('Ctrl Pts',(-3.2592751058595,12.2,9.98628276165277));
#234592=CARTESIAN_POINT('Ctrl Pts',(-3.26121016215456,12.2,9.98986177345009));
#234593=CARTESIAN_POINT('Ctrl Pts',(-3.26318629436744,12.2,9.99348826166115));
#234594=CARTESIAN_POINT('Ctrl Pts',(-3.26488012189057,12.2,9.99659667996642));
#234595=CARTESIAN_POINT('Ctrl Pts',(-3.26660412830504,12.2,9.99973998038289));
#234596=CARTESIAN_POINT('Ctrl Pts',(-3.26835841574921,12.2,10.0029174077818));
#234597=CARTESIAN_POINT('Ctrl Pts',(-3.27011270319338,12.2,10.0060948351807));
#234598=CARTESIAN_POINT('Ctrl Pts',(-3.27189727326186,12.2,10.0093063905831));
#234599=CARTESIAN_POINT('Ctrl Pts',(-3.27371221977718,12.2,10.0125513371296));
#234600=CARTESIAN_POINT('Ctrl Pts',(-3.27552716645736,12.2,10.0157962839708));
#234601=CARTESIAN_POINT('Ctrl Pts',(-3.27737249207549,12.2,10.0190746216309));
#234602=CARTESIAN_POINT('Ctrl Pts',(-3.27924828868987,12.2,10.022385629562));
#234603=CARTESIAN_POINT('Ctrl Pts',(-3.28112408513387,12.2,10.0256966371923));
#234604=CARTESIAN_POINT('Ctrl Pts',(-3.28303035277036,12.2,10.0290403113476));
#234605=CARTESIAN_POINT('Ctrl Pts',(-3.28496717903332,12.2,10.0324159479749));
#234606=CARTESIAN_POINT('Ctrl Pts',(-3.28690400529629,12.2,10.0357915846023));
#234607=CARTESIAN_POINT('Ctrl Pts',(-3.28887139188969,12.2,10.0391991836307));
#234608=CARTESIAN_POINT('Ctrl Pts',(-3.29086942033179,12.2,10.0426380494257));
#234609=CARTESIAN_POINT('Ctrl Pts',(-3.29253444409405,12.2,10.0455037710257));
#234610=CARTESIAN_POINT('Ctrl Pts',(-3.29422074766736,12.2,10.0483912065221));
#234611=CARTESIAN_POINT('Ctrl Pts',(-3.29592837718012,12.2,10.0512999622848));
#234612=CARTESIAN_POINT('Ctrl Pts',(-3.29763600669288,12.2,10.0542087180476));
#234613=CARTESIAN_POINT('Ctrl Pts',(-3.29936496202567,12.2,10.0571387952304));
#234614=CARTESIAN_POINT('Ctrl Pts',(-3.30111528813566,12.2,10.0600898027987));
#234615=CARTESIAN_POINT('Ctrl Pts',(-3.30286561424566,12.2,10.0630408103671));
#234616=CARTESIAN_POINT('Ctrl Pts',(-3.3046373103465,12.2,10.0660127511514));
#234617=CARTESIAN_POINT('Ctrl Pts',(-3.3064304189657,12.2,10.0690052419983));
#234618=CARTESIAN_POINT('Ctrl Pts',(-3.3082235275849,12.2,10.0719977328452));
#234619=CARTESIAN_POINT('Ctrl Pts',(-3.31003804933333,12.2,10.0750107746777));
#234620=CARTESIAN_POINT('Ctrl Pts',(-3.31187402225,12.2,10.0780439912749));
#234621=CARTESIAN_POINT('Ctrl Pts',(-3.31370999516666,12.2,10.0810772078722));
#234622=CARTESIAN_POINT('Ctrl Pts',(-3.31556742195911,12.2,10.0841305979709));
#234623=CARTESIAN_POINT('Ctrl Pts',(-3.31744634050936,12.2,10.0872037954849));
#234624=CARTESIAN_POINT('Ctrl Pts',(-3.31932525905961,12.2,10.0902769929989));
#234625=CARTESIAN_POINT('Ctrl Pts',(-3.32122566964693,12.2,10.0933699945971));
#234626=CARTESIAN_POINT('Ctrl Pts',(-3.32314760742583,12.2,10.0964824386953));
#234627=CARTESIAN_POINT('Ctrl Pts',(-3.32506954520472,12.2,10.0995948827935));
#234628=CARTESIAN_POINT('Ctrl Pts',(-3.3270130109442,12.2,10.1027267661829));
#234629=CARTESIAN_POINT('Ctrl Pts',(-3.32897804032031,12.2,10.1058777329895));
#234630=CARTESIAN_POINT('Ctrl Pts',(-3.33094306969641,12.2,10.109028699796));
#234631=CARTESIAN_POINT('Ctrl Pts',(-3.33292966250359,12.2,10.1121987499762));
#234632=CARTESIAN_POINT('Ctrl Pts',(-3.33493785121653,12.2,10.1153875286785));
#234633=CARTESIAN_POINT('Ctrl Pts',(-3.33694603992947,12.2,10.1185763073808));
#234634=CARTESIAN_POINT('Ctrl Pts',(-3.33897582562212,12.2,10.1217838150371));
#234635=CARTESIAN_POINT('Ctrl Pts',(-3.341027239235,12.2,10.1250097044136));
#234636=CARTESIAN_POINT('Ctrl Pts',(-3.34307865284788,12.2,10.12823559379));
#234637=CARTESIAN_POINT('Ctrl Pts',(-3.34515169463332,12.2,10.1314798639918));
#234638=CARTESIAN_POINT('Ctrl Pts',(-3.347246394774,12.2,10.13474217191));
#234639=CARTESIAN_POINT('Ctrl Pts',(-3.34934109468635,12.2,10.1380044794726));
#234640=CARTESIAN_POINT('Ctrl Pts',(-3.35145745234407,12.2,10.1412848267573));
#234641=CARTESIAN_POINT('Ctrl Pts',(-3.35359549717868,12.2,10.1445828725769));
#234642=CARTESIAN_POINT('Ctrl Pts',(-3.35573354224635,12.2,10.147880918756));
#234643=CARTESIAN_POINT('Ctrl Pts',(-3.35789327309978,12.2,10.1511966652487));
#234644=CARTESIAN_POINT('Ctrl Pts',(-3.36007471747301,12.2,10.154529778789));
#234645=CARTESIAN_POINT('Ctrl Pts',(-3.36225616184624,12.2,10.1578628923292));
#234646=CARTESIAN_POINT('Ctrl Pts',(-3.36445931938858,12.2,10.1612133721887));
#234647=CARTESIAN_POINT('Ctrl Pts',(-3.36668421619232,12.2,10.1645808900345));
#234648=CARTESIAN_POINT('Ctrl Pts',(-3.36890911299606,12.2,10.1679484078802));
#234649=CARTESIAN_POINT('Ctrl Pts',(-3.37115574774714,12.2,10.1713329633753));
#234650=CARTESIAN_POINT('Ctrl Pts',(-3.37342414626175,12.2,10.1747342338218));
#234651=CARTESIAN_POINT('Ctrl Pts',(-3.37569254477636,12.2,10.1781355042684));
#234652=CARTESIAN_POINT('Ctrl Pts',(-3.37798270410007,12.2,10.1815534888374));
#234653=CARTESIAN_POINT('Ctrl Pts',(-3.38029464930727,12.2,10.1849878675171));
#234654=CARTESIAN_POINT('Ctrl Pts',(-3.38260659451446,12.2,10.1884222461968));
#234655=CARTESIAN_POINT('Ctrl Pts',(-3.38494032557501,12.2,10.1918730190686));
#234656=CARTESIAN_POINT('Ctrl Pts',(-3.38729586154608,12.2,10.1953398710816));
#234657=CARTESIAN_POINT('Ctrl Pts',(-3.38918029042563,12.2,10.1981133528432));
#234658=CARTESIAN_POINT('Ctrl Pts',(-3.39107867605716,12.2,10.2008971257044));
#234659=CARTESIAN_POINT('Ctrl Pts',(-3.39299102653591,12.2,10.2036910291637));
#234660=CARTESIAN_POINT('Ctrl Pts',(-3.3949033767541,12.2,10.2064849322425));
#234661=CARTESIAN_POINT('Ctrl Pts',(-3.39682969380659,12.2,10.2092889669479));
#234662=CARTESIAN_POINT('Ctrl Pts',(-3.39876998509151,12.2,10.212102974995));
#234663=CARTESIAN_POINT('Ctrl Pts',(-3.4007102766408,12.2,10.2149169834255));
#234664=CARTESIAN_POINT('Ctrl Pts',(-3.40266454477786,12.2,10.2177409653266));
#234665=CARTESIAN_POINT('Ctrl Pts',(-3.40463279638604,12.2,10.2205747644817));
#234666=CARTESIAN_POINT('Ctrl Pts',(-3.40660104772605,12.2,10.2234085632507));
#234667=CARTESIAN_POINT('Ctrl Pts',(-3.40858328470009,12.2,10.2262521778303));
#234668=CARTESIAN_POINT('Ctrl Pts',(-3.41057951346875,12.2,10.2291054567943));
#234669=CARTESIAN_POINT('Ctrl Pts',(-3.41257574250939,12.2,10.2319587361471));
#234670=CARTESIAN_POINT('Ctrl Pts',(-3.41458596445438,12.2,10.2348216778638));
#234671=CARTESIAN_POINT('Ctrl Pts',(-3.41661018723228,12.2,10.2376941297432));
#234672=CARTESIAN_POINT('Ctrl Pts',(-3.41863440973437,12.2,10.2405665812312));
#234673=CARTESIAN_POINT('Ctrl Pts',(-3.42067263302535,12.2,10.243448542084));
#234674=CARTESIAN_POINT('Ctrl Pts',(-3.42272486435613,12.2,10.2463398615689));
#234675=CARTESIAN_POINT('Ctrl Pts',(-3.42477709596653,12.2,10.2492311814477));
#234676=CARTESIAN_POINT('Ctrl Pts',(-3.42684333537578,12.2,10.2521318602606));
#234677=CARTESIAN_POINT('Ctrl Pts',(-3.42892359077642,12.2,10.2550417470436));
#234678=CARTESIAN_POINT('Ctrl Pts',(-3.43100384589363,12.2,10.2579516334301));
#234679=CARTESIAN_POINT('Ctrl Pts',(-3.43309811610132,12.2,10.2608707296476));
#234680=CARTESIAN_POINT('Ctrl Pts',(-3.43520640737197,12.2,10.2637988857962));
#234681=CARTESIAN_POINT('Ctrl Pts',(-3.43731469892987,12.2,10.2667270423437));
#234682=CARTESIAN_POINT('Ctrl Pts',(-3.43943701277246,12.2,10.2696642592505));
#234683=CARTESIAN_POINT('Ctrl Pts',(-3.441573353,12.2,10.2726103893));
#234684=CARTESIAN_POINT('Ctrl Pts',(-3.44370969322754,12.2,10.2755565193494));
#234685=CARTESIAN_POINT('Ctrl Pts',(-3.44586006123727,12.2,10.2785115640471));
#234686=CARTESIAN_POINT('Ctrl Pts',(-3.44802446207889,12.2,10.2814753760429));
#234687=CARTESIAN_POINT('Ctrl Pts',(-3.45018886262561,12.2,10.2844391876348));
#234688=CARTESIAN_POINT('Ctrl Pts',(-3.45236729561783,12.2,10.2874117685059));
#234689=CARTESIAN_POINT('Ctrl Pts',(-3.45455976678185,12.2,10.2903929728313));
#234690=CARTESIAN_POINT('Ctrl Pts',(-3.45675223824459,12.2,10.2933741775628));
#234691=CARTESIAN_POINT('Ctrl Pts',(-3.45895874662397,12.2,10.2963640064009));
#234692=CARTESIAN_POINT('Ctrl Pts',(-3.46117929807973,12.2,10.2993623177318));
#234693=CARTESIAN_POINT('Ctrl Pts',(-3.46339984923295,12.2,10.3023606286542));
#234694=CARTESIAN_POINT('Ctrl Pts',(-3.4656344423705,12.2,10.3053674211172));
#234695=CARTESIAN_POINT('Ctrl Pts',(-3.46788308157464,12.2,10.3083825535369));
#234696=CARTESIAN_POINT('Ctrl Pts',(-3.47013172108516,12.2,10.3113976863673));
#234697=CARTESIAN_POINT('Ctrl Pts',(-3.47239440733028,12.2,10.3144211612114));
#234698=CARTESIAN_POINT('Ctrl Pts',(-3.47467114234711,12.2,10.3174528366399));
#234699=CARTESIAN_POINT('Ctrl Pts',(-3.47694787705374,12.2,10.3204845116554));
#234700=CARTESIAN_POINT('Ctrl Pts',(-3.47923866226773,12.2,10.3235243868145));
#234701=CARTESIAN_POINT('Ctrl Pts',(-3.48154350007838,12.2,10.3265723245092));
#234702=CARTESIAN_POINT('Ctrl Pts',(-3.48384833820305,12.2,10.3296202626192));
#234703=CARTESIAN_POINT('Ctrl Pts',(-3.48616722792945,12.2,10.3326762637497));
#234704=CARTESIAN_POINT('Ctrl Pts',(-3.48850017472419,12.2,10.3357401892505));
#234705=CARTESIAN_POINT('Ctrl Pts',(-3.49083312120106,12.2,10.3388041143339));
#234706=CARTESIAN_POINT('Ctrl Pts',(-3.49318012223099,12.2,10.3418759657323));
#234707=CARTESIAN_POINT('Ctrl Pts',(-3.49554118143247,12.2,10.3449556055781));
#234708=CARTESIAN_POINT('Ctrl Pts',(-3.49790224095564,12.2,10.3480352458436));
#234709=CARTESIAN_POINT('Ctrl Pts',(-3.500277358181,12.2,10.3511226757644));
#234710=CARTESIAN_POINT('Ctrl Pts',(-3.50266653497879,12.2,10.3542177605447));
#234711=CARTESIAN_POINT('Ctrl Pts',(-3.50505571145104,12.2,10.3573128449033));
#234712=CARTESIAN_POINT('Ctrl Pts',(-3.50745894693715,12.2,10.3604155837631));
#234713=CARTESIAN_POINT('Ctrl Pts',(-3.50987624340478,12.2,10.3635258435081));
#234714=CARTESIAN_POINT('Ctrl Pts',(-3.51229354020175,12.2,10.3666361036768));
#234715=CARTESIAN_POINT('Ctrl Pts',(-3.51472489772667,12.2,10.3697538860703));
#234716=CARTESIAN_POINT('Ctrl Pts',(-3.51717031726001,12.2,10.3728790569771));
#234717=CARTESIAN_POINT('Ctrl Pts',(-3.51961573646016,12.2,10.3760042274581));
#234718=CARTESIAN_POINT('Ctrl Pts',(-3.52207521794367,12.2,10.3791367884607));
#234719=CARTESIAN_POINT('Ctrl Pts',(-3.52454876162892,12.2,10.3822766062033));
#234720=CARTESIAN_POINT('Ctrl Pts',(-3.52702230565118,12.2,10.3854164243736));
#234721=CARTESIAN_POINT('Ctrl Pts',(-3.52950991046368,12.2,10.3885635023003));
#234722=CARTESIAN_POINT('Ctrl Pts',(-3.53201157926666,12.2,10.3917177072499));
#234723=CARTESIAN_POINT('Ctrl Pts',(-3.53451324806963,12.2,10.3948719121996));
#234724=CARTESIAN_POINT('Ctrl Pts',(-3.53702897848819,12.2,10.3980332456585));
#234725=CARTESIAN_POINT('Ctrl Pts',(-3.53955877190529,12.2,10.4012015797763));
#234726=CARTESIAN_POINT('Ctrl Pts',(-3.54208856497771,12.2,10.4043699134625));
#234727=CARTESIAN_POINT('Ctrl Pts',(-3.54463242003439,12.2,10.4075452463144));
#234728=CARTESIAN_POINT('Ctrl Pts',(-3.54719033649102,12.2,10.4107274519982));
#234729=CARTESIAN_POINT('Ctrl Pts',(-3.54974825329616,12.2,10.4139096581156));
#234730=CARTESIAN_POINT('Ctrl Pts',(-3.55232023240676,12.2,10.4170987356293));
#234731=CARTESIAN_POINT('Ctrl Pts',(-3.55490627140033,12.2,10.4202945599637));
#234732=CARTESIAN_POINT('Ctrl Pts',(-3.55749231004154,12.2,10.4234903838627));
#234733=CARTESIAN_POINT('Ctrl Pts',(-3.56009240990104,12.2,10.4266929540727));
#234734=CARTESIAN_POINT('Ctrl Pts',(-3.5627065683531,12.2,10.429902143921));
#234735=CARTESIAN_POINT('Ctrl Pts',(-3.56532072716133,12.2,10.4331113342066));
#234736=CARTESIAN_POINT('Ctrl Pts',(-3.56794894534067,12.2,10.4363271470235));
#234737=CARTESIAN_POINT('Ctrl Pts',(-3.5705912202078,12.2,10.4395494552551));
#234738=CARTESIAN_POINT('Ctrl Pts',(-3.57323349471492,12.2,10.4427717630476));
#234739=CARTESIAN_POINT('Ctrl Pts',(-3.57588982754871,12.2,10.4460005664673));
#234740=CARTESIAN_POINT('Ctrl Pts',(-3.57856021479592,12.2,10.4492357450305));
#234741=CARTESIAN_POINT('Ctrl Pts',(-3.58123060240697,12.2,10.4524709240346));
#234742=CARTESIAN_POINT('Ctrl Pts',(-3.58391504561995,12.2,10.4557124753742));
#234743=CARTESIAN_POINT('Ctrl Pts',(-3.58661354171241,12.2,10.4589602782739));
#234744=CARTESIAN_POINT('Ctrl Pts',(-3.58931203743721,12.2,10.462208080731));
#234745=CARTESIAN_POINT('Ctrl Pts',(-3.59202458546189,12.2,10.4654621349174));
#234746=CARTESIAN_POINT('Ctrl Pts',(-3.59475118323754,12.2,10.4687223199836));
#234747=CARTESIAN_POINT('Ctrl Pts',(-3.5974777813847,12.2,10.471982505494));
#234748=CARTESIAN_POINT('Ctrl Pts',(-3.60021842976976,12.2,10.4752488211395));
#234749=CARTESIAN_POINT('Ctrl Pts',(-3.60297312454354,12.2,10.4785211462772));
#234750=CARTESIAN_POINT('Ctrl Pts',(-3.60572781894201,12.2,10.481793470969));
#234751=CARTESIAN_POINT('Ctrl Pts',(-3.6084965606601,12.2,10.4850718073905));
#234752=CARTESIAN_POINT('Ctrl Pts',(-3.61127934448668,12.2,10.4883560339547));
#234753=CARTESIAN_POINT('Ctrl Pts',(-3.61406212869242,12.2,10.4916402609663));
#234754=CARTESIAN_POINT('Ctrl Pts',(-3.61685895664683,12.2,10.4949303804037));
#234755=CARTESIAN_POINT('Ctrl Pts',(-3.61966982279999,12.2,10.49822627325));
#234756=CARTESIAN_POINT('Ctrl Pts',(-3.62318340529995,12.2,10.5023461390832));
#234757=CARTESIAN_POINT('Ctrl Pts',(-3.62671892428574,12.2,10.5064750249501));
#234758=CARTESIAN_POINT('Ctrl Pts',(-3.63027637096861,12.2,10.5106127035106));
#234759=CARTESIAN_POINT('Ctrl Pts',(-3.63312232808224,12.2,10.5139228460883));
#234760=CARTESIAN_POINT('Ctrl Pts',(-3.63598232039704,12.2,10.5172386164151));
#234761=CARTESIAN_POINT('Ctrl Pts',(-3.63885634077177,12.2,10.5205598981986));
#234762=CARTESIAN_POINT('Ctrl Pts',(-3.64173036153809,12.2,10.5238811804346));
#234763=CARTESIAN_POINT('Ctrl Pts',(-3.64461841053906,12.2,10.5272079721989));
#234764=CARTESIAN_POINT('Ctrl Pts',(-3.647520483975,12.2,10.5305401629916));
#234765=CARTESIAN_POINT('Ctrl Pts',(-3.65042255741093,12.2,10.5338723537843));
#234766=CARTESIAN_POINT('Ctrl Pts',(-3.65333865578462,12.2,10.537209939386));
#234767=CARTESIAN_POINT('Ctrl Pts',(-3.65626877194575,12.2,10.5405528090132));
#234768=CARTESIAN_POINT('Ctrl Pts',(-3.65846635886699,12.2,10.5430599610058));
#234769=CARTESIAN_POINT('Ctrl Pts',(-3.66067183178057,12.2,10.5455700840516));
#234770=CARTESIAN_POINT('Ctrl Pts',(-3.66288518818664,12.2,10.5480831307529));
#234771=CARTESIAN_POINT('Ctrl Pts',(-3.66509854459271,12.2,10.5505961774541));
#234772=CARTESIAN_POINT('Ctrl Pts',(-3.66731978342341,12.2,10.5531121483658));
#234773=CARTESIAN_POINT('Ctrl Pts',(-3.66954890330144,12.2,10.5556309949829));
#234774=CARTESIAN_POINT('Ctrl Pts',(-3.67177802317947,12.2,10.5581498416));
#234775=CARTESIAN_POINT('Ctrl Pts',(-3.67401502376491,12.2,10.5606715651084));
#234776=CARTESIAN_POINT('Ctrl Pts',(-3.676259902225,12.2,10.563196116725));
#234777=CARTESIAN_POINT('Ctrl Pts',(-3.67850478068509,12.2,10.5657206683416));
#234778=CARTESIAN_POINT('Ctrl Pts',(-3.6807575386199,12.2,10.5682480502498));
#234779=CARTESIAN_POINT('Ctrl Pts',(-3.68301817103705,12.2,10.5707782142409));
#234780=CARTESIAN_POINT('Ctrl Pts',(-3.6852788034542,12.2,10.573308378232));
#234781=CARTESIAN_POINT('Ctrl Pts',(-3.6875473112629,12.2,10.5758413236252));
#234782=CARTESIAN_POINT('Ctrl Pts',(-3.68982369179298,12.2,10.5783770052844));
#234783=CARTESIAN_POINT('Ctrl Pts',(-3.69210007232306,12.2,10.5809126869436));
#234784=CARTESIAN_POINT('Ctrl Pts',(-3.6943843261847,12.2,10.5834511038387));
#234785=CARTESIAN_POINT('Ctrl Pts',(-3.69667645001699,12.2,10.5859922099127));
#234786=CARTESIAN_POINT('Ctrl Pts',(-3.69896857426568,12.2,10.5885333164482));
#234787=CARTESIAN_POINT('Ctrl Pts',(-3.70126856795,12.2,10.591077112568));
#234788=CARTESIAN_POINT('Ctrl Pts',(-3.70357642874479,12.2,10.5936235520634));
#234789=CARTESIAN_POINT('Ctrl Pts',(-3.70588428912032,12.2,10.5961699910962));
#234790=CARTESIAN_POINT('Ctrl Pts',(-3.70820001685383,12.2,10.598719073504));
#234791=CARTESIAN_POINT('Ctrl Pts',(-3.71052360777008,12.2,10.6012707530365));
#234792=CARTESIAN_POINT('Ctrl Pts',(-3.71284719868633,12.2,10.603822432569));
#234793=CARTESIAN_POINT('Ctrl Pts',(-3.71517865447647,12.2,10.6063767092336));
#234794=CARTESIAN_POINT('Ctrl Pts',(-3.71751797077713,12.2,10.608933537819));
#234795=CARTESIAN_POINT('Ctrl Pts',(-3.7198572870778,12.2,10.6114903664044));
#234796=CARTESIAN_POINT('Ctrl Pts',(-3.72220446275609,12.2,10.6140497471957));
#234797=CARTESIAN_POINT('Ctrl Pts',(-3.72455949751453,12.2,10.6166116347393));
#234798=CARTESIAN_POINT('Ctrl Pts',(-3.72691453227296,12.2,10.6191735222829));
#234799=CARTESIAN_POINT('Ctrl Pts',(-3.72927742419522,12.2,10.6217379156804));
#234800=CARTESIAN_POINT('Ctrl Pts',(-3.73164817052505,12.2,10.6243047707536));
#234801=CARTESIAN_POINT('Ctrl Pts',(-3.73401891685488,12.2,10.6268716258267));
#234802=CARTESIAN_POINT('Ctrl Pts',(-3.73639751738422,12.2,10.6294409428998));
#234803=CARTESIAN_POINT('Ctrl Pts',(-3.73878396875475,12.2,10.6320126769727));
#234804=CARTESIAN_POINT('Ctrl Pts',(-3.74117042055882,12.2,10.6345844115127));
#234805=CARTESIAN_POINT('Ctrl Pts',(-3.74356472289017,12.2,10.6371585625036));
#234806=CARTESIAN_POINT('Ctrl Pts',(-3.74596687274035,12.2,10.639735086045));
#234807=CARTESIAN_POINT('Ctrl Pts',(-3.74836902215414,12.2,10.6423116091184));
#234808=CARTESIAN_POINT('Ctrl Pts',(-3.75077902015069,12.2,10.644890504264));
#234809=CARTESIAN_POINT('Ctrl Pts',(-3.75319686072621,12.2,10.6474717275077));
#234810=CARTESIAN_POINT('Ctrl Pts',(-3.75561470130172,12.2,10.6500529507515));
#234811=CARTESIAN_POINT('Ctrl Pts',(-3.75804038713647,12.2,10.652636502409));
#234812=CARTESIAN_POINT('Ctrl Pts',(-3.76047391154872,12.2,10.6552223380235));
#234813=CARTESIAN_POINT('Ctrl Pts',(-3.76290743596097,12.2,10.6578081736381));
#234814=CARTESIAN_POINT('Ctrl Pts',(-3.76534880048897,12.2,10.6603962933774));
#234815=CARTESIAN_POINT('Ctrl Pts',(-3.767798001775,12.2,10.6629866534916));
#234816=CARTESIAN_POINT('Ctrl Pts',(-3.77024720306104,12.2,10.6655770136059));
#234817=CARTESIAN_POINT('Ctrl Pts',(-3.7727042400717,12.2,10.668169614095));
#234818=CARTESIAN_POINT('Ctrl Pts',(-3.77516911077313,12.2,10.6707644111672));
#234819=CARTESIAN_POINT('Ctrl Pts',(-3.77763398147455,12.2,10.6733592082394));
#234820=CARTESIAN_POINT('Ctrl Pts',(-3.78010668293379,12.2,10.6759562019948));
#234821=CARTESIAN_POINT('Ctrl Pts',(-3.78258721421758,12.2,10.6785553499834));
#234822=CARTESIAN_POINT('Ctrl Pts',(-3.78506774595201,12.2,10.6811544984441));
#234823=CARTESIAN_POINT('Ctrl Pts',(-3.787556105997,12.2,10.6837557992389));
#234824=CARTESIAN_POINT('Ctrl Pts',(-3.79005229077751,12.2,10.6863592113258));
#234825=CARTESIAN_POINT('Ctrl Pts',(-3.79254847510455,12.2,10.6889626229399));
#234826=CARTESIAN_POINT('Ctrl Pts',(-3.79505248375092,12.2,10.6915681452187));
#234827=CARTESIAN_POINT('Ctrl Pts',(-3.79756431320273,12.2,10.6941757354628));
#234828=CARTESIAN_POINT('Ctrl Pts',(-3.80007614265454,12.2,10.696783325707));
#234829=CARTESIAN_POINT('Ctrl Pts',(-3.80259579270012,12.2,10.6993929837127));
#234830=CARTESIAN_POINT('Ctrl Pts',(-3.80512325902562,12.2,10.7020046667847));
#234831=CARTESIAN_POINT('Ctrl Pts',(-3.80765072535113,12.2,10.7046163498566));
#234832=CARTESIAN_POINT('Ctrl Pts',(-3.81018600785905,12.2,10.7072300574283));
#234833=CARTESIAN_POINT('Ctrl Pts',(-3.81272910222501,12.2,10.7098457485));
#234834=CARTESIAN_POINT('Ctrl Pts',(-3.81527219659096,12.2,10.7124614395716));
#234835=CARTESIAN_POINT('Ctrl Pts',(-3.81782310329824,12.2,10.7150791136598));
#234836=CARTESIAN_POINT('Ctrl Pts',(-3.82038181720456,12.2,10.7176987287728));
#234837=CARTESIAN_POINT('Ctrl Pts',(-3.82294053111088,12.2,10.7203183438857));
#234838=CARTESIAN_POINT('Ctrl Pts',(-3.8255070539345,12.2,10.7229398988736));
#234839=CARTESIAN_POINT('Ctrl Pts',(-3.82808137901035,12.2,10.7255633536591));
#234840=CARTESIAN_POINT('Ctrl Pts',(-3.83065570408619,12.2,10.7281868084446));
#234841=CARTESIAN_POINT('Ctrl Pts',(-3.8332378332639,12.2,10.7308121627396));
#234842=CARTESIAN_POINT('Ctrl Pts',(-3.83582776062707,12.2,10.7334393729356));
#234843=CARTESIAN_POINT('Ctrl Pts',(-3.83841768846073,12.2,10.7360665836088));
#234844=CARTESIAN_POINT('Ctrl Pts',(-3.8410154146883,12.2,10.7386956518243));
#234845=CARTESIAN_POINT('Ctrl Pts',(-3.84362093502635,12.2,10.7413265355402));
#234846=CARTESIAN_POINT('Ctrl Pts',(-3.84622645489106,12.2,10.7439574187782));
#234847=CARTESIAN_POINT('Ctrl Pts',(-3.84883976986375,12.2,10.7465901191161));
#234848=CARTESIAN_POINT('Ctrl Pts',(-3.85146087376917,12.2,10.7492245942705));
#234849=CARTESIAN_POINT('Ctrl Pts',(-3.85408197767459,12.2,10.7518590694249));
#234850=CARTESIAN_POINT('Ctrl Pts',(-3.85671087233616,12.2,10.7544953204529));
#234851=CARTESIAN_POINT('Ctrl Pts',(-3.85934755071074,12.2,10.7571333045357));
#234852=CARTESIAN_POINT('Ctrl Pts',(-3.86286312171717,12.2,10.7606506164864));
#234853=CARTESIAN_POINT('Ctrl Pts',(-3.86639253259233,12.2,10.7641710075372));
#234854=CARTESIAN_POINT('Ctrl Pts',(-3.86993577091234,12.2,10.7676943824156));
#234855=CARTESIAN_POINT('Ctrl Pts',(-3.87259320025582,12.2,10.7703369141744));
#234856=CARTESIAN_POINT('Ctrl Pts',(-3.87525840799319,12.2,10.7729811257754));
#234857=CARTESIAN_POINT('Ctrl Pts',(-3.87793138975772,12.2,10.7756269785351));
#234858=CARTESIAN_POINT('Ctrl Pts',(-3.88060437103665,12.2,10.7782728308142));
#234859=CARTESIAN_POINT('Ctrl Pts',(-3.88328512609018,12.2,10.7809203265349));
#234860=CARTESIAN_POINT('Ctrl Pts',(-3.88597364982652,12.2,10.7835694230221));
#234861=CARTESIAN_POINT('Ctrl Pts',(-3.88955834797884,12.2,10.7871015515113));
#234862=CARTESIAN_POINT('Ctrl Pts',(-3.89315685641974,12.2,10.7906365222355));
#234863=CARTESIAN_POINT('Ctrl Pts',(-3.89676916219258,12.2,10.7941742225116));
#234864=CARTESIAN_POINT('Ctrl Pts',(-3.90038146845759,12.2,10.7977119232698));
#234865=CARTESIAN_POINT('Ctrl Pts',(-3.90400756999021,12.2,10.8012523489275));
#234866=CARTESIAN_POINT('Ctrl Pts',(-3.90764746004228,12.2,10.8047954455155));
#234867=CARTESIAN_POINT('Ctrl Pts',(-3.91037737733337,12.2,10.8074527677151));
#234868=CARTESIAN_POINT('Ctrl Pts',(-3.91311505247005,12.2,10.8101115985174));
#234869=CARTESIAN_POINT('Ctrl Pts',(-3.91586047900006,12.2,10.812771925));
#234870=CARTESIAN_POINT('Ctrl Pts',(-4.27433547000006,15.2,10.676144262));
#234871=CARTESIAN_POINT('Ctrl Pts',(-4.27433547000006,11.6,10.676144262));
#234872=CARTESIAN_POINT('Ctrl Pts',(-4.27439112800006,15.2,10.675381706));
#234873=CARTESIAN_POINT('Ctrl Pts',(-4.27439112800006,11.6,10.675381706));
#234874=CARTESIAN_POINT('Ctrl Pts',(-4.27450212700006,15.2,10.673857013));
#234875=CARTESIAN_POINT('Ctrl Pts',(-4.27450212700006,11.6,10.673857013));
#234876=CARTESIAN_POINT('Ctrl Pts',(-4.27466766800006,15.2,10.67157123));
#234877=CARTESIAN_POINT('Ctrl Pts',(-4.27466766800006,11.6,10.67157123));
#234878=CARTESIAN_POINT('Ctrl Pts',(-4.27488647400006,15.2,10.668526034));
#234879=CARTESIAN_POINT('Ctrl Pts',(-4.27488647400006,11.6,10.668526034));
#234880=CARTESIAN_POINT('Ctrl Pts',(-4.27515679000006,15.2,10.664723728));
#234881=CARTESIAN_POINT('Ctrl Pts',(-4.27515679000006,11.6,10.664723728));
#234882=CARTESIAN_POINT('Ctrl Pts',(-4.27542391400006,15.2,10.660925612));
#234883=CARTESIAN_POINT('Ctrl Pts',(-4.27542391400006,11.6,10.660925612));
#234884=CARTESIAN_POINT('Ctrl Pts',(-4.27568784900005,15.2,10.65713169));
#234885=CARTESIAN_POINT('Ctrl Pts',(-4.27568784900005,11.6,10.65713169));
#234886=CARTESIAN_POINT('Ctrl Pts',(-4.27594859700006,15.2,10.653341964));
#234887=CARTESIAN_POINT('Ctrl Pts',(-4.27594859700006,11.6,10.653341964));
#234888=CARTESIAN_POINT('Ctrl Pts',(-4.27620616000006,15.2,10.649556438));
#234889=CARTESIAN_POINT('Ctrl Pts',(-4.27620616000006,11.6,10.649556438));
#234890=CARTESIAN_POINT('Ctrl Pts',(-4.27646054400006,15.2,10.645775122));
#234891=CARTESIAN_POINT('Ctrl Pts',(-4.27646054400006,11.6,10.645775122));
#234892=CARTESIAN_POINT('Ctrl Pts',(-4.27671175300006,15.2,10.64199802));
#234893=CARTESIAN_POINT('Ctrl Pts',(-4.27671175300006,11.6,10.64199802));
#234894=CARTESIAN_POINT('Ctrl Pts',(-4.27695979400006,15.2,10.638225144));
#234895=CARTESIAN_POINT('Ctrl Pts',(-4.27695979400006,11.6,10.638225144));
#234896=CARTESIAN_POINT('Ctrl Pts',(-4.27720467300006,15.2,10.634456501));
#234897=CARTESIAN_POINT('Ctrl Pts',(-4.27720467300006,11.6,10.634456501));
#234898=CARTESIAN_POINT('Ctrl Pts',(-4.27744639700006,15.2,10.630692101));
#234899=CARTESIAN_POINT('Ctrl Pts',(-4.27744639700006,11.6,10.630692101));
#234900=CARTESIAN_POINT('Ctrl Pts',(-4.27768497200006,15.2,10.626931954));
#234901=CARTESIAN_POINT('Ctrl Pts',(-4.27768497200006,11.6,10.626931954));
#234902=CARTESIAN_POINT('Ctrl Pts',(-4.27792040200006,15.2,10.623176065));
#234903=CARTESIAN_POINT('Ctrl Pts',(-4.27792040200006,11.6,10.623176065));
#234904=CARTESIAN_POINT('Ctrl Pts',(-4.27815269400006,15.2,10.619424443));
#234905=CARTESIAN_POINT('Ctrl Pts',(-4.27815269400006,11.6,10.619424443));
#234906=CARTESIAN_POINT('Ctrl Pts',(-4.27838185100006,15.2,10.615677095));
#234907=CARTESIAN_POINT('Ctrl Pts',(-4.27838185100006,11.6,10.615677095));
#234908=CARTESIAN_POINT('Ctrl Pts',(-4.27860787900006,15.2,10.611934026));
#234909=CARTESIAN_POINT('Ctrl Pts',(-4.27860787900006,11.6,10.611934026));
#234910=CARTESIAN_POINT('Ctrl Pts',(-4.27883078100006,15.2,10.608195244));
#234911=CARTESIAN_POINT('Ctrl Pts',(-4.27883078100006,11.6,10.608195244));
#234912=CARTESIAN_POINT('Ctrl Pts',(-4.27905056400006,15.2,10.604460756));
#234913=CARTESIAN_POINT('Ctrl Pts',(-4.27905056400006,11.6,10.604460756));
#234914=CARTESIAN_POINT('Ctrl Pts',(-4.27926723000006,15.2,10.600730568));
#234915=CARTESIAN_POINT('Ctrl Pts',(-4.27926723000006,11.6,10.600730568));
#234916=CARTESIAN_POINT('Ctrl Pts',(-4.27948078700005,15.2,10.597004691));
#234917=CARTESIAN_POINT('Ctrl Pts',(-4.27948078700005,11.6,10.597004691));
#234918=CARTESIAN_POINT('Ctrl Pts',(-4.27969124100006,15.2,10.593283129));
#234919=CARTESIAN_POINT('Ctrl Pts',(-4.27969124100006,11.6,10.593283129));
#234920=CARTESIAN_POINT('Ctrl Pts',(-4.27989859400006,15.2,10.589565891));
#234921=CARTESIAN_POINT('Ctrl Pts',(-4.27989859400006,11.6,10.589565891));
#234922=CARTESIAN_POINT('Ctrl Pts',(-4.28010285400005,15.2,10.585852986));
#234923=CARTESIAN_POINT('Ctrl Pts',(-4.28010285400005,11.6,10.585852986));
#234924=CARTESIAN_POINT('Ctrl Pts',(-4.28030402700006,15.2,10.58214442));
#234925=CARTESIAN_POINT('Ctrl Pts',(-4.28030402700006,11.6,10.58214442));
#234926=CARTESIAN_POINT('Ctrl Pts',(-4.28050211700006,15.2,10.578440201));
#234927=CARTESIAN_POINT('Ctrl Pts',(-4.28050211700006,11.6,10.578440201));
#234928=CARTESIAN_POINT('Ctrl Pts',(-4.28069713000006,15.2,10.574740338));
#234929=CARTESIAN_POINT('Ctrl Pts',(-4.28069713000006,11.6,10.574740338));
#234930=CARTESIAN_POINT('Ctrl Pts',(-4.28088907200006,15.2,10.571044836));
#234931=CARTESIAN_POINT('Ctrl Pts',(-4.28088907200006,11.6,10.571044836));
#234932=CARTESIAN_POINT('Ctrl Pts',(-4.28107794500006,15.2,10.567353704));
#234933=CARTESIAN_POINT('Ctrl Pts',(-4.28107794500006,11.6,10.567353704));
#234934=CARTESIAN_POINT('Ctrl Pts',(-4.28126375700006,15.2,10.563666949));
#234935=CARTESIAN_POINT('Ctrl Pts',(-4.28126375700006,11.6,10.563666949));
#234936=CARTESIAN_POINT('Ctrl Pts',(-4.28144651400006,15.2,10.559984579));
#234937=CARTESIAN_POINT('Ctrl Pts',(-4.28144651400006,11.6,10.559984579));
#234938=CARTESIAN_POINT('Ctrl Pts',(-4.28162621900006,15.2,10.556306601));
#234939=CARTESIAN_POINT('Ctrl Pts',(-4.28162621900006,11.6,10.556306601));
#234940=CARTESIAN_POINT('Ctrl Pts',(-4.28180287800005,15.2,10.552633022));
#234941=CARTESIAN_POINT('Ctrl Pts',(-4.28180287800005,11.6,10.552633022));
#234942=CARTESIAN_POINT('Ctrl Pts',(-4.28197649800006,15.2,10.54896385));
#234943=CARTESIAN_POINT('Ctrl Pts',(-4.28197649800006,11.6,10.54896385));
#234944=CARTESIAN_POINT('Ctrl Pts',(-4.28214708400006,15.2,10.545299092));
#234945=CARTESIAN_POINT('Ctrl Pts',(-4.28214708400006,11.6,10.545299092));
#234946=CARTESIAN_POINT('Ctrl Pts',(-4.28231464000006,15.2,10.541638759));
#234947=CARTESIAN_POINT('Ctrl Pts',(-4.28231464000006,11.6,10.541638759));
#234948=CARTESIAN_POINT('Ctrl Pts',(-4.28247917400006,15.2,10.537982855));
#234949=CARTESIAN_POINT('Ctrl Pts',(-4.28247917400006,11.6,10.537982855));
#234950=CARTESIAN_POINT('Ctrl Pts',(-4.28264068800006,15.2,10.534331388));
#234951=CARTESIAN_POINT('Ctrl Pts',(-4.28264068800006,11.6,10.534331388));
#234952=CARTESIAN_POINT('Ctrl Pts',(-4.28279919100006,15.2,10.530684368));
#234953=CARTESIAN_POINT('Ctrl Pts',(-4.28279919100006,11.6,10.530684368));
#234954=CARTESIAN_POINT('Ctrl Pts',(-4.28295468700005,15.2,10.5270418));
#234955=CARTESIAN_POINT('Ctrl Pts',(-4.28295468700005,11.6,10.5270418));
#234956=CARTESIAN_POINT('Ctrl Pts',(-4.28310718100006,15.2,10.523403693));
#234957=CARTESIAN_POINT('Ctrl Pts',(-4.28310718100006,11.6,10.523403693));
#234958=CARTESIAN_POINT('Ctrl Pts',(-4.28325667900006,15.2,10.519770053));
#234959=CARTESIAN_POINT('Ctrl Pts',(-4.28325667900006,11.6,10.519770053));
#234960=CARTESIAN_POINT('Ctrl Pts',(-4.28340318700006,15.2,10.51614089));
#234961=CARTESIAN_POINT('Ctrl Pts',(-4.28340318700006,11.6,10.51614089));
#234962=CARTESIAN_POINT('Ctrl Pts',(-4.28354671000006,15.2,10.51251621));
#234963=CARTESIAN_POINT('Ctrl Pts',(-4.28354671000006,11.6,10.51251621));
#234964=CARTESIAN_POINT('Ctrl Pts',(-4.28368725400006,15.2,10.508896023));
#234965=CARTESIAN_POINT('Ctrl Pts',(-4.28368725400006,11.6,10.508896023));
#234966=CARTESIAN_POINT('Ctrl Pts',(-4.28382482400006,15.2,10.505280333));
#234967=CARTESIAN_POINT('Ctrl Pts',(-4.28382482400006,11.6,10.505280333));
#234968=CARTESIAN_POINT('Ctrl Pts',(-4.28395942700006,15.2,10.50166915));
#234969=CARTESIAN_POINT('Ctrl Pts',(-4.28395942700006,11.6,10.50166915));
#234970=CARTESIAN_POINT('Ctrl Pts',(-4.28409106600006,15.2,10.498062482));
#234971=CARTESIAN_POINT('Ctrl Pts',(-4.28409106600006,11.6,10.498062482));
#234972=CARTESIAN_POINT('Ctrl Pts',(-4.28421975000005,15.2,10.494460336));
#234973=CARTESIAN_POINT('Ctrl Pts',(-4.28421975000005,11.6,10.494460336));
#234974=CARTESIAN_POINT('Ctrl Pts',(-4.28434548300006,15.2,10.49086272));
#234975=CARTESIAN_POINT('Ctrl Pts',(-4.28434548300006,11.6,10.49086272));
#234976=CARTESIAN_POINT('Ctrl Pts',(-4.28446827000006,15.2,10.487269641));
#234977=CARTESIAN_POINT('Ctrl Pts',(-4.28446827000006,11.6,10.487269641));
#234978=CARTESIAN_POINT('Ctrl Pts',(-4.28458811800006,15.2,10.483681106));
#234979=CARTESIAN_POINT('Ctrl Pts',(-4.28458811800006,11.6,10.483681106));
#234980=CARTESIAN_POINT('Ctrl Pts',(-4.28470503200006,15.2,10.480097126));
#234981=CARTESIAN_POINT('Ctrl Pts',(-4.28470503200006,11.6,10.480097126));
#234982=CARTESIAN_POINT('Ctrl Pts',(-4.28481901900006,15.2,10.476517706));
#234983=CARTESIAN_POINT('Ctrl Pts',(-4.28481901900006,11.6,10.476517706));
#234984=CARTESIAN_POINT('Ctrl Pts',(-4.28493008300006,15.2,10.472942855));
#234985=CARTESIAN_POINT('Ctrl Pts',(-4.28493008300006,11.6,10.472942855));
#234986=CARTESIAN_POINT('Ctrl Pts',(-4.28503823100006,15.2,10.469372579));
#234987=CARTESIAN_POINT('Ctrl Pts',(-4.28503823100006,11.6,10.469372579));
#234988=CARTESIAN_POINT('Ctrl Pts',(-4.28514346700006,15.2,10.465806888));
#234989=CARTESIAN_POINT('Ctrl Pts',(-4.28514346700006,11.6,10.465806888));
#234990=CARTESIAN_POINT('Ctrl Pts',(-4.28524579900006,15.2,10.462245788));
#234991=CARTESIAN_POINT('Ctrl Pts',(-4.28524579900006,11.6,10.462245788));
#234992=CARTESIAN_POINT('Ctrl Pts',(-4.28534523200006,15.2,10.458689289));
#234993=CARTESIAN_POINT('Ctrl Pts',(-4.28534523200006,11.6,10.458689289));
#234994=CARTESIAN_POINT('Ctrl Pts',(-4.28544177100005,15.2,10.455137396));
#234995=CARTESIAN_POINT('Ctrl Pts',(-4.28544177100005,11.6,10.455137396));
#234996=CARTESIAN_POINT('Ctrl Pts',(-4.28553542400006,15.2,10.45159012));
#234997=CARTESIAN_POINT('Ctrl Pts',(-4.28553542400006,11.6,10.45159012));
#234998=CARTESIAN_POINT('Ctrl Pts',(-4.28562619500005,15.2,10.448047467));
#234999=CARTESIAN_POINT('Ctrl Pts',(-4.28562619500005,11.6,10.448047467));
#235000=CARTESIAN_POINT('Ctrl Pts',(-4.28571409100006,15.2,10.444509444));
#235001=CARTESIAN_POINT('Ctrl Pts',(-4.28571409100006,11.6,10.444509444));
#235002=CARTESIAN_POINT('Ctrl Pts',(-4.28579911600006,15.2,10.440976059));
#235003=CARTESIAN_POINT('Ctrl Pts',(-4.28579911600006,11.6,10.440976059));
#235004=CARTESIAN_POINT('Ctrl Pts',(-4.28588127900006,15.2,10.437447322));
#235005=CARTESIAN_POINT('Ctrl Pts',(-4.28588127900006,11.6,10.437447322));
#235006=CARTESIAN_POINT('Ctrl Pts',(-4.28596058300006,15.2,10.433923239));
#235007=CARTESIAN_POINT('Ctrl Pts',(-4.28596058300006,11.6,10.433923239));
#235008=CARTESIAN_POINT('Ctrl Pts',(-4.28603703500006,15.2,10.430403819));
#235009=CARTESIAN_POINT('Ctrl Pts',(-4.28603703500006,11.6,10.430403819));
#235010=CARTESIAN_POINT('Ctrl Pts',(-4.28611064200005,15.2,10.42688907));
#235011=CARTESIAN_POINT('Ctrl Pts',(-4.28611064200005,11.6,10.42688907));
#235012=CARTESIAN_POINT('Ctrl Pts',(-4.28618140900006,15.2,10.423378997));
#235013=CARTESIAN_POINT('Ctrl Pts',(-4.28618140900006,11.6,10.423378997));
#235014=CARTESIAN_POINT('Ctrl Pts',(-4.28624934300006,15.2,10.419873611));
#235015=CARTESIAN_POINT('Ctrl Pts',(-4.28624934300006,11.6,10.419873611));
#235016=CARTESIAN_POINT('Ctrl Pts',(-4.28631444800006,15.2,10.41637292));
#235017=CARTESIAN_POINT('Ctrl Pts',(-4.28631444800006,11.6,10.41637292));
#235018=CARTESIAN_POINT('Ctrl Pts',(-4.28637673200006,15.2,10.41287693));
#235019=CARTESIAN_POINT('Ctrl Pts',(-4.28637673200006,11.6,10.41287693));
#235020=CARTESIAN_POINT('Ctrl Pts',(-4.28643620100006,15.2,10.409385651));
#235021=CARTESIAN_POINT('Ctrl Pts',(-4.28643620100006,11.6,10.409385651));
#235022=CARTESIAN_POINT('Ctrl Pts',(-4.28649285900006,15.2,10.405899089));
#235023=CARTESIAN_POINT('Ctrl Pts',(-4.28649285900006,11.6,10.405899089));
#235024=CARTESIAN_POINT('Ctrl Pts',(-4.28654671400006,15.2,10.402417252));
#235025=CARTESIAN_POINT('Ctrl Pts',(-4.28654671400006,11.6,10.402417252));
#235026=CARTESIAN_POINT('Ctrl Pts',(-4.28659777200005,15.2,10.39894015));
#235027=CARTESIAN_POINT('Ctrl Pts',(-4.28659777200005,11.6,10.39894015));
#235028=CARTESIAN_POINT('Ctrl Pts',(-4.28664603900006,15.2,10.395467789));
#235029=CARTESIAN_POINT('Ctrl Pts',(-4.28664603900006,11.6,10.395467789));
#235030=CARTESIAN_POINT('Ctrl Pts',(-4.28669152200006,15.2,10.392000178));
#235031=CARTESIAN_POINT('Ctrl Pts',(-4.28669152200006,11.6,10.392000178));
#235032=CARTESIAN_POINT('Ctrl Pts',(-4.28673422400006,15.2,10.388537325));
#235033=CARTESIAN_POINT('Ctrl Pts',(-4.28673422400006,11.6,10.388537325));
#235034=CARTESIAN_POINT('Ctrl Pts',(-4.28677415500006,15.2,10.385079237));
#235035=CARTESIAN_POINT('Ctrl Pts',(-4.28677415500006,11.6,10.385079237));
#235036=CARTESIAN_POINT('Ctrl Pts',(-4.28681131900006,15.2,10.381625923));
#235037=CARTESIAN_POINT('Ctrl Pts',(-4.28681131900006,11.6,10.381625923));
#235038=CARTESIAN_POINT('Ctrl Pts',(-4.28684572400006,15.2,10.378177391));
#235039=CARTESIAN_POINT('Ctrl Pts',(-4.28684572400006,11.6,10.378177391));
#235040=CARTESIAN_POINT('Ctrl Pts',(-4.28687737400006,15.2,10.374733649));
#235041=CARTESIAN_POINT('Ctrl Pts',(-4.28687737400006,11.6,10.374733649));
#235042=CARTESIAN_POINT('Ctrl Pts',(-4.28690627700006,15.2,10.371294705));
#235043=CARTESIAN_POINT('Ctrl Pts',(-4.28690627700006,11.6,10.371294705));
#235044=CARTESIAN_POINT('Ctrl Pts',(-4.28693243800006,15.2,10.367860566));
#235045=CARTESIAN_POINT('Ctrl Pts',(-4.28693243800006,11.6,10.367860566));
#235046=CARTESIAN_POINT('Ctrl Pts',(-4.28695586400006,15.2,10.364431242));
#235047=CARTESIAN_POINT('Ctrl Pts',(-4.28695586400006,11.6,10.364431242));
#235048=CARTESIAN_POINT('Ctrl Pts',(-4.28697656200006,15.2,10.361006739));
#235049=CARTESIAN_POINT('Ctrl Pts',(-4.28697656200006,11.6,10.361006739));
#235050=CARTESIAN_POINT('Ctrl Pts',(-4.28699453700006,15.2,10.357587066));
#235051=CARTESIAN_POINT('Ctrl Pts',(-4.28699453700006,11.6,10.357587066));
#235052=CARTESIAN_POINT('Ctrl Pts',(-4.28700979600006,15.2,10.354172232));
#235053=CARTESIAN_POINT('Ctrl Pts',(-4.28700979600006,11.6,10.354172232));
#235054=CARTESIAN_POINT('Ctrl Pts',(-4.28702234600006,15.2,10.350762244));
#235055=CARTESIAN_POINT('Ctrl Pts',(-4.28702234600006,11.6,10.350762244));
#235056=CARTESIAN_POINT('Ctrl Pts',(-4.28703219200006,15.2,10.347357111));
#235057=CARTESIAN_POINT('Ctrl Pts',(-4.28703219200006,11.6,10.347357111));
#235058=CARTESIAN_POINT('Ctrl Pts',(-4.28703934200006,15.2,10.34395684));
#235059=CARTESIAN_POINT('Ctrl Pts',(-4.28703934200006,11.6,10.34395684));
#235060=CARTESIAN_POINT('Ctrl Pts',(-4.28704380100006,15.2,10.340561439));
#235061=CARTESIAN_POINT('Ctrl Pts',(-4.28704380100006,11.6,10.340561439));
#235062=CARTESIAN_POINT('Ctrl Pts',(-4.28704557600006,15.2,10.337170919));
#235063=CARTESIAN_POINT('Ctrl Pts',(-4.28704557600006,11.6,10.337170919));
#235064=CARTESIAN_POINT('Ctrl Pts',(-4.28704467500006,15.2,10.333785284));
#235065=CARTESIAN_POINT('Ctrl Pts',(-4.28704467500006,11.6,10.333785284));
#235066=CARTESIAN_POINT('Ctrl Pts',(-4.28704110100006,15.2,10.330404545));
#235067=CARTESIAN_POINT('Ctrl Pts',(-4.28704110100006,11.6,10.330404545));
#235068=CARTESIAN_POINT('Ctrl Pts',(-4.28703486500006,15.2,10.327028709));
#235069=CARTESIAN_POINT('Ctrl Pts',(-4.28703486500006,11.6,10.327028709));
#235070=CARTESIAN_POINT('Ctrl Pts',(-4.28702596900005,15.2,10.323657785));
#235071=CARTESIAN_POINT('Ctrl Pts',(-4.28702596900005,11.6,10.323657785));
#235072=CARTESIAN_POINT('Ctrl Pts',(-4.28701442200006,15.2,10.32029178));
#235073=CARTESIAN_POINT('Ctrl Pts',(-4.28701442200006,11.6,10.32029178));
#235074=CARTESIAN_POINT('Ctrl Pts',(-4.28700023100006,15.2,10.316930703));
#235075=CARTESIAN_POINT('Ctrl Pts',(-4.28700023100006,11.6,10.316930703));
#235076=CARTESIAN_POINT('Ctrl Pts',(-4.28698340200006,15.2,10.313574563));
#235077=CARTESIAN_POINT('Ctrl Pts',(-4.28698340200006,11.6,10.313574563));
#235078=CARTESIAN_POINT('Ctrl Pts',(-4.28696394100006,15.2,10.310223367));
#235079=CARTESIAN_POINT('Ctrl Pts',(-4.28696394100006,11.6,10.310223367));
#235080=CARTESIAN_POINT('Ctrl Pts',(-4.28694185400006,15.2,10.306877124));
#235081=CARTESIAN_POINT('Ctrl Pts',(-4.28694185400006,11.6,10.306877124));
#235082=CARTESIAN_POINT('Ctrl Pts',(-4.28691715100006,15.2,10.303535841));
#235083=CARTESIAN_POINT('Ctrl Pts',(-4.28691715100006,11.6,10.303535841));
#235084=CARTESIAN_POINT('Ctrl Pts',(-4.28688983500006,15.2,10.300199529));
#235085=CARTESIAN_POINT('Ctrl Pts',(-4.28688983500006,11.6,10.300199529));
#235086=CARTESIAN_POINT('Ctrl Pts',(-4.28685991400005,15.2,10.296868193));
#235087=CARTESIAN_POINT('Ctrl Pts',(-4.28685991400005,11.6,10.296868193));
#235088=CARTESIAN_POINT('Ctrl Pts',(-4.28682739500006,15.2,10.293541843));
#235089=CARTESIAN_POINT('Ctrl Pts',(-4.28682739500006,11.6,10.293541843));
#235090=CARTESIAN_POINT('Ctrl Pts',(-4.28679228500005,15.2,10.290220487));
#235091=CARTESIAN_POINT('Ctrl Pts',(-4.28679228500005,11.6,10.290220487));
#235092=CARTESIAN_POINT('Ctrl Pts',(-4.28675459000006,15.2,10.286904134));
#235093=CARTESIAN_POINT('Ctrl Pts',(-4.28675459000006,11.6,10.286904134));
#235094=CARTESIAN_POINT('Ctrl Pts',(-4.28671431600006,15.2,10.283592791));
#235095=CARTESIAN_POINT('Ctrl Pts',(-4.28671431600006,11.6,10.283592791));
#235096=CARTESIAN_POINT('Ctrl Pts',(-4.28667147200006,15.2,10.280286467));
#235097=CARTESIAN_POINT('Ctrl Pts',(-4.28667147200006,11.6,10.280286467));
#235098=CARTESIAN_POINT('Ctrl Pts',(-4.28662606400006,15.2,10.276985171));
#235099=CARTESIAN_POINT('Ctrl Pts',(-4.28662606400006,11.6,10.276985171));
#235100=CARTESIAN_POINT('Ctrl Pts',(-4.28657809700006,15.2,10.27368891));
#235101=CARTESIAN_POINT('Ctrl Pts',(-4.28657809700006,11.6,10.27368891));
#235102=CARTESIAN_POINT('Ctrl Pts',(-4.28652758000006,15.2,10.270397693));
#235103=CARTESIAN_POINT('Ctrl Pts',(-4.28652758000006,11.6,10.270397693));
#235104=CARTESIAN_POINT('Ctrl Pts',(-4.28647452000006,15.2,10.267111529));
#235105=CARTESIAN_POINT('Ctrl Pts',(-4.28647452000006,11.6,10.267111529));
#235106=CARTESIAN_POINT('Ctrl Pts',(-4.28641892300006,15.2,10.263830426));
#235107=CARTESIAN_POINT('Ctrl Pts',(-4.28641892300006,11.6,10.263830426));
#235108=CARTESIAN_POINT('Ctrl Pts',(-4.28636079500006,15.2,10.260554392));
#235109=CARTESIAN_POINT('Ctrl Pts',(-4.28636079500006,11.6,10.260554392));
#235110=CARTESIAN_POINT('Ctrl Pts',(-4.28630014400006,15.2,10.257283436));
#235111=CARTESIAN_POINT('Ctrl Pts',(-4.28630014400006,11.6,10.257283436));
#235112=CARTESIAN_POINT('Ctrl Pts',(-4.28623697700006,15.2,10.254017566));
#235113=CARTESIAN_POINT('Ctrl Pts',(-4.28623697700006,11.6,10.254017566));
#235114=CARTESIAN_POINT('Ctrl Pts',(-4.28617130100006,15.2,10.25075679));
#235115=CARTESIAN_POINT('Ctrl Pts',(-4.28617130100006,11.6,10.25075679));
#235116=CARTESIAN_POINT('Ctrl Pts',(-4.28610312300005,15.2,10.247501117));
#235117=CARTESIAN_POINT('Ctrl Pts',(-4.28610312300005,11.6,10.247501117));
#235118=CARTESIAN_POINT('Ctrl Pts',(-4.28603245100006,15.2,10.244250555));
#235119=CARTESIAN_POINT('Ctrl Pts',(-4.28603245100006,11.6,10.244250555));
#235120=CARTESIAN_POINT('Ctrl Pts',(-4.28595928900006,15.2,10.241005114));
#235121=CARTESIAN_POINT('Ctrl Pts',(-4.28595928900006,11.6,10.241005114));
#235122=CARTESIAN_POINT('Ctrl Pts',(-4.28588364700006,15.2,10.237764801));
#235123=CARTESIAN_POINT('Ctrl Pts',(-4.28588364700006,11.6,10.237764801));
#235124=CARTESIAN_POINT('Ctrl Pts',(-4.28580553100006,15.2,10.234529626));
#235125=CARTESIAN_POINT('Ctrl Pts',(-4.28580553100006,11.6,10.234529626));
#235126=CARTESIAN_POINT('Ctrl Pts',(-4.28572494800005,15.2,10.231299595));
#235127=CARTESIAN_POINT('Ctrl Pts',(-4.28572494800005,11.6,10.231299595));
#235128=CARTESIAN_POINT('Ctrl Pts',(-4.28564190400006,15.2,10.228074718));
#235129=CARTESIAN_POINT('Ctrl Pts',(-4.28564190400006,11.6,10.228074718));
#235130=CARTESIAN_POINT('Ctrl Pts',(-4.28555640900006,15.2,10.224855003));
#235131=CARTESIAN_POINT('Ctrl Pts',(-4.28555640900006,11.6,10.224855003));
#235132=CARTESIAN_POINT('Ctrl Pts',(-4.28546846800006,15.2,10.22164046));
#235133=CARTESIAN_POINT('Ctrl Pts',(-4.28546846800006,11.6,10.22164046));
#235134=CARTESIAN_POINT('Ctrl Pts',(-4.28537809000006,15.2,10.218431096));
#235135=CARTESIAN_POINT('Ctrl Pts',(-4.28537809000006,11.6,10.218431096));
#235136=CARTESIAN_POINT('Ctrl Pts',(-4.28528527900006,15.2,10.215226921));
#235137=CARTESIAN_POINT('Ctrl Pts',(-4.28528527900006,11.6,10.215226921));
#235138=CARTESIAN_POINT('Ctrl Pts',(-4.28519004500005,15.2,10.212027942));
#235139=CARTESIAN_POINT('Ctrl Pts',(-4.28519004500005,11.6,10.212027942));
#235140=CARTESIAN_POINT('Ctrl Pts',(-4.28509239400006,15.2,10.208834168));
#235141=CARTESIAN_POINT('Ctrl Pts',(-4.28509239400006,11.6,10.208834168));
#235142=CARTESIAN_POINT('Ctrl Pts',(-4.28499233400006,15.2,10.205645608));
#235143=CARTESIAN_POINT('Ctrl Pts',(-4.28499233400006,11.6,10.205645608));
#235144=CARTESIAN_POINT('Ctrl Pts',(-4.28488987300006,15.2,10.202462271));
#235145=CARTESIAN_POINT('Ctrl Pts',(-4.28488987300006,11.6,10.202462271));
#235146=CARTESIAN_POINT('Ctrl Pts',(-4.28478501700006,15.2,10.199284165));
#235147=CARTESIAN_POINT('Ctrl Pts',(-4.28478501700006,11.6,10.199284165));
#235148=CARTESIAN_POINT('Ctrl Pts',(-4.28467777300006,15.2,10.196111298));
#235149=CARTESIAN_POINT('Ctrl Pts',(-4.28467777300006,11.6,10.196111298));
#235150=CARTESIAN_POINT('Ctrl Pts',(-4.28456814900006,15.2,10.19294368));
#235151=CARTESIAN_POINT('Ctrl Pts',(-4.28456814900006,11.6,10.19294368));
#235152=CARTESIAN_POINT('Ctrl Pts',(-4.28445615200006,15.2,10.189781319));
#235153=CARTESIAN_POINT('Ctrl Pts',(-4.28445615200006,11.6,10.189781319));
#235154=CARTESIAN_POINT('Ctrl Pts',(-4.28434179100006,15.2,10.186624224));
#235155=CARTESIAN_POINT('Ctrl Pts',(-4.28434179100006,11.6,10.186624224));
#235156=CARTESIAN_POINT('Ctrl Pts',(-4.28422507200006,15.2,10.183472403));
#235157=CARTESIAN_POINT('Ctrl Pts',(-4.28422507200006,11.6,10.183472403));
#235158=CARTESIAN_POINT('Ctrl Pts',(-4.28410600200006,15.2,10.180325865));
#235159=CARTESIAN_POINT('Ctrl Pts',(-4.28410600200006,11.6,10.180325865));
#235160=CARTESIAN_POINT('Ctrl Pts',(-4.28398458900006,15.2,10.177184619));
#235161=CARTESIAN_POINT('Ctrl Pts',(-4.28398458900006,11.6,10.177184619));
#235162=CARTESIAN_POINT('Ctrl Pts',(-4.28386084200006,15.2,10.174048675));
#235163=CARTESIAN_POINT('Ctrl Pts',(-4.28386084200006,11.6,10.174048675));
#235164=CARTESIAN_POINT('Ctrl Pts',(-4.28373476600005,15.2,10.170918039));
#235165=CARTESIAN_POINT('Ctrl Pts',(-4.28373476600005,11.6,10.170918039));
#235166=CARTESIAN_POINT('Ctrl Pts',(-4.28360637100006,15.2,10.167792721));
#235167=CARTESIAN_POINT('Ctrl Pts',(-4.28360637100006,11.6,10.167792721));
#235168=CARTESIAN_POINT('Ctrl Pts',(-4.28347566200006,15.2,10.16467273));
#235169=CARTESIAN_POINT('Ctrl Pts',(-4.28347566200006,11.6,10.16467273));
#235170=CARTESIAN_POINT('Ctrl Pts',(-4.28334264800006,15.2,10.161558074));
#235171=CARTESIAN_POINT('Ctrl Pts',(-4.28334264800006,11.6,10.161558074));
#235172=CARTESIAN_POINT('Ctrl Pts',(-4.28320733700006,15.2,10.158448764));
#235173=CARTESIAN_POINT('Ctrl Pts',(-4.28320733700006,11.6,10.158448764));
#235174=CARTESIAN_POINT('Ctrl Pts',(-4.28306973600006,15.2,10.155344806));
#235175=CARTESIAN_POINT('Ctrl Pts',(-4.28306973600006,11.6,10.155344806));
#235176=CARTESIAN_POINT('Ctrl Pts',(-4.28292985300006,15.2,10.15224621));
#235177=CARTESIAN_POINT('Ctrl Pts',(-4.28292985300006,11.6,10.15224621));
#235178=CARTESIAN_POINT('Ctrl Pts',(-4.28278769500006,15.2,10.149152986));
#235179=CARTESIAN_POINT('Ctrl Pts',(-4.28278769500006,11.6,10.149152986));
#235180=CARTESIAN_POINT('Ctrl Pts',(-4.28264327100006,15.2,10.146065141));
#235181=CARTESIAN_POINT('Ctrl Pts',(-4.28264327100006,11.6,10.146065141));
#235182=CARTESIAN_POINT('Ctrl Pts',(-4.28249658600006,15.2,10.142982684));
#235183=CARTESIAN_POINT('Ctrl Pts',(-4.28249658600006,11.6,10.142982684));
#235184=CARTESIAN_POINT('Ctrl Pts',(-4.28234765100005,15.2,10.139905626));
#235185=CARTESIAN_POINT('Ctrl Pts',(-4.28234765100005,11.6,10.139905626));
#235186=CARTESIAN_POINT('Ctrl Pts',(-4.28219647300006,15.2,10.136833973));
#235187=CARTESIAN_POINT('Ctrl Pts',(-4.28219647300006,11.6,10.136833973));
#235188=CARTESIAN_POINT('Ctrl Pts',(-4.28204305800006,15.2,10.133767736));
#235189=CARTESIAN_POINT('Ctrl Pts',(-4.28204305800006,11.6,10.133767736));
#235190=CARTESIAN_POINT('Ctrl Pts',(-4.28188741600006,15.2,10.130706923));
#235191=CARTESIAN_POINT('Ctrl Pts',(-4.28188741600006,11.6,10.130706923));
#235192=CARTESIAN_POINT('Ctrl Pts',(-4.28172955300006,15.2,10.127651543));
#235193=CARTESIAN_POINT('Ctrl Pts',(-4.28172955300006,11.6,10.127651543));
#235194=CARTESIAN_POINT('Ctrl Pts',(-4.28156947900006,15.2,10.124601605));
#235195=CARTESIAN_POINT('Ctrl Pts',(-4.28156947900006,11.6,10.124601605));
#235196=CARTESIAN_POINT('Ctrl Pts',(-4.28140720000005,15.2,10.121557118));
#235197=CARTESIAN_POINT('Ctrl Pts',(-4.28140720000005,11.6,10.121557118));
#235198=CARTESIAN_POINT('Ctrl Pts',(-4.28124272500006,15.2,10.118518091));
#235199=CARTESIAN_POINT('Ctrl Pts',(-4.28124272500006,11.6,10.118518091));
#235200=CARTESIAN_POINT('Ctrl Pts',(-4.28107606100006,15.2,10.115484532));
#235201=CARTESIAN_POINT('Ctrl Pts',(-4.28107606100006,11.6,10.115484532));
#235202=CARTESIAN_POINT('Ctrl Pts',(-4.28090721700006,15.2,10.112456452));
#235203=CARTESIAN_POINT('Ctrl Pts',(-4.28090721700006,11.6,10.112456452));
#235204=CARTESIAN_POINT('Ctrl Pts',(-4.28073620000006,15.2,10.109433858));
#235205=CARTESIAN_POINT('Ctrl Pts',(-4.28073620000006,11.6,10.109433858));
#235206=CARTESIAN_POINT('Ctrl Pts',(-4.28056301900006,15.2,10.106416761));
#235207=CARTESIAN_POINT('Ctrl Pts',(-4.28056301900006,11.6,10.106416761));
#235208=CARTESIAN_POINT('Ctrl Pts',(-4.28038768100006,15.2,10.103405168));
#235209=CARTESIAN_POINT('Ctrl Pts',(-4.28038768100006,11.6,10.103405168));
#235210=CARTESIAN_POINT('Ctrl Pts',(-4.28021019500005,15.2,10.10039909));
#235211=CARTESIAN_POINT('Ctrl Pts',(-4.28021019500005,11.6,10.10039909));
#235212=CARTESIAN_POINT('Ctrl Pts',(-4.28003056900006,15.2,10.097398534));
#235213=CARTESIAN_POINT('Ctrl Pts',(-4.28003056900006,11.6,10.097398534));
#235214=CARTESIAN_POINT('Ctrl Pts',(-4.27984881000006,15.2,10.094403512));
#235215=CARTESIAN_POINT('Ctrl Pts',(-4.27984881000006,11.6,10.094403512));
#235216=CARTESIAN_POINT('Ctrl Pts',(-4.27966492800006,15.2,10.09141403));
#235217=CARTESIAN_POINT('Ctrl Pts',(-4.27966492800006,11.6,10.09141403));
#235218=CARTESIAN_POINT('Ctrl Pts',(-4.27947893000006,15.2,10.088430098));
#235219=CARTESIAN_POINT('Ctrl Pts',(-4.27947893000006,11.6,10.088430098));
#235220=CARTESIAN_POINT('Ctrl Pts',(-4.27929082400006,15.2,10.085451726));
#235221=CARTESIAN_POINT('Ctrl Pts',(-4.27929082400006,11.6,10.085451726));
#235222=CARTESIAN_POINT('Ctrl Pts',(-4.27910061900006,15.2,10.082478922));
#235223=CARTESIAN_POINT('Ctrl Pts',(-4.27910061900006,11.6,10.082478922));
#235224=CARTESIAN_POINT('Ctrl Pts',(-4.27890832200006,15.2,10.079511697));
#235225=CARTESIAN_POINT('Ctrl Pts',(-4.27890832200006,11.6,10.079511697));
#235226=CARTESIAN_POINT('Ctrl Pts',(-4.27871394300006,15.2,10.076550059));
#235227=CARTESIAN_POINT('Ctrl Pts',(-4.27871394300006,11.6,10.076550059));
#235228=CARTESIAN_POINT('Ctrl Pts',(-4.27851748900006,15.2,10.073594016));
#235229=CARTESIAN_POINT('Ctrl Pts',(-4.27851748900006,11.6,10.073594016));
#235230=CARTESIAN_POINT('Ctrl Pts',(-4.27831896900006,15.2,10.070643579));
#235231=CARTESIAN_POINT('Ctrl Pts',(-4.27831896900006,11.6,10.070643579));
#235232=CARTESIAN_POINT('Ctrl Pts',(-4.27811839100006,15.2,10.067698756));
#235233=CARTESIAN_POINT('Ctrl Pts',(-4.27811839100006,11.6,10.067698756));
#235234=CARTESIAN_POINT('Ctrl Pts',(-4.27791576400006,15.2,10.064759557));
#235235=CARTESIAN_POINT('Ctrl Pts',(-4.27791576400006,11.6,10.064759557));
#235236=CARTESIAN_POINT('Ctrl Pts',(-4.27771109500005,15.2,10.061825991));
#235237=CARTESIAN_POINT('Ctrl Pts',(-4.27771109500005,11.6,10.061825991));
#235238=CARTESIAN_POINT('Ctrl Pts',(-4.27750439400006,15.2,10.058898068));
#235239=CARTESIAN_POINT('Ctrl Pts',(-4.27750439400006,11.6,10.058898068));
#235240=CARTESIAN_POINT('Ctrl Pts',(-4.27729566900005,15.2,10.055975795));
#235241=CARTESIAN_POINT('Ctrl Pts',(-4.27729566900005,11.6,10.055975795));
#235242=CARTESIAN_POINT('Ctrl Pts',(-4.27708492800006,15.2,10.053059184));
#235243=CARTESIAN_POINT('Ctrl Pts',(-4.27708492800006,11.6,10.053059184));
#235244=CARTESIAN_POINT('Ctrl Pts',(-4.27687217900006,15.2,10.050148243));
#235245=CARTESIAN_POINT('Ctrl Pts',(-4.27687217900006,11.6,10.050148243));
#235246=CARTESIAN_POINT('Ctrl Pts',(-4.27665743200006,15.2,10.047242981));
#235247=CARTESIAN_POINT('Ctrl Pts',(-4.27665743200006,11.6,10.047242981));
#235248=CARTESIAN_POINT('Ctrl Pts',(-4.27644069500006,15.2,10.044343408));
#235249=CARTESIAN_POINT('Ctrl Pts',(-4.27644069500006,11.6,10.044343408));
#235250=CARTESIAN_POINT('Ctrl Pts',(-4.27622197600006,15.2,10.041449533));
#235251=CARTESIAN_POINT('Ctrl Pts',(-4.27622197600006,11.6,10.041449533));
#235252=CARTESIAN_POINT('Ctrl Pts',(-4.27600128400006,15.2,10.038561365));
#235253=CARTESIAN_POINT('Ctrl Pts',(-4.27600128400006,11.6,10.038561365));
#235254=CARTESIAN_POINT('Ctrl Pts',(-4.27577862800006,15.2,10.035678915));
#235255=CARTESIAN_POINT('Ctrl Pts',(-4.27577862800006,11.6,10.035678915));
#235256=CARTESIAN_POINT('Ctrl Pts',(-4.27555401700006,15.2,10.032802191));
#235257=CARTESIAN_POINT('Ctrl Pts',(-4.27555401700006,11.6,10.032802191));
#235258=CARTESIAN_POINT('Ctrl Pts',(-4.27532745900006,15.2,10.029931202));
#235259=CARTESIAN_POINT('Ctrl Pts',(-4.27532745900006,11.6,10.029931202));
#235260=CARTESIAN_POINT('Ctrl Pts',(-4.27509896100006,15.2,10.027065958));
#235261=CARTESIAN_POINT('Ctrl Pts',(-4.27509896100006,11.6,10.027065958));
#235262=CARTESIAN_POINT('Ctrl Pts',(-4.27486853600006,15.2,10.024206469));
#235263=CARTESIAN_POINT('Ctrl Pts',(-4.27486853600006,11.6,10.024206469));
#235264=CARTESIAN_POINT('Ctrl Pts',(-4.27463618900005,15.2,10.021352743));
#235265=CARTESIAN_POINT('Ctrl Pts',(-4.27463618900005,11.6,10.021352743));
#235266=CARTESIAN_POINT('Ctrl Pts',(-4.27440193100006,15.2,10.018504792));
#235267=CARTESIAN_POINT('Ctrl Pts',(-4.27440193100006,11.6,10.018504792));
#235268=CARTESIAN_POINT('Ctrl Pts',(-4.27416577000006,15.2,10.015662623));
#235269=CARTESIAN_POINT('Ctrl Pts',(-4.27416577000006,11.6,10.015662623));
#235270=CARTESIAN_POINT('Ctrl Pts',(-4.27392771400006,15.2,10.012826246));
#235271=CARTESIAN_POINT('Ctrl Pts',(-4.27392771400006,11.6,10.012826246));
#235272=CARTESIAN_POINT('Ctrl Pts',(-4.27368777400006,15.2,10.009995672));
#235273=CARTESIAN_POINT('Ctrl Pts',(-4.27368777400006,11.6,10.009995672));
#235274=CARTESIAN_POINT('Ctrl Pts',(-4.27344595700006,15.2,10.007170908));
#235275=CARTESIAN_POINT('Ctrl Pts',(-4.27344595700006,11.6,10.007170908));
#235276=CARTESIAN_POINT('Ctrl Pts',(-4.27320227300005,15.2,10.004351966));
#235277=CARTESIAN_POINT('Ctrl Pts',(-4.27320227300005,11.6,10.004351966));
#235278=CARTESIAN_POINT('Ctrl Pts',(-4.27295673100006,15.2,10.001538855));
#235279=CARTESIAN_POINT('Ctrl Pts',(-4.27295673100006,11.6,10.001538855));
#235280=CARTESIAN_POINT('Ctrl Pts',(-4.27270933900005,15.2,9.99873158399998));
#235281=CARTESIAN_POINT('Ctrl Pts',(-4.27270933900005,11.6,9.99873158399998));
#235282=CARTESIAN_POINT('Ctrl Pts',(-4.27246010700006,15.2,9.99593016199999));
#235283=CARTESIAN_POINT('Ctrl Pts',(-4.27246010700006,11.6,9.99593016199999));
#235284=CARTESIAN_POINT('Ctrl Pts',(-4.27220904400006,15.2,9.99313459999998));
#235285=CARTESIAN_POINT('Ctrl Pts',(-4.27220904400006,11.6,9.99313459999998));
#235286=CARTESIAN_POINT('Ctrl Pts',(-4.27195615900006,15.2,9.99034490599998));
#235287=CARTESIAN_POINT('Ctrl Pts',(-4.27195615900006,11.6,9.99034490599998));
#235288=CARTESIAN_POINT('Ctrl Pts',(-4.27170146000006,15.2,9.98756109299999));
#235289=CARTESIAN_POINT('Ctrl Pts',(-4.27170146000006,11.6,9.98756109299999));
#235290=CARTESIAN_POINT('Ctrl Pts',(-4.27144495900006,15.2,9.98478316599999));
#235291=CARTESIAN_POINT('Ctrl Pts',(-4.27144495900006,11.6,9.98478316599999));
#235292=CARTESIAN_POINT('Ctrl Pts',(-4.27118666200006,15.2,9.98201113799999));
#235293=CARTESIAN_POINT('Ctrl Pts',(-4.27118666200006,11.6,9.98201113799999));
#235294=CARTESIAN_POINT('Ctrl Pts',(-4.27092658000006,15.2,9.97924501799999));
#235295=CARTESIAN_POINT('Ctrl Pts',(-4.27092658000006,11.6,9.97924501799999));
#235296=CARTESIAN_POINT('Ctrl Pts',(-4.27066472200006,15.2,9.97648481499999));
#235297=CARTESIAN_POINT('Ctrl Pts',(-4.27066472200006,11.6,9.97648481499999));
#235298=CARTESIAN_POINT('Ctrl Pts',(-4.27040109700005,15.2,9.97373053899998));
#235299=CARTESIAN_POINT('Ctrl Pts',(-4.27040109700005,11.6,9.97373053899998));
#235300=CARTESIAN_POINT('Ctrl Pts',(-4.27013571500006,15.2,9.97098220099998));
#235301=CARTESIAN_POINT('Ctrl Pts',(-4.27013571500006,11.6,9.97098220099998));
#235302=CARTESIAN_POINT('Ctrl Pts',(-4.26986858400006,15.2,9.96823980899999));
#235303=CARTESIAN_POINT('Ctrl Pts',(-4.26986858400006,11.6,9.96823980899999));
#235304=CARTESIAN_POINT('Ctrl Pts',(-4.26959971500006,15.2,9.96550337299999));
#235305=CARTESIAN_POINT('Ctrl Pts',(-4.26959971500006,11.6,9.96550337299999));
#235306=CARTESIAN_POINT('Ctrl Pts',(-4.26932911600006,15.2,9.96277290399998));
#235307=CARTESIAN_POINT('Ctrl Pts',(-4.26932911600006,11.6,9.96277290399998));
#235308=CARTESIAN_POINT('Ctrl Pts',(-4.26905679700006,15.2,9.96004841099998));
#235309=CARTESIAN_POINT('Ctrl Pts',(-4.26905679700006,11.6,9.96004841099998));
#235310=CARTESIAN_POINT('Ctrl Pts',(-4.26878276800006,15.2,9.95732990399999));
#235311=CARTESIAN_POINT('Ctrl Pts',(-4.26878276800006,11.6,9.95732990399999));
#235312=CARTESIAN_POINT('Ctrl Pts',(-4.26850703700006,15.2,9.95461739299999));
#235313=CARTESIAN_POINT('Ctrl Pts',(-4.26850703700006,11.6,9.95461739299999));
#235314=CARTESIAN_POINT('Ctrl Pts',(-4.26822961600006,15.2,9.95191088699999));
#235315=CARTESIAN_POINT('Ctrl Pts',(-4.26822961600006,11.6,9.95191088699999));
#235316=CARTESIAN_POINT('Ctrl Pts',(-4.26795051200005,15.2,9.94921039699998));
#235317=CARTESIAN_POINT('Ctrl Pts',(-4.26795051200005,11.6,9.94921039699998));
#235318=CARTESIAN_POINT('Ctrl Pts',(-4.26766973600006,15.2,9.94651593299999));
#235319=CARTESIAN_POINT('Ctrl Pts',(-4.26766973600006,11.6,9.94651593299999));
#235320=CARTESIAN_POINT('Ctrl Pts',(-4.26738729700006,15.2,9.94382750399998));
#235321=CARTESIAN_POINT('Ctrl Pts',(-4.26738729700006,11.6,9.94382750399998));
#235322=CARTESIAN_POINT('Ctrl Pts',(-4.26710320500006,15.2,9.94114511999998));
#235323=CARTESIAN_POINT('Ctrl Pts',(-4.26710320500006,11.6,9.94114511999998));
#235324=CARTESIAN_POINT('Ctrl Pts',(-4.26681747000006,15.2,9.93846879199998));
#235325=CARTESIAN_POINT('Ctrl Pts',(-4.26681747000006,11.6,9.93846879199998));
#235326=CARTESIAN_POINT('Ctrl Pts',(-4.26653010100006,15.2,9.93579852999999));
#235327=CARTESIAN_POINT('Ctrl Pts',(-4.26653010100006,11.6,9.93579852999999));
#235328=CARTESIAN_POINT('Ctrl Pts',(-4.26624110800006,15.2,9.93313434199998));
#235329=CARTESIAN_POINT('Ctrl Pts',(-4.26624110800006,11.6,9.93313434199998));
#235330=CARTESIAN_POINT('Ctrl Pts',(-4.26595050100006,15.2,9.93047623999999));
#235331=CARTESIAN_POINT('Ctrl Pts',(-4.26595050100006,11.6,9.93047623999999));
#235332=CARTESIAN_POINT('Ctrl Pts',(-4.26565828900006,15.2,9.92782423299998));
#235333=CARTESIAN_POINT('Ctrl Pts',(-4.26565828900006,11.6,9.92782423299998));
#235334=CARTESIAN_POINT('Ctrl Pts',(-4.26536448300006,15.2,9.92517833199998));
#235335=CARTESIAN_POINT('Ctrl Pts',(-4.26536448300006,11.6,9.92517833199998));
#235336=CARTESIAN_POINT('Ctrl Pts',(-4.26506909200006,15.2,9.92253854599999));
#235337=CARTESIAN_POINT('Ctrl Pts',(-4.26506909200006,11.6,9.92253854599999));
#235338=CARTESIAN_POINT('Ctrl Pts',(-4.26477212700005,15.2,9.91990488699999));
#235339=CARTESIAN_POINT('Ctrl Pts',(-4.26477212700005,11.6,9.91990488699999));
#235340=CARTESIAN_POINT('Ctrl Pts',(-4.26447359700005,15.2,9.91727736199999));
#235341=CARTESIAN_POINT('Ctrl Pts',(-4.26447359700005,11.6,9.91727736199999));
#235342=CARTESIAN_POINT('Ctrl Pts',(-4.26417351300006,15.2,9.91465598399999));
#235343=CARTESIAN_POINT('Ctrl Pts',(-4.26417351300006,11.6,9.91465598399999));
#235344=CARTESIAN_POINT('Ctrl Pts',(-4.26387188300006,15.2,9.91204076199999));
#235345=CARTESIAN_POINT('Ctrl Pts',(-4.26387188300006,11.6,9.91204076199999));
#235346=CARTESIAN_POINT('Ctrl Pts',(-4.26356871900006,15.2,9.90943170599999));
#235347=CARTESIAN_POINT('Ctrl Pts',(-4.26356871900006,11.6,9.90943170599999));
#235348=CARTESIAN_POINT('Ctrl Pts',(-4.26326403000005,15.2,9.90682882699998));
#235349=CARTESIAN_POINT('Ctrl Pts',(-4.26326403000005,11.6,9.90682882699998));
#235350=CARTESIAN_POINT('Ctrl Pts',(-4.26295782600006,15.2,9.90423213399998));
#235351=CARTESIAN_POINT('Ctrl Pts',(-4.26295782600006,11.6,9.90423213399998));
#235352=CARTESIAN_POINT('Ctrl Pts',(-4.26265011800006,15.2,9.90164163799999));
#235353=CARTESIAN_POINT('Ctrl Pts',(-4.26265011800006,11.6,9.90164163799999));
#235354=CARTESIAN_POINT('Ctrl Pts',(-4.26234091700006,15.2,9.89905734999999));
#235355=CARTESIAN_POINT('Ctrl Pts',(-4.26234091700006,11.6,9.89905734999999));
#235356=CARTESIAN_POINT('Ctrl Pts',(-4.26203023000006,15.2,9.89647927799999));
#235357=CARTESIAN_POINT('Ctrl Pts',(-4.26203023000006,11.6,9.89647927799999));
#235358=CARTESIAN_POINT('Ctrl Pts',(-4.26171807100006,15.2,9.89390743499998));
#235359=CARTESIAN_POINT('Ctrl Pts',(-4.26171807100006,11.6,9.89390743499998));
#235360=CARTESIAN_POINT('Ctrl Pts',(-4.26140444800006,15.2,9.89134182899999));
#235361=CARTESIAN_POINT('Ctrl Pts',(-4.26140444800006,11.6,9.89134182899999));
#235362=CARTESIAN_POINT('Ctrl Pts',(-4.26108937200006,15.2,9.88878247099999));
#235363=CARTESIAN_POINT('Ctrl Pts',(-4.26108937200006,11.6,9.88878247099999));
#235364=CARTESIAN_POINT('Ctrl Pts',(-4.26077285200006,15.2,9.88622937299999));
#235365=CARTESIAN_POINT('Ctrl Pts',(-4.26077285200006,11.6,9.88622937299999));
#235366=CARTESIAN_POINT('Ctrl Pts',(-4.26045490200006,15.2,9.88368254399998));
#235367=CARTESIAN_POINT('Ctrl Pts',(-4.26045490200006,11.6,9.88368254399998));
#235368=CARTESIAN_POINT('Ctrl Pts',(-4.26013552800006,15.2,9.88114199399998));
#235369=CARTESIAN_POINT('Ctrl Pts',(-4.26013552800006,11.6,9.88114199399998));
#235370=CARTESIAN_POINT('Ctrl Pts',(-4.25981474300006,15.2,9.87860773299998));
#235371=CARTESIAN_POINT('Ctrl Pts',(-4.25981474300006,11.6,9.87860773299998));
#235372=CARTESIAN_POINT('Ctrl Pts',(-4.25949255700006,15.2,9.87607977399998));
#235373=CARTESIAN_POINT('Ctrl Pts',(-4.25949255700006,11.6,9.87607977399998));
#235374=CARTESIAN_POINT('Ctrl Pts',(-4.25916898100006,15.2,9.87355812399999));
#235375=CARTESIAN_POINT('Ctrl Pts',(-4.25916898100006,11.6,9.87355812399999));
#235376=CARTESIAN_POINT('Ctrl Pts',(-4.25884402500006,15.2,9.87104279699999));
#235377=CARTESIAN_POINT('Ctrl Pts',(-4.25884402500006,11.6,9.87104279699999));
#235378=CARTESIAN_POINT('Ctrl Pts',(-4.25851769900006,15.2,9.86853380099999));
#235379=CARTESIAN_POINT('Ctrl Pts',(-4.25851769900006,11.6,9.86853380099999));
#235380=CARTESIAN_POINT('Ctrl Pts',(-4.25819001500006,15.2,9.86603114699999));
#235381=CARTESIAN_POINT('Ctrl Pts',(-4.25819001500006,11.6,9.86603114699999));
#235382=CARTESIAN_POINT('Ctrl Pts',(-4.25786098300006,15.2,9.86353484599999));
#235383=CARTESIAN_POINT('Ctrl Pts',(-4.25786098300006,11.6,9.86353484599999));
#235384=CARTESIAN_POINT('Ctrl Pts',(-4.25753061300005,15.2,9.86104490899999));
#235385=CARTESIAN_POINT('Ctrl Pts',(-4.25753061300005,11.6,9.86104490899999));
#235386=CARTESIAN_POINT('Ctrl Pts',(-4.25719891700005,15.2,9.85856134499999));
#235387=CARTESIAN_POINT('Ctrl Pts',(-4.25719891700005,11.6,9.85856134499999));
#235388=CARTESIAN_POINT('Ctrl Pts',(-4.25686590500006,15.2,9.85608416599998));
#235389=CARTESIAN_POINT('Ctrl Pts',(-4.25686590500006,11.6,9.85608416599998));
#235390=CARTESIAN_POINT('Ctrl Pts',(-4.25653158900006,15.2,9.85361338199999));
#235391=CARTESIAN_POINT('Ctrl Pts',(-4.25653158900006,11.6,9.85361338199999));
#235392=CARTESIAN_POINT('Ctrl Pts',(-4.25619597800006,15.2,9.85114900499998));
#235393=CARTESIAN_POINT('Ctrl Pts',(-4.25619597800006,11.6,9.85114900499998));
#235394=CARTESIAN_POINT('Ctrl Pts',(-4.25585908500006,15.2,9.84869104299998));
#235395=CARTESIAN_POINT('Ctrl Pts',(-4.25585908500006,11.6,9.84869104299998));
#235396=CARTESIAN_POINT('Ctrl Pts',(-4.25552091900006,15.2,9.84623950899999));
#235397=CARTESIAN_POINT('Ctrl Pts',(-4.25552091900006,11.6,9.84623950899999));
#235398=CARTESIAN_POINT('Ctrl Pts',(-4.25518149200006,15.2,9.84379441199999));
#235399=CARTESIAN_POINT('Ctrl Pts',(-4.25518149200006,11.6,9.84379441199999));
#235400=CARTESIAN_POINT('Ctrl Pts',(-4.25484081400006,15.2,9.84135576499998));
#235401=CARTESIAN_POINT('Ctrl Pts',(-4.25484081400006,11.6,9.84135576499998));
#235402=CARTESIAN_POINT('Ctrl Pts',(-4.25449889700006,15.2,9.83892357599998));
#235403=CARTESIAN_POINT('Ctrl Pts',(-4.25449889700006,11.6,9.83892357599998));
#235404=CARTESIAN_POINT('Ctrl Pts',(-4.25415575200006,15.2,9.83649785799999));
#235405=CARTESIAN_POINT('Ctrl Pts',(-4.25415575200006,11.6,9.83649785799999));
#235406=CARTESIAN_POINT('Ctrl Pts',(-4.25381139100006,15.2,9.83407861999999));
#235407=CARTESIAN_POINT('Ctrl Pts',(-4.25381139100006,11.6,9.83407861999999));
#235408=CARTESIAN_POINT('Ctrl Pts',(-4.25346582400006,15.2,9.83166587499999));
#235409=CARTESIAN_POINT('Ctrl Pts',(-4.25346582400006,11.6,9.83166587499999));
#235410=CARTESIAN_POINT('Ctrl Pts',(-4.25311906200006,15.2,9.82925963199998));
#235411=CARTESIAN_POINT('Ctrl Pts',(-4.25311906200006,11.6,9.82925963199998));
#235412=CARTESIAN_POINT('Ctrl Pts',(-4.25277111700006,15.2,9.82685990299998));
#235413=CARTESIAN_POINT('Ctrl Pts',(-4.25277111700006,11.6,9.82685990299998));
#235414=CARTESIAN_POINT('Ctrl Pts',(-4.25242199900006,15.2,9.82446669799998));
#235415=CARTESIAN_POINT('Ctrl Pts',(-4.25242199900006,11.6,9.82446669799998));
#235416=CARTESIAN_POINT('Ctrl Pts',(-4.25207172200006,15.2,9.82208002899998));
#235417=CARTESIAN_POINT('Ctrl Pts',(-4.25207172200006,11.6,9.82208002899998));
#235418=CARTESIAN_POINT('Ctrl Pts',(-4.25172029400006,15.2,9.81969990599998));
#235419=CARTESIAN_POINT('Ctrl Pts',(-4.25172029400006,11.6,9.81969990599998));
#235420=CARTESIAN_POINT('Ctrl Pts',(-4.25136773000006,15.2,9.81732633999999));
#235421=CARTESIAN_POINT('Ctrl Pts',(-4.25136773000006,11.6,9.81732633999999));
#235422=CARTESIAN_POINT('Ctrl Pts',(-4.25101403800006,15.2,9.81495934199998));
#235423=CARTESIAN_POINT('Ctrl Pts',(-4.25101403800006,11.6,9.81495934199998));
#235424=CARTESIAN_POINT('Ctrl Pts',(-4.25065923100005,15.2,9.81259892299999));
#235425=CARTESIAN_POINT('Ctrl Pts',(-4.25065923100005,11.6,9.81259892299999));
#235426=CARTESIAN_POINT('Ctrl Pts',(-4.25030332100006,15.2,9.81024509399998));
#235427=CARTESIAN_POINT('Ctrl Pts',(-4.25030332100006,11.6,9.81024509399998));
#235428=CARTESIAN_POINT('Ctrl Pts',(-4.24994631900006,15.2,9.80789786699999));
#235429=CARTESIAN_POINT('Ctrl Pts',(-4.24994631900006,11.6,9.80789786699999));
#235430=CARTESIAN_POINT('Ctrl Pts',(-4.24958823700006,15.2,9.80555725299999));
#235431=CARTESIAN_POINT('Ctrl Pts',(-4.24958823700006,11.6,9.80555725299999));
#235432=CARTESIAN_POINT('Ctrl Pts',(-4.24922908600006,15.2,9.80322326199998));
#235433=CARTESIAN_POINT('Ctrl Pts',(-4.24922908600006,11.6,9.80322326199998));
#235434=CARTESIAN_POINT('Ctrl Pts',(-4.24886887800006,15.2,9.80089590599999));
#235435=CARTESIAN_POINT('Ctrl Pts',(-4.24886887800006,11.6,9.80089590599999));
#235436=CARTESIAN_POINT('Ctrl Pts',(-4.24850762500006,15.2,9.79857519499999));
#235437=CARTESIAN_POINT('Ctrl Pts',(-4.24850762500006,11.6,9.79857519499999));
#235438=CARTESIAN_POINT('Ctrl Pts',(-4.24814533900006,15.2,9.79626114099998));
#235439=CARTESIAN_POINT('Ctrl Pts',(-4.24814533900006,11.6,9.79626114099998));
#235440=CARTESIAN_POINT('Ctrl Pts',(-4.24778203100006,15.2,9.79395375599999));
#235441=CARTESIAN_POINT('Ctrl Pts',(-4.24778203100006,11.6,9.79395375599999));
#235442=CARTESIAN_POINT('Ctrl Pts',(-4.24741771300006,15.2,9.79165304999999));
#235443=CARTESIAN_POINT('Ctrl Pts',(-4.24741771300006,11.6,9.79165304999999));
#235444=CARTESIAN_POINT('Ctrl Pts',(-4.24705239800006,15.2,9.78935903399999));
#235445=CARTESIAN_POINT('Ctrl Pts',(-4.24705239800006,11.6,9.78935903399999));
#235446=CARTESIAN_POINT('Ctrl Pts',(-4.24668609600006,15.2,9.78707172099998));
#235447=CARTESIAN_POINT('Ctrl Pts',(-4.24668609600006,11.6,9.78707172099998));
#235448=CARTESIAN_POINT('Ctrl Pts',(-4.24631882000006,15.2,9.78479112099999));
#235449=CARTESIAN_POINT('Ctrl Pts',(-4.24631882000006,11.6,9.78479112099999));
#235450=CARTESIAN_POINT('Ctrl Pts',(-4.24595058300006,15.2,9.78251724599998));
#235451=CARTESIAN_POINT('Ctrl Pts',(-4.24595058300006,11.6,9.78251724599998));
#235452=CARTESIAN_POINT('Ctrl Pts',(-4.24558139600006,15.2,9.78025010599998));
#235453=CARTESIAN_POINT('Ctrl Pts',(-4.24558139600006,11.6,9.78025010599998));
#235454=CARTESIAN_POINT('Ctrl Pts',(-4.24521127100006,15.2,9.77798971399999));
#235455=CARTESIAN_POINT('Ctrl Pts',(-4.24521127100006,11.6,9.77798971399999));
#235456=CARTESIAN_POINT('Ctrl Pts',(-4.24484022100006,15.2,9.77573607999998));
#235457=CARTESIAN_POINT('Ctrl Pts',(-4.24484022100006,11.6,9.77573607999998));
#235458=CARTESIAN_POINT('Ctrl Pts',(-4.24446825700006,15.2,9.77348921599998));
#235459=CARTESIAN_POINT('Ctrl Pts',(-4.24446825700006,11.6,9.77348921599998));
#235460=CARTESIAN_POINT('Ctrl Pts',(-4.24409539300005,15.2,9.77124913399999));
#235461=CARTESIAN_POINT('Ctrl Pts',(-4.24409539300005,11.6,9.77124913399999));
#235462=CARTESIAN_POINT('Ctrl Pts',(-4.24372163900006,15.2,9.76901584499998));
#235463=CARTESIAN_POINT('Ctrl Pts',(-4.24372163900006,11.6,9.76901584499998));
#235464=CARTESIAN_POINT('Ctrl Pts',(-4.24334701000006,15.2,9.76678936199999));
#235465=CARTESIAN_POINT('Ctrl Pts',(-4.24334701000006,11.6,9.76678936199999));
#235466=CARTESIAN_POINT('Ctrl Pts',(-4.24297151500006,15.2,9.76456969299999));
#235467=CARTESIAN_POINT('Ctrl Pts',(-4.24297151500006,11.6,9.76456969299999));
#235468=CARTESIAN_POINT('Ctrl Pts',(-4.24259517000006,15.2,9.76235685299999));
#235469=CARTESIAN_POINT('Ctrl Pts',(-4.24259517000006,11.6,9.76235685299999));
#235470=CARTESIAN_POINT('Ctrl Pts',(-4.24221798600006,15.2,9.76015085199998));
#235471=CARTESIAN_POINT('Ctrl Pts',(-4.24221798600006,11.6,9.76015085199998));
#235472=CARTESIAN_POINT('Ctrl Pts',(-4.24183997500006,15.2,9.75795170199999));
#235473=CARTESIAN_POINT('Ctrl Pts',(-4.24183997500006,11.6,9.75795170199999));
#235474=CARTESIAN_POINT('Ctrl Pts',(-4.24146114900006,15.2,9.75575941499999));
#235475=CARTESIAN_POINT('Ctrl Pts',(-4.24146114900006,11.6,9.75575941499999));
#235476=CARTESIAN_POINT('Ctrl Pts',(-4.24108152400006,15.2,9.75357400099998));
#235477=CARTESIAN_POINT('Ctrl Pts',(-4.24108152400006,11.6,9.75357400099998));
#235478=CARTESIAN_POINT('Ctrl Pts',(-4.24070110900006,15.2,9.75139547399999));
#235479=CARTESIAN_POINT('Ctrl Pts',(-4.24070110900006,11.6,9.75139547399999));
#235480=CARTESIAN_POINT('Ctrl Pts',(-4.24031991700006,15.2,9.74922384499998));
#235481=CARTESIAN_POINT('Ctrl Pts',(-4.24031991700006,11.6,9.74922384499998));
#235482=CARTESIAN_POINT('Ctrl Pts',(-4.23993796200006,15.2,9.74705912499999));
#235483=CARTESIAN_POINT('Ctrl Pts',(-4.23993796200006,11.6,9.74705912499999));
#235484=CARTESIAN_POINT('Ctrl Pts',(-4.23955525800006,15.2,9.74490132499999));
#235485=CARTESIAN_POINT('Ctrl Pts',(-4.23955525800006,11.6,9.74490132499999));
#235486=CARTESIAN_POINT('Ctrl Pts',(-4.23917181600006,15.2,9.74275045999999));
#235487=CARTESIAN_POINT('Ctrl Pts',(-4.23917181600006,11.6,9.74275045999999));
#235488=CARTESIAN_POINT('Ctrl Pts',(-4.23878764900006,15.2,9.74060653899999));
#235489=CARTESIAN_POINT('Ctrl Pts',(-4.23878764900006,11.6,9.74060653899999));
#235490=CARTESIAN_POINT('Ctrl Pts',(-4.23840277000005,15.2,9.73846957399999));
#235491=CARTESIAN_POINT('Ctrl Pts',(-4.23840277000005,11.6,9.73846957399999));
#235492=CARTESIAN_POINT('Ctrl Pts',(-4.23801719200006,15.2,9.73633957899998));
#235493=CARTESIAN_POINT('Ctrl Pts',(-4.23801719200006,11.6,9.73633957899998));
#235494=CARTESIAN_POINT('Ctrl Pts',(-4.23763092900006,15.2,9.73421656399999));
#235495=CARTESIAN_POINT('Ctrl Pts',(-4.23763092900006,11.6,9.73421656399999));
#235496=CARTESIAN_POINT('Ctrl Pts',(-4.23724399200006,15.2,9.73210054199999));
#235497=CARTESIAN_POINT('Ctrl Pts',(-4.23724399200006,11.6,9.73210054199999));
#235498=CARTESIAN_POINT('Ctrl Pts',(-4.23685639800006,15.2,9.72999152399998));
#235499=CARTESIAN_POINT('Ctrl Pts',(-4.23685639800006,11.6,9.72999152399998));
#235500=CARTESIAN_POINT('Ctrl Pts',(-4.23646815600006,15.2,9.72788952199998));
#235501=CARTESIAN_POINT('Ctrl Pts',(-4.23646815600006,11.6,9.72788952199998));
#235502=CARTESIAN_POINT('Ctrl Pts',(-4.23607928100005,15.2,9.72579454999998));
#235503=CARTESIAN_POINT('Ctrl Pts',(-4.23607928100005,11.6,9.72579454999998));
#235504=CARTESIAN_POINT('Ctrl Pts',(-4.23568978700006,15.2,9.72370661699999));
#235505=CARTESIAN_POINT('Ctrl Pts',(-4.23568978700006,11.6,9.72370661699999));
#235506=CARTESIAN_POINT('Ctrl Pts',(-4.23529968600006,15.2,9.72162573799999));
#235507=CARTESIAN_POINT('Ctrl Pts',(-4.23529968600006,11.6,9.72162573799999));
#235508=CARTESIAN_POINT('Ctrl Pts',(-4.23490899300006,15.2,9.71955192299998));
#235509=CARTESIAN_POINT('Ctrl Pts',(-4.23490899300006,11.6,9.71955192299998));
#235510=CARTESIAN_POINT('Ctrl Pts',(-4.23451772000006,15.2,9.71748518599998));
#235511=CARTESIAN_POINT('Ctrl Pts',(-4.23451772000006,11.6,9.71748518599998));
#235512=CARTESIAN_POINT('Ctrl Pts',(-4.23412588100006,15.2,9.71542553699998));
#235513=CARTESIAN_POINT('Ctrl Pts',(-4.23412588100006,11.6,9.71542553699998));
#235514=CARTESIAN_POINT('Ctrl Pts',(-4.23373349000006,15.2,9.71337299099999));
#235515=CARTESIAN_POINT('Ctrl Pts',(-4.23373349000006,11.6,9.71337299099999));
#235516=CARTESIAN_POINT('Ctrl Pts',(-4.23334055900006,15.2,9.71132755799999));
#235517=CARTESIAN_POINT('Ctrl Pts',(-4.23334055900006,11.6,9.71132755799999));
#235518=CARTESIAN_POINT('Ctrl Pts',(-4.23294710300006,15.2,9.70928924999999));
#235519=CARTESIAN_POINT('Ctrl Pts',(-4.23294710300006,11.6,9.70928924999999));
#235520=CARTESIAN_POINT('Ctrl Pts',(-4.23255313500006,15.2,9.70725808199998));
#235521=CARTESIAN_POINT('Ctrl Pts',(-4.23255313500006,11.6,9.70725808199998));
#235522=CARTESIAN_POINT('Ctrl Pts',(-4.23215867100006,15.2,9.70523406399998));
#235523=CARTESIAN_POINT('Ctrl Pts',(-4.23215867100006,11.6,9.70523406399998));
#235524=CARTESIAN_POINT('Ctrl Pts',(-4.23176372200006,15.2,9.70321720899998));
#235525=CARTESIAN_POINT('Ctrl Pts',(-4.23176372200006,11.6,9.70321720899998));
#235526=CARTESIAN_POINT('Ctrl Pts',(-4.23136830300006,15.2,9.70120752899999));
#235527=CARTESIAN_POINT('Ctrl Pts',(-4.23136830300006,11.6,9.70120752899999));
#235528=CARTESIAN_POINT('Ctrl Pts',(-4.23097242800006,15.2,9.69920503799998));
#235529=CARTESIAN_POINT('Ctrl Pts',(-4.23097242800006,11.6,9.69920503799998));
#235530=CARTESIAN_POINT('Ctrl Pts',(-4.23057611000006,15.2,9.69720974699998));
#235531=CARTESIAN_POINT('Ctrl Pts',(-4.23057611000006,11.6,9.69720974699998));
#235532=CARTESIAN_POINT('Ctrl Pts',(-4.23017936500006,15.2,9.69522166899999));
#235533=CARTESIAN_POINT('Ctrl Pts',(-4.23017936500006,11.6,9.69522166899999));
#235534=CARTESIAN_POINT('Ctrl Pts',(-4.22978220600006,15.2,9.69324081599999));
#235535=CARTESIAN_POINT('Ctrl Pts',(-4.22978220600006,11.6,9.69324081599999));
#235536=CARTESIAN_POINT('Ctrl Pts',(-4.22938464600006,15.2,9.69126720099998));
#235537=CARTESIAN_POINT('Ctrl Pts',(-4.22938464600006,11.6,9.69126720099998));
#235538=CARTESIAN_POINT('Ctrl Pts',(-4.22898670100006,15.2,9.68930083699998));
#235539=CARTESIAN_POINT('Ctrl Pts',(-4.22898670100006,11.6,9.68930083699998));
#235540=CARTESIAN_POINT('Ctrl Pts',(-4.22858838400006,15.2,9.68734173599999));
#235541=CARTESIAN_POINT('Ctrl Pts',(-4.22858838400006,11.6,9.68734173599999));
#235542=CARTESIAN_POINT('Ctrl Pts',(-4.22818971000006,15.2,9.68538991099999));
#235543=CARTESIAN_POINT('Ctrl Pts',(-4.22818971000006,11.6,9.68538991099999));
#235544=CARTESIAN_POINT('Ctrl Pts',(-4.22779069300006,15.2,9.68344537499998));
#235545=CARTESIAN_POINT('Ctrl Pts',(-4.22779069300006,11.6,9.68344537499998));
#235546=CARTESIAN_POINT('Ctrl Pts',(-4.22739134800006,15.2,9.68150814099998));
#235547=CARTESIAN_POINT('Ctrl Pts',(-4.22739134800006,11.6,9.68150814099998));
#235548=CARTESIAN_POINT('Ctrl Pts',(-4.22699168900006,15.2,9.67957821999999));
#235549=CARTESIAN_POINT('Ctrl Pts',(-4.22699168900006,11.6,9.67957821999999));
#235550=CARTESIAN_POINT('Ctrl Pts',(-4.22659173000006,15.2,9.67765562699999));
#235551=CARTESIAN_POINT('Ctrl Pts',(-4.22659173000006,11.6,9.67765562699999));
#235552=CARTESIAN_POINT('Ctrl Pts',(-4.22619148700006,15.2,9.67574037199999));
#235553=CARTESIAN_POINT('Ctrl Pts',(-4.22619148700006,11.6,9.67574037199999));
#235554=CARTESIAN_POINT('Ctrl Pts',(-4.22579097300006,15.2,9.67383247099999));
#235555=CARTESIAN_POINT('Ctrl Pts',(-4.22579097300006,11.6,9.67383247099999));
#235556=CARTESIAN_POINT('Ctrl Pts',(-4.22539020400006,15.2,9.67193193599999));
#235557=CARTESIAN_POINT('Ctrl Pts',(-4.22539020400006,11.6,9.67193193599999));
#235558=CARTESIAN_POINT('Ctrl Pts',(-4.22498919400006,15.2,9.67003877999998));
#235559=CARTESIAN_POINT('Ctrl Pts',(-4.22498919400006,11.6,9.67003877999998));
#235560=CARTESIAN_POINT('Ctrl Pts',(-4.22458795900006,15.2,9.66815301399999));
#235561=CARTESIAN_POINT('Ctrl Pts',(-4.22458795900006,11.6,9.66815301399999));
#235562=CARTESIAN_POINT('Ctrl Pts',(-4.22418651100006,15.2,9.66627465399998));
#235563=CARTESIAN_POINT('Ctrl Pts',(-4.22418651100006,11.6,9.66627465399998));
#235564=CARTESIAN_POINT('Ctrl Pts',(-4.22378486900006,15.2,9.66440371099999));
#235565=CARTESIAN_POINT('Ctrl Pts',(-4.22378486900006,11.6,9.66440371099999));
#235566=CARTESIAN_POINT('Ctrl Pts',(-4.22338304400006,15.2,9.66254019799998));
#235567=CARTESIAN_POINT('Ctrl Pts',(-4.22338304400006,11.6,9.66254019799998));
#235568=CARTESIAN_POINT('Ctrl Pts',(-4.22298105500006,15.2,9.66068412999999));
#235569=CARTESIAN_POINT('Ctrl Pts',(-4.22298105500006,11.6,9.66068412999999));
#235570=CARTESIAN_POINT('Ctrl Pts',(-4.22257891300006,15.2,9.65883551899999));
#235571=CARTESIAN_POINT('Ctrl Pts',(-4.22257891300006,11.6,9.65883551899999));
#235572=CARTESIAN_POINT('Ctrl Pts',(-4.22217663700006,15.2,9.65699437699998));
#235573=CARTESIAN_POINT('Ctrl Pts',(-4.22217663700006,11.6,9.65699437699998));
#235574=CARTESIAN_POINT('Ctrl Pts',(-4.22177423900005,15.2,9.65516071999998));
#235575=CARTESIAN_POINT('Ctrl Pts',(-4.22177423900005,11.6,9.65516071999998));
#235576=CARTESIAN_POINT('Ctrl Pts',(-4.22137173800006,15.2,9.65333455899999));
#235577=CARTESIAN_POINT('Ctrl Pts',(-4.22137173800006,11.6,9.65333455899999));
#235578=CARTESIAN_POINT('Ctrl Pts',(-4.22096914500006,15.2,9.65151590699998));
#235579=CARTESIAN_POINT('Ctrl Pts',(-4.22096914500006,11.6,9.65151590699998));
#235580=CARTESIAN_POINT('Ctrl Pts',(-4.22056647800006,15.2,9.64970477999999));
#235581=CARTESIAN_POINT('Ctrl Pts',(-4.22056647800006,11.6,9.64970477999999));
#235582=CARTESIAN_POINT('Ctrl Pts',(-4.22016375200006,15.2,9.64790118999998));
#235583=CARTESIAN_POINT('Ctrl Pts',(-4.22016375200006,11.6,9.64790118999998));
#235584=CARTESIAN_POINT('Ctrl Pts',(-4.21976098500005,15.2,9.64610514899999));
#235585=CARTESIAN_POINT('Ctrl Pts',(-4.21976098500005,11.6,9.64610514899999));
#235586=CARTESIAN_POINT('Ctrl Pts',(-4.21935818800006,15.2,9.64431667199998));
#235587=CARTESIAN_POINT('Ctrl Pts',(-4.21935818800006,11.6,9.64431667199998));
#235588=CARTESIAN_POINT('Ctrl Pts',(-4.21895537900006,15.2,9.64253577199998));
#235589=CARTESIAN_POINT('Ctrl Pts',(-4.21895537900006,11.6,9.64253577199998));
#235590=CARTESIAN_POINT('Ctrl Pts',(-4.21855257300006,15.2,9.64076246299998));
#235591=CARTESIAN_POINT('Ctrl Pts',(-4.21855257300006,11.6,9.64076246299998));
#235592=CARTESIAN_POINT('Ctrl Pts',(-4.21814978800006,15.2,9.63899675899999));
#235593=CARTESIAN_POINT('Ctrl Pts',(-4.21814978800006,11.6,9.63899675899999));
#235594=CARTESIAN_POINT('Ctrl Pts',(-4.21774703800006,15.2,9.63723867199998));
#235595=CARTESIAN_POINT('Ctrl Pts',(-4.21774703800006,11.6,9.63723867199998));
#235596=CARTESIAN_POINT('Ctrl Pts',(-4.21734434000006,15.2,9.63548821799998));
#235597=CARTESIAN_POINT('Ctrl Pts',(-4.21734434000006,11.6,9.63548821799998));
#235598=CARTESIAN_POINT('Ctrl Pts',(-4.21694170800006,15.2,9.63374540799999));
#235599=CARTESIAN_POINT('Ctrl Pts',(-4.21694170800006,11.6,9.63374540799999));
#235600=CARTESIAN_POINT('Ctrl Pts',(-4.21653916000006,15.2,9.63201025699998));
#235601=CARTESIAN_POINT('Ctrl Pts',(-4.21653916000006,11.6,9.63201025699998));
#235602=CARTESIAN_POINT('Ctrl Pts',(-4.21613671100006,15.2,9.63028277899999));
#235603=CARTESIAN_POINT('Ctrl Pts',(-4.21613671100006,11.6,9.63028277899999));
#235604=CARTESIAN_POINT('Ctrl Pts',(-4.21573437800006,15.2,9.62856298799998));
#235605=CARTESIAN_POINT('Ctrl Pts',(-4.21573437800006,11.6,9.62856298799998));
#235606=CARTESIAN_POINT('Ctrl Pts',(-4.21533217800006,15.2,9.62685089699999));
#235607=CARTESIAN_POINT('Ctrl Pts',(-4.21533217800006,11.6,9.62685089699999));
#235608=CARTESIAN_POINT('Ctrl Pts',(-4.21493012500005,15.2,9.62514652099999));
#235609=CARTESIAN_POINT('Ctrl Pts',(-4.21493012500005,11.6,9.62514652099999));
#235610=CARTESIAN_POINT('Ctrl Pts',(-4.21452823700006,15.2,9.62344987199998));
#235611=CARTESIAN_POINT('Ctrl Pts',(-4.21452823700006,11.6,9.62344987199998));
#235612=CARTESIAN_POINT('Ctrl Pts',(-4.21412653100006,15.2,9.62176096799999));
#235613=CARTESIAN_POINT('Ctrl Pts',(-4.21412653100006,11.6,9.62176096799999));
#235614=CARTESIAN_POINT('Ctrl Pts',(-4.21372502200006,15.2,9.62007981799999));
#235615=CARTESIAN_POINT('Ctrl Pts',(-4.21372502200006,11.6,9.62007981799999));
#235616=CARTESIAN_POINT('Ctrl Pts',(-4.21332372900006,15.2,9.61840643899999));
#235617=CARTESIAN_POINT('Ctrl Pts',(-4.21332372900006,11.6,9.61840643899999));
#235618=CARTESIAN_POINT('Ctrl Pts',(-4.21292266500005,15.2,9.61674084599998));
#235619=CARTESIAN_POINT('Ctrl Pts',(-4.21292266500005,11.6,9.61674084599998));
#235620=CARTESIAN_POINT('Ctrl Pts',(-4.21252185100006,15.2,9.61508304999998));
#235621=CARTESIAN_POINT('Ctrl Pts',(-4.21252185100006,11.6,9.61508304999998));
#235622=CARTESIAN_POINT('Ctrl Pts',(-4.21212130000006,15.2,9.61343306699998));
#235623=CARTESIAN_POINT('Ctrl Pts',(-4.21212130000006,11.6,9.61343306699998));
#235624=CARTESIAN_POINT('Ctrl Pts',(-4.21172103100006,15.2,9.61179091199998));
#235625=CARTESIAN_POINT('Ctrl Pts',(-4.21172103100006,11.6,9.61179091199998));
#235626=CARTESIAN_POINT('Ctrl Pts',(-4.21132106100006,15.2,9.61015659799998));
#235627=CARTESIAN_POINT('Ctrl Pts',(-4.21132106100006,11.6,9.61015659799998));
#235628=CARTESIAN_POINT('Ctrl Pts',(-4.21092140700006,15.2,9.60853013999999));
#235629=CARTESIAN_POINT('Ctrl Pts',(-4.21092140700006,11.6,9.60853013999999));
#235630=CARTESIAN_POINT('Ctrl Pts',(-4.21052208400006,15.2,9.60691155199999));
#235631=CARTESIAN_POINT('Ctrl Pts',(-4.21052208400006,11.6,9.60691155199999));
#235632=CARTESIAN_POINT('Ctrl Pts',(-4.21012311300006,15.2,9.60530084899998));
#235633=CARTESIAN_POINT('Ctrl Pts',(-4.21012311300006,11.6,9.60530084899998));
#235634=CARTESIAN_POINT('Ctrl Pts',(-4.20972450800006,15.2,9.60369804499998));
#235635=CARTESIAN_POINT('Ctrl Pts',(-4.20972450800006,11.6,9.60369804499998));
#235636=CARTESIAN_POINT('Ctrl Pts',(-4.20932628800006,15.2,9.60210315399999));
#235637=CARTESIAN_POINT('Ctrl Pts',(-4.20932628800006,11.6,9.60210315399999));
#235638=CARTESIAN_POINT('Ctrl Pts',(-4.20892847000006,15.2,9.60051619099998));
#235639=CARTESIAN_POINT('Ctrl Pts',(-4.20892847000006,11.6,9.60051619099998));
#235640=CARTESIAN_POINT('Ctrl Pts',(-4.20853107200006,15.2,9.59893717199999));
#235641=CARTESIAN_POINT('Ctrl Pts',(-4.20853107200006,11.6,9.59893717199999));
#235642=CARTESIAN_POINT('Ctrl Pts',(-4.20813411000006,15.2,9.59736610999999));
#235643=CARTESIAN_POINT('Ctrl Pts',(-4.20813411000006,11.6,9.59736610999999));
#235644=CARTESIAN_POINT('Ctrl Pts',(-4.20773760400006,15.2,9.59580301999999));
#235645=CARTESIAN_POINT('Ctrl Pts',(-4.20773760400006,11.6,9.59580301999999));
#235646=CARTESIAN_POINT('Ctrl Pts',(-4.20734156900005,15.2,9.59424791599999));
#235647=CARTESIAN_POINT('Ctrl Pts',(-4.20734156900005,11.6,9.59424791599999));
#235648=CARTESIAN_POINT('Ctrl Pts',(-4.20694602600006,15.2,9.59270081399998));
#235649=CARTESIAN_POINT('Ctrl Pts',(-4.20694602600006,11.6,9.59270081399998));
#235650=CARTESIAN_POINT('Ctrl Pts',(-4.20655098900006,15.2,9.59116172999998));
#235651=CARTESIAN_POINT('Ctrl Pts',(-4.20655098900006,11.6,9.59116172999998));
#235652=CARTESIAN_POINT('Ctrl Pts',(-4.20615648000005,15.2,9.58963067599999));
#235653=CARTESIAN_POINT('Ctrl Pts',(-4.20615648000005,11.6,9.58963067599999));
#235654=CARTESIAN_POINT('Ctrl Pts',(-4.20576251400006,15.2,9.58810766899998));
#235655=CARTESIAN_POINT('Ctrl Pts',(-4.20576251400006,11.6,9.58810766899998));
#235656=CARTESIAN_POINT('Ctrl Pts',(-4.20536911100006,15.2,9.58659272299998));
#235657=CARTESIAN_POINT('Ctrl Pts',(-4.20536911100006,11.6,9.58659272299998));
#235658=CARTESIAN_POINT('Ctrl Pts',(-4.20497628800006,15.2,9.58508585299998));
#235659=CARTESIAN_POINT('Ctrl Pts',(-4.20497628800006,11.6,9.58508585299998));
#235660=CARTESIAN_POINT('Ctrl Pts',(-4.20458406400006,15.2,9.58358707499999));
#235661=CARTESIAN_POINT('Ctrl Pts',(-4.20458406400006,11.6,9.58358707499999));
#235662=CARTESIAN_POINT('Ctrl Pts',(-4.20419245700006,15.2,9.58209640399998));
#235663=CARTESIAN_POINT('Ctrl Pts',(-4.20419245700006,11.6,9.58209640399998));
#235664=CARTESIAN_POINT('Ctrl Pts',(-4.20380148500006,15.2,9.58061385399999));
#235665=CARTESIAN_POINT('Ctrl Pts',(-4.20380148500006,11.6,9.58061385399999));
#235666=CARTESIAN_POINT('Ctrl Pts',(-4.20341116800006,15.2,9.57913944099998));
#235667=CARTESIAN_POINT('Ctrl Pts',(-4.20341116800006,11.6,9.57913944099998));
#235668=CARTESIAN_POINT('Ctrl Pts',(-4.20302152300006,15.2,9.57767318099998));
#235669=CARTESIAN_POINT('Ctrl Pts',(-4.20302152300006,11.6,9.57767318099998));
#235670=CARTESIAN_POINT('Ctrl Pts',(-4.20263256900006,15.2,9.57621508899998));
#235671=CARTESIAN_POINT('Ctrl Pts',(-4.20263256900006,11.6,9.57621508899998));
#235672=CARTESIAN_POINT('Ctrl Pts',(-4.20224432600006,15.2,9.57476517899998));
#235673=CARTESIAN_POINT('Ctrl Pts',(-4.20224432600006,11.6,9.57476517899998));
#235674=CARTESIAN_POINT('Ctrl Pts',(-4.20185681200006,15.2,9.57332346799999));
#235675=CARTESIAN_POINT('Ctrl Pts',(-4.20185681200006,11.6,9.57332346799999));
#235676=CARTESIAN_POINT('Ctrl Pts',(-4.20147004500006,15.2,9.57188997099998));
#235677=CARTESIAN_POINT('Ctrl Pts',(-4.20147004500006,11.6,9.57188997099998));
#235678=CARTESIAN_POINT('Ctrl Pts',(-4.20108404600006,15.2,9.57046470299998));
#235679=CARTESIAN_POINT('Ctrl Pts',(-4.20108404600006,11.6,9.57046470299998));
#235680=CARTESIAN_POINT('Ctrl Pts',(-4.20069883300005,15.2,9.56904768099999));
#235681=CARTESIAN_POINT('Ctrl Pts',(-4.20069883300005,11.6,9.56904768099999));
#235682=CARTESIAN_POINT('Ctrl Pts',(-4.20031442400005,15.2,9.56763891999999));
#235683=CARTESIAN_POINT('Ctrl Pts',(-4.20031442400005,11.6,9.56763891999999));
#235684=CARTESIAN_POINT('Ctrl Pts',(-4.19993084100006,15.2,9.56623843399999));
#235685=CARTESIAN_POINT('Ctrl Pts',(-4.19993084100006,11.6,9.56623843399999));
#235686=CARTESIAN_POINT('Ctrl Pts',(-4.19954810100006,15.2,9.56484624099998));
#235687=CARTESIAN_POINT('Ctrl Pts',(-4.19954810100006,11.6,9.56484624099998));
#235688=CARTESIAN_POINT('Ctrl Pts',(-4.19916622500006,15.2,9.56346235699998));
#235689=CARTESIAN_POINT('Ctrl Pts',(-4.19916622500006,11.6,9.56346235699998));
#235690=CARTESIAN_POINT('Ctrl Pts',(-4.19878523200006,15.2,9.56208679599998));
#235691=CARTESIAN_POINT('Ctrl Pts',(-4.19878523200006,11.6,9.56208679599998));
#235692=CARTESIAN_POINT('Ctrl Pts',(-4.19840514200006,15.2,9.56071957599999));
#235693=CARTESIAN_POINT('Ctrl Pts',(-4.19840514200006,11.6,9.56071957599999));
#235694=CARTESIAN_POINT('Ctrl Pts',(-4.19802597400006,15.2,9.55936071099998));
#235695=CARTESIAN_POINT('Ctrl Pts',(-4.19802597400006,11.6,9.55936071099998));
#235696=CARTESIAN_POINT('Ctrl Pts',(-4.19764774800006,15.2,9.55801021899998));
#235697=CARTESIAN_POINT('Ctrl Pts',(-4.19764774800006,11.6,9.55801021899998));
#235698=CARTESIAN_POINT('Ctrl Pts',(-4.19727048400006,15.2,9.55666811399999));
#235699=CARTESIAN_POINT('Ctrl Pts',(-4.19727048400006,11.6,9.55666811399999));
#235700=CARTESIAN_POINT('Ctrl Pts',(-4.19689420300006,15.2,9.55533441399999));
#235701=CARTESIAN_POINT('Ctrl Pts',(-4.19689420300006,11.6,9.55533441399999));
#235702=CARTESIAN_POINT('Ctrl Pts',(-4.19651892300006,15.2,9.55400913399998));
#235703=CARTESIAN_POINT('Ctrl Pts',(-4.19651892300006,11.6,9.55400913399998));
#235704=CARTESIAN_POINT('Ctrl Pts',(-4.19614466600006,15.2,9.55269229099999));
#235705=CARTESIAN_POINT('Ctrl Pts',(-4.19614466600006,11.6,9.55269229099999));
#235706=CARTESIAN_POINT('Ctrl Pts',(-4.19577145300006,15.2,9.55138390099999));
#235707=CARTESIAN_POINT('Ctrl Pts',(-4.19577145300006,11.6,9.55138390099999));
#235708=CARTESIAN_POINT('Ctrl Pts',(-4.19539930100005,15.2,9.55008397999999));
#235709=CARTESIAN_POINT('Ctrl Pts',(-4.19539930100005,11.6,9.55008397999999));
#235710=CARTESIAN_POINT('Ctrl Pts',(-4.19502823500006,15.2,9.54879254499998));
#235711=CARTESIAN_POINT('Ctrl Pts',(-4.19502823500006,11.6,9.54879254499998));
#235712=CARTESIAN_POINT('Ctrl Pts',(-4.19465827200006,15.2,9.54750961399998));
#235713=CARTESIAN_POINT('Ctrl Pts',(-4.19465827200006,11.6,9.54750961399998));
#235714=CARTESIAN_POINT('Ctrl Pts',(-4.19428943400006,15.2,9.54623519999998));
#235715=CARTESIAN_POINT('Ctrl Pts',(-4.19428943400006,11.6,9.54623519999998));
#235716=CARTESIAN_POINT('Ctrl Pts',(-4.19392174100006,15.2,9.54496932299998));
#235717=CARTESIAN_POINT('Ctrl Pts',(-4.19392174100006,11.6,9.54496932299998));
#235718=CARTESIAN_POINT('Ctrl Pts',(-4.19355521500006,15.2,9.54371199799999));
#235719=CARTESIAN_POINT('Ctrl Pts',(-4.19355521500006,11.6,9.54371199799999));
#235720=CARTESIAN_POINT('Ctrl Pts',(-4.19318987800006,15.2,9.54246324299999));
#235721=CARTESIAN_POINT('Ctrl Pts',(-4.19318987800006,11.6,9.54246324299999));
#235722=CARTESIAN_POINT('Ctrl Pts',(-4.19282574800006,15.2,9.54122307299999));
#235723=CARTESIAN_POINT('Ctrl Pts',(-4.19282574800006,11.6,9.54122307299999));
#235724=CARTESIAN_POINT('Ctrl Pts',(-4.19246284900006,15.2,9.53999150599999));
#235725=CARTESIAN_POINT('Ctrl Pts',(-4.19246284900006,11.6,9.53999150599999));
#235726=CARTESIAN_POINT('Ctrl Pts',(-4.19210120000006,15.2,9.53876855899999));
#235727=CARTESIAN_POINT('Ctrl Pts',(-4.19210120000006,11.6,9.53876855899999));
#235728=CARTESIAN_POINT('Ctrl Pts',(-4.19174082500006,15.2,9.53755424899999));
#235729=CARTESIAN_POINT('Ctrl Pts',(-4.19174082500006,11.6,9.53755424899999));
#235730=CARTESIAN_POINT('Ctrl Pts',(-4.19138174300006,15.2,9.53634859299999));
#235731=CARTESIAN_POINT('Ctrl Pts',(-4.19138174300006,11.6,9.53634859299999));
#235732=CARTESIAN_POINT('Ctrl Pts',(-4.19102397700006,15.2,9.53515160799999));
#235733=CARTESIAN_POINT('Ctrl Pts',(-4.19102397700006,11.6,9.53515160799999));
#235734=CARTESIAN_POINT('Ctrl Pts',(-4.19066754800006,15.2,9.53396331099999));
#235735=CARTESIAN_POINT('Ctrl Pts',(-4.19066754800006,11.6,9.53396331099999));
#235736=CARTESIAN_POINT('Ctrl Pts',(-4.19031247800006,15.2,9.53278371999998));
#235737=CARTESIAN_POINT('Ctrl Pts',(-4.19031247800006,11.6,9.53278371999998));
#235738=CARTESIAN_POINT('Ctrl Pts',(-4.18995878900006,15.2,9.53161285199998));
#235739=CARTESIAN_POINT('Ctrl Pts',(-4.18995878900006,11.6,9.53161285199998));
#235740=CARTESIAN_POINT('Ctrl Pts',(-4.18960650400006,15.2,9.53045072299999));
#235741=CARTESIAN_POINT('Ctrl Pts',(-4.18960650400006,11.6,9.53045072299999));
#235742=CARTESIAN_POINT('Ctrl Pts',(-4.18925564400006,15.2,9.52929735399999));
#235743=CARTESIAN_POINT('Ctrl Pts',(-4.18925564400006,11.6,9.52929735399999));
#235744=CARTESIAN_POINT('Ctrl Pts',(-4.18890623100006,15.2,9.52815275899999));
#235745=CARTESIAN_POINT('Ctrl Pts',(-4.18890623100006,11.6,9.52815275899999));
#235746=CARTESIAN_POINT('Ctrl Pts',(-4.18855828800006,15.2,9.52701695699999));
#235747=CARTESIAN_POINT('Ctrl Pts',(-4.18855828800006,11.6,9.52701695699999));
#235748=CARTESIAN_POINT('Ctrl Pts',(-4.18821183700006,15.2,9.52588996599999));
#235749=CARTESIAN_POINT('Ctrl Pts',(-4.18821183700006,11.6,9.52588996599999));
#235750=CARTESIAN_POINT('Ctrl Pts',(-4.18786690100006,15.2,9.52477180399999));
#235751=CARTESIAN_POINT('Ctrl Pts',(-4.18786690100006,11.6,9.52477180399999));
#235752=CARTESIAN_POINT('Ctrl Pts',(-4.18752350300006,15.2,9.52366248799999));
#235753=CARTESIAN_POINT('Ctrl Pts',(-4.18752350300006,11.6,9.52366248799999));
#235754=CARTESIAN_POINT('Ctrl Pts',(-4.18718166500006,15.2,9.52256203599998));
#235755=CARTESIAN_POINT('Ctrl Pts',(-4.18718166500006,11.6,9.52256203599998));
#235756=CARTESIAN_POINT('Ctrl Pts',(-4.18684141000006,15.2,9.52147046599999));
#235757=CARTESIAN_POINT('Ctrl Pts',(-4.18684141000006,11.6,9.52147046599999));
#235758=CARTESIAN_POINT('Ctrl Pts',(-4.18650276200006,15.2,9.52038779699999));
#235759=CARTESIAN_POINT('Ctrl Pts',(-4.18650276200006,11.6,9.52038779699999));
#235760=CARTESIAN_POINT('Ctrl Pts',(-4.18616574200006,15.2,9.51931404499998));
#235761=CARTESIAN_POINT('Ctrl Pts',(-4.18616574200006,11.6,9.51931404499998));
#235762=CARTESIAN_POINT('Ctrl Pts',(-4.18583037600006,15.2,9.51824923099998));
#235763=CARTESIAN_POINT('Ctrl Pts',(-4.18583037600006,11.6,9.51824923099998));
#235764=CARTESIAN_POINT('Ctrl Pts',(-4.18549668600006,15.2,9.51719337099998));
#235765=CARTESIAN_POINT('Ctrl Pts',(-4.18549668600006,11.6,9.51719337099998));
#235766=CARTESIAN_POINT('Ctrl Pts',(-4.18516469500006,15.2,9.51614648399998));
#235767=CARTESIAN_POINT('Ctrl Pts',(-4.18516469500006,11.6,9.51614648399998));
#235768=CARTESIAN_POINT('Ctrl Pts',(-4.18483442700006,15.2,9.51510858999999));
#235769=CARTESIAN_POINT('Ctrl Pts',(-4.18483442700006,11.6,9.51510858999999));
#235770=CARTESIAN_POINT('Ctrl Pts',(-4.18450590700005,15.2,9.51407970499999));
#235771=CARTESIAN_POINT('Ctrl Pts',(-4.18450590700005,11.6,9.51407970499999));
#235772=CARTESIAN_POINT('Ctrl Pts',(-4.18417915700006,15.2,9.51305984799999));
#235773=CARTESIAN_POINT('Ctrl Pts',(-4.18417915700006,11.6,9.51305984799999));
#235774=CARTESIAN_POINT('Ctrl Pts',(-4.18385420200006,15.2,9.51204903999999));
#235775=CARTESIAN_POINT('Ctrl Pts',(-4.18385420200006,11.6,9.51204903999999));
#235776=CARTESIAN_POINT('Ctrl Pts',(-4.18353106500006,15.2,9.51104729699999));
#235777=CARTESIAN_POINT('Ctrl Pts',(-4.18353106500006,11.6,9.51104729699999));
#235778=CARTESIAN_POINT('Ctrl Pts',(-4.18320977200006,15.2,9.51005463899998));
#235779=CARTESIAN_POINT('Ctrl Pts',(-4.18320977200006,11.6,9.51005463899998));
#235780=CARTESIAN_POINT('Ctrl Pts',(-4.18289034700006,15.2,9.50907108499998));
#235781=CARTESIAN_POINT('Ctrl Pts',(-4.18289034700006,11.6,9.50907108499998));
#235782=CARTESIAN_POINT('Ctrl Pts',(-4.18257281300006,15.2,9.50809665399999));
#235783=CARTESIAN_POINT('Ctrl Pts',(-4.18257281300006,11.6,9.50809665399999));
#235784=CARTESIAN_POINT('Ctrl Pts',(-4.18225719600006,15.2,9.50713136399998));
#235785=CARTESIAN_POINT('Ctrl Pts',(-4.18225719600006,11.6,9.50713136399998));
#235786=CARTESIAN_POINT('Ctrl Pts',(-4.18194352100006,15.2,9.50617523599998));
#235787=CARTESIAN_POINT('Ctrl Pts',(-4.18194352100006,11.6,9.50617523599998));
#235788=CARTESIAN_POINT('Ctrl Pts',(-4.18163181000006,15.2,9.50522828699999));
#235789=CARTESIAN_POINT('Ctrl Pts',(-4.18163181000006,11.6,9.50522828699999));
#235790=CARTESIAN_POINT('Ctrl Pts',(-4.18132209200006,15.2,9.50429053799999));
#235791=CARTESIAN_POINT('Ctrl Pts',(-4.18132209200006,11.6,9.50429053799999));
#235792=CARTESIAN_POINT('Ctrl Pts',(-4.18101438900006,15.2,9.50336200799999));
#235793=CARTESIAN_POINT('Ctrl Pts',(-4.18101438900006,11.6,9.50336200799999));
#235794=CARTESIAN_POINT('Ctrl Pts',(-4.18070872900006,15.2,9.50244271599999));
#235795=CARTESIAN_POINT('Ctrl Pts',(-4.18070872900006,11.6,9.50244271599999));
#235796=CARTESIAN_POINT('Ctrl Pts',(-4.18040513600006,15.2,9.50153268199998));
#235797=CARTESIAN_POINT('Ctrl Pts',(-4.18040513600006,11.6,9.50153268199998));
#235798=CARTESIAN_POINT('Ctrl Pts',(-4.18010363500006,15.2,9.50063192499999));
#235799=CARTESIAN_POINT('Ctrl Pts',(-4.18010363500006,11.6,9.50063192499999));
#235800=CARTESIAN_POINT('Ctrl Pts',(-4.17980425200006,15.2,9.49974046699998));
#235801=CARTESIAN_POINT('Ctrl Pts',(-4.17980425200006,11.6,9.49974046699998));
#235802=CARTESIAN_POINT('Ctrl Pts',(-4.17950701400006,15.2,9.49885832499999));
#235803=CARTESIAN_POINT('Ctrl Pts',(-4.17950701400006,11.6,9.49885832499999));
#235804=CARTESIAN_POINT('Ctrl Pts',(-4.17921364400006,15.2,9.49799054599998));
#235805=CARTESIAN_POINT('Ctrl Pts',(-4.17921364400006,11.6,9.49799054599998));
#235806=CARTESIAN_POINT('Ctrl Pts',(-4.17898102000006,15.2,9.49730470699999));
#235807=CARTESIAN_POINT('Ctrl Pts',(-4.17898102000006,11.6,9.49730470699999));
#235808=CARTESIAN_POINT('Ctrl Pts',(-4.17880795500006,15.2,9.49679570899999));
#235809=CARTESIAN_POINT('Ctrl Pts',(-4.17880795500006,11.6,9.49679570899999));
#235810=CARTESIAN_POINT('Ctrl Pts',(-4.17869357200006,15.2,9.49645984699998));
#235811=CARTESIAN_POINT('Ctrl Pts',(-4.17869357200006,11.6,9.49645984699998));
#235812=CARTESIAN_POINT('Ctrl Pts',(-4.17863732200006,15.2,9.49629481199998));
#235813=CARTESIAN_POINT('Ctrl Pts',(-4.17863732200006,11.6,9.49629481199998));
#235814=CARTESIAN_POINT('',(-4.17863732200006,12.2,9.49629481099999));
#235815=CARTESIAN_POINT('',(-4.17863732200006,15.2,9.49629481099999));
#235816=CARTESIAN_POINT('',(-4.17863732200006,12.2,9.49629481099999));
#235817=CARTESIAN_POINT('Ctrl Pts',(-4.27433547000006,12.2,10.676144262));
#235818=CARTESIAN_POINT('Ctrl Pts',(-4.2747065234345,12.2,10.671060553948));
#235819=CARTESIAN_POINT('Ctrl Pts',(-4.2750690771701,12.2,10.6659880182638));
#235820=CARTESIAN_POINT('Ctrl Pts',(-4.27542311679964,12.2,10.6609266596558));
#235821=CARTESIAN_POINT('Ctrl Pts',(-4.27568864649767,12.2,10.6571306410445));
#235822=CARTESIAN_POINT('Ctrl Pts',(-4.2759493913633,12.2,10.6533409101855));
#235823=CARTESIAN_POINT('Ctrl Pts',(-4.2762053652829,12.2,10.649557489718));
#235824=CARTESIAN_POINT('Ctrl Pts',(-4.27646133920251,12.2,10.6457740692505));
#235825=CARTESIAN_POINT('Ctrl Pts',(-4.27671254300291,12.2,10.6419969605181));
#235826=CARTESIAN_POINT('Ctrl Pts',(-4.27695900353521,12.2,10.638226201864));
#235827=CARTESIAN_POINT('Ctrl Pts',(-4.27736977110396,12.2,10.6319416038789));
#235828=CARTESIAN_POINT('Ctrl Pts',(-4.2777673688425,12.2,10.6256746519071));
#235829=CARTESIAN_POINT('Ctrl Pts',(-4.27815191030016,12.2,10.6194255110747));
#235830=CARTESIAN_POINT('Ctrl Pts',(-4.27838263516637,12.2,10.6156760267115));
#235831=CARTESIAN_POINT('Ctrl Pts',(-4.27860865834068,12.2,10.6119329518277));
#235832=CARTESIAN_POINT('Ctrl Pts',(-4.27883000120862,12.2,10.6081963174882));
#235833=CARTESIAN_POINT('Ctrl Pts',(-4.27905134407656,12.2,10.6044596831487));
#235834=CARTESIAN_POINT('Ctrl Pts',(-4.27926800538995,12.2,10.600729488635));
#235835=CARTESIAN_POINT('Ctrl Pts',(-4.27948001121656,12.2,10.597005769795));
#235836=CARTESIAN_POINT('Ctrl Pts',(-4.27969201704318,12.2,10.593282050955));
#235837=CARTESIAN_POINT('Ctrl Pts',(-4.27989936530154,12.2,10.5895648059536));
#235838=CARTESIAN_POINT('Ctrl Pts',(-4.28010208221125,12.2,10.5858540711712));
#235839=CARTESIAN_POINT('Ctrl Pts',(-4.28030479912095,12.2,10.5821433363888));
#235840=CARTESIAN_POINT('Ctrl Pts',(-4.28050288434764,12.2,10.5784391108726));
#235841=CARTESIAN_POINT('Ctrl Pts',(-4.28069636217457,12.2,10.5747414290894));
#235842=CARTESIAN_POINT('Ctrl Pts',(-4.28088984003665,12.2,10.5710437466344));
#235843=CARTESIAN_POINT('Ctrl Pts',(-4.2810787083641,12.2,10.567352606848));
#235844=CARTESIAN_POINT('Ctrl Pts',(-4.28126299326526,12.2,10.5636680444384));
#235845=CARTESIAN_POINT('Ctrl Pts',(-4.281508706411,12.2,10.5587552956745));
#235846=CARTESIAN_POINT('Ctrl Pts',(-4.28174626834262,12.2,10.5538542388258));
#235847=CARTESIAN_POINT('Ctrl Pts',(-4.2819757394916,12.2,10.5489649535366));
#235848=CARTESIAN_POINT('Ctrl Pts',(-4.28214784286115,12.2,10.5452979894032));
#235849=CARTESIAN_POINT('Ctrl Pts',(-4.28231539458777,12.2,10.5416376492828));
#235850=CARTESIAN_POINT('Ctrl Pts',(-4.28247841904058,12.2,10.537983964665));
#235851=CARTESIAN_POINT('Ctrl Pts',(-4.28264144349338,12.2,10.5343302800471));
#235852=CARTESIAN_POINT('Ctrl Pts',(-4.28279994102149,12.2,10.5306832527622));
#235853=CARTESIAN_POINT('Ctrl Pts',(-4.28295393647485,12.2,10.5270429160185));
#235854=CARTESIAN_POINT('Ctrl Pts',(-4.28310793195617,12.2,10.5234025786136));
#235855=CARTESIAN_POINT('Ctrl Pts',(-4.28325742481123,12.2,10.5197689313521));
#235856=CARTESIAN_POINT('Ctrl Pts',(-4.28340244079003,12.2,10.5161420099926));
#235857=CARTESIAN_POINT('Ctrl Pts',(-4.28354745674248,12.2,10.512515089292));
#235858=CARTESIAN_POINT('Ctrl Pts',(-4.28368799532503,12.2,10.5088948948327));
#235859=CARTESIAN_POINT('Ctrl Pts',(-4.28382408224304,12.2,10.5052814590342));
#235860=CARTESIAN_POINT('Ctrl Pts',(-4.28396016916104,12.2,10.5016680232358));
#235861=CARTESIAN_POINT('Ctrl Pts',(-4.28409180340222,12.2,10.4980613483429));
#235862=CARTESIAN_POINT('Ctrl Pts',(-4.28421901227221,12.2,10.4944614680993));
#235863=CARTESIAN_POINT('Ctrl Pts',(-4.2843462211422,12.2,10.4908615878557));
#235864=CARTESIAN_POINT('Ctrl Pts',(-4.28446900302106,12.2,10.4872685014029));
#235865=CARTESIAN_POINT('Ctrl Pts',(-4.28458738451676,12.2,10.4836822446999));
#235866=CARTESIAN_POINT('Ctrl Pts',(-4.28470576601246,12.2,10.4800959879969));
#235867=CARTESIAN_POINT('Ctrl Pts',(-4.28481974750833,12.2,10.4765165618769));
#235868=CARTESIAN_POINT('Ctrl Pts',(-4.28492935396307,12.2,10.4729439991728));
#235869=CARTESIAN_POINT('Ctrl Pts',(-4.2850389604178,12.2,10.4693714364686));
#235870=CARTESIAN_POINT('Ctrl Pts',(-4.2851441913145,12.2,10.4658057377307));
#235871=CARTESIAN_POINT('Ctrl Pts',(-4.28524507422809,12.2,10.4622469389841));
#235872=CARTESIAN_POINT('Ctrl Pts',(-4.28534595716001,12.2,10.458688139591));
#235873=CARTESIAN_POINT('Ctrl Pts',(-4.28544249107404,12.2,10.4551362394581));
#235874=CARTESIAN_POINT('Ctrl Pts',(-4.28553470354518,12.2,10.4515912749855));
#235875=CARTESIAN_POINT('Ctrl Pts',(-4.28562691599958,12.2,10.4480463111568));
#235876=CARTESIAN_POINT('Ctrl Pts',(-4.28571480596557,12.2,10.4445082806642));
#235877=CARTESIAN_POINT('Ctrl Pts',(-4.28579840046622,12.2,10.4409772202835));
#235878=CARTESIAN_POINT('Ctrl Pts',(-4.28588199496686,12.2,10.4374461599028));
#235879=CARTESIAN_POINT('Ctrl Pts',(-4.28596129374462,12.2,10.4339220701717));
#235880=CARTESIAN_POINT('Ctrl Pts',(-4.28603632374153,12.2,10.4304049863417));
#235881=CARTESIAN_POINT('Ctrl Pts',(-4.28611135373843,12.2,10.4268879025117));
#235882=CARTESIAN_POINT('Ctrl Pts',(-4.28618211578584,12.2,10.4233778225227));
#235883=CARTESIAN_POINT('Ctrl Pts',(-4.28624863578342,12.2,10.4198747847333));
#235884=CARTESIAN_POINT('Ctrl Pts',(-4.28631515578101,12.2,10.4163717469438));
#235885=CARTESIAN_POINT('Ctrl Pts',(-4.28637743427876,12.2,10.4128757504375));
#235886=CARTESIAN_POINT('Ctrl Pts',(-4.28643549827702,12.2,10.409386830647));
#235887=CARTESIAN_POINT('Ctrl Pts',(-4.28649356227528,12.2,10.4058979108565));
#235888=CARTESIAN_POINT('Ctrl Pts',(-4.28654741120594,12.2,10.4024160668704));
#235889=CARTESIAN_POINT('Ctrl Pts',(-4.28659707424877,12.2,10.3989413359473));
#235890=CARTESIAN_POINT('Ctrl Pts',(-4.28664673729159,12.2,10.3954666050241));
#235891=CARTESIAN_POINT('Ctrl Pts',(-4.28669221410867,12.2,10.3919989867295));
#235892=CARTESIAN_POINT('Ctrl Pts',(-4.28673353119108,12.2,10.388538517021));
#235893=CARTESIAN_POINT('Ctrl Pts',(-4.28677484828098,12.2,10.3850780466838));
#235894=CARTESIAN_POINT('Ctrl Pts',(-4.28681200728638,12.2,10.3816247245819));
#235895=CARTESIAN_POINT('Ctrl Pts',(-4.28684503529062,12.2,10.3781785877487));
#235896=CARTESIAN_POINT('Ctrl Pts',(-4.2868890726196,12.2,10.3735837396812));
#235897=CARTESIAN_POINT('Ctrl Pts',(-4.2869257653162,12.2,10.3690016644425));
#235898=CARTESIAN_POINT('Ctrl Pts',(-4.28695518198094,12.2,10.3644324476486));
#235899=CARTESIAN_POINT('Ctrl Pts',(-4.2869772444805,12.2,10.3610055348975));
#235900=CARTESIAN_POINT('Ctrl Pts',(-4.28699521373003,12.2,10.3575858545576));
#235901=CARTESIAN_POINT('Ctrl Pts',(-4.28700911873069,12.2,10.3541734441769));
#235902=CARTESIAN_POINT('Ctrl Pts',(-4.28702302373135,12.2,10.3507610337962));
#235903=CARTESIAN_POINT('Ctrl Pts',(-4.28703286426514,12.2,10.3473558933516));
#235904=CARTESIAN_POINT('Ctrl Pts',(-4.28703866926548,12.2,10.3439580582657));
#235905=CARTESIAN_POINT('Ctrl Pts',(-4.28704447426688,12.2,10.3405602225625));
#235906=CARTESIAN_POINT('Ctrl Pts',(-4.2870462437338,12.2,10.3371696939698));
#235907=CARTESIAN_POINT('Ctrl Pts',(-4.28704400681626,12.2,10.3337865072291));
#235908=CARTESIAN_POINT('Ctrl Pts',(-4.28704176989913,12.2,10.330403321103));
#235909=CARTESIAN_POINT('Ctrl Pts',(-4.28703552706555,12.2,10.3270274781099));
#235910=CARTESIAN_POINT('Ctrl Pts',(-4.28702530623224,12.2,10.3236590143996));
#235911=CARTESIAN_POINT('Ctrl Pts',(-4.28701508539893,12.2,10.3202905506893));
#235912=CARTESIAN_POINT('Ctrl Pts',(-4.28700088849951,12.2,10.31692946624));
#235913=CARTESIAN_POINT('Ctrl Pts',(-4.28698274400007,12.2,10.3135757990134));
#235914=CARTESIAN_POINT('Ctrl Pts',(-4.28696459950062,12.2,10.3102221317867));
#235915=CARTESIAN_POINT('Ctrl Pts',(-4.28694250683259,12.2,10.3068758804302));
#235916=CARTESIAN_POINT('Ctrl Pts',(-4.28691649779177,12.2,10.303537083703));
#235917=CARTESIAN_POINT('Ctrl Pts',(-4.28688181906753,12.2,10.299085354329));
#235918=CARTESIAN_POINT('Ctrl Pts',(-4.28684017474549,12.2,10.294646875694));
#235919=CARTESIAN_POINT('Ctrl Pts',(-4.28679163874214,12.2,10.2902217370098));
#235920=CARTESIAN_POINT('Ctrl Pts',(-4.28674310274541,12.2,10.2857965989284));
#235921=CARTESIAN_POINT('Ctrl Pts',(-4.28668767350513,12.2,10.281384800212));
#235922=CARTESIAN_POINT('Ctrl Pts',(-4.28662542428844,12.2,10.2769864301263));
#235923=CARTESIAN_POINT('Ctrl Pts',(-4.28656317506327,12.2,10.2725880594413));
#235924=CARTESIAN_POINT('Ctrl Pts',(-4.28649410615311,12.2,10.2682031168017));
#235925=CARTESIAN_POINT('Ctrl Pts',(-4.28641829025571,12.2,10.263831692624));
#235926=CARTESIAN_POINT('Ctrl Pts',(-4.28634247436864,12.2,10.2594602690419));
#235927=CARTESIAN_POINT('Ctrl Pts',(-4.28625991067458,12.2,10.2551023641315));
#235928=CARTESIAN_POINT('Ctrl Pts',(-4.28617067551565,12.2,10.2507580660969));
#235929=CARTESIAN_POINT('Ctrl Pts',(-4.28608144034455,12.2,10.2464137674704));
#235930=CARTESIAN_POINT('Ctrl Pts',(-4.2859855331171,12.2,10.2420830764593));
#235931=CARTESIAN_POINT('Ctrl Pts',(-4.28588302849997,12.2,10.2377660851138));
#235932=CARTESIAN_POINT('Ctrl Pts',(-4.28578052389681,12.2,10.2334490943565));
#235933=CARTESIAN_POINT('Ctrl Pts',(-4.28567142076814,12.2,10.2291458008511));
#235934=CARTESIAN_POINT('Ctrl Pts',(-4.28555579755016,12.2,10.2248562965974));
#235935=CARTESIAN_POINT('Ctrl Pts',(-4.28544017431643,12.2,10.2205667917593));
#235936=CARTESIAN_POINT('Ctrl Pts',(-4.28531802998582,12.2,10.2162910774664));
#235937=CARTESIAN_POINT('Ctrl Pts',(-4.28518944075618,12.2,10.2120292429017));
#235938=CARTESIAN_POINT('Ctrl Pts',(-4.28502870422787,12.2,10.2067019499861));
#235939=CARTESIAN_POINT('Ctrl Pts',(-4.28485790027205,12.2,10.2013963461367));
#235940=CARTESIAN_POINT('Ctrl Pts',(-4.28467717797987,12.2,10.1961126098878));
#235941=CARTESIAN_POINT('Ctrl Pts',(-4.28453260015794,12.2,10.1918856212343));
#235942=CARTESIAN_POINT('Ctrl Pts',(-4.28438167610898,12.2,10.187672629227));
#235943=CARTESIAN_POINT('Ctrl Pts',(-4.28422448428119,12.2,10.1834737243593));
#235944=CARTESIAN_POINT('Ctrl Pts',(-4.28406729243199,12.2,10.1792748189195));
#235945=CARTESIAN_POINT('Ctrl Pts',(-4.28390383270413,12.2,10.1750900033216));
#235946=CARTESIAN_POINT('Ctrl Pts',(-4.28373418619449,12.2,10.1709193681508));
#235947=CARTESIAN_POINT('Ctrl Pts',(-4.28356453970795,12.2,10.1667487335482));
#235948=CARTESIAN_POINT('Ctrl Pts',(-4.28338870502266,12.2,10.1625922801512));
#235949=CARTESIAN_POINT('Ctrl Pts',(-4.28320676453816,12.2,10.1584501027105));
#235950=CARTESIAN_POINT('Ctrl Pts',(-4.28302482402886,12.2,10.1543079247055));
#235951=CARTESIAN_POINT('Ctrl Pts',(-4.2828367775892,12.2,10.1501800218122));
#235952=CARTESIAN_POINT('Ctrl Pts',(-4.28264270579995,12.2,10.1460664880138));
#235953=CARTESIAN_POINT('Ctrl Pts',(-4.2823515981425,12.2,10.1398961878767));
#235954=CARTESIAN_POINT('Ctrl Pts',(-4.28204693588855,12.2,10.1337582201124));
#235955=CARTESIAN_POINT('Ctrl Pts',(-4.28172900023402,12.2,10.1276529038328));
#235956=CARTESIAN_POINT('Ctrl Pts',(-4.28151704311174,12.2,10.12358269261));
#235957=CARTESIAN_POINT('Ctrl Pts',(-4.28129918708875,12.2,10.1195269932723));
#235958=CARTESIAN_POINT('Ctrl Pts',(-4.28107551596507,12.2,10.1154859013864));
#235959=CARTESIAN_POINT('Ctrl Pts',(-4.28085184487187,12.2,10.111444810051));
#235960=CARTESIAN_POINT('Ctrl Pts',(-4.28062235906594,12.2,10.1074183267127));
#235961=CARTESIAN_POINT('Ctrl Pts',(-4.2803871440302,12.2,10.1034065473725));
#235962=CARTESIAN_POINT('Ctrl Pts',(-4.28015192896241,12.2,10.0993947674857));
#235963=CARTESIAN_POINT('Ctrl Pts',(-4.27991098485616,12.2,10.0953976926212));
#235964=CARTESIAN_POINT('Ctrl Pts',(-4.27966439900824,12.2,10.0914154174972));
#235965=CARTESIAN_POINT('Ctrl Pts',(-4.27941781319392,12.2,10.0874331429158));
#235966=CARTESIAN_POINT('Ctrl Pts',(-4.27916558455114,12.2,10.083465668519));
#235967=CARTESIAN_POINT('Ctrl Pts',(-4.27890780151722,12.2,10.0795130943962));
#235968=CARTESIAN_POINT('Ctrl Pts',(-4.27865001844819,12.2,10.0755605197348));
#235969=CARTESIAN_POINT('Ctrl Pts',(-4.27838668119251,12.2,10.0716228424832));
#235970=CARTESIAN_POINT('Ctrl Pts',(-4.27811787873341,12.2,10.0677001619916));
#235971=CARTESIAN_POINT('Ctrl Pts',(-4.27784907627432,12.2,10.0637774815));
#235972=CARTESIAN_POINT('Ctrl Pts',(-4.27757480808126,12.2,10.059869798263));
#235973=CARTESIAN_POINT('Ctrl Pts',(-4.27729516495435,12.2,10.0559772098302));
#235974=CARTESIAN_POINT('Ctrl Pts',(-4.27701552186555,12.2,10.0520846219277));
#235975=CARTESIAN_POINT('Ctrl Pts',(-4.27673050254173,12.2,10.0482071298711));
#235976=CARTESIAN_POINT('Ctrl Pts',(-4.27644019950861,12.2,10.0443448325026));
#235977=CARTESIAN_POINT('Ctrl Pts',(-4.27614989643593,12.2,10.0404825346078));
#235978=CARTESIAN_POINT('Ctrl Pts',(-4.27585430870949,12.2,10.0366354319501));
#235979=CARTESIAN_POINT('Ctrl Pts',(-4.27555353019256,12.2,10.0328036241318));
#235980=CARTESIAN_POINT('Ctrl Pts',(-4.27525275171662,12.2,10.0289718168355));
#235981=CARTESIAN_POINT('Ctrl Pts',(-4.27494678016914,12.2,10.0251553036538));
#235982=CARTESIAN_POINT('Ctrl Pts',(-4.27463571125046,12.2,10.0213541870191));
#235983=CARTESIAN_POINT('Ctrl Pts',(-4.27432464228939,12.2,10.0175530698665));
#235984=CARTESIAN_POINT('Ctrl Pts',(-4.27400847515131,12.2,10.0137673486649));
#235985=CARTESIAN_POINT('Ctrl Pts',(-4.27368730472844,12.2,10.0099971239946));
#235986=CARTESIAN_POINT('Ctrl Pts',(-4.27336613434934,12.2,10.006226899838));
#235987=CARTESIAN_POINT('Ctrl Pts',(-4.27303996060248,12.2,10.0024721738233));
#235988=CARTESIAN_POINT('Ctrl Pts',(-4.27270887901876,12.2,9.99873304657241));
#235989=CARTESIAN_POINT('Ctrl Pts',(-4.27237779738992,12.2,9.99499391881202));
#235990=CARTESIAN_POINT('Ctrl Pts',(-4.27204180844105,12.2,9.99127039013132));
#235991=CARTESIAN_POINT('Ctrl Pts',(-4.27170100942217,12.2,9.98756256426363));
#235992=CARTESIAN_POINT('Ctrl Pts',(-4.27136021044972,12.2,9.98385473890112));
#235993=CARTESIAN_POINT('Ctrl Pts',(-4.27101460124211,12.2,9.98016261534298));
#235994=CARTESIAN_POINT('Ctrl Pts',(-4.27066428030921,12.2,9.97648629729179));
#235995=CARTESIAN_POINT('Ctrl Pts',(-4.27031395932858,12.2,9.9728099787397));
#235996=CARTESIAN_POINT('Ctrl Pts',(-4.26995892684053,12.2,9.96914946685526));
#235997=CARTESIAN_POINT('Ctrl Pts',(-4.2695992824873,12.2,9.96550486443546));
#235998=CARTESIAN_POINT('Ctrl Pts',(-4.26923963818306,12.2,9.96186026251223));
#235999=CARTESIAN_POINT('Ctrl Pts',(-4.26887538143253,12.2,9.95823157145245));
#236000=CARTESIAN_POINT('Ctrl Pts',(-4.2685066145187,12.2,9.95461889485727));
#236001=CARTESIAN_POINT('Ctrl Pts',(-4.26813784755462,12.2,9.95100621776984));
#236002=CARTESIAN_POINT('Ctrl Pts',(-4.26776456999435,12.2,9.94740955630047));
#236003=CARTESIAN_POINT('Ctrl Pts',(-4.26738688374982,12.2,9.94382901525582));
#236004=CARTESIAN_POINT('Ctrl Pts',(-4.26700919755674,12.2,9.94024847469902));
#236005=CARTESIAN_POINT('Ctrl Pts',(-4.26662710346733,12.2,9.93668405593333));
#236006=CARTESIAN_POINT('Ctrl Pts',(-4.26624070455491,12.2,9.93313586405506));
#236007=CARTESIAN_POINT('Ctrl Pts',(-4.26585430558985,12.2,9.92958767169334));
#236008=CARTESIAN_POINT('Ctrl Pts',(-4.26546360139382,12.2,9.92605570684429));
#236009=CARTESIAN_POINT('Ctrl Pts',(-4.26506869848341,12.2,9.92254007770825));
#236010=CARTESIAN_POINT('Ctrl Pts',(-4.26467379557299,12.2,9.91902444857221));
#236011=CARTESIAN_POINT('Ctrl Pts',(-4.26427469426488,12.2,9.91552515396028));
#236012=CARTESIAN_POINT('Ctrl Pts',(-4.26387149940915,12.2,9.91204230293883));
#236013=CARTESIAN_POINT('Ctrl Pts',(-4.26346830460836,12.2,9.9085594523919));
#236014=CARTESIAN_POINT('Ctrl Pts',(-4.26306101635192,12.2,9.90509304465542));
#236015=CARTESIAN_POINT('Ctrl Pts',(-4.26264974471702,12.2,9.90164318997728));
#236016=CARTESIAN_POINT('Ctrl Pts',(-4.26223847302608,12.2,9.8981933348291));
#236017=CARTESIAN_POINT('Ctrl Pts',(-4.26182321624367,12.2,9.89476003202304));
#236018=CARTESIAN_POINT('Ctrl Pts',(-4.26140408466487,12.2,9.89134339044965));
#236019=CARTESIAN_POINT('Ctrl Pts',(-4.26098495314319,12.2,9.88792674934179));
#236020=CARTESIAN_POINT('Ctrl Pts',(-4.26056194661368,12.2,9.88452677233173));
#236021=CARTESIAN_POINT('Ctrl Pts',(-4.26013517525992,12.2,9.88114356655165));
#236022=CARTESIAN_POINT('Ctrl Pts',(-4.25970840384802,12.2,9.87776036031061));
#236023=CARTESIAN_POINT('Ctrl Pts',(-4.25927786927716,12.2,9.87439392724852));
#236024=CARTESIAN_POINT('Ctrl Pts',(-4.25884368245371,12.2,9.87104437928898));
#236025=CARTESIAN_POINT('Ctrl Pts',(-4.25840949568942,12.2,9.86769483178581));
#236026=CARTESIAN_POINT('Ctrl Pts',(-4.25797165759425,12.2,9.86436216844285));
#236027=CARTESIAN_POINT('Ctrl Pts',(-4.25753028151945,12.2,9.86104650254614));
#236028=CARTESIAN_POINT('Ctrl Pts',(-4.25697856138085,12.2,9.85690191983642));
#236029=CARTESIAN_POINT('Ctrl Pts',(-4.25642131451988,12.2,9.85278389537457));
#236030=CARTESIAN_POINT('Ctrl Pts',(-4.25585876681183,12.2,9.84869265023431));
#236031=CARTESIAN_POINT('Ctrl Pts',(-4.25529621910378,12.2,9.84460140509407));
#236032=CARTESIAN_POINT('Ctrl Pts',(-4.2547283681252,12.2,9.84053693985943));
#236033=CARTESIAN_POINT('Ctrl Pts',(-4.25415544798371,12.2,9.83649947803545));
#236034=CARTESIAN_POINT('Ctrl Pts',(-4.25358252784223,12.2,9.83246201621147));
#236035=CARTESIAN_POINT('Ctrl Pts',(-4.25300453683896,12.2,9.8284515587888));
#236036=CARTESIAN_POINT('Ctrl Pts',(-4.25242170920007,12.2,9.82446833198325));
#236037=CARTESIAN_POINT('Ctrl Pts',(-4.25183888156118,12.2,9.8204851051777));
#236038=CARTESIAN_POINT('Ctrl Pts',(-4.25125121781118,12.2,9.81652910891104));
#236039=CARTESIAN_POINT('Ctrl Pts',(-4.25065895524174,12.2,9.81260057050826));
#236040=CARTESIAN_POINT('Ctrl Pts',(-4.2500666926723,12.2,9.80867203210549));
#236041=CARTESIAN_POINT('Ctrl Pts',(-4.24946983258581,12.2,9.80477095492088));
#236042=CARTESIAN_POINT('Ctrl Pts',(-4.24886861674974,12.2,9.80089756726447));
#236043=CARTESIAN_POINT('Ctrl Pts',(-4.24814715777266,12.2,9.79624950224567));
#236044=CARTESIAN_POINT('Ctrl Pts',(-4.24741942834645,12.2,9.79164131051814));
#236045=CARTESIAN_POINT('Ctrl Pts',(-4.24668585254002,12.2,9.78707339951571));
#236046=CARTESIAN_POINT('Ctrl Pts',(-4.2460745393458,12.2,9.78326680687536));
#236047=CARTESIAN_POINT('Ctrl Pts',(-4.24545916916256,12.2,9.77948818608018));
#236048=CARTESIAN_POINT('Ctrl Pts',(-4.24483999256554,12.2,9.77573777274536));
#236049=CARTESIAN_POINT('Ctrl Pts',(-4.24397314531621,12.2,9.77048719399486));
#236050=CARTESIAN_POINT('Ctrl Pts',(-4.24309883772286,12.2,9.76529190508791));
#236051=CARTESIAN_POINT('Ctrl Pts',(-4.24221777920889,12.2,9.76015256451001));
#236052=CARTESIAN_POINT('Ctrl Pts',(-4.24158845170871,12.2,9.75648160701153));
#236053=CARTESIAN_POINT('Ctrl Pts',(-4.24095568009751,12.2,9.75283919465116));
#236054=CARTESIAN_POINT('Ctrl Pts',(-4.24031972620845,12.2,9.74922557201375));
#236055=CARTESIAN_POINT('Ctrl Pts',(-4.2396837723194,12.2,9.74561194937635));
#236056=CARTESIAN_POINT('Ctrl Pts',(-4.23904464084114,12.2,9.74202711456287));
#236057=CARTESIAN_POINT('Ctrl Pts',(-4.23840259518385,12.2,9.7384713160539));
#236058=CARTESIAN_POINT('Ctrl Pts',(-4.23776054952657,12.2,9.73491551754493));
#236059=CARTESIAN_POINT('Ctrl Pts',(-4.23711559314335,12.2,9.73138875573448));
#236060=CARTESIAN_POINT('Ctrl Pts',(-4.23646799765702,12.2,9.72789127900078));
#236061=CARTESIAN_POINT('Ctrl Pts',(-4.2358204021707,12.2,9.72439380226707));
#236062=CARTESIAN_POINT('Ctrl Pts',(-4.23517016980378,12.2,9.72092561085328));
#236063=CARTESIAN_POINT('Ctrl Pts',(-4.2345175784147,12.2,9.71748695759181));
#236064=CARTESIAN_POINT('Ctrl Pts',(-4.23386498709676,12.2,9.71404830470516));
#236065=CARTESIAN_POINT('Ctrl Pts',(-4.23321003576421,12.2,9.71063918967047));
#236066=CARTESIAN_POINT('Ctrl Pts',(-4.23255301104433,12.2,9.70725986996694));
#236067=CARTESIAN_POINT('Ctrl Pts',(-4.23189598625284,12.2,9.70388054989506));
#236068=CARTESIAN_POINT('Ctrl Pts',(-4.2312368871308,12.2,9.70053102310878));
#236069=CARTESIAN_POINT('Ctrl Pts',(-4.2305760033115,12.2,9.69721155067576));
#236070=CARTESIAN_POINT('Ctrl Pts',(-4.2299151194922,12.2,9.69389207824274));
#236071=CARTESIAN_POINT('Ctrl Pts',(-4.22925245200468,12.2,9.69060265873773));
#236072=CARTESIAN_POINT('Ctrl Pts',(-4.22858829481882,12.2,9.68734355537835));
#236073=CARTESIAN_POINT('Ctrl Pts',(-4.22779130615235,12.2,9.68343263113394));
#236074=CARTESIAN_POINT('Ctrl Pts',(-4.22699217381486,12.2,9.6795653639219));
#236075=CARTESIAN_POINT('Ctrl Pts',(-4.22619141918777,12.2,9.67574221004985));
#236076=CARTESIAN_POINT('Ctrl Pts',(-4.22539066463342,12.2,9.67191905652509));
#236077=CARTESIAN_POINT('Ctrl Pts',(-4.22458828779082,12.2,9.66814002206272));
#236078=CARTESIAN_POINT('Ctrl Pts',(-4.22378482331636,12.2,9.66440556851488));
#236079=CARTESIAN_POINT('Ctrl Pts',(-4.2229813588419,12.2,9.66067111496704));
#236080=CARTESIAN_POINT('Ctrl Pts',(-4.22217680665631,12.2,9.65698124692656));
#236081=CARTESIAN_POINT('Ctrl Pts',(-4.22137171510227,12.2,9.65333643647374));
#236082=CARTESIAN_POINT('Ctrl Pts',(-4.22056662347509,12.2,9.64969162568985));
#236083=CARTESIAN_POINT('Ctrl Pts',(-4.21976099198116,12.2,9.64609187621979));
#236084=CARTESIAN_POINT('Ctrl Pts',(-4.21895537968725,12.2,9.64253766936251));
#236085=CARTESIAN_POINT('Ctrl Pts',(-4.21814976746651,12.2,9.63898346282806));
#236086=CARTESIAN_POINT('Ctrl Pts',(-4.21734417902692,12.2,9.63547480160025));
#236087=CARTESIAN_POINT('Ctrl Pts',(-4.21653918472285,12.2,9.6320121750614));
#236088=CARTESIAN_POINT('Ctrl Pts',(-4.21573419041879,12.2,9.62854954852252));
#236089=CARTESIAN_POINT('Ctrl Pts',(-4.2149297924647,12.2,9.62513295846334));
#236090=CARTESIAN_POINT('Ctrl Pts',(-4.21412658032717,12.2,9.62176290675044));
#236091=CARTESIAN_POINT('Ctrl Pts',(-4.21332336818964,12.2,9.61839285503754));
#236092=CARTESIAN_POINT('Ctrl Pts',(-4.21252134197498,12.2,9.61506933917448));
#236093=CARTESIAN_POINT('Ctrl Pts',(-4.21172110583728,12.2,9.61179287262372));
#236094=CARTESIAN_POINT('Ctrl Pts',(-4.21092086962689,12.2,9.60851640577534));
#236095=CARTESIAN_POINT('Ctrl Pts',(-4.21012242359162,12.2,9.60528698742304));
#236096=CARTESIAN_POINT('Ctrl Pts',(-4.20932638846501,12.2,9.60210513583504));
#236097=CARTESIAN_POINT('Ctrl Pts',(-4.20853035341071,12.2,9.59892328453606));
#236098=CARTESIAN_POINT('Ctrl Pts',(-4.20773672958122,12.2,9.59578900219158));
#236099=CARTESIAN_POINT('Ctrl Pts',(-4.20694615260982,12.2,9.59270281863497));
#236100=CARTESIAN_POINT('Ctrl Pts',(-4.20615557563842,12.2,9.58961663507837));
#236101=CARTESIAN_POINT('Ctrl Pts',(-4.20536804630726,12.2,9.58657854854546));
#236102=CARTESIAN_POINT('Ctrl Pts',(-4.20458421833549,12.2,9.58358910206744));
#236103=CARTESIAN_POINT('Ctrl Pts',(-4.20380039029253,12.2,9.58059965531788));
#236104=CARTESIAN_POINT('Ctrl Pts',(-4.20302026224988,12.2,9.57765884706463));
#236105=CARTESIAN_POINT('Ctrl Pts',(-4.20224450820779,12.2,9.57476722857584));
#236106=CARTESIAN_POINT('Ctrl Pts',(-4.20133946193105,12.2,9.57139367406625));
#236107=CARTESIAN_POINT('Ctrl Pts',(-4.20044036512269,12.2,9.56808707192141));
#236108=CARTESIAN_POINT('Ctrl Pts',(-4.19954831706672,12.2,9.56484831853584));
#236109=CARTESIAN_POINT('Ctrl Pts',(-4.19878370435803,12.2,9.56207224388113));
#236110=CARTESIAN_POINT('Ctrl Pts',(-4.1980242714748,12.2,9.55934601747287));
#236111=CARTESIAN_POINT('Ctrl Pts',(-4.197270729684,12.2,9.55667021507928));
#236112=CARTESIAN_POINT('Ctrl Pts',(-4.19651718796165,12.2,9.55399441292872));
#236113=CARTESIAN_POINT('Ctrl Pts',(-4.1957695365185,12.2,9.55136903429433));
#236114=CARTESIAN_POINT('Ctrl Pts',(-4.19502851079205,12.2,9.5487946709594));
#236115=CARTESIAN_POINT('Ctrl Pts',(-4.1942874850656,12.2,9.54622030762448));
#236116=CARTESIAN_POINT('Ctrl Pts',(-4.19355308117839,12.2,9.54369695800809));
#236117=CARTESIAN_POINT('Ctrl Pts',(-4.19282605578763,12.2,9.541225224011));
#236118=CARTESIAN_POINT('Ctrl Pts',(-4.19209903033082,12.2,9.5387534897894));
#236119=CARTESIAN_POINT('Ctrl Pts',(-4.19137938308842,12.2,9.53633337259027));
#236120=CARTESIAN_POINT('Ctrl Pts',(-4.19066788768123,12.2,9.53396548726263));
#236121=CARTESIAN_POINT('Ctrl Pts',(-4.18995639233869,12.2,9.53159760215006));
#236122=CARTESIAN_POINT('Ctrl Pts',(-4.18925305123314,12.2,9.52928194966766));
#236123=CARTESIAN_POINT('Ctrl Pts',(-4.18855866100837,12.2,9.52701915974989));
#236124=CARTESIAN_POINT('Ctrl Pts',(-4.18786427078361,12.2,9.52475636983213));
#236125=CARTESIAN_POINT('Ctrl Pts',(-4.18717883320019,12.2,9.5225464444494));
#236126=CARTESIAN_POINT('Ctrl Pts',(-4.18650316910709,12.2,9.5203900265003));
#236127=CARTESIAN_POINT('Ctrl Pts',(-4.18582750495263,12.2,9.51823360835532));
#236128=CARTESIAN_POINT('Ctrl Pts',(-4.18516161557193,12.2,9.51613070056786));
#236129=CARTESIAN_POINT('Ctrl Pts',(-4.18450634945362,12.2,9.51408196179326));
#236130=CARTESIAN_POINT('Ctrl Pts',(-4.18385108339483,12.2,9.51203322320476));
#236131=CARTESIAN_POINT('Ctrl Pts',(-4.18320643897126,12.2,9.51003865696222));
#236132=CARTESIAN_POINT('Ctrl Pts',(-4.18257329224142,12.2,9.50809893927401));
#236133=CARTESIAN_POINT('Ctrl Pts',(-4.18194014551157,12.2,9.50615922158582));
#236134=CARTESIAN_POINT('Ctrl Pts',(-4.1813184946867,12.2,9.50427435327746));
#236135=CARTESIAN_POINT('Ctrl Pts',(-4.18070924579163,12.2,9.50244503059149));
#236136=CARTESIAN_POINT('Ctrl Pts',(-4.18000137932716,12.2,9.50031960009414));
#236137=CARTESIAN_POINT('Ctrl Pts',(-4.17931024776035,12.2,9.49826914627287));
#236138=CARTESIAN_POINT('Ctrl Pts',(-4.17863732200006,12.2,9.49629481199998));
#236139=CARTESIAN_POINT('Ctrl Pts',(-4.17863732200006,15.2,9.49629481199998));
#236140=CARTESIAN_POINT('Ctrl Pts',(-4.17921371838994,15.2,9.49798593339028));
#236141=CARTESIAN_POINT('Ctrl Pts',(-4.17980347320432,15.2,9.49973290402222));
#236142=CARTESIAN_POINT('Ctrl Pts',(-4.18040565894242,15.2,9.50153500107752));
#236143=CARTESIAN_POINT('Ctrl Pts',(-4.18101074872453,15.2,9.50334578875573));
#236144=CARTESIAN_POINT('Ctrl Pts',(-4.1816283933862,15.2,9.50521223961533));
#236145=CARTESIAN_POINT('Ctrl Pts',(-4.18225768153594,15.2,9.50713365465256));
#236146=CARTESIAN_POINT('Ctrl Pts',(-4.18288696962852,15.2,9.50905506951527));
#236147=CARTESIAN_POINT('Ctrl Pts',(-4.18352790475704,15.2,9.5110314483653));
#236148=CARTESIAN_POINT('Ctrl Pts',(-4.18417960573337,15.2,9.51306211020822));
#236149=CARTESIAN_POINT('Ctrl Pts',(-4.1848313067097,15.2,9.51509277205115));
#236150=CARTESIAN_POINT('Ctrl Pts',(-4.18549377339311,15.2,9.51717771630879));
#236151=CARTESIAN_POINT('Ctrl Pts',(-4.18616615540168,15.2,9.51931627925147));
#236152=CARTESIAN_POINT('Ctrl Pts',(-4.18683853747134,15.2,9.5214548423884));
#236153=CARTESIAN_POINT('Ctrl Pts',(-4.18752083262044,15.2,9.52364702327699));
#236154=CARTESIAN_POINT('Ctrl Pts',(-4.1882122158254,15.2,9.52589217348629));
#236155=CARTESIAN_POINT('Ctrl Pts',(-4.18890359896757,15.2,9.52813732349166));
#236156=CARTESIAN_POINT('Ctrl Pts',(-4.18960406803121,15.2,9.53043544456723));
#236157=CARTESIAN_POINT('Ctrl Pts',(-4.1903128232587,15.2,9.53278590074263));
#236158=CARTESIAN_POINT('Ctrl Pts',(-4.19102157848618,15.2,9.53513635691803));
#236159=CARTESIAN_POINT('Ctrl Pts',(-4.19173861711225,15.2,9.53753914979113));
#236160=CARTESIAN_POINT('Ctrl Pts',(-4.19246316150225,15.2,9.53999366086634));
#236161=CARTESIAN_POINT('Ctrl Pts',(-4.19318770595807,15.2,9.54244817216449));
#236162=CARTESIAN_POINT('Ctrl Pts',(-4.19391975577318,15.2,9.54495440119413));
#236163=CARTESIAN_POINT('Ctrl Pts',(-4.19465855331391,15.2,9.54751174358699));
#236164=CARTESIAN_POINT('Ctrl Pts',(-4.19539735078753,15.2,9.55006908574756));
#236165=CARTESIAN_POINT('Ctrl Pts',(-4.19614289568474,15.2,9.55267754192277));
#236166=CARTESIAN_POINT('Ctrl Pts',(-4.19689445332436,15.2,9.55533651916169));
#236167=CARTESIAN_POINT('Ctrl Pts',(-4.1977712706161,15.2,9.55843865943478));
#236168=CARTESIAN_POINT('Ctrl Pts',(-4.1986562689413,15.2,9.56160956489805));
#236169=CARTESIAN_POINT('Ctrl Pts',(-4.19954831706672,15.2,9.56484831853583));
#236170=CARTESIAN_POINT('Ctrl Pts',(-4.2004403651227,15.2,9.56808707192145));
#236171=CARTESIAN_POINT('Ctrl Pts',(-4.20133946193105,15.2,9.57139367406625));
#236172=CARTESIAN_POINT('Ctrl Pts',(-4.20224450820779,15.2,9.57476722857585));
#236173=CARTESIAN_POINT('Ctrl Pts',(-4.20302026224988,15.2,9.57765884706465));
#236174=CARTESIAN_POINT('Ctrl Pts',(-4.20380039029253,15.2,9.58059965531788));
#236175=CARTESIAN_POINT('Ctrl Pts',(-4.20458421833549,15.2,9.58358910206742));
#236176=CARTESIAN_POINT('Ctrl Pts',(-4.20549868427881,15.2,9.58707678953456));
#236177=CARTESIAN_POINT('Ctrl Pts',(-4.20641818769237,15.2,9.59063067933664));
#236178=CARTESIAN_POINT('Ctrl Pts',(-4.20734169189859,15.2,9.59424991633104));
#236179=CARTESIAN_POINT('Ctrl Pts',(-4.2083971253285,15.2,9.59838618738307));
#236180=CARTESIAN_POINT('Ctrl Pts',(-4.20945778375829,15.2,9.60260780484146));
#236181=CARTESIAN_POINT('Ctrl Pts',(-4.21052217185471,15.2,9.60691352288959));
#236182=CARTESIAN_POINT('Ctrl Pts',(-4.2113204629814,15.2,9.61014281164567));
#236183=CARTESIAN_POINT('Ctrl Pts',(-4.21212085226043,15.2,9.61341940851326));
#236184=CARTESIAN_POINT('Ctrl Pts',(-4.21292272751096,15.2,9.61674279561319));
#236185=CARTESIAN_POINT('Ctrl Pts',(-4.21385824852733,15.2,9.62062008011029));
#236186=CARTESIAN_POINT('Ctrl Pts',(-4.21479579237643,15.2,9.62456105328443));
#236187=CARTESIAN_POINT('Ctrl Pts',(-4.21573441113736,15.2,9.62856491264251));
#236188=CARTESIAN_POINT('Ctrl Pts',(-4.21667302997136,15.2,9.63256877231232));
#236189=CARTESIAN_POINT('Ctrl Pts',(-4.2176127251419,15.2,9.63663551817651));
#236190=CARTESIAN_POINT('Ctrl Pts',(-4.21855257821636,15.2,9.64076436423164));
#236191=CARTESIAN_POINT('Ctrl Pts',(-4.21935816652408,15.2,9.64430337495235));
#236192=CARTESIAN_POINT('Ctrl Pts',(-4.22016386916651,15.2,9.64788801128926));
#236193=CARTESIAN_POINT('Ctrl Pts',(-4.22096912638729,15.2,9.65151778782094));
#236194=CARTESIAN_POINT('Ctrl Pts',(-4.2217743836812,15.2,9.65514756468235));
#236195=CARTESIAN_POINT('Ctrl Pts',(-4.22257919142725,15.2,9.65882248044371));
#236196=CARTESIAN_POINT('Ctrl Pts',(-4.22338300301115,15.2,9.66254205958484));
#236197=CARTESIAN_POINT('Ctrl Pts',(-4.22418681452204,15.2,9.6662616383881));
#236198=CARTESIAN_POINT('Ctrl Pts',(-4.2249896287625,15.2,9.67002587872989));
#236199=CARTESIAN_POINT('Ctrl Pts',(-4.22579090923339,15.2,9.67383431250824));
#236200=CARTESIAN_POINT('Ctrl Pts',(-4.22659218970429,15.2,9.67764274628658));
#236201=CARTESIAN_POINT('Ctrl Pts',(-4.2273919355869,15.2,9.68149537398921));
#236202=CARTESIAN_POINT('Ctrl Pts',(-4.22818962418122,15.2,9.6853917328731));
#236203=CARTESIAN_POINT('Ctrl Pts',(-4.22885436470064,15.2,9.68863869872765));
#236204=CARTESIAN_POINT('Ctrl Pts',(-4.22951767659558,15.2,9.69191603427981));
#236205=CARTESIAN_POINT('Ctrl Pts',(-4.23017926145678,15.2,9.69522347504213));
#236206=CARTESIAN_POINT('Ctrl Pts',(-4.23097316333349,15.2,9.69919240417321));
#236207=CARTESIAN_POINT('Ctrl Pts',(-4.23176458125156,15.2,9.70320468565965));
#236208=CARTESIAN_POINT('Ctrl Pts',(-4.23255301104433,15.2,9.70725986996693));
#236209=CARTESIAN_POINT('Ctrl Pts',(-4.23321003576421,15.2,9.71063918967048));
#236210=CARTESIAN_POINT('Ctrl Pts',(-4.23386498709675,15.2,9.71404830470513));
#236211=CARTESIAN_POINT('Ctrl Pts',(-4.2345175784147,15.2,9.71748695759181));
#236212=CARTESIAN_POINT('Ctrl Pts',(-4.23517016980379,15.2,9.72092561085331));
#236213=CARTESIAN_POINT('Ctrl Pts',(-4.23582040217069,15.2,9.72439380226706));
#236214=CARTESIAN_POINT('Ctrl Pts',(-4.23646799765702,15.2,9.72789127900078));
#236215=CARTESIAN_POINT('Ctrl Pts',(-4.23737463135201,15.2,9.73278774650424));
#236216=CARTESIAN_POINT('Ctrl Pts',(-4.23827609342614,15.2,9.73774161429728));
#236217=CARTESIAN_POINT('Ctrl Pts',(-4.23917163474972,15.2,9.74275219602297));
#236218=CARTESIAN_POINT('Ctrl Pts',(-4.23993924155866,15.2,9.74704698013636));
#236219=CARTESIAN_POINT('Ctrl Pts',(-4.24070250021962,15.2,9.75138343396793));
#236220=CARTESIAN_POINT('Ctrl Pts',(-4.24146094910906,15.2,9.75576113280609));
#236221=CARTESIAN_POINT('Ctrl Pts',(-4.24209298987322,15.2,9.75940921530378));
#236222=CARTESIAN_POINT('Ctrl Pts',(-4.24272169185712,15.2,9.76308593987567));
#236223=CARTESIAN_POINT('Ctrl Pts',(-4.24334679348582,15.2,9.76679106512824));
#236224=CARTESIAN_POINT('Ctrl Pts',(-4.24409691548114,15.2,9.77123721567362));
#236225=CARTESIAN_POINT('Ctrl Pts',(-4.2448418516324,15.2,9.77572426313554));
#236226=CARTESIAN_POINT('Ctrl Pts',(-4.24558116158898,15.2,9.78025179346843));
#236227=CARTESIAN_POINT('Ctrl Pts',(-4.24644368977094,15.2,9.78553391157326));
#236228=CARTESIAN_POINT('Ctrl Pts',(-4.247298559351,15.2,9.79087113116104));
#236229=CARTESIAN_POINT('Ctrl Pts',(-4.24814508343819,15.2,9.79626280778627));
#236230=CARTESIAN_POINT('Ctrl Pts',(-4.24874974353813,15.2,9.8001140056156));
#236231=CARTESIAN_POINT('Ctrl Pts',(-4.24935014721639,15.2,9.80399298727936));
#236232=CARTESIAN_POINT('Ctrl Pts',(-4.24994604895274,15.2,9.80789951998627));
#236233=CARTESIAN_POINT('Ctrl Pts',(-4.2508994917179,15.2,9.81414997223214));
#236234=CARTESIAN_POINT('Ctrl Pts',(-4.25184140905278,15.2,9.82047095736259));
#236235=CARTESIAN_POINT('Ctrl Pts',(-4.25277082370742,15.2,9.82686153349416));
#236236=CARTESIAN_POINT('Ctrl Pts',(-4.25346788474588,15.2,9.83165446591934));
#236237=CARTESIAN_POINT('Ctrl Pts',(-4.25415791115355,15.2,9.83648654525185));
#236238=CARTESIAN_POINT('Ctrl Pts',(-4.25484050430775,15.2,9.84135738001288));
#236239=CARTESIAN_POINT('Ctrl Pts',(-4.25563686289465,15.2,9.84704001990375));
#236240=CARTESIAN_POINT('Ctrl Pts',(-4.25642309746418,15.2,9.85277540969495));
#236241=CARTESIAN_POINT('Ctrl Pts',(-4.25719858794428,15.2,9.85856294069254));
#236242=CARTESIAN_POINT('Ctrl Pts',(-4.25764172541323,15.2,9.8618701016488));
#236243=CARTESIAN_POINT('Ctrl Pts',(-4.25808135401352,15.2,9.86519428752709));
#236244=CARTESIAN_POINT('Ctrl Pts',(-4.2585173594837,15.2,9.8685353865022));
#236245=CARTESIAN_POINT('Ctrl Pts',(-4.25895336489447,15.2,9.87187648502209));
#236246=CARTESIAN_POINT('Ctrl Pts',(-4.25938574655631,15.2,9.87523449595351));
#236247=CARTESIAN_POINT('Ctrl Pts',(-4.25981439268832,15.2,9.87860930789814));
#236248=CARTESIAN_POINT('Ctrl Pts',(-4.26035020039713,15.2,9.88282782317378));
#236249=CARTESIAN_POINT('Ctrl Pts',(-4.26088017021993,15.2,9.88707258871565));
#236250=CARTESIAN_POINT('Ctrl Pts',(-4.26140408466487,15.2,9.89134339044964));
#236251=CARTESIAN_POINT('Ctrl Pts',(-4.26182321624367,15.2,9.89476003202305));
#236252=CARTESIAN_POINT('Ctrl Pts',(-4.26223847302608,15.2,9.89819333482909));
#236253=CARTESIAN_POINT('Ctrl Pts',(-4.26264974471702,15.2,9.90164318997727));
#236254=CARTESIAN_POINT('Ctrl Pts',(-4.26306101635192,15.2,9.90509304465541));
#236255=CARTESIAN_POINT('Ctrl Pts',(-4.26346830460836,15.2,9.90855945239188));
#236256=CARTESIAN_POINT('Ctrl Pts',(-4.26387149940915,15.2,9.91204230293881));
#236257=CARTESIAN_POINT('Ctrl Pts',(-4.26427469426487,15.2,9.91552515396027));
#236258=CARTESIAN_POINT('Ctrl Pts',(-4.26467379557299,15.2,9.9190244485722));
#236259=CARTESIAN_POINT('Ctrl Pts',(-4.26506869848341,15.2,9.92254007770824));
#236260=CARTESIAN_POINT('Ctrl Pts',(-4.26556232709453,15.2,9.92693461388879));
#236261=CARTESIAN_POINT('Ctrl Pts',(-4.26604939472039,15.2,9.9313546749043));
#236262=CARTESIAN_POINT('Ctrl Pts',(-4.26652969500033,15.2,9.93580004853568));
#236263=CARTESIAN_POINT('Ctrl Pts',(-4.26691393519288,15.2,9.93935634715005));
#236264=CARTESIAN_POINT('Ctrl Pts',(-4.26729384461615,15.2,9.94292884718883));
#236265=CARTESIAN_POINT('Ctrl Pts',(-4.26766932019701,15.2,9.94651744117152));
#236266=CARTESIAN_POINT('Ctrl Pts',(-4.26804479582903,15.2,9.95010603564316));
#236267=CARTESIAN_POINT('Ctrl Pts',(-4.26841583695788,15.2,9.95371072518317));
#236268=CARTESIAN_POINT('Ctrl Pts',(-4.26878234253341,15.2,9.95733140299159));
#236269=CARTESIAN_POINT('Ctrl Pts',(-4.26914884810893,15.2,9.9609520808));
#236270=CARTESIAN_POINT('Ctrl Pts',(-4.26951081723672,15.2,9.96458874757144));
#236271=CARTESIAN_POINT('Ctrl Pts',(-4.2698681495335,15.2,9.96824129860545));
#236272=CARTESIAN_POINT('Ctrl Pts',(-4.27022548178158,15.2,9.9718938491418));
#236273=CARTESIAN_POINT('Ctrl Pts',(-4.27057817702668,15.2,9.97556228326248));
#236274=CARTESIAN_POINT('Ctrl Pts',(-4.27092613599984,15.2,9.97924649725576));
#236275=CARTESIAN_POINT('Ctrl Pts',(-4.2712740950204,15.2,9.98293071175102));
#236276=CARTESIAN_POINT('Ctrl Pts',(-4.27161731734856,15.2,9.98663070625335));
#236277=CARTESIAN_POINT('Ctrl Pts',(-4.27195570558873,15.2,9.99034637679078));
#236278=CARTESIAN_POINT('Ctrl Pts',(-4.27254788493986,15.2,9.9968487994719));
#236279=CARTESIAN_POINT('Ctrl Pts',(-4.27312525655407,15.2,10.0033992315922));
#236280=CARTESIAN_POINT('Ctrl Pts',(-4.27368730472844,15.2,10.0099971239946));
#236281=CARTESIAN_POINT('Ctrl Pts',(-4.27400847515131,15.2,10.0137673486648));
#236282=CARTESIAN_POINT('Ctrl Pts',(-4.2743246422894,15.2,10.0175530698666));
#236283=CARTESIAN_POINT('Ctrl Pts',(-4.27463571125046,15.2,10.0213541870191));
#236284=CARTESIAN_POINT('Ctrl Pts',(-4.27494678016913,15.2,10.0251553036538));
#236285=CARTESIAN_POINT('Ctrl Pts',(-4.27525275171662,15.2,10.0289718168355));
#236286=CARTESIAN_POINT('Ctrl Pts',(-4.27555353019256,15.2,10.0328036241318));
#236287=CARTESIAN_POINT('Ctrl Pts',(-4.27585430870949,15.2,10.0366354319501));
#236288=CARTESIAN_POINT('Ctrl Pts',(-4.27614989643593,15.2,10.0404825346078));
#236289=CARTESIAN_POINT('Ctrl Pts',(-4.27644019950861,15.2,10.0443448325026));
#236290=CARTESIAN_POINT('Ctrl Pts',(-4.27680307832968,15.2,10.0491727046079));
#236291=CARTESIAN_POINT('Ctrl Pts',(-4.27715770080089,15.2,10.0540243188455));
#236292=CARTESIAN_POINT('Ctrl Pts',(-4.27750388802267,15.2,10.0588994808606));
#236293=CARTESIAN_POINT('Ctrl Pts',(-4.27778083777745,15.2,10.0627996101538));
#236294=CARTESIAN_POINT('Ctrl Pts',(-4.27805239009721,15.2,10.0667148098635));
#236295=CARTESIAN_POINT('Ctrl Pts',(-4.27831845446491,15.2,10.070644981874));
#236296=CARTESIAN_POINT('Ctrl Pts',(-4.27865103495171,15.2,10.0755576972888));
#236297=CARTESIAN_POINT('Ctrl Pts',(-4.27897504112487,15.2,10.0804938051893));
#236298=CARTESIAN_POINT('Ctrl Pts',(-4.27929029919678,15.2,10.0854531174493));
#236299=CARTESIAN_POINT('Ctrl Pts',(-4.27954250566806,15.2,10.0894205674736));
#236300=CARTESIAN_POINT('Ctrl Pts',(-4.27978911339308,15.2,10.093402866558));
#236301=CARTESIAN_POINT('Ctrl Pts',(-4.28003003579472,15.2,10.0973999177768));
#236302=CARTESIAN_POINT('Ctrl Pts',(-4.28039141936436,15.2,10.1033954940604));
#236303=CARTESIAN_POINT('Ctrl Pts',(-4.28074000931003,15.2,10.109424264108));
#236304=CARTESIAN_POINT('Ctrl Pts',(-4.28107551596507,15.2,10.1154859013864));
#236305=CARTESIAN_POINT('Ctrl Pts',(-4.28129918708875,15.2,10.1195269932723));
#236306=CARTESIAN_POINT('Ctrl Pts',(-4.28151704311174,15.2,10.12358269261));
#236307=CARTESIAN_POINT('Ctrl Pts',(-4.28172900023402,15.2,10.1276529038328));
#236308=CARTESIAN_POINT('Ctrl Pts',(-4.28199394662242,15.2,10.132740667584));
#236309=CARTESIAN_POINT('Ctrl Pts',(-4.28224967473366,15.2,10.1378511060601));
#236310=CARTESIAN_POINT('Ctrl Pts',(-4.28249602349531,15.2,10.1429840343042));
#236311=CARTESIAN_POINT('Ctrl Pts',(-4.28274237225697,15.2,10.1481169625483));
#236312=CARTESIAN_POINT('Ctrl Pts',(-4.28297933891394,15.2,10.1532723804865));
#236313=CARTESIAN_POINT('Ctrl Pts',(-4.28320676453816,15.2,10.1584501027105));
#236314=CARTESIAN_POINT('Ctrl Pts',(-4.28338870502266,15.2,10.1625922801511));
#236315=CARTESIAN_POINT('Ctrl Pts',(-4.28356453970795,15.2,10.1667487335482));
#236316=CARTESIAN_POINT('Ctrl Pts',(-4.28373418619449,15.2,10.1709193681508));
#236317=CARTESIAN_POINT('Ctrl Pts',(-4.28390383270413,15.2,10.1750900033216));
#236318=CARTESIAN_POINT('Ctrl Pts',(-4.28406729243199,15.2,10.1792748189195));
#236319=CARTESIAN_POINT('Ctrl Pts',(-4.28422448428119,15.2,10.1834737243593));
#236320=CARTESIAN_POINT('Ctrl Pts',(-4.28438167610898,15.2,10.187672629227));
#236321=CARTESIAN_POINT('Ctrl Pts',(-4.28453260015794,15.2,10.1918856212343));
#236322=CARTESIAN_POINT('Ctrl Pts',(-4.28467717797987,15.2,10.1961126098878));
#236323=CARTESIAN_POINT('Ctrl Pts',(-4.2848217558215,15.2,10.2003395991173));
#236324=CARTESIAN_POINT('Ctrl Pts',(-4.28495998530959,15.2,10.2045805832818));
#236325=CARTESIAN_POINT('Ctrl Pts',(-4.2850917917608,15.2,10.2088354718479));
#236326=CARTESIAN_POINT('Ctrl Pts',(-4.28522359819404,15.2,10.2130903598343));
#236327=CARTESIAN_POINT('Ctrl Pts',(-4.28534898008323,15.2,10.2173591505687));
#236328=CARTESIAN_POINT('Ctrl Pts',(-4.28546785869113,15.2,10.2216417541536));
#236329=CARTESIAN_POINT('Ctrl Pts',(-4.28558673731522,15.2,10.2259243583219));
#236330=CARTESIAN_POINT('Ctrl Pts',(-4.28569911563389,15.2,10.2302207757055));
#236331=CARTESIAN_POINT('Ctrl Pts',(-4.28580491425033,15.2,10.2345309123858));
#236332=CARTESIAN_POINT('Ctrl Pts',(-4.28591071285237,15.2,10.2388410484787));
#236333=CARTESIAN_POINT('Ctrl Pts',(-4.2860099334585,15.2,10.2431649054134));
#236334=CARTESIAN_POINT('Ctrl Pts',(-4.28610249945161,15.2,10.2475023940574));
#236335=CARTESIAN_POINT('Ctrl Pts',(-4.28621820695246,15.2,10.2529242553057));
#236336=CARTESIAN_POINT('Ctrl Pts',(-4.28632352038913,15.2,10.2583674126997));
#236337=CARTESIAN_POINT('Ctrl Pts',(-4.28641829025571,15.2,10.263831692624));
#236338=CARTESIAN_POINT('Ctrl Pts',(-4.2865320141018,15.2,10.2703888288905));
#236339=CARTESIAN_POINT('Ctrl Pts',(-4.28663055673067,15.2,10.2769763806085));
#236340=CARTESIAN_POINT('Ctrl Pts',(-4.28671367348414,15.2,10.2835940464713));
#236341=CARTESIAN_POINT('Ctrl Pts',(-4.28676908464557,15.2,10.288005823112));
#236342=CARTESIAN_POINT('Ctrl Pts',(-4.28681763861068,15.2,10.2924309831509));
#236343=CARTESIAN_POINT('Ctrl Pts',(-4.28685926449661,15.2,10.2968694391205));
#236344=CARTESIAN_POINT('Ctrl Pts',(-4.28690089038822,15.2,10.3013078956949));
#236345=CARTESIAN_POINT('Ctrl Pts',(-4.28693558675733,15.2,10.3057596469692));
#236346=CARTESIAN_POINT('Ctrl Pts',(-4.2869632845374,15.2,10.3102246058812));
#236347=CARTESIAN_POINT('Ctrl Pts',(-4.28700483120372,15.2,10.3169220436409));
#236348=CARTESIAN_POINT('Ctrl Pts',(-4.28703062650878,15.2,10.3236491973451));
#236349=CARTESIAN_POINT('Ctrl Pts',(-4.28704043542509,15.2,10.3304057707665));
#236350=CARTESIAN_POINT('Ctrl Pts',(-4.28704533988324,15.2,10.3337840574773));
#236351=CARTESIAN_POINT('Ctrl Pts',(-4.28704624763323,15.2,10.3371696990708));
#236352=CARTESIAN_POINT('Ctrl Pts',(-4.28704313000869,15.2,10.3405626588219));
#236353=CARTESIAN_POINT('Ctrl Pts',(-4.28704001238415,15.2,10.343955618573));
#236354=CARTESIAN_POINT('Ctrl Pts',(-4.28703286856856,15.2,10.3473558971951));
#236355=CARTESIAN_POINT('Ctrl Pts',(-4.28702167002721,15.2,10.3507634570741));
#236356=CARTESIAN_POINT('Ctrl Pts',(-4.28700673863739,15.2,10.3553068706586));
#236357=CARTESIAN_POINT('Ctrl Pts',(-4.28698459864969,15.2,10.3598632302321));
#236358=CARTESIAN_POINT('Ctrl Pts',(-4.28695518198094,15.2,10.3644324476486));
#236359=CARTESIAN_POINT('Ctrl Pts',(-4.2869257653162,15.2,10.3690016644425));
#236360=CARTESIAN_POINT('Ctrl Pts',(-4.2868890726196,15.2,10.3735837396813));
#236361=CARTESIAN_POINT('Ctrl Pts',(-4.28684503529062,15.2,10.3781785877487));
#236362=CARTESIAN_POINT('Ctrl Pts',(-4.28681200728638,15.2,10.3816247245818));
#236363=CARTESIAN_POINT('Ctrl Pts',(-4.28677484828098,15.2,10.3850780466838));
#236364=CARTESIAN_POINT('Ctrl Pts',(-4.28673353119107,15.2,10.388538517021));
#236365=CARTESIAN_POINT('Ctrl Pts',(-4.28669221410867,15.2,10.3919989867296));
#236366=CARTESIAN_POINT('Ctrl Pts',(-4.28664673729159,15.2,10.3954666050241));
#236367=CARTESIAN_POINT('Ctrl Pts',(-4.28659707424877,15.2,10.3989413359473));
#236368=CARTESIAN_POINT('Ctrl Pts',(-4.28653085686134,15.2,10.4035743103011));
#236369=CARTESIAN_POINT('Ctrl Pts',(-4.28645719745508,15.2,10.4082199292731));
#236370=CARTESIAN_POINT('Ctrl Pts',(-4.28637602823998,15.2,10.4128781073359));
#236371=CARTESIAN_POINT('Ctrl Pts',(-4.2863151513259,15.2,10.4163717410417));
#236372=CARTESIAN_POINT('Ctrl Pts',(-4.28625005169543,15.2,10.4198724393804));
#236373=CARTESIAN_POINT('Ctrl Pts',(-4.2861807007402,15.2,10.4233801679603));
#236374=CARTESIAN_POINT('Ctrl Pts',(-4.28611134977236,15.2,10.4268878971774));
#236375=CARTESIAN_POINT('Ctrl Pts',(-4.28603774857834,15.2,10.4304026542049));
#236376=CARTESIAN_POINT('Ctrl Pts',(-4.2859598699831,15.2,10.4339244055093));
#236377=CARTESIAN_POINT('Ctrl Pts',(-4.28588199140202,15.2,10.437446156174));
#236378=CARTESIAN_POINT('Ctrl Pts',(-4.28579983431833,15.2,10.4409749009018));
#236379=CARTESIAN_POINT('Ctrl Pts',(-4.28571337327498,15.2,10.4445106042007));
#236380=CARTESIAN_POINT('Ctrl Pts',(-4.28562691223164,15.2,10.4480463074996));
#236381=CARTESIAN_POINT('Ctrl Pts',(-4.28553614595324,15.2,10.451588966932));
#236382=CARTESIAN_POINT('Ctrl Pts',(-4.28544104945631,15.2,10.4551385505953));
#236383=CARTESIAN_POINT('Ctrl Pts',(-4.28531425413284,15.2,10.4598713285981));
#236384=CARTESIAN_POINT('Ctrl Pts',(-4.28517975971091,15.2,10.4646164143845));
#236385=CARTESIAN_POINT('Ctrl Pts',(-4.28503750305668,15.2,10.4693737244388));
#236386=CARTESIAN_POINT('Ctrl Pts',(-4.28489524638305,15.2,10.4741310351412));
#236387=CARTESIAN_POINT('Ctrl Pts',(-4.28474522652536,15.2,10.4789005686615));
#236388=CARTESIAN_POINT('Ctrl Pts',(-4.28458738451676,15.2,10.4836822446999));
#236389=CARTESIAN_POINT('Ctrl Pts',(-4.28446900302105,15.2,10.487268501403));
#236390=CARTESIAN_POINT('Ctrl Pts',(-4.2843462211422,15.2,10.4908615878557));
#236391=CARTESIAN_POINT('Ctrl Pts',(-4.28421901227221,15.2,10.4944614680993));
#236392=CARTESIAN_POINT('Ctrl Pts',(-4.28404940043015,15.2,10.4992613088601));
#236393=CARTESIAN_POINT('Ctrl Pts',(-4.28387192050986,15.2,10.5040732302728));
#236394=CARTESIAN_POINT('Ctrl Pts',(-4.28368651048981,15.2,10.508897148));
#236395=CARTESIAN_POINT('Ctrl Pts',(-4.28354745298739,15.2,10.5125150859667));
#236396=CARTESIAN_POINT('Ctrl Pts',(-4.28340393492889,15.2,10.5161397719106));
#236397=CARTESIAN_POINT('Ctrl Pts',(-4.28325593147555,15.2,10.5197711726125));
#236398=CARTESIAN_POINT('Ctrl Pts',(-4.2831079280222,15.2,10.5234025733145));
#236399=CARTESIAN_POINT('Ctrl Pts',(-4.28295543912772,15.2,10.527040687749));
#236400=CARTESIAN_POINT('Ctrl Pts',(-4.28279843925842,15.2,10.5306854810333));
#236401=CARTESIAN_POINT('Ctrl Pts',(-4.28253677280009,15.2,10.5367601367277));
#236402=CARTESIAN_POINT('Ctrl Pts',(-4.28226257845127,15.2,10.5428533464254));
#236403=CARTESIAN_POINT('Ctrl Pts',(-4.2819757394916,15.2,10.5489649535366));
#236404=CARTESIAN_POINT('Ctrl Pts',(-4.28174626834262,15.2,10.5538542388258));
#236405=CARTESIAN_POINT('Ctrl Pts',(-4.281508706411,15.2,10.5587552956745));
#236406=CARTESIAN_POINT('Ctrl Pts',(-4.28126299326526,15.2,10.5636680444384));
#236407=CARTESIAN_POINT('Ctrl Pts',(-4.28095585180797,15.2,10.5698089808952));
#236408=CARTESIAN_POINT('Ctrl Pts',(-4.28063597617033,15.2,10.575968186299));
#236409=CARTESIAN_POINT('Ctrl Pts',(-4.28030325631027,15.2,10.5821455059503));
#236410=CARTESIAN_POINT('Ctrl Pts',(-4.27997053645021,15.2,10.5883228256015));
#236411=CARTESIAN_POINT('Ctrl Pts',(-4.27962497293089,15.2,10.5945182582029));
#236412=CARTESIAN_POINT('Ctrl Pts',(-4.279266452775,15.2,10.6007316449704));
#236413=CARTESIAN_POINT('Ctrl Pts',(-4.27905134068927,15.2,10.6044596768954));
#236414=CARTESIAN_POINT('Ctrl Pts',(-4.27883156299022,15.2,10.6081941721879));
#236415=CARTESIAN_POINT('Ctrl Pts',(-4.27860709758235,15.2,10.6119350969261));
#236416=CARTESIAN_POINT('Ctrl Pts',(-4.27823298855564,15.2,10.6181699717163));
#236417=CARTESIAN_POINT('Ctrl Pts',(-4.27784585964581,15.2,10.624422708598));
#236418=CARTESIAN_POINT('Ctrl Pts',(-4.27744560978577,15.2,10.6306931633881));
#236419=CARTESIAN_POINT('Ctrl Pts',(-4.27720545983485,15.2,10.634455436809));
#236420=CARTESIAN_POINT('Ctrl Pts',(-4.27696058651593,15.2,10.6382240885234));
#236421=CARTESIAN_POINT('Ctrl Pts',(-4.27671096093733,15.2,10.6419990772812));
#236422=CARTESIAN_POINT('Ctrl Pts',(-4.27646133540409,15.2,10.6457740653533));
#236423=CARTESIAN_POINT('Ctrl Pts',(-4.27620695657065,15.2,10.6495553893138));
#236424=CARTESIAN_POINT('Ctrl Pts',(-4.27594780073323,15.2,10.6533430147828));
#236425=CARTESIAN_POINT('Ctrl Pts',(-4.27568864489581,15.2,10.6571306402518));
#236426=CARTESIAN_POINT('Ctrl Pts',(-4.27542471209421,15.2,10.660924565292));
#236427=CARTESIAN_POINT('Ctrl Pts',(-4.27515599200001,15.2,10.6647247759375));
#236428=CARTESIAN_POINT('Ctrl Pts',(-4.27488727190581,15.2,10.668524986583));
#236429=CARTESIAN_POINT('Ctrl Pts',(-4.27461376005061,15.2,10.6723314813073));
#236430=CARTESIAN_POINT('Ctrl Pts',(-4.27433547000006,15.2,10.676144262));
#236431=CARTESIAN_POINT('Origin',(-5.66257110645729E-14,15.2,-1.77635683940025E-14));
#236432=CARTESIAN_POINT('',(-4.5738377119823,15.2,9.31239140029717));
#236433=CARTESIAN_POINT('',(-4.5738377119823,12.2,9.31239140029717));
#236434=CARTESIAN_POINT('',(-4.57383771200006,15.2,9.31239139999998));
#236435=CARTESIAN_POINT('Origin',(-5.66257110645729E-14,12.2,-1.77635683940025E-14));
#236436=CARTESIAN_POINT('Origin',(-5.66257110645729E-14,15.2,-1.77635683940025E-14));
#236437=CARTESIAN_POINT('Origin',(-5.66257110645729E-14,15.2,-1.77635683940025E-14));
#236438=CARTESIAN_POINT('',(-5.41482055400006,15.2,10.145428447));
#236439=CARTESIAN_POINT('',(-5.75020264100006,15.2,9.95917514599999));
#236440=CARTESIAN_POINT('Origin',(-5.66257110645729E-14,15.2,-1.77635683940025E-14));
#236441=CARTESIAN_POINT('',(-5.75020264100006,12.2,9.95917514599999));
#236442=CARTESIAN_POINT('',(-5.75020264100006,15.2,9.95917514599999));
#236443=CARTESIAN_POINT('',(-5.41482055400006,12.2,10.145428447));
#236444=CARTESIAN_POINT('Origin',(-5.66257110645729E-14,12.2,-1.77635683940025E-14));
#236445=CARTESIAN_POINT('',(-5.41482055400006,15.2,10.145428447));
#236446=CARTESIAN_POINT('Ctrl Pts',(-5.75020264100006,15.2,9.95917514599999));
#236447=CARTESIAN_POINT('Ctrl Pts',(-5.75020264100006,11.6,9.95917514599999));
#236448=CARTESIAN_POINT('Ctrl Pts',(-5.75014921100006,15.2,9.95841243099999));
#236449=CARTESIAN_POINT('Ctrl Pts',(-5.75014921100006,11.6,9.95841243099999));
#236450=CARTESIAN_POINT('Ctrl Pts',(-5.75004209300006,15.2,9.95688745999999));
#236451=CARTESIAN_POINT('Ctrl Pts',(-5.75004209300006,11.6,9.95688745999999));
#236452=CARTESIAN_POINT('Ctrl Pts',(-5.74988064800006,15.2,9.95460138499999));
#236453=CARTESIAN_POINT('Ctrl Pts',(-5.74988064800006,11.6,9.95460138499999));
#236454=CARTESIAN_POINT('Ctrl Pts',(-5.74966385000006,15.2,9.95155604499999));
#236455=CARTESIAN_POINT('Ctrl Pts',(-5.74966385000006,11.6,9.95155604499999));
#236456=CARTESIAN_POINT('Ctrl Pts',(-5.74939029000006,15.2,9.94775396999999));
#236457=CARTESIAN_POINT('Ctrl Pts',(-5.74939029000006,11.6,9.94775396999999));
#236458=CARTESIAN_POINT('Ctrl Pts',(-5.74911416700005,15.2,9.94395649799999));
#236459=CARTESIAN_POINT('Ctrl Pts',(-5.74911416700005,11.6,9.94395649799999));
#236460=CARTESIAN_POINT('Ctrl Pts',(-5.74883548500006,15.2,9.94016363199999));
#236461=CARTESIAN_POINT('Ctrl Pts',(-5.74883548500006,11.6,9.94016363199999));
#236462=CARTESIAN_POINT('Ctrl Pts',(-5.74855424400006,15.2,9.93637536999999));
#236463=CARTESIAN_POINT('Ctrl Pts',(-5.74855424400006,11.6,9.93637536999999));
#236464=CARTESIAN_POINT('Ctrl Pts',(-5.74827044900006,15.2,9.93259172099999));
#236465=CARTESIAN_POINT('Ctrl Pts',(-5.74827044900006,11.6,9.93259172099999));
#236466=CARTESIAN_POINT('Ctrl Pts',(-5.74798410500006,15.2,9.92881268999999));
#236467=CARTESIAN_POINT('Ctrl Pts',(-5.74798410500006,11.6,9.92881268999999));
#236468=CARTESIAN_POINT('Ctrl Pts',(-5.74769522100006,15.2,9.92503828399999));
#236469=CARTESIAN_POINT('Ctrl Pts',(-5.74769522100006,11.6,9.92503828399999));
#236470=CARTESIAN_POINT('Ctrl Pts',(-5.74740380000006,15.2,9.92126850899999));
#236471=CARTESIAN_POINT('Ctrl Pts',(-5.74740380000006,11.6,9.92126850899999));
#236472=CARTESIAN_POINT('Ctrl Pts',(-5.74710985300006,15.2,9.91750337599999));
#236473=CARTESIAN_POINT('Ctrl Pts',(-5.74710985300006,11.6,9.91750337599999));
#236474=CARTESIAN_POINT('Ctrl Pts',(-5.74681338800006,15.2,9.91374289199998));
#236475=CARTESIAN_POINT('Ctrl Pts',(-5.74681338800006,11.6,9.91374289199998));
#236476=CARTESIAN_POINT('Ctrl Pts',(-5.74651440900006,15.2,9.90998706399999));
#236477=CARTESIAN_POINT('Ctrl Pts',(-5.74651440900006,11.6,9.90998706399999));
#236478=CARTESIAN_POINT('Ctrl Pts',(-5.74621292500006,15.2,9.90623589899998));
#236479=CARTESIAN_POINT('Ctrl Pts',(-5.74621292500006,11.6,9.90623589899998));
#236480=CARTESIAN_POINT('Ctrl Pts',(-5.74590894000006,15.2,9.90248940599999));
#236481=CARTESIAN_POINT('Ctrl Pts',(-5.74590894000006,11.6,9.90248940599999));
#236482=CARTESIAN_POINT('Ctrl Pts',(-5.74560246200006,15.2,9.89874758699998));
#236483=CARTESIAN_POINT('Ctrl Pts',(-5.74560246200006,11.6,9.89874758699998));
#236484=CARTESIAN_POINT('Ctrl Pts',(-5.74529349500006,15.2,9.89501044999999));
#236485=CARTESIAN_POINT('Ctrl Pts',(-5.74529349500006,11.6,9.89501044999999));
#236486=CARTESIAN_POINT('Ctrl Pts',(-5.74498204400006,15.2,9.89127800199999));
#236487=CARTESIAN_POINT('Ctrl Pts',(-5.74498204400006,11.6,9.89127800199999));
#236488=CARTESIAN_POINT('Ctrl Pts',(-5.74466811600006,15.2,9.88755024699999));
#236489=CARTESIAN_POINT('Ctrl Pts',(-5.74466811600006,11.6,9.88755024699999));
#236490=CARTESIAN_POINT('Ctrl Pts',(-5.74435171600006,15.2,9.88382719299998));
#236491=CARTESIAN_POINT('Ctrl Pts',(-5.74435171600006,11.6,9.88382719299998));
#236492=CARTESIAN_POINT('Ctrl Pts',(-5.74403285200006,15.2,9.88010884599999));
#236493=CARTESIAN_POINT('Ctrl Pts',(-5.74403285200006,11.6,9.88010884599999));
#236494=CARTESIAN_POINT('Ctrl Pts',(-5.74371152900006,15.2,9.87639521399998));
#236495=CARTESIAN_POINT('Ctrl Pts',(-5.74371152900006,11.6,9.87639521399998));
#236496=CARTESIAN_POINT('Ctrl Pts',(-5.74338775500006,15.2,9.87268630299998));
#236497=CARTESIAN_POINT('Ctrl Pts',(-5.74338775500006,11.6,9.87268630299998));
#236498=CARTESIAN_POINT('Ctrl Pts',(-5.74306153500006,15.2,9.86898211999998));
#236499=CARTESIAN_POINT('Ctrl Pts',(-5.74306153500006,11.6,9.86898211999998));
#236500=CARTESIAN_POINT('Ctrl Pts',(-5.74273287600006,15.2,9.86528267199999));
#236501=CARTESIAN_POINT('Ctrl Pts',(-5.74273287600006,11.6,9.86528267199999));
#236502=CARTESIAN_POINT('Ctrl Pts',(-5.74240178500006,15.2,9.86158796599998));
#236503=CARTESIAN_POINT('Ctrl Pts',(-5.74240178500006,11.6,9.86158796599998));
#236504=CARTESIAN_POINT('Ctrl Pts',(-5.74206826800006,15.2,9.85789800899998));
#236505=CARTESIAN_POINT('Ctrl Pts',(-5.74206826800006,11.6,9.85789800899998));
#236506=CARTESIAN_POINT('Ctrl Pts',(-5.74173233000006,15.2,9.85421280699999));
#236507=CARTESIAN_POINT('Ctrl Pts',(-5.74173233000006,11.6,9.85421280699999));
#236508=CARTESIAN_POINT('Ctrl Pts',(-5.74139397800006,15.2,9.85053236499999));
#236509=CARTESIAN_POINT('Ctrl Pts',(-5.74139397800006,11.6,9.85053236499999));
#236510=CARTESIAN_POINT('Ctrl Pts',(-5.74105321900006,15.2,9.84685669199998));
#236511=CARTESIAN_POINT('Ctrl Pts',(-5.74105321900006,11.6,9.84685669199998));
#236512=CARTESIAN_POINT('Ctrl Pts',(-5.74071005800006,15.2,9.84318579399999));
#236513=CARTESIAN_POINT('Ctrl Pts',(-5.74071005800006,11.6,9.84318579399999));
#236514=CARTESIAN_POINT('Ctrl Pts',(-5.74036450400006,15.2,9.83951967699999));
#236515=CARTESIAN_POINT('Ctrl Pts',(-5.74036450400006,11.6,9.83951967699999));
#236516=CARTESIAN_POINT('Ctrl Pts',(-5.74001656100006,15.2,9.83585834899999));
#236517=CARTESIAN_POINT('Ctrl Pts',(-5.74001656100006,11.6,9.83585834899999));
#236518=CARTESIAN_POINT('Ctrl Pts',(-5.73966623600006,15.2,9.83220181499998));
#236519=CARTESIAN_POINT('Ctrl Pts',(-5.73966623600006,11.6,9.83220181499998));
#236520=CARTESIAN_POINT('Ctrl Pts',(-5.73931353600006,15.2,9.82855008299998));
#236521=CARTESIAN_POINT('Ctrl Pts',(-5.73931353600006,11.6,9.82855008299998));
#236522=CARTESIAN_POINT('Ctrl Pts',(-5.73895846700006,15.2,9.82490316099998));
#236523=CARTESIAN_POINT('Ctrl Pts',(-5.73895846700006,11.6,9.82490316099998));
#236524=CARTESIAN_POINT('Ctrl Pts',(-5.73860103600006,15.2,9.82126105199999));
#236525=CARTESIAN_POINT('Ctrl Pts',(-5.73860103600006,11.6,9.82126105199999));
#236526=CARTESIAN_POINT('Ctrl Pts',(-5.73824124900006,15.2,9.81762376799999));
#236527=CARTESIAN_POINT('Ctrl Pts',(-5.73824124900006,11.6,9.81762376799999));
#236528=CARTESIAN_POINT('Ctrl Pts',(-5.73787911300006,15.2,9.81399130999998));
#236529=CARTESIAN_POINT('Ctrl Pts',(-5.73787911300006,11.6,9.81399130999998));
#236530=CARTESIAN_POINT('Ctrl Pts',(-5.73751463500006,15.2,9.81036368899998));
#236531=CARTESIAN_POINT('Ctrl Pts',(-5.73751463500006,11.6,9.81036368899998));
#236532=CARTESIAN_POINT('Ctrl Pts',(-5.73714782000006,15.2,9.80674091099999));
#236533=CARTESIAN_POINT('Ctrl Pts',(-5.73714782000006,11.6,9.80674091099999));
#236534=CARTESIAN_POINT('Ctrl Pts',(-5.73677867600006,15.2,9.80312298099999));
#236535=CARTESIAN_POINT('Ctrl Pts',(-5.73677867600006,11.6,9.80312298099999));
#236536=CARTESIAN_POINT('Ctrl Pts',(-5.73640720900006,15.2,9.79950990699999));
#236537=CARTESIAN_POINT('Ctrl Pts',(-5.73640720900006,11.6,9.79950990699999));
#236538=CARTESIAN_POINT('Ctrl Pts',(-5.73603342500006,15.2,9.79590169699998));
#236539=CARTESIAN_POINT('Ctrl Pts',(-5.73603342500006,11.6,9.79590169699998));
#236540=CARTESIAN_POINT('Ctrl Pts',(-5.73565733200006,15.2,9.79229835499999));
#236541=CARTESIAN_POINT('Ctrl Pts',(-5.73565733200006,11.6,9.79229835499999));
#236542=CARTESIAN_POINT('Ctrl Pts',(-5.73527893600006,15.2,9.78869988999998));
#236543=CARTESIAN_POINT('Ctrl Pts',(-5.73527893600006,11.6,9.78869988999998));
#236544=CARTESIAN_POINT('Ctrl Pts',(-5.73489824300006,15.2,9.78510630799999));
#236545=CARTESIAN_POINT('Ctrl Pts',(-5.73489824300006,11.6,9.78510630799999));
#236546=CARTESIAN_POINT('Ctrl Pts',(-5.73451526200006,15.2,9.78151761599998));
#236547=CARTESIAN_POINT('Ctrl Pts',(-5.73451526200006,11.6,9.78151761599998));
#236548=CARTESIAN_POINT('Ctrl Pts',(-5.73412999600006,15.2,9.77793381999999));
#236549=CARTESIAN_POINT('Ctrl Pts',(-5.73412999600006,11.6,9.77793381999999));
#236550=CARTESIAN_POINT('Ctrl Pts',(-5.73374245400006,15.2,9.77435492899998));
#236551=CARTESIAN_POINT('Ctrl Pts',(-5.73374245400006,11.6,9.77435492899998));
#236552=CARTESIAN_POINT('Ctrl Pts',(-5.73335264400006,15.2,9.77078094799998));
#236553=CARTESIAN_POINT('Ctrl Pts',(-5.73335264400006,11.6,9.77078094799998));
#236554=CARTESIAN_POINT('Ctrl Pts',(-5.73296057100006,15.2,9.76721188399999));
#236555=CARTESIAN_POINT('Ctrl Pts',(-5.73296057100006,11.6,9.76721188399999));
#236556=CARTESIAN_POINT('Ctrl Pts',(-5.73256624100006,15.2,9.76364774399999));
#236557=CARTESIAN_POINT('Ctrl Pts',(-5.73256624100006,11.6,9.76364774399999));
#236558=CARTESIAN_POINT('Ctrl Pts',(-5.73216966200006,15.2,9.76008853499999));
#236559=CARTESIAN_POINT('Ctrl Pts',(-5.73216966200006,11.6,9.76008853499999));
#236560=CARTESIAN_POINT('Ctrl Pts',(-5.73177084200006,15.2,9.75653426499999));
#236561=CARTESIAN_POINT('Ctrl Pts',(-5.73177084200006,11.6,9.75653426499999));
#236562=CARTESIAN_POINT('Ctrl Pts',(-5.73136978500006,15.2,9.75298493899999));
#236563=CARTESIAN_POINT('Ctrl Pts',(-5.73136978500006,11.6,9.75298493899999));
#236564=CARTESIAN_POINT('Ctrl Pts',(-5.73096649900006,15.2,9.74944056499999));
#236565=CARTESIAN_POINT('Ctrl Pts',(-5.73096649900006,11.6,9.74944056499999));
#236566=CARTESIAN_POINT('Ctrl Pts',(-5.73056099300006,15.2,9.74590114899998));
#236567=CARTESIAN_POINT('Ctrl Pts',(-5.73056099300006,11.6,9.74590114899998));
#236568=CARTESIAN_POINT('Ctrl Pts',(-5.73015327100006,15.2,9.74236669799998));
#236569=CARTESIAN_POINT('Ctrl Pts',(-5.73015327100006,11.6,9.74236669799998));
#236570=CARTESIAN_POINT('Ctrl Pts',(-5.72974334100006,15.2,9.73883721999999));
#236571=CARTESIAN_POINT('Ctrl Pts',(-5.72974334100006,11.6,9.73883721999999));
#236572=CARTESIAN_POINT('Ctrl Pts',(-5.72933121000006,15.2,9.73531272199999));
#236573=CARTESIAN_POINT('Ctrl Pts',(-5.72933121000006,11.6,9.73531272199999));
#236574=CARTESIAN_POINT('Ctrl Pts',(-5.72891688500006,15.2,9.73179320899998));
#236575=CARTESIAN_POINT('Ctrl Pts',(-5.72891688500006,11.6,9.73179320899998));
#236576=CARTESIAN_POINT('Ctrl Pts',(-5.72850037300006,15.2,9.72827868899999));
#236577=CARTESIAN_POINT('Ctrl Pts',(-5.72850037300006,11.6,9.72827868899999));
#236578=CARTESIAN_POINT('Ctrl Pts',(-5.72808168000006,15.2,9.72476916899998));
#236579=CARTESIAN_POINT('Ctrl Pts',(-5.72808168000006,11.6,9.72476916899998));
#236580=CARTESIAN_POINT('Ctrl Pts',(-5.72766081400006,15.2,9.72126465699999));
#236581=CARTESIAN_POINT('Ctrl Pts',(-5.72766081400006,11.6,9.72126465699999));
#236582=CARTESIAN_POINT('Ctrl Pts',(-5.72723778200006,15.2,9.71776515799998));
#236583=CARTESIAN_POINT('Ctrl Pts',(-5.72723778200006,11.6,9.71776515799998));
#236584=CARTESIAN_POINT('Ctrl Pts',(-5.72681259100006,15.2,9.71427067999999));
#236585=CARTESIAN_POINT('Ctrl Pts',(-5.72681259100006,11.6,9.71427067999999));
#236586=CARTESIAN_POINT('Ctrl Pts',(-5.72638524800006,15.2,9.71078122899998));
#236587=CARTESIAN_POINT('Ctrl Pts',(-5.72638524800006,11.6,9.71078122899998));
#236588=CARTESIAN_POINT('Ctrl Pts',(-5.72595575900006,15.2,9.70729681399998));
#236589=CARTESIAN_POINT('Ctrl Pts',(-5.72595575900006,11.6,9.70729681399998));
#236590=CARTESIAN_POINT('Ctrl Pts',(-5.72552413200006,15.2,9.70381743999998));
#236591=CARTESIAN_POINT('Ctrl Pts',(-5.72552413200006,11.6,9.70381743999998));
#236592=CARTESIAN_POINT('Ctrl Pts',(-5.72509037500006,15.2,9.70034311599999));
#236593=CARTESIAN_POINT('Ctrl Pts',(-5.72509037500006,11.6,9.70034311599999));
#236594=CARTESIAN_POINT('Ctrl Pts',(-5.72465449300006,15.2,9.69687384599998));
#236595=CARTESIAN_POINT('Ctrl Pts',(-5.72465449300006,11.6,9.69687384599998));
#236596=CARTESIAN_POINT('Ctrl Pts',(-5.72421649500006,15.2,9.69340963899998));
#236597=CARTESIAN_POINT('Ctrl Pts',(-5.72421649500006,11.6,9.69340963899998));
#236598=CARTESIAN_POINT('Ctrl Pts',(-5.72377638800006,15.2,9.68995050099998));
#236599=CARTESIAN_POINT('Ctrl Pts',(-5.72377638800006,11.6,9.68995050099998));
#236600=CARTESIAN_POINT('Ctrl Pts',(-5.72333417800006,15.2,9.68649644199999));
#236601=CARTESIAN_POINT('Ctrl Pts',(-5.72333417800006,11.6,9.68649644199999));
#236602=CARTESIAN_POINT('Ctrl Pts',(-5.72288987300006,15.2,9.68304746399999));
#236603=CARTESIAN_POINT('Ctrl Pts',(-5.72288987300006,11.6,9.68304746399999));
#236604=CARTESIAN_POINT('Ctrl Pts',(-5.72244348000006,15.2,9.67960357899998));
#236605=CARTESIAN_POINT('Ctrl Pts',(-5.72244348000006,11.6,9.67960357899998));
#236606=CARTESIAN_POINT('Ctrl Pts',(-5.72199500700005,15.2,9.67616478899998));
#236607=CARTESIAN_POINT('Ctrl Pts',(-5.72199500700005,11.6,9.67616478899998));
#236608=CARTESIAN_POINT('Ctrl Pts',(-5.72154446100006,15.2,9.67273110599999));
#236609=CARTESIAN_POINT('Ctrl Pts',(-5.72154446100006,11.6,9.67273110599999));
#236610=CARTESIAN_POINT('Ctrl Pts',(-5.72109184700006,15.2,9.66930253499999));
#236611=CARTESIAN_POINT('Ctrl Pts',(-5.72109184700006,11.6,9.66930253499999));
#236612=CARTESIAN_POINT('Ctrl Pts',(-5.72063717600006,15.2,9.66587908099999));
#236613=CARTESIAN_POINT('Ctrl Pts',(-5.72063717600006,11.6,9.66587908099999));
#236614=CARTESIAN_POINT('Ctrl Pts',(-5.72018045300006,15.2,9.66246075399999));
#236615=CARTESIAN_POINT('Ctrl Pts',(-5.72018045300006,11.6,9.66246075399999));
#236616=CARTESIAN_POINT('Ctrl Pts',(-5.71972168400006,15.2,9.65904755899999));
#236617=CARTESIAN_POINT('Ctrl Pts',(-5.71972168400006,11.6,9.65904755899999));
#236618=CARTESIAN_POINT('Ctrl Pts',(-5.71926088000006,15.2,9.65563950599999));
#236619=CARTESIAN_POINT('Ctrl Pts',(-5.71926088000006,11.6,9.65563950599999));
#236620=CARTESIAN_POINT('Ctrl Pts',(-5.71879804600006,15.2,9.65223659799998));
#236621=CARTESIAN_POINT('Ctrl Pts',(-5.71879804600006,11.6,9.65223659799998));
#236622=CARTESIAN_POINT('Ctrl Pts',(-5.71833319100006,15.2,9.64883884499999));
#236623=CARTESIAN_POINT('Ctrl Pts',(-5.71833319100006,11.6,9.64883884499999));
#236624=CARTESIAN_POINT('Ctrl Pts',(-5.71786631900006,15.2,9.64544625299999));
#236625=CARTESIAN_POINT('Ctrl Pts',(-5.71786631900006,11.6,9.64544625299999));
#236626=CARTESIAN_POINT('Ctrl Pts',(-5.71739744200006,15.2,9.64205882999998));
#236627=CARTESIAN_POINT('Ctrl Pts',(-5.71739744200006,11.6,9.64205882999998));
#236628=CARTESIAN_POINT('Ctrl Pts',(-5.71692656400006,15.2,9.63867658199998));
#236629=CARTESIAN_POINT('Ctrl Pts',(-5.71692656400006,11.6,9.63867658199998));
#236630=CARTESIAN_POINT('Ctrl Pts',(-5.71645369500006,15.2,9.63529951699999));
#236631=CARTESIAN_POINT('Ctrl Pts',(-5.71645369500006,11.6,9.63529951699999));
#236632=CARTESIAN_POINT('Ctrl Pts',(-5.71597884000006,15.2,9.63192764199999));
#236633=CARTESIAN_POINT('Ctrl Pts',(-5.71597884000006,11.6,9.63192764199999));
#236634=CARTESIAN_POINT('Ctrl Pts',(-5.71550200800006,15.2,9.62856096299999));
#236635=CARTESIAN_POINT('Ctrl Pts',(-5.71550200800006,11.6,9.62856096299999));
#236636=CARTESIAN_POINT('Ctrl Pts',(-5.71502320600006,15.2,9.62519948899999));
#236637=CARTESIAN_POINT('Ctrl Pts',(-5.71502320600006,11.6,9.62519948899999));
#236638=CARTESIAN_POINT('Ctrl Pts',(-5.71454244100006,15.2,9.62184322599999));
#236639=CARTESIAN_POINT('Ctrl Pts',(-5.71454244100006,11.6,9.62184322599999));
#236640=CARTESIAN_POINT('Ctrl Pts',(-5.71405972300006,15.2,9.61849218099999));
#236641=CARTESIAN_POINT('Ctrl Pts',(-5.71405972300006,11.6,9.61849218099999));
#236642=CARTESIAN_POINT('Ctrl Pts',(-5.71357505700006,15.2,9.61514635999999));
#236643=CARTESIAN_POINT('Ctrl Pts',(-5.71357505700006,11.6,9.61514635999999));
#236644=CARTESIAN_POINT('Ctrl Pts',(-5.71308845100006,15.2,9.61180577299999));
#236645=CARTESIAN_POINT('Ctrl Pts',(-5.71308845100006,11.6,9.61180577299999));
#236646=CARTESIAN_POINT('Ctrl Pts',(-5.71259991400006,15.2,9.60847042699999));
#236647=CARTESIAN_POINT('Ctrl Pts',(-5.71259991400006,11.6,9.60847042699999));
#236648=CARTESIAN_POINT('Ctrl Pts',(-5.71210945300006,15.2,9.60514032599999));
#236649=CARTESIAN_POINT('Ctrl Pts',(-5.71210945300006,11.6,9.60514032599999));
#236650=CARTESIAN_POINT('Ctrl Pts',(-5.71161707500006,15.2,9.60181547999999));
#236651=CARTESIAN_POINT('Ctrl Pts',(-5.71161707500006,11.6,9.60181547999999));
#236652=CARTESIAN_POINT('Ctrl Pts',(-5.71112278800006,15.2,9.59849589599998));
#236653=CARTESIAN_POINT('Ctrl Pts',(-5.71112278800006,11.6,9.59849589599998));
#236654=CARTESIAN_POINT('Ctrl Pts',(-5.71062660000006,15.2,9.59518157899998));
#236655=CARTESIAN_POINT('Ctrl Pts',(-5.71062660000006,11.6,9.59518157899998));
#236656=CARTESIAN_POINT('Ctrl Pts',(-5.71012851900006,15.2,9.59187253999998));
#236657=CARTESIAN_POINT('Ctrl Pts',(-5.71012851900006,11.6,9.59187253999998));
#236658=CARTESIAN_POINT('Ctrl Pts',(-5.70962855200006,15.2,9.58856878299999));
#236659=CARTESIAN_POINT('Ctrl Pts',(-5.70962855200006,11.6,9.58856878299999));
#236660=CARTESIAN_POINT('Ctrl Pts',(-5.70912670800006,15.2,9.58527031499998));
#236661=CARTESIAN_POINT('Ctrl Pts',(-5.70912670800006,11.6,9.58527031499998));
#236662=CARTESIAN_POINT('Ctrl Pts',(-5.70862299300006,15.2,9.58197714699999));
#236663=CARTESIAN_POINT('Ctrl Pts',(-5.70862299300006,11.6,9.58197714699999));
#236664=CARTESIAN_POINT('Ctrl Pts',(-5.70811741600005,15.2,9.57868928199998));
#236665=CARTESIAN_POINT('Ctrl Pts',(-5.70811741600005,11.6,9.57868928199998));
#236666=CARTESIAN_POINT('Ctrl Pts',(-5.70760998500006,15.2,9.57540672899999));
#236667=CARTESIAN_POINT('Ctrl Pts',(-5.70760998500006,11.6,9.57540672899999));
#236668=CARTESIAN_POINT('Ctrl Pts',(-5.70710070700006,15.2,9.57212949599998));
#236669=CARTESIAN_POINT('Ctrl Pts',(-5.70710070700006,11.6,9.57212949599998));
#236670=CARTESIAN_POINT('Ctrl Pts',(-5.70658959100006,15.2,9.56885758899999));
#236671=CARTESIAN_POINT('Ctrl Pts',(-5.70658959100006,11.6,9.56885758899999));
#236672=CARTESIAN_POINT('Ctrl Pts',(-5.70607664400006,15.2,9.56559101699998));
#236673=CARTESIAN_POINT('Ctrl Pts',(-5.70607664400006,11.6,9.56559101699998));
#236674=CARTESIAN_POINT('Ctrl Pts',(-5.70556187300006,15.2,9.56232978499998));
#236675=CARTESIAN_POINT('Ctrl Pts',(-5.70556187300006,11.6,9.56232978499998));
#236676=CARTESIAN_POINT('Ctrl Pts',(-5.70504528900006,15.2,9.55907390199998));
#236677=CARTESIAN_POINT('Ctrl Pts',(-5.70504528900006,11.6,9.55907390199998));
#236678=CARTESIAN_POINT('Ctrl Pts',(-5.70452689700006,15.2,9.55582337399999));
#236679=CARTESIAN_POINT('Ctrl Pts',(-5.70452689700006,11.6,9.55582337399999));
#236680=CARTESIAN_POINT('Ctrl Pts',(-5.70400670700006,15.2,9.55257820999999));
#236681=CARTESIAN_POINT('Ctrl Pts',(-5.70400670700006,11.6,9.55257820999999));
#236682=CARTESIAN_POINT('Ctrl Pts',(-5.70348472500006,15.2,9.54933841599999));
#236683=CARTESIAN_POINT('Ctrl Pts',(-5.70348472500006,11.6,9.54933841599999));
#236684=CARTESIAN_POINT('Ctrl Pts',(-5.70296096200006,15.2,9.54610399999999));
#236685=CARTESIAN_POINT('Ctrl Pts',(-5.70296096200006,11.6,9.54610399999999));
#236686=CARTESIAN_POINT('Ctrl Pts',(-5.70243542200005,15.2,9.54287496899998));
#236687=CARTESIAN_POINT('Ctrl Pts',(-5.70243542200005,11.6,9.54287496899998));
#236688=CARTESIAN_POINT('Ctrl Pts',(-5.70190811700006,15.2,9.53965132899998));
#236689=CARTESIAN_POINT('Ctrl Pts',(-5.70190811700006,11.6,9.53965132899998));
#236690=CARTESIAN_POINT('Ctrl Pts',(-5.70137905300006,15.2,9.53643308999998));
#236691=CARTESIAN_POINT('Ctrl Pts',(-5.70137905300006,11.6,9.53643308999998));
#236692=CARTESIAN_POINT('Ctrl Pts',(-5.70084823800006,15.2,9.53322025799999));
#236693=CARTESIAN_POINT('Ctrl Pts',(-5.70084823800006,11.6,9.53322025799999));
#236694=CARTESIAN_POINT('Ctrl Pts',(-5.70031568100006,15.2,9.53001284099999));
#236695=CARTESIAN_POINT('Ctrl Pts',(-5.70031568100006,11.6,9.53001284099999));
#236696=CARTESIAN_POINT('Ctrl Pts',(-5.69978139000006,15.2,9.52681084599998));
#236697=CARTESIAN_POINT('Ctrl Pts',(-5.69978139000006,11.6,9.52681084599998));
#236698=CARTESIAN_POINT('Ctrl Pts',(-5.69924537300006,15.2,9.52361427899999));
#236699=CARTESIAN_POINT('Ctrl Pts',(-5.69924537300006,11.6,9.52361427899999));
#236700=CARTESIAN_POINT('Ctrl Pts',(-5.69870763900005,15.2,9.52042314999998));
#236701=CARTESIAN_POINT('Ctrl Pts',(-5.69870763900005,11.6,9.52042314999998));
#236702=CARTESIAN_POINT('Ctrl Pts',(-5.69816819400006,15.2,9.51723746499999));
#236703=CARTESIAN_POINT('Ctrl Pts',(-5.69816819400006,11.6,9.51723746499999));
#236704=CARTESIAN_POINT('Ctrl Pts',(-5.69762704900006,15.2,9.51405723099998));
#236705=CARTESIAN_POINT('Ctrl Pts',(-5.69762704900006,11.6,9.51405723099998));
#236706=CARTESIAN_POINT('Ctrl Pts',(-5.69708421000006,15.2,9.51088245499999));
#236707=CARTESIAN_POINT('Ctrl Pts',(-5.69708421000006,11.6,9.51088245499999));
#236708=CARTESIAN_POINT('Ctrl Pts',(-5.69653968800006,15.2,9.50771314699999));
#236709=CARTESIAN_POINT('Ctrl Pts',(-5.69653968800006,11.6,9.50771314699999));
#236710=CARTESIAN_POINT('Ctrl Pts',(-5.69599348800006,15.2,9.50454931199998));
#236711=CARTESIAN_POINT('Ctrl Pts',(-5.69599348800006,11.6,9.50454931199998));
#236712=CARTESIAN_POINT('Ctrl Pts',(-5.69544562100006,15.2,9.50139095799998));
#236713=CARTESIAN_POINT('Ctrl Pts',(-5.69544562100006,11.6,9.50139095799998));
#236714=CARTESIAN_POINT('Ctrl Pts',(-5.69489609500006,15.2,9.49823809399999));
#236715=CARTESIAN_POINT('Ctrl Pts',(-5.69489609500006,11.6,9.49823809399999));
#236716=CARTESIAN_POINT('Ctrl Pts',(-5.69434491600005,15.2,9.49509072499998));
#236717=CARTESIAN_POINT('Ctrl Pts',(-5.69434491600005,11.6,9.49509072499998));
#236718=CARTESIAN_POINT('Ctrl Pts',(-5.69379209600006,15.2,9.49194885999999));
#236719=CARTESIAN_POINT('Ctrl Pts',(-5.69379209600006,11.6,9.49194885999999));
#236720=CARTESIAN_POINT('Ctrl Pts',(-5.69323764100006,15.2,9.48881250699999));
#236721=CARTESIAN_POINT('Ctrl Pts',(-5.69323764100006,11.6,9.48881250699999));
#236722=CARTESIAN_POINT('Ctrl Pts',(-5.69268155900006,15.2,9.48568167099998));
#236723=CARTESIAN_POINT('Ctrl Pts',(-5.69268155900006,11.6,9.48568167099998));
#236724=CARTESIAN_POINT('Ctrl Pts',(-5.69212386100006,15.2,9.48255636199999));
#236725=CARTESIAN_POINT('Ctrl Pts',(-5.69212386100006,11.6,9.48255636199999));
#236726=CARTESIAN_POINT('Ctrl Pts',(-5.69156455400006,15.2,9.47943658699998));
#236727=CARTESIAN_POINT('Ctrl Pts',(-5.69156455400006,11.6,9.47943658699998));
#236728=CARTESIAN_POINT('Ctrl Pts',(-5.69100364700006,15.2,9.47632235299999));
#236729=CARTESIAN_POINT('Ctrl Pts',(-5.69100364700006,11.6,9.47632235299999));
#236730=CARTESIAN_POINT('Ctrl Pts',(-5.69044114800006,15.2,9.47321366899999));
#236731=CARTESIAN_POINT('Ctrl Pts',(-5.69044114800006,11.6,9.47321366899999));
#236732=CARTESIAN_POINT('Ctrl Pts',(-5.68987706600006,15.2,9.47011053899999));
#236733=CARTESIAN_POINT('Ctrl Pts',(-5.68987706600006,11.6,9.47011053899999));
#236734=CARTESIAN_POINT('Ctrl Pts',(-5.68931140900006,15.2,9.46701297399999));
#236735=CARTESIAN_POINT('Ctrl Pts',(-5.68931140900006,11.6,9.46701297399999));
#236736=CARTESIAN_POINT('Ctrl Pts',(-5.68874418700006,15.2,9.46392098099999));
#236737=CARTESIAN_POINT('Ctrl Pts',(-5.68874418700006,11.6,9.46392098099999));
#236738=CARTESIAN_POINT('Ctrl Pts',(-5.68817540700006,15.2,9.46083456599998));
#236739=CARTESIAN_POINT('Ctrl Pts',(-5.68817540700006,11.6,9.46083456599998));
#236740=CARTESIAN_POINT('Ctrl Pts',(-5.68760507800006,15.2,9.45775373799999));
#236741=CARTESIAN_POINT('Ctrl Pts',(-5.68760507800006,11.6,9.45775373799999));
#236742=CARTESIAN_POINT('Ctrl Pts',(-5.68703321000006,15.2,9.45467850399999));
#236743=CARTESIAN_POINT('Ctrl Pts',(-5.68703321000006,11.6,9.45467850399999));
#236744=CARTESIAN_POINT('Ctrl Pts',(-5.68645981100006,15.2,9.45160887199999));
#236745=CARTESIAN_POINT('Ctrl Pts',(-5.68645981100006,11.6,9.45160887199999));
#236746=CARTESIAN_POINT('Ctrl Pts',(-5.68588489000006,15.2,9.44854484899999));
#236747=CARTESIAN_POINT('Ctrl Pts',(-5.68588489000006,11.6,9.44854484899999));
#236748=CARTESIAN_POINT('Ctrl Pts',(-5.68530845500006,15.2,9.44548644399998));
#236749=CARTESIAN_POINT('Ctrl Pts',(-5.68530845500006,11.6,9.44548644399998));
#236750=CARTESIAN_POINT('Ctrl Pts',(-5.68473051600006,15.2,9.44243366199998));
#236751=CARTESIAN_POINT('Ctrl Pts',(-5.68473051600006,11.6,9.44243366199998));
#236752=CARTESIAN_POINT('Ctrl Pts',(-5.68415108000006,15.2,9.43938651299998));
#236753=CARTESIAN_POINT('Ctrl Pts',(-5.68415108000006,11.6,9.43938651299998));
#236754=CARTESIAN_POINT('Ctrl Pts',(-5.68357015700006,15.2,9.43634500399998));
#236755=CARTESIAN_POINT('Ctrl Pts',(-5.68357015700006,11.6,9.43634500399998));
#236756=CARTESIAN_POINT('Ctrl Pts',(-5.68298775600006,15.2,9.43330914299998));
#236757=CARTESIAN_POINT('Ctrl Pts',(-5.68298775600006,11.6,9.43330914299998));
#236758=CARTESIAN_POINT('Ctrl Pts',(-5.68240388700006,15.2,9.43027893699998));
#236759=CARTESIAN_POINT('Ctrl Pts',(-5.68240388700006,11.6,9.43027893699998));
#236760=CARTESIAN_POINT('Ctrl Pts',(-5.68181855600006,15.2,9.42725439299998));
#236761=CARTESIAN_POINT('Ctrl Pts',(-5.68181855600006,11.6,9.42725439299998));
#236762=CARTESIAN_POINT('Ctrl Pts',(-5.68123177500006,15.2,9.42423552099999));
#236763=CARTESIAN_POINT('Ctrl Pts',(-5.68123177500006,11.6,9.42423552099999));
#236764=CARTESIAN_POINT('Ctrl Pts',(-5.68064355000006,15.2,9.42122232699998));
#236765=CARTESIAN_POINT('Ctrl Pts',(-5.68064355000006,11.6,9.42122232699998));
#236766=CARTESIAN_POINT('Ctrl Pts',(-5.68005389300006,15.2,9.41821481799998));
#236767=CARTESIAN_POINT('Ctrl Pts',(-5.68005389300006,11.6,9.41821481799998));
#236768=CARTESIAN_POINT('Ctrl Pts',(-5.67946281200006,15.2,9.41521300399998));
#236769=CARTESIAN_POINT('Ctrl Pts',(-5.67946281200006,11.6,9.41521300399998));
#236770=CARTESIAN_POINT('Ctrl Pts',(-5.67887031500006,15.2,9.41221689099999));
#236771=CARTESIAN_POINT('Ctrl Pts',(-5.67887031500006,11.6,9.41221689099999));
#236772=CARTESIAN_POINT('Ctrl Pts',(-5.67827641300005,15.2,9.40922648699999));
#236773=CARTESIAN_POINT('Ctrl Pts',(-5.67827641300005,11.6,9.40922648699999));
#236774=CARTESIAN_POINT('Ctrl Pts',(-5.67768111200006,15.2,9.40624179999999));
#236775=CARTESIAN_POINT('Ctrl Pts',(-5.67768111200006,11.6,9.40624179999999));
#236776=CARTESIAN_POINT('Ctrl Pts',(-5.67708442500006,15.2,9.40326283799998));
#236777=CARTESIAN_POINT('Ctrl Pts',(-5.67708442500006,11.6,9.40326283799998));
#236778=CARTESIAN_POINT('Ctrl Pts',(-5.67648635800006,15.2,9.40028960799999));
#236779=CARTESIAN_POINT('Ctrl Pts',(-5.67648635800006,11.6,9.40028960799999));
#236780=CARTESIAN_POINT('Ctrl Pts',(-5.67588692200006,15.2,9.39732211899998));
#236781=CARTESIAN_POINT('Ctrl Pts',(-5.67588692200006,11.6,9.39732211899998));
#236782=CARTESIAN_POINT('Ctrl Pts',(-5.67528612600006,15.2,9.39436037699998));
#236783=CARTESIAN_POINT('Ctrl Pts',(-5.67528612600006,11.6,9.39436037699998));
#236784=CARTESIAN_POINT('Ctrl Pts',(-5.67468397900006,15.2,9.39140439199999));
#236785=CARTESIAN_POINT('Ctrl Pts',(-5.67468397900006,11.6,9.39140439199999));
#236786=CARTESIAN_POINT('Ctrl Pts',(-5.67408048900006,15.2,9.38845416899999));
#236787=CARTESIAN_POINT('Ctrl Pts',(-5.67408048900006,11.6,9.38845416899999));
#236788=CARTESIAN_POINT('Ctrl Pts',(-5.67347566800006,15.2,9.38550971899998));
#236789=CARTESIAN_POINT('Ctrl Pts',(-5.67347566800006,11.6,9.38550971899998));
#236790=CARTESIAN_POINT('Ctrl Pts',(-5.67286952300006,15.2,9.38257104699998));
#236791=CARTESIAN_POINT('Ctrl Pts',(-5.67286952300006,11.6,9.38257104699998));
#236792=CARTESIAN_POINT('Ctrl Pts',(-5.67226206500006,15.2,9.37963816299998));
#236793=CARTESIAN_POINT('Ctrl Pts',(-5.67226206500006,11.6,9.37963816299998));
#236794=CARTESIAN_POINT('Ctrl Pts',(-5.67165330200006,15.2,9.37671107499998));
#236795=CARTESIAN_POINT('Ctrl Pts',(-5.67165330200006,11.6,9.37671107499998));
#236796=CARTESIAN_POINT('Ctrl Pts',(-5.67104324500006,15.2,9.37378978899999));
#236797=CARTESIAN_POINT('Ctrl Pts',(-5.67104324500006,11.6,9.37378978899999));
#236798=CARTESIAN_POINT('Ctrl Pts',(-5.67043190200006,15.2,9.37087431299998));
#236799=CARTESIAN_POINT('Ctrl Pts',(-5.67043190200006,11.6,9.37087431299998));
#236800=CARTESIAN_POINT('Ctrl Pts',(-5.66981928200006,15.2,9.36796465599999));
#236801=CARTESIAN_POINT('Ctrl Pts',(-5.66981928200006,11.6,9.36796465599999));
#236802=CARTESIAN_POINT('Ctrl Pts',(-5.66920539700006,15.2,9.36506082599998));
#236803=CARTESIAN_POINT('Ctrl Pts',(-5.66920539700006,11.6,9.36506082599998));
#236804=CARTESIAN_POINT('Ctrl Pts',(-5.66859025400006,15.2,9.36216282899998));
#236805=CARTESIAN_POINT('Ctrl Pts',(-5.66859025400006,11.6,9.36216282899998));
#236806=CARTESIAN_POINT('Ctrl Pts',(-5.66797386300006,15.2,9.35927067599999));
#236807=CARTESIAN_POINT('Ctrl Pts',(-5.66797386300006,11.6,9.35927067599999));
#236808=CARTESIAN_POINT('Ctrl Pts',(-5.66735623500006,15.2,9.35638437199999));
#236809=CARTESIAN_POINT('Ctrl Pts',(-5.66735623500006,11.6,9.35638437199999));
#236810=CARTESIAN_POINT('Ctrl Pts',(-5.66673737800006,15.2,9.35350392799998));
#236811=CARTESIAN_POINT('Ctrl Pts',(-5.66673737800006,11.6,9.35350392799998));
#236812=CARTESIAN_POINT('Ctrl Pts',(-5.66611730300006,15.2,9.35062934799999));
#236813=CARTESIAN_POINT('Ctrl Pts',(-5.66611730300006,11.6,9.35062934799999));
#236814=CARTESIAN_POINT('Ctrl Pts',(-5.66549601900006,15.2,9.34776064299999));
#236815=CARTESIAN_POINT('Ctrl Pts',(-5.66549601900006,11.6,9.34776064299999));
#236816=CARTESIAN_POINT('Ctrl Pts',(-5.66487353500006,15.2,9.34489782099998));
#236817=CARTESIAN_POINT('Ctrl Pts',(-5.66487353500006,11.6,9.34489782099998));
#236818=CARTESIAN_POINT('Ctrl Pts',(-5.66424986200006,15.2,9.34204088699998));
#236819=CARTESIAN_POINT('Ctrl Pts',(-5.66424986200006,11.6,9.34204088699998));
#236820=CARTESIAN_POINT('Ctrl Pts',(-5.66362500900006,15.2,9.33918985199998));
#236821=CARTESIAN_POINT('Ctrl Pts',(-5.66362500900006,11.6,9.33918985199998));
#236822=CARTESIAN_POINT('Ctrl Pts',(-5.66299898600006,15.2,9.33634472299998));
#236823=CARTESIAN_POINT('Ctrl Pts',(-5.66299898600006,11.6,9.33634472299998));
#236824=CARTESIAN_POINT('Ctrl Pts',(-5.66237180200006,15.2,9.33350550899998));
#236825=CARTESIAN_POINT('Ctrl Pts',(-5.66237180200006,11.6,9.33350550899998));
#236826=CARTESIAN_POINT('Ctrl Pts',(-5.66174346800006,15.2,9.33067221699999));
#236827=CARTESIAN_POINT('Ctrl Pts',(-5.66174346800006,11.6,9.33067221699999));
#236828=CARTESIAN_POINT('Ctrl Pts',(-5.66111399400006,15.2,9.32784485499998));
#236829=CARTESIAN_POINT('Ctrl Pts',(-5.66111399400006,11.6,9.32784485499998));
#236830=CARTESIAN_POINT('Ctrl Pts',(-5.66048338800006,15.2,9.32502342999998));
#236831=CARTESIAN_POINT('Ctrl Pts',(-5.66048338800006,11.6,9.32502342999998));
#236832=CARTESIAN_POINT('Ctrl Pts',(-5.65985166300006,15.2,9.32220795299998));
#236833=CARTESIAN_POINT('Ctrl Pts',(-5.65985166300006,11.6,9.32220795299998));
#236834=CARTESIAN_POINT('Ctrl Pts',(-5.65921882600006,15.2,9.31939842899999));
#236835=CARTESIAN_POINT('Ctrl Pts',(-5.65921882600006,11.6,9.31939842899999));
#236836=CARTESIAN_POINT('Ctrl Pts',(-5.65858488900005,15.2,9.31659486699999));
#236837=CARTESIAN_POINT('Ctrl Pts',(-5.65858488900005,11.6,9.31659486699999));
#236838=CARTESIAN_POINT('Ctrl Pts',(-5.65794986000006,15.2,9.31379727699999));
#236839=CARTESIAN_POINT('Ctrl Pts',(-5.65794986000006,11.6,9.31379727699999));
#236840=CARTESIAN_POINT('Ctrl Pts',(-5.65731375200006,15.2,9.31100566499998));
#236841=CARTESIAN_POINT('Ctrl Pts',(-5.65731375200006,11.6,9.31100566499998));
#236842=CARTESIAN_POINT('Ctrl Pts',(-5.65667657200006,15.2,9.30822003899999));
#236843=CARTESIAN_POINT('Ctrl Pts',(-5.65667657200006,11.6,9.30822003899999));
#236844=CARTESIAN_POINT('Ctrl Pts',(-5.65603833200006,15.2,9.30544040799998));
#236845=CARTESIAN_POINT('Ctrl Pts',(-5.65603833200006,11.6,9.30544040799998));
#236846=CARTESIAN_POINT('Ctrl Pts',(-5.65539904000006,15.2,9.30266678099999));
#236847=CARTESIAN_POINT('Ctrl Pts',(-5.65539904000006,11.6,9.30266678099999));
#236848=CARTESIAN_POINT('Ctrl Pts',(-5.65475870900006,15.2,9.29989916499999));
#236849=CARTESIAN_POINT('Ctrl Pts',(-5.65475870900006,11.6,9.29989916499999));
#236850=CARTESIAN_POINT('Ctrl Pts',(-5.65411734800006,15.2,9.29713756699999));
#236851=CARTESIAN_POINT('Ctrl Pts',(-5.65411734800006,11.6,9.29713756699999));
#236852=CARTESIAN_POINT('Ctrl Pts',(-5.65347496700006,15.2,9.29438199899998));
#236853=CARTESIAN_POINT('Ctrl Pts',(-5.65347496700006,11.6,9.29438199899998));
#236854=CARTESIAN_POINT('Ctrl Pts',(-5.65283157700006,15.2,9.29163246499999));
#236855=CARTESIAN_POINT('Ctrl Pts',(-5.65283157700006,11.6,9.29163246499999));
#236856=CARTESIAN_POINT('Ctrl Pts',(-5.65218718700006,15.2,9.28888897499998));
#236857=CARTESIAN_POINT('Ctrl Pts',(-5.65218718700006,11.6,9.28888897499998));
#236858=CARTESIAN_POINT('Ctrl Pts',(-5.65154180700006,15.2,9.28615153699998));
#236859=CARTESIAN_POINT('Ctrl Pts',(-5.65154180700006,11.6,9.28615153699998));
#236860=CARTESIAN_POINT('Ctrl Pts',(-5.65089545000006,15.2,9.28342015999998));
#236861=CARTESIAN_POINT('Ctrl Pts',(-5.65089545000006,11.6,9.28342015999998));
#236862=CARTESIAN_POINT('Ctrl Pts',(-5.65024812400006,15.2,9.28069485099999));
#236863=CARTESIAN_POINT('Ctrl Pts',(-5.65024812400006,11.6,9.28069485099999));
#236864=CARTESIAN_POINT('Ctrl Pts',(-5.64959984100006,15.2,9.27797561899999));
#236865=CARTESIAN_POINT('Ctrl Pts',(-5.64959984100006,11.6,9.27797561899999));
#236866=CARTESIAN_POINT('Ctrl Pts',(-5.64895061000006,15.2,9.27526247199999));
#236867=CARTESIAN_POINT('Ctrl Pts',(-5.64895061000006,11.6,9.27526247199999));
#236868=CARTESIAN_POINT('Ctrl Pts',(-5.64830044100006,15.2,9.27255541899999));
#236869=CARTESIAN_POINT('Ctrl Pts',(-5.64830044100006,11.6,9.27255541899999));
#236870=CARTESIAN_POINT('Ctrl Pts',(-5.64764934600006,15.2,9.26985446699998));
#236871=CARTESIAN_POINT('Ctrl Pts',(-5.64764934600006,11.6,9.26985446699998));
#236872=CARTESIAN_POINT('Ctrl Pts',(-5.64699733600006,15.2,9.26715962499999));
#236873=CARTESIAN_POINT('Ctrl Pts',(-5.64699733600006,11.6,9.26715962499999));
#236874=CARTESIAN_POINT('Ctrl Pts',(-5.64634442000005,15.2,9.26447090199999));
#236875=CARTESIAN_POINT('Ctrl Pts',(-5.64634442000005,11.6,9.26447090199999));
#236876=CARTESIAN_POINT('Ctrl Pts',(-5.64569060900006,15.2,9.26178830599999));
#236877=CARTESIAN_POINT('Ctrl Pts',(-5.64569060900006,11.6,9.26178830599999));
#236878=CARTESIAN_POINT('Ctrl Pts',(-5.64503591600006,15.2,9.25911184399999));
#236879=CARTESIAN_POINT('Ctrl Pts',(-5.64503591600006,11.6,9.25911184399999));
#236880=CARTESIAN_POINT('Ctrl Pts',(-5.64438034700006,15.2,9.25644152499999));
#236881=CARTESIAN_POINT('Ctrl Pts',(-5.64438034700006,11.6,9.25644152499999));
#236882=CARTESIAN_POINT('Ctrl Pts',(-5.64372391600005,15.2,9.25377735799999));
#236883=CARTESIAN_POINT('Ctrl Pts',(-5.64372391600005,11.6,9.25377735799999));
#236884=CARTESIAN_POINT('Ctrl Pts',(-5.64306663300005,15.2,9.25111935199999));
#236885=CARTESIAN_POINT('Ctrl Pts',(-5.64306663300005,11.6,9.25111935199999));
#236886=CARTESIAN_POINT('Ctrl Pts',(-5.64240850900006,15.2,9.24846751399999));
#236887=CARTESIAN_POINT('Ctrl Pts',(-5.64240850900006,11.6,9.24846751399999));
#236888=CARTESIAN_POINT('Ctrl Pts',(-5.64174955500006,15.2,9.24582185199998));
#236889=CARTESIAN_POINT('Ctrl Pts',(-5.64174955500006,11.6,9.24582185199998));
#236890=CARTESIAN_POINT('Ctrl Pts',(-5.64108978100006,15.2,9.24318237599999));
#236891=CARTESIAN_POINT('Ctrl Pts',(-5.64108978100006,11.6,9.24318237599999));
#236892=CARTESIAN_POINT('Ctrl Pts',(-5.64042919800006,15.2,9.24054909399998));
#236893=CARTESIAN_POINT('Ctrl Pts',(-5.64042919800006,11.6,9.24054909399998));
#236894=CARTESIAN_POINT('Ctrl Pts',(-5.63976781800006,15.2,9.23792201399999));
#236895=CARTESIAN_POINT('Ctrl Pts',(-5.63976781800006,11.6,9.23792201399999));
#236896=CARTESIAN_POINT('Ctrl Pts',(-5.63910565000006,15.2,9.23530114499999));
#236897=CARTESIAN_POINT('Ctrl Pts',(-5.63910565000006,11.6,9.23530114499999));
#236898=CARTESIAN_POINT('Ctrl Pts',(-5.63844270700006,15.2,9.23268649399999));
#236899=CARTESIAN_POINT('Ctrl Pts',(-5.63844270700006,11.6,9.23268649399999));
#236900=CARTESIAN_POINT('Ctrl Pts',(-5.63777899900006,15.2,9.23007807199999));
#236901=CARTESIAN_POINT('Ctrl Pts',(-5.63777899900006,11.6,9.23007807199999));
#236902=CARTESIAN_POINT('Ctrl Pts',(-5.63711453700006,15.2,9.22747588499998));
#236903=CARTESIAN_POINT('Ctrl Pts',(-5.63711453700006,11.6,9.22747588499998));
#236904=CARTESIAN_POINT('Ctrl Pts',(-5.63644933200006,15.2,9.22487994299999));
#236905=CARTESIAN_POINT('Ctrl Pts',(-5.63644933200006,11.6,9.22487994299999));
#236906=CARTESIAN_POINT('Ctrl Pts',(-5.63578339500006,15.2,9.22229025499998));
#236907=CARTESIAN_POINT('Ctrl Pts',(-5.63578339500006,11.6,9.22229025499998));
#236908=CARTESIAN_POINT('Ctrl Pts',(-5.63511673800006,15.2,9.21970682799999));
#236909=CARTESIAN_POINT('Ctrl Pts',(-5.63511673800006,11.6,9.21970682799999));
#236910=CARTESIAN_POINT('Ctrl Pts',(-5.63444937200006,15.2,9.21712967099998));
#236911=CARTESIAN_POINT('Ctrl Pts',(-5.63444937200006,11.6,9.21712967099998));
#236912=CARTESIAN_POINT('Ctrl Pts',(-5.63378130700006,15.2,9.21455879299998));
#236913=CARTESIAN_POINT('Ctrl Pts',(-5.63378130700006,11.6,9.21455879299998));
#236914=CARTESIAN_POINT('Ctrl Pts',(-5.63311255600006,15.2,9.21199420299999));
#236915=CARTESIAN_POINT('Ctrl Pts',(-5.63311255600006,11.6,9.21199420299999));
#236916=CARTESIAN_POINT('Ctrl Pts',(-5.63244312900006,15.2,9.20943590799999));
#236917=CARTESIAN_POINT('Ctrl Pts',(-5.63244312900006,11.6,9.20943590799999));
#236918=CARTESIAN_POINT('Ctrl Pts',(-5.63177303700006,15.2,9.20688391799998));
#236919=CARTESIAN_POINT('Ctrl Pts',(-5.63177303700006,11.6,9.20688391799998));
#236920=CARTESIAN_POINT('Ctrl Pts',(-5.63110229300006,15.2,9.20433824199998));
#236921=CARTESIAN_POINT('Ctrl Pts',(-5.63110229300006,11.6,9.20433824199998));
#236922=CARTESIAN_POINT('Ctrl Pts',(-5.63043090700006,15.2,9.20179888799998));
#236923=CARTESIAN_POINT('Ctrl Pts',(-5.63043090700006,11.6,9.20179888799998));
#236924=CARTESIAN_POINT('Ctrl Pts',(-5.62975889100006,15.2,9.19926586199999));
#236925=CARTESIAN_POINT('Ctrl Pts',(-5.62975889100006,11.6,9.19926586199999));
#236926=CARTESIAN_POINT('Ctrl Pts',(-5.62908625600006,15.2,9.19673917799999));
#236927=CARTESIAN_POINT('Ctrl Pts',(-5.62908625600006,11.6,9.19673917799999));
#236928=CARTESIAN_POINT('Ctrl Pts',(-5.62841301500006,15.2,9.19421884099999));
#236929=CARTESIAN_POINT('Ctrl Pts',(-5.62841301500006,11.6,9.19421884099999));
#236930=CARTESIAN_POINT('Ctrl Pts',(-5.62773917800006,15.2,9.19170486099999));
#236931=CARTESIAN_POINT('Ctrl Pts',(-5.62773917800006,11.6,9.19170486099999));
#236932=CARTESIAN_POINT('Ctrl Pts',(-5.62706475600006,15.2,9.18919724599998));
#236933=CARTESIAN_POINT('Ctrl Pts',(-5.62706475600006,11.6,9.18919724599998));
#236934=CARTESIAN_POINT('Ctrl Pts',(-5.62638976200006,15.2,9.18669600399999));
#236935=CARTESIAN_POINT('Ctrl Pts',(-5.62638976200006,11.6,9.18669600399999));
#236936=CARTESIAN_POINT('Ctrl Pts',(-5.62571420700006,15.2,9.18420114599999));
#236937=CARTESIAN_POINT('Ctrl Pts',(-5.62571420700006,11.6,9.18420114599999));
#236938=CARTESIAN_POINT('Ctrl Pts',(-5.62503810400006,15.2,9.18171267899999));
#236939=CARTESIAN_POINT('Ctrl Pts',(-5.62503810400006,11.6,9.18171267899999));
#236940=CARTESIAN_POINT('Ctrl Pts',(-5.62436146300006,15.2,9.17923061299999));
#236941=CARTESIAN_POINT('Ctrl Pts',(-5.62436146300006,11.6,9.17923061299999));
#236942=CARTESIAN_POINT('Ctrl Pts',(-5.62368429600006,15.2,9.17675495599998));
#236943=CARTESIAN_POINT('Ctrl Pts',(-5.62368429600006,11.6,9.17675495599998));
#236944=CARTESIAN_POINT('Ctrl Pts',(-5.62300661500006,15.2,9.17428571699999));
#236945=CARTESIAN_POINT('Ctrl Pts',(-5.62300661500006,11.6,9.17428571699999));
#236946=CARTESIAN_POINT('Ctrl Pts',(-5.62232843300006,15.2,9.17182290399998));
#236947=CARTESIAN_POINT('Ctrl Pts',(-5.62232843300006,11.6,9.17182290399998));
#236948=CARTESIAN_POINT('Ctrl Pts',(-5.62164976000005,15.2,9.16936652699999));
#236949=CARTESIAN_POINT('Ctrl Pts',(-5.62164976000005,11.6,9.16936652699999));
#236950=CARTESIAN_POINT('Ctrl Pts',(-5.62097061000006,15.2,9.16691659399999));
#236951=CARTESIAN_POINT('Ctrl Pts',(-5.62097061000006,11.6,9.16691659399999));
#236952=CARTESIAN_POINT('Ctrl Pts',(-5.62029099200006,15.2,9.16447311499999));
#236953=CARTESIAN_POINT('Ctrl Pts',(-5.62029099200006,11.6,9.16447311499999));
#236954=CARTESIAN_POINT('Ctrl Pts',(-5.61961092000006,15.2,9.16203609799998));
#236955=CARTESIAN_POINT('Ctrl Pts',(-5.61961092000006,11.6,9.16203609799998));
#236956=CARTESIAN_POINT('Ctrl Pts',(-5.61893040700006,15.2,9.15960555299998));
#236957=CARTESIAN_POINT('Ctrl Pts',(-5.61893040700006,11.6,9.15960555299998));
#236958=CARTESIAN_POINT('Ctrl Pts',(-5.61824946300006,15.2,9.15718148599998));
#236959=CARTESIAN_POINT('Ctrl Pts',(-5.61824946300006,11.6,9.15718148599998));
#236960=CARTESIAN_POINT('Ctrl Pts',(-5.61756810100006,15.2,9.15476390999999));
#236961=CARTESIAN_POINT('Ctrl Pts',(-5.61756810100006,11.6,9.15476390999999));
#236962=CARTESIAN_POINT('Ctrl Pts',(-5.61688633400006,15.2,9.15235282999999));
#236963=CARTESIAN_POINT('Ctrl Pts',(-5.61688633400006,11.6,9.15235282999999));
#236964=CARTESIAN_POINT('Ctrl Pts',(-5.61620417200006,15.2,9.14994825799998));
#236965=CARTESIAN_POINT('Ctrl Pts',(-5.61620417200006,11.6,9.14994825799998));
#236966=CARTESIAN_POINT('Ctrl Pts',(-5.61552163000006,15.2,9.14755020199999));
#236967=CARTESIAN_POINT('Ctrl Pts',(-5.61552163000006,11.6,9.14755020199999));
#236968=CARTESIAN_POINT('Ctrl Pts',(-5.61483871800006,15.2,9.14515866899999));
#236969=CARTESIAN_POINT('Ctrl Pts',(-5.61483871800006,11.6,9.14515866899999));
#236970=CARTESIAN_POINT('Ctrl Pts',(-5.61415544800006,15.2,9.14277367099999));
#236971=CARTESIAN_POINT('Ctrl Pts',(-5.61415544800006,11.6,9.14277367099999));
#236972=CARTESIAN_POINT('Ctrl Pts',(-5.61347183500006,15.2,9.14039521599998));
#236973=CARTESIAN_POINT('Ctrl Pts',(-5.61347183500006,11.6,9.14039521599998));
#236974=CARTESIAN_POINT('Ctrl Pts',(-5.61278788900006,15.2,9.13802331199999));
#236975=CARTESIAN_POINT('Ctrl Pts',(-5.61278788900006,11.6,9.13802331199999));
#236976=CARTESIAN_POINT('Ctrl Pts',(-5.61210362400006,15.2,9.13565796999999));
#236977=CARTESIAN_POINT('Ctrl Pts',(-5.61210362400006,11.6,9.13565796999999));
#236978=CARTESIAN_POINT('Ctrl Pts',(-5.61141905000006,15.2,9.13329919799999));
#236979=CARTESIAN_POINT('Ctrl Pts',(-5.61141905000006,11.6,9.13329919799999));
#236980=CARTESIAN_POINT('Ctrl Pts',(-5.61073418300006,15.2,9.13094700499999));
#236981=CARTESIAN_POINT('Ctrl Pts',(-5.61073418300006,11.6,9.13094700499999));
#236982=CARTESIAN_POINT('Ctrl Pts',(-5.61004903300006,15.2,9.12860139899998));
#236983=CARTESIAN_POINT('Ctrl Pts',(-5.61004903300006,11.6,9.12860139899998));
#236984=CARTESIAN_POINT('Ctrl Pts',(-5.60936361400006,15.2,9.12626239199999));
#236985=CARTESIAN_POINT('Ctrl Pts',(-5.60936361400006,11.6,9.12626239199999));
#236986=CARTESIAN_POINT('Ctrl Pts',(-5.60867793700006,15.2,9.12392998999999));
#236987=CARTESIAN_POINT('Ctrl Pts',(-5.60867793700006,11.6,9.12392998999999));
#236988=CARTESIAN_POINT('Ctrl Pts',(-5.60799201700006,15.2,9.12160420499998));
#236989=CARTESIAN_POINT('Ctrl Pts',(-5.60799201700006,11.6,9.12160420499998));
#236990=CARTESIAN_POINT('Ctrl Pts',(-5.60730586500005,15.2,9.11928504299999));
#236991=CARTESIAN_POINT('Ctrl Pts',(-5.60730586500005,11.6,9.11928504299999));
#236992=CARTESIAN_POINT('Ctrl Pts',(-5.60661949400005,15.2,9.11697251599998));
#236993=CARTESIAN_POINT('Ctrl Pts',(-5.60661949400005,11.6,9.11697251599998));
#236994=CARTESIAN_POINT('Ctrl Pts',(-5.60593291600005,15.2,9.11466663299999));
#236995=CARTESIAN_POINT('Ctrl Pts',(-5.60593291600005,11.6,9.11466663299999));
#236996=CARTESIAN_POINT('Ctrl Pts',(-5.60524614600006,15.2,9.11236740199998));
#236997=CARTESIAN_POINT('Ctrl Pts',(-5.60524614600006,11.6,9.11236740199998));
#236998=CARTESIAN_POINT('Ctrl Pts',(-5.60455919600006,15.2,9.11007483299999));
#236999=CARTESIAN_POINT('Ctrl Pts',(-5.60455919600006,11.6,9.11007483299999));
#237000=CARTESIAN_POINT('Ctrl Pts',(-5.60387207800006,15.2,9.10778893299998));
#237001=CARTESIAN_POINT('Ctrl Pts',(-5.60387207800006,11.6,9.10778893299998));
#237002=CARTESIAN_POINT('Ctrl Pts',(-5.60318480600006,15.2,9.10550971499998));
#237003=CARTESIAN_POINT('Ctrl Pts',(-5.60318480600006,11.6,9.10550971499998));
#237004=CARTESIAN_POINT('Ctrl Pts',(-5.60249739200006,15.2,9.10323718699999));
#237005=CARTESIAN_POINT('Ctrl Pts',(-5.60249739200006,11.6,9.10323718699999));
#237006=CARTESIAN_POINT('Ctrl Pts',(-5.60180985100006,15.2,9.10097135599998));
#237007=CARTESIAN_POINT('Ctrl Pts',(-5.60180985100006,11.6,9.10097135599998));
#237008=CARTESIAN_POINT('Ctrl Pts',(-5.60112219400006,15.2,9.09871223399998));
#237009=CARTESIAN_POINT('Ctrl Pts',(-5.60112219400006,11.6,9.09871223399998));
#237010=CARTESIAN_POINT('Ctrl Pts',(-5.60043443500006,15.2,9.09645982999999));
#237011=CARTESIAN_POINT('Ctrl Pts',(-5.60043443500006,11.6,9.09645982999999));
#237012=CARTESIAN_POINT('Ctrl Pts',(-5.59974658800006,15.2,9.09421415199999));
#237013=CARTESIAN_POINT('Ctrl Pts',(-5.59974658800006,11.6,9.09421415199999));
#237014=CARTESIAN_POINT('Ctrl Pts',(-5.59905866400006,15.2,9.09197521199999));
#237015=CARTESIAN_POINT('Ctrl Pts',(-5.59905866400006,11.6,9.09197521199999));
#237016=CARTESIAN_POINT('Ctrl Pts',(-5.59837067900006,15.2,9.08974301499999));
#237017=CARTESIAN_POINT('Ctrl Pts',(-5.59837067900006,11.6,9.08974301499999));
#237018=CARTESIAN_POINT('Ctrl Pts',(-5.59768264500006,15.2,9.08751757599998));
#237019=CARTESIAN_POINT('Ctrl Pts',(-5.59768264500006,11.6,9.08751757599998));
#237020=CARTESIAN_POINT('Ctrl Pts',(-5.59699457500006,15.2,9.08529889999999));
#237021=CARTESIAN_POINT('Ctrl Pts',(-5.59699457500006,11.6,9.08529889999999));
#237022=CARTESIAN_POINT('Ctrl Pts',(-5.59630648300006,15.2,9.08308699799999));
#237023=CARTESIAN_POINT('Ctrl Pts',(-5.59630648300006,11.6,9.08308699799999));
#237024=CARTESIAN_POINT('Ctrl Pts',(-5.59561838300006,15.2,9.08088187899999));
#237025=CARTESIAN_POINT('Ctrl Pts',(-5.59561838300006,11.6,9.08088187899999));
#237026=CARTESIAN_POINT('Ctrl Pts',(-5.59493028800006,15.2,9.07868355399999));
#237027=CARTESIAN_POINT('Ctrl Pts',(-5.59493028800006,11.6,9.07868355399999));
#237028=CARTESIAN_POINT('Ctrl Pts',(-5.59424221100006,15.2,9.07649203199998));
#237029=CARTESIAN_POINT('Ctrl Pts',(-5.59424221100006,11.6,9.07649203199998));
#237030=CARTESIAN_POINT('Ctrl Pts',(-5.59355416600006,15.2,9.07430732199998));
#237031=CARTESIAN_POINT('Ctrl Pts',(-5.59355416600006,11.6,9.07430732199998));
#237032=CARTESIAN_POINT('Ctrl Pts',(-5.59286616700006,15.2,9.07212943299999));
#237033=CARTESIAN_POINT('Ctrl Pts',(-5.59286616700006,11.6,9.07212943299999));
#237034=CARTESIAN_POINT('Ctrl Pts',(-5.59217822700006,15.2,9.06995837499998));
#237035=CARTESIAN_POINT('Ctrl Pts',(-5.59217822700006,11.6,9.06995837499998));
#237036=CARTESIAN_POINT('Ctrl Pts',(-5.59149036100006,15.2,9.06779415799999));
#237037=CARTESIAN_POINT('Ctrl Pts',(-5.59149036100006,11.6,9.06779415799999));
#237038=CARTESIAN_POINT('Ctrl Pts',(-5.59080258200006,15.2,9.06563679099998));
#237039=CARTESIAN_POINT('Ctrl Pts',(-5.59080258200006,11.6,9.06563679099998));
#237040=CARTESIAN_POINT('Ctrl Pts',(-5.59011490400006,15.2,9.06348628499998));
#237041=CARTESIAN_POINT('Ctrl Pts',(-5.59011490400006,11.6,9.06348628499998));
#237042=CARTESIAN_POINT('Ctrl Pts',(-5.58942734000006,15.2,9.06134264799999));
#237043=CARTESIAN_POINT('Ctrl Pts',(-5.58942734000006,11.6,9.06134264799999));
#237044=CARTESIAN_POINT('Ctrl Pts',(-5.58873990500006,15.2,9.05920589099999));
#237045=CARTESIAN_POINT('Ctrl Pts',(-5.58873990500006,11.6,9.05920589099999));
#237046=CARTESIAN_POINT('Ctrl Pts',(-5.58805261400006,15.2,9.05707602299999));
#237047=CARTESIAN_POINT('Ctrl Pts',(-5.58805261400006,11.6,9.05707602299999));
#237048=CARTESIAN_POINT('Ctrl Pts',(-5.58736547800006,15.2,9.05495305299999));
#237049=CARTESIAN_POINT('Ctrl Pts',(-5.58736547800006,11.6,9.05495305299999));
#237050=CARTESIAN_POINT('Ctrl Pts',(-5.58667851500006,15.2,9.05283699299999));
#237051=CARTESIAN_POINT('Ctrl Pts',(-5.58667851500006,11.6,9.05283699299999));
#237052=CARTESIAN_POINT('Ctrl Pts',(-5.58599173500006,15.2,9.05072784999999));
#237053=CARTESIAN_POINT('Ctrl Pts',(-5.58599173500006,11.6,9.05072784999999));
#237054=CARTESIAN_POINT('Ctrl Pts',(-5.58530515500006,15.2,9.04862563599998));
#237055=CARTESIAN_POINT('Ctrl Pts',(-5.58530515500006,11.6,9.04862563599998));
#237056=CARTESIAN_POINT('Ctrl Pts',(-5.58461878900006,15.2,9.04653035999999));
#237057=CARTESIAN_POINT('Ctrl Pts',(-5.58461878900006,11.6,9.04653035999999));
#237058=CARTESIAN_POINT('Ctrl Pts',(-5.58393265100006,15.2,9.04444203099998));
#237059=CARTESIAN_POINT('Ctrl Pts',(-5.58393265100006,11.6,9.04444203099998));
#237060=CARTESIAN_POINT('Ctrl Pts',(-5.58324675400006,15.2,9.04236066099998));
#237061=CARTESIAN_POINT('Ctrl Pts',(-5.58324675400006,11.6,9.04236066099998));
#237062=CARTESIAN_POINT('Ctrl Pts',(-5.58256111400006,15.2,9.04028625599998));
#237063=CARTESIAN_POINT('Ctrl Pts',(-5.58256111400006,11.6,9.04028625599998));
#237064=CARTESIAN_POINT('Ctrl Pts',(-5.58187574600006,15.2,9.03821882999999));
#237065=CARTESIAN_POINT('Ctrl Pts',(-5.58187574600006,11.6,9.03821882999999));
#237066=CARTESIAN_POINT('Ctrl Pts',(-5.58119066300006,15.2,9.03615839199999));
#237067=CARTESIAN_POINT('Ctrl Pts',(-5.58119066300006,11.6,9.03615839199999));
#237068=CARTESIAN_POINT('Ctrl Pts',(-5.58050588000006,15.2,9.03410494999999));
#237069=CARTESIAN_POINT('Ctrl Pts',(-5.58050588000006,11.6,9.03410494999999));
#237070=CARTESIAN_POINT('Ctrl Pts',(-5.57982141200006,15.2,9.03205851399999));
#237071=CARTESIAN_POINT('Ctrl Pts',(-5.57982141200006,11.6,9.03205851399999));
#237072=CARTESIAN_POINT('Ctrl Pts',(-5.57913727300006,15.2,9.03001909699999));
#237073=CARTESIAN_POINT('Ctrl Pts',(-5.57913727300006,11.6,9.03001909699999));
#237074=CARTESIAN_POINT('Ctrl Pts',(-5.57845347900006,15.2,9.02798670599999));
#237075=CARTESIAN_POINT('Ctrl Pts',(-5.57845347900006,11.6,9.02798670599999));
#237076=CARTESIAN_POINT('Ctrl Pts',(-5.57777004300006,15.2,9.02596135299999));
#237077=CARTESIAN_POINT('Ctrl Pts',(-5.57777004300006,11.6,9.02596135299999));
#237078=CARTESIAN_POINT('Ctrl Pts',(-5.57708698100006,15.2,9.02394304599999));
#237079=CARTESIAN_POINT('Ctrl Pts',(-5.57708698100006,11.6,9.02394304599999));
#237080=CARTESIAN_POINT('Ctrl Pts',(-5.57640430800006,15.2,9.02193179699999));
#237081=CARTESIAN_POINT('Ctrl Pts',(-5.57640430800006,11.6,9.02193179699999));
#237082=CARTESIAN_POINT('Ctrl Pts',(-5.57572203700006,15.2,9.01992761499999));
#237083=CARTESIAN_POINT('Ctrl Pts',(-5.57572203700006,11.6,9.01992761499999));
#237084=CARTESIAN_POINT('Ctrl Pts',(-5.57504018500006,15.2,9.01793050999999));
#237085=CARTESIAN_POINT('Ctrl Pts',(-5.57504018500006,11.6,9.01793050999999));
#237086=CARTESIAN_POINT('Ctrl Pts',(-5.57435876800006,15.2,9.01594049299998));
#237087=CARTESIAN_POINT('Ctrl Pts',(-5.57435876800006,11.6,9.01594049299998));
#237088=CARTESIAN_POINT('Ctrl Pts',(-5.57367779900006,15.2,9.01395757299999));
#237089=CARTESIAN_POINT('Ctrl Pts',(-5.57367779900006,11.6,9.01395757299999));
#237090=CARTESIAN_POINT('Ctrl Pts',(-5.57299729300006,15.2,9.01198176199999));
#237091=CARTESIAN_POINT('Ctrl Pts',(-5.57299729300006,11.6,9.01198176199999));
#237092=CARTESIAN_POINT('Ctrl Pts',(-5.57231726600006,15.2,9.01001306799999));
#237093=CARTESIAN_POINT('Ctrl Pts',(-5.57231726600006,11.6,9.01001306799999));
#237094=CARTESIAN_POINT('Ctrl Pts',(-5.57163773400006,15.2,9.00805150299998));
#237095=CARTESIAN_POINT('Ctrl Pts',(-5.57163773400006,11.6,9.00805150299998));
#237096=CARTESIAN_POINT('Ctrl Pts',(-5.57095871100006,15.2,9.00609707599998));
#237097=CARTESIAN_POINT('Ctrl Pts',(-5.57095871100006,11.6,9.00609707599998));
#237098=CARTESIAN_POINT('Ctrl Pts',(-5.57028021400006,15.2,9.00414979799999));
#237099=CARTESIAN_POINT('Ctrl Pts',(-5.57028021400006,11.6,9.00414979799999));
#237100=CARTESIAN_POINT('Ctrl Pts',(-5.56960225700006,15.2,9.00220967899998));
#237101=CARTESIAN_POINT('Ctrl Pts',(-5.56960225700006,11.6,9.00220967899998));
#237102=CARTESIAN_POINT('Ctrl Pts',(-5.56892485500006,15.2,9.00027672899999));
#237103=CARTESIAN_POINT('Ctrl Pts',(-5.56892485500006,11.6,9.00027672899999));
#237104=CARTESIAN_POINT('Ctrl Pts',(-5.56824802500006,15.2,8.99835095899999));
#237105=CARTESIAN_POINT('Ctrl Pts',(-5.56824802500006,11.6,8.99835095899999));
#237106=CARTESIAN_POINT('Ctrl Pts',(-5.56757178200006,15.2,8.99643237899999));
#237107=CARTESIAN_POINT('Ctrl Pts',(-5.56757178200006,11.6,8.99643237899999));
#237108=CARTESIAN_POINT('Ctrl Pts',(-5.56689614200006,15.2,8.99452099999999));
#237109=CARTESIAN_POINT('Ctrl Pts',(-5.56689614200006,11.6,8.99452099999999));
#237110=CARTESIAN_POINT('Ctrl Pts',(-5.56622112000006,15.2,8.99261682999999));
#237111=CARTESIAN_POINT('Ctrl Pts',(-5.56622112000006,11.6,8.99261682999999));
#237112=CARTESIAN_POINT('Ctrl Pts',(-5.56554673300006,15.2,8.99071988199999));
#237113=CARTESIAN_POINT('Ctrl Pts',(-5.56554673300006,11.6,8.99071988199999));
#237114=CARTESIAN_POINT('Ctrl Pts',(-5.56487299500006,15.2,8.98883016799999));
#237115=CARTESIAN_POINT('Ctrl Pts',(-5.56487299500006,11.6,8.98883016799999));
#237116=CARTESIAN_POINT('Ctrl Pts',(-5.56419992400006,15.2,8.98694769299999));
#237117=CARTESIAN_POINT('Ctrl Pts',(-5.56419992400006,11.6,8.98694769299999));
#237118=CARTESIAN_POINT('Ctrl Pts',(-5.56352753400006,15.2,8.98507247299998));
#237119=CARTESIAN_POINT('Ctrl Pts',(-5.56352753400006,11.6,8.98507247299998));
#237120=CARTESIAN_POINT('Ctrl Pts',(-5.56285584300006,15.2,8.98320451499998));
#237121=CARTESIAN_POINT('Ctrl Pts',(-5.56285584300006,11.6,8.98320451499998));
#237122=CARTESIAN_POINT('Ctrl Pts',(-5.56218486400006,15.2,8.98134383099999));
#237123=CARTESIAN_POINT('Ctrl Pts',(-5.56218486400006,11.6,8.98134383099999));
#237124=CARTESIAN_POINT('Ctrl Pts',(-5.56151461700006,15.2,8.97949043099998));
#237125=CARTESIAN_POINT('Ctrl Pts',(-5.56151461700006,11.6,8.97949043099998));
#237126=CARTESIAN_POINT('Ctrl Pts',(-5.56084511600006,15.2,8.97764432799999));
#237127=CARTESIAN_POINT('Ctrl Pts',(-5.56084511600006,11.6,8.97764432799999));
#237128=CARTESIAN_POINT('Ctrl Pts',(-5.56017637800006,15.2,8.97580552899999));
#237129=CARTESIAN_POINT('Ctrl Pts',(-5.56017637800006,11.6,8.97580552899999));
#237130=CARTESIAN_POINT('Ctrl Pts',(-5.55950841800006,15.2,8.97397404599998));
#237131=CARTESIAN_POINT('Ctrl Pts',(-5.55950841800006,11.6,8.97397404599998));
#237132=CARTESIAN_POINT('Ctrl Pts',(-5.55884125300006,15.2,8.97214989099999));
#237133=CARTESIAN_POINT('Ctrl Pts',(-5.55884125300006,11.6,8.97214989099999));
#237134=CARTESIAN_POINT('Ctrl Pts',(-5.55817490100006,15.2,8.97033307399998));
#237135=CARTESIAN_POINT('Ctrl Pts',(-5.55817490100006,11.6,8.97033307399998));
#237136=CARTESIAN_POINT('Ctrl Pts',(-5.55750937700005,15.2,8.96852360499999));
#237137=CARTESIAN_POINT('Ctrl Pts',(-5.55750937700005,11.6,8.96852360499999));
#237138=CARTESIAN_POINT('Ctrl Pts',(-5.55684469700005,15.2,8.96672149499998));
#237139=CARTESIAN_POINT('Ctrl Pts',(-5.55684469700005,11.6,8.96672149499998));
#237140=CARTESIAN_POINT('Ctrl Pts',(-5.55618088000006,15.2,8.96492675499999));
#237141=CARTESIAN_POINT('Ctrl Pts',(-5.55618088000006,11.6,8.96492675499999));
#237142=CARTESIAN_POINT('Ctrl Pts',(-5.55551794000006,15.2,8.96313939699999));
#237143=CARTESIAN_POINT('Ctrl Pts',(-5.55551794000006,11.6,8.96313939699999));
#237144=CARTESIAN_POINT('Ctrl Pts',(-5.55485589600006,15.2,8.96135942899999));
#237145=CARTESIAN_POINT('Ctrl Pts',(-5.55485589600006,11.6,8.96135942899999));
#237146=CARTESIAN_POINT('Ctrl Pts',(-5.55419476400006,15.2,8.95958686499998));
#237147=CARTESIAN_POINT('Ctrl Pts',(-5.55419476400006,11.6,8.95958686499998));
#237148=CARTESIAN_POINT('Ctrl Pts',(-5.55353456000006,15.2,8.95782171299999));
#237149=CARTESIAN_POINT('Ctrl Pts',(-5.55353456000006,11.6,8.95782171299999));
#237150=CARTESIAN_POINT('Ctrl Pts',(-5.55287530200006,15.2,8.95606398699999));
#237151=CARTESIAN_POINT('Ctrl Pts',(-5.55287530200006,11.6,8.95606398699999));
#237152=CARTESIAN_POINT('Ctrl Pts',(-5.55221700600006,15.2,8.95431369599999));
#237153=CARTESIAN_POINT('Ctrl Pts',(-5.55221700600006,11.6,8.95431369599999));
#237154=CARTESIAN_POINT('Ctrl Pts',(-5.55155969100006,15.2,8.95257084999999));
#237155=CARTESIAN_POINT('Ctrl Pts',(-5.55155969100006,11.6,8.95257084999999));
#237156=CARTESIAN_POINT('Ctrl Pts',(-5.55090337300006,15.2,8.95083546399999));
#237157=CARTESIAN_POINT('Ctrl Pts',(-5.55090337300006,11.6,8.95083546399999));
#237158=CARTESIAN_POINT('Ctrl Pts',(-5.55024806800006,15.2,8.94910754499998));
#237159=CARTESIAN_POINT('Ctrl Pts',(-5.55024806800006,11.6,8.94910754499998));
#237160=CARTESIAN_POINT('Ctrl Pts',(-5.54959379600006,15.2,8.94738710499999));
#237161=CARTESIAN_POINT('Ctrl Pts',(-5.54959379600006,11.6,8.94738710499999));
#237162=CARTESIAN_POINT('Ctrl Pts',(-5.54894057200006,15.2,8.94567415599998));
#237163=CARTESIAN_POINT('Ctrl Pts',(-5.54894057200006,11.6,8.94567415599998));
#237164=CARTESIAN_POINT('Ctrl Pts',(-5.54828841500006,15.2,8.94396870899998));
#237165=CARTESIAN_POINT('Ctrl Pts',(-5.54828841500006,11.6,8.94396870899998));
#237166=CARTESIAN_POINT('Ctrl Pts',(-5.54763734200006,15.2,8.94227077499998));
#237167=CARTESIAN_POINT('Ctrl Pts',(-5.54763734200006,11.6,8.94227077499998));
#237168=CARTESIAN_POINT('Ctrl Pts',(-5.54698737000006,15.2,8.94058036599999));
#237169=CARTESIAN_POINT('Ctrl Pts',(-5.54698737000006,11.6,8.94058036599999));
#237170=CARTESIAN_POINT('Ctrl Pts',(-5.54633851800006,15.2,8.93889749199998));
#237171=CARTESIAN_POINT('Ctrl Pts',(-5.54633851800006,11.6,8.93889749199998));
#237172=CARTESIAN_POINT('Ctrl Pts',(-5.54569080200006,15.2,8.93722216299999));
#237173=CARTESIAN_POINT('Ctrl Pts',(-5.54569080200006,11.6,8.93722216299999));
#237174=CARTESIAN_POINT('Ctrl Pts',(-5.54504424100006,15.2,8.93555439299998));
#237175=CARTESIAN_POINT('Ctrl Pts',(-5.54504424100006,11.6,8.93555439299998));
#237176=CARTESIAN_POINT('Ctrl Pts',(-5.54439885200006,15.2,8.93389419199998));
#237177=CARTESIAN_POINT('Ctrl Pts',(-5.54439885200006,11.6,8.93389419199998));
#237178=CARTESIAN_POINT('Ctrl Pts',(-5.54375465500006,15.2,8.93224157199998));
#237179=CARTESIAN_POINT('Ctrl Pts',(-5.54375465500006,11.6,8.93224157199998));
#237180=CARTESIAN_POINT('Ctrl Pts',(-5.54311166500006,15.2,8.93059654399998));
#237181=CARTESIAN_POINT('Ctrl Pts',(-5.54311166500006,11.6,8.93059654399998));
#237182=CARTESIAN_POINT('Ctrl Pts',(-5.54246990300006,15.2,8.92895911799998));
#237183=CARTESIAN_POINT('Ctrl Pts',(-5.54246990300006,11.6,8.92895911799998));
#237184=CARTESIAN_POINT('Ctrl Pts',(-5.54182938400006,15.2,8.92732930799998));
#237185=CARTESIAN_POINT('Ctrl Pts',(-5.54182938400006,11.6,8.92732930799998));
#237186=CARTESIAN_POINT('Ctrl Pts',(-5.54119012900006,15.2,8.92570712399999));
#237187=CARTESIAN_POINT('Ctrl Pts',(-5.54119012900006,11.6,8.92570712399999));
#237188=CARTESIAN_POINT('Ctrl Pts',(-5.54055215600005,15.2,8.92409257799999));
#237189=CARTESIAN_POINT('Ctrl Pts',(-5.54055215600005,11.6,8.92409257799999));
#237190=CARTESIAN_POINT('Ctrl Pts',(-5.53991548100006,15.2,8.92248568099999));
#237191=CARTESIAN_POINT('Ctrl Pts',(-5.53991548100006,11.6,8.92248568099999));
#237192=CARTESIAN_POINT('Ctrl Pts',(-5.53928012500006,15.2,8.92088644499999));
#237193=CARTESIAN_POINT('Ctrl Pts',(-5.53928012500006,11.6,8.92088644499999));
#237194=CARTESIAN_POINT('Ctrl Pts',(-5.53864610500006,15.2,8.91929488199998));
#237195=CARTESIAN_POINT('Ctrl Pts',(-5.53864610500006,11.6,8.91929488199998));
#237196=CARTESIAN_POINT('Ctrl Pts',(-5.53801344100005,15.2,8.91771100199998));
#237197=CARTESIAN_POINT('Ctrl Pts',(-5.53801344100005,11.6,8.91771100199998));
#237198=CARTESIAN_POINT('Ctrl Pts',(-5.53738215100006,15.2,8.91613481799999));
#237199=CARTESIAN_POINT('Ctrl Pts',(-5.53738215100006,11.6,8.91613481799999));
#237200=CARTESIAN_POINT('Ctrl Pts',(-5.53675225300006,15.2,8.91456634199999));
#237201=CARTESIAN_POINT('Ctrl Pts',(-5.53675225300006,11.6,8.91456634199999));
#237202=CARTESIAN_POINT('Ctrl Pts',(-5.53612376700006,15.2,8.91300558499999));
#237203=CARTESIAN_POINT('Ctrl Pts',(-5.53612376700006,11.6,8.91300558499999));
#237204=CARTESIAN_POINT('Ctrl Pts',(-5.53549671100006,15.2,8.91145255899998));
#237205=CARTESIAN_POINT('Ctrl Pts',(-5.53549671100006,11.6,8.91145255899998));
#237206=CARTESIAN_POINT('Ctrl Pts',(-5.53487110500006,15.2,8.90990727499998));
#237207=CARTESIAN_POINT('Ctrl Pts',(-5.53487110500006,11.6,8.90990727499998));
#237208=CARTESIAN_POINT('Ctrl Pts',(-5.53424696700006,15.2,8.90836974599999));
#237209=CARTESIAN_POINT('Ctrl Pts',(-5.53424696700006,11.6,8.90836974599999));
#237210=CARTESIAN_POINT('Ctrl Pts',(-5.53362431700006,15.2,8.90683998299998));
#237211=CARTESIAN_POINT('Ctrl Pts',(-5.53362431700006,11.6,8.90683998299998));
#237212=CARTESIAN_POINT('Ctrl Pts',(-5.53300317300006,15.2,8.90531799899998));
#237213=CARTESIAN_POINT('Ctrl Pts',(-5.53300317300006,11.6,8.90531799899998));
#237214=CARTESIAN_POINT('Ctrl Pts',(-5.53238355700006,15.2,8.90380380499998));
#237215=CARTESIAN_POINT('Ctrl Pts',(-5.53238355700006,11.6,8.90380380499998));
#237216=CARTESIAN_POINT('Ctrl Pts',(-5.53176548500006,15.2,8.90229741299999));
#237217=CARTESIAN_POINT('Ctrl Pts',(-5.53176548500006,11.6,8.90229741299999));
#237218=CARTESIAN_POINT('Ctrl Pts',(-5.53114897900006,15.2,8.90079883599999));
#237219=CARTESIAN_POINT('Ctrl Pts',(-5.53114897900006,11.6,8.90079883599999));
#237220=CARTESIAN_POINT('Ctrl Pts',(-5.53053405700005,15.2,8.89930808399999));
#237221=CARTESIAN_POINT('Ctrl Pts',(-5.53053405700005,11.6,8.89930808399999));
#237222=CARTESIAN_POINT('Ctrl Pts',(-5.52992074000006,15.2,8.89782517099999));
#237223=CARTESIAN_POINT('Ctrl Pts',(-5.52992074000006,11.6,8.89782517099999));
#237224=CARTESIAN_POINT('Ctrl Pts',(-5.52930904600006,15.2,8.89635010899998));
#237225=CARTESIAN_POINT('Ctrl Pts',(-5.52930904600006,11.6,8.89635010899998));
#237226=CARTESIAN_POINT('Ctrl Pts',(-5.52869899600006,15.2,8.89488290899998));
#237227=CARTESIAN_POINT('Ctrl Pts',(-5.52869899600006,11.6,8.89488290899998));
#237228=CARTESIAN_POINT('Ctrl Pts',(-5.52809061100006,15.2,8.89342358399999));
#237229=CARTESIAN_POINT('Ctrl Pts',(-5.52809061100006,11.6,8.89342358399999));
#237230=CARTESIAN_POINT('Ctrl Pts',(-5.52748390800006,15.2,8.89197214599999));
#237231=CARTESIAN_POINT('Ctrl Pts',(-5.52748390800006,11.6,8.89197214599999));
#237232=CARTESIAN_POINT('Ctrl Pts',(-5.52687891000006,15.2,8.89052860699999));
#237233=CARTESIAN_POINT('Ctrl Pts',(-5.52687891000006,11.6,8.89052860699999));
#237234=CARTESIAN_POINT('Ctrl Pts',(-5.52627563500006,15.2,8.88909297999999));
#237235=CARTESIAN_POINT('Ctrl Pts',(-5.52627563500006,11.6,8.88909297999999));
#237236=CARTESIAN_POINT('Ctrl Pts',(-5.52567410500005,15.2,8.88766527599999));
#237237=CARTESIAN_POINT('Ctrl Pts',(-5.52567410500005,11.6,8.88766527599999));
#237238=CARTESIAN_POINT('Ctrl Pts',(-5.52507433900006,15.2,8.88624550999998));
#237239=CARTESIAN_POINT('Ctrl Pts',(-5.52507433900006,11.6,8.88624550999998));
#237240=CARTESIAN_POINT('Ctrl Pts',(-5.52447635900006,15.2,8.88483369099998));
#237241=CARTESIAN_POINT('Ctrl Pts',(-5.52447635900006,11.6,8.88483369099998));
#237242=CARTESIAN_POINT('Ctrl Pts',(-5.52388018300006,15.2,8.88342983299999));
#237243=CARTESIAN_POINT('Ctrl Pts',(-5.52388018300006,11.6,8.88342983299999));
#237244=CARTESIAN_POINT('Ctrl Pts',(-5.52328583400006,15.2,8.88203394999999));
#237245=CARTESIAN_POINT('Ctrl Pts',(-5.52328583400006,11.6,8.88203394999999));
#237246=CARTESIAN_POINT('Ctrl Pts',(-5.52269333100006,15.2,8.88064605199999));
#237247=CARTESIAN_POINT('Ctrl Pts',(-5.52269333100006,11.6,8.88064605199999));
#237248=CARTESIAN_POINT('Ctrl Pts',(-5.52210269600006,15.2,8.87926615299998));
#237249=CARTESIAN_POINT('Ctrl Pts',(-5.52210269600006,11.6,8.87926615299998));
#237250=CARTESIAN_POINT('Ctrl Pts',(-5.52151394900006,15.2,8.87789426599999));
#237251=CARTESIAN_POINT('Ctrl Pts',(-5.52151394900006,11.6,8.87789426599999));
#237252=CARTESIAN_POINT('Ctrl Pts',(-5.52092711200006,15.2,8.87653040299998));
#237253=CARTESIAN_POINT('Ctrl Pts',(-5.52092711200006,11.6,8.87653040299998));
#237254=CARTESIAN_POINT('Ctrl Pts',(-5.52034220400006,15.2,8.87517457499998));
#237255=CARTESIAN_POINT('Ctrl Pts',(-5.52034220400006,11.6,8.87517457499998));
#237256=CARTESIAN_POINT('Ctrl Pts',(-5.51975924900006,15.2,8.87382679799998));
#237257=CARTESIAN_POINT('Ctrl Pts',(-5.51975924900006,11.6,8.87382679799998));
#237258=CARTESIAN_POINT('Ctrl Pts',(-5.51917826500006,15.2,8.87248708199999));
#237259=CARTESIAN_POINT('Ctrl Pts',(-5.51917826500006,11.6,8.87248708199999));
#237260=CARTESIAN_POINT('Ctrl Pts',(-5.51859927600006,15.2,8.87115544199998));
#237261=CARTESIAN_POINT('Ctrl Pts',(-5.51859927600006,11.6,8.87115544199998));
#237262=CARTESIAN_POINT('Ctrl Pts',(-5.51802230300006,15.2,8.86983188899999));
#237263=CARTESIAN_POINT('Ctrl Pts',(-5.51802230300006,11.6,8.86983188899999));
#237264=CARTESIAN_POINT('Ctrl Pts',(-5.51744736700006,15.2,8.86851643699998));
#237265=CARTESIAN_POINT('Ctrl Pts',(-5.51744736700006,11.6,8.86851643699998));
#237266=CARTESIAN_POINT('Ctrl Pts',(-5.51687448900006,15.2,8.86720909899999));
#237267=CARTESIAN_POINT('Ctrl Pts',(-5.51687448900006,11.6,8.86720909899999));
#237268=CARTESIAN_POINT('Ctrl Pts',(-5.51630369100006,15.2,8.86590988699999));
#237269=CARTESIAN_POINT('Ctrl Pts',(-5.51630369100006,11.6,8.86590988699999));
#237270=CARTESIAN_POINT('Ctrl Pts',(-5.51573499600006,15.2,8.86461881499999));
#237271=CARTESIAN_POINT('Ctrl Pts',(-5.51573499600006,11.6,8.86461881499999));
#237272=CARTESIAN_POINT('Ctrl Pts',(-5.51516842500006,15.2,8.86333589499999));
#237273=CARTESIAN_POINT('Ctrl Pts',(-5.51516842500006,11.6,8.86333589499999));
#237274=CARTESIAN_POINT('Ctrl Pts',(-5.51460400000006,15.2,8.86206114199998));
#237275=CARTESIAN_POINT('Ctrl Pts',(-5.51460400000006,11.6,8.86206114199998));
#237276=CARTESIAN_POINT('Ctrl Pts',(-5.51404174200006,15.2,8.86079456799998));
#237277=CARTESIAN_POINT('Ctrl Pts',(-5.51404174200006,11.6,8.86079456799998));
#237278=CARTESIAN_POINT('Ctrl Pts',(-5.51348167600006,15.2,8.85953618499999));
#237279=CARTESIAN_POINT('Ctrl Pts',(-5.51348167600006,11.6,8.85953618499999));
#237280=CARTESIAN_POINT('Ctrl Pts',(-5.51292382200006,15.2,8.85828600699998));
#237281=CARTESIAN_POINT('Ctrl Pts',(-5.51292382200006,11.6,8.85828600699998));
#237282=CARTESIAN_POINT('Ctrl Pts',(-5.51236820400006,15.2,8.85704404899998));
#237283=CARTESIAN_POINT('Ctrl Pts',(-5.51236820400006,11.6,8.85704404899998));
#237284=CARTESIAN_POINT('Ctrl Pts',(-5.51181484300006,15.2,8.85581032199998));
#237285=CARTESIAN_POINT('Ctrl Pts',(-5.51181484300006,11.6,8.85581032199998));
#237286=CARTESIAN_POINT('Ctrl Pts',(-5.51126376200005,15.2,8.85458484099999));
#237287=CARTESIAN_POINT('Ctrl Pts',(-5.51126376200005,11.6,8.85458484099999));
#237288=CARTESIAN_POINT('Ctrl Pts',(-5.51071498500006,15.2,8.85336761899998));
#237289=CARTESIAN_POINT('Ctrl Pts',(-5.51071498500006,11.6,8.85336761899998));
#237290=CARTESIAN_POINT('Ctrl Pts',(-5.51016853400006,15.2,8.85215866799999));
#237291=CARTESIAN_POINT('Ctrl Pts',(-5.51016853400006,11.6,8.85215866799999));
#237292=CARTESIAN_POINT('Ctrl Pts',(-5.50962443100006,15.2,8.85095800399998));
#237293=CARTESIAN_POINT('Ctrl Pts',(-5.50962443100006,11.6,8.85095800399998));
#237294=CARTESIAN_POINT('Ctrl Pts',(-5.50908270000006,15.2,8.84976563899999));
#237295=CARTESIAN_POINT('Ctrl Pts',(-5.50908270000006,11.6,8.84976563899999));
#237296=CARTESIAN_POINT('Ctrl Pts',(-5.50854336400006,15.2,8.84858158699998));
#237297=CARTESIAN_POINT('Ctrl Pts',(-5.50854336400006,11.6,8.84858158699998));
#237298=CARTESIAN_POINT('Ctrl Pts',(-5.50800644600006,15.2,8.84740586199998));
#237299=CARTESIAN_POINT('Ctrl Pts',(-5.50800644600006,11.6,8.84740586199998));
#237300=CARTESIAN_POINT('Ctrl Pts',(-5.50747197000006,15.2,8.84623847599999));
#237301=CARTESIAN_POINT('Ctrl Pts',(-5.50747197000006,11.6,8.84623847599999));
#237302=CARTESIAN_POINT('Ctrl Pts',(-5.50693996000006,15.2,8.84507944399999));
#237303=CARTESIAN_POINT('Ctrl Pts',(-5.50693996000006,11.6,8.84507944399999));
#237304=CARTESIAN_POINT('Ctrl Pts',(-5.50641043800006,15.2,8.84392878099998));
#237305=CARTESIAN_POINT('Ctrl Pts',(-5.50641043800006,11.6,8.84392878099998));
#237306=CARTESIAN_POINT('Ctrl Pts',(-5.50588342800006,15.2,8.84278649899999));
#237307=CARTESIAN_POINT('Ctrl Pts',(-5.50588342800006,11.6,8.84278649899999));
#237308=CARTESIAN_POINT('Ctrl Pts',(-5.50535895400006,15.2,8.84165261399998));
#237309=CARTESIAN_POINT('Ctrl Pts',(-5.50535895400006,11.6,8.84165261399998));
#237310=CARTESIAN_POINT('Ctrl Pts',(-5.50483704200006,15.2,8.84052713699998));
#237311=CARTESIAN_POINT('Ctrl Pts',(-5.50483704200006,11.6,8.84052713699998));
#237312=CARTESIAN_POINT('Ctrl Pts',(-5.50431771200006,15.2,8.83941008399999));
#237313=CARTESIAN_POINT('Ctrl Pts',(-5.50431771200006,11.6,8.83941008399999));
#237314=CARTESIAN_POINT('Ctrl Pts',(-5.50380099200006,15.2,8.83830146899999));
#237315=CARTESIAN_POINT('Ctrl Pts',(-5.50380099200006,11.6,8.83830146899999));
#237316=CARTESIAN_POINT('Ctrl Pts',(-5.50328690400006,15.2,8.83720130499999));
#237317=CARTESIAN_POINT('Ctrl Pts',(-5.50328690400006,11.6,8.83720130499999));
#237318=CARTESIAN_POINT('Ctrl Pts',(-5.50277547400006,15.2,8.83610960699999));
#237319=CARTESIAN_POINT('Ctrl Pts',(-5.50277547400006,11.6,8.83610960699999));
#237320=CARTESIAN_POINT('Ctrl Pts',(-5.50226672400006,15.2,8.83502638999998));
#237321=CARTESIAN_POINT('Ctrl Pts',(-5.50226672400006,11.6,8.83502638999998));
#237322=CARTESIAN_POINT('Ctrl Pts',(-5.50176068200006,15.2,8.83395166599998));
#237323=CARTESIAN_POINT('Ctrl Pts',(-5.50176068200006,11.6,8.83395166599998));
#237324=CARTESIAN_POINT('Ctrl Pts',(-5.50125736900006,15.2,8.83288545099998));
#237325=CARTESIAN_POINT('Ctrl Pts',(-5.50125736900006,11.6,8.83288545099998));
#237326=CARTESIAN_POINT('Ctrl Pts',(-5.50075681300005,15.2,8.83182775999998));
#237327=CARTESIAN_POINT('Ctrl Pts',(-5.50075681300005,11.6,8.83182775999998));
#237328=CARTESIAN_POINT('Ctrl Pts',(-5.50025903800006,15.2,8.83077860499998));
#237329=CARTESIAN_POINT('Ctrl Pts',(-5.50025903800006,11.6,8.83077860499998));
#237330=CARTESIAN_POINT('Ctrl Pts',(-5.49976406900006,15.2,8.82973800399999));
#237331=CARTESIAN_POINT('Ctrl Pts',(-5.49976406900006,11.6,8.82973800399999));
#237332=CARTESIAN_POINT('Ctrl Pts',(-5.49927193100006,15.2,8.82870596699998));
#237333=CARTESIAN_POINT('Ctrl Pts',(-5.49927193100006,11.6,8.82870596699998));
#237334=CARTESIAN_POINT('Ctrl Pts',(-5.49878265000006,15.2,8.82768251199998));
#237335=CARTESIAN_POINT('Ctrl Pts',(-5.49878265000006,11.6,8.82768251199998));
#237336=CARTESIAN_POINT('Ctrl Pts',(-5.49829625000006,15.2,8.82666765299999));
#237337=CARTESIAN_POINT('Ctrl Pts',(-5.49829625000006,11.6,8.82666765299999));
#237338=CARTESIAN_POINT('Ctrl Pts',(-5.49781275900005,15.2,8.82566140499998));
#237339=CARTESIAN_POINT('Ctrl Pts',(-5.49781275900005,11.6,8.82566140499998));
#237340=CARTESIAN_POINT('Ctrl Pts',(-5.49733220000006,15.2,8.82466378199998));
#237341=CARTESIAN_POINT('Ctrl Pts',(-5.49733220000006,11.6,8.82466378199998));
#237342=CARTESIAN_POINT('Ctrl Pts',(-5.49685460100005,15.2,8.82367479799999));
#237343=CARTESIAN_POINT('Ctrl Pts',(-5.49685460100005,11.6,8.82367479799999));
#237344=CARTESIAN_POINT('Ctrl Pts',(-5.49637998700006,15.2,8.82269446999998));
#237345=CARTESIAN_POINT('Ctrl Pts',(-5.49637998700006,11.6,8.82269446999998));
#237346=CARTESIAN_POINT('Ctrl Pts',(-5.49590838400006,15.2,8.82172280999999));
#237347=CARTESIAN_POINT('Ctrl Pts',(-5.49590838400006,11.6,8.82172280999999));
#237348=CARTESIAN_POINT('Ctrl Pts',(-5.49543982000006,15.2,8.82075983599999));
#237349=CARTESIAN_POINT('Ctrl Pts',(-5.49543982000006,11.6,8.82075983599999));
#237350=CARTESIAN_POINT('Ctrl Pts',(-5.49497431900006,15.2,8.81980556199998));
#237351=CARTESIAN_POINT('Ctrl Pts',(-5.49497431900006,11.6,8.81980556199998));
#237352=CARTESIAN_POINT('Ctrl Pts',(-5.49451190900006,15.2,8.81886000199999));
#237353=CARTESIAN_POINT('Ctrl Pts',(-5.49451190900006,11.6,8.81886000199999));
#237354=CARTESIAN_POINT('Ctrl Pts',(-5.49405261600006,15.2,8.81792317399999));
#237355=CARTESIAN_POINT('Ctrl Pts',(-5.49405261600006,11.6,8.81792317399999));
#237356=CARTESIAN_POINT('Ctrl Pts',(-5.49359646800006,15.2,8.81699508999999));
#237357=CARTESIAN_POINT('Ctrl Pts',(-5.49359646800006,11.6,8.81699508999999));
#237358=CARTESIAN_POINT('Ctrl Pts',(-5.49314349000006,15.2,8.81607576599999));
#237359=CARTESIAN_POINT('Ctrl Pts',(-5.49314349000006,11.6,8.81607576599999));
#237360=CARTESIAN_POINT('Ctrl Pts',(-5.49269371000006,15.2,8.81516521899999));
#237361=CARTESIAN_POINT('Ctrl Pts',(-5.49269371000006,11.6,8.81516521899999));
#237362=CARTESIAN_POINT('Ctrl Pts',(-5.49224715600006,15.2,8.81426346299998));
#237363=CARTESIAN_POINT('Ctrl Pts',(-5.49224715600006,11.6,8.81426346299998));
#237364=CARTESIAN_POINT('Ctrl Pts',(-5.49180385400006,15.2,8.81337051399999));
#237365=CARTESIAN_POINT('Ctrl Pts',(-5.49180385400006,11.6,8.81337051399999));
#237366=CARTESIAN_POINT('Ctrl Pts',(-5.49136383300006,15.2,8.81248638799999));
#237367=CARTESIAN_POINT('Ctrl Pts',(-5.49136383300006,11.6,8.81248638799999));
#237368=CARTESIAN_POINT('Ctrl Pts',(-5.49092711900006,15.2,8.81161109899999));
#237369=CARTESIAN_POINT('Ctrl Pts',(-5.49092711900006,11.6,8.81161109899999));
#237370=CARTESIAN_POINT('Ctrl Pts',(-5.49049374100006,15.2,8.81074466399999));
#237371=CARTESIAN_POINT('Ctrl Pts',(-5.49049374100006,11.6,8.81074466399999));
#237372=CARTESIAN_POINT('Ctrl Pts',(-5.49006372600005,15.2,8.80988709899999));
#237373=CARTESIAN_POINT('Ctrl Pts',(-5.49006372600005,11.6,8.80988709899999));
#237374=CARTESIAN_POINT('Ctrl Pts',(-5.48963710300006,15.2,8.80903841899999));
#237375=CARTESIAN_POINT('Ctrl Pts',(-5.48963710300006,11.6,8.80903841899999));
#237376=CARTESIAN_POINT('Ctrl Pts',(-5.48921390000006,15.2,8.80819863999999));
#237377=CARTESIAN_POINT('Ctrl Pts',(-5.48921390000006,11.6,8.80819863999999));
#237378=CARTESIAN_POINT('Ctrl Pts',(-5.48879414500006,15.2,8.80736777799999));
#237379=CARTESIAN_POINT('Ctrl Pts',(-5.48879414500006,11.6,8.80736777799999));
#237380=CARTESIAN_POINT('Ctrl Pts',(-5.48838026300006,15.2,8.80655058299999));
#237381=CARTESIAN_POINT('Ctrl Pts',(-5.48838026300006,11.6,8.80655058299999));
#237382=CARTESIAN_POINT('Ctrl Pts',(-5.48805240300006,15.2,8.80590482999999));
#237383=CARTESIAN_POINT('Ctrl Pts',(-5.48805240300006,11.6,8.80590482999999));
#237384=CARTESIAN_POINT('Ctrl Pts',(-5.48780866100006,15.2,8.80542564399999));
#237385=CARTESIAN_POINT('Ctrl Pts',(-5.48780866100006,11.6,8.80542564399999));
#237386=CARTESIAN_POINT('Ctrl Pts',(-5.48764764400006,15.2,8.80510947799999));
#237387=CARTESIAN_POINT('Ctrl Pts',(-5.48764764400006,11.6,8.80510947799999));
#237388=CARTESIAN_POINT('Ctrl Pts',(-5.48756848000005,15.2,8.80495412799998));
#237389=CARTESIAN_POINT('Ctrl Pts',(-5.48756848000005,11.6,8.80495412799998));
#237390=CARTESIAN_POINT('',(-5.48756847926628,12.2,8.8049541278923));
#237391=CARTESIAN_POINT('',(-5.48756847926628,15.2,8.8049541278923));
#237392=CARTESIAN_POINT('',(-5.48756847900005,12.2,8.80495412799998));
#237393=CARTESIAN_POINT('Ctrl Pts',(-5.75020264100006,12.2,9.95917514599999));
#237394=CARTESIAN_POINT('Ctrl Pts',(-5.74993549095152,12.2,9.9553615703072));
#237395=CARTESIAN_POINT('Ctrl Pts',(-5.74966449066059,12.2,9.9515548942664));
#237396=CARTESIAN_POINT('Ctrl Pts',(-5.74938964931735,12.2,9.9477551211625));
#237397=CARTESIAN_POINT('Ctrl Pts',(-5.74911480797412,12.2,9.9439553480586));
#237398=CARTESIAN_POINT('Ctrl Pts',(-5.74883612314145,12.2,9.94016247891821));
#237399=CARTESIAN_POINT('Ctrl Pts',(-5.74855360555471,12.2,9.93637652394917));
#237400=CARTESIAN_POINT('Ctrl Pts',(-5.74827108796797,12.2,9.93259056898012));
#237401=CARTESIAN_POINT('Ctrl Pts',(-5.7479847387856,12.2,9.9288115322695));
#237402=CARTESIAN_POINT('Ctrl Pts',(-5.74769458688,12.2,9.92503944261393));
#237403=CARTESIAN_POINT('Ctrl Pts',(-5.74740443492168,12.2,9.92126735227309));
#237404=CARTESIAN_POINT('Ctrl Pts',(-5.74711048097896,12.2,9.91750221114257));
#237405=CARTESIAN_POINT('Ctrl Pts',(-5.74681275947684,12.2,9.91374405518067));
#237406=CARTESIAN_POINT('Ctrl Pts',(-5.74641579756416,12.2,9.9087331817027));
#237407=CARTESIAN_POINT('Ctrl Pts',(-5.74601213592458,12.2,9.90373472732586));
#237408=CARTESIAN_POINT('Ctrl Pts',(-5.74560183979189,12.2,9.89874875789932));
#237409=CARTESIAN_POINT('Ctrl Pts',(-5.7452941176784,12.2,9.89500928065957));
#237410=CARTESIAN_POINT('Ctrl Pts',(-5.74498266154822,12.2,9.89127682692236));
#237411=CARTESIAN_POINT('Ctrl Pts',(-5.74466749808602,12.2,9.88755142295411));
#237412=CARTESIAN_POINT('Ctrl Pts',(-5.74435233462383,12.2,9.88382601898586));
#237413=CARTESIAN_POINT('Ctrl Pts',(-5.7440334642415,12.2,9.88010766589182));
#237414=CARTESIAN_POINT('Ctrl Pts',(-5.7437109162954,12.2,9.87639639506733));
#237415=CARTESIAN_POINT('Ctrl Pts',(-5.74338836829068,12.2,9.87268512356862));
#237416=CARTESIAN_POINT('Ctrl Pts',(-5.74306214242661,12.2,9.86898093364698));
#237417=CARTESIAN_POINT('Ctrl Pts',(-5.74273226791983,12.2,9.86528385669397));
#237418=CARTESIAN_POINT('Ctrl Pts',(-5.74240239347298,12.2,9.8615867804126));
#237419=CARTESIAN_POINT('Ctrl Pts',(-5.74206887086801,12.2,9.85789681791419));
#237420=CARTESIAN_POINT('Ctrl Pts',(-5.74173172646327,12.2,9.85421399663196));
#237421=CARTESIAN_POINT('Ctrl Pts',(-5.74139458205854,12.2,9.85053117534973));
#237422=CARTESIAN_POINT('Ctrl Pts',(-5.7410538166555,12.2,9.84685549606329));
#237423=CARTESIAN_POINT('Ctrl Pts',(-5.7407094597081,12.2,9.84318698926327));
#237424=CARTESIAN_POINT('Ctrl Pts',(-5.74025031713242,12.2,9.8382956470854));
#237425=CARTESIAN_POINT('Ctrl Pts',(-5.73978478907412,12.2,9.83341705457963));
#237426=CARTESIAN_POINT('Ctrl Pts',(-5.73931294383556,12.2,9.82855128625382));
#237427=CARTESIAN_POINT('Ctrl Pts',(-5.7388410985327,12.2,9.82368551726505));
#237428=CARTESIAN_POINT('Ctrl Pts',(-5.73836293617649,12.2,9.81883257119429));
#237429=CARTESIAN_POINT('Ctrl Pts',(-5.73787852748342,12.2,9.81399251920826));
#237430=CARTESIAN_POINT('Ctrl Pts',(-5.73751522099661,12.2,9.81036248054847));
#237431=CARTESIAN_POINT('Ctrl Pts',(-5.73714840027663,12.2,9.80673969659675));
#237432=CARTESIAN_POINT('Ctrl Pts',(-5.73677809529038,12.2,9.80312419539415));
#237433=CARTESIAN_POINT('Ctrl Pts',(-5.73640779030415,12.2,9.79950869419157));
#237434=CARTESIAN_POINT('Ctrl Pts',(-5.73603400032777,12.2,9.79590047784658));
#237435=CARTESIAN_POINT('Ctrl Pts',(-5.73565675632303,12.2,9.79229957492169));
#237436=CARTESIAN_POINT('Ctrl Pts',(-5.73527951231829,12.2,9.7886986719968));
#237437=CARTESIAN_POINT('Ctrl Pts',(-5.73489881386939,12.2,9.78510508405244));
#237438=CARTESIAN_POINT('Ctrl Pts',(-5.73451469088382,12.2,9.78151884080674));
#237439=CARTESIAN_POINT('Ctrl Pts',(-5.73413056782845,12.2,9.77793259690953));
#237440=CARTESIAN_POINT('Ctrl Pts',(-5.73374301927213,12.2,9.77435369890607));
#237441=CARTESIAN_POINT('Ctrl Pts',(-5.73335207817319,12.2,9.77078217647135));
#237442=CARTESIAN_POINT('Ctrl Pts',(-5.73296113714526,12.2,9.76721065468546));
#237443=CARTESIAN_POINT('Ctrl Pts',(-5.73256680065918,12.2,9.76364650816581));
#237444=CARTESIAN_POINT('Ctrl Pts',(-5.73216910167334,12.2,9.76008976933738));
#237445=CARTESIAN_POINT('Ctrl Pts',(-5.73177140268751,12.2,9.75653303050894));
#237446=CARTESIAN_POINT('Ctrl Pts',(-5.73137033940206,12.2,9.75298369883793));
#237447=CARTESIAN_POINT('Ctrl Pts',(-5.73096594395841,12.2,9.74944180450826));
#237448=CARTESIAN_POINT('Ctrl Pts',(-5.73056154851477,12.2,9.7458999101786));
#237449=CARTESIAN_POINT('Ctrl Pts',(-5.73015382069627,12.2,9.74236545274034));
#237450=CARTESIAN_POINT('Ctrl Pts',(-5.72974279079483,12.2,9.73883846536783));
#237451=CARTESIAN_POINT('Ctrl Pts',(-5.72933176089338,12.2,9.73531147799533));
#237452=CARTESIAN_POINT('Ctrl Pts',(-5.72891742976949,12.2,9.73179195911153));
#237453=CARTESIAN_POINT('Ctrl Pts',(-5.72849982784751,12.2,9.72827993968783));
#237454=CARTESIAN_POINT('Ctrl Pts',(-5.72808222592554,12.2,9.72476792026413));
#237455=CARTESIAN_POINT('Ctrl Pts',(-5.72766135324335,12.2,9.72126340178625));
#237456=CARTESIAN_POINT('Ctrl Pts',(-5.72723724234253,12.2,9.71776641399561));
#237457=CARTESIAN_POINT('Ctrl Pts',(-5.72681313136466,12.2,9.71426942556968));
#237458=CARTESIAN_POINT('Ctrl Pts',(-5.72638578180256,12.2,9.7107799679459));
#237459=CARTESIAN_POINT('Ctrl Pts',(-5.72595522440622,12.2,9.70729807352422));
#237460=CARTESIAN_POINT('Ctrl Pts',(-5.72552466708808,12.2,9.70381617973508));
#237461=CARTESIAN_POINT('Ctrl Pts',(-5.72509090325346,12.2,9.70034184909557));
#237462=CARTESIAN_POINT('Ctrl Pts',(-5.72465396393573,12.2,9.69687511134718));
#237463=CARTESIAN_POINT('Ctrl Pts',(-5.72407137820521,12.2,9.69225279455926));
#237464=CARTESIAN_POINT('Ctrl Pts',(-5.72348314890852,12.2,9.6876439789108));
#237465=CARTESIAN_POINT('Ctrl Pts',(-5.72288935109454,12.2,9.68304873783347));
#237466=CARTESIAN_POINT('Ctrl Pts',(-5.72244400271384,12.2,9.67960230686893));
#237467=CARTESIAN_POINT('Ctrl Pts',(-5.72199552346502,12.2,9.67616351120767));
#237468=CARTESIAN_POINT('Ctrl Pts',(-5.72154394414852,12.2,9.67273238474793));
#237469=CARTESIAN_POINT('Ctrl Pts',(-5.72109236474997,12.2,9.66930125766486));
#237470=CARTESIAN_POINT('Ctrl Pts',(-5.72063768680056,12.2,9.66587779716734));
#237471=CARTESIAN_POINT('Ctrl Pts',(-5.72017994144195,12.2,9.66246203629698));
#237472=CARTESIAN_POINT('Ctrl Pts',(-5.71972219616651,12.2,9.65904627604715));
#237473=CARTESIAN_POINT('Ctrl Pts',(-5.71926138459955,12.2,9.65563821605519));
#237474=CARTESIAN_POINT('Ctrl Pts',(-5.7187975406578,12.2,9.65223788634609));
#237475=CARTESIAN_POINT('Ctrl Pts',(-5.71833369671606,12.2,9.64883755663699));
#237476=CARTESIAN_POINT('Ctrl Pts',(-5.71786681870139,12.2,9.64544495857255));
#237477=CARTESIAN_POINT('Ctrl Pts',(-5.71739694179965,12.2,9.64206012376353));
#237478=CARTESIAN_POINT('Ctrl Pts',(-5.71692706489791,12.2,9.63867528895451));
#237479=CARTESIAN_POINT('Ctrl Pts',(-5.71645418855203,12.2,9.6352982172959));
#237480=CARTESIAN_POINT('Ctrl Pts',(-5.71597834573384,12.2,9.63192894102801));
#237481=CARTESIAN_POINT('Ctrl Pts',(-5.71550250291565,12.2,9.62855966476013));
#237482=CARTESIAN_POINT('Ctrl Pts',(-5.71502369361811,12.2,9.62519818419446));
#237483=CARTESIAN_POINT('Ctrl Pts',(-5.71454195276087,12.2,9.62184453085728));
#237484=CARTESIAN_POINT('Ctrl Pts',(-5.71406021190362,12.2,9.6184908775201));
#237485=CARTESIAN_POINT('Ctrl Pts',(-5.71357553915492,12.2,9.61514504987407));
#237486=CARTESIAN_POINT('Ctrl Pts',(-5.7130879683397,12.2,9.61180708395261));
#237487=CARTESIAN_POINT('Ctrl Pts',(-5.71243787386034,12.2,9.60735646231972));
#237488=CARTESIAN_POINT('Ctrl Pts',(-5.71178262856641,12.2,9.60291981283576));
#237489=CARTESIAN_POINT('Ctrl Pts',(-5.71112231274963,12.2,9.59849721279693));
#237490=CARTESIAN_POINT('Ctrl Pts',(-5.71046199702282,12.2,9.59407461336068));
#237491=CARTESIAN_POINT('Ctrl Pts',(-5.70979661216269,12.2,9.58966606351618));
#237492=CARTESIAN_POINT('Ctrl Pts',(-5.70912624038468,12.2,9.58527164065176));
#237493=CARTESIAN_POINT('Ctrl Pts',(-5.70845586851532,12.2,9.58087721718861));
#237494=CARTESIAN_POINT('Ctrl Pts',(-5.70778050929827,12.2,9.57649692026289));
#237495=CARTESIAN_POINT('Ctrl Pts',(-5.70710024748341,12.2,9.57213082752493));
#237496=CARTESIAN_POINT('Ctrl Pts',(-5.70641998566856,12.2,9.56776473478699));
#237497=CARTESIAN_POINT('Ctrl Pts',(-5.70573482013369,12.2,9.56341284680068));
#237498=CARTESIAN_POINT('Ctrl Pts',(-5.70504483692893,12.2,9.55907524006574));
#237499=CARTESIAN_POINT('Ctrl Pts',(-5.70418235806398,12.2,9.55365323253354));
#237500=CARTESIAN_POINT('Ctrl Pts',(-5.70331235030193,12.2,9.54825354162456));
#237501=CARTESIAN_POINT('Ctrl Pts',(-5.70243498081483,12.2,9.54287631748661));
#237502=CARTESIAN_POINT('Ctrl Pts',(-5.70173308511039,12.2,9.5385745374729));
#237503=CARTESIAN_POINT('Ctrl Pts',(-5.70102647864994,12.2,9.53428713733559));
#237504=CARTESIAN_POINT('Ctrl Pts',(-5.70031524750008,12.2,9.53001419649159));
#237505=CARTESIAN_POINT('Ctrl Pts',(-5.6996040163502,12.2,9.52574125564758));
#237506=CARTESIAN_POINT('Ctrl Pts',(-5.69888816126923,12.2,9.52148277250805));
#237507=CARTESIAN_POINT('Ctrl Pts',(-5.69816776884062,12.2,9.51723882705606));
#237508=CARTESIAN_POINT('Ctrl Pts',(-5.69744737651016,12.2,9.5129948821823));
#237509=CARTESIAN_POINT('Ctrl Pts',(-5.69672244811368,12.2,9.50876547365796));
#237510=CARTESIAN_POINT('Ctrl Pts',(-5.69599307122557,12.2,9.50455068226114));
#237511=CARTESIAN_POINT('Ctrl Pts',(-5.69526369423808,12.2,9.50033589029005));
#237512=CARTESIAN_POINT('Ctrl Pts',(-5.69452986974228,12.2,9.49613571546167));
#237513=CARTESIAN_POINT('Ctrl Pts',(-5.69379168714604,12.2,9.49195023729062));
#237514=CARTESIAN_POINT('Ctrl Pts',(-5.69305350465039,12.2,9.48776475968983));
#237515=CARTESIAN_POINT('Ctrl Pts',(-5.6923109623803,12.2,9.48359397737877));
#237516=CARTESIAN_POINT('Ctrl Pts',(-5.69156415405275,12.2,9.47943797260649));
#237517=CARTESIAN_POINT('Ctrl Pts',(-5.69081734562345,12.2,9.47528196726795));
#237518=CARTESIAN_POINT('Ctrl Pts',(-5.69006626941694,12.2,9.47114073810043));
#237519=CARTESIAN_POINT('Ctrl Pts',(-5.68931101761546,12.2,9.46701436639292));
#237520=CARTESIAN_POINT('Ctrl Pts',(-5.68855576591689,12.2,9.46288799524762));
#237521=CARTESIAN_POINT('Ctrl Pts',(-5.68779633764698,12.2,9.45877648099271));
#237522=CARTESIAN_POINT('Ctrl Pts',(-5.68703282732078,12.2,9.45467990482663));
#237523=CARTESIAN_POINT('Ctrl Pts',(-5.68626931689054,12.2,9.45058332810239));
#237524=CARTESIAN_POINT('Ctrl Pts',(-5.68550172414315,12.2,9.44650168983546));
#237525=CARTESIAN_POINT('Ctrl Pts',(-5.68473014171196,12.2,9.44243506989263));
#237526=CARTESIAN_POINT('Ctrl Pts',(-5.68395855938589,12.2,9.43836845050387));
#237527=CARTESIAN_POINT('Ctrl Pts',(-5.68318298730471,12.2,9.43431685203927));
#237528=CARTESIAN_POINT('Ctrl Pts',(-5.68240352166316,12.2,9.43028035311073));
#237529=CARTESIAN_POINT('Ctrl Pts',(-5.68142918953157,12.2,9.42523472903758));
#237530=CARTESIAN_POINT('Ctrl Pts',(-5.68044877176978,12.2,9.4202127011226));
#237531=CARTESIAN_POINT('Ctrl Pts',(-5.67946245808954,12.2,9.41521442959361));
#237532=CARTESIAN_POINT('Ctrl Pts',(-5.67867340710234,12.2,9.4112158121525));
#237533=CARTESIAN_POINT('Ctrl Pts',(-5.67788058174245,12.2,9.40723239801872));
#237534=CARTESIAN_POINT('Ctrl Pts',(-5.67708407997659,12.2,9.40326427069235));
#237535=CARTESIAN_POINT('Ctrl Pts',(-5.67628757831925,12.2,9.39929614390663));
#237536=CARTESIAN_POINT('Ctrl Pts',(-5.67548740023762,12.2,9.39534330398449));
#237537=CARTESIAN_POINT('Ctrl Pts',(-5.67468364341482,12.2,9.39140583319371));
#237538=CARTESIAN_POINT('Ctrl Pts',(-5.67387988648249,12.2,9.38746836186645));
#237539=CARTESIAN_POINT('Ctrl Pts',(-5.67307255176684,12.2,9.3835462594334));
#237540=CARTESIAN_POINT('Ctrl Pts',(-5.67226173877452,12.2,9.3796396119806));
#237541=CARTESIAN_POINT('Ctrl Pts',(-5.67145092589267,12.2,9.37573296506008));
#237542=CARTESIAN_POINT('Ctrl Pts',(-5.67063663471935,12.2,9.37184177027394));
#237543=CARTESIAN_POINT('Ctrl Pts',(-5.66981896584209,12.2,9.36796611336693));
#237544=CARTESIAN_POINT('Ctrl Pts',(-5.66900129685342,12.2,9.36409045593187));
#237545=CARTESIAN_POINT('Ctrl Pts',(-5.66818025009777,12.2,9.36023033498444));
#237546=CARTESIAN_POINT('Ctrl Pts',(-5.66735592777507,12.2,9.35638583694158));
#237547=CARTESIAN_POINT('Ctrl Pts',(-5.66653160545237,12.2,9.35254133889872));
#237548=CARTESIAN_POINT('Ctrl Pts',(-5.6657040078654,12.2,9.34871246241046));
#237549=CARTESIAN_POINT('Ctrl Pts',(-5.66487323759757,12.2,9.34489929242648));
#237550=CARTESIAN_POINT('Ctrl Pts',(-5.66404246744294,12.2,9.34108612296205));
#237551=CARTESIAN_POINT('Ctrl Pts',(-5.66320852526101,12.2,9.33728865905224));
#237552=CARTESIAN_POINT('Ctrl Pts',(-5.66237151449231,12.2,9.33350698951084));
#237553=CARTESIAN_POINT('Ctrl Pts',(-5.66153450360957,12.2,9.32972531945419));
#237554=CARTESIAN_POINT('Ctrl Pts',(-5.66069442522793,12.2,9.3259594407618));
#237555=CARTESIAN_POINT('Ctrl Pts',(-5.6598513849039,12.2,9.32220944067015));
#237556=CARTESIAN_POINT('Ctrl Pts',(-5.65900834469473,12.2,9.31845944108943));
#237557=CARTESIAN_POINT('Ctrl Pts',(-5.65816234165263,12.2,9.3147253192317));
#237558=CARTESIAN_POINT('Ctrl Pts',(-5.6573134841111,12.2,9.31100716181236));
#237559=CARTESIAN_POINT('Ctrl Pts',(-5.6564646264539,12.2,9.30728900388642));
#237560=CARTESIAN_POINT('Ctrl Pts',(-5.65561291175167,12.2,9.30358681100157));
#237561=CARTESIAN_POINT('Ctrl Pts',(-5.6547584513844,12.2,9.29990066900679));
#237562=CARTESIAN_POINT('Ctrl Pts',(-5.65390399113354,12.2,9.29621452751426));
#237563=CARTESIAN_POINT('Ctrl Pts',(-5.65304678491376,12.2,9.29254443906502));
#237564=CARTESIAN_POINT('Ctrl Pts',(-5.65218693959533,12.2,9.28889048830712));
#237565=CARTESIAN_POINT('Ctrl Pts',(-5.65132709415975,12.2,9.28523653705136));
#237566=CARTESIAN_POINT('Ctrl Pts',(-5.65046461226275,12.2,9.28159872521422));
#237567=CARTESIAN_POINT('Ctrl Pts',(-5.64959960393766,12.2,9.27797713996233));
#237568=CARTESIAN_POINT('Ctrl Pts',(-5.64873459573042,12.2,9.27435555520388));
#237569=CARTESIAN_POINT('Ctrl Pts',(-5.64786705917064,12.2,9.27075019753865));
#237570=CARTESIAN_POINT('Ctrl Pts',(-5.64699710964295,12.2,9.26716115526246));
#237571=CARTESIAN_POINT('Ctrl Pts',(-5.64612715999673,12.2,9.26357211249726));
#237572=CARTESIAN_POINT('Ctrl Pts',(-5.64525479677636,12.2,9.2599993859021));
#237573=CARTESIAN_POINT('Ctrl Pts',(-5.64438013139521,12.2,9.25644306270936));
#237574=CARTESIAN_POINT('Ctrl Pts',(-5.64350546613323,12.2,9.25288674000116));
#237575=CARTESIAN_POINT('Ctrl Pts',(-5.64262850091339,12.2,9.24934682310634));
#237576=CARTESIAN_POINT('Ctrl Pts',(-5.64174935015214,12.2,9.24582339905934));
#237577=CARTESIAN_POINT('Ctrl Pts',(-5.64087019927111,12.2,9.24229997453227));
#237578=CARTESIAN_POINT('Ctrl Pts',(-5.63998886233218,12.2,9.23879304540355));
#237579=CARTESIAN_POINT('Ctrl Pts',(-5.63910545622447,12.2,9.23530269953089));
#237580=CARTESIAN_POINT('Ctrl Pts',(-5.63822205023712,12.2,9.23181235413379));
#237581=CARTESIAN_POINT('Ctrl Pts',(-5.63733657580295,12.2,9.22833859254533));
#237582=CARTESIAN_POINT('Ctrl Pts',(-5.63644914915349,12.2,9.22488150704849));
#237583=CARTESIAN_POINT('Ctrl Pts',(-5.6355617223831,12.2,9.22142442108061));
#237584=CARTESIAN_POINT('Ctrl Pts',(-5.63467234491252,12.2,9.21798400961427));
#237585=CARTESIAN_POINT('Ctrl Pts',(-5.63378113547506,12.2,9.21456036498324));
#237586=CARTESIAN_POINT('Ctrl Pts',(-5.63288992603761,12.2,9.21113672035222));
#237587=CARTESIAN_POINT('Ctrl Pts',(-5.63199688453049,12.2,9.20772984133425));
#237588=CARTESIAN_POINT('Ctrl Pts',(-5.63110213237044,12.2,9.204339821929));
#237589=CARTESIAN_POINT('Ctrl Pts',(-5.62998369235324,12.2,9.20010229836526));
#237590=CARTESIAN_POINT('Ctrl Pts',(-5.62886257929101,12.2,9.19589111373222));
#237591=CARTESIAN_POINT('Ctrl Pts',(-5.62773903191369,12.2,9.19170645279728));
#237592=CARTESIAN_POINT('Ctrl Pts',(-5.62684019386486,12.2,9.18835872350197));
#237593=CARTESIAN_POINT('Ctrl Pts',(-5.625939797677,12.2,9.18502796708053));
#237594=CARTESIAN_POINT('Ctrl Pts',(-5.62503796951673,12.2,9.18171427923325));
#237595=CARTESIAN_POINT('Ctrl Pts',(-5.62391068437783,12.2,9.17757216964991));
#237596=CARTESIAN_POINT('Ctrl Pts',(-5.62278115828237,12.2,9.17345672844954));
#237597=CARTESIAN_POINT('Ctrl Pts',(-5.62164964070778,12.2,9.16936813801436));
#237598=CARTESIAN_POINT('Ctrl Pts',(-5.6207444267221,12.2,9.16609726593362));
#237599=CARTESIAN_POINT('Ctrl Pts',(-5.61983793607136,12.2,9.16284357976905));
#237600=CARTESIAN_POINT('Ctrl Pts',(-5.61893029942346,12.2,9.15960717308741));
#237601=CARTESIAN_POINT('Ctrl Pts',(-5.61802266265188,12.2,9.15637076596481));
#237602=CARTESIAN_POINT('Ctrl Pts',(-5.61711387828576,12.2,9.15315163833275));
#237603=CARTESIAN_POINT('Ctrl Pts',(-5.61620407695839,12.2,9.14994988699158));
#237604=CARTESIAN_POINT('Ctrl Pts',(-5.61506682536117,12.2,9.14594769803325));
#237605=CARTESIAN_POINT('Ctrl Pts',(-5.61392798338796,12.2,9.14197265617118));
#237606=CARTESIAN_POINT('Ctrl Pts',(-5.6127878092161,12.2,9.13802495247277));
#237607=CARTESIAN_POINT('Ctrl Pts',(-5.61141960025961,12.2,9.1332877082068));
#237608=CARTESIAN_POINT('Ctrl Pts',(-5.61004947107491,12.2,9.12858982978641));
#237609=CARTESIAN_POINT('Ctrl Pts',(-5.60867787629147,12.2,9.12393164445396));
#237610=CARTESIAN_POINT('Ctrl Pts',(-5.60753488059709,12.2,9.12004982320255));
#237611=CARTESIAN_POINT('Ctrl Pts',(-5.60639086607488,12.2,9.11619556654622));
#237612=CARTESIAN_POINT('Ctrl Pts',(-5.60524610107492,12.2,9.11236906772532));
#237613=CARTESIAN_POINT('Ctrl Pts',(-5.60410133607495,12.2,9.10854256890443));
#237614=CARTESIAN_POINT('Ctrl Pts',(-5.60295581869722,12.2,9.10474382618153));
#237615=CARTESIAN_POINT('Ctrl Pts',(-5.6018098221,12.2,9.10097303347169));
#237616=CARTESIAN_POINT('Ctrl Pts',(-5.60066382550279,12.2,9.09720224076185));
#237617=CARTESIAN_POINT('Ctrl Pts',(-5.59951734752811,12.2,9.09345939971335));
#237618=CARTESIAN_POINT('Ctrl Pts',(-5.59837066675902,12.2,9.08974470441861));
#237619=CARTESIAN_POINT('Ctrl Pts',(-5.59722398598992,12.2,9.08603000912386));
#237620=CARTESIAN_POINT('Ctrl Pts',(-5.59607710063339,12.2,9.08234345933323));
#237621=CARTESIAN_POINT('Ctrl Pts',(-5.59493029250839,12.2,9.07868525474991));
#237622=CARTESIAN_POINT('Ctrl Pts',(-5.59378348438339,12.2,9.07502705016658));
#237623=CARTESIAN_POINT('Ctrl Pts',(-5.5926367517213,12.2,9.07139718914201));
#237624=CARTESIAN_POINT('Ctrl Pts',(-5.59149038275776,12.2,9.06779587051462));
#237625=CARTESIAN_POINT('Ctrl Pts',(-5.59034401379422,12.2,9.06419455188722));
#237626=CARTESIAN_POINT('Ctrl Pts',(-5.58919800655289,12.2,9.06062177750013));
#237627=CARTESIAN_POINT('Ctrl Pts',(-5.58805265273349,12.2,9.05707774729331));
#237628=CARTESIAN_POINT('Ctrl Pts',(-5.58667822820014,12.2,9.05282491119965));
#237629=CARTESIAN_POINT('Ctrl Pts',(-5.58530474388339,12.2,9.04861346827768));
#237630=CARTESIAN_POINT('Ctrl Pts',(-5.58393271134984,12.2,9.04444377092733));
#237631=CARTESIAN_POINT('Ctrl Pts',(-5.58278935086367,12.2,9.04096902300913));
#237632=CARTESIAN_POINT('Ctrl Pts',(-5.58164699923366,12.2,9.03752326494521));
#237633=CARTESIAN_POINT('Ctrl Pts',(-5.58050595874235,12.2,9.0341067015268));
#237634=CARTESIAN_POINT('Ctrl Pts',(-5.57936491825104,12.2,9.03069013810839));
#237635=CARTESIAN_POINT('Ctrl Pts',(-5.57822518878895,12.2,9.02730277234991));
#237636=CARTESIAN_POINT('Ctrl Pts',(-5.57708707823338,12.2,9.02394481047491));
#237637=CARTESIAN_POINT('Ctrl Pts',(-5.57594896767782,12.2,9.0205868485999));
#237638=CARTESIAN_POINT('Ctrl Pts',(-5.57481247511014,12.2,9.01725829134079));
#237639=CARTESIAN_POINT('Ctrl Pts',(-5.57367791475777,12.2,9.01395935021478));
#237640=CARTESIAN_POINT('Ctrl Pts',(-5.57254335440539,12.2,9.01066040908877));
#237641=CARTESIAN_POINT('Ctrl Pts',(-5.5714107252538,12.2,9.00739108364779));
#237642=CARTESIAN_POINT('Ctrl Pts',(-5.57028034893447,12.2,9.00415158753824));
#237643=CARTESIAN_POINT('Ctrl Pts',(-5.56892389740056,12.2,9.000264192348));
#237644=CARTESIAN_POINT('Ctrl Pts',(-5.56757068516641,12.2,8.99641975147935));
#237645=CARTESIAN_POINT('Ctrl Pts',(-5.56622127879861,12.2,8.99261863569892));
#237646=CARTESIAN_POINT('Ctrl Pts',(-5.56464697128781,12.2,8.98818400039156));
#237647=CARTESIAN_POINT('Ctrl Pts',(-5.56307783979562,12.2,8.98380833995238));
#237648=CARTESIAN_POINT('Ctrl Pts',(-5.56151480345205,12.2,8.97949225499847));
#237649=CARTESIAN_POINT('Ctrl Pts',(-5.56017505808426,12.2,8.97579275380143));
#237650=CARTESIAN_POINT('Ctrl Pts',(-5.55883978913277,12.2,8.97213702198428));
#237651=CARTESIAN_POINT('Ctrl Pts',(-5.55750958809756,12.2,8.96852544494693));
#237652=CARTESIAN_POINT('Ctrl Pts',(-5.55617938706234,12.2,8.96491386790956));
#237653=CARTESIAN_POINT('Ctrl Pts',(-5.55485425574631,12.2,8.9613464458006));
#237654=CARTESIAN_POINT('Ctrl Pts',(-5.5535347966272,12.2,8.95782356984224));
#237655=CARTESIAN_POINT('Ctrl Pts',(-5.55221533738825,12.2,8.9543006935639));
#237656=CARTESIAN_POINT('Ctrl Pts',(-5.5509015511998,12.2,8.95082236482315));
#237657=CARTESIAN_POINT('Ctrl Pts',(-5.54959405796215,12.2,8.94738897755463));
#237658=CARTESIAN_POINT('Ctrl Pts',(-5.54828656484325,12.2,8.94395559059797));
#237659=CARTESIAN_POINT('Ctrl Pts',(-5.54698536469283,12.2,8.94056714961191));
#237660=CARTESIAN_POINT('Ctrl Pts',(-5.54569109073397,12.2,8.9372240527181));
#237661=CARTESIAN_POINT('Ctrl Pts',(-5.54418110437024,12.2,8.93332377280619));
#237662=CARTESIAN_POINT('Ctrl Pts',(-5.5426805454644,12.2,8.92948521613576));
#237663=CARTESIAN_POINT('Ctrl Pts',(-5.5411904494138,12.2,8.92570903331536));
#237664=CARTESIAN_POINT('Ctrl Pts',(-5.53970035347921,12.2,8.92193285078899));
#237665=CARTESIAN_POINT('Ctrl Pts',(-5.538220717002,12.2,8.91821904147287));
#237666=CARTESIAN_POINT('Ctrl Pts',(-5.53675260612054,12.2,8.91456827209934));
#237667=CARTESIAN_POINT('Ctrl Pts',(-5.53549422521805,12.2,8.91143904084229));
#237668=CARTESIAN_POINT('Ctrl Pts',(-5.53424431178302,12.2,8.90835612258975));
#237669=CARTESIAN_POINT('Ctrl Pts',(-5.53300355488246,12.2,8.90531994634296));
#237670=CARTESIAN_POINT('Ctrl Pts',(-5.5317627980946,12.2,8.90228377037196));
#237671=CARTESIAN_POINT('Ctrl Pts',(-5.5305311975227,12.2,8.89929433457227));
#237672=CARTESIAN_POINT('Ctrl Pts',(-5.52930945706666,12.2,8.89635207467712));
#237673=CARTESIAN_POINT('Ctrl Pts',(-5.52808771661062,12.2,8.89340981478197));
#237674=CARTESIAN_POINT('Ctrl Pts',(-5.52687583869639,12.2,8.8905147286601));
#237675=CARTESIAN_POINT('Ctrl Pts',(-5.52567454615598,12.2,8.88766726076028));
#237676=CARTESIAN_POINT('Ctrl Pts',(-5.52447325350644,12.2,8.88481979260182));
#237677=CARTESIAN_POINT('Ctrl Pts',(-5.52328254651625,12.2,8.88201993990632));
#237678=CARTESIAN_POINT('Ctrl Pts',(-5.52210316795247,12.2,8.87926815584179));
#237679=CARTESIAN_POINT('Ctrl Pts',(-5.52072722645542,12.2,8.87605774147475));
#237680=CARTESIAN_POINT('Ctrl Pts',(-5.51936670204286,12.2,8.872912750883));
#237681=CARTESIAN_POINT('Ctrl Pts',(-5.51802281237559,12.2,8.86983391452923));
#237682=CARTESIAN_POINT('Ctrl Pts',(-5.51687090681198,12.2,8.86719491163209));
#237683=CARTESIAN_POINT('Ctrl Pts',(-5.51573122094952,12.2,8.86460451174798));
#237684=CARTESIAN_POINT('Ctrl Pts',(-5.51460454172202,12.2,8.8620631866116));
#237685=CARTESIAN_POINT('Ctrl Pts',(-5.51347786259685,12.2,8.85952186170608));
#237686=CARTESIAN_POINT('Ctrl Pts',(-5.5123641921156,12.2,8.85702960658179));
#237687=CARTESIAN_POINT('Ctrl Pts',(-5.51126433798386,12.2,8.85458690574268));
#237688=CARTESIAN_POINT('Ctrl Pts',(-5.51016448385213,12.2,8.85214420490356));
#237689=CARTESIAN_POINT('Ctrl Pts',(-5.50907844657921,12.2,8.84975105569927));
#237690=CARTESIAN_POINT('Ctrl Pts',(-5.50800705661713,12.2,8.84740794703099));
#237691=CARTESIAN_POINT('Ctrl Pts',(-5.50693566655775,12.2,8.84506483814988));
#237692=CARTESIAN_POINT('Ctrl Pts',(-5.50587892557387,12.2,8.84277177049773));
#237693=CARTESIAN_POINT('Ctrl Pts',(-5.50483768746601,12.2,8.84052924276642));
#237694=CARTESIAN_POINT('Ctrl Pts',(-5.50379644945272,12.2,8.83828671523881));
#237695=CARTESIAN_POINT('Ctrl Pts',(-5.50277071518834,12.2,8.83609472958039));
#237696=CARTESIAN_POINT('Ctrl Pts',(-5.50176136430836,12.2,8.83395379324156));
#237697=CARTESIAN_POINT('Ctrl Pts',(-5.50075201342838,12.2,8.83181285690271));
#237698=CARTESIAN_POINT('Ctrl Pts',(-5.49975904705876,12.2,8.82972297281965));
#237699=CARTESIAN_POINT('Ctrl Pts',(-5.49878337037779,12.2,8.82768466120553));
#237700=CARTESIAN_POINT('Ctrl Pts',(-5.49780769360818,12.2,8.82564634940626));
#237701=CARTESIAN_POINT('Ctrl Pts',(-5.49684930633088,12.2,8.82365961269094));
#237702=CARTESIAN_POINT('Ctrl Pts',(-5.49590914361422,12.2,8.82172498125569));
#237703=CARTESIAN_POINT('Ctrl Pts',(-5.49481228723953,12.2,8.81946791151152));
#237704=CARTESIAN_POINT('Ctrl Pts',(-5.49374023430851,12.2,8.81728176750281));
#237705=CARTESIAN_POINT('Ctrl Pts',(-5.49269451657012,12.2,8.81516741694201));
#237706=CARTESIAN_POINT('Ctrl Pts',(-5.49179818697538,12.2,8.81335511624967));
#237707=CARTESIAN_POINT('Ctrl Pts',(-5.49092120719362,12.2,8.81159556257829));
#237708=CARTESIAN_POINT('Ctrl Pts',(-5.49006457389832,12.2,8.80988932007226));
#237709=CARTESIAN_POINT('Ctrl Pts',(-5.48921205189506,12.2,8.80819126643918));
#237710=CARTESIAN_POINT('Ctrl Pts',(-5.48837968070687,12.2,8.80654601357679));
#237711=CARTESIAN_POINT('Ctrl Pts',(-5.48756848000005,12.2,8.80495412799998));
#237712=CARTESIAN_POINT('Ctrl Pts',(-5.48756848000005,15.2,8.80495412799998));
#237713=CARTESIAN_POINT('Ctrl Pts',(-5.48837968070687,15.2,8.80654601357679));
#237714=CARTESIAN_POINT('Ctrl Pts',(-5.48921205189504,15.2,8.80819126643915));
#237715=CARTESIAN_POINT('Ctrl Pts',(-5.49006457389831,15.2,8.80988932007225));
#237716=CARTESIAN_POINT('Ctrl Pts',(-5.49092120719362,15.2,8.8115955625783));
#237717=CARTESIAN_POINT('Ctrl Pts',(-5.49179818697536,15.2,8.81335511624963));
#237718=CARTESIAN_POINT('Ctrl Pts',(-5.49269451657011,15.2,8.81516741694201));
#237719=CARTESIAN_POINT('Ctrl Pts',(-5.49359084608345,15.2,8.81697971746977));
#237720=CARTESIAN_POINT('Ctrl Pts',(-5.49450652515063,15.2,8.81884476540288));
#237721=CARTESIAN_POINT('Ctrl Pts',(-5.49544058578336,15.2,8.82076201099989));
#237722=CARTESIAN_POINT('Ctrl Pts',(-5.49637464641609,15.2,8.82267925659689));
#237723=CARTESIAN_POINT('Ctrl Pts',(-5.49732709035238,15.2,8.82464870093832));
#237724=CARTESIAN_POINT('Ctrl Pts',(-5.49829697711458,15.2,8.82666980554617));
#237725=CARTESIAN_POINT('Ctrl Pts',(-5.49926686396487,15.2,8.82869091033763));
#237726=CARTESIAN_POINT('Ctrl Pts',(-5.50025419360363,15.2,8.83076367833718));
#237727=CARTESIAN_POINT('Ctrl Pts',(-5.50125805832612,15.2,8.83288758220641));
#237728=CARTESIAN_POINT('Ctrl Pts',(-5.50226192295742,15.2,8.8350114858827));
#237729=CARTESIAN_POINT('Ctrl Pts',(-5.50328231865006,15.2,8.83718652781323));
#237730=CARTESIAN_POINT('Ctrl Pts',(-5.5043183644505,15.2,8.83941219349258));
#237731=CARTESIAN_POINT('Ctrl Pts',(-5.50535441025094,15.2,8.84163785917193));
#237732=CARTESIAN_POINT('Ctrl Pts',(-5.50640610429802,15.2,8.84391414896002));
#237733=CARTESIAN_POINT('Ctrl Pts',(-5.5074725864253,15.2,8.84624056437332));
#237734=CARTESIAN_POINT('Ctrl Pts',(-5.50853906864946,15.2,8.84856697999794));
#237735=CARTESIAN_POINT('Ctrl Pts',(-5.50962034222604,15.2,8.85094351624675));
#237736=CARTESIAN_POINT('Ctrl Pts',(-5.51071556661954,15.2,8.85336968704797));
#237737=CARTESIAN_POINT('Ctrl Pts',(-5.51181079091355,15.2,8.85579585762881));
#237738=CARTESIAN_POINT('Ctrl Pts',(-5.51291996980978,15.2,8.85827166116062));
#237739=CARTESIAN_POINT('Ctrl Pts',(-5.51404229001959,15.2,8.86079661590439));
#237740=CARTESIAN_POINT('Ctrl Pts',(-5.51516461022939,15.2,8.86332157064815));
#237741=CARTESIAN_POINT('Ctrl Pts',(-5.51630007107144,15.2,8.86589567752959));
#237742=CARTESIAN_POINT('Ctrl Pts',(-5.51744788144586,15.2,8.86851846534883));
#237743=CARTESIAN_POINT('Ctrl Pts',(-5.51859569182028,15.2,8.87114125316808));
#237744=CARTESIAN_POINT('Ctrl Pts',(-5.5197558527907,15.2,8.87381272284725));
#237745=CARTESIAN_POINT('Ctrl Pts',(-5.52092759416398,15.2,8.87653241149513));
#237746=CARTESIAN_POINT('Ctrl Pts',(-5.52209933564371,15.2,8.87925210039004));
#237747=CARTESIAN_POINT('Ctrl Pts',(-5.52328265745795,15.2,8.88202000658138));
#237748=CARTESIAN_POINT('Ctrl Pts',(-5.52447681010683,15.2,8.88483568140355));
#237749=CARTESIAN_POINT('Ctrl Pts',(-5.52567096264723,15.2,8.88765135596996));
#237750=CARTESIAN_POINT('Ctrl Pts',(-5.52687594692147,15.2,8.89051479484123));
#237751=CARTESIAN_POINT('Ctrl Pts',(-5.52809103154949,15.2,8.89342555574859));
#237752=CARTESIAN_POINT('Ctrl Pts',(-5.52930611617751,15.2,8.89633631665595));
#237753=CARTESIAN_POINT('Ctrl Pts',(-5.53053130171095,15.2,8.89929439942638));
#237754=CARTESIAN_POINT('Ctrl Pts',(-5.53176587633214,15.2,8.90229936639737));
#237755=CARTESIAN_POINT('Ctrl Pts',(-5.53300045106547,15.2,8.90530433364132));
#237756=CARTESIAN_POINT('Ctrl Pts',(-5.53424441464971,15.2,8.90835618651478));
#237757=CARTESIAN_POINT('Ctrl Pts',(-5.53549707355168,15.2,8.91145449468562));
#237758=CARTESIAN_POINT('Ctrl Pts',(-5.53716728530718,15.2,8.91558557196529));
#237759=CARTESIAN_POINT('Ctrl Pts',(-5.53885295407835,15.2,8.91979923571209));
#237760=CARTESIAN_POINT('Ctrl Pts',(-5.54055248061121,15.2,8.92409449043401));
#237761=CARTESIAN_POINT('Ctrl Pts',(-5.5418271254819,15.2,8.9273159314023));
#237762=CARTESIAN_POINT('Ctrl Pts',(-5.54310956685195,15.2,8.93058326810023));
#237763=CARTESIAN_POINT('Ctrl Pts',(-5.54439914988813,15.2,8.93389608706122));
#237764=CARTESIAN_POINT('Ctrl Pts',(-5.54568873292429,15.2,8.9372089060222));
#237765=CARTESIAN_POINT('Ctrl Pts',(-5.54698545873912,15.2,8.94056720793066));
#237766=CARTESIAN_POINT('Ctrl Pts',(-5.548288685858,15.2,8.94397058688728));
#237767=CARTESIAN_POINT('Ctrl Pts',(-5.54959191309526,15.2,8.94737396615303));
#237768=CARTESIAN_POINT('Ctrl Pts',(-5.55090164314147,15.2,8.95082242237315));
#237769=CARTESIAN_POINT('Ctrl Pts',(-5.55221725129677,15.2,8.95431555748214));
#237770=CARTESIAN_POINT('Ctrl Pts',(-5.5537521272987,15.2,8.95839088130004));
#237771=CARTESIAN_POINT('Ctrl Pts',(-5.5552950027022,15.2,8.96252701461721));
#237772=CARTESIAN_POINT('Ctrl Pts',(-5.55684491256358,15.2,8.9667233371162));
#237773=CARTESIAN_POINT('Ctrl Pts',(-5.55817340688563,15.2,8.97032018539255));
#237774=CARTESIAN_POINT('Ctrl Pts',(-5.55950707039987,15.2,8.97396125362317));
#237775=CARTESIAN_POINT('Ctrl Pts',(-5.56084530680633,15.2,8.97764615424259));
#237776=CARTESIAN_POINT('Ctrl Pts',(-5.56218354309126,15.2,8.98133105452729));
#237777=CARTESIAN_POINT('Ctrl Pts',(-5.56352635542562,15.2,8.98505979070993));
#237778=CARTESIAN_POINT('Ctrl Pts',(-5.5648731617161,15.2,8.98883197783986));
#237779=CARTESIAN_POINT('Ctrl Pts',(-5.56599550033229,15.2,8.99197546722902));
#237780=CARTESIAN_POINT('Ctrl Pts',(-5.56712061307784,15.2,8.9951491329666));
#237781=CARTESIAN_POINT('Ctrl Pts',(-5.56824817175838,15.2,8.99835275650824));
#237782=CARTESIAN_POINT('Ctrl Pts',(-5.56937573043893,15.2,9.00155638004988));
#237783=CARTESIAN_POINT('Ctrl Pts',(-5.57050573425664,15.2,9.0047899622257));
#237784=CARTESIAN_POINT('Ctrl Pts',(-5.57163786127567,15.2,9.00805328751836));
#237785=CARTESIAN_POINT('Ctrl Pts',(-5.57276998829469,15.2,9.01131661281102));
#237786=CARTESIAN_POINT('Ctrl Pts',(-5.57390423831316,15.2,9.01460968192142));
#237787=CARTESIAN_POINT('Ctrl Pts',(-5.57504029379936,15.2,9.01793228220072));
#237788=CARTESIAN_POINT('Ctrl Pts',(-5.57617634928556,15.2,9.02125488248005));
#237789=CARTESIAN_POINT('Ctrl Pts',(-5.57731421228004,15.2,9.02460701374191));
#237790=CARTESIAN_POINT('Ctrl Pts',(-5.57845356859958,15.2,9.0279884656879));
#237791=CARTESIAN_POINT('Ctrl Pts',(-5.5795929249191,15.2,9.03136991763389));
#237792=CARTESIAN_POINT('Ctrl Pts',(-5.5807337767866,15.2,9.03478069173103));
#237793=CARTESIAN_POINT('Ctrl Pts',(-5.5818758173993,15.2,9.038220577391));
#237794=CARTESIAN_POINT('Ctrl Pts',(-5.58301785801198,15.2,9.04166046305097));
#237795=CARTESIAN_POINT('Ctrl Pts',(-5.58416108892741,15.2,9.04512946387174));
#237796=CARTESIAN_POINT('Ctrl Pts',(-5.58530520864971,15.2,9.04862737095745));
#237797=CARTESIAN_POINT('Ctrl Pts',(-5.586449328372,15.2,9.05212527804315));
#237798=CARTESIAN_POINT('Ctrl Pts',(-5.58759433792207,15.2,9.05565209412931));
#237799=CARTESIAN_POINT('Ctrl Pts',(-5.58873994111656,15.2,9.05920761371498));
#237800=CARTESIAN_POINT('Ctrl Pts',(-5.58988554418619,15.2,9.06276313291309));
#237801=CARTESIAN_POINT('Ctrl Pts',(-5.59103174240287,15.2,9.06634735731795));
#237802=CARTESIAN_POINT('Ctrl Pts',(-5.59217824533343,15.2,9.06996008476906));
#237803=CARTESIAN_POINT('Ctrl Pts',(-5.59332474838896,15.2,9.07357281261395));
#237804=CARTESIAN_POINT('Ctrl Pts',(-5.59447155673893,15.2,9.0772140417278));
#237805=CARTESIAN_POINT('Ctrl Pts',(-5.59561838410005,15.2,9.08088357700327));
#237806=CARTESIAN_POINT('Ctrl Pts',(-5.59699457700837,15.2,9.0852870195738));
#237807=CARTESIAN_POINT('Ctrl Pts',(-5.59837080003111,15.2,9.08973121982136));
#237808=CARTESIAN_POINT('Ctrl Pts',(-5.59974656892481,15.2,9.09421583687551));
#237809=CARTESIAN_POINT('Ctrl Pts',(-5.60112233769354,15.2,9.09870045352233));
#237810=CARTESIAN_POINT('Ctrl Pts',(-5.60249765169999,15.2,9.10322548737409));
#237811=CARTESIAN_POINT('Ctrl Pts',(-5.60387203948339,15.2,9.10779060345824));
#237812=CARTESIAN_POINT('Ctrl Pts',(-5.60501736267784,15.2,9.11159486699994));
#237813=CARTESIAN_POINT('Ctrl Pts',(-5.60616204281116,15.2,9.1154269623499));
#237814=CARTESIAN_POINT('Ctrl Pts',(-5.60730581024172,15.2,9.11928670172491));
#237815=CARTESIAN_POINT('Ctrl Pts',(-5.60844957767228,15.2,9.12314644109992));
#237816=CARTESIAN_POINT('Ctrl Pts',(-5.60959243311217,15.2,9.12703382065645));
#237817=CARTESIAN_POINT('Ctrl Pts',(-5.61073411228401,15.2,9.13094865178538));
#237818=CARTESIAN_POINT('Ctrl Pts',(-5.61187579145585,15.2,9.13486348291431));
#237819=CARTESIAN_POINT('Ctrl Pts',(-5.61301629485239,15.2,9.1388057639527));
#237820=CARTESIAN_POINT('Ctrl Pts',(-5.61415536228288,15.2,9.14277530700969));
#237821=CARTESIAN_POINT('Ctrl Pts',(-5.61529442971336,15.2,9.14674485006667));
#237822=CARTESIAN_POINT('Ctrl Pts',(-5.61643206056331,15.2,9.15074165550071));
#237823=CARTESIAN_POINT('Ctrl Pts',(-5.61756799979934,15.2,9.15476553432159));
#237824=CARTESIAN_POINT('Ctrl Pts',(-5.61847675111387,15.2,9.15798463711512));
#237825=CARTESIAN_POINT('Ctrl Pts',(-5.61938441988889,15.2,9.16122106714949));
#237826=CARTESIAN_POINT('Ctrl Pts',(-5.62029087836019,15.2,9.16447473004455));
#237827=CARTESIAN_POINT('Ctrl Pts',(-5.62165056625239,15.2,9.16935522505212));
#237828=CARTESIAN_POINT('Ctrl Pts',(-5.62300752557406,15.2,9.17427449394248));
#237829=CARTESIAN_POINT('Ctrl Pts',(-5.62436133164763,15.2,9.17923221579866));
#237830=CARTESIAN_POINT('Ctrl Pts',(-5.62548950331412,15.2,9.18336365045365));
#237831=CARTESIAN_POINT('Ctrl Pts',(-5.62661548441389,15.2,9.1875217914062));
#237832=CARTESIAN_POINT('Ctrl Pts',(-5.62773903191369,15.2,9.19170645279729));
#237833=CARTESIAN_POINT('Ctrl Pts',(-5.62863786984005,15.2,9.19505418163649));
#237834=CARTESIAN_POINT('Ctrl Pts',(-5.6295351495047,15.2,9.19841888476983));
#237835=CARTESIAN_POINT('Ctrl Pts',(-5.63043074949112,15.2,9.20180047006429));
#237836=CARTESIAN_POINT('Ctrl Pts',(-5.63132634959957,15.2,9.20518205581948));
#237837=CARTESIAN_POINT('Ctrl Pts',(-5.63222026960582,15.2,9.20858052142326));
#237838=CARTESIAN_POINT('Ctrl Pts',(-5.63311238715426,15.2,9.21199577733332));
#237839=CARTESIAN_POINT('Ctrl Pts',(-5.63400450458114,15.2,9.21541103277805));
#237840=CARTESIAN_POINT('Ctrl Pts',(-5.63489482026935,15.2,9.21884307782336));
#237841=CARTESIAN_POINT('Ctrl Pts',(-5.63578321491908,15.2,9.22229181998481));
#237842=CARTESIAN_POINT('Ctrl Pts',(-5.63667160968986,15.2,9.22574056261614));
#237843=CARTESIAN_POINT('Ctrl Pts',(-5.63755808296118,15.2,9.22920600362623));
#237844=CARTESIAN_POINT('Ctrl Pts',(-5.63844251588672,15.2,9.23268805171361));
#237845=CARTESIAN_POINT('Ctrl Pts',(-5.63932694869176,15.2,9.23617009932656));
#237846=CARTESIAN_POINT('Ctrl Pts',(-5.64020934203601,15.2,9.23966875339003));
#237847=CARTESIAN_POINT('Ctrl Pts',(-5.64108957868642,15.2,9.24318392421271));
#237848=CARTESIAN_POINT('Ctrl Pts',(-5.64196981545676,15.2,9.24669909551434));
#237849=CARTESIAN_POINT('Ctrl Pts',(-5.64284789486573,15.2,9.25023078388459));
#237850=CARTESIAN_POINT('Ctrl Pts',(-5.64372370307997,15.2,9.25377889852347));
#237851=CARTESIAN_POINT('Ctrl Pts',(-5.64459951117489,15.2,9.25732701267892));
#237852=CARTESIAN_POINT('Ctrl Pts',(-5.6454730461678,15.2,9.26089155483734));
#237853=CARTESIAN_POINT('Ctrl Pts',(-5.64634419614031,15.2,9.26447243322206));
#237854=CARTESIAN_POINT('Ctrl Pts',(-5.6472153462315,15.2,9.26805331209466));
#237855=CARTESIAN_POINT('Ctrl Pts',(-5.64808411009603,15.2,9.27165052980303));
#237856=CARTESIAN_POINT('Ctrl Pts',(-5.64895037558753,15.2,9.27526399577882));
#237857=CARTESIAN_POINT('Ctrl Pts',(-5.64981664096099,15.2,9.27887746126226));
#237858=CARTESIAN_POINT('Ctrl Pts',(-5.6506804058044,15.2,9.2825071761591));
#237859=CARTESIAN_POINT('Ctrl Pts',(-5.6515415625676,15.2,9.28615305163715));
#237860=CARTESIAN_POINT('Ctrl Pts',(-5.65240271944813,15.2,9.28979892761194));
#237861=CARTESIAN_POINT('Ctrl Pts',(-5.65326126612513,15.2,9.29346096444077));
#237862=CARTESIAN_POINT('Ctrl Pts',(-5.65411709300898,15.2,9.29713907443577));
#237863=CARTESIAN_POINT('Ctrl Pts',(-5.65497291977623,15.2,9.30081718392962));
#237864=CARTESIAN_POINT('Ctrl Pts',(-5.65582602800805,15.2,9.30451136711493));
#237865=CARTESIAN_POINT('Ctrl Pts',(-5.65667630682771,15.2,9.30822153714331));
#237866=CARTESIAN_POINT('Ctrl Pts',(-5.65752658576323,15.2,9.3119317076772));
#237867=CARTESIAN_POINT('Ctrl Pts',(-5.65837403603183,15.2,9.31565786302655));
#237868=CARTESIAN_POINT('Ctrl Pts',(-5.65921855096674,15.2,9.31939991950826));
#237869=CARTESIAN_POINT('Ctrl Pts',(-5.66027419457785,15.2,9.32407748985547));
#237870=CARTESIAN_POINT('Ctrl Pts',(-5.66132525094591,15.2,9.32877990219764));
#237871=CARTESIAN_POINT('Ctrl Pts',(-5.6623715144923,15.2,9.33350698951083));
#237872=CARTESIAN_POINT('Ctrl Pts',(-5.663208525261,15.2,9.33728865905223));
#237873=CARTESIAN_POINT('Ctrl Pts',(-5.66404246744295,15.2,9.34108612296205));
#237874=CARTESIAN_POINT('Ctrl Pts',(-5.66487323759757,15.2,9.34489929242647));
#237875=CARTESIAN_POINT('Ctrl Pts',(-5.66591170037575,15.2,9.34966575464665));
#237876=CARTESIAN_POINT('Ctrl Pts',(-5.66694520574292,15.2,9.35445675794985));
#237877=CARTESIAN_POINT('Ctrl Pts',(-5.66797355359056,15.2,9.35927213767007));
#237878=CARTESIAN_POINT('Ctrl Pts',(-5.66900190143821,15.2,9.36408751739028));
#237879=CARTESIAN_POINT('Ctrl Pts',(-5.67002509118624,15.2,9.36892727354967));
#237880=CARTESIAN_POINT('Ctrl Pts',(-5.67104292339023,15.2,9.37379124094371));
#237881=CARTESIAN_POINT('Ctrl Pts',(-5.6718571891978,15.2,9.37768241507101));
#237882=CARTESIAN_POINT('Ctrl Pts',(-5.67266802738892,15.2,9.38158908314757));
#237883=CARTESIAN_POINT('Ctrl Pts',(-5.67347533709937,15.2,9.38551116386238));
#237884=CARTESIAN_POINT('Ctrl Pts',(-5.67428264669981,15.2,9.3894332440428));
#237885=CARTESIAN_POINT('Ctrl Pts',(-5.67508642826762,15.2,9.39337073568389));
#237886=CARTESIAN_POINT('Ctrl Pts',(-5.67588658186924,15.2,9.39732355513697));
#237887=CARTESIAN_POINT('Ctrl Pts',(-5.67688677395304,15.2,9.40226457985725));
#237888=CARTESIAN_POINT('Ctrl Pts',(-5.67788129892583,15.2,9.40722955454376));
#237889=CARTESIAN_POINT('Ctrl Pts',(-5.67886996357909,15.2,9.41221831759741));
#237890=CARTESIAN_POINT('Ctrl Pts',(-5.67985862823235,15.2,9.41720708065103));
#237891=CARTESIAN_POINT('Ctrl Pts',(-5.68084143453745,15.2,9.42221963124322));
#237892=CARTESIAN_POINT('Ctrl Pts',(-5.68181819333666,15.2,9.42725581038204));
#237893=CARTESIAN_POINT('Ctrl Pts',(-5.68259960041862,15.2,9.43128475391268));
#237894=CARTESIAN_POINT('Ctrl Pts',(-5.68337713665193,15.2,9.43532881861802));
#237895=CARTESIAN_POINT('Ctrl Pts',(-5.68415070830494,15.2,9.43938792334023));
#237896=CARTESIAN_POINT('Ctrl Pts',(-5.68492427985255,15.2,9.44344702750939));
#237897=CARTESIAN_POINT('Ctrl Pts',(-5.68569388470651,15.2,9.44752117148939));
#237898=CARTESIAN_POINT('Ctrl Pts',(-5.68645943036657,15.2,9.45161027359803));
#237899=CARTESIAN_POINT('Ctrl Pts',(-5.68722497613093,15.2,9.45569937626379));
#237900=CARTESIAN_POINT('Ctrl Pts',(-5.68798646369477,15.2,9.45980343745117));
#237901=CARTESIAN_POINT('Ctrl Pts',(-5.68874379751725,15.2,9.46392237552773));
#237902=CARTESIAN_POINT('Ctrl Pts',(-5.68950113123655,15.2,9.46804131304309));
#237903=CARTESIAN_POINT('Ctrl Pts',(-5.69025431255785,15.2,9.47217512884282));
#237904=CARTESIAN_POINT('Ctrl Pts',(-5.69100324888595,15.2,9.47632373977996));
#237905=CARTESIAN_POINT('Ctrl Pts',(-5.69193941937261,15.2,9.48150950387533));
#237906=CARTESIAN_POINT('Ctrl Pts',(-5.69286895895104,15.2,9.4867183898619));
#237907=CARTESIAN_POINT('Ctrl Pts',(-5.69379168714604,15.2,9.49195023729061));
#237908=CARTESIAN_POINT('Ctrl Pts',(-5.69452986974229,15.2,9.49613571546169));
#237909=CARTESIAN_POINT('Ctrl Pts',(-5.69526369423808,15.2,9.50033589029004));
#237910=CARTESIAN_POINT('Ctrl Pts',(-5.69599307122557,15.2,9.50455068226113));
#237911=CARTESIAN_POINT('Ctrl Pts',(-5.69672244811368,15.2,9.50876547365795));
#237912=CARTESIAN_POINT('Ctrl Pts',(-5.69744737651016,15.2,9.51299488218227));
#237913=CARTESIAN_POINT('Ctrl Pts',(-5.69816776884062,15.2,9.51723882705605));
#237914=CARTESIAN_POINT('Ctrl Pts',(-5.69888816126923,15.2,9.52148277250805));
#237915=CARTESIAN_POINT('Ctrl Pts',(-5.6996040163502,15.2,9.52574125564758));
#237916=CARTESIAN_POINT('Ctrl Pts',(-5.70031524750007,15.2,9.53001419649159));
#237917=CARTESIAN_POINT('Ctrl Pts',(-5.70102647864994,15.2,9.53428713733559));
#237918=CARTESIAN_POINT('Ctrl Pts',(-5.70173308511039,15.2,9.53857453747291));
#237919=CARTESIAN_POINT('Ctrl Pts',(-5.70243498081483,15.2,9.54287631748663));
#237920=CARTESIAN_POINT('Ctrl Pts',(-5.70331235030193,15.2,9.54825354162458));
#237921=CARTESIAN_POINT('Ctrl Pts',(-5.70418235806398,15.2,9.55365323253357));
#237922=CARTESIAN_POINT('Ctrl Pts',(-5.70504483692893,15.2,9.55907524006574));
#237923=CARTESIAN_POINT('Ctrl Pts',(-5.70573482013369,15.2,9.56341284680066));
#237924=CARTESIAN_POINT('Ctrl Pts',(-5.70641998566856,15.2,9.56776473478698));
#237925=CARTESIAN_POINT('Ctrl Pts',(-5.70710024748341,15.2,9.57213082752493));
#237926=CARTESIAN_POINT('Ctrl Pts',(-5.70778050929827,15.2,9.57649692026288));
#237927=CARTESIAN_POINT('Ctrl Pts',(-5.70845586851532,15.2,9.58087721718862));
#237928=CARTESIAN_POINT('Ctrl Pts',(-5.70912624038468,15.2,9.58527164065176));
#237929=CARTESIAN_POINT('Ctrl Pts',(-5.70962901924102,15.2,9.58856745794975));
#237930=CARTESIAN_POINT('Ctrl Pts',(-5.71012899295645,15.2,9.59187122166135));
#237931=CARTESIAN_POINT('Ctrl Pts',(-5.7106261268379,15.2,9.5951828990824));
#237932=CARTESIAN_POINT('Ctrl Pts',(-5.71112326071935,15.2,9.59849457650346));
#237933=CARTESIAN_POINT('Ctrl Pts',(-5.71161755495503,15.2,9.60181416741631));
#237934=CARTESIAN_POINT('Ctrl Pts',(-5.71210897381193,15.2,9.60514164008776));
#237935=CARTESIAN_POINT('Ctrl Pts',(-5.71260039266882,15.2,9.60846911275921));
#237936=CARTESIAN_POINT('Ctrl Pts',(-5.71308893673439,15.2,9.61180446530472));
#237937=CARTESIAN_POINT('Ctrl Pts',(-5.71357457200841,15.2,9.61514766847493));
#237938=CARTESIAN_POINT('Ctrl Pts',(-5.71406020728244,15.2,9.61849087164514));
#237939=CARTESIAN_POINT('Ctrl Pts',(-5.71454293244824,15.2,9.62184192355668));
#237940=CARTESIAN_POINT('Ctrl Pts',(-5.71502271522273,15.2,9.62520079139228));
#237941=CARTESIAN_POINT('Ctrl Pts',(-5.71566242564682,15.2,9.62967928224652));
#237942=CARTESIAN_POINT('Ctrl Pts',(-5.71629690240109,15.2,9.63417167009037));
#237943=CARTESIAN_POINT('Ctrl Pts',(-5.71692606629968,15.2,9.63867787839555));
#237944=CARTESIAN_POINT('Ctrl Pts',(-5.71771252113005,15.2,9.64431063847005));
#237945=CARTESIAN_POINT('Ctrl Pts',(-5.71849067527367,15.2,9.64996499311837));
#237946=CARTESIAN_POINT('Ctrl Pts',(-5.71926037263409,15.2,9.65564079305067));
#237947=CARTESIAN_POINT('Ctrl Pts',(-5.71972219103355,15.2,9.65904627288631));
#237948=CARTESIAN_POINT('Ctrl Pts',(-5.72018096653319,15.2,9.66245947332991));
#237949=CARTESIAN_POINT('Ctrl Pts',(-5.72063666305803,15.2,9.66588036308127));
#237950=CARTESIAN_POINT('Ctrl Pts',(-5.72109235958287,15.2,9.66930125283264));
#237951=CARTESIAN_POINT('Ctrl Pts',(-5.72154497974812,15.2,9.67272983001225));
#237952=CARTESIAN_POINT('Ctrl Pts',(-5.72199448873382,15.2,9.67616606569472));
#237953=CARTESIAN_POINT('Ctrl Pts',(-5.72259383402086,15.2,9.68074771306325));
#237954=CARTESIAN_POINT('Ctrl Pts',(-5.72318765166253,15.2,9.68534297297453));
#237955=CARTESIAN_POINT('Ctrl Pts',(-5.72377586217057,15.2,9.68995176992973));
#237956=CARTESIAN_POINT('Ctrl Pts',(-5.72436407275876,15.2,9.69456056751288));
#237957=CARTESIAN_POINT('Ctrl Pts',(-5.72494667749919,15.2,9.69918290426117));
#237958=CARTESIAN_POINT('Ctrl Pts',(-5.72552359947508,15.2,9.70381870245827));
#237959=CARTESIAN_POINT('Ctrl Pts',(-5.7259562909177,15.2,9.70729555079027));
#237960=CARTESIAN_POINT('Ctrl Pts',(-5.7263857865021,15.2,9.71077997264693));
#237961=CARTESIAN_POINT('Ctrl Pts',(-5.72681205294523,15.2,9.71427193639443));
#237962=CARTESIAN_POINT('Ctrl Pts',(-5.72723831938836,15.2,9.71776390014192));
#237963=CARTESIAN_POINT('Ctrl Pts',(-5.7276613577794,15.2,9.72126340479125));
#237964=CARTESIAN_POINT('Ctrl Pts',(-5.7280811366605,15.2,9.72477042029647));
#237965=CARTESIAN_POINT('Ctrl Pts',(-5.72850091554159,15.2,9.7282774358017));
#237966=CARTESIAN_POINT('Ctrl Pts',(-5.72891743400788,15.2,9.73179196267777));
#237967=CARTESIAN_POINT('Ctrl Pts',(-5.72933066140999,15.2,9.73531396750714));
#237968=CARTESIAN_POINT('Ctrl Pts',(-5.72974388888716,15.2,9.73883597297633));
#237969=CARTESIAN_POINT('Ctrl Pts',(-5.73015382556341,15.2,9.74236545763926));
#237970=CARTESIAN_POINT('Ctrl Pts',(-5.73056043912205,15.2,9.74590239102933));
#237971=CARTESIAN_POINT('Ctrl Pts',(-5.73110259041047,15.2,9.75061830114518));
#237972=CARTESIAN_POINT('Ctrl Pts',(-5.73163883638298,15.2,9.75534745111485));
#237973=CARTESIAN_POINT('Ctrl Pts',(-5.73216910167334,15.2,9.76008976933737));
#237974=CARTESIAN_POINT('Ctrl Pts',(-5.73256680065918,15.2,9.76364650816578));
#237975=CARTESIAN_POINT('Ctrl Pts',(-5.73296113714526,15.2,9.76721065468546));
#237976=CARTESIAN_POINT('Ctrl Pts',(-5.73335207817319,15.2,9.77078217647135));
#237977=CARTESIAN_POINT('Ctrl Pts',(-5.73387333292443,15.2,9.77554420595173));
#237978=CARTESIAN_POINT('Ctrl Pts',(-5.73438855558706,15.2,9.78031934826769));
#237979=CARTESIAN_POINT('Ctrl Pts',(-5.73489767095043,15.2,9.78510753049486));
#237980=CARTESIAN_POINT('Ctrl Pts',(-5.73527950743827,15.2,9.78869866683903));
#237981=CARTESIAN_POINT('Ctrl Pts',(-5.73565790982831,15.2,9.79229713869466));
#237982=CARTESIAN_POINT('Ctrl Pts',(-5.73603284773307,15.2,9.79590291403834));
#237983=CARTESIAN_POINT('Ctrl Pts',(-5.73640778563784,15.2,9.79950868938202));
#237984=CARTESIAN_POINT('Ctrl Pts',(-5.73677925878964,15.2,9.80312176930429));
#237985=CARTESIAN_POINT('Ctrl Pts',(-5.73714723769324,15.2,9.80674212263043));
#237986=CARTESIAN_POINT('Ctrl Pts',(-5.73751521659685,15.2,9.81036247595658));
#237987=CARTESIAN_POINT('Ctrl Pts',(-5.73787970076735,15.2,9.8139901034239));
#237988=CARTESIAN_POINT('Ctrl Pts',(-5.73824066167139,15.2,9.81762497379087));
#237989=CARTESIAN_POINT('Ctrl Pts',(-5.738601622641,15.2,9.82125984481817));
#237990=CARTESIAN_POINT('Ctrl Pts',(-5.73895905982627,15.2,9.82490195918079));
#237991=CARTESIAN_POINT('Ctrl Pts',(-5.73931294383556,15.2,9.82855128625383));
#237992=CARTESIAN_POINT('Ctrl Pts',(-5.73966682778055,15.2,9.83220061266392));
#237993=CARTESIAN_POINT('Ctrl Pts',(-5.74001715879615,15.2,9.83585715292475));
#237994=CARTESIAN_POINT('Ctrl Pts',(-5.74036390684213,15.2,9.83952087493385));
#237995=CARTESIAN_POINT('Ctrl Pts',(-5.74094182027308,15.2,9.84562707850421));
#237996=CARTESIAN_POINT('Ctrl Pts',(-5.7415097845072,15.2,9.8517532334744));
#237997=CARTESIAN_POINT('Ctrl Pts',(-5.74206766283972,15.2,9.85789919854551));
#237998=CARTESIAN_POINT('Ctrl Pts',(-5.74240238982707,15.2,9.86158677745418));
#237999=CARTESIAN_POINT('Ctrl Pts',(-5.74273348638127,15.2,9.86528148937079));
#238000=CARTESIAN_POINT('Ctrl Pts',(-5.74306092528571,15.2,9.86898330415355));
#238001=CARTESIAN_POINT('Ctrl Pts',(-5.74338836419016,15.2,9.8726851189363));
#238002=CARTESIAN_POINT('Ctrl Pts',(-5.74371214432723,15.2,9.8763940359381));
#238003=CARTESIAN_POINT('Ctrl Pts',(-5.74403223727537,15.2,9.88011002473664));
#238004=CARTESIAN_POINT('Ctrl Pts',(-5.7444590278535,15.2,9.88506467624303));
#238005=CARTESIAN_POINT('Ctrl Pts',(-5.74487926264892,15.2,9.89003189909693));
#238006=CARTESIAN_POINT('Ctrl Pts',(-5.74529287394912,15.2,9.89501162141076));
#238007=CARTESIAN_POINT('Ctrl Pts',(-5.74560308249471,15.2,9.89874641399425));
#238008=CARTESIAN_POINT('Ctrl Pts',(-5.74590956580592,15.2,9.90248823867143));
#238009=CARTESIAN_POINT('Ctrl Pts',(-5.74621229984941,15.2,9.90623706775886));
#238010=CARTESIAN_POINT('Ctrl Pts',(-5.74651503383789,15.2,9.90998589616525));
#238011=CARTESIAN_POINT('Ctrl Pts',(-5.74681401800992,15.2,9.91374173087964));
#238012=CARTESIAN_POINT('Ctrl Pts',(-5.74710922349887,15.2,9.91750453866021));
#238013=CARTESIAN_POINT('Ctrl Pts',(-5.74740442898781,15.2,9.92126734644077));
#238014=CARTESIAN_POINT('Ctrl Pts',(-5.7476958564595,15.2,9.92503712840675));
#238015=CARTESIAN_POINT('Ctrl Pts',(-5.74798346995034,15.2,9.92881384624504));
#238016=CARTESIAN_POINT('Ctrl Pts',(-5.74836695458738,15.2,9.93384946980072));
#238017=CARTESIAN_POINT('Ctrl Pts',(-5.74874365740803,15.2,9.93889742376812));
#238018=CARTESIAN_POINT('Ctrl Pts',(-5.74911352715627,15.2,9.94395764863093));
#238019=CARTESIAN_POINT('Ctrl Pts',(-5.7494833969549,15.2,9.94901787418319));
#238020=CARTESIAN_POINT('Ctrl Pts',(-5.74984644090299,15.2,9.95409037794774));
#238021=CARTESIAN_POINT('Ctrl Pts',(-5.75020264100006,15.2,9.95917514599999));
#238022=CARTESIAN_POINT('Ctrl Pts',(-4.57383771200006,15.2,9.31239140099999));
#238023=CARTESIAN_POINT('Ctrl Pts',(-4.57383771200006,11.6,9.31239140099999));
#238024=CARTESIAN_POINT('Ctrl Pts',(-4.57392774300006,15.2,9.31254071599999));
#238025=CARTESIAN_POINT('Ctrl Pts',(-4.57392774300006,11.6,9.31254071599999));
#238026=CARTESIAN_POINT('Ctrl Pts',(-4.57411102300005,15.2,9.31284451799998));
#238027=CARTESIAN_POINT('Ctrl Pts',(-4.57411102300005,11.6,9.31284451799998));
#238028=CARTESIAN_POINT('Ctrl Pts',(-4.57438896300006,15.2,9.31330471299999));
#238029=CARTESIAN_POINT('Ctrl Pts',(-4.57438896300006,11.6,9.31330471299999));
#238030=CARTESIAN_POINT('Ctrl Pts',(-4.57476383600006,15.2,9.31392435799999));
#238031=CARTESIAN_POINT('Ctrl Pts',(-4.57476383600006,11.6,9.31392435799999));
#238032=CARTESIAN_POINT('Ctrl Pts',(-4.57523877600006,15.2,9.31470764399998));
#238033=CARTESIAN_POINT('Ctrl Pts',(-4.57523877600006,11.6,9.31470764399998));
#238034=CARTESIAN_POINT('Ctrl Pts',(-4.57572221400006,15.2,9.31550313999999));
#238035=CARTESIAN_POINT('Ctrl Pts',(-4.57572221400006,11.6,9.31550313999999));
#238036=CARTESIAN_POINT('Ctrl Pts',(-4.57621139800006,15.2,9.31630627599999));
#238037=CARTESIAN_POINT('Ctrl Pts',(-4.57621139800006,11.6,9.31630627599999));
#238038=CARTESIAN_POINT('Ctrl Pts',(-4.57670633000006,15.2,9.31711702099999));
#238039=CARTESIAN_POINT('Ctrl Pts',(-4.57670633000006,11.6,9.31711702099999));
#238040=CARTESIAN_POINT('Ctrl Pts',(-4.57720701300006,15.2,9.31793534099998));
#238041=CARTESIAN_POINT('Ctrl Pts',(-4.57720701300006,11.6,9.31793534099998));
#238042=CARTESIAN_POINT('Ctrl Pts',(-4.57771344700006,15.2,9.31876120399998));
#238043=CARTESIAN_POINT('Ctrl Pts',(-4.57771344700006,11.6,9.31876120399998));
#238044=CARTESIAN_POINT('Ctrl Pts',(-4.57822563400006,15.2,9.31959457899998));
#238045=CARTESIAN_POINT('Ctrl Pts',(-4.57822563400006,11.6,9.31959457899998));
#238046=CARTESIAN_POINT('Ctrl Pts',(-4.57874357500006,15.2,9.32043543399999));
#238047=CARTESIAN_POINT('Ctrl Pts',(-4.57874357500006,11.6,9.32043543399999));
#238048=CARTESIAN_POINT('Ctrl Pts',(-4.57926727100006,15.2,9.32128373599999));
#238049=CARTESIAN_POINT('Ctrl Pts',(-4.57926727100006,11.6,9.32128373599999));
#238050=CARTESIAN_POINT('Ctrl Pts',(-4.57979672400006,15.2,9.32213945399998));
#238051=CARTESIAN_POINT('Ctrl Pts',(-4.57979672400006,11.6,9.32213945399998));
#238052=CARTESIAN_POINT('Ctrl Pts',(-4.58033193500006,15.2,9.32300255699998));
#238053=CARTESIAN_POINT('Ctrl Pts',(-4.58033193500006,11.6,9.32300255699998));
#238054=CARTESIAN_POINT('Ctrl Pts',(-4.58087290500006,15.2,9.32387301399999));
#238055=CARTESIAN_POINT('Ctrl Pts',(-4.58087290500006,11.6,9.32387301399999));
#238056=CARTESIAN_POINT('Ctrl Pts',(-4.58141963700006,15.2,9.32475079299999));
#238057=CARTESIAN_POINT('Ctrl Pts',(-4.58141963700006,11.6,9.32475079299999));
#238058=CARTESIAN_POINT('Ctrl Pts',(-4.58197213000005,15.2,9.32563586399999));
#238059=CARTESIAN_POINT('Ctrl Pts',(-4.58197213000005,11.6,9.32563586399999));
#238060=CARTESIAN_POINT('Ctrl Pts',(-4.58253038600006,15.2,9.32652819599999));
#238061=CARTESIAN_POINT('Ctrl Pts',(-4.58253038600006,11.6,9.32652819599999));
#238062=CARTESIAN_POINT('Ctrl Pts',(-4.58309440700006,15.2,9.32742775599999));
#238063=CARTESIAN_POINT('Ctrl Pts',(-4.58309440700006,11.6,9.32742775599999));
#238064=CARTESIAN_POINT('Ctrl Pts',(-4.58366419400006,15.2,9.32833451799999));
#238065=CARTESIAN_POINT('Ctrl Pts',(-4.58366419400006,11.6,9.32833451799999));
#238066=CARTESIAN_POINT('Ctrl Pts',(-4.58423974600006,15.2,9.32924844799999));
#238067=CARTESIAN_POINT('Ctrl Pts',(-4.58423974600006,11.6,9.32924844799999));
#238068=CARTESIAN_POINT('Ctrl Pts',(-4.58482106700006,15.2,9.33016951699998));
#238069=CARTESIAN_POINT('Ctrl Pts',(-4.58482106700006,11.6,9.33016951699998));
#238070=CARTESIAN_POINT('Ctrl Pts',(-4.58540815800006,15.2,9.33109769499998));
#238071=CARTESIAN_POINT('Ctrl Pts',(-4.58540815800006,11.6,9.33109769499998));
#238072=CARTESIAN_POINT('Ctrl Pts',(-4.58600101700006,15.2,9.33203295199998));
#238073=CARTESIAN_POINT('Ctrl Pts',(-4.58600101700006,11.6,9.33203295199998));
#238074=CARTESIAN_POINT('Ctrl Pts',(-4.58659964900006,15.2,9.33297525799999));
#238075=CARTESIAN_POINT('Ctrl Pts',(-4.58659964900006,11.6,9.33297525799999));
#238076=CARTESIAN_POINT('Ctrl Pts',(-4.58720405300006,15.2,9.33392458399998));
#238077=CARTESIAN_POINT('Ctrl Pts',(-4.58720405300006,11.6,9.33392458399998));
#238078=CARTESIAN_POINT('Ctrl Pts',(-4.58781423100006,15.2,9.33488089999998));
#238079=CARTESIAN_POINT('Ctrl Pts',(-4.58781423100006,11.6,9.33488089999998));
#238080=CARTESIAN_POINT('Ctrl Pts',(-4.58843018200006,15.2,9.33584417599998));
#238081=CARTESIAN_POINT('Ctrl Pts',(-4.58843018200006,11.6,9.33584417599998));
#238082=CARTESIAN_POINT('Ctrl Pts',(-4.58905191000006,15.2,9.33681438399999));
#238083=CARTESIAN_POINT('Ctrl Pts',(-4.58905191000006,11.6,9.33681438399999));
#238084=CARTESIAN_POINT('Ctrl Pts',(-4.58967941300005,15.2,9.33779149299999));
#238085=CARTESIAN_POINT('Ctrl Pts',(-4.58967941300005,11.6,9.33779149299999));
#238086=CARTESIAN_POINT('Ctrl Pts',(-4.59031269500006,15.2,9.33877547699998));
#238087=CARTESIAN_POINT('Ctrl Pts',(-4.59031269500006,11.6,9.33877547699998));
#238088=CARTESIAN_POINT('Ctrl Pts',(-4.59095175400006,15.2,9.33976630499998));
#238089=CARTESIAN_POINT('Ctrl Pts',(-4.59095175400006,11.6,9.33976630499998));
#238090=CARTESIAN_POINT('Ctrl Pts',(-4.59159659200005,15.2,9.34076394799998));
#238091=CARTESIAN_POINT('Ctrl Pts',(-4.59159659200005,11.6,9.34076394799998));
#238092=CARTESIAN_POINT('Ctrl Pts',(-4.59224721200005,15.2,9.34176837899999));
#238093=CARTESIAN_POINT('Ctrl Pts',(-4.59224721200005,11.6,9.34176837899999));
#238094=CARTESIAN_POINT('Ctrl Pts',(-4.59290361300006,15.2,9.34277956799999));
#238095=CARTESIAN_POINT('Ctrl Pts',(-4.59290361300006,11.6,9.34277956799999));
#238096=CARTESIAN_POINT('Ctrl Pts',(-4.59356579600006,15.2,9.34379748799999));
#238097=CARTESIAN_POINT('Ctrl Pts',(-4.59356579600006,11.6,9.34379748799999));
#238098=CARTESIAN_POINT('Ctrl Pts',(-4.59423376100006,15.2,9.34482210999998));
#238099=CARTESIAN_POINT('Ctrl Pts',(-4.59423376100006,11.6,9.34482210999998));
#238100=CARTESIAN_POINT('Ctrl Pts',(-4.59490751000006,15.2,9.34585340599998));
#238101=CARTESIAN_POINT('Ctrl Pts',(-4.59490751000006,11.6,9.34585340599998));
#238102=CARTESIAN_POINT('Ctrl Pts',(-4.59558704400005,15.2,9.34689134799999));
#238103=CARTESIAN_POINT('Ctrl Pts',(-4.59558704400005,11.6,9.34689134799999));
#238104=CARTESIAN_POINT('Ctrl Pts',(-4.59627236400006,15.2,9.34793590899999));
#238105=CARTESIAN_POINT('Ctrl Pts',(-4.59627236400006,11.6,9.34793590899999));
#238106=CARTESIAN_POINT('Ctrl Pts',(-4.59696347000006,15.2,9.34898706099998));
#238107=CARTESIAN_POINT('Ctrl Pts',(-4.59696347000006,11.6,9.34898706099998));
#238108=CARTESIAN_POINT('Ctrl Pts',(-4.59766036300006,15.2,9.35004477499999));
#238109=CARTESIAN_POINT('Ctrl Pts',(-4.59766036300006,11.6,9.35004477499999));
#238110=CARTESIAN_POINT('Ctrl Pts',(-4.59836304400006,15.2,9.35110902499999));
#238111=CARTESIAN_POINT('Ctrl Pts',(-4.59836304400006,11.6,9.35110902499999));
#238112=CARTESIAN_POINT('Ctrl Pts',(-4.59907151400006,15.2,9.35217978299999));
#238113=CARTESIAN_POINT('Ctrl Pts',(-4.59907151400006,11.6,9.35217978299999));
#238114=CARTESIAN_POINT('Ctrl Pts',(-4.59978577200006,15.2,9.35325702199999));
#238115=CARTESIAN_POINT('Ctrl Pts',(-4.59978577200006,11.6,9.35325702199999));
#238116=CARTESIAN_POINT('Ctrl Pts',(-4.60050582200005,15.2,9.35434071699999));
#238117=CARTESIAN_POINT('Ctrl Pts',(-4.60050582200005,11.6,9.35434071699999));
#238118=CARTESIAN_POINT('Ctrl Pts',(-4.60123166200006,15.2,9.35543083699999));
#238119=CARTESIAN_POINT('Ctrl Pts',(-4.60123166200006,11.6,9.35543083699999));
#238120=CARTESIAN_POINT('Ctrl Pts',(-4.60196329300006,15.2,9.35652735799999));
#238121=CARTESIAN_POINT('Ctrl Pts',(-4.60196329300006,11.6,9.35652735799999));
#238122=CARTESIAN_POINT('Ctrl Pts',(-4.60270071600006,15.2,9.35763025299998));
#238123=CARTESIAN_POINT('Ctrl Pts',(-4.60270071600006,11.6,9.35763025299998));
#238124=CARTESIAN_POINT('Ctrl Pts',(-4.60344393200006,15.2,9.35873949499998));
#238125=CARTESIAN_POINT('Ctrl Pts',(-4.60344393200006,11.6,9.35873949499998));
#238126=CARTESIAN_POINT('Ctrl Pts',(-4.60419294300006,15.2,9.35985505699998));
#238127=CARTESIAN_POINT('Ctrl Pts',(-4.60419294300006,11.6,9.35985505699998));
#238128=CARTESIAN_POINT('Ctrl Pts',(-4.60494774600006,15.2,9.36097691299998));
#238129=CARTESIAN_POINT('Ctrl Pts',(-4.60494774600006,11.6,9.36097691299998));
#238130=CARTESIAN_POINT('Ctrl Pts',(-4.60570834500006,15.2,9.36210503599998));
#238131=CARTESIAN_POINT('Ctrl Pts',(-4.60570834500006,11.6,9.36210503599998));
#238132=CARTESIAN_POINT('Ctrl Pts',(-4.60647473900006,15.2,9.36323940099999));
#238133=CARTESIAN_POINT('Ctrl Pts',(-4.60647473900006,11.6,9.36323940099999));
#238134=CARTESIAN_POINT('Ctrl Pts',(-4.60724692800006,15.2,9.36437998099999));
#238135=CARTESIAN_POINT('Ctrl Pts',(-4.60724692800006,11.6,9.36437998099999));
#238136=CARTESIAN_POINT('Ctrl Pts',(-4.60802491400006,15.2,9.36552675199999));
#238137=CARTESIAN_POINT('Ctrl Pts',(-4.60802491400006,11.6,9.36552675199999));
#238138=CARTESIAN_POINT('Ctrl Pts',(-4.60880869800006,15.2,9.36667968599998));
#238139=CARTESIAN_POINT('Ctrl Pts',(-4.60880869800006,11.6,9.36667968599998));
#238140=CARTESIAN_POINT('Ctrl Pts',(-4.60959827800006,15.2,9.36783875799998));
#238141=CARTESIAN_POINT('Ctrl Pts',(-4.60959827800006,11.6,9.36783875799998));
#238142=CARTESIAN_POINT('Ctrl Pts',(-4.61039365600006,15.2,9.36900394299998));
#238143=CARTESIAN_POINT('Ctrl Pts',(-4.61039365600006,11.6,9.36900394299998));
#238144=CARTESIAN_POINT('Ctrl Pts',(-4.61119483300005,15.2,9.37017521399999));
#238145=CARTESIAN_POINT('Ctrl Pts',(-4.61119483300005,11.6,9.37017521399999));
#238146=CARTESIAN_POINT('Ctrl Pts',(-4.61200180900006,15.2,9.37135254599998));
#238147=CARTESIAN_POINT('Ctrl Pts',(-4.61200180900006,11.6,9.37135254599998));
#238148=CARTESIAN_POINT('Ctrl Pts',(-4.61281458500006,15.2,9.37253591599998));
#238149=CARTESIAN_POINT('Ctrl Pts',(-4.61281458500006,11.6,9.37253591599998));
#238150=CARTESIAN_POINT('Ctrl Pts',(-4.61363316000006,15.2,9.37372529599998));
#238151=CARTESIAN_POINT('Ctrl Pts',(-4.61363316000006,11.6,9.37372529599998));
#238152=CARTESIAN_POINT('Ctrl Pts',(-4.61445753500006,15.2,9.37492066099999));
#238153=CARTESIAN_POINT('Ctrl Pts',(-4.61445753500006,11.6,9.37492066099999));
#238154=CARTESIAN_POINT('Ctrl Pts',(-4.61528771100006,15.2,9.37612198899998));
#238155=CARTESIAN_POINT('Ctrl Pts',(-4.61528771100006,11.6,9.37612198899998));
#238156=CARTESIAN_POINT('Ctrl Pts',(-4.61612368800006,15.2,9.37732925099999));
#238157=CARTESIAN_POINT('Ctrl Pts',(-4.61612368800006,11.6,9.37732925099999));
#238158=CARTESIAN_POINT('Ctrl Pts',(-4.61696546700006,15.2,9.37854242499998));
#238159=CARTESIAN_POINT('Ctrl Pts',(-4.61696546700006,11.6,9.37854242499998));
#238160=CARTESIAN_POINT('Ctrl Pts',(-4.61781304700006,15.2,9.37976148599999));
#238161=CARTESIAN_POINT('Ctrl Pts',(-4.61781304700006,11.6,9.37976148599999));
#238162=CARTESIAN_POINT('Ctrl Pts',(-4.61866643000006,15.2,9.38098640999998));
#238163=CARTESIAN_POINT('Ctrl Pts',(-4.61866643000006,11.6,9.38098640999998));
#238164=CARTESIAN_POINT('Ctrl Pts',(-4.61952561600006,15.2,9.38221716999998));
#238165=CARTESIAN_POINT('Ctrl Pts',(-4.61952561600006,11.6,9.38221716999998));
#238166=CARTESIAN_POINT('Ctrl Pts',(-4.62039060400006,15.2,9.38345374299999));
#238167=CARTESIAN_POINT('Ctrl Pts',(-4.62039060400006,11.6,9.38345374299999));
#238168=CARTESIAN_POINT('Ctrl Pts',(-4.62126139600006,15.2,9.38469610499999));
#238169=CARTESIAN_POINT('Ctrl Pts',(-4.62126139600006,11.6,9.38469610499999));
#238170=CARTESIAN_POINT('Ctrl Pts',(-4.62213799200006,15.2,9.38594423299998));
#238171=CARTESIAN_POINT('Ctrl Pts',(-4.62213799200006,11.6,9.38594423299998));
#238172=CARTESIAN_POINT('Ctrl Pts',(-4.62302039000006,15.2,9.38719810099998));
#238173=CARTESIAN_POINT('Ctrl Pts',(-4.62302039000006,11.6,9.38719810099998));
#238174=CARTESIAN_POINT('Ctrl Pts',(-4.62390859300006,15.2,9.38845768599998));
#238175=CARTESIAN_POINT('Ctrl Pts',(-4.62390859300006,11.6,9.38845768599998));
#238176=CARTESIAN_POINT('Ctrl Pts',(-4.62480260100006,15.2,9.38972296299998));
#238177=CARTESIAN_POINT('Ctrl Pts',(-4.62480260100006,11.6,9.38972296299998));
#238178=CARTESIAN_POINT('Ctrl Pts',(-4.62570241200006,15.2,9.39099390799999));
#238179=CARTESIAN_POINT('Ctrl Pts',(-4.62570241200006,11.6,9.39099390799999));
#238180=CARTESIAN_POINT('Ctrl Pts',(-4.62660802900006,15.2,9.39227049999998));
#238181=CARTESIAN_POINT('Ctrl Pts',(-4.62660802900006,11.6,9.39227049999998));
#238182=CARTESIAN_POINT('Ctrl Pts',(-4.62751945100006,15.2,9.39355271299998));
#238183=CARTESIAN_POINT('Ctrl Pts',(-4.62751945100006,11.6,9.39355271299998));
#238184=CARTESIAN_POINT('Ctrl Pts',(-4.62843667800006,15.2,9.39484052499999));
#238185=CARTESIAN_POINT('Ctrl Pts',(-4.62843667800006,11.6,9.39484052499999));
#238186=CARTESIAN_POINT('Ctrl Pts',(-4.62935971000006,15.2,9.39613391099999));
#238187=CARTESIAN_POINT('Ctrl Pts',(-4.62935971000006,11.6,9.39613391099999));
#238188=CARTESIAN_POINT('Ctrl Pts',(-4.63028854800006,15.2,9.39743284799999));
#238189=CARTESIAN_POINT('Ctrl Pts',(-4.63028854800006,11.6,9.39743284799999));
#238190=CARTESIAN_POINT('Ctrl Pts',(-4.63122319200005,15.2,9.39873731299999));
#238191=CARTESIAN_POINT('Ctrl Pts',(-4.63122319200005,11.6,9.39873731299999));
#238192=CARTESIAN_POINT('Ctrl Pts',(-4.63216364200006,15.2,9.40004728399998));
#238193=CARTESIAN_POINT('Ctrl Pts',(-4.63216364200006,11.6,9.40004728399998));
#238194=CARTESIAN_POINT('Ctrl Pts',(-4.63310989700005,15.2,9.40136273599999));
#238195=CARTESIAN_POINT('Ctrl Pts',(-4.63310989700005,11.6,9.40136273599999));
#238196=CARTESIAN_POINT('Ctrl Pts',(-4.63406195900006,15.2,9.40268364799999));
#238197=CARTESIAN_POINT('Ctrl Pts',(-4.63406195900006,11.6,9.40268364799999));
#238198=CARTESIAN_POINT('Ctrl Pts',(-4.63501982700006,15.2,9.40400999499998));
#238199=CARTESIAN_POINT('Ctrl Pts',(-4.63501982700006,11.6,9.40400999499998));
#238200=CARTESIAN_POINT('Ctrl Pts',(-4.63598350100006,15.2,9.40534175599998));
#238201=CARTESIAN_POINT('Ctrl Pts',(-4.63598350100006,11.6,9.40534175599998));
#238202=CARTESIAN_POINT('Ctrl Pts',(-4.63695298200006,15.2,9.40667890699999));
#238203=CARTESIAN_POINT('Ctrl Pts',(-4.63695298200006,11.6,9.40667890699999));
#238204=CARTESIAN_POINT('Ctrl Pts',(-4.63792827000006,15.2,9.40802142699999));
#238205=CARTESIAN_POINT('Ctrl Pts',(-4.63792827000006,11.6,9.40802142699999));
#238206=CARTESIAN_POINT('Ctrl Pts',(-4.63890936300006,15.2,9.40936929099998));
#238207=CARTESIAN_POINT('Ctrl Pts',(-4.63890936300006,11.6,9.40936929099998));
#238208=CARTESIAN_POINT('Ctrl Pts',(-4.63989626400005,15.2,9.41072247999998));
#238209=CARTESIAN_POINT('Ctrl Pts',(-4.63989626400005,11.6,9.41072247999998));
#238210=CARTESIAN_POINT('Ctrl Pts',(-4.64088897100006,15.2,9.41208096799999));
#238211=CARTESIAN_POINT('Ctrl Pts',(-4.64088897100006,11.6,9.41208096799999));
#238212=CARTESIAN_POINT('Ctrl Pts',(-4.64188748400006,15.2,9.41344473399998));
#238213=CARTESIAN_POINT('Ctrl Pts',(-4.64188748400006,11.6,9.41344473399998));
#238214=CARTESIAN_POINT('Ctrl Pts',(-4.64289180500006,15.2,9.41481375799999));
#238215=CARTESIAN_POINT('Ctrl Pts',(-4.64289180500006,11.6,9.41481375799999));
#238216=CARTESIAN_POINT('Ctrl Pts',(-4.64390193100006,15.2,9.41618801499999));
#238217=CARTESIAN_POINT('Ctrl Pts',(-4.64390193100006,11.6,9.41618801499999));
#238218=CARTESIAN_POINT('Ctrl Pts',(-4.64491786500006,15.2,9.41756748299999));
#238219=CARTESIAN_POINT('Ctrl Pts',(-4.64491786500006,11.6,9.41756748299999));
#238220=CARTESIAN_POINT('Ctrl Pts',(-4.64593960400006,15.2,9.41895214299999));
#238221=CARTESIAN_POINT('Ctrl Pts',(-4.64593960400006,11.6,9.41895214299999));
#238222=CARTESIAN_POINT('Ctrl Pts',(-4.64696715100006,15.2,9.42034196999998));
#238223=CARTESIAN_POINT('Ctrl Pts',(-4.64696715100006,11.6,9.42034196999998));
#238224=CARTESIAN_POINT('Ctrl Pts',(-4.64800050300005,15.2,9.42173694399998));
#238225=CARTESIAN_POINT('Ctrl Pts',(-4.64800050300005,11.6,9.42173694399998));
#238226=CARTESIAN_POINT('Ctrl Pts',(-4.64903966300006,15.2,9.42313704299998));
#238227=CARTESIAN_POINT('Ctrl Pts',(-4.64903966300006,11.6,9.42313704299998));
#238228=CARTESIAN_POINT('Ctrl Pts',(-4.65008462800006,15.2,9.42454224399999));
#238229=CARTESIAN_POINT('Ctrl Pts',(-4.65008462800006,11.6,9.42454224399999));
#238230=CARTESIAN_POINT('Ctrl Pts',(-4.65113540000006,15.2,9.42595252799999));
#238231=CARTESIAN_POINT('Ctrl Pts',(-4.65113540000006,11.6,9.42595252799999));
#238232=CARTESIAN_POINT('Ctrl Pts',(-4.65219197700006,15.2,9.42736787099999));
#238233=CARTESIAN_POINT('Ctrl Pts',(-4.65219197700006,11.6,9.42736787099999));
#238234=CARTESIAN_POINT('Ctrl Pts',(-4.65325436000006,15.2,9.42878825399998));
#238235=CARTESIAN_POINT('Ctrl Pts',(-4.65325436000006,11.6,9.42878825399998));
#238236=CARTESIAN_POINT('Ctrl Pts',(-4.65432255000006,15.2,9.43021365399999));
#238237=CARTESIAN_POINT('Ctrl Pts',(-4.65432255000006,11.6,9.43021365399999));
#238238=CARTESIAN_POINT('Ctrl Pts',(-4.65539654500006,15.2,9.43164404899999));
#238239=CARTESIAN_POINT('Ctrl Pts',(-4.65539654500006,11.6,9.43164404899999));
#238240=CARTESIAN_POINT('Ctrl Pts',(-4.65647634500006,15.2,9.43307941999999));
#238241=CARTESIAN_POINT('Ctrl Pts',(-4.65647634500006,11.6,9.43307941999999));
#238242=CARTESIAN_POINT('Ctrl Pts',(-4.65756195100006,15.2,9.43451974499999));
#238243=CARTESIAN_POINT('Ctrl Pts',(-4.65756195100006,11.6,9.43451974499999));
#238244=CARTESIAN_POINT('Ctrl Pts',(-4.65865336200006,15.2,9.43596500399998));
#238245=CARTESIAN_POINT('Ctrl Pts',(-4.65865336200006,11.6,9.43596500399998));
#238246=CARTESIAN_POINT('Ctrl Pts',(-4.65975057800006,15.2,9.43741517399998));
#238247=CARTESIAN_POINT('Ctrl Pts',(-4.65975057800006,11.6,9.43741517399998));
#238248=CARTESIAN_POINT('Ctrl Pts',(-4.66085359800006,15.2,9.43887023499999));
#238249=CARTESIAN_POINT('Ctrl Pts',(-4.66085359800006,11.6,9.43887023499999));
#238250=CARTESIAN_POINT('Ctrl Pts',(-4.66196242400006,15.2,9.44033016699999));
#238251=CARTESIAN_POINT('Ctrl Pts',(-4.66196242400006,11.6,9.44033016699999));
#238252=CARTESIAN_POINT('Ctrl Pts',(-4.66307705300006,15.2,9.44179494899998));
#238253=CARTESIAN_POINT('Ctrl Pts',(-4.66307705300006,11.6,9.44179494899998));
#238254=CARTESIAN_POINT('Ctrl Pts',(-4.66419748600006,15.2,9.44326456099999));
#238255=CARTESIAN_POINT('Ctrl Pts',(-4.66419748600006,11.6,9.44326456099999));
#238256=CARTESIAN_POINT('Ctrl Pts',(-4.66532372300006,15.2,9.44473897999998));
#238257=CARTESIAN_POINT('Ctrl Pts',(-4.66532372300006,11.6,9.44473897999998));
#238258=CARTESIAN_POINT('Ctrl Pts',(-4.66645576400006,15.2,9.44621818799998));
#238259=CARTESIAN_POINT('Ctrl Pts',(-4.66645576400006,11.6,9.44621818799998));
#238260=CARTESIAN_POINT('Ctrl Pts',(-4.66759360800006,15.2,9.44770216299998));
#238261=CARTESIAN_POINT('Ctrl Pts',(-4.66759360800006,11.6,9.44770216299998));
#238262=CARTESIAN_POINT('Ctrl Pts',(-4.66873725400006,15.2,9.44919088699999));
#238263=CARTESIAN_POINT('Ctrl Pts',(-4.66873725400006,11.6,9.44919088699999));
#238264=CARTESIAN_POINT('Ctrl Pts',(-4.66988670400006,15.2,9.45068433699999));
#238265=CARTESIAN_POINT('Ctrl Pts',(-4.66988670400006,11.6,9.45068433699999));
#238266=CARTESIAN_POINT('Ctrl Pts',(-4.67104195500006,15.2,9.45218249399998));
#238267=CARTESIAN_POINT('Ctrl Pts',(-4.67104195500006,11.6,9.45218249399998));
#238268=CARTESIAN_POINT('Ctrl Pts',(-4.67220300900006,15.2,9.45368533799999));
#238269=CARTESIAN_POINT('Ctrl Pts',(-4.67220300900006,11.6,9.45368533799999));
#238270=CARTESIAN_POINT('Ctrl Pts',(-4.67336986400006,15.2,9.45519284899999));
#238271=CARTESIAN_POINT('Ctrl Pts',(-4.67336986400006,11.6,9.45519284899999));
#238272=CARTESIAN_POINT('Ctrl Pts',(-4.67454252000006,15.2,9.45670500699999));
#238273=CARTESIAN_POINT('Ctrl Pts',(-4.67454252000006,11.6,9.45670500699999));
#238274=CARTESIAN_POINT('Ctrl Pts',(-4.67572097800006,15.2,9.45822179199999));
#238275=CARTESIAN_POINT('Ctrl Pts',(-4.67572097800006,11.6,9.45822179199999));
#238276=CARTESIAN_POINT('Ctrl Pts',(-4.67690523600006,15.2,9.45974318399998));
#238277=CARTESIAN_POINT('Ctrl Pts',(-4.67690523600006,11.6,9.45974318399998));
#238278=CARTESIAN_POINT('Ctrl Pts',(-4.67809529500006,15.2,9.46126916199999));
#238279=CARTESIAN_POINT('Ctrl Pts',(-4.67809529500006,11.6,9.46126916199999));
#238280=CARTESIAN_POINT('Ctrl Pts',(-4.67929115300006,15.2,9.46279970999999));
#238281=CARTESIAN_POINT('Ctrl Pts',(-4.67929115300006,11.6,9.46279970999999));
#238282=CARTESIAN_POINT('Ctrl Pts',(-4.68049281000006,15.2,9.46433480499999));
#238283=CARTESIAN_POINT('Ctrl Pts',(-4.68049281000006,11.6,9.46433480499999));
#238284=CARTESIAN_POINT('Ctrl Pts',(-4.68170026700006,15.2,9.46587442799999));
#238285=CARTESIAN_POINT('Ctrl Pts',(-4.68170026700006,11.6,9.46587442799999));
#238286=CARTESIAN_POINT('Ctrl Pts',(-4.68291352300006,15.2,9.46741856099998));
#238287=CARTESIAN_POINT('Ctrl Pts',(-4.68291352300006,11.6,9.46741856099998));
#238288=CARTESIAN_POINT('Ctrl Pts',(-4.68413257500006,15.2,9.46896718199999));
#238289=CARTESIAN_POINT('Ctrl Pts',(-4.68413257500006,11.6,9.46896718199999));
#238290=CARTESIAN_POINT('Ctrl Pts',(-4.68535742700006,15.2,9.47052027399998));
#238291=CARTESIAN_POINT('Ctrl Pts',(-4.68535742700006,11.6,9.47052027399998));
#238292=CARTESIAN_POINT('Ctrl Pts',(-4.68658807500006,15.2,9.47207781699999));
#238293=CARTESIAN_POINT('Ctrl Pts',(-4.68658807500006,11.6,9.47207781699999));
#238294=CARTESIAN_POINT('Ctrl Pts',(-4.68782452000006,15.2,9.47363979199999));
#238295=CARTESIAN_POINT('Ctrl Pts',(-4.68782452000006,11.6,9.47363979199999));
#238296=CARTESIAN_POINT('Ctrl Pts',(-4.68906676200006,15.2,9.47520617899999));
#238297=CARTESIAN_POINT('Ctrl Pts',(-4.68906676200006,11.6,9.47520617899999));
#238298=CARTESIAN_POINT('Ctrl Pts',(-4.69031479900006,15.2,9.47677695899999));
#238299=CARTESIAN_POINT('Ctrl Pts',(-4.69031479900006,11.6,9.47677695899999));
#238300=CARTESIAN_POINT('Ctrl Pts',(-4.69156863100006,15.2,9.47835211399998));
#238301=CARTESIAN_POINT('Ctrl Pts',(-4.69156863100006,11.6,9.47835211399998));
#238302=CARTESIAN_POINT('Ctrl Pts',(-4.69282825900006,15.2,9.47993162399998));
#238303=CARTESIAN_POINT('Ctrl Pts',(-4.69282825900006,11.6,9.47993162399998));
#238304=CARTESIAN_POINT('Ctrl Pts',(-4.69409368100006,15.2,9.48151547099998));
#238305=CARTESIAN_POINT('Ctrl Pts',(-4.69409368100006,11.6,9.48151547099998));
#238306=CARTESIAN_POINT('Ctrl Pts',(-4.69536489600006,15.2,9.48310363499999));
#238307=CARTESIAN_POINT('Ctrl Pts',(-4.69536489600006,11.6,9.48310363499999));
#238308=CARTESIAN_POINT('Ctrl Pts',(-4.69664190500006,15.2,9.48469609699998));
#238309=CARTESIAN_POINT('Ctrl Pts',(-4.69664190500006,11.6,9.48469609699998));
#238310=CARTESIAN_POINT('Ctrl Pts',(-4.69792470700006,15.2,9.48629284099999));
#238311=CARTESIAN_POINT('Ctrl Pts',(-4.69792470700006,11.6,9.48629284099999));
#238312=CARTESIAN_POINT('Ctrl Pts',(-4.69921330000005,15.2,9.48789384499998));
#238313=CARTESIAN_POINT('Ctrl Pts',(-4.69921330000005,11.6,9.48789384499998));
#238314=CARTESIAN_POINT('Ctrl Pts',(-4.70050768500006,15.2,9.48949909199998));
#238315=CARTESIAN_POINT('Ctrl Pts',(-4.70050768500006,11.6,9.48949909199998));
#238316=CARTESIAN_POINT('Ctrl Pts',(-4.70180786100006,15.2,9.49110856299999));
#238317=CARTESIAN_POINT('Ctrl Pts',(-4.70180786100006,11.6,9.49110856299999));
#238318=CARTESIAN_POINT('Ctrl Pts',(-4.70311382900006,15.2,9.49272224099998));
#238319=CARTESIAN_POINT('Ctrl Pts',(-4.70311382900006,11.6,9.49272224099998));
#238320=CARTESIAN_POINT('Ctrl Pts',(-4.70442558400006,15.2,9.49434010499999));
#238321=CARTESIAN_POINT('Ctrl Pts',(-4.70442558400006,11.6,9.49434010499999));
#238322=CARTESIAN_POINT('Ctrl Pts',(-4.70574313000006,15.2,9.49596213799998));
#238323=CARTESIAN_POINT('Ctrl Pts',(-4.70574313000006,11.6,9.49596213799998));
#238324=CARTESIAN_POINT('Ctrl Pts',(-4.70706646400005,15.2,9.49758832299998));
#238325=CARTESIAN_POINT('Ctrl Pts',(-4.70706646400005,11.6,9.49758832299998));
#238326=CARTESIAN_POINT('Ctrl Pts',(-4.70839558700006,15.2,9.49921863999998));
#238327=CARTESIAN_POINT('Ctrl Pts',(-4.70839558700006,11.6,9.49921863999998));
#238328=CARTESIAN_POINT('Ctrl Pts',(-4.70973049600006,15.2,9.50085307099998));
#238329=CARTESIAN_POINT('Ctrl Pts',(-4.70973049600006,11.6,9.50085307099998));
#238330=CARTESIAN_POINT('Ctrl Pts',(-4.71107119200005,15.2,9.50249159799998));
#238331=CARTESIAN_POINT('Ctrl Pts',(-4.71107119200005,11.6,9.50249159799998));
#238332=CARTESIAN_POINT('Ctrl Pts',(-4.71241767400006,15.2,9.50413420399999));
#238333=CARTESIAN_POINT('Ctrl Pts',(-4.71241767400006,11.6,9.50413420399999));
#238334=CARTESIAN_POINT('Ctrl Pts',(-4.71376994200006,15.2,9.50578086899998));
#238335=CARTESIAN_POINT('Ctrl Pts',(-4.71376994200006,11.6,9.50578086899998));
#238336=CARTESIAN_POINT('Ctrl Pts',(-4.71512799400006,15.2,9.50743157599998));
#238337=CARTESIAN_POINT('Ctrl Pts',(-4.71512799400006,11.6,9.50743157599998));
#238338=CARTESIAN_POINT('Ctrl Pts',(-4.71649183100006,15.2,9.50908630899999));
#238339=CARTESIAN_POINT('Ctrl Pts',(-4.71649183100006,11.6,9.50908630899999));
#238340=CARTESIAN_POINT('Ctrl Pts',(-4.71786144900006,15.2,9.51074504599998));
#238341=CARTESIAN_POINT('Ctrl Pts',(-4.71786144900006,11.6,9.51074504599998));
#238342=CARTESIAN_POINT('Ctrl Pts',(-4.71923685300006,15.2,9.51240777399999));
#238343=CARTESIAN_POINT('Ctrl Pts',(-4.71923685300006,11.6,9.51240777399999));
#238344=CARTESIAN_POINT('Ctrl Pts',(-4.72061803600006,15.2,9.51407447099999));
#238345=CARTESIAN_POINT('Ctrl Pts',(-4.72061803600006,11.6,9.51407447099999));
#238346=CARTESIAN_POINT('Ctrl Pts',(-4.72200500100006,15.2,9.51574512299998));
#238347=CARTESIAN_POINT('Ctrl Pts',(-4.72200500100006,11.6,9.51574512299998));
#238348=CARTESIAN_POINT('Ctrl Pts',(-4.72339774700006,15.2,9.51741970899998));
#238349=CARTESIAN_POINT('Ctrl Pts',(-4.72339774700006,11.6,9.51741970899998));
#238350=CARTESIAN_POINT('Ctrl Pts',(-4.72479627200006,15.2,9.51909821399998));
#238351=CARTESIAN_POINT('Ctrl Pts',(-4.72479627200006,11.6,9.51909821399998));
#238352=CARTESIAN_POINT('Ctrl Pts',(-4.72620057700006,15.2,9.52078061999998));
#238353=CARTESIAN_POINT('Ctrl Pts',(-4.72620057700006,11.6,9.52078061999998));
#238354=CARTESIAN_POINT('Ctrl Pts',(-4.72761065900006,15.2,9.52246690899998));
#238355=CARTESIAN_POINT('Ctrl Pts',(-4.72761065900006,11.6,9.52246690899998));
#238356=CARTESIAN_POINT('Ctrl Pts',(-4.72902651900006,15.2,9.52415706299998));
#238357=CARTESIAN_POINT('Ctrl Pts',(-4.72902651900006,11.6,9.52415706299998));
#238358=CARTESIAN_POINT('Ctrl Pts',(-4.73044815600006,15.2,9.52585106599999));
#238359=CARTESIAN_POINT('Ctrl Pts',(-4.73044815600006,11.6,9.52585106599999));
#238360=CARTESIAN_POINT('Ctrl Pts',(-4.73187556800006,15.2,9.52754889999999));
#238361=CARTESIAN_POINT('Ctrl Pts',(-4.73187556800006,11.6,9.52754889999999));
#238362=CARTESIAN_POINT('Ctrl Pts',(-4.73330875600006,15.2,9.52925054899998));
#238363=CARTESIAN_POINT('Ctrl Pts',(-4.73330875600006,11.6,9.52925054899998));
#238364=CARTESIAN_POINT('Ctrl Pts',(-4.73474771700006,15.2,9.53095599399998));
#238365=CARTESIAN_POINT('Ctrl Pts',(-4.73474771700006,11.6,9.53095599399998));
#238366=CARTESIAN_POINT('Ctrl Pts',(-4.73619245300006,15.2,9.53266521799998));
#238367=CARTESIAN_POINT('Ctrl Pts',(-4.73619245300006,11.6,9.53266521799998));
#238368=CARTESIAN_POINT('Ctrl Pts',(-4.73764296000006,15.2,9.53437820499998));
#238369=CARTESIAN_POINT('Ctrl Pts',(-4.73764296000006,11.6,9.53437820499998));
#238370=CARTESIAN_POINT('Ctrl Pts',(-4.73909923900006,15.2,9.53609493799998));
#238371=CARTESIAN_POINT('Ctrl Pts',(-4.73909923900006,11.6,9.53609493799998));
#238372=CARTESIAN_POINT('Ctrl Pts',(-4.74056129000005,15.2,9.53781539999999));
#238373=CARTESIAN_POINT('Ctrl Pts',(-4.74056129000005,11.6,9.53781539999999));
#238374=CARTESIAN_POINT('Ctrl Pts',(-4.74202911100006,15.2,9.53953957299999));
#238375=CARTESIAN_POINT('Ctrl Pts',(-4.74202911100006,11.6,9.53953957299999));
#238376=CARTESIAN_POINT('Ctrl Pts',(-4.74350270100006,15.2,9.54126744099998));
#238377=CARTESIAN_POINT('Ctrl Pts',(-4.74350270100006,11.6,9.54126744099998));
#238378=CARTESIAN_POINT('Ctrl Pts',(-4.74498205900006,15.2,9.54299898599999));
#238379=CARTESIAN_POINT('Ctrl Pts',(-4.74498205900006,11.6,9.54299898599999));
#238380=CARTESIAN_POINT('Ctrl Pts',(-4.74646718500006,15.2,9.54473419399999));
#238381=CARTESIAN_POINT('Ctrl Pts',(-4.74646718500006,11.6,9.54473419399999));
#238382=CARTESIAN_POINT('Ctrl Pts',(-4.74795807700006,15.2,9.54647304599998));
#238383=CARTESIAN_POINT('Ctrl Pts',(-4.74795807700006,11.6,9.54647304599998));
#238384=CARTESIAN_POINT('Ctrl Pts',(-4.74945473400005,15.2,9.54821552599999));
#238385=CARTESIAN_POINT('Ctrl Pts',(-4.74945473400005,11.6,9.54821552599999));
#238386=CARTESIAN_POINT('Ctrl Pts',(-4.75095715700006,15.2,9.54996161699999));
#238387=CARTESIAN_POINT('Ctrl Pts',(-4.75095715700006,11.6,9.54996161699999));
#238388=CARTESIAN_POINT('Ctrl Pts',(-4.75246534500006,15.2,9.55171130299998));
#238389=CARTESIAN_POINT('Ctrl Pts',(-4.75246534500006,11.6,9.55171130299998));
#238390=CARTESIAN_POINT('Ctrl Pts',(-4.75397929400006,15.2,9.55346456799998));
#238391=CARTESIAN_POINT('Ctrl Pts',(-4.75397929400006,11.6,9.55346456799998));
#238392=CARTESIAN_POINT('Ctrl Pts',(-4.75549900600006,15.2,9.55522139399999));
#238393=CARTESIAN_POINT('Ctrl Pts',(-4.75549900600006,11.6,9.55522139399999));
#238394=CARTESIAN_POINT('Ctrl Pts',(-4.75702447800006,15.2,9.55698176499999));
#238395=CARTESIAN_POINT('Ctrl Pts',(-4.75702447800006,11.6,9.55698176499999));
#238396=CARTESIAN_POINT('Ctrl Pts',(-4.75855571100006,15.2,9.55874566599999));
#238397=CARTESIAN_POINT('Ctrl Pts',(-4.75855571100006,11.6,9.55874566599999));
#238398=CARTESIAN_POINT('Ctrl Pts',(-4.76009270400006,15.2,9.56051307899998));
#238399=CARTESIAN_POINT('Ctrl Pts',(-4.76009270400006,11.6,9.56051307899998));
#238400=CARTESIAN_POINT('Ctrl Pts',(-4.76163545500006,15.2,9.56228398899999));
#238401=CARTESIAN_POINT('Ctrl Pts',(-4.76163545500006,11.6,9.56228398899999));
#238402=CARTESIAN_POINT('Ctrl Pts',(-4.76318396200006,15.2,9.56405837999998));
#238403=CARTESIAN_POINT('Ctrl Pts',(-4.76318396200006,11.6,9.56405837999998));
#238404=CARTESIAN_POINT('Ctrl Pts',(-4.76473822700005,15.2,9.56583623399998));
#238405=CARTESIAN_POINT('Ctrl Pts',(-4.76473822700005,11.6,9.56583623399998));
#238406=CARTESIAN_POINT('Ctrl Pts',(-4.76629824600006,15.2,9.56761753699999));
#238407=CARTESIAN_POINT('Ctrl Pts',(-4.76629824600006,11.6,9.56761753699999));
#238408=CARTESIAN_POINT('Ctrl Pts',(-4.76786402100006,15.2,9.56940227099999));
#238409=CARTESIAN_POINT('Ctrl Pts',(-4.76786402100006,11.6,9.56940227099999));
#238410=CARTESIAN_POINT('Ctrl Pts',(-4.76943554800005,15.2,9.57119042099999));
#238411=CARTESIAN_POINT('Ctrl Pts',(-4.76943554800005,11.6,9.57119042099999));
#238412=CARTESIAN_POINT('Ctrl Pts',(-4.77101282700006,15.2,9.57298197199999));
#238413=CARTESIAN_POINT('Ctrl Pts',(-4.77101282700006,11.6,9.57298197199999));
#238414=CARTESIAN_POINT('Ctrl Pts',(-4.77259585800006,15.2,9.57477690599998));
#238415=CARTESIAN_POINT('Ctrl Pts',(-4.77259585800006,11.6,9.57477690599998));
#238416=CARTESIAN_POINT('Ctrl Pts',(-4.77418464000006,15.2,9.57657520799999));
#238417=CARTESIAN_POINT('Ctrl Pts',(-4.77418464000006,11.6,9.57657520799999));
#238418=CARTESIAN_POINT('Ctrl Pts',(-4.77577917000006,15.2,9.57837686299998));
#238419=CARTESIAN_POINT('Ctrl Pts',(-4.77577917000006,11.6,9.57837686299998));
#238420=CARTESIAN_POINT('Ctrl Pts',(-4.77737944900006,15.2,9.58018185499999));
#238421=CARTESIAN_POINT('Ctrl Pts',(-4.77737944900006,11.6,9.58018185499999));
#238422=CARTESIAN_POINT('Ctrl Pts',(-4.77898547500006,15.2,9.58199016699999));
#238423=CARTESIAN_POINT('Ctrl Pts',(-4.77898547500006,11.6,9.58199016699999));
#238424=CARTESIAN_POINT('Ctrl Pts',(-4.78059724700006,15.2,9.58380178399998));
#238425=CARTESIAN_POINT('Ctrl Pts',(-4.78059724700006,11.6,9.58380178399998));
#238426=CARTESIAN_POINT('Ctrl Pts',(-4.78221476400006,15.2,9.58561669099998));
#238427=CARTESIAN_POINT('Ctrl Pts',(-4.78221476400006,11.6,9.58561669099998));
#238428=CARTESIAN_POINT('Ctrl Pts',(-4.78383802500006,15.2,9.58743487199998));
#238429=CARTESIAN_POINT('Ctrl Pts',(-4.78383802500006,11.6,9.58743487199998));
#238430=CARTESIAN_POINT('Ctrl Pts',(-4.78546702900006,15.2,9.58925631099999));
#238431=CARTESIAN_POINT('Ctrl Pts',(-4.78546702900006,11.6,9.58925631099999));
#238432=CARTESIAN_POINT('Ctrl Pts',(-4.78710177500006,15.2,9.59108099199998));
#238433=CARTESIAN_POINT('Ctrl Pts',(-4.78710177500006,11.6,9.59108099199998));
#238434=CARTESIAN_POINT('Ctrl Pts',(-4.78874226100006,15.2,9.59290890199998));
#238435=CARTESIAN_POINT('Ctrl Pts',(-4.78874226100006,11.6,9.59290890199998));
#238436=CARTESIAN_POINT('Ctrl Pts',(-4.79038848700006,15.2,9.59474002299999));
#238437=CARTESIAN_POINT('Ctrl Pts',(-4.79038848700006,11.6,9.59474002299999));
#238438=CARTESIAN_POINT('Ctrl Pts',(-4.79204045200006,15.2,9.59657433899999));
#238439=CARTESIAN_POINT('Ctrl Pts',(-4.79204045200006,11.6,9.59657433899999));
#238440=CARTESIAN_POINT('Ctrl Pts',(-4.79369815400006,15.2,9.59841183799998));
#238441=CARTESIAN_POINT('Ctrl Pts',(-4.79369815400006,11.6,9.59841183799998));
#238442=CARTESIAN_POINT('Ctrl Pts',(-4.79536159200006,15.2,9.60025250299999));
#238443=CARTESIAN_POINT('Ctrl Pts',(-4.79536159200006,11.6,9.60025250299999));
#238444=CARTESIAN_POINT('Ctrl Pts',(-4.79703076500006,15.2,9.60209631699998));
#238445=CARTESIAN_POINT('Ctrl Pts',(-4.79703076500006,11.6,9.60209631699998));
#238446=CARTESIAN_POINT('Ctrl Pts',(-4.79870567300006,15.2,9.60394326799998));
#238447=CARTESIAN_POINT('Ctrl Pts',(-4.79870567300006,11.6,9.60394326799998));
#238448=CARTESIAN_POINT('Ctrl Pts',(-4.80038631200006,15.2,9.60579333799998));
#238449=CARTESIAN_POINT('Ctrl Pts',(-4.80038631200006,11.6,9.60579333799998));
#238450=CARTESIAN_POINT('Ctrl Pts',(-4.80207268400005,15.2,9.60764651399998));
#238451=CARTESIAN_POINT('Ctrl Pts',(-4.80207268400005,11.6,9.60764651399998));
#238452=CARTESIAN_POINT('Ctrl Pts',(-4.80376478700006,15.2,9.60950277999999));
#238453=CARTESIAN_POINT('Ctrl Pts',(-4.80376478700006,11.6,9.60950277999999));
#238454=CARTESIAN_POINT('Ctrl Pts',(-4.80546261900006,15.2,9.61136212099999));
#238455=CARTESIAN_POINT('Ctrl Pts',(-4.80546261900006,11.6,9.61136212099999));
#238456=CARTESIAN_POINT('Ctrl Pts',(-4.80716617900006,15.2,9.61322452199998));
#238457=CARTESIAN_POINT('Ctrl Pts',(-4.80716617900006,11.6,9.61322452199998));
#238458=CARTESIAN_POINT('Ctrl Pts',(-4.80887546500006,15.2,9.61508996699998));
#238459=CARTESIAN_POINT('Ctrl Pts',(-4.80887546500006,11.6,9.61508996699998));
#238460=CARTESIAN_POINT('Ctrl Pts',(-4.81059047700006,15.2,9.61695844399999));
#238461=CARTESIAN_POINT('Ctrl Pts',(-4.81059047700006,11.6,9.61695844399999));
#238462=CARTESIAN_POINT('Ctrl Pts',(-4.81231121400006,15.2,9.61882993499999));
#238463=CARTESIAN_POINT('Ctrl Pts',(-4.81231121400006,11.6,9.61882993499999));
#238464=CARTESIAN_POINT('Ctrl Pts',(-4.81403767400006,15.2,9.62070442599998));
#238465=CARTESIAN_POINT('Ctrl Pts',(-4.81403767400006,11.6,9.62070442599998));
#238466=CARTESIAN_POINT('Ctrl Pts',(-4.81576985700006,15.2,9.62258190399999));
#238467=CARTESIAN_POINT('Ctrl Pts',(-4.81576985700006,11.6,9.62258190399999));
#238468=CARTESIAN_POINT('Ctrl Pts',(-4.81750776000006,15.2,9.62446235199998));
#238469=CARTESIAN_POINT('Ctrl Pts',(-4.81750776000006,11.6,9.62446235199998));
#238470=CARTESIAN_POINT('Ctrl Pts',(-4.81925138400006,15.2,9.62634575599999));
#238471=CARTESIAN_POINT('Ctrl Pts',(-4.81925138400006,11.6,9.62634575599999));
#238472=CARTESIAN_POINT('Ctrl Pts',(-4.82100072500006,15.2,9.62823210199998));
#238473=CARTESIAN_POINT('Ctrl Pts',(-4.82100072500006,11.6,9.62823210199998));
#238474=CARTESIAN_POINT('Ctrl Pts',(-4.82275578500006,15.2,9.63012137399998));
#238475=CARTESIAN_POINT('Ctrl Pts',(-4.82275578500006,11.6,9.63012137399998));
#238476=CARTESIAN_POINT('Ctrl Pts',(-4.82451656000006,15.2,9.63201355899999));
#238477=CARTESIAN_POINT('Ctrl Pts',(-4.82451656000006,11.6,9.63201355899999));
#238478=CARTESIAN_POINT('Ctrl Pts',(-4.82628304900006,15.2,9.63390864199998));
#238479=CARTESIAN_POINT('Ctrl Pts',(-4.82628304900006,11.6,9.63390864199998));
#238480=CARTESIAN_POINT('Ctrl Pts',(-4.82805525200006,15.2,9.63580660699999));
#238481=CARTESIAN_POINT('Ctrl Pts',(-4.82805525200006,11.6,9.63580660699999));
#238482=CARTESIAN_POINT('Ctrl Pts',(-4.82983316700006,15.2,9.63770744199999));
#238483=CARTESIAN_POINT('Ctrl Pts',(-4.82983316700006,11.6,9.63770744199999));
#238484=CARTESIAN_POINT('Ctrl Pts',(-4.83161679300006,15.2,9.63961113099998));
#238485=CARTESIAN_POINT('Ctrl Pts',(-4.83161679300006,11.6,9.63961113099998));
#238486=CARTESIAN_POINT('Ctrl Pts',(-4.83340612800006,15.2,9.64151765999999));
#238487=CARTESIAN_POINT('Ctrl Pts',(-4.83340612800006,11.6,9.64151765999999));
#238488=CARTESIAN_POINT('Ctrl Pts',(-4.83520117200006,15.2,9.64342701399998));
#238489=CARTESIAN_POINT('Ctrl Pts',(-4.83520117200006,11.6,9.64342701399998));
#238490=CARTESIAN_POINT('Ctrl Pts',(-4.83700192300006,15.2,9.64533917999999));
#238491=CARTESIAN_POINT('Ctrl Pts',(-4.83700192300006,11.6,9.64533917999999));
#238492=CARTESIAN_POINT('Ctrl Pts',(-4.83880838000006,15.2,9.64725414299998));
#238493=CARTESIAN_POINT('Ctrl Pts',(-4.83880838000006,11.6,9.64725414299998));
#238494=CARTESIAN_POINT('Ctrl Pts',(-4.84062054100006,15.2,9.64917188799999));
#238495=CARTESIAN_POINT('Ctrl Pts',(-4.84062054100006,11.6,9.64917188799999));
#238496=CARTESIAN_POINT('Ctrl Pts',(-4.84243840500006,15.2,9.65109240199999));
#238497=CARTESIAN_POINT('Ctrl Pts',(-4.84243840500006,11.6,9.65109240199999));
#238498=CARTESIAN_POINT('Ctrl Pts',(-4.84426197000006,15.2,9.65301567099999));
#238499=CARTESIAN_POINT('Ctrl Pts',(-4.84426197000006,11.6,9.65301567099999));
#238500=CARTESIAN_POINT('Ctrl Pts',(-4.84609123600006,15.2,9.65494167999999));
#238501=CARTESIAN_POINT('Ctrl Pts',(-4.84609123600006,11.6,9.65494167999999));
#238502=CARTESIAN_POINT('Ctrl Pts',(-4.84792620100006,15.2,9.65687041299999));
#238503=CARTESIAN_POINT('Ctrl Pts',(-4.84792620100006,11.6,9.65687041299999));
#238504=CARTESIAN_POINT('Ctrl Pts',(-4.84976686400006,15.2,9.65880186099999));
#238505=CARTESIAN_POINT('Ctrl Pts',(-4.84976686400006,11.6,9.65880186099999));
#238506=CARTESIAN_POINT('Ctrl Pts',(-4.85161322400006,15.2,9.66073600499998));
#238507=CARTESIAN_POINT('Ctrl Pts',(-4.85161322400006,11.6,9.66073600499998));
#238508=CARTESIAN_POINT('Ctrl Pts',(-4.85346527800006,15.2,9.66267283399999));
#238509=CARTESIAN_POINT('Ctrl Pts',(-4.85346527800006,11.6,9.66267283399999));
#238510=CARTESIAN_POINT('Ctrl Pts',(-4.85532302500006,15.2,9.66461233499999));
#238511=CARTESIAN_POINT('Ctrl Pts',(-4.85532302500006,11.6,9.66461233499999));
#238512=CARTESIAN_POINT('Ctrl Pts',(-4.85718646500006,15.2,9.66655448999998));
#238513=CARTESIAN_POINT('Ctrl Pts',(-4.85718646500006,11.6,9.66655448999998));
#238514=CARTESIAN_POINT('Ctrl Pts',(-4.85905559600006,15.2,9.66849928799999));
#238515=CARTESIAN_POINT('Ctrl Pts',(-4.85905559600006,11.6,9.66849928799999));
#238516=CARTESIAN_POINT('Ctrl Pts',(-4.86093041600006,15.2,9.67044671499998));
#238517=CARTESIAN_POINT('Ctrl Pts',(-4.86093041600006,11.6,9.67044671499998));
#238518=CARTESIAN_POINT('Ctrl Pts',(-4.86281092400006,15.2,9.67239675599998));
#238519=CARTESIAN_POINT('Ctrl Pts',(-4.86281092400006,11.6,9.67239675599998));
#238520=CARTESIAN_POINT('Ctrl Pts',(-4.86469712000006,15.2,9.67434939899999));
#238521=CARTESIAN_POINT('Ctrl Pts',(-4.86469712000006,11.6,9.67434939899999));
#238522=CARTESIAN_POINT('Ctrl Pts',(-4.86658900000006,15.2,9.67630462899999));
#238523=CARTESIAN_POINT('Ctrl Pts',(-4.86658900000006,11.6,9.67630462899999));
#238524=CARTESIAN_POINT('Ctrl Pts',(-4.86848656400006,15.2,9.67826243299999));
#238525=CARTESIAN_POINT('Ctrl Pts',(-4.86848656400006,11.6,9.67826243299999));
#238526=CARTESIAN_POINT('Ctrl Pts',(-4.87038981000006,15.2,9.68022279599998));
#238527=CARTESIAN_POINT('Ctrl Pts',(-4.87038981000006,11.6,9.68022279599998));
#238528=CARTESIAN_POINT('Ctrl Pts',(-4.87229873800006,15.2,9.68218570599999));
#238529=CARTESIAN_POINT('Ctrl Pts',(-4.87229873800006,11.6,9.68218570599999));
#238530=CARTESIAN_POINT('Ctrl Pts',(-4.87421334500006,15.2,9.68415114799999));
#238531=CARTESIAN_POINT('Ctrl Pts',(-4.87421334500006,11.6,9.68415114799999));
#238532=CARTESIAN_POINT('Ctrl Pts',(-4.87613363000006,15.2,9.68611911099998));
#238533=CARTESIAN_POINT('Ctrl Pts',(-4.87613363000006,11.6,9.68611911099998));
#238534=CARTESIAN_POINT('Ctrl Pts',(-4.87805959200006,15.2,9.68808957899999));
#238535=CARTESIAN_POINT('Ctrl Pts',(-4.87805959200006,11.6,9.68808957899999));
#238536=CARTESIAN_POINT('Ctrl Pts',(-4.87999122900006,15.2,9.69006253899998));
#238537=CARTESIAN_POINT('Ctrl Pts',(-4.87999122900006,11.6,9.69006253899998));
#238538=CARTESIAN_POINT('Ctrl Pts',(-4.88192854000006,15.2,9.69203797799998));
#238539=CARTESIAN_POINT('Ctrl Pts',(-4.88192854000006,11.6,9.69203797799998));
#238540=CARTESIAN_POINT('Ctrl Pts',(-4.88387152300006,15.2,9.69401588199998));
#238541=CARTESIAN_POINT('Ctrl Pts',(-4.88387152300006,11.6,9.69401588199998));
#238542=CARTESIAN_POINT('Ctrl Pts',(-4.88582017800006,15.2,9.69599623899999));
#238543=CARTESIAN_POINT('Ctrl Pts',(-4.88582017800006,11.6,9.69599623899999));
#238544=CARTESIAN_POINT('Ctrl Pts',(-4.88777450100006,15.2,9.69797903399999));
#238545=CARTESIAN_POINT('Ctrl Pts',(-4.88777450100006,11.6,9.69797903399999));
#238546=CARTESIAN_POINT('Ctrl Pts',(-4.88973449200006,15.2,9.69996425399999));
#238547=CARTESIAN_POINT('Ctrl Pts',(-4.88973449200006,11.6,9.69996425399999));
#238548=CARTESIAN_POINT('Ctrl Pts',(-4.89170014900006,15.2,9.70195188799998));
#238549=CARTESIAN_POINT('Ctrl Pts',(-4.89170014900006,11.6,9.70195188799998));
#238550=CARTESIAN_POINT('Ctrl Pts',(-4.89367147200006,15.2,9.70394191899998));
#238551=CARTESIAN_POINT('Ctrl Pts',(-4.89367147200006,11.6,9.70394191899998));
#238552=CARTESIAN_POINT('Ctrl Pts',(-4.89564845800006,15.2,9.70593433699998));
#238553=CARTESIAN_POINT('Ctrl Pts',(-4.89564845800006,11.6,9.70593433699998));
#238554=CARTESIAN_POINT('Ctrl Pts',(-4.89763110500006,15.2,9.70792912699999));
#238555=CARTESIAN_POINT('Ctrl Pts',(-4.89763110500006,11.6,9.70792912699999));
#238556=CARTESIAN_POINT('Ctrl Pts',(-4.89961941300006,15.2,9.70992627699999));
#238557=CARTESIAN_POINT('Ctrl Pts',(-4.89961941300006,11.6,9.70992627699999));
#238558=CARTESIAN_POINT('Ctrl Pts',(-4.90161338000005,15.2,9.71192577199999));
#238559=CARTESIAN_POINT('Ctrl Pts',(-4.90161338000005,11.6,9.71192577199999));
#238560=CARTESIAN_POINT('Ctrl Pts',(-4.90361300500005,15.2,9.71392760099998));
#238561=CARTESIAN_POINT('Ctrl Pts',(-4.90361300500005,11.6,9.71392760099998));
#238562=CARTESIAN_POINT('Ctrl Pts',(-4.90561828400006,15.2,9.71593175099999));
#238563=CARTESIAN_POINT('Ctrl Pts',(-4.90561828400006,11.6,9.71593175099999));
#238564=CARTESIAN_POINT('Ctrl Pts',(-4.90762921800005,15.2,9.71793820799999));
#238565=CARTESIAN_POINT('Ctrl Pts',(-4.90762921800005,11.6,9.71793820799999));
#238566=CARTESIAN_POINT('Ctrl Pts',(-4.90964580500005,15.2,9.71994695899999));
#238567=CARTESIAN_POINT('Ctrl Pts',(-4.90964580500005,11.6,9.71994695899999));
#238568=CARTESIAN_POINT('Ctrl Pts',(-4.91166804300006,15.2,9.72195799099998));
#238569=CARTESIAN_POINT('Ctrl Pts',(-4.91166804300006,11.6,9.72195799099998));
#238570=CARTESIAN_POINT('Ctrl Pts',(-4.91369593100006,15.2,9.72397129099999));
#238571=CARTESIAN_POINT('Ctrl Pts',(-4.91369593100006,11.6,9.72397129099999));
#238572=CARTESIAN_POINT('Ctrl Pts',(-4.91572946500006,15.2,9.72598684699998));
#238573=CARTESIAN_POINT('Ctrl Pts',(-4.91572946500006,11.6,9.72598684699998));
#238574=CARTESIAN_POINT('Ctrl Pts',(-4.91776864800006,15.2,9.72800464599998));
#238575=CARTESIAN_POINT('Ctrl Pts',(-4.91776864800006,11.6,9.72800464599998));
#238576=CARTESIAN_POINT('Ctrl Pts',(-4.91981347500006,15.2,9.73002467499999));
#238577=CARTESIAN_POINT('Ctrl Pts',(-4.91981347500006,11.6,9.73002467499999));
#238578=CARTESIAN_POINT('Ctrl Pts',(-4.92186394500005,15.2,9.73204692099999));
#238579=CARTESIAN_POINT('Ctrl Pts',(-4.92186394500005,11.6,9.73204692099999));
#238580=CARTESIAN_POINT('Ctrl Pts',(-4.92392005600006,15.2,9.73407136999998));
#238581=CARTESIAN_POINT('Ctrl Pts',(-4.92392005600006,11.6,9.73407136999998));
#238582=CARTESIAN_POINT('Ctrl Pts',(-4.92598180900006,15.2,9.73609801199999));
#238583=CARTESIAN_POINT('Ctrl Pts',(-4.92598180900006,11.6,9.73609801199999));
#238584=CARTESIAN_POINT('Ctrl Pts',(-4.92804919800006,15.2,9.73812683299998));
#238585=CARTESIAN_POINT('Ctrl Pts',(-4.92804919800006,11.6,9.73812683299998));
#238586=CARTESIAN_POINT('Ctrl Pts',(-4.93012222500006,15.2,9.74015781999999));
#238587=CARTESIAN_POINT('Ctrl Pts',(-4.93012222500006,11.6,9.74015781999999));
#238588=CARTESIAN_POINT('Ctrl Pts',(-4.93220088800006,15.2,9.74219095999998));
#238589=CARTESIAN_POINT('Ctrl Pts',(-4.93220088800006,11.6,9.74219095999998));
#238590=CARTESIAN_POINT('Ctrl Pts',(-4.93428518500005,15.2,9.74422624199999));
#238591=CARTESIAN_POINT('Ctrl Pts',(-4.93428518500005,11.6,9.74422624199999));
#238592=CARTESIAN_POINT('Ctrl Pts',(-4.93637511200006,15.2,9.74626365299999));
#238593=CARTESIAN_POINT('Ctrl Pts',(-4.93637511200006,11.6,9.74626365299999));
#238594=CARTESIAN_POINT('Ctrl Pts',(-4.93847067100006,15.2,9.74830317899999));
#238595=CARTESIAN_POINT('Ctrl Pts',(-4.93847067100006,11.6,9.74830317899999));
#238596=CARTESIAN_POINT('Ctrl Pts',(-4.94057185900005,15.2,9.75034480899998));
#238597=CARTESIAN_POINT('Ctrl Pts',(-4.94057185900005,11.6,9.75034480899998));
#238598=CARTESIAN_POINT('Ctrl Pts',(-4.94267867400006,15.2,9.75238852899999));
#238599=CARTESIAN_POINT('Ctrl Pts',(-4.94267867400006,11.6,9.75238852899999));
#238600=CARTESIAN_POINT('Ctrl Pts',(-4.94479111300006,15.2,9.75443432799998));
#238601=CARTESIAN_POINT('Ctrl Pts',(-4.94479111300006,11.6,9.75443432799998));
#238602=CARTESIAN_POINT('Ctrl Pts',(-4.94690917700006,15.2,9.75648219399999));
#238603=CARTESIAN_POINT('Ctrl Pts',(-4.94690917700006,11.6,9.75648219399999));
#238604=CARTESIAN_POINT('Ctrl Pts',(-4.94903286400006,15.2,9.75853211399999));
#238605=CARTESIAN_POINT('Ctrl Pts',(-4.94903286400006,11.6,9.75853211399999));
#238606=CARTESIAN_POINT('Ctrl Pts',(-4.95116217100006,15.2,9.76058407399999));
#238607=CARTESIAN_POINT('Ctrl Pts',(-4.95116217100006,11.6,9.76058407399999));
#238608=CARTESIAN_POINT('Ctrl Pts',(-4.95329709600006,15.2,9.76263806399999));
#238609=CARTESIAN_POINT('Ctrl Pts',(-4.95329709600006,11.6,9.76263806399999));
#238610=CARTESIAN_POINT('Ctrl Pts',(-4.95543763800006,15.2,9.76469406999998));
#238611=CARTESIAN_POINT('Ctrl Pts',(-4.95543763800006,11.6,9.76469406999998));
#238612=CARTESIAN_POINT('Ctrl Pts',(-4.95758379700006,15.2,9.76675208199998));
#238613=CARTESIAN_POINT('Ctrl Pts',(-4.95758379700006,11.6,9.76675208199998));
#238614=CARTESIAN_POINT('Ctrl Pts',(-4.95973556900006,15.2,9.76881208499999));
#238615=CARTESIAN_POINT('Ctrl Pts',(-4.95973556900006,11.6,9.76881208499999));
#238616=CARTESIAN_POINT('Ctrl Pts',(-4.96189295400006,15.2,9.77087406899999));
#238617=CARTESIAN_POINT('Ctrl Pts',(-4.96189295400006,11.6,9.77087406899999));
#238618=CARTESIAN_POINT('Ctrl Pts',(-4.96405594800006,15.2,9.77293802099998));
#238619=CARTESIAN_POINT('Ctrl Pts',(-4.96405594800006,11.6,9.77293802099998));
#238620=CARTESIAN_POINT('Ctrl Pts',(-4.96622455200006,15.2,9.77500392799998));
#238621=CARTESIAN_POINT('Ctrl Pts',(-4.96622455200006,11.6,9.77500392799998));
#238622=CARTESIAN_POINT('Ctrl Pts',(-4.96839876200006,15.2,9.77707177899998));
#238623=CARTESIAN_POINT('Ctrl Pts',(-4.96839876200006,11.6,9.77707177899998));
#238624=CARTESIAN_POINT('Ctrl Pts',(-4.97057857800006,15.2,9.77914156199999));
#238625=CARTESIAN_POINT('Ctrl Pts',(-4.97057857800006,11.6,9.77914156199999));
#238626=CARTESIAN_POINT('Ctrl Pts',(-4.97276399800006,15.2,9.78121326499998));
#238627=CARTESIAN_POINT('Ctrl Pts',(-4.97276399800006,11.6,9.78121326499998));
#238628=CARTESIAN_POINT('Ctrl Pts',(-4.97495501900006,15.2,9.78328687399999));
#238629=CARTESIAN_POINT('Ctrl Pts',(-4.97495501900006,11.6,9.78328687399999));
#238630=CARTESIAN_POINT('Ctrl Pts',(-4.97715164100006,15.2,9.78536237999998));
#238631=CARTESIAN_POINT('Ctrl Pts',(-4.97715164100006,11.6,9.78536237999998));
#238632=CARTESIAN_POINT('Ctrl Pts',(-4.97935386100006,15.2,9.78743976799999));
#238633=CARTESIAN_POINT('Ctrl Pts',(-4.97935386100006,11.6,9.78743976799999));
#238634=CARTESIAN_POINT('Ctrl Pts',(-4.98156167800006,15.2,9.78951902899999));
#238635=CARTESIAN_POINT('Ctrl Pts',(-4.98156167800006,11.6,9.78951902899999));
#238636=CARTESIAN_POINT('Ctrl Pts',(-4.98377508900006,15.2,9.79160014799999));
#238637=CARTESIAN_POINT('Ctrl Pts',(-4.98377508900006,11.6,9.79160014799999));
#238638=CARTESIAN_POINT('Ctrl Pts',(-4.98599409400006,15.2,9.79368311599998));
#238639=CARTESIAN_POINT('Ctrl Pts',(-4.98599409400006,11.6,9.79368311599998));
#238640=CARTESIAN_POINT('Ctrl Pts',(-4.98821869000006,15.2,9.79576792099999));
#238641=CARTESIAN_POINT('Ctrl Pts',(-4.98821869000006,11.6,9.79576792099999));
#238642=CARTESIAN_POINT('Ctrl Pts',(-4.99044887700006,15.2,9.79785454799998));
#238643=CARTESIAN_POINT('Ctrl Pts',(-4.99044887700006,11.6,9.79785454799998));
#238644=CARTESIAN_POINT('Ctrl Pts',(-4.99268465100006,15.2,9.79994298899998));
#238645=CARTESIAN_POINT('Ctrl Pts',(-4.99268465100006,11.6,9.79994298899998));
#238646=CARTESIAN_POINT('Ctrl Pts',(-4.99492601100005,15.2,9.80203322899998));
#238647=CARTESIAN_POINT('Ctrl Pts',(-4.99492601100005,11.6,9.80203322899998));
#238648=CARTESIAN_POINT('Ctrl Pts',(-4.99717295600006,15.2,9.80412525899998));
#238649=CARTESIAN_POINT('Ctrl Pts',(-4.99717295600006,11.6,9.80412525899998));
#238650=CARTESIAN_POINT('Ctrl Pts',(-4.99942548400006,15.2,9.80621906499999));
#238651=CARTESIAN_POINT('Ctrl Pts',(-4.99942548400006,11.6,9.80621906499999));
#238652=CARTESIAN_POINT('Ctrl Pts',(-5.00168359100006,15.2,9.80831463699998));
#238653=CARTESIAN_POINT('Ctrl Pts',(-5.00168359100006,11.6,9.80831463699998));
#238654=CARTESIAN_POINT('Ctrl Pts',(-5.00394727800006,15.2,9.81041196199998));
#238655=CARTESIAN_POINT('Ctrl Pts',(-5.00394727800006,11.6,9.81041196199998));
#238656=CARTESIAN_POINT('Ctrl Pts',(-5.00621654300006,15.2,9.81251102999998));
#238657=CARTESIAN_POINT('Ctrl Pts',(-5.00621654300006,11.6,9.81251102999998));
#238658=CARTESIAN_POINT('Ctrl Pts',(-5.00849138300006,15.2,9.81461182699999));
#238659=CARTESIAN_POINT('Ctrl Pts',(-5.00849138300006,11.6,9.81461182699999));
#238660=CARTESIAN_POINT('Ctrl Pts',(-5.01077179700006,15.2,9.81671434299999));
#238661=CARTESIAN_POINT('Ctrl Pts',(-5.01077179700006,11.6,9.81671434299999));
#238662=CARTESIAN_POINT('Ctrl Pts',(-5.01305778100006,15.2,9.81881856699999));
#238663=CARTESIAN_POINT('Ctrl Pts',(-5.01305778100006,11.6,9.81881856699999));
#238664=CARTESIAN_POINT('Ctrl Pts',(-5.01534933700006,15.2,9.82092448699999));
#238665=CARTESIAN_POINT('Ctrl Pts',(-5.01534933700006,11.6,9.82092448699999));
#238666=CARTESIAN_POINT('Ctrl Pts',(-5.01764646100006,15.2,9.82303208999999));
#238667=CARTESIAN_POINT('Ctrl Pts',(-5.01764646100006,11.6,9.82303208999999));
#238668=CARTESIAN_POINT('Ctrl Pts',(-5.01994915100005,15.2,9.82514136699999));
#238669=CARTESIAN_POINT('Ctrl Pts',(-5.01994915100005,11.6,9.82514136699999));
#238670=CARTESIAN_POINT('Ctrl Pts',(-5.02225740500006,15.2,9.82725230399998));
#238671=CARTESIAN_POINT('Ctrl Pts',(-5.02225740500006,11.6,9.82725230399998));
#238672=CARTESIAN_POINT('Ctrl Pts',(-5.02457122300005,15.2,9.82936489099998));
#238673=CARTESIAN_POINT('Ctrl Pts',(-5.02457122300005,11.6,9.82936489099998));
#238674=CARTESIAN_POINT('Ctrl Pts',(-5.02689060100006,15.2,9.83147911699999));
#238675=CARTESIAN_POINT('Ctrl Pts',(-5.02689060100006,11.6,9.83147911699999));
#238676=CARTESIAN_POINT('Ctrl Pts',(-5.02921553800006,15.2,9.83359496999999));
#238677=CARTESIAN_POINT('Ctrl Pts',(-5.02921553800006,11.6,9.83359496999999));
#238678=CARTESIAN_POINT('Ctrl Pts',(-5.03154603200006,15.2,9.83571243799998));
#238679=CARTESIAN_POINT('Ctrl Pts',(-5.03154603200006,11.6,9.83571243799998));
#238680=CARTESIAN_POINT('Ctrl Pts',(-5.03388208200006,15.2,9.83783151099999));
#238681=CARTESIAN_POINT('Ctrl Pts',(-5.03388208200006,11.6,9.83783151099999));
#238682=CARTESIAN_POINT('Ctrl Pts',(-5.03622368600006,15.2,9.83995217699999));
#238683=CARTESIAN_POINT('Ctrl Pts',(-5.03622368600006,11.6,9.83995217699999));
#238684=CARTESIAN_POINT('Ctrl Pts',(-5.03857084100006,15.2,9.84207442399999));
#238685=CARTESIAN_POINT('Ctrl Pts',(-5.03857084100006,11.6,9.84207442399999));
#238686=CARTESIAN_POINT('Ctrl Pts',(-5.04092354500006,15.2,9.84419824299999));
#238687=CARTESIAN_POINT('Ctrl Pts',(-5.04092354500006,11.6,9.84419824299999));
#238688=CARTESIAN_POINT('Ctrl Pts',(-5.04328179800006,15.2,9.84632361999999));
#238689=CARTESIAN_POINT('Ctrl Pts',(-5.04328179800006,11.6,9.84632361999999));
#238690=CARTESIAN_POINT('Ctrl Pts',(-5.04564559600006,15.2,9.84845054499999));
#238691=CARTESIAN_POINT('Ctrl Pts',(-5.04564559600006,11.6,9.84845054499999));
#238692=CARTESIAN_POINT('Ctrl Pts',(-5.04801493800006,15.2,9.85057900699999));
#238693=CARTESIAN_POINT('Ctrl Pts',(-5.04801493800006,11.6,9.85057900699999));
#238694=CARTESIAN_POINT('Ctrl Pts',(-5.05038982300006,15.2,9.85270899499999));
#238695=CARTESIAN_POINT('Ctrl Pts',(-5.05038982300006,11.6,9.85270899499999));
#238696=CARTESIAN_POINT('Ctrl Pts',(-5.05277024800006,15.2,9.85484049699998));
#238697=CARTESIAN_POINT('Ctrl Pts',(-5.05277024800006,11.6,9.85484049699998));
#238698=CARTESIAN_POINT('Ctrl Pts',(-5.05515621200006,15.2,9.85697350299999));
#238699=CARTESIAN_POINT('Ctrl Pts',(-5.05515621200006,11.6,9.85697350299999));
#238700=CARTESIAN_POINT('Ctrl Pts',(-5.05754771100006,15.2,9.85910800099998));
#238701=CARTESIAN_POINT('Ctrl Pts',(-5.05754771100006,11.6,9.85910800099998));
#238702=CARTESIAN_POINT('Ctrl Pts',(-5.05994474700006,15.2,9.86124398099999));
#238703=CARTESIAN_POINT('Ctrl Pts',(-5.05994474700006,11.6,9.86124398099999));
#238704=CARTESIAN_POINT('Ctrl Pts',(-5.06234731400006,15.2,9.86338143099999));
#238705=CARTESIAN_POINT('Ctrl Pts',(-5.06234731400006,11.6,9.86338143099999));
#238706=CARTESIAN_POINT('Ctrl Pts',(-5.06475541200006,15.2,9.86552034099999));
#238707=CARTESIAN_POINT('Ctrl Pts',(-5.06475541200006,11.6,9.86552034099999));
#238708=CARTESIAN_POINT('Ctrl Pts',(-5.06716903900006,15.2,9.86766069799998));
#238709=CARTESIAN_POINT('Ctrl Pts',(-5.06716903900006,11.6,9.86766069799998));
#238710=CARTESIAN_POINT('Ctrl Pts',(-5.06958819300006,15.2,9.86980249299998));
#238711=CARTESIAN_POINT('Ctrl Pts',(-5.06958819300006,11.6,9.86980249299998));
#238712=CARTESIAN_POINT('Ctrl Pts',(-5.07201287200005,15.2,9.87194571499998));
#238713=CARTESIAN_POINT('Ctrl Pts',(-5.07201287200005,11.6,9.87194571499998));
#238714=CARTESIAN_POINT('Ctrl Pts',(-5.07444307400006,15.2,9.87409035099999));
#238715=CARTESIAN_POINT('Ctrl Pts',(-5.07444307400006,11.6,9.87409035099999));
#238716=CARTESIAN_POINT('Ctrl Pts',(-5.07687879800006,15.2,9.87623639299999));
#238717=CARTESIAN_POINT('Ctrl Pts',(-5.07687879800006,11.6,9.87623639299999));
#238718=CARTESIAN_POINT('Ctrl Pts',(-5.07932004000006,15.2,9.87838382899999));
#238719=CARTESIAN_POINT('Ctrl Pts',(-5.07932004000006,11.6,9.87838382899999));
#238720=CARTESIAN_POINT('Ctrl Pts',(-5.08176679900005,15.2,9.88053264699998));
#238721=CARTESIAN_POINT('Ctrl Pts',(-5.08176679900005,11.6,9.88053264699998));
#238722=CARTESIAN_POINT('Ctrl Pts',(-5.08421907400006,15.2,9.88268283699998));
#238723=CARTESIAN_POINT('Ctrl Pts',(-5.08421907400006,11.6,9.88268283699998));
#238724=CARTESIAN_POINT('Ctrl Pts',(-5.08667686200006,15.2,9.88483438899999));
#238725=CARTESIAN_POINT('Ctrl Pts',(-5.08667686200006,11.6,9.88483438899999));
#238726=CARTESIAN_POINT('Ctrl Pts',(-5.08914016200006,15.2,9.88698729199999));
#238727=CARTESIAN_POINT('Ctrl Pts',(-5.08914016200006,11.6,9.88698729199999));
#238728=CARTESIAN_POINT('Ctrl Pts',(-5.09160897100006,15.2,9.88914153399998));
#238729=CARTESIAN_POINT('Ctrl Pts',(-5.09160897100006,11.6,9.88914153399998));
#238730=CARTESIAN_POINT('Ctrl Pts',(-5.09408328700006,15.2,9.89129710499999));
#238731=CARTESIAN_POINT('Ctrl Pts',(-5.09408328700006,11.6,9.89129710499999));
#238732=CARTESIAN_POINT('Ctrl Pts',(-5.09656311000006,15.2,9.89345399499998));
#238733=CARTESIAN_POINT('Ctrl Pts',(-5.09656311000006,11.6,9.89345399499998));
#238734=CARTESIAN_POINT('Ctrl Pts',(-5.09904843500006,15.2,9.89561219199998));
#238735=CARTESIAN_POINT('Ctrl Pts',(-5.09904843500006,11.6,9.89561219199998));
#238736=CARTESIAN_POINT('Ctrl Pts',(-5.10153926200006,15.2,9.89777168599998));
#238737=CARTESIAN_POINT('Ctrl Pts',(-5.10153926200006,11.6,9.89777168599998));
#238738=CARTESIAN_POINT('Ctrl Pts',(-5.10403558800006,15.2,9.89993246799998));
#238739=CARTESIAN_POINT('Ctrl Pts',(-5.10403558800006,11.6,9.89993246799998));
#238740=CARTESIAN_POINT('Ctrl Pts',(-5.10653741200006,15.2,9.90209452499998));
#238741=CARTESIAN_POINT('Ctrl Pts',(-5.10653741200006,11.6,9.90209452499998));
#238742=CARTESIAN_POINT('Ctrl Pts',(-5.10904473100006,15.2,9.90425784699998));
#238743=CARTESIAN_POINT('Ctrl Pts',(-5.10904473100006,11.6,9.90425784699998));
#238744=CARTESIAN_POINT('Ctrl Pts',(-5.11155754400006,15.2,9.90642242299998));
#238745=CARTESIAN_POINT('Ctrl Pts',(-5.11155754400006,11.6,9.90642242299998));
#238746=CARTESIAN_POINT('Ctrl Pts',(-5.11407584900006,15.2,9.90858824399999));
#238747=CARTESIAN_POINT('Ctrl Pts',(-5.11407584900006,11.6,9.90858824399999));
#238748=CARTESIAN_POINT('Ctrl Pts',(-5.11659964300006,15.2,9.91075529899998));
#238749=CARTESIAN_POINT('Ctrl Pts',(-5.11659964300006,11.6,9.91075529899998));
#238750=CARTESIAN_POINT('Ctrl Pts',(-5.11912892400006,15.2,9.91292357699999));
#238751=CARTESIAN_POINT('Ctrl Pts',(-5.11912892400006,11.6,9.91292357699999));
#238752=CARTESIAN_POINT('Ctrl Pts',(-5.12166369100005,15.2,9.91509306699999));
#238753=CARTESIAN_POINT('Ctrl Pts',(-5.12166369100005,11.6,9.91509306699999));
#238754=CARTESIAN_POINT('Ctrl Pts',(-5.12420394100006,15.2,9.91726375999999));
#238755=CARTESIAN_POINT('Ctrl Pts',(-5.12420394100006,11.6,9.91726375999999));
#238756=CARTESIAN_POINT('Ctrl Pts',(-5.12674967300006,15.2,9.91943564499999));
#238757=CARTESIAN_POINT('Ctrl Pts',(-5.12674967300006,11.6,9.91943564499999));
#238758=CARTESIAN_POINT('Ctrl Pts',(-5.12930088400006,15.2,9.92160870999999));
#238759=CARTESIAN_POINT('Ctrl Pts',(-5.12930088400006,11.6,9.92160870999999));
#238760=CARTESIAN_POINT('Ctrl Pts',(-5.13185757200006,15.2,9.92378294799998));
#238761=CARTESIAN_POINT('Ctrl Pts',(-5.13185757200006,11.6,9.92378294799998));
#238762=CARTESIAN_POINT('Ctrl Pts',(-5.13441973600006,15.2,9.92595834399999));
#238763=CARTESIAN_POINT('Ctrl Pts',(-5.13441973600006,11.6,9.92595834399999));
#238764=CARTESIAN_POINT('Ctrl Pts',(-5.13698737300006,15.2,9.92813489299999));
#238765=CARTESIAN_POINT('Ctrl Pts',(-5.13698737300006,11.6,9.92813489299999));
#238766=CARTESIAN_POINT('Ctrl Pts',(-5.13956048100006,15.2,9.93031258099998));
#238767=CARTESIAN_POINT('Ctrl Pts',(-5.13956048100006,11.6,9.93031258099998));
#238768=CARTESIAN_POINT('Ctrl Pts',(-5.14213905800006,15.2,9.93249139799998));
#238769=CARTESIAN_POINT('Ctrl Pts',(-5.14213905800006,11.6,9.93249139799998));
#238770=CARTESIAN_POINT('Ctrl Pts',(-5.14472310200006,15.2,9.93467133499998));
#238771=CARTESIAN_POINT('Ctrl Pts',(-5.14472310200006,11.6,9.93467133499998));
#238772=CARTESIAN_POINT('Ctrl Pts',(-5.14731261100006,15.2,9.93685238099999));
#238773=CARTESIAN_POINT('Ctrl Pts',(-5.14731261100006,11.6,9.93685238099999));
#238774=CARTESIAN_POINT('Ctrl Pts',(-5.14990758400006,15.2,9.93903452699998));
#238775=CARTESIAN_POINT('Ctrl Pts',(-5.14990758400006,11.6,9.93903452699998));
#238776=CARTESIAN_POINT('Ctrl Pts',(-5.15250801600006,15.2,9.94121776099998));
#238777=CARTESIAN_POINT('Ctrl Pts',(-5.15250801600006,11.6,9.94121776099998));
#238778=CARTESIAN_POINT('Ctrl Pts',(-5.15511390900006,15.2,9.94340207299999));
#238779=CARTESIAN_POINT('Ctrl Pts',(-5.15511390900006,11.6,9.94340207299999));
#238780=CARTESIAN_POINT('Ctrl Pts',(-5.15772525600006,15.2,9.94558745399999));
#238781=CARTESIAN_POINT('Ctrl Pts',(-5.15772525600006,11.6,9.94558745399999));
#238782=CARTESIAN_POINT('Ctrl Pts',(-5.16034206000006,15.2,9.94777389299998));
#238783=CARTESIAN_POINT('Ctrl Pts',(-5.16034206000006,11.6,9.94777389299998));
#238784=CARTESIAN_POINT('Ctrl Pts',(-5.16296431600006,15.2,9.94996137999999));
#238785=CARTESIAN_POINT('Ctrl Pts',(-5.16296431600006,11.6,9.94996137999999));
#238786=CARTESIAN_POINT('Ctrl Pts',(-5.16559202200006,15.2,9.95214990599998));
#238787=CARTESIAN_POINT('Ctrl Pts',(-5.16559202200006,11.6,9.95214990599998));
#238788=CARTESIAN_POINT('Ctrl Pts',(-5.16822517700006,15.2,9.95433945799999));
#238789=CARTESIAN_POINT('Ctrl Pts',(-5.16822517700006,11.6,9.95433945799999));
#238790=CARTESIAN_POINT('Ctrl Pts',(-5.17086377800006,15.2,9.95653002999998));
#238791=CARTESIAN_POINT('Ctrl Pts',(-5.17086377800006,11.6,9.95653002999998));
#238792=CARTESIAN_POINT('Ctrl Pts',(-5.17350782200006,15.2,9.95872160899999));
#238793=CARTESIAN_POINT('Ctrl Pts',(-5.17350782200006,11.6,9.95872160899999));
#238794=CARTESIAN_POINT('Ctrl Pts',(-5.17615730900006,15.2,9.96091418599999));
#238795=CARTESIAN_POINT('Ctrl Pts',(-5.17615730900006,11.6,9.96091418599999));
#238796=CARTESIAN_POINT('Ctrl Pts',(-5.17881223600006,15.2,9.96310774999999));
#238797=CARTESIAN_POINT('Ctrl Pts',(-5.17881223600006,11.6,9.96310774999999));
#238798=CARTESIAN_POINT('Ctrl Pts',(-5.18147260100006,15.2,9.96530229299999));
#238799=CARTESIAN_POINT('Ctrl Pts',(-5.18147260100006,11.6,9.96530229299999));
#238800=CARTESIAN_POINT('Ctrl Pts',(-5.18413840200005,15.2,9.96749780299999));
#238801=CARTESIAN_POINT('Ctrl Pts',(-5.18413840200005,11.6,9.96749780299999));
#238802=CARTESIAN_POINT('Ctrl Pts',(-5.18680963500006,15.2,9.96969427199998));
#238803=CARTESIAN_POINT('Ctrl Pts',(-5.18680963500006,11.6,9.96969427199998));
#238804=CARTESIAN_POINT('Ctrl Pts',(-5.18948630100006,15.2,9.97189168799999));
#238805=CARTESIAN_POINT('Ctrl Pts',(-5.18948630100006,11.6,9.97189168799999));
#238806=CARTESIAN_POINT('Ctrl Pts',(-5.19216839500006,15.2,9.97409004199999));
#238807=CARTESIAN_POINT('Ctrl Pts',(-5.19216839500006,11.6,9.97409004199999));
#238808=CARTESIAN_POINT('Ctrl Pts',(-5.19485591800006,15.2,9.97628932499998));
#238809=CARTESIAN_POINT('Ctrl Pts',(-5.19485591800006,11.6,9.97628932499998));
#238810=CARTESIAN_POINT('Ctrl Pts',(-5.19754886400006,15.2,9.97848952599998));
#238811=CARTESIAN_POINT('Ctrl Pts',(-5.19754886400006,11.6,9.97848952599998));
#238812=CARTESIAN_POINT('Ctrl Pts',(-5.20024723500006,15.2,9.98069063599999));
#238813=CARTESIAN_POINT('Ctrl Pts',(-5.20024723500006,11.6,9.98069063599999));
#238814=CARTESIAN_POINT('Ctrl Pts',(-5.20295102500006,15.2,9.98289264499999));
#238815=CARTESIAN_POINT('Ctrl Pts',(-5.20295102500006,11.6,9.98289264499999));
#238816=CARTESIAN_POINT('Ctrl Pts',(-5.20566023400006,15.2,9.98509554099999));
#238817=CARTESIAN_POINT('Ctrl Pts',(-5.20566023400006,11.6,9.98509554099999));
#238818=CARTESIAN_POINT('Ctrl Pts',(-5.20837486000006,15.2,9.98729931899998));
#238819=CARTESIAN_POINT('Ctrl Pts',(-5.20837486000006,11.6,9.98729931899998));
#238820=CARTESIAN_POINT('Ctrl Pts',(-5.21109490000006,15.2,9.98950396499998));
#238821=CARTESIAN_POINT('Ctrl Pts',(-5.21109490000006,11.6,9.98950396499998));
#238822=CARTESIAN_POINT('Ctrl Pts',(-5.21382035100006,15.2,9.99170947099999));
#238823=CARTESIAN_POINT('Ctrl Pts',(-5.21382035100006,11.6,9.99170947099999));
#238824=CARTESIAN_POINT('Ctrl Pts',(-5.21655121300006,15.2,9.99391582499998));
#238825=CARTESIAN_POINT('Ctrl Pts',(-5.21655121300006,11.6,9.99391582499998));
#238826=CARTESIAN_POINT('Ctrl Pts',(-5.21928748300006,15.2,9.99612302199999));
#238827=CARTESIAN_POINT('Ctrl Pts',(-5.21928748300006,11.6,9.99612302199999));
#238828=CARTESIAN_POINT('Ctrl Pts',(-5.22202915800006,15.2,9.99833104799999));
#238829=CARTESIAN_POINT('Ctrl Pts',(-5.22202915800006,11.6,9.99833104799999));
#238830=CARTESIAN_POINT('Ctrl Pts',(-5.22477623600006,15.2,10.000539896));
#238831=CARTESIAN_POINT('Ctrl Pts',(-5.22477623600006,11.6,10.000539896));
#238832=CARTESIAN_POINT('Ctrl Pts',(-5.22752871700006,15.2,10.002749555));
#238833=CARTESIAN_POINT('Ctrl Pts',(-5.22752871700006,11.6,10.002749555));
#238834=CARTESIAN_POINT('Ctrl Pts',(-5.23028659500006,15.2,10.004960015));
#238835=CARTESIAN_POINT('Ctrl Pts',(-5.23028659500006,11.6,10.004960015));
#238836=CARTESIAN_POINT('Ctrl Pts',(-5.23304987100006,15.2,10.007171268));
#238837=CARTESIAN_POINT('Ctrl Pts',(-5.23304987100006,11.6,10.007171268));
#238838=CARTESIAN_POINT('Ctrl Pts',(-5.23581854200006,15.2,10.009383303));
#238839=CARTESIAN_POINT('Ctrl Pts',(-5.23581854200006,11.6,10.009383303));
#238840=CARTESIAN_POINT('Ctrl Pts',(-5.23859260500006,15.2,10.011596111));
#238841=CARTESIAN_POINT('Ctrl Pts',(-5.23859260500006,11.6,10.011596111));
#238842=CARTESIAN_POINT('Ctrl Pts',(-5.24137205800006,15.2,10.013809682));
#238843=CARTESIAN_POINT('Ctrl Pts',(-5.24137205800006,11.6,10.013809682));
#238844=CARTESIAN_POINT('Ctrl Pts',(-5.24415689800006,15.2,10.016024007));
#238845=CARTESIAN_POINT('Ctrl Pts',(-5.24415689800006,11.6,10.016024007));
#238846=CARTESIAN_POINT('Ctrl Pts',(-5.24694712600006,15.2,10.018239077));
#238847=CARTESIAN_POINT('Ctrl Pts',(-5.24694712600006,11.6,10.018239077));
#238848=CARTESIAN_POINT('Ctrl Pts',(-5.24974273600006,15.2,10.020454882));
#238849=CARTESIAN_POINT('Ctrl Pts',(-5.24974273600006,11.6,10.020454882));
#238850=CARTESIAN_POINT('Ctrl Pts',(-5.25254372800006,15.2,10.022671411));
#238851=CARTESIAN_POINT('Ctrl Pts',(-5.25254372800006,11.6,10.022671411));
#238852=CARTESIAN_POINT('Ctrl Pts',(-5.25535010000006,15.2,10.024888657));
#238853=CARTESIAN_POINT('Ctrl Pts',(-5.25535010000006,11.6,10.024888657));
#238854=CARTESIAN_POINT('Ctrl Pts',(-5.25816184700005,15.2,10.02710661));
#238855=CARTESIAN_POINT('Ctrl Pts',(-5.25816184700005,11.6,10.02710661));
#238856=CARTESIAN_POINT('Ctrl Pts',(-5.26097897100006,15.2,10.02932526));
#238857=CARTESIAN_POINT('Ctrl Pts',(-5.26097897100006,11.6,10.02932526));
#238858=CARTESIAN_POINT('Ctrl Pts',(-5.26380146600006,15.2,10.031544597));
#238859=CARTESIAN_POINT('Ctrl Pts',(-5.26380146600006,11.6,10.031544597));
#238860=CARTESIAN_POINT('Ctrl Pts',(-5.26662933100006,15.2,10.033764612));
#238861=CARTESIAN_POINT('Ctrl Pts',(-5.26662933100006,11.6,10.033764612));
#238862=CARTESIAN_POINT('Ctrl Pts',(-5.26946256500006,15.2,10.035985297));
#238863=CARTESIAN_POINT('Ctrl Pts',(-5.26946256500006,11.6,10.035985297));
#238864=CARTESIAN_POINT('Ctrl Pts',(-5.27230116500006,15.2,10.038206641));
#238865=CARTESIAN_POINT('Ctrl Pts',(-5.27230116500006,11.6,10.038206641));
#238866=CARTESIAN_POINT('Ctrl Pts',(-5.27514512800006,15.2,10.040428636));
#238867=CARTESIAN_POINT('Ctrl Pts',(-5.27514512800006,11.6,10.040428636));
#238868=CARTESIAN_POINT('Ctrl Pts',(-5.27799445100006,15.2,10.042651272));
#238869=CARTESIAN_POINT('Ctrl Pts',(-5.27799445100006,11.6,10.042651272));
#238870=CARTESIAN_POINT('Ctrl Pts',(-5.28084913500006,15.2,10.044874539));
#238871=CARTESIAN_POINT('Ctrl Pts',(-5.28084913500006,11.6,10.044874539));
#238872=CARTESIAN_POINT('Ctrl Pts',(-5.28370917500006,15.2,10.047098429));
#238873=CARTESIAN_POINT('Ctrl Pts',(-5.28370917500006,11.6,10.047098429));
#238874=CARTESIAN_POINT('Ctrl Pts',(-5.28657456900006,15.2,10.049322933));
#238875=CARTESIAN_POINT('Ctrl Pts',(-5.28657456900006,11.6,10.049322933));
#238876=CARTESIAN_POINT('Ctrl Pts',(-5.28944531600006,15.2,10.05154804));
#238877=CARTESIAN_POINT('Ctrl Pts',(-5.28944531600006,11.6,10.05154804));
#238878=CARTESIAN_POINT('Ctrl Pts',(-5.29232141300006,15.2,10.053773742));
#238879=CARTESIAN_POINT('Ctrl Pts',(-5.29232141300006,11.6,10.053773742));
#238880=CARTESIAN_POINT('Ctrl Pts',(-5.29520285700006,15.2,10.056000029));
#238881=CARTESIAN_POINT('Ctrl Pts',(-5.29520285700006,11.6,10.056000029));
#238882=CARTESIAN_POINT('Ctrl Pts',(-5.29808964700006,15.2,10.058226893));
#238883=CARTESIAN_POINT('Ctrl Pts',(-5.29808964700006,11.6,10.058226893));
#238884=CARTESIAN_POINT('Ctrl Pts',(-5.30098178000006,15.2,10.060454325));
#238885=CARTESIAN_POINT('Ctrl Pts',(-5.30098178000006,11.6,10.060454325));
#238886=CARTESIAN_POINT('Ctrl Pts',(-5.30387925400006,15.2,10.062682315));
#238887=CARTESIAN_POINT('Ctrl Pts',(-5.30387925400006,11.6,10.062682315));
#238888=CARTESIAN_POINT('Ctrl Pts',(-5.30678206600006,15.2,10.064910854));
#238889=CARTESIAN_POINT('Ctrl Pts',(-5.30678206600006,11.6,10.064910854));
#238890=CARTESIAN_POINT('Ctrl Pts',(-5.30969021500006,15.2,10.067139933));
#238891=CARTESIAN_POINT('Ctrl Pts',(-5.30969021500006,11.6,10.067139933));
#238892=CARTESIAN_POINT('Ctrl Pts',(-5.31260369800005,15.2,10.069369543));
#238893=CARTESIAN_POINT('Ctrl Pts',(-5.31260369800005,11.6,10.069369543));
#238894=CARTESIAN_POINT('Ctrl Pts',(-5.31552251300006,15.2,10.071599674));
#238895=CARTESIAN_POINT('Ctrl Pts',(-5.31552251300006,11.6,10.071599674));
#238896=CARTESIAN_POINT('Ctrl Pts',(-5.31844665700006,15.2,10.073830318));
#238897=CARTESIAN_POINT('Ctrl Pts',(-5.31844665700006,11.6,10.073830318));
#238898=CARTESIAN_POINT('Ctrl Pts',(-5.32137612800006,15.2,10.076061465));
#238899=CARTESIAN_POINT('Ctrl Pts',(-5.32137612800006,11.6,10.076061465));
#238900=CARTESIAN_POINT('Ctrl Pts',(-5.32431092300006,15.2,10.078293108));
#238901=CARTESIAN_POINT('Ctrl Pts',(-5.32431092300006,11.6,10.078293108));
#238902=CARTESIAN_POINT('Ctrl Pts',(-5.32725104100006,15.2,10.080525236));
#238903=CARTESIAN_POINT('Ctrl Pts',(-5.32725104100006,11.6,10.080525236));
#238904=CARTESIAN_POINT('Ctrl Pts',(-5.33019647900006,15.2,10.08275784));
#238905=CARTESIAN_POINT('Ctrl Pts',(-5.33019647900006,11.6,10.08275784));
#238906=CARTESIAN_POINT('Ctrl Pts',(-5.33314723600006,15.2,10.084990912));
#238907=CARTESIAN_POINT('Ctrl Pts',(-5.33314723600006,11.6,10.084990912));
#238908=CARTESIAN_POINT('Ctrl Pts',(-5.33610330800006,15.2,10.087224443));
#238909=CARTESIAN_POINT('Ctrl Pts',(-5.33610330800006,11.6,10.087224443));
#238910=CARTESIAN_POINT('Ctrl Pts',(-5.33906469200006,15.2,10.089458424));
#238911=CARTESIAN_POINT('Ctrl Pts',(-5.33906469200006,11.6,10.089458424));
#238912=CARTESIAN_POINT('Ctrl Pts',(-5.34203138800006,15.2,10.091692848));
#238913=CARTESIAN_POINT('Ctrl Pts',(-5.34203138800006,11.6,10.091692848));
#238914=CARTESIAN_POINT('Ctrl Pts',(-5.34500339300005,15.2,10.093927703));
#238915=CARTESIAN_POINT('Ctrl Pts',(-5.34500339300005,11.6,10.093927703));
#238916=CARTESIAN_POINT('Ctrl Pts',(-5.34798070300006,15.2,10.096162981));
#238917=CARTESIAN_POINT('Ctrl Pts',(-5.34798070300006,11.6,10.096162981));
#238918=CARTESIAN_POINT('Ctrl Pts',(-5.35096331800006,15.2,10.098398674));
#238919=CARTESIAN_POINT('Ctrl Pts',(-5.35096331800006,11.6,10.098398674));
#238920=CARTESIAN_POINT('Ctrl Pts',(-5.35395123500006,15.2,10.100634772));
#238921=CARTESIAN_POINT('Ctrl Pts',(-5.35395123500006,11.6,10.100634772));
#238922=CARTESIAN_POINT('Ctrl Pts',(-5.35694445000006,15.2,10.102871266));
#238923=CARTESIAN_POINT('Ctrl Pts',(-5.35694445000006,11.6,10.102871266));
#238924=CARTESIAN_POINT('Ctrl Pts',(-5.35994296100006,15.2,10.105108146));
#238925=CARTESIAN_POINT('Ctrl Pts',(-5.35994296100006,11.6,10.105108146));
#238926=CARTESIAN_POINT('Ctrl Pts',(-5.36294676700006,15.2,10.107345405));
#238927=CARTESIAN_POINT('Ctrl Pts',(-5.36294676700006,11.6,10.107345405));
#238928=CARTESIAN_POINT('Ctrl Pts',(-5.36595586500006,15.2,10.109583033));
#238929=CARTESIAN_POINT('Ctrl Pts',(-5.36595586500006,11.6,10.109583033));
#238930=CARTESIAN_POINT('Ctrl Pts',(-5.36897025300005,15.2,10.111821023));
#238931=CARTESIAN_POINT('Ctrl Pts',(-5.36897025300005,11.6,10.111821023));
#238932=CARTESIAN_POINT('Ctrl Pts',(-5.37198992800006,15.2,10.114059368));
#238933=CARTESIAN_POINT('Ctrl Pts',(-5.37198992800006,11.6,10.114059368));
#238934=CARTESIAN_POINT('Ctrl Pts',(-5.37501489000006,15.2,10.116298058));
#238935=CARTESIAN_POINT('Ctrl Pts',(-5.37501489000006,11.6,10.116298058));
#238936=CARTESIAN_POINT('Ctrl Pts',(-5.37804513400006,15.2,10.118537086));
#238937=CARTESIAN_POINT('Ctrl Pts',(-5.37804513400006,11.6,10.118537086));
#238938=CARTESIAN_POINT('Ctrl Pts',(-5.38108066000006,15.2,10.120776443));
#238939=CARTESIAN_POINT('Ctrl Pts',(-5.38108066000006,11.6,10.120776443));
#238940=CARTESIAN_POINT('Ctrl Pts',(-5.38412146300006,15.2,10.123016119));
#238941=CARTESIAN_POINT('Ctrl Pts',(-5.38412146300006,11.6,10.123016119));
#238942=CARTESIAN_POINT('Ctrl Pts',(-5.38716754200006,15.2,10.125256103));
#238943=CARTESIAN_POINT('Ctrl Pts',(-5.38716754200006,11.6,10.125256103));
#238944=CARTESIAN_POINT('Ctrl Pts',(-5.39021889300006,15.2,10.127496384));
#238945=CARTESIAN_POINT('Ctrl Pts',(-5.39021889300006,11.6,10.127496384));
#238946=CARTESIAN_POINT('Ctrl Pts',(-5.39327551300006,15.2,10.129736951));
#238947=CARTESIAN_POINT('Ctrl Pts',(-5.39327551300006,11.6,10.129736951));
#238948=CARTESIAN_POINT('Ctrl Pts',(-5.39633740000006,15.2,10.131977797));
#238949=CARTESIAN_POINT('Ctrl Pts',(-5.39633740000006,11.6,10.131977797));
#238950=CARTESIAN_POINT('Ctrl Pts',(-5.39940455200006,15.2,10.134218911));
#238951=CARTESIAN_POINT('Ctrl Pts',(-5.39940455200006,11.6,10.134218911));
#238952=CARTESIAN_POINT('Ctrl Pts',(-5.40247696800006,15.2,10.136460288));
#238953=CARTESIAN_POINT('Ctrl Pts',(-5.40247696800006,11.6,10.136460288));
#238954=CARTESIAN_POINT('Ctrl Pts',(-5.40555464400006,15.2,10.138701926));
#238955=CARTESIAN_POINT('Ctrl Pts',(-5.40555464400006,11.6,10.138701926));
#238956=CARTESIAN_POINT('Ctrl Pts',(-5.40863758200006,15.2,10.140943822));
#238957=CARTESIAN_POINT('Ctrl Pts',(-5.40863758200006,11.6,10.140943822));
#238958=CARTESIAN_POINT('Ctrl Pts',(-5.41110814000006,15.2,10.142737544));
#238959=CARTESIAN_POINT('Ctrl Pts',(-5.41110814000006,11.6,10.142737544));
#238960=CARTESIAN_POINT('Ctrl Pts',(-5.41296342700006,15.2,10.144082951));
#238961=CARTESIAN_POINT('Ctrl Pts',(-5.41296342700006,11.6,10.144082951));
#238962=CARTESIAN_POINT('Ctrl Pts',(-5.41420133600006,15.2,10.14497994));
#238963=CARTESIAN_POINT('Ctrl Pts',(-5.41420133600006,11.6,10.14497994));
#238964=CARTESIAN_POINT('Ctrl Pts',(-5.41482055400006,15.2,10.145428447));
#238965=CARTESIAN_POINT('Ctrl Pts',(-5.41482055400006,11.6,10.145428447));
#238966=CARTESIAN_POINT('Ctrl Pts',(-4.57383771200006,15.2,9.31239140099999));
#238967=CARTESIAN_POINT('Ctrl Pts',(-4.57476026596749,15.2,9.31392144227075));
#238968=CARTESIAN_POINT('Ctrl Pts',(-4.57571693063136,15.2,9.31549767344762));
#238969=CARTESIAN_POINT('Ctrl Pts',(-4.57670776761648,15.2,9.31711891458901));
#238970=CARTESIAN_POINT('Ctrl Pts',(-4.57770338291839,15.2,9.3187479741747));
#238971=CARTESIAN_POINT('Ctrl Pts',(-4.57873349932321,15.2,9.32042248440087));
#238972=CARTESIAN_POINT('Ctrl Pts',(-4.57979816360307,15.2,9.32214130041629));
#238973=CARTESIAN_POINT('Ctrl Pts',(-4.58086282778624,15.2,9.32386011627559));
#238974=CARTESIAN_POINT('Ctrl Pts',(-4.58196204052454,15.2,9.3256232394989));
#238975=CARTESIAN_POINT('Ctrl Pts',(-4.58309584848333,15.2,9.32742955643324));
#238976=CARTESIAN_POINT('Ctrl Pts',(-4.58422965644212,15.2,9.32923587336759));
#238977=CARTESIAN_POINT('Ctrl Pts',(-4.58539805581099,15.2,9.33108538570202));
#238978=CARTESIAN_POINT('Ctrl Pts',(-4.5866010919087,15.2,9.33297701280869));
#238979=CARTESIAN_POINT('Ctrl Pts',(-4.58780412811569,15.2,9.33486864008717));
#238980=CARTESIAN_POINT('Ctrl Pts',(-4.58904179835032,15.2,9.3368023811214));
#238981=CARTESIAN_POINT('Ctrl Pts',(-4.59031413942202,15.2,9.33877718823185));
#238982=CARTESIAN_POINT('Ctrl Pts',(-4.59158648037816,15.2,9.3407519951629));
#238983=CARTESIAN_POINT('Ctrl Pts',(-4.59289349278484,15.2,9.34276786523277));
#238984=CARTESIAN_POINT('Ctrl Pts',(-4.59423520699227,15.2,9.34482377850085));
#238985=CARTESIAN_POINT('Ctrl Pts',(-4.59557692119971,15.2,9.34687969176892));
#238986=CARTESIAN_POINT('Ctrl Pts',(-4.59695334020937,15.2,9.34897564855469));
#238987=CARTESIAN_POINT('Ctrl Pts',(-4.59836449115657,15.2,9.35111065189206));
#238988=CARTESIAN_POINT('Ctrl Pts',(-4.59977564223195,15.2,9.35324565542336));
#238989=CARTESIAN_POINT('Ctrl Pts',(-4.60122152508665,15.2,9.35541970736789));
#238990=CARTESIAN_POINT('Ctrl Pts',(-4.60270216441973,15.2,9.35763183999105));
#238991=CARTESIAN_POINT('Ctrl Pts',(-4.60418280361831,15.2,9.35984397241328));
#238992=CARTESIAN_POINT('Ctrl Pts',(-4.6056982021311,15.2,9.36209418225622));
#238993=CARTESIAN_POINT('Ctrl Pts',(-4.60724837732629,15.2,9.3643815288414));
#238994=CARTESIAN_POINT('Ctrl Pts',(-4.60879855252149,15.2,9.3666688754266));
#238995=CARTESIAN_POINT('Ctrl Pts',(-4.61038350695556,15.2,9.3689933576671));
#238996=CARTESIAN_POINT('Ctrl Pts',(-4.6120032588952,15.2,9.37135405532975));
#238997=CARTESIAN_POINT('Ctrl Pts',(-4.61362301083484,15.2,9.3737147529924));
#238998=CARTESIAN_POINT('Ctrl Pts',(-4.61527755807128,15.2,9.37611166566726));
#238999=CARTESIAN_POINT('Ctrl Pts',(-4.61696691709086,15.2,9.37854389649315));
#239000=CARTESIAN_POINT('Ctrl Pts',(-4.6186562762639,15.2,9.38097612753998));
#239001=CARTESIAN_POINT('Ctrl Pts',(-4.62038044845697,15.2,9.38344367610693));
#239002=CARTESIAN_POINT('Ctrl Pts',(-4.62213944263767,15.2,9.38594566816143));
#239003=CARTESIAN_POINT('Ctrl Pts',(-4.6238984366586,15.2,9.38844765998867));
#239004=CARTESIAN_POINT('Ctrl Pts',(-4.62569225330738,15.2,9.3909840917222));
#239005=CARTESIAN_POINT('Ctrl Pts',(-4.62752090224917,15.2,9.39355411272376));
#239006=CARTESIAN_POINT('Ctrl Pts',(-4.62934955119095,15.2,9.39612413372532));
#239007=CARTESIAN_POINT('Ctrl Pts',(-4.63121303150607,15.2,9.39872774061056));
#239008=CARTESIAN_POINT('Ctrl Pts',(-4.63311134851809,15.2,9.40136410067924));
#239009=CARTESIAN_POINT('Ctrl Pts',(-4.63500966570253,15.2,9.4040004609874));
#239010=CARTESIAN_POINT('Ctrl Pts',(-4.63694282087363,15.2,9.40666957294035));
#239011=CARTESIAN_POINT('Ctrl Pts',(-4.63891081506573,15.2,9.40937062233894));
#239012=CARTESIAN_POINT('Ctrl Pts',(-4.64087880907908,15.2,9.41207167149219));
#239013=CARTESIAN_POINT('Ctrl Pts',(-4.64288164336394,15.2,9.4148046567033));
#239014=CARTESIAN_POINT('Ctrl Pts',(-4.64491931629907,15.2,9.41756878094868));
#239015=CARTESIAN_POINT('Ctrl Pts',(-4.64695698923421,15.2,9.42033290519406));
#239016=CARTESIAN_POINT('Ctrl Pts',(-4.64902950220755,15.2,9.42312816917165));
#239017=CARTESIAN_POINT('Ctrl Pts',(-4.6511368510453,15.2,9.42595379248362));
#239018=CARTESIAN_POINT('Ctrl Pts',(-4.65359542481695,15.2,9.42925035318534));
#239019=CARTESIAN_POINT('Ctrl Pts',(-4.65610141511994,15.2,9.43258823538629));
#239020=CARTESIAN_POINT('Ctrl Pts',(-4.65865481324068,15.2,9.43596623177363));
#239021=CARTESIAN_POINT('Ctrl Pts',(-4.66084344008771,15.2,9.4388616570982));
#239022=CARTESIAN_POINT('Ctrl Pts',(-4.66306689591328,15.2,9.44178655333729));
#239023=CARTESIAN_POINT('Ctrl Pts',(-4.66532517374552,15.2,9.44474017689466));
#239024=CARTESIAN_POINT('Ctrl Pts',(-4.66758345178288,15.2,9.44769380072034));
#239025=CARTESIAN_POINT('Ctrl Pts',(-4.66987655041343,15.2,9.45067615305848));
#239026=CARTESIAN_POINT('Ctrl Pts',(-4.67220445949194,15.2,9.45368650504122));
#239027=CARTESIAN_POINT('Ctrl Pts',(-4.67453236835901,15.2,9.45669685675053));
#239028=CARTESIAN_POINT('Ctrl Pts',(-4.67689508776213,15.2,9.45973520739468));
#239029=CARTESIAN_POINT('Ctrl Pts',(-4.67929260275832,15.2,9.46280084678327));
#239030=CARTESIAN_POINT('Ctrl Pts',(-4.68169011775453,15.2,9.46586648617186));
#239031=CARTESIAN_POINT('Ctrl Pts',(-4.68412243088815,15.2,9.46895940989894));
#239032=CARTESIAN_POINT('Ctrl Pts',(-4.68658952400309,15.2,9.4720789246899));
#239033=CARTESIAN_POINT('Ctrl Pts',(-4.68864543500689,15.2,9.47467852044349));
#239034=CARTESIAN_POINT('Ctrl Pts',(-4.69072549924712,15.2,9.47729657986748));
#239035=CARTESIAN_POINT('Ctrl Pts',(-4.69282970737086,15.2,9.47993270806098));
#239036=CARTESIAN_POINT('Ctrl Pts',(-4.6949339154946,15.2,9.48256883625449));
#239037=CARTESIAN_POINT('Ctrl Pts',(-4.6970622661773,15.2,9.48522303222623));
#239038=CARTESIAN_POINT('Ctrl Pts',(-4.6992147478427,15.2,9.48789490555864));
#239039=CARTESIAN_POINT('Ctrl Pts',(-4.70136722950811,15.2,9.49056677889104));
#239040=CARTESIAN_POINT('Ctrl Pts',(-4.70354384382776,15.2,9.49325633019734));
#239041=CARTESIAN_POINT('Ctrl Pts',(-4.70574457703213,15.2,9.49596317597347));
#239042=CARTESIAN_POINT('Ctrl Pts',(-4.70882560356623,15.2,9.49975276011908));
#239043=CARTESIAN_POINT('Ctrl Pts',(-4.71195390343062,15.2,9.50357623959669));
#239044=CARTESIAN_POINT('Ctrl Pts',(-4.71512944035681,15.2,9.50743258263018));
#239045=CARTESIAN_POINT('Ctrl Pts',(-4.71739768098306,15.2,9.51018711332549));
#239046=CARTESIAN_POINT('Ctrl Pts',(-4.71969002076825,15.2,9.51295841089987));
#239047=CARTESIAN_POINT('Ctrl Pts',(-4.72200644651065,15.2,9.51574610687361));
#239048=CARTESIAN_POINT('Ctrl Pts',(-4.72432287225306,15.2,9.51853380284735));
#239049=CARTESIAN_POINT('Ctrl Pts',(-4.72666338292401,15.2,9.52133789712864));
#239050=CARTESIAN_POINT('Ctrl Pts',(-4.72902796355096,15.2,9.52415802560216));
#239051=CARTESIAN_POINT('Ctrl Pts',(-4.73186546020021,15.2,9.52754217964744));
#239052=CARTESIAN_POINT('Ctrl Pts',(-4.73473761700197,15.2,9.53094942444381));
#239053=CARTESIAN_POINT('Ctrl Pts',(-4.73764440299298,15.2,9.5343791415015));
#239054=CARTESIAN_POINT('Ctrl Pts',(-4.74006672474018,15.2,9.53723723915343));
#239055=CARTESIAN_POINT('Ctrl Pts',(-4.74251309794936,15.2,9.54011094335487));
#239056=CARTESIAN_POINT('Ctrl Pts',(-4.74498350114504,15.2,9.54299990189731));
#239057=CARTESIAN_POINT('Ctrl Pts',(-4.74794798487213,15.2,9.54646665202229));
#239058=CARTESIAN_POINT('Ctrl Pts',(-4.75094707373819,15.2,9.54995537003719));
#239059=CARTESIAN_POINT('Ctrl Pts',(-4.75398073454314,15.2,9.5534654580754));
#239060=CARTESIAN_POINT('Ctrl Pts',(-4.75650878530578,15.2,9.55639053154686));
#239061=CARTESIAN_POINT('Ctrl Pts',(-4.75906084568695,15.2,9.5593304440794));
#239062=CARTESIAN_POINT('Ctrl Pts',(-4.76163689403192,15.2,9.56228485923167));
#239063=CARTESIAN_POINT('Ctrl Pts',(-4.76421294237689,15.2,9.56523927438394));
#239064=CARTESIAN_POINT('Ctrl Pts',(-4.76681298099999,15.2,9.56820818934995));
#239065=CARTESIAN_POINT('Ctrl Pts',(-4.76943698599999,15.2,9.57119127122495));
#239066=CARTESIAN_POINT('Ctrl Pts',(-4.77206099099999,15.2,9.57417435309995));
#239067=CARTESIAN_POINT('Ctrl Pts',(-4.77470896513332,15.2,9.57717160057217));
#239068=CARTESIAN_POINT('Ctrl Pts',(-4.77738088575833,15.2,9.58018268501661));
#239069=CARTESIAN_POINT('Ctrl Pts',(-4.78005280638332,15.2,9.58319376946106));
#239070=CARTESIAN_POINT('Ctrl Pts',(-4.78274867302241,15.2,9.58621869019334));
#239071=CARTESIAN_POINT('Ctrl Pts',(-4.78546846449315,15.2,9.58925712152662));
#239072=CARTESIAN_POINT('Ctrl Pts',(-4.7881882559639,15.2,9.5922955528599));
#239073=CARTESIAN_POINT('Ctrl Pts',(-4.79093197165212,15.2,9.59534749539425));
#239074=CARTESIAN_POINT('Ctrl Pts',(-4.79369958818114,15.2,9.59841262970049));
#239075=CARTESIAN_POINT('Ctrl Pts',(-4.79646720471015,15.2,9.60147776400672));
#239076=CARTESIAN_POINT('Ctrl Pts',(-4.79925872137746,15.2,9.60455608719596));
#239077=CARTESIAN_POINT('Ctrl Pts',(-4.80207411693426,15.2,9.60764728671052));
#239078=CARTESIAN_POINT('Ctrl Pts',(-4.80432643319557,15.2,9.61012024612001));
#239079=CARTESIAN_POINT('Ctrl Pts',(-4.80659403095663,15.2,9.61260144500197));
#239080=CARTESIAN_POINT('Ctrl Pts',(-4.80887689616048,15.2,9.61509072458878));
#239081=CARTESIAN_POINT('Ctrl Pts',(-4.81115976167537,15.2,9.61758000451475));
#239082=CARTESIAN_POINT('Ctrl Pts',(-4.81345789653998,15.2,9.62007736431501));
#239083=CARTESIAN_POINT('Ctrl Pts',(-4.8157712872226,15.2,9.62258264672984));
#239084=CARTESIAN_POINT('Ctrl Pts',(-4.81808467759003,15.2,9.62508792880332));
#239085=CARTESIAN_POINT('Ctrl Pts',(-4.82041332386271,15.2,9.6276011322502));
#239086=CARTESIAN_POINT('Ctrl Pts',(-4.82275721339178,15.2,9.63012210182111));
#239087=CARTESIAN_POINT('Ctrl Pts',(-4.8251011032402,15.2,9.63264307173551));
#239088=CARTESIAN_POINT('Ctrl Pts',(-4.82746023410303,15.2,9.63517180770189));
#239089=CARTESIAN_POINT('Ctrl Pts',(-4.82983459474329,15.2,9.63770815551836));
#239090=CARTESIAN_POINT('Ctrl Pts',(-4.83280254538185,15.2,9.64087859011614));
#239091=CARTESIAN_POINT('Ctrl Pts',(-4.83579429141281,15.2,9.64406091733611));
#239092=CARTESIAN_POINT('Ctrl Pts',(-4.83880980620569,15.2,9.64725483872557));
#239093=CARTESIAN_POINT('Ctrl Pts',(-4.84122221784278,15.2,9.64980997562827));
#239094=CARTESIAN_POINT('Ctrl Pts',(-4.84364984006019,15.2,9.65237253423784));
#239095=CARTESIAN_POINT('Ctrl Pts',(-4.84609266035894,15.2,9.65494236063813));
#239096=CARTESIAN_POINT('Ctrl Pts',(-4.84853548099051,15.2,9.65751218738855));
#239097=CARTESIAN_POINT('Ctrl Pts',(-4.85099350050283,15.2,9.66008928352968));
#239098=CARTESIAN_POINT('Ctrl Pts',(-4.85346670126002,15.2,9.66267350196005));
#239099=CARTESIAN_POINT('Ctrl Pts',(-4.85593990168022,15.2,9.66525772003833));
#239100=CARTESIAN_POINT('Ctrl Pts',(-4.85842828586079,15.2,9.66784905781328));
#239101=CARTESIAN_POINT('Ctrl Pts',(-4.86093183759901,15.2,9.67044736810013));
#239102=CARTESIAN_POINT('Ctrl Pts',(-4.86343538967833,15.2,9.67304567874101));
#239103=CARTESIAN_POINT('Ctrl Pts',(-4.86595411115633,15.2,9.67565096279927));
#239104=CARTESIAN_POINT('Ctrl Pts',(-4.86848798451667,15.2,9.67826307277497));
#239105=CARTESIAN_POINT('Ctrl Pts',(-4.871021857877,15.2,9.68087518275067));
#239106=CARTESIAN_POINT('Ctrl Pts',(-4.87357088501963,15.2,9.68349411850492));
#239107=CARTESIAN_POINT('Ctrl Pts',(-4.87613504966092,15.2,9.68611973770425));
#239108=CARTESIAN_POINT('Ctrl Pts',(-4.87934025493847,15.2,9.6894017611668));
#239109=CARTESIAN_POINT('Ctrl Pts',(-4.88256911357549,15.2,9.69269422372325));
#239110=CARTESIAN_POINT('Ctrl Pts',(-4.88582159460791,15.2,9.69599684808464));
#239111=CARTESIAN_POINT('Ctrl Pts',(-4.88907407599485,15.2,9.69929947280602));
#239112=CARTESIAN_POINT('Ctrl Pts',(-4.89235017880925,15.2,9.70261225813285));
#239113=CARTESIAN_POINT('Ctrl Pts',(-4.89564987283507,15.2,9.70593492959035));
#239114=CARTESIAN_POINT('Ctrl Pts',(-4.89828962819959,15.2,9.70859306690122));
#239115=CARTESIAN_POINT('Ctrl Pts',(-4.90094448255246,15.2,9.71125752991908));
#239116=CARTESIAN_POINT('Ctrl Pts',(-4.90361441854349,15.2,9.71392818124345));
#239117=CARTESIAN_POINT('Ctrl Pts',(-4.90628435417074,15.2,9.71659883220395));
#239118=CARTESIAN_POINT('Ctrl Pts',(-4.90896937153359,15.2,9.71927567117847));
#239119=CARTESIAN_POINT('Ctrl Pts',(-4.91166945503354,15.2,9.72195855756964));
#239120=CARTESIAN_POINT('Ctrl Pts',(-4.91436953890137,15.2,9.72464144432635));
#239121=CARTESIAN_POINT('Ctrl Pts',(-4.91708468775954,15.2,9.72733038059476));
#239122=CARTESIAN_POINT('Ctrl Pts',(-4.91981488574166,15.2,9.73002522924162));
#239123=CARTESIAN_POINT('Ctrl Pts',(-4.92254508372378,15.2,9.73272007788849));
#239124=CARTESIAN_POINT('Ctrl Pts',(-4.92529033043266,15.2,9.73542083757215));
#239125=CARTESIAN_POINT('Ctrl Pts',(-4.92805060791798,15.2,9.73812737494249));
#239126=CARTESIAN_POINT('Ctrl Pts',(-4.93150095421049,15.2,9.74151054610225));
#239127=CARTESIAN_POINT('Ctrl Pts',(-4.9349747893646,15.2,9.74490274330435));
#239128=CARTESIAN_POINT('Ctrl Pts',(-4.93847207780089,15.2,9.74830370453012));
#239129=CARTESIAN_POINT('Ctrl Pts',(-4.94126990900737,15.2,9.75102447395558));
#239130=CARTESIAN_POINT('Ctrl Pts',(-4.9440827488653,15.2,9.75375085150939));
#239131=CARTESIAN_POINT('Ctrl Pts',(-4.94691058274166,15.2,9.75648270749163));
#239132=CARTESIAN_POINT('Ctrl Pts',(-4.95044537489446,15.2,9.75989752728333));
#239133=CARTESIAN_POINT('Ctrl Pts',(-4.95400359138006,15.2,9.76332090234733));
#239134=CARTESIAN_POINT('Ctrl Pts',(-4.95758520028529,15.2,9.7667525797935));
#239135=CARTESIAN_POINT('Ctrl Pts',(-4.96045048717524,15.2,9.76949792152602));
#239136=CARTESIAN_POINT('Ctrl Pts',(-4.96333074418707,15.2,9.77224857637798));
#239137=CARTESIAN_POINT('Ctrl Pts',(-4.96622595305998,15.2,9.77500441354105));
#239138=CARTESIAN_POINT('Ctrl Pts',(-4.96912116232735,15.2,9.77776025107961));
#239139=CARTESIAN_POINT('Ctrl Pts',(-4.97203132389892,15.2,9.78052127271589));
#239140=CARTESIAN_POINT('Ctrl Pts',(-4.97495641922499,15.2,9.78328734819996));
#239141=CARTESIAN_POINT('Ctrl Pts',(-4.97788151455105,15.2,9.78605342368403));
#239142=CARTESIAN_POINT('Ctrl Pts',(-4.98082154396223,15.2,9.78882455369373));
#239143=CARTESIAN_POINT('Ctrl Pts',(-4.98377648795814,15.2,9.79160061067886));
#239144=CARTESIAN_POINT('Ctrl Pts',(-4.98673143155143,15.2,9.79437666728574));
#239145=CARTESIAN_POINT('Ctrl Pts',(-4.98970129161222,15.2,9.79715765280033));
#239146=CARTESIAN_POINT('Ctrl Pts',(-4.99268604725613,15.2,9.79994343857227));
#239147=CARTESIAN_POINT('Ctrl Pts',(-4.99567080330671,15.2,9.80272922472378));
#239148=CARTESIAN_POINT('Ctrl Pts',(-4.99867045681854,15.2,9.80551981199932));
#239149=CARTESIAN_POINT('Ctrl Pts',(-5.00168498641251,15.2,9.80831507568061));
#239150=CARTESIAN_POINT('Ctrl Pts',(-5.00469951559576,15.2,9.81111033898105));
#239151=CARTESIAN_POINT('Ctrl Pts',(-5.0077289243289,15.2,9.81391027793642));
#239152=CARTESIAN_POINT('Ctrl Pts',(-5.01077318930126,15.2,9.81671476976241));
#239153=CARTESIAN_POINT('Ctrl Pts',(-5.01457852082781,15.2,9.82022038483147));
#239154=CARTESIAN_POINT('Ctrl Pts',(-5.01840706932721,15.2,9.82373311438685));
#239155=CARTESIAN_POINT('Ctrl Pts',(-5.0222587957149,15.2,9.8272527162615));
#239156=CARTESIAN_POINT('Ctrl Pts',(-5.025340176993,15.2,9.83006839791467));
#239157=CARTESIAN_POINT('Ctrl Pts',(-5.02843639195027,15.2,9.83288847990333));
#239158=CARTESIAN_POINT('Ctrl Pts',(-5.03154742144318,15.2,9.83571283964316));
#239159=CARTESIAN_POINT('Ctrl Pts',(-5.03465845051223,15.2,9.83853719899818));
#239160=CARTESIAN_POINT('Ctrl Pts',(-5.03778429444,15.2,9.84136583653362));
#239161=CARTESIAN_POINT('Ctrl Pts',(-5.04092493196006,15.2,9.84419863230176));
#239162=CARTESIAN_POINT('Ctrl Pts',(-5.04406556990802,15.2,9.84703142845587));
#239163=CARTESIAN_POINT('Ctrl Pts',(-5.04722100165779,15.2,9.84986838148272));
#239164=CARTESIAN_POINT('Ctrl Pts',(-5.05039120827597,15.2,9.85270937374893));
#239165=CARTESIAN_POINT('Ctrl Pts',(-5.05356141446222,15.2,9.85555036562805));
#239166=CARTESIAN_POINT('Ctrl Pts',(-5.0567463944388,15.2,9.85839539608307));
#239167=CARTESIAN_POINT('Ctrl Pts',(-5.05994612933577,15.2,9.86124434810325));
#239168=CARTESIAN_POINT('Ctrl Pts',(-5.06314586466869,15.2,9.86409330051159));
#239169=CARTESIAN_POINT('Ctrl Pts',(-5.0663603525594,15.2,9.86694617314427));
#239170=CARTESIAN_POINT('Ctrl Pts',(-5.06958957451412,15.2,9.86980284996687));
#239171=CARTESIAN_POINT('Ctrl Pts',(-5.07281879602887,15.2,9.87265952640025));
#239172=CARTESIAN_POINT('Ctrl Pts',(-5.07606275176289,15.2,9.87552000617176));
#239173=CARTESIAN_POINT('Ctrl Pts',(-5.07932141871721,15.2,9.87838417404834));
#239174=CARTESIAN_POINT('Ctrl Pts',(-5.08258008611553,15.2,9.88124834231517));
#239175=CARTESIAN_POINT('Ctrl Pts',(-5.08585346667749,15.2,9.88411619782126));
#239176=CARTESIAN_POINT('Ctrl Pts',(-5.08914153926058,15.2,9.8869876267686));
#239177=CARTESIAN_POINT('Ctrl Pts',(-5.09325162976544,15.2,9.89057691275715));
#239178=CARTESIAN_POINT('Ctrl Pts',(-5.09738467648186,15.2,9.89417177972964));
#239179=CARTESIAN_POINT('Ctrl Pts',(-5.1015406370386,15.2,9.89777200820212));
#239180=CARTESIAN_POINT('Ctrl Pts',(-5.1048654052122,15.2,9.90065219074466));
#239181=CARTESIAN_POINT('Ctrl Pts',(-5.10820483833011,15.2,9.90353580377543));
#239182=CARTESIAN_POINT('Ctrl Pts',(-5.11155891644328,15.2,9.90642273376129));
#239183=CARTESIAN_POINT('Ctrl Pts',(-5.11575151442747,15.2,9.91003139653861));
#239184=CARTESIAN_POINT('Ctrl Pts',(-5.1199669927257,15.2,9.91364524398836));
#239185=CARTESIAN_POINT('Ctrl Pts',(-5.12420531099141,15.2,9.91726405757157));
#239186=CARTESIAN_POINT('Ctrl Pts',(-5.12844362925711,15.2,9.92088287115478));
#239187=CARTESIAN_POINT('Ctrl Pts',(-5.13270478658228,15.2,9.92450664837962));
#239188=CARTESIAN_POINT('Ctrl Pts',(-5.13698874046996,15.2,9.92813517754603));
#239189=CARTESIAN_POINT('Ctrl Pts',(-5.1404159037669,15.2,9.93103800103736));
#239190=CARTESIAN_POINT('Ctrl Pts',(-5.1438576560605,15.2,9.93394386255447));
#239191=CARTESIAN_POINT('Ctrl Pts',(-5.14731397724949,15.2,9.93685265621291));
#239192=CARTESIAN_POINT('Ctrl Pts',(-5.14990621790577,15.2,9.93903425125858));
#239193=CARTESIAN_POINT('Ctrl Pts',(-5.15250665283528,15.2,9.94121749463809));
#239194=CARTESIAN_POINT('Ctrl Pts',(-5.1551152725857,15.2,9.94340234023529));
#239195=CARTESIAN_POINT('Ctrl Pts',(-5.15859343209497,15.2,9.94631546756593));
#239196=CARTESIAN_POINT('Ctrl Pts',(-5.16208614350369,15.2,9.94923144470889));
#239197=CARTESIAN_POINT('Ctrl Pts',(-5.1655933836599,15.2,9.95215016208109));
#239198=CARTESIAN_POINT('Ctrl Pts',(-5.16822381437438,15.2,9.95433920060733));
#239199=CARTESIAN_POINT('Ctrl Pts',(-5.17086241754123,15.2,9.95652978147573));
#239200=CARTESIAN_POINT('Ctrl Pts',(-5.17350918330201,15.2,9.95872185896119));
#239201=CARTESIAN_POINT('Ctrl Pts',(-5.17615594858197,15.2,9.96091393604842));
#239202=CARTESIAN_POINT('Ctrl Pts',(-5.17881087761979,15.2,9.96310750943556));
#239203=CARTESIAN_POINT('Ctrl Pts',(-5.18147396027375,15.2,9.9653025350226));
#239204=CARTESIAN_POINT('Ctrl Pts',(-5.18413704292771,15.2,9.96749756060964));
#239205=CARTESIAN_POINT('Ctrl Pts',(-5.18680827830424,15.2,9.96969403832184));
#239206=CARTESIAN_POINT('Ctrl Pts',(-5.18948765805245,15.2,9.97189192250198));
#239207=CARTESIAN_POINT('Ctrl Pts',(-5.19216703780065,15.2,9.97408980668212));
#239208=CARTESIAN_POINT('Ctrl Pts',(-5.1948545619333,15.2,9.97628909860128));
#239209=CARTESIAN_POINT('Ctrl Pts',(-5.19755022018089,15.2,9.97848975323964));
#239210=CARTESIAN_POINT('Ctrl Pts',(-5.20204298409011,15.2,9.98215751110351));
#239211=CARTESIAN_POINT('Ctrl Pts',(-5.20655834381664,15.2,9.98582905468885));
#239212=CARTESIAN_POINT('Ctrl Pts',(-5.211096252775,15.2,9.98950417996664));
#239213=CARTESIAN_POINT('Ctrl Pts',(-5.21381899805108,15.2,9.99170925505321));
#239214=CARTESIAN_POINT('Ctrl Pts',(-5.21654986176848,15.2,9.99391561852303));
#239215=CARTESIAN_POINT('Ctrl Pts',(-5.21928883395992,15.2,9.9961232290677));
#239216=CARTESIAN_POINT('Ctrl Pts',(-5.22385378777816,15.2,9.99980258010917));
#239217=CARTESIAN_POINT('Ctrl Pts',(-5.22844126430996,15.2,10.0034853915535));
#239218=CARTESIAN_POINT('Ctrl Pts',(-5.23305121974749,15.2,10.0071714635146));
#239219=CARTESIAN_POINT('Ctrl Pts',(-5.23581719290951,15.2,10.009383106611));
#239220=CARTESIAN_POINT('Ctrl Pts',(-5.23859125816533,15.2,10.0115959230892));
#239221=CARTESIAN_POINT('Ctrl Pts',(-5.24137340448022,15.2,10.0138098702587));
#239222=CARTESIAN_POINT('Ctrl Pts',(-5.24415555079511,15.2,10.0160238174281));
#239223=CARTESIAN_POINT('Ctrl Pts',(-5.24694578005942,15.2,10.0182388963809));
#239224=CARTESIAN_POINT('Ctrl Pts',(-5.24974408087331,15.2,10.0204550625502));
#239225=CARTESIAN_POINT('Ctrl Pts',(-5.25254238219556,15.2,10.0226712291221));
#239226=CARTESIAN_POINT('Ctrl Pts',(-5.25534875605342,15.2,10.0248884837444));
#239227=CARTESIAN_POINT('Ctrl Pts',(-5.25816319179689,15.2,10.0271067847336));
#239228=CARTESIAN_POINT('Ctrl Pts',(-5.26285391735428,15.2,10.0308039525116));
#239229=CARTESIAN_POINT('Ctrl Pts',(-5.26756703761759,15.2,10.0345040229674));
#239230=CARTESIAN_POINT('Ctrl Pts',(-5.27230250636941,15.2,10.0382068042176));
#239231=CARTESIAN_POINT('Ctrl Pts',(-5.27514378751726,15.2,10.040428472887));
#239232=CARTESIAN_POINT('Ctrl Pts',(-5.27799311282972,15.2,10.0426511173498));
#239233=CARTESIAN_POINT('Ctrl Pts',(-5.28085047457791,15.2,10.0448746951719));
#239234=CARTESIAN_POINT('Ctrl Pts',(-5.2837078363261,15.2,10.0470982729939));
#239235=CARTESIAN_POINT('Ctrl Pts',(-5.28657323216704,15.2,10.0493227853067));
#239236=CARTESIAN_POINT('Ctrl Pts',(-5.28944665381334,15.2,10.0515481889759));
#239237=CARTESIAN_POINT('Ctrl Pts',(-5.29232007545964,15.2,10.0537735926451));
#239238=CARTESIAN_POINT('Ctrl Pts',(-5.29520152157165,15.2,10.0559998878642));
#239239=CARTESIAN_POINT('Ctrl Pts',(-5.29809098275833,15.2,10.0582270349916));
#239240=CARTESIAN_POINT('Ctrl Pts',(-5.30098044394502,15.2,10.0604541821191));
#239241=CARTESIAN_POINT('Ctrl Pts',(-5.30387791968971,15.2,10.0626821805881));
#239242=CARTESIAN_POINT('Ctrl Pts',(-5.30678339991677,15.2,10.0649109887571));
#239243=CARTESIAN_POINT('Ctrl Pts',(-5.30968888014384,15.2,10.067139796926));
#239244=CARTESIAN_POINT('Ctrl Pts',(-5.31260236536263,15.2,10.0693694150215));
#239245=CARTESIAN_POINT('Ctrl Pts',(-5.31552384469318,15.2,10.0715998018018));
#239246=CARTESIAN_POINT('Ctrl Pts',(-5.31844532402372,15.2,10.0738301885821));
#239247=CARTESIAN_POINT('Ctrl Pts',(-5.32137479686746,15.2,10.0760613441946));
#239248=CARTESIAN_POINT('Ctrl Pts',(-5.32431225309297,15.2,10.0782932287801));
#239249=CARTESIAN_POINT('Ctrl Pts',(-5.32724970985212,15.2,10.080525113771));
#239250=CARTESIAN_POINT('Ctrl Pts',(-5.33019515076354,15.2,10.0827577261622));
#239251=CARTESIAN_POINT('Ctrl Pts',(-5.33314856540219,15.2,10.0849910272368));
#239252=CARTESIAN_POINT('Ctrl Pts',(-5.33610197950431,15.2,10.0872243279058));
#239253=CARTESIAN_POINT('Ctrl Pts',(-5.33906336546433,15.2,10.0894583174414));
#239254=CARTESIAN_POINT('Ctrl Pts',(-5.34203271556546,15.2,10.0916929560269));
#239255=CARTESIAN_POINT('Ctrl Pts',(-5.34500206566659,15.2,10.0939275946124));
#239256=CARTESIAN_POINT('Ctrl Pts',(-5.34797937788091,15.2,10.0961628806231));
#239257=CARTESIAN_POINT('Ctrl Pts',(-5.35096464349439,15.2,10.0983987752604));
#239258=CARTESIAN_POINT('Ctrl Pts',(-5.35394990910786,15.2,10.1006346698976));
#239259=CARTESIAN_POINT('Ctrl Pts',(-5.35694312649271,15.2,10.1028711720024));
#239260=CARTESIAN_POINT('Ctrl Pts',(-5.35994428473061,15.2,10.1051082407229));
#239261=CARTESIAN_POINT('Ctrl Pts',(-5.36294544296851,15.2,10.1073453094435));
#239262=CARTESIAN_POINT('Ctrl Pts',(-5.36595454318158,15.2,10.1095829447707));
#239263=CARTESIAN_POINT('Ctrl Pts',(-5.36897157444628,15.2,10.111821111481));
#239264=CARTESIAN_POINT('Ctrl Pts',(-5.37198860571097,15.2,10.1140592781913));
#239265=CARTESIAN_POINT('Ctrl Pts',(-5.37501356911677,15.2,10.1162979761266));
#239266=CARTESIAN_POINT('Ctrl Pts',(-5.37804645379717,15.2,10.1185371677535));
#239267=CARTESIAN_POINT('Ctrl Pts',(-5.38107933902854,15.2,10.1207763597872));
#239268=CARTESIAN_POINT('Ctrl Pts',(-5.38412014552048,15.2,10.1230160458294));
#239269=CARTESIAN_POINT('Ctrl Pts',(-5.38716886067296,15.2,10.1252561777383));
#239270=CARTESIAN_POINT('Ctrl Pts',(-5.39123381328652,15.2,10.1282430196053));
#239271=CARTESIAN_POINT('Ctrl Pts',(-5.39531282323273,15.2,10.1312306500592));
#239272=CARTESIAN_POINT('Ctrl Pts',(-5.39940586797222,15.2,10.1342189767729));
#239273=CARTESIAN_POINT('Ctrl Pts',(-5.40452217431482,15.2,10.1379543854705));
#239274=CARTESIAN_POINT('Ctrl Pts',(-5.40966040287515,15.2,10.1416908878519));
#239275=CARTESIAN_POINT('Ctrl Pts',(-5.41482055400006,15.2,10.145428447));
#239276=CARTESIAN_POINT('Ctrl Pts',(-4.57383771200006,12.2,9.31239140099999));
#239277=CARTESIAN_POINT('Ctrl Pts',(-4.57476026596749,12.2,9.31392144227075));
#239278=CARTESIAN_POINT('Ctrl Pts',(-4.57571693063136,12.2,9.31549767344762));
#239279=CARTESIAN_POINT('Ctrl Pts',(-4.57670776761648,12.2,9.31711891458901));
#239280=CARTESIAN_POINT('Ctrl Pts',(-4.57770338291839,12.2,9.3187479741747));
#239281=CARTESIAN_POINT('Ctrl Pts',(-4.57873349932321,12.2,9.32042248440087));
#239282=CARTESIAN_POINT('Ctrl Pts',(-4.57979816360307,12.2,9.32214130041629));
#239283=CARTESIAN_POINT('Ctrl Pts',(-4.58086282778624,12.2,9.32386011627559));
#239284=CARTESIAN_POINT('Ctrl Pts',(-4.58196204052454,12.2,9.3256232394989));
#239285=CARTESIAN_POINT('Ctrl Pts',(-4.58309584848333,12.2,9.32742955643324));
#239286=CARTESIAN_POINT('Ctrl Pts',(-4.58422965644212,12.2,9.32923587336759));
#239287=CARTESIAN_POINT('Ctrl Pts',(-4.58539805581098,12.2,9.33108538570202));
#239288=CARTESIAN_POINT('Ctrl Pts',(-4.5866010919087,12.2,9.33297701280868));
#239289=CARTESIAN_POINT('Ctrl Pts',(-4.58780412811569,12.2,9.33486864008716));
#239290=CARTESIAN_POINT('Ctrl Pts',(-4.58904179835032,12.2,9.3368023811214));
#239291=CARTESIAN_POINT('Ctrl Pts',(-4.59031413942202,12.2,9.33877718823185));
#239292=CARTESIAN_POINT('Ctrl Pts',(-4.59158648037816,12.2,9.3407519951629));
#239293=CARTESIAN_POINT('Ctrl Pts',(-4.59289349278484,12.2,9.34276786523277));
#239294=CARTESIAN_POINT('Ctrl Pts',(-4.59423520699227,12.2,9.34482377850085));
#239295=CARTESIAN_POINT('Ctrl Pts',(-4.59557692119971,12.2,9.34687969176892));
#239296=CARTESIAN_POINT('Ctrl Pts',(-4.59695334020937,12.2,9.34897564855469));
#239297=CARTESIAN_POINT('Ctrl Pts',(-4.59836449115657,12.2,9.35111065189206));
#239298=CARTESIAN_POINT('Ctrl Pts',(-4.59977564223195,12.2,9.35324565542336));
#239299=CARTESIAN_POINT('Ctrl Pts',(-4.60122152508665,12.2,9.35541970736789));
#239300=CARTESIAN_POINT('Ctrl Pts',(-4.60270216441973,12.2,9.35763183999105));
#239301=CARTESIAN_POINT('Ctrl Pts',(-4.60442957677324,12.2,9.36021266108334));
#239302=CARTESIAN_POINT('Ctrl Pts',(-4.60620429860251,12.2,9.36284530880486));
#239303=CARTESIAN_POINT('Ctrl Pts',(-4.60802636339002,12.2,9.36552829264974));
#239304=CARTESIAN_POINT('Ctrl Pts',(-4.60958813339028,12.2,9.36782799335679));
#239305=CARTESIAN_POINT('Ctrl Pts',(-4.61118468385317,12.2,9.3701646730684));
#239306=CARTESIAN_POINT('Ctrl Pts',(-4.61281603494449,12.2,9.37253741878356));
#239307=CARTESIAN_POINT('Ctrl Pts',(-4.61444738588763,12.2,9.37491016428319));
#239308=CARTESIAN_POINT('Ctrl Pts',(-4.61611353471978,12.2,9.37731897119552));
#239309=CARTESIAN_POINT('Ctrl Pts',(-4.61781449782618,12.2,9.37976295185827));
#239310=CARTESIAN_POINT('Ctrl Pts',(-4.61951546093257,12.2,9.38220693252101));
#239311=CARTESIAN_POINT('Ctrl Pts',(-4.62125123994448,12.2,9.38468608118922));
#239312=CARTESIAN_POINT('Ctrl Pts',(-4.62302184112864,12.2,9.38719953009641));
#239313=CARTESIAN_POINT('Ctrl Pts',(-4.6247924423128,12.2,9.38971297900361));
#239314=CARTESIAN_POINT('Ctrl Pts',(-4.62659787004367,12.2,9.39226072433133));
#239315=CARTESIAN_POINT('Ctrl Pts',(-4.62843812905775,12.2,9.39484191823525));
#239316=CARTESIAN_POINT('Ctrl Pts',(-4.63027838823899,12.2,9.39742311237363));
#239317=CARTESIAN_POINT('Ctrl Pts',(-4.63215348059029,12.2,9.40003775161533));
#239318=CARTESIAN_POINT('Ctrl Pts',(-4.63406341061257,12.2,9.40268500692767));
#239319=CARTESIAN_POINT('Ctrl Pts',(-4.63597334046135,12.2,9.40533226199957));
#239320=CARTESIAN_POINT('Ctrl Pts',(-4.63791810764904,12.2,9.40801213166054));
#239321=CARTESIAN_POINT('Ctrl Pts',(-4.63989771540892,12.2,9.41072380464395));
#239322=CARTESIAN_POINT('Ctrl Pts',(-4.6418773231688,12.2,9.41343547762736));
#239323=CARTESIAN_POINT('Ctrl Pts',(-4.64389176980347,12.2,9.41617895134211));
#239324=CARTESIAN_POINT('Ctrl Pts',(-4.64594105572663,12.2,9.41895343448918));
#239325=CARTESIAN_POINT('Ctrl Pts',(-4.64799034183593,12.2,9.42172791788825));
#239326=CARTESIAN_POINT('Ctrl Pts',(-4.65007446833195,12.2,9.4245334084654));
#239327=CARTESIAN_POINT('Ctrl Pts',(-4.65219342861563,12.2,9.42736913112128));
#239328=CARTESIAN_POINT('Ctrl Pts',(-4.65431238870683,12.2,9.43020485351956));
#239329=CARTESIAN_POINT('Ctrl Pts',(-4.65646618639365,12.2,9.43307080644905));
#239330=CARTESIAN_POINT('Ctrl Pts',(-4.65865481324067,12.2,9.43596623177362));
#239331=CARTESIAN_POINT('Ctrl Pts',(-4.6608434400877,12.2,9.4388616570982));
#239332=CARTESIAN_POINT('Ctrl Pts',(-4.66306689591328,12.2,9.44178655333729));
#239333=CARTESIAN_POINT('Ctrl Pts',(-4.66532517374552,12.2,9.44474017689466));
#239334=CARTESIAN_POINT('Ctrl Pts',(-4.66758345178288,12.2,9.44769380072034));
#239335=CARTESIAN_POINT('Ctrl Pts',(-4.66987655041343,12.2,9.45067615305848));
#239336=CARTESIAN_POINT('Ctrl Pts',(-4.67220445949194,12.2,9.45368650504122));
#239337=CARTESIAN_POINT('Ctrl Pts',(-4.67453236835901,12.2,9.45669685675053));
#239338=CARTESIAN_POINT('Ctrl Pts',(-4.67689508776212,12.2,9.45973520739468));
#239339=CARTESIAN_POINT('Ctrl Pts',(-4.67929260275832,12.2,9.46280084678327));
#239340=CARTESIAN_POINT('Ctrl Pts',(-4.68169011775452,12.2,9.46586648617185));
#239341=CARTESIAN_POINT('Ctrl Pts',(-4.68412243088815,12.2,9.46895940989894));
#239342=CARTESIAN_POINT('Ctrl Pts',(-4.68658952400309,12.2,9.4720789246899));
#239343=CARTESIAN_POINT('Ctrl Pts',(-4.68864543500689,12.2,9.47467852044349));
#239344=CARTESIAN_POINT('Ctrl Pts',(-4.69072549924711,12.2,9.47729657986747));
#239345=CARTESIAN_POINT('Ctrl Pts',(-4.69282970737085,12.2,9.47993270806097));
#239346=CARTESIAN_POINT('Ctrl Pts',(-4.6949339154946,12.2,9.48256883625448));
#239347=CARTESIAN_POINT('Ctrl Pts',(-4.6970622661773,12.2,9.48522303222622));
#239348=CARTESIAN_POINT('Ctrl Pts',(-4.6992147478427,12.2,9.48789490555864));
#239349=CARTESIAN_POINT('Ctrl Pts',(-4.70136722950811,12.2,9.49056677889104));
#239350=CARTESIAN_POINT('Ctrl Pts',(-4.70354384382777,12.2,9.49325633019736));
#239351=CARTESIAN_POINT('Ctrl Pts',(-4.70574457703214,12.2,9.49596317597348));
#239352=CARTESIAN_POINT('Ctrl Pts',(-4.70794531023652,12.2,9.49867002174962));
#239353=CARTESIAN_POINT('Ctrl Pts',(-4.71017016228889,12.2,9.50139416217774));
#239354=CARTESIAN_POINT('Ctrl Pts',(-4.71241912048333,12.2,9.50413521877494));
#239355=CARTESIAN_POINT('Ctrl Pts',(-4.71466807867776,12.2,9.50687627537216));
#239356=CARTESIAN_POINT('Ctrl Pts',(-4.71694114226853,12.2,9.50963424797214));
#239357=CARTESIAN_POINT('Ctrl Pts',(-4.71923829783458,12.2,9.51240876631813));
#239358=CARTESIAN_POINT('Ctrl Pts',(-4.7219948844137,12.2,9.51573818821234));
#239359=CARTESIAN_POINT('Ctrl Pts',(-4.72478616143365,12.2,9.51909143503971));
#239360=CARTESIAN_POINT('Ctrl Pts',(-4.72761210332947,12.2,9.5224678750827));
#239361=CARTESIAN_POINT('Ctrl Pts',(-4.72996705499488,12.2,9.52528157522075));
#239362=CARTESIAN_POINT('Ctrl Pts',(-4.7323460798498,12.2,9.52811138336476));
#239363=CARTESIAN_POINT('Ctrl Pts',(-4.73474916054298,12.2,9.53095693857228));
#239364=CARTESIAN_POINT('Ctrl Pts',(-4.73715224123617,12.2,9.53380249377979));
#239365=CARTESIAN_POINT('Ctrl Pts',(-4.73957937754315,12.2,9.53666379824648));
#239366=CARTESIAN_POINT('Ctrl Pts',(-4.74203055324866,12.2,9.53954049673171));
#239367=CARTESIAN_POINT('Ctrl Pts',(-4.7454621992898,12.2,9.54356787467374));
#239368=CARTESIAN_POINT('Ctrl Pts',(-4.74894095910263,12.2,9.54762542499845));
#239369=CARTESIAN_POINT('Ctrl Pts',(-4.75246678546484,12.2,9.55171219792427));
#239370=CARTESIAN_POINT('Ctrl Pts',(-4.7549852328272,12.2,9.55463132139726));
#239371=CARTESIAN_POINT('Ctrl Pts',(-4.75752769061257,12.2,9.55756535308842));
#239372=CARTESIAN_POINT('Ctrl Pts',(-4.76009414379801,12.2,9.56051395358395));
#239373=CARTESIAN_POINT('Ctrl Pts',(-4.76266059698344,12.2,9.56346255407949));
#239374=CARTESIAN_POINT('Ctrl Pts',(-4.7652510413178,12.2,9.56642572413825));
#239375=CARTESIAN_POINT('Ctrl Pts',(-4.7678654593753,12.2,9.5694031253894));
#239376=CARTESIAN_POINT('Ctrl Pts',(-4.77047987743282,12.2,9.57238052664055));
#239377=CARTESIAN_POINT('Ctrl Pts',(-4.7731182668074,12.2,9.57537216075861));
#239378=CARTESIAN_POINT('Ctrl Pts',(-4.77578060757324,12.2,9.57837769763475));
#239379=CARTESIAN_POINT('Ctrl Pts',(-4.77844294833908,12.2,9.58138323451087));
#239380=CARTESIAN_POINT('Ctrl Pts',(-4.7811292404081,12.2,9.58440267245112));
#239381=CARTESIAN_POINT('Ctrl Pts',(-4.7838394611045,12.2,9.58743568689668));
#239382=CARTESIAN_POINT('Ctrl Pts',(-4.78654968150549,12.2,9.59046870101163));
#239383=CARTESIAN_POINT('Ctrl Pts',(-4.78928383057515,12.2,9.59351529082321));
#239384=CARTESIAN_POINT('Ctrl Pts',(-4.79204188589758,12.2,9.59657513430806));
#239385=CARTESIAN_POINT('Ctrl Pts',(-4.79479994152064,12.2,9.59963497812644));
#239386=CARTESIAN_POINT('Ctrl Pts',(-4.79758190235162,12.2,9.60270807775291));
#239387=CARTESIAN_POINT('Ctrl Pts',(-4.80038774484966,12.2,9.6057941140713));
#239388=CARTESIAN_POINT('Ctrl Pts',(-4.80263241897043,12.2,9.60826294326056));
#239389=CARTESIAN_POINT('Ctrl Pts',(-4.80489237982827,12.2,9.6107400537771));
#239390=CARTESIAN_POINT('Ctrl Pts',(-4.80716761051822,12.2,9.61322528303498));
#239391=CARTESIAN_POINT('Ctrl Pts',(-4.80944284089817,12.2,9.61571051195425));
#239392=CARTESIAN_POINT('Ctrl Pts',(-4.81173334270475,12.2,9.61820386151296));
#239393=CARTESIAN_POINT('Ctrl Pts',(-4.81403910434802,12.2,9.62070517230767));
#239394=CARTESIAN_POINT('Ctrl Pts',(-4.81634486630545,12.2,9.62320648344316));
#239395=CARTESIAN_POINT('Ctrl Pts',(-4.81866588735043,12.2,9.6257157563322));
#239396=CARTESIAN_POINT('Ctrl Pts',(-4.82100215469999,12.2,9.62823283352495));
#239397=CARTESIAN_POINT('Ctrl Pts',(-4.82333842204956,12.2,9.63074991071771));
#239398=CARTESIAN_POINT('Ctrl Pts',(-4.82568993509809,12.2,9.63327479296411));
#239399=CARTESIAN_POINT('Ctrl Pts',(-4.8280566803953,12.2,9.6358073248807));
#239400=CARTESIAN_POINT('Ctrl Pts',(-4.83042342537005,12.2,9.63833985645222));
#239401=CARTESIAN_POINT('Ctrl Pts',(-4.83280540244183,12.2,9.64088003873382));
#239402=CARTESIAN_POINT('Ctrl Pts',(-4.8352025987567,12.2,9.64342771698156));
#239403=CARTESIAN_POINT('Ctrl Pts',(-4.8375997953982,12.2,9.64597539557641));
#239404=CARTESIAN_POINT('Ctrl Pts',(-4.84001221130751,12.2,9.64853057063131));
#239405=CARTESIAN_POINT('Ctrl Pts',(-4.84243983066359,12.2,9.6510930911606));
#239406=CARTESIAN_POINT('Ctrl Pts',(-4.84486744968889,12.2,9.65365561134075));
#239407=CARTESIAN_POINT('Ctrl Pts',(-4.84731027312334,12.2,9.65622547540048));
#239408=CARTESIAN_POINT('Ctrl Pts',(-4.84976828803252,12.2,9.65880253485601));
#239409=CARTESIAN_POINT('Ctrl Pts',(-4.85222630327661,12.2,9.66137959466266));
#239410=CARTESIAN_POINT('Ctrl Pts',(-4.85469950740546,12.2,9.66396385021861));
#239411=CARTESIAN_POINT('Ctrl Pts',(-4.85718788811116,12.2,9.66655515110101));
#239412=CARTESIAN_POINT('Ctrl Pts',(-4.85967626847782,12.2,9.66914645163035));
#239413=CARTESIAN_POINT('Ctrl Pts',(-4.86217982392334,12.2,9.67174479865601));
#239414=CARTESIAN_POINT('Ctrl Pts',(-4.86469854082757,12.2,9.67435004555372));
#239415=CARTESIAN_POINT('Ctrl Pts',(-4.86721725807497,12.2,9.67695529280638));
#239416=CARTESIAN_POINT('Ctrl Pts',(-4.86975113472418,12.2,9.67956743921541));
#239417=CARTESIAN_POINT('Ctrl Pts',(-4.87230015797519,12.2,9.68218633924745));
#239418=CARTESIAN_POINT('Ctrl Pts',(-4.87484918087891,12.2,9.68480523892268));
#239419=CARTESIAN_POINT('Ctrl Pts',(-4.87741334870079,12.2,9.68743089394396));
#239420=CARTESIAN_POINT('Ctrl Pts',(-4.87999264711747,12.2,9.6900631583597));
#239421=CARTESIAN_POINT('Ctrl Pts',(-4.88257194588559,12.2,9.69269542313408));
#239422=CARTESIAN_POINT('Ctrl Pts',(-4.88516637549803,12.2,9.69533429833834));
#239423=CARTESIAN_POINT('Ctrl Pts',(-4.8877759181968,12.2,9.69797964048295));
#239424=CARTESIAN_POINT('Ctrl Pts',(-4.89038546054003,12.2,9.70062498226713));
#239425=CARTESIAN_POINT('Ctrl Pts',(-4.89301011783022,12.2,9.70327679264166));
#239426=CARTESIAN_POINT('Ctrl Pts',(-4.89564987283507,12.2,9.70593492959036));
#239427=CARTESIAN_POINT('Ctrl Pts',(-4.8982896281996,12.2,9.70859306690123));
#239428=CARTESIAN_POINT('Ctrl Pts',(-4.90094448255246,12.2,9.71125752991908));
#239429=CARTESIAN_POINT('Ctrl Pts',(-4.90361441854349,12.2,9.71392818124345));
#239430=CARTESIAN_POINT('Ctrl Pts',(-4.90628435417074,12.2,9.71659883220395));
#239431=CARTESIAN_POINT('Ctrl Pts',(-4.90896937153359,12.2,9.71927567117847));
#239432=CARTESIAN_POINT('Ctrl Pts',(-4.91166945503354,12.2,9.72195855756964));
#239433=CARTESIAN_POINT('Ctrl Pts',(-4.91436953890137,12.2,9.72464144432635));
#239434=CARTESIAN_POINT('Ctrl Pts',(-4.91708468775954,12.2,9.72733038059476));
#239435=CARTESIAN_POINT('Ctrl Pts',(-4.91981488574166,12.2,9.73002522924162));
#239436=CARTESIAN_POINT('Ctrl Pts',(-4.92254508372378,12.2,9.73272007788849));
#239437=CARTESIAN_POINT('Ctrl Pts',(-4.92529033043266,12.2,9.73542083757215));
#239438=CARTESIAN_POINT('Ctrl Pts',(-4.92805060791798,12.2,9.73812737494249));
#239439=CARTESIAN_POINT('Ctrl Pts',(-4.93150095421049,12.2,9.74151054610225));
#239440=CARTESIAN_POINT('Ctrl Pts',(-4.9349747893646,12.2,9.74490274330435));
#239441=CARTESIAN_POINT('Ctrl Pts',(-4.93847207780089,12.2,9.74830370453012));
#239442=CARTESIAN_POINT('Ctrl Pts',(-4.94126990900737,12.2,9.75102447395558));
#239443=CARTESIAN_POINT('Ctrl Pts',(-4.9440827488653,12.2,9.75375085150939));
#239444=CARTESIAN_POINT('Ctrl Pts',(-4.94691058274166,12.2,9.75648270749163));
#239445=CARTESIAN_POINT('Ctrl Pts',(-4.94973841661802,12.2,9.75921456347388));
#239446=CARTESIAN_POINT('Ctrl Pts',(-4.9525812420822,12.2,9.76195189447893));
#239447=CARTESIAN_POINT('Ctrl Pts',(-4.95543904268393,12.2,9.76469457190673));
#239448=CARTESIAN_POINT('Ctrl Pts',(-4.95829684289628,12.2,9.76743724896085));
#239449=CARTESIAN_POINT('Ctrl Pts',(-4.96116961884604,12.2,9.77018527197734));
#239450=CARTESIAN_POINT('Ctrl Pts',(-4.96405735045637,12.2,9.77293850976476));
#239451=CARTESIAN_POINT('Ctrl Pts',(-4.96694508246016,12.2,9.7756917479273));
#239452=CARTESIAN_POINT('Ctrl Pts',(-4.96984777142485,12.2,9.77845020178681));
#239453=CARTESIAN_POINT('Ctrl Pts',(-4.97276539875204,12.2,9.78121374199347));
#239454=CARTESIAN_POINT('Ctrl Pts',(-4.97568302568169,12.2,9.78397728182361));
#239455=CARTESIAN_POINT('Ctrl Pts',(-4.97861559135946,12.2,9.78674590821701));
#239456=CARTESIAN_POINT('Ctrl Pts',(-4.98156307628418,12.2,9.78951949332327));
#239457=CARTESIAN_POINT('Ctrl Pts',(-4.98451056161049,12.2,9.79229307880742));
#239458=CARTESIAN_POINT('Ctrl Pts',(-4.98747296679975,12.2,9.79507162412833));
#239459=CARTESIAN_POINT('Ctrl Pts',(-4.99045027401854,12.2,9.79785500166922));
#239460=CARTESIAN_POINT('Ctrl Pts',(-4.99342758083166,12.2,9.80063837883087));
#239461=CARTESIAN_POINT('Ctrl Pts',(-4.99641978861896,12.2,9.80342658877003));
#239462=CARTESIAN_POINT('Ctrl Pts',(-4.9994268783554,12.2,9.80621950606972));
#239463=CARTESIAN_POINT('Ctrl Pts',(-5.00243396850156,12.2,9.80901242374994));
#239464=CARTESIAN_POINT('Ctrl Pts',(-5.00545594083468,12.2,9.81181004931772));
#239465=CARTESIAN_POINT('Ctrl Pts',(-5.0084927767234,12.2,9.81461225697076));
#239466=CARTESIAN_POINT('Ctrl Pts',(-5.01152961219835,12.2,9.817414464242));
#239467=CARTESIAN_POINT('Ctrl Pts',(-5.01458130980638,12.2,9.82022125617337));
#239468=CARTESIAN_POINT('Ctrl Pts',(-5.01764785199863,12.2,9.82303250799866));
#239469=CARTESIAN_POINT('Ctrl Pts',(-5.0214810300523,12.2,9.82654657306755));
#239470=CARTESIAN_POINT('Ctrl Pts',(-5.02533740099083,12.2,9.83006760720912));
#239471=CARTESIAN_POINT('Ctrl Pts',(-5.02921692680806,12.2,9.83359537335714));
#239472=CARTESIAN_POINT('Ctrl Pts',(-5.03232054763099,12.2,9.83641758642936));
#239473=CARTESIAN_POINT('Ctrl Pts',(-5.03543898912901,12.2,9.83924410764632));
#239474=CARTESIAN_POINT('Ctrl Pts',(-5.03857222852295,12.2,9.84207481718975));
#239475=CARTESIAN_POINT('Ctrl Pts',(-5.04170546748999,12.2,9.8449055263475));
#239476=CARTESIAN_POINT('Ctrl Pts',(-5.04485350569852,12.2,9.84774042287108));
#239477=CARTESIAN_POINT('Ctrl Pts',(-5.04801632321622,12.2,9.85057938802747));
#239478=CARTESIAN_POINT('Ctrl Pts',(-5.05117914116484,12.2,9.85341835357065));
#239479=CARTESIAN_POINT('Ctrl Pts',(-5.05435673855256,12.2,9.85626138720605));
#239480=CARTESIAN_POINT('Ctrl Pts',(-5.05754909518551,12.2,9.85910837148525));
#239481=CARTESIAN_POINT('Ctrl Pts',(-5.0607414513835,12.2,9.86195535537653));
#239482=CARTESIAN_POINT('Ctrl Pts',(-5.06394856671036,12.2,9.86480629036144));
#239483=CARTESIAN_POINT('Ctrl Pts',(-5.06717042022323,12.2,9.86766105701654));
#239484=CARTESIAN_POINT('Ctrl Pts',(-5.07039227417506,12.2,9.8705158240606));
#239485=CARTESIAN_POINT('Ctrl Pts',(-5.07362886695891,12.2,9.87337442401065));
#239486=CARTESIAN_POINT('Ctrl Pts',(-5.07688017752499,12.2,9.87623674149997));
#239487=CARTESIAN_POINT('Ctrl Pts',(-5.08013148809106,12.2,9.87909905898929));
#239488=CARTESIAN_POINT('Ctrl Pts',(-5.08339751522832,12.2,9.88196509166517));
#239489=CARTESIAN_POINT('Ctrl Pts',(-5.08667824051974,12.2,9.88483472721083));
#239490=CARTESIAN_POINT('Ctrl Pts',(-5.08995896536416,12.2,9.8877043623655));
#239491=CARTESIAN_POINT('Ctrl Pts',(-5.09325438740614,12.2,9.89057759854236));
#239492=CARTESIAN_POINT('Ctrl Pts',(-5.09656448553942,12.2,9.89345432176468));
#239493=CARTESIAN_POINT('Ctrl Pts',(-5.09987458412369,12.2,9.89633104537896));
#239494=CARTESIAN_POINT('Ctrl Pts',(-5.10319935768475,12.2,9.89921125672229));
#239495=CARTESIAN_POINT('Ctrl Pts',(-5.10653878631267,12.2,9.90209484171311));
#239496=CARTESIAN_POINT('Ctrl Pts',(-5.1098782144856,12.2,9.90497842631103));
#239497=CARTESIAN_POINT('Ctrl Pts',(-5.11323229825945,12.2,9.90786538397246));
#239498=CARTESIAN_POINT('Ctrl Pts',(-5.11660101448308,12.2,9.91075560451373));
#239499=CARTESIAN_POINT('Ctrl Pts',(-5.11912755176556,12.2,9.91292327001814));
#239500=CARTESIAN_POINT('Ctrl Pts',(-5.12166232012438,12.2,9.91509276950053));
#239501=CARTESIAN_POINT('Ctrl Pts',(-5.12420531099141,12.2,9.91726405757157));
#239502=CARTESIAN_POINT('Ctrl Pts',(-5.12674830185844,12.2,9.91943534564261));
#239503=CARTESIAN_POINT('Ctrl Pts',(-5.12929951468617,12.2,9.92160842102179));
#239504=CARTESIAN_POINT('Ctrl Pts',(-5.13185894042538,12.2,9.9237832371092));
#239505=CARTESIAN_POINT('Ctrl Pts',(-5.13527150838763,12.2,9.92668299215579));
#239506=CARTESIAN_POINT('Ctrl Pts',(-5.13869867745111,12.2,9.92958584293589));
#239507=CARTESIAN_POINT('Ctrl Pts',(-5.14214042475012,12.2,9.93249167798341));
#239508=CARTESIAN_POINT('Ctrl Pts',(-5.14472173498992,12.2,9.9346710540711));
#239509=CARTESIAN_POINT('Ctrl Pts',(-5.14731124624545,12.2,9.93685210977489));
#239510=CARTESIAN_POINT('Ctrl Pts',(-5.14990894852532,12.2,9.93903479877876));
#239511=CARTESIAN_POINT('Ctrl Pts',(-5.1525066508052,12.2,9.94121748778262));
#239512=CARTESIAN_POINT('Ctrl Pts',(-5.15511254422633,12.2,9.94340180893082));
#239513=CARTESIAN_POINT('Ctrl Pts',(-5.15772661967765,12.2,9.9455877180854));
#239514=CARTESIAN_POINT('Ctrl Pts',(-5.16034069512897,12.2,9.94777362723999));
#239515=CARTESIAN_POINT('Ctrl Pts',(-5.16296295342327,12.2,9.94996112395252));
#239516=CARTESIAN_POINT('Ctrl Pts',(-5.1655933836599,12.2,9.95215016208109));
#239517=CARTESIAN_POINT('Ctrl Pts',(-5.16822381437438,12.2,9.95433920060733));
#239518=CARTESIAN_POINT('Ctrl Pts',(-5.17086241754122,12.2,9.95652978147573));
#239519=CARTESIAN_POINT('Ctrl Pts',(-5.17350918330201,12.2,9.95872185896119));
#239520=CARTESIAN_POINT('Ctrl Pts',(-5.17615594858197,12.2,9.96091393604842));
#239521=CARTESIAN_POINT('Ctrl Pts',(-5.17881087761979,12.2,9.96310750943556));
#239522=CARTESIAN_POINT('Ctrl Pts',(-5.18147396027375,12.2,9.9653025350226));
#239523=CARTESIAN_POINT('Ctrl Pts',(-5.18413704292771,12.2,9.96749756060964));
#239524=CARTESIAN_POINT('Ctrl Pts',(-5.18680827830424,12.2,9.96969403832184));
#239525=CARTESIAN_POINT('Ctrl Pts',(-5.18948765805245,12.2,9.97189192250198));
#239526=CARTESIAN_POINT('Ctrl Pts',(-5.19216703780065,12.2,9.97408980668212));
#239527=CARTESIAN_POINT('Ctrl Pts',(-5.19485456193329,12.2,9.97628909860128));
#239528=CARTESIAN_POINT('Ctrl Pts',(-5.19755022018089,12.2,9.97848975323964));
#239529=CARTESIAN_POINT('Ctrl Pts',(-5.20024587842848,12.2,9.98069040787801));
#239530=CARTESIAN_POINT('Ctrl Pts',(-5.20294967075378,12.2,9.98289242505667));
#239531=CARTESIAN_POINT('Ctrl Pts',(-5.20566158794621,12.2,9.98509576118484));
#239532=CARTESIAN_POINT('Ctrl Pts',(-5.20837350513864,12.2,9.987299097313));
#239533=CARTESIAN_POINT('Ctrl Pts',(-5.21109354685551,12.2,9.98950375336609));
#239534=CARTESIAN_POINT('Ctrl Pts',(-5.21382170313026,12.2,9.99170968257742));
#239535=CARTESIAN_POINT('Ctrl Pts',(-5.21654985990064,12.2,9.99391561218949));
#239536=CARTESIAN_POINT('Ctrl Pts',(-5.21928613254833,12.2,9.99612281737696));
#239537=CARTESIAN_POINT('Ctrl Pts',(-5.22203050936495,12.2,9.99833125394809));
#239538=CARTESIAN_POINT('Ctrl Pts',(-5.22568967762284,12.2,10.0012758353743));
#239539=CARTESIAN_POINT('Ctrl Pts',(-5.22936325569896,12.2,10.0042226061868));
#239540=CARTESIAN_POINT('Ctrl Pts',(-5.23305121974749,12.2,10.0071714635146));
#239541=CARTESIAN_POINT('Ctrl Pts',(-5.23581719290951,12.2,10.009383106611));
#239542=CARTESIAN_POINT('Ctrl Pts',(-5.23859125816533,12.2,10.0115959230892));
#239543=CARTESIAN_POINT('Ctrl Pts',(-5.24137340448021,12.2,10.0138098702587));
#239544=CARTESIAN_POINT('Ctrl Pts',(-5.24415555079511,12.2,10.0160238174281));
#239545=CARTESIAN_POINT('Ctrl Pts',(-5.24694578005942,12.2,10.0182388963809));
#239546=CARTESIAN_POINT('Ctrl Pts',(-5.24974408087331,12.2,10.0204550625502));
#239547=CARTESIAN_POINT('Ctrl Pts',(-5.25254238219556,12.2,10.0226712291221));
#239548=CARTESIAN_POINT('Ctrl Pts',(-5.25534875605342,12.2,10.0248884837444));
#239549=CARTESIAN_POINT('Ctrl Pts',(-5.25816319179689,12.2,10.0271067847336));
#239550=CARTESIAN_POINT('Ctrl Pts',(-5.26097762702906,12.2,10.0293250853198));
#239551=CARTESIAN_POINT('Ctrl Pts',(-5.26380012431079,12.2,10.0315444305893));
#239552=CARTESIAN_POINT('Ctrl Pts',(-5.266630673542,12.2,10.033764779717));
#239553=CARTESIAN_POINT('Ctrl Pts',(-5.26946122277321,12.2,10.0359851288448));
#239554=CARTESIAN_POINT('Ctrl Pts',(-5.27229982520972,12.2,10.038206481656));
#239555=CARTESIAN_POINT('Ctrl Pts',(-5.27514646803592,12.2,10.040428796252));
#239556=CARTESIAN_POINT('Ctrl Pts',(-5.27894199163181,12.2,10.0433918822454));
#239557=CARTESIAN_POINT('Ctrl Pts',(-5.28275181314442,12.2,10.0463566772549));
#239558=CARTESIAN_POINT('Ctrl Pts',(-5.28657590660809,12.2,10.04932308329));
#239559=CARTESIAN_POINT('Ctrl Pts',(-5.28944397735713,12.2,10.0515478883215));
#239560=CARTESIAN_POINT('Ctrl Pts',(-5.29232007685848,12.2,10.0537735986116));
#239561=CARTESIAN_POINT('Ctrl Pts',(-5.29520419411207,12.2,10.056000173727));
#239562=CARTESIAN_POINT('Ctrl Pts',(-5.29808831084171,12.2,10.0582267484379));
#239563=CARTESIAN_POINT('Ctrl Pts',(-5.30098044610427,12.2,10.0604541888238));
#239564=CARTESIAN_POINT('Ctrl Pts',(-5.30388058883292,12.2,10.0626824524929));
#239565=CARTESIAN_POINT('Ctrl Pts',(-5.30678073156158,12.2,10.064910716162));
#239566=CARTESIAN_POINT('Ctrl Pts',(-5.30968888229533,12.2,10.0671398035896));
#239567=CARTESIAN_POINT('Ctrl Pts',(-5.31260503099433,12.2,10.0693696732687));
#239568=CARTESIAN_POINT('Ctrl Pts',(-5.31552117969334,12.2,10.0715995429478));
#239569=CARTESIAN_POINT('Ctrl Pts',(-5.31844532627391,12.2,10.0738301947855));
#239570=CARTESIAN_POINT('Ctrl Pts',(-5.32137745901401,12.2,10.0760615889646));
#239571=CARTESIAN_POINT('Ctrl Pts',(-5.32430959175411,12.2,10.0782929831437));
#239572=CARTESIAN_POINT('Ctrl Pts',(-5.32724971121994,12.2,10.0805251195378));
#239573=CARTESIAN_POINT('Ctrl Pts',(-5.33019780840379,12.2,10.0827579567483));
#239574=CARTESIAN_POINT('Ctrl Pts',(-5.33314590558764,12.2,10.0849907939588));
#239575=CARTESIAN_POINT('Ctrl Pts',(-5.33610197956263,12.2,10.0872243325942));
#239576=CARTESIAN_POINT('Ctrl Pts',(-5.33906601932884,12.2,10.0894585342213));
#239577=CARTESIAN_POINT('Ctrl Pts',(-5.34203005963352,12.2,10.0916927362542));
#239578=CARTESIAN_POINT('Ctrl Pts',(-5.34500206706547,12.2,10.0939276001457));
#239579=CARTESIAN_POINT('Ctrl Pts',(-5.34798202987464,12.2,10.0961630852207));
#239580=CARTESIAN_POINT('Ctrl Pts',(-5.35096199214246,12.2,10.0983985698895));
#239581=CARTESIAN_POINT('Ctrl Pts',(-5.35394991167131,12.2,10.1006346766355));
#239582=CARTESIAN_POINT('Ctrl Pts',(-5.35694577458804,12.2,10.1028713629577));
#239583=CARTESIAN_POINT('Ctrl Pts',(-5.35994163750477,12.2,10.1051080492799));
#239584=CARTESIAN_POINT('Ctrl Pts',(-5.36294544513714,12.2,10.1073453154085));
#239585=CARTESIAN_POINT('Ctrl Pts',(-5.36595718782008,12.2,10.1095831237439));
#239586=CARTESIAN_POINT('Ctrl Pts',(-5.36896893050303,12.2,10.1118209320793));
#239587=CARTESIAN_POINT('Ctrl Pts',(-5.37198860785999,12.2,10.1140592842313));
#239588=CARTESIAN_POINT('Ctrl Pts',(-5.37501621054167,12.2,10.1162981424833));
#239589=CARTESIAN_POINT('Ctrl Pts',(-5.37804381322335,12.2,10.1185370007353));
#239590=CARTESIAN_POINT('Ctrl Pts',(-5.38107934096302,12.2,10.1207763667539));
#239591=CARTESIAN_POINT('Ctrl Pts',(-5.3841227816434,12.2,10.1230161957558));
#239592=CARTESIAN_POINT('Ctrl Pts',(-5.38716622232378,12.2,10.1252560247578));
#239593=CARTESIAN_POINT('Ctrl Pts',(-5.39021757578411,12.2,10.1274963145027));
#239594=CARTESIAN_POINT('Ctrl Pts',(-5.39327682915818,12.2,10.1297370202831));
#239595=CARTESIAN_POINT('Ctrl Pts',(-5.39735583402745,12.2,10.1327246282618));
#239596=CARTESIAN_POINT('Ctrl Pts',(-5.40144888360935,12.2,10.135712968183));
#239597=CARTESIAN_POINT('Ctrl Pts',(-5.40555595979698,12.2,10.1387019907558));
#239598=CARTESIAN_POINT('Ctrl Pts',(-5.40863626665791,12.2,10.1409437574818));
#239599=CARTESIAN_POINT('Ctrl Pts',(-5.4117244634376,12.2,10.1431859115926));
#239600=CARTESIAN_POINT('Ctrl Pts',(-5.41482055400006,12.2,10.145428447));
#239601=CARTESIAN_POINT('Origin',(-5.66257110645729E-14,15.2,-1.77635683940025E-14));
#239602=CARTESIAN_POINT('',(-5.85257411492611,15.2,8.56667970922507));
#239603=CARTESIAN_POINT('',(-5.85257411492611,12.2,8.56667970922507));
#239604=CARTESIAN_POINT('',(-5.85257411500006,15.2,8.56667970899998));
#239605=CARTESIAN_POINT('Origin',(-5.66257110645729E-14,12.2,-1.77635683940025E-14));
#239606=CARTESIAN_POINT('Origin',(-5.66257110645729E-14,15.2,-1.77635683940025E-14));
#239607=CARTESIAN_POINT('Origin',(-5.66257110645729E-14,15.2,-1.77635683940025E-14));
#239608=CARTESIAN_POINT('',(-6.80355049700006,15.2,9.27155330199999));
#239609=CARTESIAN_POINT('',(-7.10901226959732,15.2,9.03946594391174));
#239610=CARTESIAN_POINT('Origin',(-5.66257110645729E-14,15.2,-1.77635683940025E-14));
#239611=CARTESIAN_POINT('',(-7.10901226959732,12.2,9.03946594391174));
#239612=CARTESIAN_POINT('',(-7.10901227000006,15.2,9.03946594399999));
#239613=CARTESIAN_POINT('',(-6.80355049700006,12.2,9.27155330199999));
#239614=CARTESIAN_POINT('Origin',(-5.66257110645729E-14,12.2,-1.77635683940025E-14));
#239615=CARTESIAN_POINT('',(-6.80355049700006,15.2,9.27155330199999));
#239616=CARTESIAN_POINT('Ctrl Pts',(-5.85257411500006,15.2,8.56667970999998));
#239617=CARTESIAN_POINT('Ctrl Pts',(-5.85257411500006,11.6,8.56667970999998));
#239618=CARTESIAN_POINT('Ctrl Pts',(-5.85268447900006,15.2,8.56681469199999));
#239619=CARTESIAN_POINT('Ctrl Pts',(-5.85268447900006,11.6,8.56681469199999));
#239620=CARTESIAN_POINT('Ctrl Pts',(-5.85290912900006,15.2,8.56708931899998));
#239621=CARTESIAN_POINT('Ctrl Pts',(-5.85290912900006,11.6,8.56708931899998));
#239622=CARTESIAN_POINT('Ctrl Pts',(-5.85324973300006,15.2,8.56750527399999));
#239623=CARTESIAN_POINT('Ctrl Pts',(-5.85324973300006,11.6,8.56750527399999));
#239624=CARTESIAN_POINT('Ctrl Pts',(-5.85370897500006,15.2,8.56806526199998));
#239625=CARTESIAN_POINT('Ctrl Pts',(-5.85370897500006,11.6,8.56806526199998));
#239626=CARTESIAN_POINT('Ctrl Pts',(-5.85429055500006,15.2,8.56877298399999));
#239627=CARTESIAN_POINT('Ctrl Pts',(-5.85429055500006,11.6,8.56877298399999));
#239628=CARTESIAN_POINT('Ctrl Pts',(-5.85488228100006,15.2,8.56949158299999));
#239629=CARTESIAN_POINT('Ctrl Pts',(-5.85488228100006,11.6,8.56949158299999));
#239630=CARTESIAN_POINT('Ctrl Pts',(-5.85548078500006,15.2,8.57021692599999));
#239631=CARTESIAN_POINT('Ctrl Pts',(-5.85548078500006,11.6,8.57021692599999));
#239632=CARTESIAN_POINT('Ctrl Pts',(-5.85608606100006,15.2,8.57094898199998));
#239633=CARTESIAN_POINT('Ctrl Pts',(-5.85608606100006,11.6,8.57094898199998));
#239634=CARTESIAN_POINT('Ctrl Pts',(-5.85669810700006,15.2,8.57168771799999));
#239635=CARTESIAN_POINT('Ctrl Pts',(-5.85669810700006,11.6,8.57168771799999));
#239636=CARTESIAN_POINT('Ctrl Pts',(-5.85731691800006,15.2,8.57243310399999));
#239637=CARTESIAN_POINT('Ctrl Pts',(-5.85731691800006,11.6,8.57243310399999));
#239638=CARTESIAN_POINT('Ctrl Pts',(-5.85794249300006,15.2,8.57318510299999));
#239639=CARTESIAN_POINT('Ctrl Pts',(-5.85794249300006,11.6,8.57318510299999));
#239640=CARTESIAN_POINT('Ctrl Pts',(-5.85857482800006,15.2,8.57394368799999));
#239641=CARTESIAN_POINT('Ctrl Pts',(-5.85857482800006,11.6,8.57394368799999));
#239642=CARTESIAN_POINT('Ctrl Pts',(-5.85921392000006,15.2,8.57470882699998));
#239643=CARTESIAN_POINT('Ctrl Pts',(-5.85921392000006,11.6,8.57470882699998));
#239644=CARTESIAN_POINT('Ctrl Pts',(-5.85985976600006,15.2,8.57548048599998));
#239645=CARTESIAN_POINT('Ctrl Pts',(-5.85985976600006,11.6,8.57548048599998));
#239646=CARTESIAN_POINT('Ctrl Pts',(-5.86051236100006,15.2,8.57625863599999));
#239647=CARTESIAN_POINT('Ctrl Pts',(-5.86051236100006,11.6,8.57625863599999));
#239648=CARTESIAN_POINT('Ctrl Pts',(-5.86117170400006,15.2,8.57704324399998));
#239649=CARTESIAN_POINT('Ctrl Pts',(-5.86117170400006,11.6,8.57704324399998));
#239650=CARTESIAN_POINT('Ctrl Pts',(-5.86183779200006,15.2,8.57783428099999));
#239651=CARTESIAN_POINT('Ctrl Pts',(-5.86183779200006,11.6,8.57783428099999));
#239652=CARTESIAN_POINT('Ctrl Pts',(-5.86251062000006,15.2,8.57863171499999));
#239653=CARTESIAN_POINT('Ctrl Pts',(-5.86251062000006,11.6,8.57863171499999));
#239654=CARTESIAN_POINT('Ctrl Pts',(-5.86319018700006,15.2,8.57943551599998));
#239655=CARTESIAN_POINT('Ctrl Pts',(-5.86319018700006,11.6,8.57943551599998));
#239656=CARTESIAN_POINT('Ctrl Pts',(-5.86387648700006,15.2,8.58024565199998));
#239657=CARTESIAN_POINT('Ctrl Pts',(-5.86387648700006,11.6,8.58024565199998));
#239658=CARTESIAN_POINT('Ctrl Pts',(-5.86456952000006,15.2,8.58106209499999));
#239659=CARTESIAN_POINT('Ctrl Pts',(-5.86456952000006,11.6,8.58106209499999));
#239660=CARTESIAN_POINT('Ctrl Pts',(-5.86526928000006,15.2,8.58188481199999));
#239661=CARTESIAN_POINT('Ctrl Pts',(-5.86526928000006,11.6,8.58188481199999));
#239662=CARTESIAN_POINT('Ctrl Pts',(-5.86597576600006,15.2,8.58271377599999));
#239663=CARTESIAN_POINT('Ctrl Pts',(-5.86597576600006,11.6,8.58271377599999));
#239664=CARTESIAN_POINT('Ctrl Pts',(-5.86668897300005,15.2,8.58354895499998));
#239665=CARTESIAN_POINT('Ctrl Pts',(-5.86668897300005,11.6,8.58354895499998));
#239666=CARTESIAN_POINT('Ctrl Pts',(-5.86740890000006,15.2,8.58439031999998));
#239667=CARTESIAN_POINT('Ctrl Pts',(-5.86740890000006,11.6,8.58439031999998));
#239668=CARTESIAN_POINT('Ctrl Pts',(-5.86813554300006,15.2,8.58523783999999));
#239669=CARTESIAN_POINT('Ctrl Pts',(-5.86813554300006,11.6,8.58523783999999));
#239670=CARTESIAN_POINT('Ctrl Pts',(-5.86886889700006,15.2,8.58609148699998));
#239671=CARTESIAN_POINT('Ctrl Pts',(-5.86886889700006,11.6,8.58609148699998));
#239672=CARTESIAN_POINT('Ctrl Pts',(-5.86960896300006,15.2,8.58695123199999));
#239673=CARTESIAN_POINT('Ctrl Pts',(-5.86960896300006,11.6,8.58695123199999));
#239674=CARTESIAN_POINT('Ctrl Pts',(-5.87035573300006,15.2,8.58781704399998));
#239675=CARTESIAN_POINT('Ctrl Pts',(-5.87035573300006,11.6,8.58781704399998));
#239676=CARTESIAN_POINT('Ctrl Pts',(-5.87110920700006,15.2,8.58868889599999));
#239677=CARTESIAN_POINT('Ctrl Pts',(-5.87110920700006,11.6,8.58868889599999));
#239678=CARTESIAN_POINT('Ctrl Pts',(-5.87186938100006,15.2,8.58956675699999));
#239679=CARTESIAN_POINT('Ctrl Pts',(-5.87186938100006,11.6,8.58956675699999));
#239680=CARTESIAN_POINT('Ctrl Pts',(-5.87263625200006,15.2,8.59045059899999));
#239681=CARTESIAN_POINT('Ctrl Pts',(-5.87263625200006,11.6,8.59045059899999));
#239682=CARTESIAN_POINT('Ctrl Pts',(-5.87340981600006,15.2,8.59134039399999));
#239683=CARTESIAN_POINT('Ctrl Pts',(-5.87340981600006,11.6,8.59134039399999));
#239684=CARTESIAN_POINT('Ctrl Pts',(-5.87419007000006,15.2,8.59223611299999));
#239685=CARTESIAN_POINT('Ctrl Pts',(-5.87419007000006,11.6,8.59223611299999));
#239686=CARTESIAN_POINT('Ctrl Pts',(-5.87497701300006,15.2,8.59313772699998));
#239687=CARTESIAN_POINT('Ctrl Pts',(-5.87497701300006,11.6,8.59313772699998));
#239688=CARTESIAN_POINT('Ctrl Pts',(-5.87577063900006,15.2,8.59404520899999));
#239689=CARTESIAN_POINT('Ctrl Pts',(-5.87577063900006,11.6,8.59404520899999));
#239690=CARTESIAN_POINT('Ctrl Pts',(-5.87657094700006,15.2,8.59495852899999));
#239691=CARTESIAN_POINT('Ctrl Pts',(-5.87657094700006,11.6,8.59495852899999));
#239692=CARTESIAN_POINT('Ctrl Pts',(-5.87737793200006,15.2,8.59587765999999));
#239693=CARTESIAN_POINT('Ctrl Pts',(-5.87737793200006,11.6,8.59587765999999));
#239694=CARTESIAN_POINT('Ctrl Pts',(-5.87819159300006,15.2,8.59680257399998));
#239695=CARTESIAN_POINT('Ctrl Pts',(-5.87819159300006,11.6,8.59680257399998));
#239696=CARTESIAN_POINT('Ctrl Pts',(-5.87901192500006,15.2,8.59773324399999));
#239697=CARTESIAN_POINT('Ctrl Pts',(-5.87901192500006,11.6,8.59773324399999));
#239698=CARTESIAN_POINT('Ctrl Pts',(-5.87983892500006,15.2,8.59866964099999));
#239699=CARTESIAN_POINT('Ctrl Pts',(-5.87983892500006,11.6,8.59866964099999));
#239700=CARTESIAN_POINT('Ctrl Pts',(-5.88067259200006,15.2,8.59961173899999));
#239701=CARTESIAN_POINT('Ctrl Pts',(-5.88067259200006,11.6,8.59961173899999));
#239702=CARTESIAN_POINT('Ctrl Pts',(-5.88151291900005,15.2,8.60055950999998));
#239703=CARTESIAN_POINT('Ctrl Pts',(-5.88151291900005,11.6,8.60055950999998));
#239704=CARTESIAN_POINT('Ctrl Pts',(-5.88235990700006,15.2,8.60151292499998));
#239705=CARTESIAN_POINT('Ctrl Pts',(-5.88235990700006,11.6,8.60151292499998));
#239706=CARTESIAN_POINT('Ctrl Pts',(-5.88321355000006,15.2,8.60247195899999));
#239707=CARTESIAN_POINT('Ctrl Pts',(-5.88321355000006,11.6,8.60247195899999));
#239708=CARTESIAN_POINT('Ctrl Pts',(-5.88407384700006,15.2,8.60343658499998));
#239709=CARTESIAN_POINT('Ctrl Pts',(-5.88407384700006,11.6,8.60343658499998));
#239710=CARTESIAN_POINT('Ctrl Pts',(-5.88494079200006,15.2,8.60440677399998));
#239711=CARTESIAN_POINT('Ctrl Pts',(-5.88494079200006,11.6,8.60440677399998));
#239712=CARTESIAN_POINT('Ctrl Pts',(-5.88581438400006,15.2,8.60538250099999));
#239713=CARTESIAN_POINT('Ctrl Pts',(-5.88581438400006,11.6,8.60538250099999));
#239714=CARTESIAN_POINT('Ctrl Pts',(-5.88669462000006,15.2,8.60636373999998));
#239715=CARTESIAN_POINT('Ctrl Pts',(-5.88669462000006,11.6,8.60636373999998));
#239716=CARTESIAN_POINT('Ctrl Pts',(-5.88758149600006,15.2,8.60735046199999));
#239717=CARTESIAN_POINT('Ctrl Pts',(-5.88758149600006,11.6,8.60735046199999));
#239718=CARTESIAN_POINT('Ctrl Pts',(-5.88847500900005,15.2,8.60834264199998));
#239719=CARTESIAN_POINT('Ctrl Pts',(-5.88847500900005,11.6,8.60834264199998));
#239720=CARTESIAN_POINT('Ctrl Pts',(-5.88937515600006,15.2,8.60934025399999));
#239721=CARTESIAN_POINT('Ctrl Pts',(-5.88937515600006,11.6,8.60934025399999));
#239722=CARTESIAN_POINT('Ctrl Pts',(-5.89028193300006,15.2,8.61034327099999));
#239723=CARTESIAN_POINT('Ctrl Pts',(-5.89028193300006,11.6,8.61034327099999));
#239724=CARTESIAN_POINT('Ctrl Pts',(-5.89119533900006,15.2,8.61135166799999));
#239725=CARTESIAN_POINT('Ctrl Pts',(-5.89119533900006,11.6,8.61135166799999));
#239726=CARTESIAN_POINT('Ctrl Pts',(-5.89211536900006,15.2,8.61236541799999));
#239727=CARTESIAN_POINT('Ctrl Pts',(-5.89211536900006,11.6,8.61236541799999));
#239728=CARTESIAN_POINT('Ctrl Pts',(-5.89304202000006,15.2,8.61338449399998));
#239729=CARTESIAN_POINT('Ctrl Pts',(-5.89304202000006,11.6,8.61338449399998));
#239730=CARTESIAN_POINT('Ctrl Pts',(-5.89397529000006,15.2,8.61440887399999));
#239731=CARTESIAN_POINT('Ctrl Pts',(-5.89397529000006,11.6,8.61440887399999));
#239732=CARTESIAN_POINT('Ctrl Pts',(-5.89491517500006,15.2,8.61543852799999));
#239733=CARTESIAN_POINT('Ctrl Pts',(-5.89491517500006,11.6,8.61543852799999));
#239734=CARTESIAN_POINT('Ctrl Pts',(-5.89586167100006,15.2,8.61647343299998));
#239735=CARTESIAN_POINT('Ctrl Pts',(-5.89586167100006,11.6,8.61647343299998));
#239736=CARTESIAN_POINT('Ctrl Pts',(-5.89681477700006,15.2,8.61751356399999));
#239737=CARTESIAN_POINT('Ctrl Pts',(-5.89681477700006,11.6,8.61751356399999));
#239738=CARTESIAN_POINT('Ctrl Pts',(-5.89777448900006,15.2,8.61855889399998));
#239739=CARTESIAN_POINT('Ctrl Pts',(-5.89777448900006,11.6,8.61855889399998));
#239740=CARTESIAN_POINT('Ctrl Pts',(-5.89874080200006,15.2,8.61960939799998));
#239741=CARTESIAN_POINT('Ctrl Pts',(-5.89874080200006,11.6,8.61960939799998));
#239742=CARTESIAN_POINT('Ctrl Pts',(-5.89971371600006,15.2,8.62066505199999));
#239743=CARTESIAN_POINT('Ctrl Pts',(-5.89971371600006,11.6,8.62066505199999));
#239744=CARTESIAN_POINT('Ctrl Pts',(-5.90069322500006,15.2,8.62172583099999));
#239745=CARTESIAN_POINT('Ctrl Pts',(-5.90069322500006,11.6,8.62172583099999));
#239746=CARTESIAN_POINT('Ctrl Pts',(-5.90167932900005,15.2,8.62279170899999));
#239747=CARTESIAN_POINT('Ctrl Pts',(-5.90167932900005,11.6,8.62279170899999));
#239748=CARTESIAN_POINT('Ctrl Pts',(-5.90267202200006,15.2,8.62386266099998));
#239749=CARTESIAN_POINT('Ctrl Pts',(-5.90267202200006,11.6,8.62386266099998));
#239750=CARTESIAN_POINT('Ctrl Pts',(-5.90367130100006,15.2,8.62493866499998));
#239751=CARTESIAN_POINT('Ctrl Pts',(-5.90367130100006,11.6,8.62493866499998));
#239752=CARTESIAN_POINT('Ctrl Pts',(-5.90467716500005,15.2,8.62601969299998));
#239753=CARTESIAN_POINT('Ctrl Pts',(-5.90467716500005,11.6,8.62601969299998));
#239754=CARTESIAN_POINT('Ctrl Pts',(-5.90568960800006,15.2,8.62710572199998));
#239755=CARTESIAN_POINT('Ctrl Pts',(-5.90568960800006,11.6,8.62710572199998));
#239756=CARTESIAN_POINT('Ctrl Pts',(-5.90670863000006,15.2,8.62819672699998));
#239757=CARTESIAN_POINT('Ctrl Pts',(-5.90670863000006,11.6,8.62819672699998));
#239758=CARTESIAN_POINT('Ctrl Pts',(-5.90773422600006,15.2,8.62929268599999));
#239759=CARTESIAN_POINT('Ctrl Pts',(-5.90773422600006,11.6,8.62929268599999));
#239760=CARTESIAN_POINT('Ctrl Pts',(-5.90876639200006,15.2,8.63039357199998));
#239761=CARTESIAN_POINT('Ctrl Pts',(-5.90876639200006,11.6,8.63039357199998));
#239762=CARTESIAN_POINT('Ctrl Pts',(-5.90980512700006,15.2,8.63149936299998));
#239763=CARTESIAN_POINT('Ctrl Pts',(-5.90980512700006,11.6,8.63149936299998));
#239764=CARTESIAN_POINT('Ctrl Pts',(-5.91085042600006,15.2,8.63261003299998));
#239765=CARTESIAN_POINT('Ctrl Pts',(-5.91085042600006,11.6,8.63261003299998));
#239766=CARTESIAN_POINT('Ctrl Pts',(-5.91190228800006,15.2,8.63372555999998));
#239767=CARTESIAN_POINT('Ctrl Pts',(-5.91190228800006,11.6,8.63372555999998));
#239768=CARTESIAN_POINT('Ctrl Pts',(-5.91296070800006,15.2,8.63484591899999));
#239769=CARTESIAN_POINT('Ctrl Pts',(-5.91296070800006,11.6,8.63484591899999));
#239770=CARTESIAN_POINT('Ctrl Pts',(-5.91402568300006,15.2,8.63597108799999));
#239771=CARTESIAN_POINT('Ctrl Pts',(-5.91402568300006,11.6,8.63597108799999));
#239772=CARTESIAN_POINT('Ctrl Pts',(-5.91509721000006,15.2,8.63710104099999));
#239773=CARTESIAN_POINT('Ctrl Pts',(-5.91509721000006,11.6,8.63710104099999));
#239774=CARTESIAN_POINT('Ctrl Pts',(-5.91617528800006,15.2,8.63823575499998));
#239775=CARTESIAN_POINT('Ctrl Pts',(-5.91617528800006,11.6,8.63823575499998));
#239776=CARTESIAN_POINT('Ctrl Pts',(-5.91725991000006,15.2,8.63937520899999));
#239777=CARTESIAN_POINT('Ctrl Pts',(-5.91725991000006,11.6,8.63937520899999));
#239778=CARTESIAN_POINT('Ctrl Pts',(-5.91835107500006,15.2,8.64051937699998));
#239779=CARTESIAN_POINT('Ctrl Pts',(-5.91835107500006,11.6,8.64051937699998));
#239780=CARTESIAN_POINT('Ctrl Pts',(-5.91944878200006,15.2,8.64166823699998));
#239781=CARTESIAN_POINT('Ctrl Pts',(-5.91944878200006,11.6,8.64166823699998));
#239782=CARTESIAN_POINT('Ctrl Pts',(-5.92055302300006,15.2,8.64282176599998));
#239783=CARTESIAN_POINT('Ctrl Pts',(-5.92055302300006,11.6,8.64282176599998));
#239784=CARTESIAN_POINT('Ctrl Pts',(-5.92166379800006,15.2,8.64397993999999));
#239785=CARTESIAN_POINT('Ctrl Pts',(-5.92166379800006,11.6,8.64397993999999));
#239786=CARTESIAN_POINT('Ctrl Pts',(-5.92278110400006,15.2,8.64514273699999));
#239787=CARTESIAN_POINT('Ctrl Pts',(-5.92278110400006,11.6,8.64514273699999));
#239788=CARTESIAN_POINT('Ctrl Pts',(-5.92390493600006,15.2,8.64631013299999));
#239789=CARTESIAN_POINT('Ctrl Pts',(-5.92390493600006,11.6,8.64631013299999));
#239790=CARTESIAN_POINT('Ctrl Pts',(-5.92503529200005,15.2,8.64748210699998));
#239791=CARTESIAN_POINT('Ctrl Pts',(-5.92503529200005,11.6,8.64748210699998));
#239792=CARTESIAN_POINT('Ctrl Pts',(-5.92617217000006,15.2,8.64865863599999));
#239793=CARTESIAN_POINT('Ctrl Pts',(-5.92617217000006,11.6,8.64865863599999));
#239794=CARTESIAN_POINT('Ctrl Pts',(-5.92731556500006,15.2,8.64983969599999));
#239795=CARTESIAN_POINT('Ctrl Pts',(-5.92731556500006,11.6,8.64983969599999));
#239796=CARTESIAN_POINT('Ctrl Pts',(-5.92846547400006,15.2,8.65102526599999));
#239797=CARTESIAN_POINT('Ctrl Pts',(-5.92846547400006,11.6,8.65102526599999));
#239798=CARTESIAN_POINT('Ctrl Pts',(-5.92962189500006,15.2,8.65221532199998));
#239799=CARTESIAN_POINT('Ctrl Pts',(-5.92962189500006,11.6,8.65221532199998));
#239800=CARTESIAN_POINT('Ctrl Pts',(-5.93078482300006,15.2,8.65340984299999));
#239801=CARTESIAN_POINT('Ctrl Pts',(-5.93078482300006,11.6,8.65340984299999));
#239802=CARTESIAN_POINT('Ctrl Pts',(-5.93195425800006,15.2,8.65460880699998));
#239803=CARTESIAN_POINT('Ctrl Pts',(-5.93195425800006,11.6,8.65460880699998));
#239804=CARTESIAN_POINT('Ctrl Pts',(-5.93313019300005,15.2,8.65581219199999));
#239805=CARTESIAN_POINT('Ctrl Pts',(-5.93313019300005,11.6,8.65581219199999));
#239806=CARTESIAN_POINT('Ctrl Pts',(-5.93431262700006,15.2,8.65701997399999));
#239807=CARTESIAN_POINT('Ctrl Pts',(-5.93431262700006,11.6,8.65701997399999));
#239808=CARTESIAN_POINT('Ctrl Pts',(-5.93550155700005,15.2,8.65823213299999));
#239809=CARTESIAN_POINT('Ctrl Pts',(-5.93550155700005,11.6,8.65823213299999));
#239810=CARTESIAN_POINT('Ctrl Pts',(-5.93669698000006,15.2,8.65944864499999));
#239811=CARTESIAN_POINT('Ctrl Pts',(-5.93669698000006,11.6,8.65944864499999));
#239812=CARTESIAN_POINT('Ctrl Pts',(-5.93789889100006,15.2,8.66066949099999));
#239813=CARTESIAN_POINT('Ctrl Pts',(-5.93789889100006,11.6,8.66066949099999));
#239814=CARTESIAN_POINT('Ctrl Pts',(-5.93910728800005,15.2,8.66189464799999));
#239815=CARTESIAN_POINT('Ctrl Pts',(-5.93910728800005,11.6,8.66189464799999));
#239816=CARTESIAN_POINT('Ctrl Pts',(-5.94032216900006,15.2,8.66312409399999));
#239817=CARTESIAN_POINT('Ctrl Pts',(-5.94032216900006,11.6,8.66312409399999));
#239818=CARTESIAN_POINT('Ctrl Pts',(-5.94154353000006,15.2,8.66435780699998));
#239819=CARTESIAN_POINT('Ctrl Pts',(-5.94154353000006,11.6,8.66435780699998));
#239820=CARTESIAN_POINT('Ctrl Pts',(-5.94277136700006,15.2,8.66559576699999));
#239821=CARTESIAN_POINT('Ctrl Pts',(-5.94277136700006,11.6,8.66559576699999));
#239822=CARTESIAN_POINT('Ctrl Pts',(-5.94400567700006,15.2,8.66683795199998));
#239823=CARTESIAN_POINT('Ctrl Pts',(-5.94400567700006,11.6,8.66683795199998));
#239824=CARTESIAN_POINT('Ctrl Pts',(-5.94524645700006,15.2,8.66808433999999));
#239825=CARTESIAN_POINT('Ctrl Pts',(-5.94524645700006,11.6,8.66808433999999));
#239826=CARTESIAN_POINT('Ctrl Pts',(-5.94649370400006,15.2,8.66933490999998));
#239827=CARTESIAN_POINT('Ctrl Pts',(-5.94649370400006,11.6,8.66933490999998));
#239828=CARTESIAN_POINT('Ctrl Pts',(-5.94774741600006,15.2,8.67058964199998));
#239829=CARTESIAN_POINT('Ctrl Pts',(-5.94774741600006,11.6,8.67058964199998));
#239830=CARTESIAN_POINT('Ctrl Pts',(-5.94900758800006,15.2,8.67184851399998));
#239831=CARTESIAN_POINT('Ctrl Pts',(-5.94900758800006,11.6,8.67184851399998));
#239832=CARTESIAN_POINT('Ctrl Pts',(-5.95027421800006,15.2,8.67311150599999));
#239833=CARTESIAN_POINT('Ctrl Pts',(-5.95027421800006,11.6,8.67311150599999));
#239834=CARTESIAN_POINT('Ctrl Pts',(-5.95154730300006,15.2,8.67437859499999));
#239835=CARTESIAN_POINT('Ctrl Pts',(-5.95154730300006,11.6,8.67437859499999));
#239836=CARTESIAN_POINT('Ctrl Pts',(-5.95282683800006,15.2,8.67564976199999));
#239837=CARTESIAN_POINT('Ctrl Pts',(-5.95282683800006,11.6,8.67564976199999));
#239838=CARTESIAN_POINT('Ctrl Pts',(-5.95411282100006,15.2,8.67692498599999));
#239839=CARTESIAN_POINT('Ctrl Pts',(-5.95411282100006,11.6,8.67692498599999));
#239840=CARTESIAN_POINT('Ctrl Pts',(-5.95540525000006,15.2,8.67820424599999));
#239841=CARTESIAN_POINT('Ctrl Pts',(-5.95540525000006,11.6,8.67820424599999));
#239842=CARTESIAN_POINT('Ctrl Pts',(-5.95670412000006,15.2,8.67948751999998));
#239843=CARTESIAN_POINT('Ctrl Pts',(-5.95670412000006,11.6,8.67948751999998));
#239844=CARTESIAN_POINT('Ctrl Pts',(-5.95800942900006,15.2,8.68077478999999));
#239845=CARTESIAN_POINT('Ctrl Pts',(-5.95800942900006,11.6,8.68077478999999));
#239846=CARTESIAN_POINT('Ctrl Pts',(-5.95932117300006,15.2,8.68206603399998));
#239847=CARTESIAN_POINT('Ctrl Pts',(-5.95932117300006,11.6,8.68206603399998));
#239848=CARTESIAN_POINT('Ctrl Pts',(-5.96063935000006,15.2,8.68336123199999));
#239849=CARTESIAN_POINT('Ctrl Pts',(-5.96063935000006,11.6,8.68336123199999));
#239850=CARTESIAN_POINT('Ctrl Pts',(-5.96196395500006,15.2,8.68466036399998));
#239851=CARTESIAN_POINT('Ctrl Pts',(-5.96196395500006,11.6,8.68466036399998));
#239852=CARTESIAN_POINT('Ctrl Pts',(-5.96329498600006,15.2,8.68596340999999));
#239853=CARTESIAN_POINT('Ctrl Pts',(-5.96329498600006,11.6,8.68596340999999));
#239854=CARTESIAN_POINT('Ctrl Pts',(-5.96463244000006,15.2,8.68727034899998));
#239855=CARTESIAN_POINT('Ctrl Pts',(-5.96463244000006,11.6,8.68727034899998));
#239856=CARTESIAN_POINT('Ctrl Pts',(-5.96597631400006,15.2,8.68858115999998));
#239857=CARTESIAN_POINT('Ctrl Pts',(-5.96597631400006,11.6,8.68858115999998));
#239858=CARTESIAN_POINT('Ctrl Pts',(-5.96732660300006,15.2,8.68989582599998));
#239859=CARTESIAN_POINT('Ctrl Pts',(-5.96732660300006,11.6,8.68989582599998));
#239860=CARTESIAN_POINT('Ctrl Pts',(-5.96868330600006,15.2,8.69121432499998));
#239861=CARTESIAN_POINT('Ctrl Pts',(-5.96868330600006,11.6,8.69121432499998));
#239862=CARTESIAN_POINT('Ctrl Pts',(-5.97004641900006,15.2,8.69253663699999));
#239863=CARTESIAN_POINT('Ctrl Pts',(-5.97004641900006,11.6,8.69253663699999));
#239864=CARTESIAN_POINT('Ctrl Pts',(-5.97141593900006,15.2,8.69386274199999));
#239865=CARTESIAN_POINT('Ctrl Pts',(-5.97141593900006,11.6,8.69386274199999));
#239866=CARTESIAN_POINT('Ctrl Pts',(-5.97279186200006,15.2,8.69519262299999));
#239867=CARTESIAN_POINT('Ctrl Pts',(-5.97279186200006,11.6,8.69519262299999));
#239868=CARTESIAN_POINT('Ctrl Pts',(-5.97417418500005,15.2,8.69652625599999));
#239869=CARTESIAN_POINT('Ctrl Pts',(-5.97417418500005,11.6,8.69652625599999));
#239870=CARTESIAN_POINT('Ctrl Pts',(-5.97556290600005,15.2,8.69786362499998));
#239871=CARTESIAN_POINT('Ctrl Pts',(-5.97556290600005,11.6,8.69786362499998));
#239872=CARTESIAN_POINT('Ctrl Pts',(-5.97695802100006,15.2,8.69920470999999));
#239873=CARTESIAN_POINT('Ctrl Pts',(-5.97695802100006,11.6,8.69920470999999));
#239874=CARTESIAN_POINT('Ctrl Pts',(-5.97835952600006,15.2,8.70054948899998));
#239875=CARTESIAN_POINT('Ctrl Pts',(-5.97835952600006,11.6,8.70054948899998));
#239876=CARTESIAN_POINT('Ctrl Pts',(-5.97976742000006,15.2,8.70189794599998));
#239877=CARTESIAN_POINT('Ctrl Pts',(-5.97976742000006,11.6,8.70189794599998));
#239878=CARTESIAN_POINT('Ctrl Pts',(-5.98118169700006,15.2,8.70325005899998));
#239879=CARTESIAN_POINT('Ctrl Pts',(-5.98118169700006,11.6,8.70325005899998));
#239880=CARTESIAN_POINT('Ctrl Pts',(-5.98260235600006,15.2,8.70460580999998));
#239881=CARTESIAN_POINT('Ctrl Pts',(-5.98260235600006,11.6,8.70460580999998));
#239882=CARTESIAN_POINT('Ctrl Pts',(-5.98402939300006,15.2,8.70596517899998));
#239883=CARTESIAN_POINT('Ctrl Pts',(-5.98402939300006,11.6,8.70596517899998));
#239884=CARTESIAN_POINT('Ctrl Pts',(-5.98546280500006,15.2,8.70732814899998));
#239885=CARTESIAN_POINT('Ctrl Pts',(-5.98546280500006,11.6,8.70732814899998));
#239886=CARTESIAN_POINT('Ctrl Pts',(-5.98690258900006,15.2,8.70869469899999));
#239887=CARTESIAN_POINT('Ctrl Pts',(-5.98690258900006,11.6,8.70869469899999));
#239888=CARTESIAN_POINT('Ctrl Pts',(-5.98834874000006,15.2,8.71006481099998));
#239889=CARTESIAN_POINT('Ctrl Pts',(-5.98834874000006,11.6,8.71006481099998));
#239890=CARTESIAN_POINT('Ctrl Pts',(-5.98980125800006,15.2,8.71143846499999));
#239891=CARTESIAN_POINT('Ctrl Pts',(-5.98980125800006,11.6,8.71143846499999));
#239892=CARTESIAN_POINT('Ctrl Pts',(-5.99126013800006,15.2,8.71281564199998));
#239893=CARTESIAN_POINT('Ctrl Pts',(-5.99126013800006,11.6,8.71281564199998));
#239894=CARTESIAN_POINT('Ctrl Pts',(-5.99272537600006,15.2,8.71419632499999));
#239895=CARTESIAN_POINT('Ctrl Pts',(-5.99272537600006,11.6,8.71419632499999));
#239896=CARTESIAN_POINT('Ctrl Pts',(-5.99419697000006,15.2,8.71558049499999));
#239897=CARTESIAN_POINT('Ctrl Pts',(-5.99419697000006,11.6,8.71558049499999));
#239898=CARTESIAN_POINT('Ctrl Pts',(-5.99567491600006,15.2,8.71696813099998));
#239899=CARTESIAN_POINT('Ctrl Pts',(-5.99567491600006,11.6,8.71696813099998));
#239900=CARTESIAN_POINT('Ctrl Pts',(-5.99715921200006,15.2,8.71835921799999));
#239901=CARTESIAN_POINT('Ctrl Pts',(-5.99715921200006,11.6,8.71835921799999));
#239902=CARTESIAN_POINT('Ctrl Pts',(-5.99864985300006,15.2,8.71975373399999));
#239903=CARTESIAN_POINT('Ctrl Pts',(-5.99864985300006,11.6,8.71975373399999));
#239904=CARTESIAN_POINT('Ctrl Pts',(-6.00014683800006,15.2,8.72115166199999));
#239905=CARTESIAN_POINT('Ctrl Pts',(-6.00014683800006,11.6,8.72115166199999));
#239906=CARTESIAN_POINT('Ctrl Pts',(-6.00165016300005,15.2,8.72255298499999));
#239907=CARTESIAN_POINT('Ctrl Pts',(-6.00165016300005,11.6,8.72255298499999));
#239908=CARTESIAN_POINT('Ctrl Pts',(-6.00315982300006,15.2,8.72395768299998));
#239909=CARTESIAN_POINT('Ctrl Pts',(-6.00315982300006,11.6,8.72395768299998));
#239910=CARTESIAN_POINT('Ctrl Pts',(-6.00467581700006,15.2,8.72536573799999));
#239911=CARTESIAN_POINT('Ctrl Pts',(-6.00467581700006,11.6,8.72536573799999));
#239912=CARTESIAN_POINT('Ctrl Pts',(-6.00619814200006,15.2,8.72677713199998));
#239913=CARTESIAN_POINT('Ctrl Pts',(-6.00619814200006,11.6,8.72677713199998));
#239914=CARTESIAN_POINT('Ctrl Pts',(-6.00772679200006,15.2,8.72819184599999));
#239915=CARTESIAN_POINT('Ctrl Pts',(-6.00772679200006,11.6,8.72819184599999));
#239916=CARTESIAN_POINT('Ctrl Pts',(-6.00926176600006,15.2,8.72960986299999));
#239917=CARTESIAN_POINT('Ctrl Pts',(-6.00926176600006,11.6,8.72960986299999));
#239918=CARTESIAN_POINT('Ctrl Pts',(-6.01080306100005,15.2,8.73103116499998));
#239919=CARTESIAN_POINT('Ctrl Pts',(-6.01080306100005,11.6,8.73103116499998));
#239920=CARTESIAN_POINT('Ctrl Pts',(-6.01235067300006,15.2,8.73245573399998));
#239921=CARTESIAN_POINT('Ctrl Pts',(-6.01235067300006,11.6,8.73245573399998));
#239922=CARTESIAN_POINT('Ctrl Pts',(-6.01390459900006,15.2,8.73388355199998));
#239923=CARTESIAN_POINT('Ctrl Pts',(-6.01390459900006,11.6,8.73388355199998));
#239924=CARTESIAN_POINT('Ctrl Pts',(-6.01546483600006,15.2,8.73531459999998));
#239925=CARTESIAN_POINT('Ctrl Pts',(-6.01546483600006,11.6,8.73531459999998));
#239926=CARTESIAN_POINT('Ctrl Pts',(-6.01703137900006,15.2,8.73674886199998));
#239927=CARTESIAN_POINT('Ctrl Pts',(-6.01703137900006,11.6,8.73674886199998));
#239928=CARTESIAN_POINT('Ctrl Pts',(-6.01860422800006,15.2,8.73818631899999));
#239929=CARTESIAN_POINT('Ctrl Pts',(-6.01860422800006,11.6,8.73818631899999));
#239930=CARTESIAN_POINT('Ctrl Pts',(-6.02018337700006,15.2,8.73962695399998));
#239931=CARTESIAN_POINT('Ctrl Pts',(-6.02018337700006,11.6,8.73962695399998));
#239932=CARTESIAN_POINT('Ctrl Pts',(-6.02176882400006,15.2,8.74107074799999));
#239933=CARTESIAN_POINT('Ctrl Pts',(-6.02176882400006,11.6,8.74107074799999));
#239934=CARTESIAN_POINT('Ctrl Pts',(-6.02336056600006,15.2,8.74251768599999));
#239935=CARTESIAN_POINT('Ctrl Pts',(-6.02336056600006,11.6,8.74251768599999));
#239936=CARTESIAN_POINT('Ctrl Pts',(-6.02495860000006,15.2,8.74396774899999));
#239937=CARTESIAN_POINT('Ctrl Pts',(-6.02495860000006,11.6,8.74396774899999));
#239938=CARTESIAN_POINT('Ctrl Pts',(-6.02656292100006,15.2,8.74542091899999));
#239939=CARTESIAN_POINT('Ctrl Pts',(-6.02656292100006,11.6,8.74542091899999));
#239940=CARTESIAN_POINT('Ctrl Pts',(-6.02817352800006,15.2,8.74687717999999));
#239941=CARTESIAN_POINT('Ctrl Pts',(-6.02817352800006,11.6,8.74687717999999));
#239942=CARTESIAN_POINT('Ctrl Pts',(-6.02979041500006,15.2,8.74833651299999));
#239943=CARTESIAN_POINT('Ctrl Pts',(-6.02979041500006,11.6,8.74833651299999));
#239944=CARTESIAN_POINT('Ctrl Pts',(-6.03141358200006,15.2,8.74979890199998));
#239945=CARTESIAN_POINT('Ctrl Pts',(-6.03141358200006,11.6,8.74979890199998));
#239946=CARTESIAN_POINT('Ctrl Pts',(-6.03304302400006,15.2,8.75126432999998));
#239947=CARTESIAN_POINT('Ctrl Pts',(-6.03304302400006,11.6,8.75126432999998));
#239948=CARTESIAN_POINT('Ctrl Pts',(-6.03467873800006,15.2,8.75273277899998));
#239949=CARTESIAN_POINT('Ctrl Pts',(-6.03467873800006,11.6,8.75273277899998));
#239950=CARTESIAN_POINT('Ctrl Pts',(-6.03632072000006,15.2,8.75420423299998));
#239951=CARTESIAN_POINT('Ctrl Pts',(-6.03632072000006,11.6,8.75420423299998));
#239952=CARTESIAN_POINT('Ctrl Pts',(-6.03796896800006,15.2,8.75567867399998));
#239953=CARTESIAN_POINT('Ctrl Pts',(-6.03796896800006,11.6,8.75567867399998));
#239954=CARTESIAN_POINT('Ctrl Pts',(-6.03962347900006,15.2,8.75715608399998));
#239955=CARTESIAN_POINT('Ctrl Pts',(-6.03962347900006,11.6,8.75715608399998));
#239956=CARTESIAN_POINT('Ctrl Pts',(-6.04128424700006,15.2,8.75863644799999));
#239957=CARTESIAN_POINT('Ctrl Pts',(-6.04128424700006,11.6,8.75863644799999));
#239958=CARTESIAN_POINT('Ctrl Pts',(-6.04295127300006,15.2,8.76011974899999));
#239959=CARTESIAN_POINT('Ctrl Pts',(-6.04295127300006,11.6,8.76011974899999));
#239960=CARTESIAN_POINT('Ctrl Pts',(-6.04462455100006,15.2,8.76160596799998));
#239961=CARTESIAN_POINT('Ctrl Pts',(-6.04462455100006,11.6,8.76160596799998));
#239962=CARTESIAN_POINT('Ctrl Pts',(-6.04630407800006,15.2,8.76309509099999));
#239963=CARTESIAN_POINT('Ctrl Pts',(-6.04630407800006,11.6,8.76309509099999));
#239964=CARTESIAN_POINT('Ctrl Pts',(-6.04798985100006,15.2,8.76458709899998));
#239965=CARTESIAN_POINT('Ctrl Pts',(-6.04798985100006,11.6,8.76458709899998));
#239966=CARTESIAN_POINT('Ctrl Pts',(-6.04968186800006,15.2,8.76608197799998));
#239967=CARTESIAN_POINT('Ctrl Pts',(-6.04968186800006,11.6,8.76608197799998));
#239968=CARTESIAN_POINT('Ctrl Pts',(-6.05138012300006,15.2,8.76757970899998));
#239969=CARTESIAN_POINT('Ctrl Pts',(-6.05138012300006,11.6,8.76757970899998));
#239970=CARTESIAN_POINT('Ctrl Pts',(-6.05308461500006,15.2,8.76908027599999));
#239971=CARTESIAN_POINT('Ctrl Pts',(-6.05308461500006,11.6,8.76908027599999));
#239972=CARTESIAN_POINT('Ctrl Pts',(-6.05479534000006,15.2,8.77058366199999));
#239973=CARTESIAN_POINT('Ctrl Pts',(-6.05479534000006,11.6,8.77058366199999));
#239974=CARTESIAN_POINT('Ctrl Pts',(-6.05651229500006,15.2,8.77208985199999));
#239975=CARTESIAN_POINT('Ctrl Pts',(-6.05651229500006,11.6,8.77208985199999));
#239976=CARTESIAN_POINT('Ctrl Pts',(-6.05823547800005,15.2,8.77359882999999));
#239977=CARTESIAN_POINT('Ctrl Pts',(-6.05823547800005,11.6,8.77359882999999));
#239978=CARTESIAN_POINT('Ctrl Pts',(-6.05996488300006,15.2,8.77511057699999));
#239979=CARTESIAN_POINT('Ctrl Pts',(-6.05996488300006,11.6,8.77511057699999));
#239980=CARTESIAN_POINT('Ctrl Pts',(-6.06170050700006,15.2,8.77662507799998));
#239981=CARTESIAN_POINT('Ctrl Pts',(-6.06170050700006,11.6,8.77662507799998));
#239982=CARTESIAN_POINT('Ctrl Pts',(-6.06344234900006,15.2,8.77814231799999));
#239983=CARTESIAN_POINT('Ctrl Pts',(-6.06344234900006,11.6,8.77814231799999));
#239984=CARTESIAN_POINT('Ctrl Pts',(-6.06519040500006,15.2,8.77966227799998));
#239985=CARTESIAN_POINT('Ctrl Pts',(-6.06519040500006,11.6,8.77966227799998));
#239986=CARTESIAN_POINT('Ctrl Pts',(-6.06694467000006,15.2,8.78118494499999));
#239987=CARTESIAN_POINT('Ctrl Pts',(-6.06694467000006,11.6,8.78118494499999));
#239988=CARTESIAN_POINT('Ctrl Pts',(-6.06870514300006,15.2,8.78271030099998));
#239989=CARTESIAN_POINT('Ctrl Pts',(-6.06870514300006,11.6,8.78271030099998));
#239990=CARTESIAN_POINT('Ctrl Pts',(-6.07047181900006,15.2,8.78423833099998));
#239991=CARTESIAN_POINT('Ctrl Pts',(-6.07047181900006,11.6,8.78423833099998));
#239992=CARTESIAN_POINT('Ctrl Pts',(-6.07224469600006,15.2,8.78576901799999));
#239993=CARTESIAN_POINT('Ctrl Pts',(-6.07224469600006,11.6,8.78576901799999));
#239994=CARTESIAN_POINT('Ctrl Pts',(-6.07402377100006,15.2,8.78730234699999));
#239995=CARTESIAN_POINT('Ctrl Pts',(-6.07402377100006,11.6,8.78730234699999));
#239996=CARTESIAN_POINT('Ctrl Pts',(-6.07580903900006,15.2,8.78883829999998));
#239997=CARTESIAN_POINT('Ctrl Pts',(-6.07580903900006,11.6,8.78883829999998));
#239998=CARTESIAN_POINT('Ctrl Pts',(-6.07760049900006,15.2,8.79037686399998));
#239999=CARTESIAN_POINT('Ctrl Pts',(-6.07760049900006,11.6,8.79037686399998));
#240000=CARTESIAN_POINT('Ctrl Pts',(-6.07939814500006,15.2,8.79191802199998));
#240001=CARTESIAN_POINT('Ctrl Pts',(-6.07939814500006,11.6,8.79191802199998));
#240002=CARTESIAN_POINT('Ctrl Pts',(-6.08120197600006,15.2,8.79346175699999));
#240003=CARTESIAN_POINT('Ctrl Pts',(-6.08120197600006,11.6,8.79346175699999));
#240004=CARTESIAN_POINT('Ctrl Pts',(-6.08301198700006,15.2,8.79500805499998));
#240005=CARTESIAN_POINT('Ctrl Pts',(-6.08301198700006,11.6,8.79500805499998));
#240006=CARTESIAN_POINT('Ctrl Pts',(-6.08482817700006,15.2,8.79655689899998));
#240007=CARTESIAN_POINT('Ctrl Pts',(-6.08482817700006,11.6,8.79655689899998));
#240008=CARTESIAN_POINT('Ctrl Pts',(-6.08665054100006,15.2,8.79810827499998));
#240009=CARTESIAN_POINT('Ctrl Pts',(-6.08665054100006,11.6,8.79810827499998));
#240010=CARTESIAN_POINT('Ctrl Pts',(-6.08847907600006,15.2,8.79966216699999));
#240011=CARTESIAN_POINT('Ctrl Pts',(-6.08847907600006,11.6,8.79966216699999));
#240012=CARTESIAN_POINT('Ctrl Pts',(-6.09031377800005,15.2,8.80121855699999));
#240013=CARTESIAN_POINT('Ctrl Pts',(-6.09031377800005,11.6,8.80121855699999));
#240014=CARTESIAN_POINT('Ctrl Pts',(-6.09215464600006,15.2,8.80277743299999));
#240015=CARTESIAN_POINT('Ctrl Pts',(-6.09215464600006,11.6,8.80277743299999));
#240016=CARTESIAN_POINT('Ctrl Pts',(-6.09400167400006,15.2,8.80433877799998));
#240017=CARTESIAN_POINT('Ctrl Pts',(-6.09400167400006,11.6,8.80433877799998));
#240018=CARTESIAN_POINT('Ctrl Pts',(-6.09585486000006,15.2,8.80590257699998));
#240019=CARTESIAN_POINT('Ctrl Pts',(-6.09585486000006,11.6,8.80590257699998));
#240020=CARTESIAN_POINT('Ctrl Pts',(-6.09771420200006,15.2,8.80746881399999));
#240021=CARTESIAN_POINT('Ctrl Pts',(-6.09771420200006,11.6,8.80746881399999));
#240022=CARTESIAN_POINT('Ctrl Pts',(-6.09957969400006,15.2,8.80903747399999));
#240023=CARTESIAN_POINT('Ctrl Pts',(-6.09957969400006,11.6,8.80903747399999));
#240024=CARTESIAN_POINT('Ctrl Pts',(-6.10145133600006,15.2,8.81060854199998));
#240025=CARTESIAN_POINT('Ctrl Pts',(-6.10145133600006,11.6,8.81060854199998));
#240026=CARTESIAN_POINT('Ctrl Pts',(-6.10332912100006,15.2,8.81218200199999));
#240027=CARTESIAN_POINT('Ctrl Pts',(-6.10332912100006,11.6,8.81218200199999));
#240028=CARTESIAN_POINT('Ctrl Pts',(-6.10521304800006,15.2,8.81375783999999));
#240029=CARTESIAN_POINT('Ctrl Pts',(-6.10521304800006,11.6,8.81375783999999));
#240030=CARTESIAN_POINT('Ctrl Pts',(-6.10710311400006,15.2,8.81533604099998));
#240031=CARTESIAN_POINT('Ctrl Pts',(-6.10710311400006,11.6,8.81533604099998));
#240032=CARTESIAN_POINT('Ctrl Pts',(-6.10899931500006,15.2,8.81691658799999));
#240033=CARTESIAN_POINT('Ctrl Pts',(-6.10899931500006,11.6,8.81691658799999));
#240034=CARTESIAN_POINT('Ctrl Pts',(-6.11090164700006,15.2,8.81849946799999));
#240035=CARTESIAN_POINT('Ctrl Pts',(-6.11090164700006,11.6,8.81849946799999));
#240036=CARTESIAN_POINT('Ctrl Pts',(-6.11281010800006,15.2,8.82008466499999));
#240037=CARTESIAN_POINT('Ctrl Pts',(-6.11281010800006,11.6,8.82008466499999));
#240038=CARTESIAN_POINT('Ctrl Pts',(-6.11472469300006,15.2,8.82167216499998));
#240039=CARTESIAN_POINT('Ctrl Pts',(-6.11472469300006,11.6,8.82167216499998));
#240040=CARTESIAN_POINT('Ctrl Pts',(-6.11664540100006,15.2,8.82326195199998));
#240041=CARTESIAN_POINT('Ctrl Pts',(-6.11664540100006,11.6,8.82326195199998));
#240042=CARTESIAN_POINT('Ctrl Pts',(-6.11857222800006,15.2,8.82485401199999));
#240043=CARTESIAN_POINT('Ctrl Pts',(-6.11857222800006,11.6,8.82485401199999));
#240044=CARTESIAN_POINT('Ctrl Pts',(-6.12050516900006,15.2,8.82644832899998));
#240045=CARTESIAN_POINT('Ctrl Pts',(-6.12050516900006,11.6,8.82644832899998));
#240046=CARTESIAN_POINT('Ctrl Pts',(-6.12244422200006,15.2,8.82804488899998));
#240047=CARTESIAN_POINT('Ctrl Pts',(-6.12244422200006,11.6,8.82804488899998));
#240048=CARTESIAN_POINT('Ctrl Pts',(-6.12438938300006,15.2,8.82964367799998));
#240049=CARTESIAN_POINT('Ctrl Pts',(-6.12438938300006,11.6,8.82964367799998));
#240050=CARTESIAN_POINT('Ctrl Pts',(-6.12634065100006,15.2,8.83124467999998));
#240051=CARTESIAN_POINT('Ctrl Pts',(-6.12634065100006,11.6,8.83124467999998));
#240052=CARTESIAN_POINT('Ctrl Pts',(-6.12829802000006,15.2,8.83284788199998));
#240053=CARTESIAN_POINT('Ctrl Pts',(-6.12829802000006,11.6,8.83284788199998));
#240054=CARTESIAN_POINT('Ctrl Pts',(-6.13026148800006,15.2,8.83445326699999));
#240055=CARTESIAN_POINT('Ctrl Pts',(-6.13026148800006,11.6,8.83445326699999));
#240056=CARTESIAN_POINT('Ctrl Pts',(-6.13223105200006,15.2,8.83606082299998));
#240057=CARTESIAN_POINT('Ctrl Pts',(-6.13223105200006,11.6,8.83606082299998));
#240058=CARTESIAN_POINT('Ctrl Pts',(-6.13420670700005,15.2,8.83767053499999));
#240059=CARTESIAN_POINT('Ctrl Pts',(-6.13420670700005,11.6,8.83767053499999));
#240060=CARTESIAN_POINT('Ctrl Pts',(-6.13618845100006,15.2,8.83928238599999));
#240061=CARTESIAN_POINT('Ctrl Pts',(-6.13618845100006,11.6,8.83928238599999));
#240062=CARTESIAN_POINT('Ctrl Pts',(-6.13817628100006,15.2,8.84089636499999));
#240063=CARTESIAN_POINT('Ctrl Pts',(-6.13817628100006,11.6,8.84089636499999));
#240064=CARTESIAN_POINT('Ctrl Pts',(-6.14017019300006,15.2,8.84251245499998));
#240065=CARTESIAN_POINT('Ctrl Pts',(-6.14017019300006,11.6,8.84251245499998));
#240066=CARTESIAN_POINT('Ctrl Pts',(-6.14217018400006,15.2,8.84413064299999));
#240067=CARTESIAN_POINT('Ctrl Pts',(-6.14217018400006,11.6,8.84413064299999));
#240068=CARTESIAN_POINT('Ctrl Pts',(-6.14417625100006,15.2,8.84575091399999));
#240069=CARTESIAN_POINT('Ctrl Pts',(-6.14417625100006,11.6,8.84575091399999));
#240070=CARTESIAN_POINT('Ctrl Pts',(-6.14618838900006,15.2,8.84737325599998));
#240071=CARTESIAN_POINT('Ctrl Pts',(-6.14618838900006,11.6,8.84737325599998));
#240072=CARTESIAN_POINT('Ctrl Pts',(-6.14820659700006,15.2,8.84899765099998));
#240073=CARTESIAN_POINT('Ctrl Pts',(-6.14820659700006,11.6,8.84899765099998));
#240074=CARTESIAN_POINT('Ctrl Pts',(-6.15023087000006,15.2,8.85062408799998));
#240075=CARTESIAN_POINT('Ctrl Pts',(-6.15023087000006,11.6,8.85062408799998));
#240076=CARTESIAN_POINT('Ctrl Pts',(-6.15226120500005,15.2,8.85225255099999));
#240077=CARTESIAN_POINT('Ctrl Pts',(-6.15226120500005,11.6,8.85225255099999));
#240078=CARTESIAN_POINT('Ctrl Pts',(-6.15429760000006,15.2,8.85388302599999));
#240079=CARTESIAN_POINT('Ctrl Pts',(-6.15429760000006,11.6,8.85388302599999));
#240080=CARTESIAN_POINT('Ctrl Pts',(-6.15634005000006,15.2,8.85551550099999));
#240081=CARTESIAN_POINT('Ctrl Pts',(-6.15634005000006,11.6,8.85551550099999));
#240082=CARTESIAN_POINT('Ctrl Pts',(-6.15838855200006,15.2,8.85714995899999));
#240083=CARTESIAN_POINT('Ctrl Pts',(-6.15838855200006,11.6,8.85714995899999));
#240084=CARTESIAN_POINT('Ctrl Pts',(-6.16044310400006,15.2,8.85878638799999));
#240085=CARTESIAN_POINT('Ctrl Pts',(-6.16044310400006,11.6,8.85878638799999));
#240086=CARTESIAN_POINT('Ctrl Pts',(-6.16250370100006,15.2,8.86042477299998));
#240087=CARTESIAN_POINT('Ctrl Pts',(-6.16250370100006,11.6,8.86042477299998));
#240088=CARTESIAN_POINT('Ctrl Pts',(-6.16457034000006,15.2,8.86206510199998));
#240089=CARTESIAN_POINT('Ctrl Pts',(-6.16457034000006,11.6,8.86206510199998));
#240090=CARTESIAN_POINT('Ctrl Pts',(-6.16664301800006,15.2,8.86370735799998));
#240091=CARTESIAN_POINT('Ctrl Pts',(-6.16664301800006,11.6,8.86370735799998));
#240092=CARTESIAN_POINT('Ctrl Pts',(-6.16872173200006,15.2,8.86535152999999));
#240093=CARTESIAN_POINT('Ctrl Pts',(-6.16872173200006,11.6,8.86535152999999));
#240094=CARTESIAN_POINT('Ctrl Pts',(-6.17080647900006,15.2,8.86699760299998));
#240095=CARTESIAN_POINT('Ctrl Pts',(-6.17080647900006,11.6,8.86699760299998));
#240096=CARTESIAN_POINT('Ctrl Pts',(-6.17289725400005,15.2,8.86864556399999));
#240097=CARTESIAN_POINT('Ctrl Pts',(-6.17289725400005,11.6,8.86864556399999));
#240098=CARTESIAN_POINT('Ctrl Pts',(-6.17499405600006,15.2,8.87029539799999));
#240099=CARTESIAN_POINT('Ctrl Pts',(-6.17499405600006,11.6,8.87029539799999));
#240100=CARTESIAN_POINT('Ctrl Pts',(-6.17709687900006,15.2,8.87194709099998));
#240101=CARTESIAN_POINT('Ctrl Pts',(-6.17709687900006,11.6,8.87194709099998));
#240102=CARTESIAN_POINT('Ctrl Pts',(-6.17920572100005,15.2,8.87360063199999));
#240103=CARTESIAN_POINT('Ctrl Pts',(-6.17920572100005,11.6,8.87360063199999));
#240104=CARTESIAN_POINT('Ctrl Pts',(-6.18132057900006,15.2,8.87525600499998));
#240105=CARTESIAN_POINT('Ctrl Pts',(-6.18132057900006,11.6,8.87525600499998));
#240106=CARTESIAN_POINT('Ctrl Pts',(-6.18344144900006,15.2,8.87691319699999));
#240107=CARTESIAN_POINT('Ctrl Pts',(-6.18344144900006,11.6,8.87691319699999));
#240108=CARTESIAN_POINT('Ctrl Pts',(-6.18556832800006,15.2,8.87857219399999));
#240109=CARTESIAN_POINT('Ctrl Pts',(-6.18556832800006,11.6,8.87857219399999));
#240110=CARTESIAN_POINT('Ctrl Pts',(-6.18770121400006,15.2,8.88023298499999));
#240111=CARTESIAN_POINT('Ctrl Pts',(-6.18770121400006,11.6,8.88023298499999));
#240112=CARTESIAN_POINT('Ctrl Pts',(-6.18984010100006,15.2,8.88189555299999));
#240113=CARTESIAN_POINT('Ctrl Pts',(-6.18984010100006,11.6,8.88189555299999));
#240114=CARTESIAN_POINT('Ctrl Pts',(-6.19198498800006,15.2,8.88355988699999));
#240115=CARTESIAN_POINT('Ctrl Pts',(-6.19198498800006,11.6,8.88355988699999));
#240116=CARTESIAN_POINT('Ctrl Pts',(-6.19413587000006,15.2,8.88522597299998));
#240117=CARTESIAN_POINT('Ctrl Pts',(-6.19413587000006,11.6,8.88522597299998));
#240118=CARTESIAN_POINT('Ctrl Pts',(-6.19629274400006,15.2,8.88689379699999));
#240119=CARTESIAN_POINT('Ctrl Pts',(-6.19629274400006,11.6,8.88689379699999));
#240120=CARTESIAN_POINT('Ctrl Pts',(-6.19845560700006,15.2,8.88856334699998));
#240121=CARTESIAN_POINT('Ctrl Pts',(-6.19845560700006,11.6,8.88856334699998));
#240122=CARTESIAN_POINT('Ctrl Pts',(-6.20062445500006,15.2,8.89023460999999));
#240123=CARTESIAN_POINT('Ctrl Pts',(-6.20062445500006,11.6,8.89023460999999));
#240124=CARTESIAN_POINT('Ctrl Pts',(-6.20279928600006,15.2,8.89190756899998));
#240125=CARTESIAN_POINT('Ctrl Pts',(-6.20279928600006,11.6,8.89190756899998));
#240126=CARTESIAN_POINT('Ctrl Pts',(-6.20498009600006,15.2,8.89358221499998));
#240127=CARTESIAN_POINT('Ctrl Pts',(-6.20498009600006,11.6,8.89358221499998));
#240128=CARTESIAN_POINT('Ctrl Pts',(-6.20716688100006,15.2,8.89525853399999));
#240129=CARTESIAN_POINT('Ctrl Pts',(-6.20716688100006,11.6,8.89525853399999));
#240130=CARTESIAN_POINT('Ctrl Pts',(-6.20935963800005,15.2,8.89693651099999));
#240131=CARTESIAN_POINT('Ctrl Pts',(-6.20935963800005,11.6,8.89693651099999));
#240132=CARTESIAN_POINT('Ctrl Pts',(-6.21155836400006,15.2,8.89861613499999));
#240133=CARTESIAN_POINT('Ctrl Pts',(-6.21155836400006,11.6,8.89861613499999));
#240134=CARTESIAN_POINT('Ctrl Pts',(-6.21376305600006,15.2,8.90029739199999));
#240135=CARTESIAN_POINT('Ctrl Pts',(-6.21376305600006,11.6,8.90029739199999));
#240136=CARTESIAN_POINT('Ctrl Pts',(-6.21597370900006,15.2,8.90198026899998));
#240137=CARTESIAN_POINT('Ctrl Pts',(-6.21597370900006,11.6,8.90198026899998));
#240138=CARTESIAN_POINT('Ctrl Pts',(-6.21819032200006,15.2,8.90366475299999));
#240139=CARTESIAN_POINT('Ctrl Pts',(-6.21819032200006,11.6,8.90366475299999));
#240140=CARTESIAN_POINT('Ctrl Pts',(-6.22041289000006,15.2,8.90535083099999));
#240141=CARTESIAN_POINT('Ctrl Pts',(-6.22041289000006,11.6,8.90535083099999));
#240142=CARTESIAN_POINT('Ctrl Pts',(-6.22264140900006,15.2,8.90703849099998));
#240143=CARTESIAN_POINT('Ctrl Pts',(-6.22264140900006,11.6,8.90703849099998));
#240144=CARTESIAN_POINT('Ctrl Pts',(-6.22487587700006,15.2,8.90872771899998));
#240145=CARTESIAN_POINT('Ctrl Pts',(-6.22487587700006,11.6,8.90872771899998));
#240146=CARTESIAN_POINT('Ctrl Pts',(-6.22711629100006,15.2,8.91041850199999));
#240147=CARTESIAN_POINT('Ctrl Pts',(-6.22711629100006,11.6,8.91041850199999));
#240148=CARTESIAN_POINT('Ctrl Pts',(-6.22936264600006,15.2,8.91211082799998));
#240149=CARTESIAN_POINT('Ctrl Pts',(-6.22936264600006,11.6,8.91211082799998));
#240150=CARTESIAN_POINT('Ctrl Pts',(-6.23161494000006,15.2,8.91380468399999));
#240151=CARTESIAN_POINT('Ctrl Pts',(-6.23161494000006,11.6,8.91380468399999));
#240152=CARTESIAN_POINT('Ctrl Pts',(-6.23387316900006,15.2,8.91550005599999));
#240153=CARTESIAN_POINT('Ctrl Pts',(-6.23387316900006,11.6,8.91550005599999));
#240154=CARTESIAN_POINT('Ctrl Pts',(-6.23613733000006,15.2,8.91719693299999));
#240155=CARTESIAN_POINT('Ctrl Pts',(-6.23613733000006,11.6,8.91719693299999));
#240156=CARTESIAN_POINT('Ctrl Pts',(-6.23840741900006,15.2,8.91889530199999));
#240157=CARTESIAN_POINT('Ctrl Pts',(-6.23840741900006,11.6,8.91889530199999));
#240158=CARTESIAN_POINT('Ctrl Pts',(-6.24068343300006,15.2,8.92059515099999));
#240159=CARTESIAN_POINT('Ctrl Pts',(-6.24068343300006,11.6,8.92059515099999));
#240160=CARTESIAN_POINT('Ctrl Pts',(-6.24296537000006,15.2,8.92229646399999));
#240161=CARTESIAN_POINT('Ctrl Pts',(-6.24296537000006,11.6,8.92229646399999));
#240162=CARTESIAN_POINT('Ctrl Pts',(-6.24525322300006,15.2,8.92399923299998));
#240163=CARTESIAN_POINT('Ctrl Pts',(-6.24525322300006,11.6,8.92399923299998));
#240164=CARTESIAN_POINT('Ctrl Pts',(-6.24754699300006,15.2,8.92570344299998));
#240165=CARTESIAN_POINT('Ctrl Pts',(-6.24754699300006,11.6,8.92570344299998));
#240166=CARTESIAN_POINT('Ctrl Pts',(-6.24984667300006,15.2,8.92740908099999));
#240167=CARTESIAN_POINT('Ctrl Pts',(-6.24984667300006,11.6,8.92740908099999));
#240168=CARTESIAN_POINT('Ctrl Pts',(-6.25215226200006,15.2,8.92911613599999));
#240169=CARTESIAN_POINT('Ctrl Pts',(-6.25215226200006,11.6,8.92911613599999));
#240170=CARTESIAN_POINT('Ctrl Pts',(-6.25446375500006,15.2,8.93082459399999));
#240171=CARTESIAN_POINT('Ctrl Pts',(-6.25446375500006,11.6,8.93082459399999));
#240172=CARTESIAN_POINT('Ctrl Pts',(-6.25678115000006,15.2,8.93253444399999));
#240173=CARTESIAN_POINT('Ctrl Pts',(-6.25678115000006,11.6,8.93253444399999));
#240174=CARTESIAN_POINT('Ctrl Pts',(-6.25910444300006,15.2,8.93424567299999));
#240175=CARTESIAN_POINT('Ctrl Pts',(-6.25910444300006,11.6,8.93424567299999));
#240176=CARTESIAN_POINT('Ctrl Pts',(-6.26143363000006,15.2,8.93595826899999));
#240177=CARTESIAN_POINT('Ctrl Pts',(-6.26143363000006,11.6,8.93595826899999));
#240178=CARTESIAN_POINT('Ctrl Pts',(-6.26376870900006,15.2,8.93767221899999));
#240179=CARTESIAN_POINT('Ctrl Pts',(-6.26376870900006,11.6,8.93767221899999));
#240180=CARTESIAN_POINT('Ctrl Pts',(-6.26610967500006,15.2,8.93938750999999));
#240181=CARTESIAN_POINT('Ctrl Pts',(-6.26610967500006,11.6,8.93938750999999));
#240182=CARTESIAN_POINT('Ctrl Pts',(-6.26845652500006,15.2,8.94110413199999));
#240183=CARTESIAN_POINT('Ctrl Pts',(-6.26845652500006,11.6,8.94110413199999));
#240184=CARTESIAN_POINT('Ctrl Pts',(-6.27080925800006,15.2,8.94282207099998));
#240185=CARTESIAN_POINT('Ctrl Pts',(-6.27080925800006,11.6,8.94282207099998));
#240186=CARTESIAN_POINT('Ctrl Pts',(-6.27316786700006,15.2,8.94454131499998));
#240187=CARTESIAN_POINT('Ctrl Pts',(-6.27316786700006,11.6,8.94454131499998));
#240188=CARTESIAN_POINT('Ctrl Pts',(-6.27553235100006,15.2,8.94626185399999));
#240189=CARTESIAN_POINT('Ctrl Pts',(-6.27553235100006,11.6,8.94626185399999));
#240190=CARTESIAN_POINT('Ctrl Pts',(-6.27790270500006,15.2,8.94798367199999));
#240191=CARTESIAN_POINT('Ctrl Pts',(-6.27790270500006,11.6,8.94798367199999));
#240192=CARTESIAN_POINT('Ctrl Pts',(-6.28027892800006,15.2,8.94970675999998));
#240193=CARTESIAN_POINT('Ctrl Pts',(-6.28027892800006,11.6,8.94970675999998));
#240194=CARTESIAN_POINT('Ctrl Pts',(-6.28266101400006,15.2,8.95143110399999));
#240195=CARTESIAN_POINT('Ctrl Pts',(-6.28266101400006,11.6,8.95143110399999));
#240196=CARTESIAN_POINT('Ctrl Pts',(-6.28504896100006,15.2,8.95315669399999));
#240197=CARTESIAN_POINT('Ctrl Pts',(-6.28504896100006,11.6,8.95315669399999));
#240198=CARTESIAN_POINT('Ctrl Pts',(-6.28744276500006,15.2,8.95488351599998));
#240199=CARTESIAN_POINT('Ctrl Pts',(-6.28744276500006,11.6,8.95488351599998));
#240200=CARTESIAN_POINT('Ctrl Pts',(-6.28984242200006,15.2,8.95661155799999));
#240201=CARTESIAN_POINT('Ctrl Pts',(-6.28984242200006,11.6,8.95661155799999));
#240202=CARTESIAN_POINT('Ctrl Pts',(-6.29224793100006,15.2,8.95834080999999));
#240203=CARTESIAN_POINT('Ctrl Pts',(-6.29224793100006,11.6,8.95834080999999));
#240204=CARTESIAN_POINT('Ctrl Pts',(-6.29465928600006,15.2,8.96007125899999));
#240205=CARTESIAN_POINT('Ctrl Pts',(-6.29465928600006,11.6,8.96007125899999));
#240206=CARTESIAN_POINT('Ctrl Pts',(-6.29707648500006,15.2,8.96180289199999));
#240207=CARTESIAN_POINT('Ctrl Pts',(-6.29707648500006,11.6,8.96180289199999));
#240208=CARTESIAN_POINT('Ctrl Pts',(-6.29949952400006,15.2,8.96353569899999));
#240209=CARTESIAN_POINT('Ctrl Pts',(-6.29949952400006,11.6,8.96353569899999));
#240210=CARTESIAN_POINT('Ctrl Pts',(-6.30192840000006,15.2,8.96526966599998));
#240211=CARTESIAN_POINT('Ctrl Pts',(-6.30192840000006,11.6,8.96526966599998));
#240212=CARTESIAN_POINT('Ctrl Pts',(-6.30436311000006,15.2,8.96700478399998));
#240213=CARTESIAN_POINT('Ctrl Pts',(-6.30436311000006,11.6,8.96700478399998));
#240214=CARTESIAN_POINT('Ctrl Pts',(-6.30680365000006,15.2,8.96874103899999));
#240215=CARTESIAN_POINT('Ctrl Pts',(-6.30680365000006,11.6,8.96874103899999));
#240216=CARTESIAN_POINT('Ctrl Pts',(-6.30925001600006,15.2,8.97047841899998));
#240217=CARTESIAN_POINT('Ctrl Pts',(-6.30925001600006,11.6,8.97047841899998));
#240218=CARTESIAN_POINT('Ctrl Pts',(-6.31170220500006,15.2,8.97221691499999));
#240219=CARTESIAN_POINT('Ctrl Pts',(-6.31170220500006,11.6,8.97221691499999));
#240220=CARTESIAN_POINT('Ctrl Pts',(-6.31416021400006,15.2,8.97395651199999));
#240221=CARTESIAN_POINT('Ctrl Pts',(-6.31416021400006,11.6,8.97395651199999));
#240222=CARTESIAN_POINT('Ctrl Pts',(-6.31662403900005,15.2,8.97569720099998));
#240223=CARTESIAN_POINT('Ctrl Pts',(-6.31662403900005,11.6,8.97569720099998));
#240224=CARTESIAN_POINT('Ctrl Pts',(-6.31909367800006,15.2,8.97743896899998));
#240225=CARTESIAN_POINT('Ctrl Pts',(-6.31909367800006,11.6,8.97743896899998));
#240226=CARTESIAN_POINT('Ctrl Pts',(-6.32156912600006,15.2,8.97918180399999));
#240227=CARTESIAN_POINT('Ctrl Pts',(-6.32156912600006,11.6,8.97918180399999));
#240228=CARTESIAN_POINT('Ctrl Pts',(-6.32405038000006,15.2,8.98092569599999));
#240229=CARTESIAN_POINT('Ctrl Pts',(-6.32405038000006,11.6,8.98092569599999));
#240230=CARTESIAN_POINT('Ctrl Pts',(-6.32653743600006,15.2,8.98267063199999));
#240231=CARTESIAN_POINT('Ctrl Pts',(-6.32653743600006,11.6,8.98267063199999));
#240232=CARTESIAN_POINT('Ctrl Pts',(-6.32903029200006,15.2,8.98441660099999));
#240233=CARTESIAN_POINT('Ctrl Pts',(-6.32903029200006,11.6,8.98441660099999));
#240234=CARTESIAN_POINT('Ctrl Pts',(-6.33152894400006,15.2,8.98616359099999));
#240235=CARTESIAN_POINT('Ctrl Pts',(-6.33152894400006,11.6,8.98616359099999));
#240236=CARTESIAN_POINT('Ctrl Pts',(-6.33403338800006,15.2,8.98791159199998));
#240237=CARTESIAN_POINT('Ctrl Pts',(-6.33403338800006,11.6,8.98791159199998));
#240238=CARTESIAN_POINT('Ctrl Pts',(-6.33654362200006,15.2,8.98966058999999));
#240239=CARTESIAN_POINT('Ctrl Pts',(-6.33654362200006,11.6,8.98966058999999));
#240240=CARTESIAN_POINT('Ctrl Pts',(-6.33905964000006,15.2,8.99141057699998));
#240241=CARTESIAN_POINT('Ctrl Pts',(-6.33905964000006,11.6,8.99141057699998));
#240242=CARTESIAN_POINT('Ctrl Pts',(-6.34158144100006,15.2,8.99316153799998));
#240243=CARTESIAN_POINT('Ctrl Pts',(-6.34158144100006,11.6,8.99316153799998));
#240244=CARTESIAN_POINT('Ctrl Pts',(-6.34410902100006,15.2,8.99491346499998));
#240245=CARTESIAN_POINT('Ctrl Pts',(-6.34410902100006,11.6,8.99491346499998));
#240246=CARTESIAN_POINT('Ctrl Pts',(-6.34664237500006,15.2,8.99666634499999));
#240247=CARTESIAN_POINT('Ctrl Pts',(-6.34664237500006,11.6,8.99666634499999));
#240248=CARTESIAN_POINT('Ctrl Pts',(-6.34918150200006,15.2,8.99842016499999));
#240249=CARTESIAN_POINT('Ctrl Pts',(-6.34918150200006,11.6,8.99842016499999));
#240250=CARTESIAN_POINT('Ctrl Pts',(-6.35172639700006,15.2,9.00017491799998));
#240251=CARTESIAN_POINT('Ctrl Pts',(-6.35172639700006,11.6,9.00017491799998));
#240252=CARTESIAN_POINT('Ctrl Pts',(-6.35427705800006,15.2,9.00193058899998));
#240253=CARTESIAN_POINT('Ctrl Pts',(-6.35427705800006,11.6,9.00193058899998));
#240254=CARTESIAN_POINT('Ctrl Pts',(-6.35683347900006,15.2,9.00368716799999));
#240255=CARTESIAN_POINT('Ctrl Pts',(-6.35683347900006,11.6,9.00368716799999));
#240256=CARTESIAN_POINT('Ctrl Pts',(-6.35939565800006,15.2,9.00544464399999));
#240257=CARTESIAN_POINT('Ctrl Pts',(-6.35939565800006,11.6,9.00544464399999));
#240258=CARTESIAN_POINT('Ctrl Pts',(-6.36196359200006,15.2,9.00720300599998));
#240259=CARTESIAN_POINT('Ctrl Pts',(-6.36196359200006,11.6,9.00720300599998));
#240260=CARTESIAN_POINT('Ctrl Pts',(-6.36453727800006,15.2,9.00896224299998));
#240261=CARTESIAN_POINT('Ctrl Pts',(-6.36453727800006,11.6,9.00896224299998));
#240262=CARTESIAN_POINT('Ctrl Pts',(-6.36711671100006,15.2,9.01072234299999));
#240263=CARTESIAN_POINT('Ctrl Pts',(-6.36711671100006,11.6,9.01072234299999));
#240264=CARTESIAN_POINT('Ctrl Pts',(-6.36970188900006,15.2,9.01248329499998));
#240265=CARTESIAN_POINT('Ctrl Pts',(-6.36970188900006,11.6,9.01248329499998));
#240266=CARTESIAN_POINT('Ctrl Pts',(-6.37229280700006,15.2,9.01424508899999));
#240267=CARTESIAN_POINT('Ctrl Pts',(-6.37229280700006,11.6,9.01424508899999));
#240268=CARTESIAN_POINT('Ctrl Pts',(-6.37488946300006,15.2,9.01600771299999));
#240269=CARTESIAN_POINT('Ctrl Pts',(-6.37488946300006,11.6,9.01600771299999));
#240270=CARTESIAN_POINT('Ctrl Pts',(-6.37749185300006,15.2,9.01777115699998));
#240271=CARTESIAN_POINT('Ctrl Pts',(-6.37749185300006,11.6,9.01777115699998));
#240272=CARTESIAN_POINT('Ctrl Pts',(-6.38009997400006,15.2,9.01953540799998));
#240273=CARTESIAN_POINT('Ctrl Pts',(-6.38009997400006,11.6,9.01953540799998));
#240274=CARTESIAN_POINT('Ctrl Pts',(-6.38271382100006,15.2,9.02130045699998));
#240275=CARTESIAN_POINT('Ctrl Pts',(-6.38271382100006,11.6,9.02130045699998));
#240276=CARTESIAN_POINT('Ctrl Pts',(-6.38533339300006,15.2,9.02306629299999));
#240277=CARTESIAN_POINT('Ctrl Pts',(-6.38533339300006,11.6,9.02306629299999));
#240278=CARTESIAN_POINT('Ctrl Pts',(-6.38795868400006,15.2,9.02483290399999));
#240279=CARTESIAN_POINT('Ctrl Pts',(-6.38795868400006,11.6,9.02483290399999));
#240280=CARTESIAN_POINT('Ctrl Pts',(-6.39058969200006,15.2,9.02660027899999));
#240281=CARTESIAN_POINT('Ctrl Pts',(-6.39058969200006,11.6,9.02660027899999));
#240282=CARTESIAN_POINT('Ctrl Pts',(-6.39322641400006,15.2,9.02836840899998));
#240283=CARTESIAN_POINT('Ctrl Pts',(-6.39322641400006,11.6,9.02836840899998));
#240284=CARTESIAN_POINT('Ctrl Pts',(-6.39586884500006,15.2,9.03013728199999));
#240285=CARTESIAN_POINT('Ctrl Pts',(-6.39586884500006,11.6,9.03013728199999));
#240286=CARTESIAN_POINT('Ctrl Pts',(-6.39851698300006,15.2,9.03190688599998));
#240287=CARTESIAN_POINT('Ctrl Pts',(-6.39851698300006,11.6,9.03190688599998));
#240288=CARTESIAN_POINT('Ctrl Pts',(-6.40117082500006,15.2,9.03367721299999));
#240289=CARTESIAN_POINT('Ctrl Pts',(-6.40117082500006,11.6,9.03367721299999));
#240290=CARTESIAN_POINT('Ctrl Pts',(-6.40383036500006,15.2,9.03544824899999));
#240291=CARTESIAN_POINT('Ctrl Pts',(-6.40383036500006,11.6,9.03544824899999));
#240292=CARTESIAN_POINT('Ctrl Pts',(-6.40649560100006,15.2,9.03721998699999));
#240293=CARTESIAN_POINT('Ctrl Pts',(-6.40649560100006,11.6,9.03721998699999));
#240294=CARTESIAN_POINT('Ctrl Pts',(-6.40916652900006,15.2,9.03899241299998));
#240295=CARTESIAN_POINT('Ctrl Pts',(-6.40916652900006,11.6,9.03899241299998));
#240296=CARTESIAN_POINT('Ctrl Pts',(-6.41184314700006,15.2,9.04076551799999));
#240297=CARTESIAN_POINT('Ctrl Pts',(-6.41184314700006,11.6,9.04076551799999));
#240298=CARTESIAN_POINT('Ctrl Pts',(-6.41452545100006,15.2,9.04253928999999));
#240299=CARTESIAN_POINT('Ctrl Pts',(-6.41452545100006,11.6,9.04253928999999));
#240300=CARTESIAN_POINT('Ctrl Pts',(-6.41721343700006,15.2,9.04431372099998));
#240301=CARTESIAN_POINT('Ctrl Pts',(-6.41721343700006,11.6,9.04431372099998));
#240302=CARTESIAN_POINT('Ctrl Pts',(-6.41990710100006,15.2,9.04608879799999));
#240303=CARTESIAN_POINT('Ctrl Pts',(-6.41990710100006,11.6,9.04608879799999));
#240304=CARTESIAN_POINT('Ctrl Pts',(-6.42260644100006,15.2,9.04786451099999));
#240305=CARTESIAN_POINT('Ctrl Pts',(-6.42260644100006,11.6,9.04786451099999));
#240306=CARTESIAN_POINT('Ctrl Pts',(-6.42531145200006,15.2,9.04964084999998));
#240307=CARTESIAN_POINT('Ctrl Pts',(-6.42531145200006,11.6,9.04964084999998));
#240308=CARTESIAN_POINT('Ctrl Pts',(-6.42802213200006,15.2,9.05141780399998));
#240309=CARTESIAN_POINT('Ctrl Pts',(-6.42802213200006,11.6,9.05141780399998));
#240310=CARTESIAN_POINT('Ctrl Pts',(-6.43073847600006,15.2,9.05319536199999));
#240311=CARTESIAN_POINT('Ctrl Pts',(-6.43073847600006,11.6,9.05319536199999));
#240312=CARTESIAN_POINT('Ctrl Pts',(-6.43346048200006,15.2,9.05497351499999));
#240313=CARTESIAN_POINT('Ctrl Pts',(-6.43346048200006,11.6,9.05497351499999));
#240314=CARTESIAN_POINT('Ctrl Pts',(-6.43618814600006,15.2,9.05675225099999));
#240315=CARTESIAN_POINT('Ctrl Pts',(-6.43618814600006,11.6,9.05675225099999));
#240316=CARTESIAN_POINT('Ctrl Pts',(-6.43892146400006,15.2,9.05853155999999));
#240317=CARTESIAN_POINT('Ctrl Pts',(-6.43892146400006,11.6,9.05853155999999));
#240318=CARTESIAN_POINT('Ctrl Pts',(-6.44166043400006,15.2,9.06031143299998));
#240319=CARTESIAN_POINT('Ctrl Pts',(-6.44166043400006,11.6,9.06031143299998));
#240320=CARTESIAN_POINT('Ctrl Pts',(-6.44440505000006,15.2,9.06209185799998));
#240321=CARTESIAN_POINT('Ctrl Pts',(-6.44440505000006,11.6,9.06209185799998));
#240322=CARTESIAN_POINT('Ctrl Pts',(-6.44715531200006,15.2,9.06387282399999));
#240323=CARTESIAN_POINT('Ctrl Pts',(-6.44715531200006,11.6,9.06387282399999));
#240324=CARTESIAN_POINT('Ctrl Pts',(-6.44991121200006,15.2,9.06565432299999));
#240325=CARTESIAN_POINT('Ctrl Pts',(-6.44991121200006,11.6,9.06565432299999));
#240326=CARTESIAN_POINT('Ctrl Pts',(-6.45267275100006,15.2,9.06743634299998));
#240327=CARTESIAN_POINT('Ctrl Pts',(-6.45267275100006,11.6,9.06743634299998));
#240328=CARTESIAN_POINT('Ctrl Pts',(-6.45543992300006,15.2,9.06921887599999));
#240329=CARTESIAN_POINT('Ctrl Pts',(-6.45543992300006,11.6,9.06921887599999));
#240330=CARTESIAN_POINT('Ctrl Pts',(-6.45821272400006,15.2,9.07100190799999));
#240331=CARTESIAN_POINT('Ctrl Pts',(-6.45821272400006,11.6,9.07100190799999));
#240332=CARTESIAN_POINT('Ctrl Pts',(-6.46099115300006,15.2,9.07278543099999));
#240333=CARTESIAN_POINT('Ctrl Pts',(-6.46099115300006,11.6,9.07278543099999));
#240334=CARTESIAN_POINT('Ctrl Pts',(-6.46377520500006,15.2,9.07456943399998));
#240335=CARTESIAN_POINT('Ctrl Pts',(-6.46377520500006,11.6,9.07456943399998));
#240336=CARTESIAN_POINT('Ctrl Pts',(-6.46656487700006,15.2,9.07635390799998));
#240337=CARTESIAN_POINT('Ctrl Pts',(-6.46656487700006,11.6,9.07635390799998));
#240338=CARTESIAN_POINT('Ctrl Pts',(-6.46936016400006,15.2,9.07813884199999));
#240339=CARTESIAN_POINT('Ctrl Pts',(-6.46936016400006,11.6,9.07813884199999));
#240340=CARTESIAN_POINT('Ctrl Pts',(-6.47216106400006,15.2,9.07992422599998));
#240341=CARTESIAN_POINT('Ctrl Pts',(-6.47216106400006,11.6,9.07992422599998));
#240342=CARTESIAN_POINT('Ctrl Pts',(-6.47496757400006,15.2,9.08171004999998));
#240343=CARTESIAN_POINT('Ctrl Pts',(-6.47496757400006,11.6,9.08171004999998));
#240344=CARTESIAN_POINT('Ctrl Pts',(-6.47777968900006,15.2,9.08349630299998));
#240345=CARTESIAN_POINT('Ctrl Pts',(-6.47777968900006,11.6,9.08349630299998));
#240346=CARTESIAN_POINT('Ctrl Pts',(-6.48059740600006,15.2,9.08528297699998));
#240347=CARTESIAN_POINT('Ctrl Pts',(-6.48059740600006,11.6,9.08528297699998));
#240348=CARTESIAN_POINT('Ctrl Pts',(-6.48342072100006,15.2,9.08707005899998));
#240349=CARTESIAN_POINT('Ctrl Pts',(-6.48342072100006,11.6,9.08707005899998));
#240350=CARTESIAN_POINT('Ctrl Pts',(-6.48624963200006,15.2,9.08885754199999));
#240351=CARTESIAN_POINT('Ctrl Pts',(-6.48624963200006,11.6,9.08885754199999));
#240352=CARTESIAN_POINT('Ctrl Pts',(-6.48908413600005,15.2,9.09064541299998));
#240353=CARTESIAN_POINT('Ctrl Pts',(-6.48908413600005,11.6,9.09064541299998));
#240354=CARTESIAN_POINT('Ctrl Pts',(-6.49192422700006,15.2,9.09243366499998));
#240355=CARTESIAN_POINT('Ctrl Pts',(-6.49192422700006,11.6,9.09243366499998));
#240356=CARTESIAN_POINT('Ctrl Pts',(-6.49476990200006,15.2,9.09422228699999));
#240357=CARTESIAN_POINT('Ctrl Pts',(-6.49476990200006,11.6,9.09422228699999));
#240358=CARTESIAN_POINT('Ctrl Pts',(-6.49762116000006,15.2,9.09601126699998));
#240359=CARTESIAN_POINT('Ctrl Pts',(-6.49762116000006,11.6,9.09601126699998));
#240360=CARTESIAN_POINT('Ctrl Pts',(-6.50047799400006,15.2,9.09780059799999));
#240361=CARTESIAN_POINT('Ctrl Pts',(-6.50047799400006,11.6,9.09780059799999));
#240362=CARTESIAN_POINT('Ctrl Pts',(-6.50334040400006,15.2,9.09959026799999));
#240363=CARTESIAN_POINT('Ctrl Pts',(-6.50334040400006,11.6,9.09959026799999));
#240364=CARTESIAN_POINT('Ctrl Pts',(-6.50620838300005,15.2,9.10138026899999));
#240365=CARTESIAN_POINT('Ctrl Pts',(-6.50620838300005,11.6,9.10138026899999));
#240366=CARTESIAN_POINT('Ctrl Pts',(-6.50908193000006,15.2,9.10317059099999));
#240367=CARTESIAN_POINT('Ctrl Pts',(-6.50908193000006,11.6,9.10317059099999));
#240368=CARTESIAN_POINT('Ctrl Pts',(-6.51196104100006,15.2,9.10496122099998));
#240369=CARTESIAN_POINT('Ctrl Pts',(-6.51196104100006,11.6,9.10496122099998));
#240370=CARTESIAN_POINT('Ctrl Pts',(-6.51484571200006,15.2,9.10675215299998));
#240371=CARTESIAN_POINT('Ctrl Pts',(-6.51484571200006,11.6,9.10675215299998));
#240372=CARTESIAN_POINT('Ctrl Pts',(-6.51773593900006,15.2,9.10854337499998));
#240373=CARTESIAN_POINT('Ctrl Pts',(-6.51773593900006,11.6,9.10854337499998));
#240374=CARTESIAN_POINT('Ctrl Pts',(-6.52063172100006,15.2,9.11033487799998));
#240375=CARTESIAN_POINT('Ctrl Pts',(-6.52063172100006,11.6,9.11033487799998));
#240376=CARTESIAN_POINT('Ctrl Pts',(-6.52353305100006,15.2,9.11212665299999));
#240377=CARTESIAN_POINT('Ctrl Pts',(-6.52353305100006,11.6,9.11212665299999));
#240378=CARTESIAN_POINT('Ctrl Pts',(-6.52643992800006,15.2,9.11391868799999));
#240379=CARTESIAN_POINT('Ctrl Pts',(-6.52643992800006,11.6,9.11391868799999));
#240380=CARTESIAN_POINT('Ctrl Pts',(-6.52935234800006,15.2,9.11571097599998));
#240381=CARTESIAN_POINT('Ctrl Pts',(-6.52935234800006,11.6,9.11571097599998));
#240382=CARTESIAN_POINT('Ctrl Pts',(-6.53227030700006,15.2,9.11750350599998));
#240383=CARTESIAN_POINT('Ctrl Pts',(-6.53227030700006,11.6,9.11750350599998));
#240384=CARTESIAN_POINT('Ctrl Pts',(-6.53519380100006,15.2,9.11929626799999));
#240385=CARTESIAN_POINT('Ctrl Pts',(-6.53519380100006,11.6,9.11929626799999));
#240386=CARTESIAN_POINT('Ctrl Pts',(-6.53812282700006,15.2,9.12108925299999));
#240387=CARTESIAN_POINT('Ctrl Pts',(-6.53812282700006,11.6,9.12108925299999));
#240388=CARTESIAN_POINT('Ctrl Pts',(-6.54105738300006,15.2,9.12288245099998));
#240389=CARTESIAN_POINT('Ctrl Pts',(-6.54105738300006,11.6,9.12288245099998));
#240390=CARTESIAN_POINT('Ctrl Pts',(-6.54399746300006,15.2,9.12467585299999));
#240391=CARTESIAN_POINT('Ctrl Pts',(-6.54399746300006,11.6,9.12467585299999));
#240392=CARTESIAN_POINT('Ctrl Pts',(-6.54694306500006,15.2,9.12646944899999));
#240393=CARTESIAN_POINT('Ctrl Pts',(-6.54694306500006,11.6,9.12646944899999));
#240394=CARTESIAN_POINT('Ctrl Pts',(-6.54989418600006,15.2,9.12826322899999));
#240395=CARTESIAN_POINT('Ctrl Pts',(-6.54989418600006,11.6,9.12826322899999));
#240396=CARTESIAN_POINT('Ctrl Pts',(-6.55285082000006,15.2,9.13005718499999));
#240397=CARTESIAN_POINT('Ctrl Pts',(-6.55285082000006,11.6,9.13005718499999));
#240398=CARTESIAN_POINT('Ctrl Pts',(-6.55581296600006,15.2,9.13185130499999));
#240399=CARTESIAN_POINT('Ctrl Pts',(-6.55581296600006,11.6,9.13185130499999));
#240400=CARTESIAN_POINT('Ctrl Pts',(-6.55878061900006,15.2,9.13364558199999));
#240401=CARTESIAN_POINT('Ctrl Pts',(-6.55878061900006,11.6,9.13364558199999));
#240402=CARTESIAN_POINT('Ctrl Pts',(-6.56175377600006,15.2,9.13544000499999));
#240403=CARTESIAN_POINT('Ctrl Pts',(-6.56175377600006,11.6,9.13544000499999));
#240404=CARTESIAN_POINT('Ctrl Pts',(-6.56473243500006,15.2,9.13723456399998));
#240405=CARTESIAN_POINT('Ctrl Pts',(-6.56473243500006,11.6,9.13723456399998));
#240406=CARTESIAN_POINT('Ctrl Pts',(-6.56771659000006,15.2,9.13902925199999));
#240407=CARTESIAN_POINT('Ctrl Pts',(-6.56771659000006,11.6,9.13902925199999));
#240408=CARTESIAN_POINT('Ctrl Pts',(-6.57070623700006,15.2,9.14082405799999));
#240409=CARTESIAN_POINT('Ctrl Pts',(-6.57070623700006,11.6,9.14082405799999));
#240410=CARTESIAN_POINT('Ctrl Pts',(-6.57370137600005,15.2,9.14261897199999));
#240411=CARTESIAN_POINT('Ctrl Pts',(-6.57370137600005,11.6,9.14261897199999));
#240412=CARTESIAN_POINT('Ctrl Pts',(-6.57670200100006,15.2,9.14441398599998));
#240413=CARTESIAN_POINT('Ctrl Pts',(-6.57670200100006,11.6,9.14441398599998));
#240414=CARTESIAN_POINT('Ctrl Pts',(-6.57970810800006,15.2,9.14620908999999));
#240415=CARTESIAN_POINT('Ctrl Pts',(-6.57970810800006,11.6,9.14620908999999));
#240416=CARTESIAN_POINT('Ctrl Pts',(-6.58271969500006,15.2,9.14800427499999));
#240417=CARTESIAN_POINT('Ctrl Pts',(-6.58271969500006,11.6,9.14800427499999));
#240418=CARTESIAN_POINT('Ctrl Pts',(-6.58573675800006,15.2,9.14979953099999));
#240419=CARTESIAN_POINT('Ctrl Pts',(-6.58573675800006,11.6,9.14979953099999));
#240420=CARTESIAN_POINT('Ctrl Pts',(-6.58875929300006,15.2,9.15159484899998));
#240421=CARTESIAN_POINT('Ctrl Pts',(-6.58875929300006,11.6,9.15159484899998));
#240422=CARTESIAN_POINT('Ctrl Pts',(-6.59178729700006,15.2,9.15339021899998));
#240423=CARTESIAN_POINT('Ctrl Pts',(-6.59178729700006,11.6,9.15339021899998));
#240424=CARTESIAN_POINT('Ctrl Pts',(-6.59482076700006,15.2,9.15518563399999));
#240425=CARTESIAN_POINT('Ctrl Pts',(-6.59482076700006,11.6,9.15518563399999));
#240426=CARTESIAN_POINT('Ctrl Pts',(-6.59785969700006,15.2,9.15698108299999));
#240427=CARTESIAN_POINT('Ctrl Pts',(-6.59785969700006,11.6,9.15698108299999));
#240428=CARTESIAN_POINT('Ctrl Pts',(-6.60090408600006,15.2,9.15877655699998));
#240429=CARTESIAN_POINT('Ctrl Pts',(-6.60090408600006,11.6,9.15877655699998));
#240430=CARTESIAN_POINT('Ctrl Pts',(-6.60395393000006,15.2,9.16057204699998));
#240431=CARTESIAN_POINT('Ctrl Pts',(-6.60395393000006,11.6,9.16057204699998));
#240432=CARTESIAN_POINT('Ctrl Pts',(-6.60700922500006,15.2,9.16236754499998));
#240433=CARTESIAN_POINT('Ctrl Pts',(-6.60700922500006,11.6,9.16236754499998));
#240434=CARTESIAN_POINT('Ctrl Pts',(-6.61006996700006,15.2,9.16416303799998));
#240435=CARTESIAN_POINT('Ctrl Pts',(-6.61006996700006,11.6,9.16416303799998));
#240436=CARTESIAN_POINT('Ctrl Pts',(-6.61313615300006,15.2,9.16595852199999));
#240437=CARTESIAN_POINT('Ctrl Pts',(-6.61313615300006,11.6,9.16595852199999));
#240438=CARTESIAN_POINT('Ctrl Pts',(-6.61620778000006,15.2,9.16775398399999));
#240439=CARTESIAN_POINT('Ctrl Pts',(-6.61620778000006,11.6,9.16775398399999));
#240440=CARTESIAN_POINT('Ctrl Pts',(-6.61928484300006,15.2,9.16954941699998));
#240441=CARTESIAN_POINT('Ctrl Pts',(-6.61928484300006,11.6,9.16954941699998));
#240442=CARTESIAN_POINT('Ctrl Pts',(-6.62236734000006,15.2,9.17134481099998));
#240443=CARTESIAN_POINT('Ctrl Pts',(-6.62236734000006,11.6,9.17134481099998));
#240444=CARTESIAN_POINT('Ctrl Pts',(-6.62545526800006,15.2,9.17314015699999));
#240445=CARTESIAN_POINT('Ctrl Pts',(-6.62545526800006,11.6,9.17314015699999));
#240446=CARTESIAN_POINT('Ctrl Pts',(-6.62854862100006,15.2,9.17493544599999));
#240447=CARTESIAN_POINT('Ctrl Pts',(-6.62854862100006,11.6,9.17493544599999));
#240448=CARTESIAN_POINT('Ctrl Pts',(-6.63164739700006,15.2,9.17673066999999));
#240449=CARTESIAN_POINT('Ctrl Pts',(-6.63164739700006,11.6,9.17673066999999));
#240450=CARTESIAN_POINT('Ctrl Pts',(-6.63475159200006,15.2,9.17852581799998));
#240451=CARTESIAN_POINT('Ctrl Pts',(-6.63475159200006,11.6,9.17852581799998));
#240452=CARTESIAN_POINT('Ctrl Pts',(-6.63786120400006,15.2,9.18032088299999));
#240453=CARTESIAN_POINT('Ctrl Pts',(-6.63786120400006,11.6,9.18032088299999));
#240454=CARTESIAN_POINT('Ctrl Pts',(-6.64097622600006,15.2,9.18211585499999));
#240455=CARTESIAN_POINT('Ctrl Pts',(-6.64097622600006,11.6,9.18211585499999));
#240456=CARTESIAN_POINT('Ctrl Pts',(-6.64409665800005,15.2,9.18391072499999));
#240457=CARTESIAN_POINT('Ctrl Pts',(-6.64409665800005,11.6,9.18391072499999));
#240458=CARTESIAN_POINT('Ctrl Pts',(-6.64722249500006,15.2,9.18570548399998));
#240459=CARTESIAN_POINT('Ctrl Pts',(-6.64722249500006,11.6,9.18570548399998));
#240460=CARTESIAN_POINT('Ctrl Pts',(-6.65035373400006,15.2,9.18750012399999));
#240461=CARTESIAN_POINT('Ctrl Pts',(-6.65035373400006,11.6,9.18750012399999));
#240462=CARTESIAN_POINT('Ctrl Pts',(-6.65349037000006,15.2,9.18929463599999));
#240463=CARTESIAN_POINT('Ctrl Pts',(-6.65349037000006,11.6,9.18929463599999));
#240464=CARTESIAN_POINT('Ctrl Pts',(-6.65663240100006,15.2,9.19108900999999));
#240465=CARTESIAN_POINT('Ctrl Pts',(-6.65663240100006,11.6,9.19108900999999));
#240466=CARTESIAN_POINT('Ctrl Pts',(-6.65977982200006,15.2,9.19288323799999));
#240467=CARTESIAN_POINT('Ctrl Pts',(-6.65977982200006,11.6,9.19288323799999));
#240468=CARTESIAN_POINT('Ctrl Pts',(-6.66293263000005,15.2,9.19467731099999));
#240469=CARTESIAN_POINT('Ctrl Pts',(-6.66293263000005,11.6,9.19467731099999));
#240470=CARTESIAN_POINT('Ctrl Pts',(-6.66609082400006,15.2,9.19647121999999));
#240471=CARTESIAN_POINT('Ctrl Pts',(-6.66609082400006,11.6,9.19647121999999));
#240472=CARTESIAN_POINT('Ctrl Pts',(-6.66925439600006,15.2,9.19826495599998));
#240473=CARTESIAN_POINT('Ctrl Pts',(-6.66925439600006,11.6,9.19826495599998));
#240474=CARTESIAN_POINT('Ctrl Pts',(-6.67242334600005,15.2,9.20005851099998));
#240475=CARTESIAN_POINT('Ctrl Pts',(-6.67242334600005,11.6,9.20005851099998));
#240476=CARTESIAN_POINT('Ctrl Pts',(-6.67559766800006,15.2,9.20185187599999));
#240477=CARTESIAN_POINT('Ctrl Pts',(-6.67559766800006,11.6,9.20185187599999));
#240478=CARTESIAN_POINT('Ctrl Pts',(-6.67877735900006,15.2,9.20364504199998));
#240479=CARTESIAN_POINT('Ctrl Pts',(-6.67877735900006,11.6,9.20364504199998));
#240480=CARTESIAN_POINT('Ctrl Pts',(-6.68196241700006,15.2,9.20543799999999));
#240481=CARTESIAN_POINT('Ctrl Pts',(-6.68196241700006,11.6,9.20543799999999));
#240482=CARTESIAN_POINT('Ctrl Pts',(-6.68515283700006,15.2,9.20723074199999));
#240483=CARTESIAN_POINT('Ctrl Pts',(-6.68515283700006,11.6,9.20723074199999));
#240484=CARTESIAN_POINT('Ctrl Pts',(-6.68834861700006,15.2,9.20902325999998));
#240485=CARTESIAN_POINT('Ctrl Pts',(-6.68834861700006,11.6,9.20902325999998));
#240486=CARTESIAN_POINT('Ctrl Pts',(-6.69154975100006,15.2,9.21081554299998));
#240487=CARTESIAN_POINT('Ctrl Pts',(-6.69154975100006,11.6,9.21081554299998));
#240488=CARTESIAN_POINT('Ctrl Pts',(-6.69475623700006,15.2,9.21260758499999));
#240489=CARTESIAN_POINT('Ctrl Pts',(-6.69475623700006,11.6,9.21260758499999));
#240490=CARTESIAN_POINT('Ctrl Pts',(-6.69796807000006,15.2,9.21439937499999));
#240491=CARTESIAN_POINT('Ctrl Pts',(-6.69796807000006,11.6,9.21439937499999));
#240492=CARTESIAN_POINT('Ctrl Pts',(-6.70118525000006,15.2,9.21619090599999));
#240493=CARTESIAN_POINT('Ctrl Pts',(-6.70118525000006,11.6,9.21619090599999));
#240494=CARTESIAN_POINT('Ctrl Pts',(-6.70440776900006,15.2,9.21798216799999));
#240495=CARTESIAN_POINT('Ctrl Pts',(-6.70440776900006,11.6,9.21798216799999));
#240496=CARTESIAN_POINT('Ctrl Pts',(-6.70763562600006,15.2,9.21977315299999));
#240497=CARTESIAN_POINT('Ctrl Pts',(-6.70763562600006,11.6,9.21977315299999));
#240498=CARTESIAN_POINT('Ctrl Pts',(-6.71086881600006,15.2,9.22156385299999));
#240499=CARTESIAN_POINT('Ctrl Pts',(-6.71086881600006,11.6,9.22156385299999));
#240500=CARTESIAN_POINT('Ctrl Pts',(-6.71410733700006,15.2,9.22335425999999));
#240501=CARTESIAN_POINT('Ctrl Pts',(-6.71410733700006,11.6,9.22335425999999));
#240502=CARTESIAN_POINT('Ctrl Pts',(-6.71735118500006,15.2,9.22514436399998));
#240503=CARTESIAN_POINT('Ctrl Pts',(-6.71735118500006,11.6,9.22514436399998));
#240504=CARTESIAN_POINT('Ctrl Pts',(-6.72060035600006,15.2,9.22693415799999));
#240505=CARTESIAN_POINT('Ctrl Pts',(-6.72060035600006,11.6,9.22693415799999));
#240506=CARTESIAN_POINT('Ctrl Pts',(-6.72385484600006,15.2,9.22872363199998));
#240507=CARTESIAN_POINT('Ctrl Pts',(-6.72385484600006,11.6,9.22872363199998));
#240508=CARTESIAN_POINT('Ctrl Pts',(-6.72711465300006,15.2,9.23051277999999));
#240509=CARTESIAN_POINT('Ctrl Pts',(-6.72711465300006,11.6,9.23051277999999));
#240510=CARTESIAN_POINT('Ctrl Pts',(-6.73037977400006,15.2,9.23230159099998));
#240511=CARTESIAN_POINT('Ctrl Pts',(-6.73037977400006,11.6,9.23230159099998));
#240512=CARTESIAN_POINT('Ctrl Pts',(-6.73365020100006,15.2,9.23409005699998));
#240513=CARTESIAN_POINT('Ctrl Pts',(-6.73365020100006,11.6,9.23409005699998));
#240514=CARTESIAN_POINT('Ctrl Pts',(-6.73692593500006,15.2,9.23587816999999));
#240515=CARTESIAN_POINT('Ctrl Pts',(-6.73692593500006,11.6,9.23587816999999));
#240516=CARTESIAN_POINT('Ctrl Pts',(-6.74020697000006,15.2,9.23766591999998));
#240517=CARTESIAN_POINT('Ctrl Pts',(-6.74020697000006,11.6,9.23766591999998));
#240518=CARTESIAN_POINT('Ctrl Pts',(-6.74349330200006,15.2,9.23945329999999));
#240519=CARTESIAN_POINT('Ctrl Pts',(-6.74349330200006,11.6,9.23945329999999));
#240520=CARTESIAN_POINT('Ctrl Pts',(-6.74678492800005,15.2,9.24124030099998));
#240521=CARTESIAN_POINT('Ctrl Pts',(-6.74678492800005,11.6,9.24124030099998));
#240522=CARTESIAN_POINT('Ctrl Pts',(-6.75008184500006,15.2,9.24302691299999));
#240523=CARTESIAN_POINT('Ctrl Pts',(-6.75008184500006,11.6,9.24302691299999));
#240524=CARTESIAN_POINT('Ctrl Pts',(-6.75338405000006,15.2,9.24481313199998));
#240525=CARTESIAN_POINT('Ctrl Pts',(-6.75338405000006,11.6,9.24481313199998));
#240526=CARTESIAN_POINT('Ctrl Pts',(-6.75669154000006,15.2,9.24659894899998));
#240527=CARTESIAN_POINT('Ctrl Pts',(-6.75669154000006,11.6,9.24659894899998));
#240528=CARTESIAN_POINT('Ctrl Pts',(-6.76000431000006,15.2,9.24838435599998));
#240529=CARTESIAN_POINT('Ctrl Pts',(-6.76000431000006,11.6,9.24838435599998));
#240530=CARTESIAN_POINT('Ctrl Pts',(-6.76332235800006,15.2,9.25016934499999));
#240531=CARTESIAN_POINT('Ctrl Pts',(-6.76332235800006,11.6,9.25016934499999));
#240532=CARTESIAN_POINT('Ctrl Pts',(-6.76664568000006,15.2,9.25195390799999));
#240533=CARTESIAN_POINT('Ctrl Pts',(-6.76664568000006,11.6,9.25195390799999));
#240534=CARTESIAN_POINT('Ctrl Pts',(-6.76997427200006,15.2,9.25373803599999));
#240535=CARTESIAN_POINT('Ctrl Pts',(-6.76997427200006,11.6,9.25373803599999));
#240536=CARTESIAN_POINT('Ctrl Pts',(-6.77330812800006,15.2,9.25552171799998));
#240537=CARTESIAN_POINT('Ctrl Pts',(-6.77330812800006,11.6,9.25552171799998));
#240538=CARTESIAN_POINT('Ctrl Pts',(-6.77664724700006,15.2,9.25730494399998));
#240539=CARTESIAN_POINT('Ctrl Pts',(-6.77664724700006,11.6,9.25730494399998));
#240540=CARTESIAN_POINT('Ctrl Pts',(-6.77999162100006,15.2,9.25908770299999));
#240541=CARTESIAN_POINT('Ctrl Pts',(-6.77999162100006,11.6,9.25908770299999));
#240542=CARTESIAN_POINT('Ctrl Pts',(-6.78334124800006,15.2,9.26086998699999));
#240543=CARTESIAN_POINT('Ctrl Pts',(-6.78334124800006,11.6,9.26086998699999));
#240544=CARTESIAN_POINT('Ctrl Pts',(-6.78669612400006,15.2,9.26265178799999));
#240545=CARTESIAN_POINT('Ctrl Pts',(-6.78669612400006,11.6,9.26265178799999));
#240546=CARTESIAN_POINT('Ctrl Pts',(-6.79005624900006,15.2,9.26443310199998));
#240547=CARTESIAN_POINT('Ctrl Pts',(-6.79005624900006,11.6,9.26443310199998));
#240548=CARTESIAN_POINT('Ctrl Pts',(-6.79342161700006,15.2,9.26621392399999));
#240549=CARTESIAN_POINT('Ctrl Pts',(-6.79342161700006,11.6,9.26621392399999));
#240550=CARTESIAN_POINT('Ctrl Pts',(-6.79679223000006,15.2,9.26799425399999));
#240551=CARTESIAN_POINT('Ctrl Pts',(-6.79679223000006,11.6,9.26799425399999));
#240552=CARTESIAN_POINT('Ctrl Pts',(-6.79949291500006,15.2,9.26941812099999));
#240553=CARTESIAN_POINT('Ctrl Pts',(-6.79949291500006,11.6,9.26941812099999));
#240554=CARTESIAN_POINT('Ctrl Pts',(-6.80152078900006,15.2,9.27048579799998));
#240555=CARTESIAN_POINT('Ctrl Pts',(-6.80152078900006,11.6,9.27048579799998));
#240556=CARTESIAN_POINT('Ctrl Pts',(-6.80287375200006,15.2,9.27119748399999));
#240557=CARTESIAN_POINT('Ctrl Pts',(-6.80287375200006,11.6,9.27119748399999));
#240558=CARTESIAN_POINT('Ctrl Pts',(-6.80355049700006,15.2,9.27155330199999));
#240559=CARTESIAN_POINT('Ctrl Pts',(-6.80355049700006,11.6,9.27155330199999));
#240560=CARTESIAN_POINT('Ctrl Pts',(-5.85257411500006,15.2,8.56667970999998));
#240561=CARTESIAN_POINT('Ctrl Pts',(-5.8537050266944,15.2,8.56806288496946));
#240562=CARTESIAN_POINT('Ctrl Pts',(-5.8548762742267,15.2,8.5694869238734));
#240563=CARTESIAN_POINT('Ctrl Pts',(-5.85608775334231,15.2,8.57095065186461));
#240564=CARTESIAN_POINT('Ctrl Pts',(-5.85730507482257,15.2,8.57242143869206));
#240565=CARTESIAN_POINT('Ctrl Pts',(-5.85856301277102,15.2,8.57393230486909));
#240566=CARTESIAN_POINT('Ctrl Pts',(-5.85986145340903,15.2,8.5754821088666));
#240567=CARTESIAN_POINT('Ctrl Pts',(-5.86115989392909,15.2,8.57703191272334));
#240568=CARTESIAN_POINT('Ctrl Pts',(-5.86249883775011,15.2,8.5786206548507));
#240569=CARTESIAN_POINT('Ctrl Pts',(-5.86387817019999,15.2,8.58024722870826));
#240570=CARTESIAN_POINT('Ctrl Pts',(-5.86525750264987,15.2,8.58187380256584));
#240571=CARTESIAN_POINT('Ctrl Pts',(-5.86667722397461,15.2,8.58353820930605));
#240572=CARTESIAN_POINT('Ctrl Pts',(-5.86813722065885,15.2,8.58523937157711));
#240573=CARTESIAN_POINT('Ctrl Pts',(-5.86959721747571,15.2,8.58694053400272));
#240574=CARTESIAN_POINT('Ctrl Pts',(-5.87109749092289,15.2,8.58867845508586));
#240575=CARTESIAN_POINT('Ctrl Pts',(-5.87263792542624,15.2,8.59045208743492));
#240576=CARTESIAN_POINT('Ctrl Pts',(-5.87417835978964,15.2,8.5922257196229));
#240577=CARTESIAN_POINT('Ctrl Pts',(-5.87575895551881,15.2,8.59403506540096));
#240578=CARTESIAN_POINT('Ctrl Pts',(-5.87737960096739,15.2,8.5958791057591));
#240579=CARTESIAN_POINT('Ctrl Pts',(-5.87927035408887,15.2,8.59803048628858));
#240580=CARTESIAN_POINT('Ctrl Pts',(-5.88121561762475,15.2,8.6002290925998));
#240581=CARTESIAN_POINT('Ctrl Pts',(-5.88321521364515,15.2,8.60247335719295));
#240582=CARTESIAN_POINT('Ctrl Pts',(-5.88492915300225,15.2,8.60439701245866));
#240583=CARTESIAN_POINT('Ctrl Pts',(-5.88668300813275,15.2,8.60635421247237));
#240584=CARTESIAN_POINT('Ctrl Pts',(-5.88847666749247,15.2,8.6083439999925));
#240585=CARTESIAN_POINT('Ctrl Pts',(-5.8902703268522,15.2,8.61033378751263));
#240586=CARTESIAN_POINT('Ctrl Pts',(-5.89210378938454,15.2,8.61235616293915));
#240587=CARTESIAN_POINT('Ctrl Pts',(-5.89397694364806,15.2,8.61441019244645));
#240588=CARTESIAN_POINT('Ctrl Pts',(-5.89585009808173,15.2,8.61646422214033));
#240589=CARTESIAN_POINT('Ctrl Pts',(-5.89776294240371,15.2,8.61854990460485));
#240590=CARTESIAN_POINT('Ctrl Pts',(-5.89971536501281,15.2,8.6206663334723));
#240591=CARTESIAN_POINT('Ctrl Pts',(-5.90166778744456,15.2,8.6227827621475));
#240592=CARTESIAN_POINT('Ctrl Pts',(-5.90365978830796,15.2,8.62492993613816));
#240593=CARTESIAN_POINT('Ctrl Pts',(-5.9056912528192,15.2,8.6271069661437));
#240594=CARTESIAN_POINT('Ctrl Pts',(-5.90772271733044,15.2,8.62928399614923));
#240595=CARTESIAN_POINT('Ctrl Pts',(-5.90979364614689,15.2,8.63149088590239));
#240596=CARTESIAN_POINT('Ctrl Pts',(-5.91190392740181,15.2,8.6337267679032));
#240597=CARTESIAN_POINT('Ctrl Pts',(-5.91401420865675,15.2,8.63596264990402));
#240598=CARTESIAN_POINT('Ctrl Pts',(-5.91616383903528,15.2,8.63822752557691));
#240599=CARTESIAN_POINT('Ctrl Pts',(-5.91835271020307,15.2,8.64052054974167));
#240600=CARTESIAN_POINT('Ctrl Pts',(-5.92054158156969,15.2,8.64281357411472));
#240601=CARTESIAN_POINT('Ctrl Pts',(-5.92276968905676,15.2,8.64513474665718));
#240602=CARTESIAN_POINT('Ctrl Pts',(-5.92503692259871,15.2,8.64748324586971));
#240603=CARTESIAN_POINT('Ctrl Pts',(-5.92730415593471,15.2,8.64983174486891));
#240604=CARTESIAN_POINT('Ctrl Pts',(-5.92961051367591,15.2,8.65220756702423));
#240605=CARTESIAN_POINT('Ctrl Pts',(-5.93195588292233,15.2,8.65460991210245));
#240606=CARTESIAN_POINT('Ctrl Pts',(-5.93430125216874,15.2,8.65701225718068));
#240607=CARTESIAN_POINT('Ctrl Pts',(-5.93668563130987,15.2,8.65944112073997));
#240608=CARTESIAN_POINT('Ctrl Pts',(-5.93910890871919,15.2,8.6618957199824));
#240609=CARTESIAN_POINT('Ctrl Pts',(-5.94153218634864,15.2,8.66435031944778));
#240610=CARTESIAN_POINT('Ctrl Pts',(-5.94399436180682,15.2,8.66683065198232));
#240611=CARTESIAN_POINT('Ctrl Pts',(-5.94649532036145,15.2,8.66933595061991));
#240612=CARTESIAN_POINT('Ctrl Pts',(-5.94899627868892,15.2,8.67184124902994));
#240613=CARTESIAN_POINT('Ctrl Pts',(-5.9515360211392,15.2,8.67437151465504));
#240614=CARTESIAN_POINT('Ctrl Pts',(-5.95411443247382,15.2,8.67692599499046));
#240615=CARTESIAN_POINT('Ctrl Pts',(-5.95669284380845,15.2,8.67948047532588));
#240616=CARTESIAN_POINT('Ctrl Pts',(-5.95930992571798,15.2,8.68205916772079));
#240617=CARTESIAN_POINT('Ctrl Pts',(-5.9619655612022,15.2,8.68466134220798));
#240618=CARTESIAN_POINT('Ctrl Pts',(-5.96462119692765,15.2,8.68726351693154));
#240619=CARTESIAN_POINT('Ctrl Pts',(-5.96731538830176,15.2,8.68988917133658));
#240620=CARTESIAN_POINT('Ctrl Pts',(-5.9700480210061,15.2,8.6925375855312));
#240621=CARTESIAN_POINT('Ctrl Pts',(-5.97323609212215,15.2,8.69562740173075));
#240622=CARTESIAN_POINT('Ctrl Pts',(-5.97647648353938,15.2,8.69874819882578));
#240623=CARTESIAN_POINT('Ctrl Pts',(-5.97976901548404,15.2,8.70189885973892));
#240624=CARTESIAN_POINT('Ctrl Pts',(-5.98259118605191,15.2,8.70459942655127));
#240625=CARTESIAN_POINT('Ctrl Pts',(-5.98545166310051,15.2,8.70732193373593));
#240626=CARTESIAN_POINT('Ctrl Pts',(-5.98835033198882,15.2,8.71006569677376));
#240627=CARTESIAN_POINT('Ctrl Pts',(-5.99076588926411,15.2,8.71235216584733));
#240628=CARTESIAN_POINT('Ctrl Pts',(-5.99320796928185,15.2,8.71465339406278));
#240629=CARTESIAN_POINT('Ctrl Pts',(-5.99567650379788,15.2,8.7169689939945));
#240630=CARTESIAN_POINT('Ctrl Pts',(-5.99863874510948,15.2,8.71974771381159));
#240631=CARTESIAN_POINT('Ctrl Pts',(-6.00163908157287,15.2,8.72254712691582));
#240632=CARTESIAN_POINT('Ctrl Pts',(-6.00467739972638,15.2,8.7253665727429));
#240633=CARTESIAN_POINT('Ctrl Pts',(-6.00720933161296,15.2,8.72771611101751));
#240634=CARTESIAN_POINT('Ctrl Pts',(-6.00976763708449,15.2,8.73007955979923));
#240635=CARTESIAN_POINT('Ctrl Pts',(-6.01235225166918,15.2,8.73245654639715));
#240636=CARTESIAN_POINT('Ctrl Pts',(-6.01493686625387,15.2,8.73483353299506));
#240637=CARTESIAN_POINT('Ctrl Pts',(-6.0175477886768,15.2,8.73722405546766));
#240638=CARTESIAN_POINT('Ctrl Pts',(-6.02018495166428,15.2,8.73962774394056));
#240639=CARTESIAN_POINT('Ctrl Pts',(-6.02282211465175,15.2,8.74203143241346));
#240640=CARTESIAN_POINT('Ctrl Pts',(-6.02548552030945,15.2,8.74444828894865));
#240641=CARTESIAN_POINT('Ctrl Pts',(-6.02817509836231,15.2,8.74687794830705));
#240642=CARTESIAN_POINT('Ctrl Pts',(-6.03086467641516,15.2,8.74930760766543));
#240643=CARTESIAN_POINT('Ctrl Pts',(-6.03358042886206,15.2,8.75175007007004));
#240644=CARTESIAN_POINT('Ctrl Pts',(-6.03632228685029,15.2,8.75420498007106));
#240645=CARTESIAN_POINT('Ctrl Pts',(-6.03906414483854,15.2,8.75665989007207));
#240646=CARTESIAN_POINT('Ctrl Pts',(-6.04183210986332,15.2,8.7591272449066));
#240647=CARTESIAN_POINT('Ctrl Pts',(-6.04462611361546,15.2,8.76160669428261));
#240648=CARTESIAN_POINT('Ctrl Pts',(-6.04742011706305,15.2,8.76408614338834));
#240649=CARTESIAN_POINT('Ctrl Pts',(-6.05024015951785,15.2,8.76657768876854));
#240650=CARTESIAN_POINT('Ctrl Pts',(-6.05308617288608,15.2,8.7690809804392));
#240651=CARTESIAN_POINT('Ctrl Pts',(-6.05593218656454,15.2,8.77158427238271));
#240652=CARTESIAN_POINT('Ctrl Pts',(-6.05880417311198,15.2,8.7740993139149));
#240653=CARTESIAN_POINT('Ctrl Pts',(-6.06170206109596,15.2,8.77662576238617));
#240654=CARTESIAN_POINT('Ctrl Pts',(-6.06459994907992,15.2,8.77915221085743));
#240655=CARTESIAN_POINT('Ctrl Pts',(-6.067523741601,15.2,8.78169006623308));
#240656=CARTESIAN_POINT('Ctrl Pts',(-6.07047336889934,15.2,8.78423899497077));
#240657=CARTESIAN_POINT('Ctrl Pts',(-6.07342299619768,15.2,8.78678792370845));
#240658=CARTESIAN_POINT('Ctrl Pts',(-6.07639846060521,15.2,8.78934792409357));
#240659=CARTESIAN_POINT('Ctrl Pts',(-6.07939969102053,15.2,8.7919186661069));
#240660=CARTESIAN_POINT('Ctrl Pts',(-6.08240092143587,15.2,8.79448940812023));
#240661=CARTESIAN_POINT('Ctrl Pts',(-6.08542792042408,15.2,8.79707089179773));
#240662=CARTESIAN_POINT('Ctrl Pts',(-6.0884806175755,15.2,8.79966279138051));
#240663=CARTESIAN_POINT('Ctrl Pts',(-6.09153331472692,15.2,8.80225469096329));
#240664=CARTESIAN_POINT('Ctrl Pts',(-6.09461171143183,15.2,8.80485700749638));
#240665=CARTESIAN_POINT('Ctrl Pts',(-6.09771573934714,15.2,8.80746941957917));
#240666=CARTESIAN_POINT('Ctrl Pts',(-6.10081976726246,15.2,8.81008183166197));
#240667=CARTESIAN_POINT('Ctrl Pts',(-6.10394942578958,15.2,8.81270433960326));
#240668=CARTESIAN_POINT('Ctrl Pts',(-6.10710464774828,15.2,8.81533662753186));
#240669=CARTESIAN_POINT('Ctrl Pts',(-6.11025986970697,15.2,8.81796891546045));
#240670=CARTESIAN_POINT('Ctrl Pts',(-6.11344065219998,15.2,8.82061098314996));
#240671=CARTESIAN_POINT('Ctrl Pts',(-6.11664693074166,15.2,8.8232625202333));
#240672=CARTESIAN_POINT('Ctrl Pts',(-6.11921195371481,15.2,8.82538375001559));
#240673=CARTESIAN_POINT('Ctrl Pts',(-6.12179329104539,15.2,8.82751103911801));
#240674=CARTESIAN_POINT('Ctrl Pts',(-6.12439091013305,15.2,8.82964423162374));
#240675=CARTESIAN_POINT('Ctrl Pts',(-6.1282873384106,15.2,8.83284402009169));
#240676=CARTESIAN_POINT('Ctrl Pts',(-6.13222039943412,15.2,8.83605709057581));
#240677=CARTESIAN_POINT('Ctrl Pts',(-6.13618997270815,15.2,8.83928291812583));
#240678=CARTESIAN_POINT('Ctrl Pts',(-6.13883635477065,15.2,8.84143346972817));
#240679=CARTESIAN_POINT('Ctrl Pts',(-6.14149896556602,15.2,8.84358969119049));
#240680=CARTESIAN_POINT('Ctrl Pts',(-6.14417776834535,15.2,8.84575143134652));
#240681=CARTESIAN_POINT('Ctrl Pts',(-6.14685657148967,15.2,8.84791317179709));
#240682=CARTESIAN_POINT('Ctrl Pts',(-6.14955156687227,15.2,8.85008043000093));
#240683=CARTESIAN_POINT('Ctrl Pts',(-6.15226271997685,15.2,8.85225305401811));
#240684=CARTESIAN_POINT('Ctrl Pts',(-6.15497387271203,15.2,8.85442567773928));
#240685=CARTESIAN_POINT('Ctrl Pts',(-6.15770118282183,15.2,8.8566036690137));
#240686=CARTESIAN_POINT('Ctrl Pts',(-6.16044461481811,15.2,8.85878687666801));
#240687=CARTESIAN_POINT('Ctrl Pts',(-6.16318804718819,15.2,8.86097008461978));
#240688=CARTESIAN_POINT('Ctrl Pts',(-6.16594759985984,15.2,8.86315851003598));
#240689=CARTESIAN_POINT('Ctrl Pts',(-6.16872324023332,15.2,8.86535200526663));
#240690=CARTESIAN_POINT('Ctrl Pts',(-6.1714988806068,15.2,8.86754550049727));
#240691=CARTESIAN_POINT('Ctrl Pts',(-6.17429060765719,15.2,8.86974406536465));
#240692=CARTESIAN_POINT('Ctrl Pts',(-6.17709838420074,15.2,8.87194755331857));
#240693=CARTESIAN_POINT('Ctrl Pts',(-6.17990616036172,15.2,8.87415104097227));
#240694=CARTESIAN_POINT('Ctrl Pts',(-6.18272998704516,15.2,8.87635945217491));
#240695=CARTESIAN_POINT('Ctrl Pts',(-6.18556982971473,15.2,8.87857264244846));
#240696=CARTESIAN_POINT('Ctrl Pts',(-6.18840967277123,15.2,8.88078583302355));
#240697=CARTESIAN_POINT('Ctrl Pts',(-6.19126553131142,15.2,8.88300380253621));
#240698=CARTESIAN_POINT('Ctrl Pts',(-6.19413736846955,15.2,8.88522640788004));
#240699=CARTESIAN_POINT('Ctrl Pts',(-6.1970092052364,15.2,8.88744901292103));
#240700=CARTESIAN_POINT('Ctrl Pts',(-6.19989702052897,15.2,8.88967625531975));
#240701=CARTESIAN_POINT('Ctrl Pts',(-6.20280078051276,15.2,8.8919079905259));
#240702=CARTESIAN_POINT('Ctrl Pts',(-6.20570454089219,15.2,8.89413972603612));
#240703=CARTESIAN_POINT('Ctrl Pts',(-6.2086242440458,15.2,8.89637595751569));
#240704=CARTESIAN_POINT('Ctrl Pts',(-6.21155985590939,15.2,8.89861654358345));
#240705=CARTESIAN_POINT('Ctrl Pts',(-6.21449546737302,15.2,8.90085712934594));
#240706=CARTESIAN_POINT('Ctrl Pts',(-6.21744698676785,15.2,8.90310206926141));
#240707=CARTESIAN_POINT('Ctrl Pts',(-6.22041437752423,15.2,8.90535122629947));
#240708=CARTESIAN_POINT('Ctrl Pts',(-6.2233817686849,15.2,8.90760038364398));
#240709=CARTESIAN_POINT('Ctrl Pts',(-6.22636503181418,15.2,8.90985375738626));
#240710=CARTESIAN_POINT('Ctrl Pts',(-6.22936413097865,15.2,8.91211121067622));
#240711=CARTESIAN_POINT('Ctrl Pts',(-6.23236322973449,15.2,8.9143686636586));
#240712=CARTESIAN_POINT('Ctrl Pts',(-6.23537816486081,15.2,8.91663019459918));
#240713=CARTESIAN_POINT('Ctrl Pts',(-6.23840889981864,15.2,8.91889567163792));
#240714=CARTESIAN_POINT('Ctrl Pts',(-6.2414396351894,15.2,8.92116114898534));
#240715=CARTESIAN_POINT('Ctrl Pts',(-6.24448617107701,15.2,8.92343056941171));
#240716=CARTESIAN_POINT('Ctrl Pts',(-6.24754847080049,15.2,8.92570380020251));
#240717=CARTESIAN_POINT('Ctrl Pts',(-6.25061077010671,15.2,8.92797703068358));
#240718=CARTESIAN_POINT('Ctrl Pts',(-6.25368883269314,15.2,8.93025407062779));
#240719=CARTESIAN_POINT('Ctrl Pts',(-6.25678262399416,15.2,8.93253478838541));
#240720=CARTESIAN_POINT('Ctrl Pts',(-6.25987641571672,15.2,8.93481550645377));
#240721=CARTESIAN_POINT('Ctrl Pts',(-6.26298593538979,15.2,8.93709990191645));
#240722=CARTESIAN_POINT('Ctrl Pts',(-6.2661111460188,15.2,8.9393878427182));
#240723=CARTESIAN_POINT('Ctrl Pts',(-6.26923635622199,15.2,8.94167578320821));
#240724=CARTESIAN_POINT('Ctrl Pts',(-6.27237725994355,15.2,8.94396727034327));
#240725=CARTESIAN_POINT('Ctrl Pts',(-6.27553381801724,15.2,8.94626217343309));
#240726=CARTESIAN_POINT('Ctrl Pts',(-6.278690376521,15.2,8.94855707683559));
#240727=CARTESIAN_POINT('Ctrl Pts',(-6.28186259152071,15.2,8.95085539533565));
#240728=CARTESIAN_POINT('Ctrl Pts',(-6.28505042524999,15.2,8.95315700201664));
#240729=CARTESIAN_POINT('Ctrl Pts',(-6.28903521719443,15.2,8.95603401021108));
#240730=CARTESIAN_POINT('Ctrl Pts',(-6.29304441381157,15.2,8.9589161537884));
#240731=CARTESIAN_POINT('Ctrl Pts',(-6.29707794501053,15.2,8.96180318546822));
#240732=CARTESIAN_POINT('Ctrl Pts',(-6.30030476970591,15.2,8.96411281062326));
#240733=CARTESIAN_POINT('Ctrl Pts',(-6.30354716929914,15.2,8.96642556458597));
#240734=CARTESIAN_POINT('Ctrl Pts',(-6.30680510597566,15.2,8.96874131989635));
#240735=CARTESIAN_POINT('Ctrl Pts',(-6.31169201165627,15.2,8.9722149533352));
#240736=CARTESIAN_POINT('Ctrl Pts',(-6.31661387607365,15.2,8.97569534314141));
#240737=CARTESIAN_POINT('Ctrl Pts',(-6.32157057776195,15.2,8.97918206841503));
#240738=CARTESIAN_POINT('Ctrl Pts',(-6.32652727900002,15.2,8.98266879337194));
#240739=CARTESIAN_POINT('Ctrl Pts',(-6.33151881653533,15.2,8.98616185404502));
#240740=CARTESIAN_POINT('Ctrl Pts',(-6.33654506776788,15.2,8.98966083700097));
#240741=CARTESIAN_POINT('Ctrl Pts',(-6.33989590222727,15.2,8.99199349251682));
#240742=CARTESIAN_POINT('Ctrl Pts',(-6.34326216468622,15.2,8.99432878125592));
#240743=CARTESIAN_POINT('Ctrl Pts',(-6.34664381870745,15.2,8.99666658038923));
#240744=CARTESIAN_POINT('Ctrl Pts',(-6.35002547226794,15.2,8.999004379204));
#240745=CARTESIAN_POINT('Ctrl Pts',(-6.35342251877061,15.2,9.00134469013906));
#240746=CARTESIAN_POINT('Ctrl Pts',(-6.35683491821284,15.2,9.00368739205848));
#240747=CARTESIAN_POINT('Ctrl Pts',(-6.36024731812,15.2,9.00603009429709));
#240748=CARTESIAN_POINT('Ctrl Pts',(-6.36367507370687,15.2,9.00837518923883));
#240749=CARTESIAN_POINT('Ctrl Pts',(-6.36711814750661,15.2,9.01072255620023));
#240750=CARTESIAN_POINT('Ctrl Pts',(-6.37056122083724,15.2,9.0130699228418));
#240751=CARTESIAN_POINT('Ctrl Pts',(-6.37401961178556,15.2,9.01541956307257));
#240752=CARTESIAN_POINT('Ctrl Pts',(-6.37749328522935,15.2,9.01777135844206));
#240753=CARTESIAN_POINT('Ctrl Pts',(-6.38183537738905,15.2,9.02071110289423));
#240754=CARTESIAN_POINT('Ctrl Pts',(-6.38620134575318,15.2,9.02365421482414));
#240755=CARTESIAN_POINT('Ctrl Pts',(-6.39059112019638,15.2,9.02660046753231));
#240756=CARTESIAN_POINT('Ctrl Pts',(-6.39410293994233,15.2,9.0289574698273));
#240757=CARTESIAN_POINT('Ctrl Pts',(-6.3976299954068,15.2,9.03131648287255));
#240758=CARTESIAN_POINT('Ctrl Pts',(-6.40117224982306,15.2,9.03367739050134));
#240759=CARTESIAN_POINT('Ctrl Pts',(-6.40471450375669,15.2,9.03603829780846));
#240760=CARTESIAN_POINT('Ctrl Pts',(-6.40827195387437,15.2,9.03840110095998));
#240761=CARTESIAN_POINT('Ctrl Pts',(-6.41184456798166,15.2,9.0407656844402));
#240762=CARTESIAN_POINT('Ctrl Pts',(-6.41720348987277,15.2,9.04431256014379));
#240763=CARTESIAN_POINT('Ctrl Pts',(-6.42259652490179,15.2,9.04786344487677));
#240764=CARTESIAN_POINT('Ctrl Pts',(-6.42802354861655,15.2,9.05141795540409));
#240765=CARTESIAN_POINT('Ctrl Pts',(-6.43164156393345,15.2,9.05378762876609));
#240766=CARTESIAN_POINT('Ctrl Pts',(-6.43527468541221,15.2,9.05615891414175));
#240767=CARTESIAN_POINT('Ctrl Pts',(-6.43892287666857,15.2,9.05853170078102));
#240768=CARTESIAN_POINT('Ctrl Pts',(-6.44439516380163,15.2,9.06209088090158));
#240769=CARTESIAN_POINT('Ctrl Pts',(-6.44990135729141,15.2,9.06565343737441));
#240770=CARTESIAN_POINT('Ctrl Pts',(-6.45544132967115,15.2,9.06921900041134));
#240771=CARTESIAN_POINT('Ctrl Pts',(-6.45913464492645,15.2,9.07159604265187));
#240772=CARTESIAN_POINT('Ctrl Pts',(-6.46284297496098,15.2,9.07397441871196));
#240773=CARTESIAN_POINT('Ctrl Pts',(-6.46656628077499,15.2,9.07635402300831));
#240774=CARTESIAN_POINT('Ctrl Pts',(-6.470289586589,15.2,9.07873362730465));
#240775=CARTESIAN_POINT('Ctrl Pts',(-6.47402786895481,15.2,9.08111445830117));
#240776=CARTESIAN_POINT('Ctrl Pts',(-6.47778109010532,15.2,9.08349640859776));
#240777=CARTESIAN_POINT('Ctrl Pts',(-6.48059600571252,15.2,9.08528287115794));
#240778=CARTESIAN_POINT('Ctrl Pts',(-6.48341932360841,15.2,9.08706996320477));
#240779=CARTESIAN_POINT('Ctrl Pts',(-6.48625103077295,15.2,9.08885763939586));
#240780=CARTESIAN_POINT('Ctrl Pts',(-6.48908273793749,15.2,9.09064531558694));
#240781=CARTESIAN_POINT('Ctrl Pts',(-6.49192283194672,15.2,9.09243357659325));
#240782=CARTESIAN_POINT('Ctrl Pts',(-6.49477129801062,15.2,9.09422237673664));
#240783=CARTESIAN_POINT('Ctrl Pts',(-6.49856925259,15.2,9.09660744348617));
#240784=CARTESIAN_POINT('Ctrl Pts',(-6.50238209094139,15.2,9.09899346830772));
#240785=CARTESIAN_POINT('Ctrl Pts',(-6.50620977434918,15.2,9.10138034883473));
#240786=CARTESIAN_POINT('Ctrl Pts',(-6.50908053755692,15.2,9.10317050963649));
#240787=CARTESIAN_POINT('Ctrl Pts',(-6.51195965244203,15.2,9.10496114953008));
#240788=CARTESIAN_POINT('Ctrl Pts',(-6.51484710165447,15.2,9.10675222591544));
#240789=CARTESIAN_POINT('Ctrl Pts',(-6.51773455034236,15.2,9.10854330197542));
#240790=CARTESIAN_POINT('Ctrl Pts',(-6.52063033495474,15.2,9.11033481415555));
#240791=CARTESIAN_POINT('Ctrl Pts',(-6.52353443828695,15.2,9.11212671838834));
#240792=CARTESIAN_POINT('Ctrl Pts',(-6.52740657588737,15.2,9.11451592392356));
#240793=CARTESIAN_POINT('Ctrl Pts',(-6.53129350428723,15.2,9.11690582679726));
#240794=CARTESIAN_POINT('Ctrl Pts',(-6.53519518368951,15.2,9.11929632354624));
#240795=CARTESIAN_POINT('Ctrl Pts',(-6.53812144337411,15.2,9.12108919618939));
#240796=CARTESIAN_POINT('Ctrl Pts',(-6.54105600216652,15.2,9.12288240300753));
#240797=CARTESIAN_POINT('Ctrl Pts',(-6.54399884285013,15.2,9.124675901109));
#240798=CARTESIAN_POINT('Ctrl Pts',(-6.5479226307847,15.2,9.12706723212817));
#240799=CARTESIAN_POINT('Ctrl Pts',(-6.55186114364701,15.2,9.12945908041037));
#240800=CARTESIAN_POINT('Ctrl Pts',(-6.55581434276936,15.2,9.13185134421828));
#240801=CARTESIAN_POINT('Ctrl Pts',(-6.55877924184182,15.2,9.13364554191125));
#240802=CARTESIAN_POINT('Ctrl Pts',(-6.56175240252545,15.2,9.13543997352207));
#240803=CARTESIAN_POINT('Ctrl Pts',(-6.56473380901396,15.2,9.13723459621502));
#240804=CARTESIAN_POINT('Ctrl Pts',(-6.56870901802639,15.2,9.13962742668962));
#240805=CARTESIAN_POINT('Ctrl Pts',(-6.572698884285,15.2,9.14202059782473));
#240806=CARTESIAN_POINT('Ctrl Pts',(-6.57670337217141,15.2,9.14441400889964));
#240807=CARTESIAN_POINT('Ctrl Pts',(-6.5807078595122,15.2,9.14680741964844));
#240808=CARTESIAN_POINT('Ctrl Pts',(-6.58472696791777,15.2,9.14920107096946));
#240809=CARTESIAN_POINT('Ctrl Pts',(-6.58876065992038,15.2,9.15159486182929));
#240810=CARTESIAN_POINT('Ctrl Pts',(-6.59279435247256,15.2,9.15398865301527));
#240811=CARTESIAN_POINT('Ctrl Pts',(-6.59684262835839,15.2,9.15638258605007));
#240812=CARTESIAN_POINT('Ctrl Pts',(-6.60090545033962,15.2,9.1587765613557));
#240813=CARTESIAN_POINT('Ctrl Pts',(-6.60395256654876,15.2,9.16057204267184));
#240814=CARTESIAN_POINT('Ctrl Pts',(-6.60700786469465,15.2,9.16236754814425));
#240815=CARTESIAN_POINT('Ctrl Pts',(-6.61007132833406,15.2,9.16416303587069));
#240816=CARTESIAN_POINT('Ctrl Pts',(-6.61313479197347,15.2,9.16595852359713));
#240817=CARTESIAN_POINT('Ctrl Pts',(-6.61620642181189,15.2,9.16775399461522));
#240818=CARTESIAN_POINT('Ctrl Pts',(-6.61928620149166,15.2,9.16954940725832));
#240819=CARTESIAN_POINT('Ctrl Pts',(-6.62236598117144,15.2,9.17134481990143));
#240820=CARTESIAN_POINT('Ctrl Pts',(-6.62545391225922,15.2,9.17314017388621));
#240821=CARTESIAN_POINT('Ctrl Pts',(-6.62854997639599,15.2,9.1749354295293));
#240822=CARTESIAN_POINT('Ctrl Pts',(-6.6337100834781,15.2,9.17792752237651));
#240823=CARTESIAN_POINT('Ctrl Pts',(-6.63889278531647,15.2,9.18091934074323));
#240824=CARTESIAN_POINT('Ctrl Pts',(-6.64409800892637,15.2,9.18391069706268));
#240825=CARTESIAN_POINT('Ctrl Pts',(-6.64722114297884,15.2,9.18570551078914));
#240826=CARTESIAN_POINT('Ctrl Pts',(-6.65035238486754,15.2,9.187500158895));
#240827=CARTESIAN_POINT('Ctrl Pts',(-6.65349171811769,15.2,9.18929460116947));
#240828=CARTESIAN_POINT('Ctrl Pts',(-6.65663105136784,15.2,9.19108904344394));
#240829=CARTESIAN_POINT('Ctrl Pts',(-6.65977847524454,15.2,9.19288327942405));
#240830=CARTESIAN_POINT('Ctrl Pts',(-6.66293397575377,15.2,9.1946772696089));
#240831=CARTESIAN_POINT('Ctrl Pts',(-6.66608947683624,15.2,9.19647126011965));
#240832=CARTESIAN_POINT('Ctrl Pts',(-6.66925305362938,15.2,9.19826500438034));
#240833=CARTESIAN_POINT('Ctrl Pts',(-6.67242468971643,15.2,9.20005846389096));
#240834=CARTESIAN_POINT('Ctrl Pts',(-6.6755963252273,15.2,9.20185192307577));
#240835=CARTESIAN_POINT('Ctrl Pts',(-6.67877601927939,15.2,9.20364509692724));
#240836=CARTESIAN_POINT('Ctrl Pts',(-6.6819637578726,15.2,9.20543794619541));
#240837=CARTESIAN_POINT('Ctrl Pts',(-6.68515149646582,15.2,9.20723079546358));
#240838=CARTESIAN_POINT('Ctrl Pts',(-6.6883472793714,15.2,9.20902332097525));
#240839=CARTESIAN_POINT('Ctrl Pts',(-6.69155108897791,15.2,9.21081548270995));
#240840=CARTESIAN_POINT('Ctrl Pts',(-6.69582283492591,15.2,9.21320503158101));
#240841=CARTESIAN_POINT('Ctrl Pts',(-6.70010885278324,15.2,9.21559393477689));
#240842=CARTESIAN_POINT('Ctrl Pts',(-6.70440910276358,15.2,9.21798209835952));
#240843=CARTESIAN_POINT('Ctrl Pts',(-6.70763429098122,15.2,9.21977322145323));
#240844=CARTESIAN_POINT('Ctrl Pts',(-6.71086748481779,15.2,9.22156392961348));
#240845=CARTESIAN_POINT('Ctrl Pts',(-6.71410866945659,15.2,9.22335418466526));
#240846=CARTESIAN_POINT('Ctrl Pts',(-6.71843024799363,15.2,9.22574119085892));
#240847=CARTESIAN_POINT('Ctrl Pts',(-6.72276603007051,15.2,9.22812739083048));
#240848=CARTESIAN_POINT('Ctrl Pts',(-6.72711598110286,15.2,9.23051269557998));
#240849=CARTESIAN_POINT('Ctrl Pts',(-6.7303784445253,15.2,9.23230167422336));
#240850=CARTESIAN_POINT('Ctrl Pts',(-6.73364887550538,15.2,9.23409014811298));
#240851=CARTESIAN_POINT('Ctrl Pts',(-6.73692725963246,15.2,9.23587807892906));
#240852=CARTESIAN_POINT('Ctrl Pts',(-6.74020564375954,15.2,9.23766600974515));
#240853=CARTESIAN_POINT('Ctrl Pts',(-6.74349197890263,15.2,9.23945339755863));
#240854=CARTESIAN_POINT('Ctrl Pts',(-6.74678625003185,15.2,9.24124020341047));
#240855=CARTESIAN_POINT('Ctrl Pts',(-6.75008052175955,15.2,9.2430270095869));
#240856=CARTESIAN_POINT('Ctrl Pts',(-6.75338273055612,15.2,9.24481323529649));
#240857=CARTESIAN_POINT('Ctrl Pts',(-6.75669286074662,15.2,9.24659884688925));
#240858=CARTESIAN_POINT('Ctrl Pts',(-6.76000299033577,15.2,9.24838445815763));
#240859=CARTESIAN_POINT('Ctrl Pts',(-6.76332104138283,15.2,9.25016945482603));
#240860=CARTESIAN_POINT('Ctrl Pts',(-6.766646997846,15.2,9.25195379942781));
#240861=CARTESIAN_POINT('Ctrl Pts',(-6.76997295430917,15.2,9.25373814402958));
#240862=CARTESIAN_POINT('Ctrl Pts',(-6.77330681482592,15.2,9.25552183562497));
#240863=CARTESIAN_POINT('Ctrl Pts',(-6.77664856080304,15.2,9.25730482727661));
#240864=CARTESIAN_POINT('Ctrl Pts',(-6.77999030678015,15.2,9.25908781892825));
#240865=CARTESIAN_POINT('Ctrl Pts',(-6.78333993605374,15.2,9.26087010917168));
#240866=CARTESIAN_POINT('Ctrl Pts',(-6.78669743619696,15.2,9.26265166624004));
#240867=CARTESIAN_POINT('Ctrl Pts',(-6.79229326997229,15.2,9.26562092812853));
#240868=CARTESIAN_POINT('Ctrl Pts',(-6.79791095410398,15.2,9.26858815135357));
#240869=CARTESIAN_POINT('Ctrl Pts',(-6.80355049700006,15.2,9.27155330199999));
#240870=CARTESIAN_POINT('Ctrl Pts',(-5.85257411500006,12.2,8.56667970999998));
#240871=CARTESIAN_POINT('Ctrl Pts',(-5.8537050266944,12.2,8.56806288496946));
#240872=CARTESIAN_POINT('Ctrl Pts',(-5.8548762742267,12.2,8.5694869238734));
#240873=CARTESIAN_POINT('Ctrl Pts',(-5.85608775334231,12.2,8.57095065186461));
#240874=CARTESIAN_POINT('Ctrl Pts',(-5.85730507482257,12.2,8.57242143869206));
#240875=CARTESIAN_POINT('Ctrl Pts',(-5.85856301277102,12.2,8.57393230486909));
#240876=CARTESIAN_POINT('Ctrl Pts',(-5.85986145340903,12.2,8.5754821088666));
#240877=CARTESIAN_POINT('Ctrl Pts',(-5.86115989392909,12.2,8.57703191272334));
#240878=CARTESIAN_POINT('Ctrl Pts',(-5.86249883775011,12.2,8.5786206548507));
#240879=CARTESIAN_POINT('Ctrl Pts',(-5.86387817019999,12.2,8.58024722870826));
#240880=CARTESIAN_POINT('Ctrl Pts',(-5.86525750264987,12.2,8.58187380256584));
#240881=CARTESIAN_POINT('Ctrl Pts',(-5.86667722397461,12.2,8.58353820930606));
#240882=CARTESIAN_POINT('Ctrl Pts',(-5.86813722065885,12.2,8.58523937157712));
#240883=CARTESIAN_POINT('Ctrl Pts',(-5.86959721747571,12.2,8.58694053400272));
#240884=CARTESIAN_POINT('Ctrl Pts',(-5.87109749092289,12.2,8.58867845508586));
#240885=CARTESIAN_POINT('Ctrl Pts',(-5.87263792542624,12.2,8.59045208743492));
#240886=CARTESIAN_POINT('Ctrl Pts',(-5.87417835978964,12.2,8.5922257196229));
#240887=CARTESIAN_POINT('Ctrl Pts',(-5.87575895551881,12.2,8.59403506540096));
#240888=CARTESIAN_POINT('Ctrl Pts',(-5.87737960096739,12.2,8.5958791057591));
#240889=CARTESIAN_POINT('Ctrl Pts',(-5.87900024641597,12.2,8.59772314611723));
#240890=CARTESIAN_POINT('Ctrl Pts',(-5.88066094034601,12.2,8.59960188503347));
#240891=CARTESIAN_POINT('Ctrl Pts',(-5.88236157069914,12.2,8.60151432962917));
#240892=CARTESIAN_POINT('Ctrl Pts',(-5.88406220120674,12.2,8.60342677439859));
#240893=CARTESIAN_POINT('Ctrl Pts',(-5.88580276684432,12.2,8.60537292884722));
#240894=CARTESIAN_POINT('Ctrl Pts',(-5.88758315544406,12.2,8.6073518267073));
#240895=CARTESIAN_POINT('Ctrl Pts',(-5.88936354388209,12.2,8.60933072438763));
#240896=CARTESIAN_POINT('Ctrl Pts',(-5.8911837544007,12.2,8.61134236845095));
#240897=CARTESIAN_POINT('Ctrl Pts',(-5.89304367483485,12.2,8.61338582004476));
#240898=CARTESIAN_POINT('Ctrl Pts',(-5.89490359526901,12.2,8.61542927163859));
#240899=CARTESIAN_POINT('Ctrl Pts',(-5.89680322566664,12.2,8.61750453153813));
#240900=CARTESIAN_POINT('Ctrl Pts',(-5.89874245209447,12.2,8.61961068537694));
#240901=CARTESIAN_POINT('Ctrl Pts',(-5.90068167852228,12.2,8.62171683921574));
#240902=CARTESIAN_POINT('Ctrl Pts',(-5.90266050315601,12.2,8.62385389007783));
#240903=CARTESIAN_POINT('Ctrl Pts',(-5.90467880958,12.2,8.62602094299706));
#240904=CARTESIAN_POINT('Ctrl Pts',(-5.90669711618733,12.2,8.62818799611313));
#240905=CARTESIAN_POINT('Ctrl Pts',(-5.90875490621511,12.2,8.63038505414048));
#240906=CARTESIAN_POINT('Ctrl Pts',(-5.91085206683112,12.2,8.63261124734639));
#240907=CARTESIAN_POINT('Ctrl Pts',(-5.91294922725662,12.2,8.63483744035008));
#240908=CARTESIAN_POINT('Ctrl Pts',(-5.91508575898494,12.2,8.6370927696049));
#240909=CARTESIAN_POINT('Ctrl Pts',(-5.917261545749,12.2,8.63937638753223));
#240910=CARTESIAN_POINT('Ctrl Pts',(-5.91943733251307,12.2,8.64166000545956));
#240911=CARTESIAN_POINT('Ctrl Pts',(-5.92165237917221,12.2,8.64397191098185));
#240912=CARTESIAN_POINT('Ctrl Pts',(-5.92390656675429,12.2,8.64631127722828));
#240913=CARTESIAN_POINT('Ctrl Pts',(-5.92616075454112,12.2,8.64865064368723));
#240914=CARTESIAN_POINT('Ctrl Pts',(-5.92845408727345,12.2,8.65101747241555));
#240915=CARTESIAN_POINT('Ctrl Pts',(-5.93078644981893,12.2,8.6534109538805));
#240916=CARTESIAN_POINT('Ctrl Pts',(-5.93311881215258,12.2,8.65580443512804));
#240917=CARTESIAN_POINT('Ctrl Pts',(-5.93549020490895,12.2,8.65822456958498));
#240918=CARTESIAN_POINT('Ctrl Pts',(-5.93790051249891,12.2,8.66067056875718));
#240919=CARTESIAN_POINT('Ctrl Pts',(-5.94031082008886,12.2,8.66311656792936));
#240920=CARTESIAN_POINT('Ctrl Pts',(-5.94276004699681,12.2,8.66558843074518));
#240921=CARTESIAN_POINT('Ctrl Pts',(-5.94524807348713,12.2,8.66808538523611));
#240922=CARTESIAN_POINT('Ctrl Pts',(-5.94773610020346,12.2,8.67058233995385));
#240923=CARTESIAN_POINT('Ctrl Pts',(-5.95026293231135,12.2,8.67310438872892));
#240924=CARTESIAN_POINT('Ctrl Pts',(-5.95282845024826,12.2,8.67565077649633));
#240925=CARTESIAN_POINT('Ctrl Pts',(-5.95539396795212,12.2,8.67819716403244));
#240926=CARTESIAN_POINT('Ctrl Pts',(-5.95799817570432,12.2,8.68076788892752));
#240927=CARTESIAN_POINT('Ctrl Pts',(-5.96064095702498,12.2,8.68336221549994));
#240928=CARTESIAN_POINT('Ctrl Pts',(-5.96328373834564,12.2,8.68595654207235));
#240929=CARTESIAN_POINT('Ctrl Pts',(-5.96596509279383,12.2,8.68857447029322));
#240930=CARTESIAN_POINT('Ctrl Pts',(-5.96868490824531,12.2,8.69121527799453));
#240931=CARTESIAN_POINT('Ctrl Pts',(-5.97140472394383,12.2,8.69385608593571));
#240932=CARTESIAN_POINT('Ctrl Pts',(-5.97416299909145,12.2,8.69651977286147));
#240933=CARTESIAN_POINT('Ctrl Pts',(-5.97695961882982,12.2,8.69920563384271));
#240934=CARTESIAN_POINT('Ctrl Pts',(-5.97975623831417,12.2,8.70189149457996));
#240935=CARTESIAN_POINT('Ctrl Pts',(-5.98259120274255,12.2,8.70459952736291));
#240936=CARTESIAN_POINT('Ctrl Pts',(-5.98546439798464,12.2,8.7073290440262));
#240937=CARTESIAN_POINT('Ctrl Pts',(-5.98833759322673,12.2,8.71005856068949));
#240938=CARTESIAN_POINT('Ctrl Pts',(-5.9912490184649,12.2,8.7128095585006));
#240939=CARTESIAN_POINT('Ctrl Pts',(-5.99419855785607,12.2,8.71558136139897));
#240940=CARTESIAN_POINT('Ctrl Pts',(-5.99665650743803,12.2,8.71789119723154));
#240941=CARTESIAN_POINT('Ctrl Pts',(-5.999140926204,12.2,8.72021548042008));
#240942=CARTESIAN_POINT('Ctrl Pts',(-6.00165174661927,12.2,8.72255382861377));
#240943=CARTESIAN_POINT('Ctrl Pts',(-6.00416256703455,12.2,8.72489217680747));
#240944=CARTESIAN_POINT('Ctrl Pts',(-6.00669978921481,12.2,8.7272445875713));
#240945=CARTESIAN_POINT('Ctrl Pts',(-6.00926334624026,12.2,8.72961068424866));
#240946=CARTESIAN_POINT('Ctrl Pts',(-6.0118269032657,12.2,8.73197678092602));
#240947=CARTESIAN_POINT('Ctrl Pts',(-6.01441679586664,12.2,8.73435656409993));
#240948=CARTESIAN_POINT('Ctrl Pts',(-6.01703295544998,12.2,8.73674966076662));
#240949=CARTESIAN_POINT('Ctrl Pts',(-6.01964911503334,12.2,8.7391427574333));
#240950=CARTESIAN_POINT('Ctrl Pts',(-6.02229154302258,12.2,8.74154916728469));
#240951=CARTESIAN_POINT('Ctrl Pts',(-6.02496017178478,12.2,8.74396852576794));
#240952=CARTESIAN_POINT('Ctrl Pts',(-6.02762880054697,12.2,8.74638788425118));
#240953=CARTESIAN_POINT('Ctrl Pts',(-6.03032362932119,12.2,8.74882019028705));
#240954=CARTESIAN_POINT('Ctrl Pts',(-6.03304459216976,12.2,8.75126508542659));
#240955=CARTESIAN_POINT('Ctrl Pts',(-6.03576555501833,12.2,8.75370998056613));
#240956=CARTESIAN_POINT('Ctrl Pts',(-6.03851265030239,12.2,8.75616746406093));
#240957=CARTESIAN_POINT('Ctrl Pts',(-6.04128581162318,12.2,8.75863718239488));
#240958=CARTESIAN_POINT('Ctrl Pts',(-6.04405897294397,12.2,8.76110690072884));
#240959=CARTESIAN_POINT('Ctrl Pts',(-6.04685820154622,12.2,8.76358885195297));
#240960=CARTESIAN_POINT('Ctrl Pts',(-6.04968342786972,12.2,8.76608269131449));
#240961=CARTESIAN_POINT('Ctrl Pts',(-6.05250865419322,12.2,8.768576530676));
#240962=CARTESIAN_POINT('Ctrl Pts',(-6.05535987785754,12.2,8.77108225413939));
#240963=CARTESIAN_POINT('Ctrl Pts',(-6.05823703390132,12.2,8.77359952261255));
#240964=CARTESIAN_POINT('Ctrl Pts',(-6.06111418994511,12.2,8.77611679108571));
#240965=CARTESIAN_POINT('Ctrl Pts',(-6.06401727443098,12.2,8.77864560073128));
#240966=CARTESIAN_POINT('Ctrl Pts',(-6.06694622234977,12.2,8.78118561760719));
#240967=CARTESIAN_POINT('Ctrl Pts',(-6.06987516994929,12.2,8.78372563420625));
#240968=CARTESIAN_POINT('Ctrl Pts',(-6.07282998071492,12.2,8.786276857245));
#240969=CARTESIAN_POINT('Ctrl Pts',(-6.07581058656847,12.2,8.7888389523815));
#240970=CARTESIAN_POINT('Ctrl Pts',(-6.07879119274691,12.2,8.79140104779728));
#240971=CARTESIAN_POINT('Ctrl Pts',(-6.08179759234439,12.2,8.7939740170629));
#240972=CARTESIAN_POINT('Ctrl Pts',(-6.08482972012007,12.2,8.79655753164537));
#240973=CARTESIAN_POINT('Ctrl Pts',(-6.08786184789574,12.2,8.79914104622784));
#240974=CARTESIAN_POINT('Ctrl Pts',(-6.0909197017099,12.2,8.80173510663794));
#240975=CARTESIAN_POINT('Ctrl Pts',(-6.09400321309667,12.2,8.80433939115098));
#240976=CARTESIAN_POINT('Ctrl Pts',(-6.09708672448344,12.2,8.80694367566402));
#240977=CARTESIAN_POINT('Ctrl Pts',(-6.10019589624247,12.2,8.80955818307048));
#240978=CARTESIAN_POINT('Ctrl Pts',(-6.10333065611952,12.2,8.81218259618701));
#240979=CARTESIAN_POINT('Ctrl Pts',(-6.10646541599657,12.2,8.81480700930354));
#240980=CARTESIAN_POINT('Ctrl Pts',(-6.10962576757645,12.2,8.8174413284776));
#240981=CARTESIAN_POINT('Ctrl Pts',(-6.11281163882513,12.2,8.82008524056044));
#240982=CARTESIAN_POINT('Ctrl Pts',(-6.11599751007381,12.2,8.82272915264328));
#240983=CARTESIAN_POINT('Ctrl Pts',(-6.11920890416203,12.2,8.82538265730971));
#240984=CARTESIAN_POINT('Ctrl Pts',(-6.12244574881345,12.2,8.8280454460592));
#240985=CARTESIAN_POINT('Ctrl Pts',(-6.12503522467571,12.2,8.8301756771749));
#240986=CARTESIAN_POINT('Ctrl Pts',(-6.1276409911997,12.2,8.8323118506449));
#240987=CARTESIAN_POINT('Ctrl Pts',(-6.13026301236389,12.2,8.83445381003581));
#240988=CARTESIAN_POINT('Ctrl Pts',(-6.13288503317083,12.2,8.83659576913488));
#240989=CARTESIAN_POINT('Ctrl Pts',(-6.13552330723175,12.2,8.83874351511705));
#240990=CARTESIAN_POINT('Ctrl Pts',(-6.13817780129148,12.2,8.84089689260732));
#240991=CARTESIAN_POINT('Ctrl Pts',(-6.14149591913739,12.2,8.84358861469019));
#240992=CARTESIAN_POINT('Ctrl Pts',(-6.14483937943672,12.2,8.84628913648997));
#240993=CARTESIAN_POINT('Ctrl Pts',(-6.1482081130465,12.2,8.84899816128117));
#240994=CARTESIAN_POINT('Ctrl Pts',(-6.15090310008119,12.2,8.85116538123226));
#240995=CARTESIAN_POINT('Ctrl Pts',(-6.15361426206229,12.2,8.85333804315749));
#240996=CARTESIAN_POINT('Ctrl Pts',(-6.15634156340415,12.2,8.85551599710769));
#240997=CARTESIAN_POINT('Ctrl Pts',(-6.15906886437442,12.2,8.85769395076114));
#240998=CARTESIAN_POINT('Ctrl Pts',(-6.16181230541788,12.2,8.85987719535591));
#240999=CARTESIAN_POINT('Ctrl Pts',(-6.16457184952455,12.2,8.86206558362111));
#241000=CARTESIAN_POINT('Ctrl Pts',(-6.16733139400721,12.2,8.86425397218447));
#241001=CARTESIAN_POINT('Ctrl Pts',(-6.17010704317239,12.2,8.86644750392904));
#241002=CARTESIAN_POINT('Ctrl Pts',(-6.1728987609367,12.2,8.86864603243807));
#241003=CARTESIAN_POINT('Ctrl Pts',(-6.17569047832064,12.2,8.87084456064756));
#241004=CARTESIAN_POINT('Ctrl Pts',(-6.17849826341207,12.2,8.87304808432517));
#241005=CARTESIAN_POINT('Ctrl Pts',(-6.18132208159866,12.2,8.87525645942121));
#241006=CARTESIAN_POINT('Ctrl Pts',(-6.18485185462046,12.2,8.87801692851691));
#241007=CARTESIAN_POINT('Ctrl Pts',(-6.18840667958956,12.2,8.88078497676334));
#241008=CARTESIAN_POINT('Ctrl Pts',(-6.19198648653269,12.2,8.8835603248185));
#241009=CARTESIAN_POINT('Ctrl Pts',(-6.19485033224328,12.2,8.88578060338364));
#241010=CARTESIAN_POINT('Ctrl Pts',(-6.19773016514467,12.2,8.88800555423823));
#241011=CARTESIAN_POINT('Ctrl Pts',(-6.20062595097021,12.2,8.89023503424894));
#241012=CARTESIAN_POINT('Ctrl Pts',(-6.20352173640121,12.2,8.89246451395588));
#241013=CARTESIAN_POINT('Ctrl Pts',(-6.20643347491972,12.2,8.89469852319395));
#241014=CARTESIAN_POINT('Ctrl Pts',(-6.20936112982526,12.2,8.89693692240018));
#241015=CARTESIAN_POINT('Ctrl Pts',(-6.21228878512968,12.2,8.8991753219114));
#241016=CARTESIAN_POINT('Ctrl Pts',(-6.21523235733809,12.2,8.90141811162485));
#241017=CARTESIAN_POINT('Ctrl Pts',(-6.21819181100042,12.2,8.90366515169204));
#241018=CARTESIAN_POINT('Ctrl Pts',(-6.22115126425952,12.2,8.90591219145307));
#241019=CARTESIAN_POINT('Ctrl Pts',(-6.22412659708769,12.2,8.90816348294659));
#241020=CARTESIAN_POINT('Ctrl Pts',(-6.22711777578594,12.2,8.91041888737288));
#241021=CARTESIAN_POINT('Ctrl Pts',(-6.23010895489176,12.2,8.91267429210646));
#241022=CARTESIAN_POINT('Ctrl Pts',(-6.23311597888741,12.2,8.91493380993174));
#241023=CARTESIAN_POINT('Ctrl Pts',(-6.23613881201039,12.2,8.91719730600985));
#241024=CARTESIAN_POINT('Ctrl Pts',(-6.23916164472152,12.2,8.91946080177955));
#241025=CARTESIAN_POINT('Ctrl Pts',(-6.24220028693525,12.2,8.92172827530357));
#241026=CARTESIAN_POINT('Ctrl Pts',(-6.24525470168394,12.2,8.92399959289528));
#241027=CARTESIAN_POINT('Ctrl Pts',(-6.24830911684879,12.2,8.92627091079644));
#241028=CARTESIAN_POINT('Ctrl Pts',(-6.25137930531514,12.2,8.92854607119243));
#241029=CARTESIAN_POINT('Ctrl Pts',(-6.25446523048333,12.2,8.93082494198331));
#241030=CARTESIAN_POINT('Ctrl Pts',(-6.25755115565152,12.2,8.93310381277419));
#241031=CARTESIAN_POINT('Ctrl Pts',(-6.26065281821597,12.2,8.93538639513491));
#241032=CARTESIAN_POINT('Ctrl Pts',(-6.26377018127636,12.2,8.93767255464877));
#241033=CARTESIAN_POINT('Ctrl Pts',(-6.26688754391201,12.2,8.93995871385113));
#241034=CARTESIAN_POINT('Ctrl Pts',(-6.27002060762435,12.2,8.94224845165325));
#241035=CARTESIAN_POINT('Ctrl Pts',(-6.27316933571452,12.2,8.9445416386984));
#241036=CARTESIAN_POINT('Ctrl Pts',(-6.27710524614898,12.2,8.94740812273918));
#241037=CARTESIAN_POINT('Ctrl Pts',(-6.28106563330555,12.2,8.9502799938222));
#241038=CARTESIAN_POINT('Ctrl Pts',(-6.28505042524998,12.2,8.95315700201663));
#241039=CARTESIAN_POINT('Ctrl Pts',(-6.28823825897927,12.2,8.95545860869762));
#241040=CARTESIAN_POINT('Ctrl Pts',(-6.29144171166596,12.2,8.95776350188735));
#241041=CARTESIAN_POINT('Ctrl Pts',(-6.29466074750965,12.2,8.96007155540234));
#241042=CARTESIAN_POINT('Ctrl Pts',(-6.29787978291474,12.2,8.96237960860286));
#241043=CARTESIAN_POINT('Ctrl Pts',(-6.30111440152655,12.2,8.96469082122153));
#241044=CARTESIAN_POINT('Ctrl Pts',(-6.30436456749779,12.2,8.96700506826507));
#241045=CARTESIAN_POINT('Ctrl Pts',(-6.30761473391185,12.2,8.96931931562392));
#241046=CARTESIAN_POINT('Ctrl Pts',(-6.3108804460394,12.2,8.97163659577479));
#241047=CARTESIAN_POINT('Ctrl Pts',(-6.31416166855315,12.2,8.973956785346));
#241048=CARTESIAN_POINT('Ctrl Pts',(-6.31744289061984,12.2,8.97627697460106));
#241049=CARTESIAN_POINT('Ctrl Pts',(-6.32073962418448,12.2,8.97860007301685));
#241050=CARTESIAN_POINT('Ctrl Pts',(-6.32405183024604,12.2,8.98092595682653));
#241051=CARTESIAN_POINT('Ctrl Pts',(-6.32819208816146,12.2,8.98383331182631));
#241052=CARTESIAN_POINT('Ctrl Pts',(-6.33235652492191,12.2,8.98674501776507));
#241053=CARTESIAN_POINT('Ctrl Pts',(-6.33654506776788,12.2,8.98966083700097));
#241054=CARTESIAN_POINT('Ctrl Pts',(-6.33989590222727,12.2,8.99199349251682));
#241055=CARTESIAN_POINT('Ctrl Pts',(-6.34326216468622,12.2,8.99432878125592));
#241056=CARTESIAN_POINT('Ctrl Pts',(-6.34664381870745,12.2,8.99666658038923));
#241057=CARTESIAN_POINT('Ctrl Pts',(-6.35002547226794,12.2,8.999004379204));
#241058=CARTESIAN_POINT('Ctrl Pts',(-6.35342251877061,12.2,9.00134469013906));
#241059=CARTESIAN_POINT('Ctrl Pts',(-6.35683491821284,12.2,9.00368739205848));
#241060=CARTESIAN_POINT('Ctrl Pts',(-6.36024731812,12.2,9.00603009429709));
#241061=CARTESIAN_POINT('Ctrl Pts',(-6.36367507370687,12.2,9.00837518923882));
#241062=CARTESIAN_POINT('Ctrl Pts',(-6.36711814750661,12.2,9.01072255620022));
#241063=CARTESIAN_POINT('Ctrl Pts',(-6.37056122083724,12.2,9.0130699228418));
#241064=CARTESIAN_POINT('Ctrl Pts',(-6.37401961178556,12.2,9.01541956307257));
#241065=CARTESIAN_POINT('Ctrl Pts',(-6.37749328522935,12.2,9.01777135844206));
#241066=CARTESIAN_POINT('Ctrl Pts',(-6.38183537738905,12.2,9.02071110289423));
#241067=CARTESIAN_POINT('Ctrl Pts',(-6.38620134575318,12.2,9.02365421482414));
#241068=CARTESIAN_POINT('Ctrl Pts',(-6.39059112019638,12.2,9.02660046753231));
#241069=CARTESIAN_POINT('Ctrl Pts',(-6.39410293994233,12.2,9.0289574698273));
#241070=CARTESIAN_POINT('Ctrl Pts',(-6.3976299954068,12.2,9.03131648287255));
#241071=CARTESIAN_POINT('Ctrl Pts',(-6.40117224982306,12.2,9.03367739050134));
#241072=CARTESIAN_POINT('Ctrl Pts',(-6.40471450375669,12.2,9.03603829780846));
#241073=CARTESIAN_POINT('Ctrl Pts',(-6.40827195387436,12.2,9.03840110095998));
#241074=CARTESIAN_POINT('Ctrl Pts',(-6.41184456798166,12.2,9.0407656844402));
#241075=CARTESIAN_POINT('Ctrl Pts',(-6.41631033598086,12.2,9.0437214140321));
#241076=CARTESIAN_POINT('Ctrl Pts',(-6.42079979358398,12.2,9.04667992758424));
#241077=CARTESIAN_POINT('Ctrl Pts',(-6.42531286892999,12.2,9.04964100355634));
#241078=CARTESIAN_POINT('Ctrl Pts',(-6.42892332940356,12.2,9.05200986446312));
#241079=CARTESIAN_POINT('Ctrl Pts',(-6.4325489052817,12.2,9.05438036537844));
#241080=CARTESIAN_POINT('Ctrl Pts',(-6.43618955981443,12.2,9.05675239445224));
#241081=CARTESIAN_POINT('Ctrl Pts',(-6.43983021385112,12.2,9.05912442320287));
#241082=CARTESIAN_POINT('Ctrl Pts',(-6.44348594688266,12.2,9.06149798139209));
#241083=CARTESIAN_POINT('Ctrl Pts',(-6.44715672104243,12.2,9.06387295687203));
#241084=CARTESIAN_POINT('Ctrl Pts',(-6.45082749570234,12.2,9.06624793267555));
#241085=CARTESIAN_POINT('Ctrl Pts',(-6.4545133114,12.2,9.06862432851192));
#241086=CARTESIAN_POINT('Ctrl Pts',(-6.45821413126935,12.2,9.07100203091937));
#241087=CARTESIAN_POINT('Ctrl Pts',(-6.46191495063446,12.2,9.07337973300286));
#241088=CARTESIAN_POINT('Ctrl Pts',(-6.46563077588266,12.2,9.07575874341663));
#241089=CARTESIAN_POINT('Ctrl Pts',(-6.46936156663168,12.2,9.07813895411081));
#241090=CARTESIAN_POINT('Ctrl Pts',(-6.47309235788902,12.2,9.08051916512929));
#241091=CARTESIAN_POINT('Ctrl Pts',(-6.47683811763048,12.2,9.08290057602204));
#241092=CARTESIAN_POINT('Ctrl Pts',(-6.48059880551923,12.2,9.0852830790516));
#241093=CARTESIAN_POINT('Ctrl Pts',(-6.48341932117959,12.2,9.08706995616146));
#241094=CARTESIAN_POINT('Ctrl Pts',(-6.48624823573766,12.2,9.08885744752187));
#241095=CARTESIAN_POINT('Ctrl Pts',(-6.48908553277242,12.2,9.09064550821503));
#241096=CARTESIAN_POINT('Ctrl Pts',(-6.49192282980717,12.2,9.09243356890818));
#241097=CARTESIAN_POINT('Ctrl Pts',(-6.49476850814347,12.2,9.09422219987002));
#241098=CARTESIAN_POINT('Ctrl Pts',(-6.49762255374738,12.2,9.09601135451331));
#241099=CARTESIAN_POINT('Ctrl Pts',(-6.50047659935128,12.2,9.09780050915658));
#241100=CARTESIAN_POINT('Ctrl Pts',(-6.50333901166296,12.2,9.09959018835817));
#241101=CARTESIAN_POINT('Ctrl Pts',(-6.50620977434918,12.2,9.10138034883473));
#241102=CARTESIAN_POINT('Ctrl Pts',(-6.50908053755692,12.2,9.10317050963649));
#241103=CARTESIAN_POINT('Ctrl Pts',(-6.51195965244202,12.2,9.10496114953008));
#241104=CARTESIAN_POINT('Ctrl Pts',(-6.51484710165447,12.2,9.10675222591543));
#241105=CARTESIAN_POINT('Ctrl Pts',(-6.51773455034236,12.2,9.10854330197542));
#241106=CARTESIAN_POINT('Ctrl Pts',(-6.52063033495474,12.2,9.11033481415555));
#241107=CARTESIAN_POINT('Ctrl Pts',(-6.52353443828695,12.2,9.11212671838834));
#241108=CARTESIAN_POINT('Ctrl Pts',(-6.52643854161916,12.2,9.11391862262114));
#241109=CARTESIAN_POINT('Ctrl Pts',(-6.52935096497388,12.2,9.11571091906048));
#241110=CARTESIAN_POINT('Ctrl Pts',(-6.53227169107683,12.2,9.11750356420372));
#241111=CARTESIAN_POINT('Ctrl Pts',(-6.53519241717978,12.2,9.11929620934696));
#241112=CARTESIAN_POINT('Ctrl Pts',(-6.53812144647338,12.2,9.12108920284848));
#241113=CARTESIAN_POINT('Ctrl Pts',(-6.54105876403333,12.2,9.12288250199165));
#241114=CARTESIAN_POINT('Ctrl Pts',(-6.54399608159328,12.2,9.12467580113483));
#241115=CARTESIAN_POINT('Ctrl Pts',(-6.54694168686957,12.2,9.12646940566967));
#241116=CARTESIAN_POINT('Ctrl Pts',(-6.54989556396983,12.2,9.12826327277112));
#241117=CARTESIAN_POINT('Ctrl Pts',(-6.55284944107009,12.2,9.13005713987257));
#241118=CARTESIAN_POINT('Ctrl Pts',(-6.55581158960254,12.2,9.13185126901174));
#241119=CARTESIAN_POINT('Ctrl Pts',(-6.55878199443371,12.2,9.13364561816116));
#241120=CARTESIAN_POINT('Ctrl Pts',(-6.56175239926489,12.2,9.13543996731057));
#241121=CARTESIAN_POINT('Ctrl Pts',(-6.56473106165852,12.2,9.1372345350573));
#241122=CARTESIAN_POINT('Ctrl Pts',(-6.56771796238219,12.2,9.13902928111706));
#241123=CARTESIAN_POINT('Ctrl Pts',(-6.57070486364848,12.2,9.14082402750287));
#241124=CARTESIAN_POINT('Ctrl Pts',(-6.5737000059838,12.2,9.14261895043041));
#241125=CARTESIAN_POINT('Ctrl Pts',(-6.57670337217141,12.2,9.14441400889964));
#241126=CARTESIAN_POINT('Ctrl Pts',(-6.57970673781341,12.2,9.14620906704277));
#241127=CARTESIAN_POINT('Ctrl Pts',(-6.58271832773829,12.2,9.14800426054422));
#241128=CARTESIAN_POINT('Ctrl Pts',(-6.58573812633763,12.2,9.14979954668734));
#241129=CARTESIAN_POINT('Ctrl Pts',(-6.58875792493697,12.2,9.15159483283046));
#241130=CARTESIAN_POINT('Ctrl Pts',(-6.59178593243258,12.2,9.15339021140869));
#241131=CARTESIAN_POINT('Ctrl Pts',(-6.59482213204442,12.2,9.15518564251828));
#241132=CARTESIAN_POINT('Ctrl Pts',(-6.59887039800967,12.2,9.15757955055568));
#241133=CARTESIAN_POINT('Ctrl Pts',(-6.60293322881538,12.2,9.15997355057371));
#241134=CARTESIAN_POINT('Ctrl Pts',(-6.60701058609168,12.2,9.16236754343356));
#241135=CARTESIAN_POINT('Ctrl Pts',(-6.61006860474332,12.2,9.16416303848616));
#241136=CARTESIAN_POINT('Ctrl Pts',(-6.61313479453896,12.2,9.16595853006379));
#241137=CARTESIAN_POINT('Ctrl Pts',(-6.61620913969521,12.2,9.16775397711639));
#241138=CARTESIAN_POINT('Ctrl Pts',(-6.61928348429296,12.2,9.16954942384282));
#241139=CARTESIAN_POINT('Ctrl Pts',(-6.62236598456526,12.2,9.17134482622757));
#241140=CARTESIAN_POINT('Ctrl Pts',(-6.62545662462036,12.2,9.17314014295401));
#241141=CARTESIAN_POINT('Ctrl Pts',(-6.62854726467546,12.2,9.17493545968046));
#241142=CARTESIAN_POINT('Ctrl Pts',(-6.63164604319621,12.2,9.17673069149854));
#241143=CARTESIAN_POINT('Ctrl Pts',(-6.63475294620833,12.2,9.17852579722499));
#241144=CARTESIAN_POINT('Ctrl Pts',(-6.63785984922046,12.2,9.18032090295143));
#241145=CARTESIAN_POINT('Ctrl Pts',(-6.64097487487391,12.2,9.18211588333622));
#241146=CARTESIAN_POINT('Ctrl Pts',(-6.64409800892637,12.2,9.18391069706268));
#241147=CARTESIAN_POINT('Ctrl Pts',(-6.64722114297884,12.2,9.18570551078914));
#241148=CARTESIAN_POINT('Ctrl Pts',(-6.65035238486753,12.2,9.187500158895));
#241149=CARTESIAN_POINT('Ctrl Pts',(-6.65349171811769,12.2,9.18929460116947));
#241150=CARTESIAN_POINT('Ctrl Pts',(-6.65663105136784,12.2,9.19108904344393));
#241151=CARTESIAN_POINT('Ctrl Pts',(-6.65977847524454,12.2,9.19288327942405));
#241152=CARTESIAN_POINT('Ctrl Pts',(-6.66293397575377,12.2,9.1946772696089));
#241153=CARTESIAN_POINT('Ctrl Pts',(-6.66608947683624,12.2,9.19647126011965));
#241154=CARTESIAN_POINT('Ctrl Pts',(-6.66925305362937,12.2,9.19826500438034));
#241155=CARTESIAN_POINT('Ctrl Pts',(-6.67242468971642,12.2,9.20005846389096));
#241156=CARTESIAN_POINT('Ctrl Pts',(-6.67559632522729,12.2,9.20185192307577));
#241157=CARTESIAN_POINT('Ctrl Pts',(-6.67877601927939,12.2,9.20364509692724));
#241158=CARTESIAN_POINT('Ctrl Pts',(-6.6819637578726,12.2,9.20543794619541));
#241159=CARTESIAN_POINT('Ctrl Pts',(-6.68515149646582,12.2,9.20723079546358));
#241160=CARTESIAN_POINT('Ctrl Pts',(-6.6883472793714,12.2,9.20902332097526));
#241161=CARTESIAN_POINT('Ctrl Pts',(-6.69155108897791,12.2,9.21081548270995));
#241162=CARTESIAN_POINT('Ctrl Pts',(-6.69475489858442,12.2,9.21260764444464));
#241163=CARTESIAN_POINT('Ctrl Pts',(-6.6979667357828,12.2,9.21439944307197));
#241164=CARTESIAN_POINT('Ctrl Pts',(-6.70118658480542,12.2,9.21619083876503));
#241165=CARTESIAN_POINT('Ctrl Pts',(-6.70440643382803,12.2,9.21798223445809));
#241166=CARTESIAN_POINT('Ctrl Pts',(-6.70763429324903,12.2,9.21977322685317));
#241167=CARTESIAN_POINT('Ctrl Pts',(-6.71087014838076,12.2,9.22156377953815));
#241168=CARTESIAN_POINT('Ctrl Pts',(-6.71410600351248,12.2,9.22335433222312));
#241169=CARTESIAN_POINT('Ctrl Pts',(-6.71734985492702,12.2,9.22514444437481));
#241170=CARTESIAN_POINT('Ctrl Pts',(-6.72060168505778,12.2,9.22693407764318));
#241171=CARTESIAN_POINT('Ctrl Pts',(-6.72493745895928,12.2,9.22932025555108));
#241172=CARTESIAN_POINT('Ctrl Pts',(-6.72928742038135,12.2,9.23170558359416));
#241173=CARTESIAN_POINT('Ctrl Pts',(-6.73365152769465,12.2,9.23408996873495));
#241174=CARTESIAN_POINT('Ctrl Pts',(-6.73692460788232,12.2,9.23587825742811));
#241175=CARTESIAN_POINT('Ctrl Pts',(-6.74020564685162,12.2,9.23766601558852));
#241176=CARTESIAN_POINT('Ctrl Pts',(-6.74349462549701,12.2,9.23945320524003));
#241177=CARTESIAN_POINT('Ctrl Pts',(-6.74678360414241,12.2,9.24124039489155));
#241178=CARTESIAN_POINT('Ctrl Pts',(-6.75008052382735,12.2,9.24302701408682));
#241179=CARTESIAN_POINT('Ctrl Pts',(-6.75338537087324,12.2,9.24481303131363));
#241180=CARTESIAN_POINT('Ctrl Pts',(-6.75669021791912,12.2,9.24659904854046));
#241181=CARTESIAN_POINT('Ctrl Pts',(-6.76000299123116,12.2,9.24838446287566));
#241182=CARTESIAN_POINT('Ctrl Pts',(-6.7633236757761,12.2,9.25016923810258));
#241183=CARTESIAN_POINT('Ctrl Pts',(-6.76664436092431,12.2,9.25195401365372));
#241184=CARTESIAN_POINT('Ctrl Pts',(-6.76997295680805,12.2,9.25373815099635));
#241185=CARTESIAN_POINT('Ctrl Pts',(-6.77330944441903,12.2,9.25552160438045));
#241186=CARTESIAN_POINT('Ctrl Pts',(-6.77775809355678,12.2,9.25789954168592));
#241187=CARTESIAN_POINT('Ctrl Pts',(-6.78222076954265,12.2,9.26027625692344));
#241188=CARTESIAN_POINT('Ctrl Pts',(-6.78669743619696,12.2,9.26265166624004));
#241189=CARTESIAN_POINT('Ctrl Pts',(-6.79229326997229,12.2,9.26562092812853));
#241190=CARTESIAN_POINT('Ctrl Pts',(-6.79791095410398,12.2,9.26858815135357));
#241191=CARTESIAN_POINT('Ctrl Pts',(-6.80355049700006,12.2,9.27155330199999));
#241192=CARTESIAN_POINT('Ctrl Pts',(-7.10901226900006,15.2,9.03946594399999));
#241193=CARTESIAN_POINT('Ctrl Pts',(-7.10901226900006,11.6,9.03946594399999));
#241194=CARTESIAN_POINT('Ctrl Pts',(-7.10885083700005,15.2,9.03871859599998));
#241195=CARTESIAN_POINT('Ctrl Pts',(-7.10885083700005,11.6,9.03871859599998));
#241196=CARTESIAN_POINT('Ctrl Pts',(-7.10852778500006,15.2,9.03722439199999));
#241197=CARTESIAN_POINT('Ctrl Pts',(-7.10852778500006,11.6,9.03722439199999));
#241198=CARTESIAN_POINT('Ctrl Pts',(-7.10804264000005,15.2,9.03498456099998));
#241199=CARTESIAN_POINT('Ctrl Pts',(-7.10804264000005,11.6,9.03498456099998));
#241200=CARTESIAN_POINT('Ctrl Pts',(-7.10739465200006,15.2,9.03200107199999));
#241201=CARTESIAN_POINT('Ctrl Pts',(-7.10739465200006,11.6,9.03200107199999));
#241202=CARTESIAN_POINT('Ctrl Pts',(-7.10658278400006,15.2,9.02827662999999));
#241203=CARTESIAN_POINT('Ctrl Pts',(-7.10658278400006,11.6,9.02827662999999));
#241204=CARTESIAN_POINT('Ctrl Pts',(-7.10576903600006,15.2,9.02455710699999));
#241205=CARTESIAN_POINT('Ctrl Pts',(-7.10576903600006,11.6,9.02455710699999));
#241206=CARTESIAN_POINT('Ctrl Pts',(-7.10495340800006,15.2,9.02084250499998));
#241207=CARTESIAN_POINT('Ctrl Pts',(-7.10495340800006,11.6,9.02084250499998));
#241208=CARTESIAN_POINT('Ctrl Pts',(-7.10413590500006,15.2,9.01713282899999));
#241209=CARTESIAN_POINT('Ctrl Pts',(-7.10413590500006,11.6,9.01713282899999));
#241210=CARTESIAN_POINT('Ctrl Pts',(-7.10331652900006,15.2,9.01342808099999));
#241211=CARTESIAN_POINT('Ctrl Pts',(-7.10331652900006,11.6,9.01342808099999));
#241212=CARTESIAN_POINT('Ctrl Pts',(-7.10249528700006,15.2,9.00972826399999));
#241213=CARTESIAN_POINT('Ctrl Pts',(-7.10249528700006,11.6,9.00972826399999));
#241214=CARTESIAN_POINT('Ctrl Pts',(-7.10167218800006,15.2,9.00603338899998));
#241215=CARTESIAN_POINT('Ctrl Pts',(-7.10167218800006,11.6,9.00603338899998));
#241216=CARTESIAN_POINT('Ctrl Pts',(-7.10084724000006,15.2,9.00234345799999));
#241217=CARTESIAN_POINT('Ctrl Pts',(-7.10084724000006,11.6,9.00234345799999));
#241218=CARTESIAN_POINT('Ctrl Pts',(-7.10002045000006,15.2,8.99865848199998));
#241219=CARTESIAN_POINT('Ctrl Pts',(-7.10002045000006,11.6,8.99865848199998));
#241220=CARTESIAN_POINT('Ctrl Pts',(-7.09919183000006,15.2,8.99497846599999));
#241221=CARTESIAN_POINT('Ctrl Pts',(-7.09919183000006,11.6,8.99497846599999));
#241222=CARTESIAN_POINT('Ctrl Pts',(-7.09836138500005,15.2,8.99130341599999));
#241223=CARTESIAN_POINT('Ctrl Pts',(-7.09836138500005,11.6,8.99130341599999));
#241224=CARTESIAN_POINT('Ctrl Pts',(-7.09752912300006,15.2,8.98763333899998));
#241225=CARTESIAN_POINT('Ctrl Pts',(-7.09752912300006,11.6,8.98763333899998));
#241226=CARTESIAN_POINT('Ctrl Pts',(-7.09669505100006,15.2,8.98396823999999));
#241227=CARTESIAN_POINT('Ctrl Pts',(-7.09669505100006,11.6,8.98396823999999));
#241228=CARTESIAN_POINT('Ctrl Pts',(-7.09585917500006,15.2,8.98030812399998));
#241229=CARTESIAN_POINT('Ctrl Pts',(-7.09585917500006,11.6,8.98030812399998));
#241230=CARTESIAN_POINT('Ctrl Pts',(-7.09502150300006,15.2,8.97665299599998));
#241231=CARTESIAN_POINT('Ctrl Pts',(-7.09502150300006,11.6,8.97665299599998));
#241232=CARTESIAN_POINT('Ctrl Pts',(-7.09418204000006,15.2,8.97300286299998));
#241233=CARTESIAN_POINT('Ctrl Pts',(-7.09418204000006,11.6,8.97300286299998));
#241234=CARTESIAN_POINT('Ctrl Pts',(-7.09334079200006,15.2,8.96935772799999));
#241235=CARTESIAN_POINT('Ctrl Pts',(-7.09334079200006,11.6,8.96935772799999));
#241236=CARTESIAN_POINT('Ctrl Pts',(-7.09249776700006,15.2,8.96571759799999));
#241237=CARTESIAN_POINT('Ctrl Pts',(-7.09249776700006,11.6,8.96571759799999));
#241238=CARTESIAN_POINT('Ctrl Pts',(-7.09165297300006,15.2,8.96208247799999));
#241239=CARTESIAN_POINT('Ctrl Pts',(-7.09165297300006,11.6,8.96208247799999));
#241240=CARTESIAN_POINT('Ctrl Pts',(-7.09080641500006,15.2,8.95845237299999));
#241241=CARTESIAN_POINT('Ctrl Pts',(-7.09080641500006,11.6,8.95845237299999));
#241242=CARTESIAN_POINT('Ctrl Pts',(-7.08995810300006,15.2,8.95482729199998));
#241243=CARTESIAN_POINT('Ctrl Pts',(-7.08995810300006,11.6,8.95482729199998));
#241244=CARTESIAN_POINT('Ctrl Pts',(-7.08910804400006,15.2,8.95120723899998));
#241245=CARTESIAN_POINT('Ctrl Pts',(-7.08910804400006,11.6,8.95120723899998));
#241246=CARTESIAN_POINT('Ctrl Pts',(-7.08825624400006,15.2,8.94759221899999));
#241247=CARTESIAN_POINT('Ctrl Pts',(-7.08825624400006,11.6,8.94759221899999));
#241248=CARTESIAN_POINT('Ctrl Pts',(-7.08740271100006,15.2,8.94398223899999));
#241249=CARTESIAN_POINT('Ctrl Pts',(-7.08740271100006,11.6,8.94398223899999));
#241250=CARTESIAN_POINT('Ctrl Pts',(-7.08654745300006,15.2,8.94037730399998));
#241251=CARTESIAN_POINT('Ctrl Pts',(-7.08654745300006,11.6,8.94037730399998));
#241252=CARTESIAN_POINT('Ctrl Pts',(-7.08569047500006,15.2,8.93677742099998));
#241253=CARTESIAN_POINT('Ctrl Pts',(-7.08569047500006,11.6,8.93677742099998));
#241254=CARTESIAN_POINT('Ctrl Pts',(-7.08483178600006,15.2,8.93318259399998));
#241255=CARTESIAN_POINT('Ctrl Pts',(-7.08483178600006,11.6,8.93318259399998));
#241256=CARTESIAN_POINT('Ctrl Pts',(-7.08397139200006,15.2,8.92959282899999));
#241257=CARTESIAN_POINT('Ctrl Pts',(-7.08397139200006,11.6,8.92959282899999));
#241258=CARTESIAN_POINT('Ctrl Pts',(-7.08310930200006,15.2,8.92600813199999));
#241259=CARTESIAN_POINT('Ctrl Pts',(-7.08310930200006,11.6,8.92600813199999));
#241260=CARTESIAN_POINT('Ctrl Pts',(-7.08224552200006,15.2,8.92242850899999));
#241261=CARTESIAN_POINT('Ctrl Pts',(-7.08224552200006,11.6,8.92242850899999));
#241262=CARTESIAN_POINT('Ctrl Pts',(-7.08138005900006,15.2,8.91885396399999));
#241263=CARTESIAN_POINT('Ctrl Pts',(-7.08138005900006,11.6,8.91885396399999));
#241264=CARTESIAN_POINT('Ctrl Pts',(-7.08051292100006,15.2,8.91528450599999));
#241265=CARTESIAN_POINT('Ctrl Pts',(-7.08051292100006,11.6,8.91528450599999));
#241266=CARTESIAN_POINT('Ctrl Pts',(-7.07964411500006,15.2,8.91172013699999));
#241267=CARTESIAN_POINT('Ctrl Pts',(-7.07964411500006,11.6,8.91172013699999));
#241268=CARTESIAN_POINT('Ctrl Pts',(-7.07877364900006,15.2,8.90816086699999));
#241269=CARTESIAN_POINT('Ctrl Pts',(-7.07877364900006,11.6,8.90816086699999));
#241270=CARTESIAN_POINT('Ctrl Pts',(-7.07790153000006,15.2,8.90460669799998));
#241271=CARTESIAN_POINT('Ctrl Pts',(-7.07790153000006,11.6,8.90460669799998));
#241272=CARTESIAN_POINT('Ctrl Pts',(-7.07702776600006,15.2,8.90105763799999));
#241273=CARTESIAN_POINT('Ctrl Pts',(-7.07702776600006,11.6,8.90105763799999));
#241274=CARTESIAN_POINT('Ctrl Pts',(-7.07615236300006,15.2,8.89751369099999));
#241275=CARTESIAN_POINT('Ctrl Pts',(-7.07615236300006,11.6,8.89751369099999));
#241276=CARTESIAN_POINT('Ctrl Pts',(-7.07527533000006,15.2,8.89397486499998));
#241277=CARTESIAN_POINT('Ctrl Pts',(-7.07527533000006,11.6,8.89397486499998));
#241278=CARTESIAN_POINT('Ctrl Pts',(-7.07439667400006,15.2,8.89044116499999));
#241279=CARTESIAN_POINT('Ctrl Pts',(-7.07439667400006,11.6,8.89044116499999));
#241280=CARTESIAN_POINT('Ctrl Pts',(-7.07351640200006,15.2,8.88691259499998));
#241281=CARTESIAN_POINT('Ctrl Pts',(-7.07351640200006,11.6,8.88691259499998));
#241282=CARTESIAN_POINT('Ctrl Pts',(-7.07263452200006,15.2,8.88338916299999));
#241283=CARTESIAN_POINT('Ctrl Pts',(-7.07263452200006,11.6,8.88338916299999));
#241284=CARTESIAN_POINT('Ctrl Pts',(-7.07175104100005,15.2,8.87987087299998));
#241285=CARTESIAN_POINT('Ctrl Pts',(-7.07175104100005,11.6,8.87987087299998));
#241286=CARTESIAN_POINT('Ctrl Pts',(-7.07086596700006,15.2,8.87635773199998));
#241287=CARTESIAN_POINT('Ctrl Pts',(-7.07086596700006,11.6,8.87635773199998));
#241288=CARTESIAN_POINT('Ctrl Pts',(-7.06997930800005,15.2,8.87284974499998));
#241289=CARTESIAN_POINT('Ctrl Pts',(-7.06997930800005,11.6,8.87284974499998));
#241290=CARTESIAN_POINT('Ctrl Pts',(-7.06909107000006,15.2,8.86934691799999));
#241291=CARTESIAN_POINT('Ctrl Pts',(-7.06909107000006,11.6,8.86934691799999));
#241292=CARTESIAN_POINT('Ctrl Pts',(-7.06820126200006,15.2,8.86584925799998));
#241293=CARTESIAN_POINT('Ctrl Pts',(-7.06820126200006,11.6,8.86584925799998));
#241294=CARTESIAN_POINT('Ctrl Pts',(-7.06730989000006,15.2,8.86235676999998));
#241295=CARTESIAN_POINT('Ctrl Pts',(-7.06730989000006,11.6,8.86235676999998));
#241296=CARTESIAN_POINT('Ctrl Pts',(-7.06641696500006,15.2,8.85886945899999));
#241297=CARTESIAN_POINT('Ctrl Pts',(-7.06641696500006,11.6,8.85886945899999));
#241298=CARTESIAN_POINT('Ctrl Pts',(-7.06552249100006,15.2,8.85538733199999));
#241299=CARTESIAN_POINT('Ctrl Pts',(-7.06552249100006,11.6,8.85538733199999));
#241300=CARTESIAN_POINT('Ctrl Pts',(-7.06462647800006,15.2,8.85191039399999));
#241301=CARTESIAN_POINT('Ctrl Pts',(-7.06462647800006,11.6,8.85191039399999));
#241302=CARTESIAN_POINT('Ctrl Pts',(-7.06372893200006,15.2,8.84843865099998));
#241303=CARTESIAN_POINT('Ctrl Pts',(-7.06372893200006,11.6,8.84843865099998));
#241304=CARTESIAN_POINT('Ctrl Pts',(-7.06282986100006,15.2,8.84497210899998));
#241305=CARTESIAN_POINT('Ctrl Pts',(-7.06282986100006,11.6,8.84497210899998));
#241306=CARTESIAN_POINT('Ctrl Pts',(-7.06192927500005,15.2,8.84151077399999));
#241307=CARTESIAN_POINT('Ctrl Pts',(-7.06192927500005,11.6,8.84151077399999));
#241308=CARTESIAN_POINT('Ctrl Pts',(-7.06102717800006,15.2,8.83805465099999));
#241309=CARTESIAN_POINT('Ctrl Pts',(-7.06102717800006,11.6,8.83805465099999));
#241310=CARTESIAN_POINT('Ctrl Pts',(-7.06012358100006,15.2,8.83460374699998));
#241311=CARTESIAN_POINT('Ctrl Pts',(-7.06012358100006,11.6,8.83460374699998));
#241312=CARTESIAN_POINT('Ctrl Pts',(-7.05921849000006,15.2,8.83115806699998));
#241313=CARTESIAN_POINT('Ctrl Pts',(-7.05921849000006,11.6,8.83115806699998));
#241314=CARTESIAN_POINT('Ctrl Pts',(-7.05831191400006,15.2,8.82771761699999));
#241315=CARTESIAN_POINT('Ctrl Pts',(-7.05831191400006,11.6,8.82771761699999));
#241316=CARTESIAN_POINT('Ctrl Pts',(-7.05740385900006,15.2,8.82428240299999));
#241317=CARTESIAN_POINT('Ctrl Pts',(-7.05740385900006,11.6,8.82428240299999));
#241318=CARTESIAN_POINT('Ctrl Pts',(-7.05649433500006,15.2,8.82085243099999));
#241319=CARTESIAN_POINT('Ctrl Pts',(-7.05649433500006,11.6,8.82085243099999));
#241320=CARTESIAN_POINT('Ctrl Pts',(-7.05558334800005,15.2,8.81742770599999));
#241321=CARTESIAN_POINT('Ctrl Pts',(-7.05558334800005,11.6,8.81742770599999));
#241322=CARTESIAN_POINT('Ctrl Pts',(-7.05467090700005,15.2,8.81400823599999));
#241323=CARTESIAN_POINT('Ctrl Pts',(-7.05467090700005,11.6,8.81400823599999));
#241324=CARTESIAN_POINT('Ctrl Pts',(-7.05375701900006,15.2,8.81059402399998));
#241325=CARTESIAN_POINT('Ctrl Pts',(-7.05375701900006,11.6,8.81059402399998));
#241326=CARTESIAN_POINT('Ctrl Pts',(-7.05284169300006,15.2,8.80718507699999));
#241327=CARTESIAN_POINT('Ctrl Pts',(-7.05284169300006,11.6,8.80718507699999));
#241328=CARTESIAN_POINT('Ctrl Pts',(-7.05192493600006,15.2,8.80378140299998));
#241329=CARTESIAN_POINT('Ctrl Pts',(-7.05192493600006,11.6,8.80378140299998));
#241330=CARTESIAN_POINT('Ctrl Pts',(-7.05100675700006,15.2,8.80038300399999));
#241331=CARTESIAN_POINT('Ctrl Pts',(-7.05100675700006,11.6,8.80038300399999));
#241332=CARTESIAN_POINT('Ctrl Pts',(-7.05008716300005,15.2,8.79698988899998));
#241333=CARTESIAN_POINT('Ctrl Pts',(-7.05008716300005,11.6,8.79698988899998));
#241334=CARTESIAN_POINT('Ctrl Pts',(-7.04916616100006,15.2,8.79360206199999));
#241335=CARTESIAN_POINT('Ctrl Pts',(-7.04916616100006,11.6,8.79360206199999));
#241336=CARTESIAN_POINT('Ctrl Pts',(-7.04824376200006,15.2,8.79021952899999));
#241337=CARTESIAN_POINT('Ctrl Pts',(-7.04824376200006,11.6,8.79021952899999));
#241338=CARTESIAN_POINT('Ctrl Pts',(-7.04731997100006,15.2,8.78684229799998));
#241339=CARTESIAN_POINT('Ctrl Pts',(-7.04731997100006,11.6,8.78684229799998));
#241340=CARTESIAN_POINT('Ctrl Pts',(-7.04639479800006,15.2,8.78347037299999));
#241341=CARTESIAN_POINT('Ctrl Pts',(-7.04639479800006,11.6,8.78347037299999));
#241342=CARTESIAN_POINT('Ctrl Pts',(-7.04546825000006,15.2,8.78010376099999));
#241343=CARTESIAN_POINT('Ctrl Pts',(-7.04546825000006,11.6,8.78010376099999));
#241344=CARTESIAN_POINT('Ctrl Pts',(-7.04454033600006,15.2,8.77674246599998));
#241345=CARTESIAN_POINT('Ctrl Pts',(-7.04454033600006,11.6,8.77674246599998));
#241346=CARTESIAN_POINT('Ctrl Pts',(-7.04361106300006,15.2,8.77338649599999));
#241347=CARTESIAN_POINT('Ctrl Pts',(-7.04361106300006,11.6,8.77338649599999));
#241348=CARTESIAN_POINT('Ctrl Pts',(-7.04268044000006,15.2,8.77003585599999));
#241349=CARTESIAN_POINT('Ctrl Pts',(-7.04268044000006,11.6,8.77003585599999));
#241350=CARTESIAN_POINT('Ctrl Pts',(-7.04174847500005,15.2,8.76669055199999));
#241351=CARTESIAN_POINT('Ctrl Pts',(-7.04174847500005,11.6,8.76669055199999));
#241352=CARTESIAN_POINT('Ctrl Pts',(-7.04081517600006,15.2,8.76335058999998));
#241353=CARTESIAN_POINT('Ctrl Pts',(-7.04081517600006,11.6,8.76335058999998));
#241354=CARTESIAN_POINT('Ctrl Pts',(-7.03988055100006,15.2,8.76001597599998));
#241355=CARTESIAN_POINT('Ctrl Pts',(-7.03988055100006,11.6,8.76001597599998));
#241356=CARTESIAN_POINT('Ctrl Pts',(-7.03894460800006,15.2,8.75668671499999));
#241357=CARTESIAN_POINT('Ctrl Pts',(-7.03894460800006,11.6,8.75668671499999));
#241358=CARTESIAN_POINT('Ctrl Pts',(-7.03800735600006,15.2,8.75336281399999));
#241359=CARTESIAN_POINT('Ctrl Pts',(-7.03800735600006,11.6,8.75336281399999));
#241360=CARTESIAN_POINT('Ctrl Pts',(-7.03706880200006,15.2,8.75004427999999));
#241361=CARTESIAN_POINT('Ctrl Pts',(-7.03706880200006,11.6,8.75004427999999));
#241362=CARTESIAN_POINT('Ctrl Pts',(-7.03612895600005,15.2,8.74673111599999));
#241363=CARTESIAN_POINT('Ctrl Pts',(-7.03612895600005,11.6,8.74673111599999));
#241364=CARTESIAN_POINT('Ctrl Pts',(-7.03518782600006,15.2,8.74342332999999));
#241365=CARTESIAN_POINT('Ctrl Pts',(-7.03518782600006,11.6,8.74342332999999));
#241366=CARTESIAN_POINT('Ctrl Pts',(-7.03424541800006,15.2,8.74012092699999));
#241367=CARTESIAN_POINT('Ctrl Pts',(-7.03424541800006,11.6,8.74012092699999));
#241368=CARTESIAN_POINT('Ctrl Pts',(-7.03330174400006,15.2,8.73682391499998));
#241369=CARTESIAN_POINT('Ctrl Pts',(-7.03330174400006,11.6,8.73682391499998));
#241370=CARTESIAN_POINT('Ctrl Pts',(-7.03235680900006,15.2,8.73353229799999));
#241371=CARTESIAN_POINT('Ctrl Pts',(-7.03235680900006,11.6,8.73353229799999));
#241372=CARTESIAN_POINT('Ctrl Pts',(-7.03141062300006,15.2,8.73024608099998));
#241373=CARTESIAN_POINT('Ctrl Pts',(-7.03141062300006,11.6,8.73024608099998));
#241374=CARTESIAN_POINT('Ctrl Pts',(-7.03046319500006,15.2,8.72696527299999));
#241375=CARTESIAN_POINT('Ctrl Pts',(-7.03046319500006,11.6,8.72696527299999));
#241376=CARTESIAN_POINT('Ctrl Pts',(-7.02951453100006,15.2,8.72368987799998));
#241377=CARTESIAN_POINT('Ctrl Pts',(-7.02951453100006,11.6,8.72368987799998));
#241378=CARTESIAN_POINT('Ctrl Pts',(-7.02856464100006,15.2,8.72041990199998));
#241379=CARTESIAN_POINT('Ctrl Pts',(-7.02856464100006,11.6,8.72041990199998));
#241380=CARTESIAN_POINT('Ctrl Pts',(-7.02761353400006,15.2,8.71715535199998));
#241381=CARTESIAN_POINT('Ctrl Pts',(-7.02761353400006,11.6,8.71715535199998));
#241382=CARTESIAN_POINT('Ctrl Pts',(-7.02666121800006,15.2,8.71389623299999));
#241383=CARTESIAN_POINT('Ctrl Pts',(-7.02666121800006,11.6,8.71389623299999));
#241384=CARTESIAN_POINT('Ctrl Pts',(-7.02570770200006,15.2,8.71064255199999));
#241385=CARTESIAN_POINT('Ctrl Pts',(-7.02570770200006,11.6,8.71064255199999));
#241386=CARTESIAN_POINT('Ctrl Pts',(-7.02475299300006,15.2,8.70739431299998));
#241387=CARTESIAN_POINT('Ctrl Pts',(-7.02475299300006,11.6,8.70739431299998));
#241388=CARTESIAN_POINT('Ctrl Pts',(-7.02379710000006,15.2,8.70415152399998));
#241389=CARTESIAN_POINT('Ctrl Pts',(-7.02379710000006,11.6,8.70415152399998));
#241390=CARTESIAN_POINT('Ctrl Pts',(-7.02284003300006,15.2,8.70091419099998));
#241391=CARTESIAN_POINT('Ctrl Pts',(-7.02284003300006,11.6,8.70091419099998));
#241392=CARTESIAN_POINT('Ctrl Pts',(-7.02188179900006,15.2,8.69768231899998));
#241393=CARTESIAN_POINT('Ctrl Pts',(-7.02188179900006,11.6,8.69768231899998));
#241394=CARTESIAN_POINT('Ctrl Pts',(-7.02092240700006,15.2,8.69445591399998));
#241395=CARTESIAN_POINT('Ctrl Pts',(-7.02092240700006,11.6,8.69445591399998));
#241396=CARTESIAN_POINT('Ctrl Pts',(-7.01996186600006,15.2,8.69123498299999));
#241397=CARTESIAN_POINT('Ctrl Pts',(-7.01996186600006,11.6,8.69123498299999));
#241398=CARTESIAN_POINT('Ctrl Pts',(-7.01900018300006,15.2,8.68801953099998));
#241399=CARTESIAN_POINT('Ctrl Pts',(-7.01900018300006,11.6,8.68801953099998));
#241400=CARTESIAN_POINT('Ctrl Pts',(-7.01803737000006,15.2,8.68480956499998));
#241401=CARTESIAN_POINT('Ctrl Pts',(-7.01803737000006,11.6,8.68480956499998));
#241402=CARTESIAN_POINT('Ctrl Pts',(-7.01707343300006,15.2,8.68160509099998));
#241403=CARTESIAN_POINT('Ctrl Pts',(-7.01707343300006,11.6,8.68160509099998));
#241404=CARTESIAN_POINT('Ctrl Pts',(-7.01610838200006,15.2,8.67840611399998));
#241405=CARTESIAN_POINT('Ctrl Pts',(-7.01610838200006,11.6,8.67840611399998));
#241406=CARTESIAN_POINT('Ctrl Pts',(-7.01514222400006,15.2,8.67521264099998));
#241407=CARTESIAN_POINT('Ctrl Pts',(-7.01514222400006,11.6,8.67521264099998));
#241408=CARTESIAN_POINT('Ctrl Pts',(-7.01417497000006,15.2,8.67202467699999));
#241409=CARTESIAN_POINT('Ctrl Pts',(-7.01417497000006,11.6,8.67202467699999));
#241410=CARTESIAN_POINT('Ctrl Pts',(-7.01320662700006,15.2,8.66884222899999));
#241411=CARTESIAN_POINT('Ctrl Pts',(-7.01320662700006,11.6,8.66884222899999));
#241412=CARTESIAN_POINT('Ctrl Pts',(-7.01223720400006,15.2,8.66566530299998));
#241413=CARTESIAN_POINT('Ctrl Pts',(-7.01223720400006,11.6,8.66566530299998));
#241414=CARTESIAN_POINT('Ctrl Pts',(-7.01126671200006,15.2,8.66249390599998));
#241415=CARTESIAN_POINT('Ctrl Pts',(-7.01126671200006,11.6,8.66249390599998));
#241416=CARTESIAN_POINT('Ctrl Pts',(-7.01029515700006,15.2,8.65932804199998));
#241417=CARTESIAN_POINT('Ctrl Pts',(-7.01029515700006,11.6,8.65932804199998));
#241418=CARTESIAN_POINT('Ctrl Pts',(-7.00932254900006,15.2,8.65616771799999));
#241419=CARTESIAN_POINT('Ctrl Pts',(-7.00932254900006,11.6,8.65616771799999));
#241420=CARTESIAN_POINT('Ctrl Pts',(-7.00834889700006,15.2,8.65301293999998));
#241421=CARTESIAN_POINT('Ctrl Pts',(-7.00834889700006,11.6,8.65301293999998));
#241422=CARTESIAN_POINT('Ctrl Pts',(-7.00737421000006,15.2,8.64986371499998));
#241423=CARTESIAN_POINT('Ctrl Pts',(-7.00737421000006,11.6,8.64986371499998));
#241424=CARTESIAN_POINT('Ctrl Pts',(-7.00639849600006,15.2,8.64672004799999));
#241425=CARTESIAN_POINT('Ctrl Pts',(-7.00639849600006,11.6,8.64672004799999));
#241426=CARTESIAN_POINT('Ctrl Pts',(-7.00542176600006,15.2,8.64358194499999));
#241427=CARTESIAN_POINT('Ctrl Pts',(-7.00542176600006,11.6,8.64358194499999));
#241428=CARTESIAN_POINT('Ctrl Pts',(-7.00444402700006,15.2,8.64044941399998));
#241429=CARTESIAN_POINT('Ctrl Pts',(-7.00444402700006,11.6,8.64044941399998));
#241430=CARTESIAN_POINT('Ctrl Pts',(-7.00346528800006,15.2,8.63732245899998));
#241431=CARTESIAN_POINT('Ctrl Pts',(-7.00346528800006,11.6,8.63732245899998));
#241432=CARTESIAN_POINT('Ctrl Pts',(-7.00248556000005,15.2,8.63420108599998));
#241433=CARTESIAN_POINT('Ctrl Pts',(-7.00248556000005,11.6,8.63420108599998));
#241434=CARTESIAN_POINT('Ctrl Pts',(-7.00150484900006,15.2,8.63108530299998));
#241435=CARTESIAN_POINT('Ctrl Pts',(-7.00150484900006,11.6,8.63108530299998));
#241436=CARTESIAN_POINT('Ctrl Pts',(-7.00052316800006,15.2,8.62797511399998));
#241437=CARTESIAN_POINT('Ctrl Pts',(-7.00052316800006,11.6,8.62797511399998));
#241438=CARTESIAN_POINT('Ctrl Pts',(-6.99954052300006,15.2,8.62487052699999));
#241439=CARTESIAN_POINT('Ctrl Pts',(-6.99954052300006,11.6,8.62487052699999));
#241440=CARTESIAN_POINT('Ctrl Pts',(-6.99855692300006,15.2,8.62177154799999));
#241441=CARTESIAN_POINT('Ctrl Pts',(-6.99855692300006,11.6,8.62177154799999));
#241442=CARTESIAN_POINT('Ctrl Pts',(-6.99757237900006,15.2,8.61867818099999));
#241443=CARTESIAN_POINT('Ctrl Pts',(-6.99757237900006,11.6,8.61867818099999));
#241444=CARTESIAN_POINT('Ctrl Pts',(-6.99658689800006,15.2,8.61559043399998));
#241445=CARTESIAN_POINT('Ctrl Pts',(-6.99658689800006,11.6,8.61559043399998));
#241446=CARTESIAN_POINT('Ctrl Pts',(-6.99560049200006,15.2,8.61250831299999));
#241447=CARTESIAN_POINT('Ctrl Pts',(-6.99560049200006,11.6,8.61250831299999));
#241448=CARTESIAN_POINT('Ctrl Pts',(-6.99461316900006,15.2,8.60943182499998));
#241449=CARTESIAN_POINT('Ctrl Pts',(-6.99461316900006,11.6,8.60943182499998));
#241450=CARTESIAN_POINT('Ctrl Pts',(-6.99362493700006,15.2,8.60636097399999));
#241451=CARTESIAN_POINT('Ctrl Pts',(-6.99362493700006,11.6,8.60636097399999));
#241452=CARTESIAN_POINT('Ctrl Pts',(-6.99263580600006,15.2,8.60329576699998));
#241453=CARTESIAN_POINT('Ctrl Pts',(-6.99263580600006,11.6,8.60329576699998));
#241454=CARTESIAN_POINT('Ctrl Pts',(-6.99164578600006,15.2,8.60023621099998));
#241455=CARTESIAN_POINT('Ctrl Pts',(-6.99164578600006,11.6,8.60023621099998));
#241456=CARTESIAN_POINT('Ctrl Pts',(-6.99065488600006,15.2,8.59718231199999));
#241457=CARTESIAN_POINT('Ctrl Pts',(-6.99065488600006,11.6,8.59718231199999));
#241458=CARTESIAN_POINT('Ctrl Pts',(-6.98966311500006,15.2,8.59413407599998));
#241459=CARTESIAN_POINT('Ctrl Pts',(-6.98966311500006,11.6,8.59413407599998));
#241460=CARTESIAN_POINT('Ctrl Pts',(-6.98867048100006,15.2,8.59109150799998));
#241461=CARTESIAN_POINT('Ctrl Pts',(-6.98867048100006,11.6,8.59109150799998));
#241462=CARTESIAN_POINT('Ctrl Pts',(-6.98767699600006,15.2,8.58805461599999));
#241463=CARTESIAN_POINT('Ctrl Pts',(-6.98767699600006,11.6,8.58805461599999));
#241464=CARTESIAN_POINT('Ctrl Pts',(-6.98668266900006,15.2,8.58502340599999));
#241465=CARTESIAN_POINT('Ctrl Pts',(-6.98668266900006,11.6,8.58502340599999));
#241466=CARTESIAN_POINT('Ctrl Pts',(-6.98568750700006,15.2,8.58199788299999));
#241467=CARTESIAN_POINT('Ctrl Pts',(-6.98568750700006,11.6,8.58199788299999));
#241468=CARTESIAN_POINT('Ctrl Pts',(-6.98469152300006,15.2,8.57897805299999));
#241469=CARTESIAN_POINT('Ctrl Pts',(-6.98469152300006,11.6,8.57897805299999));
#241470=CARTESIAN_POINT('Ctrl Pts',(-6.98369472300006,15.2,8.57596392499998));
#241471=CARTESIAN_POINT('Ctrl Pts',(-6.98369472300006,11.6,8.57596392499998));
#241472=CARTESIAN_POINT('Ctrl Pts',(-6.98269711900006,15.2,8.57295550199999));
#241473=CARTESIAN_POINT('Ctrl Pts',(-6.98269711900006,11.6,8.57295550199999));
#241474=CARTESIAN_POINT('Ctrl Pts',(-6.98169871800006,15.2,8.56995279199998));
#241475=CARTESIAN_POINT('Ctrl Pts',(-6.98169871800006,11.6,8.56995279199998));
#241476=CARTESIAN_POINT('Ctrl Pts',(-6.98069953300006,15.2,8.56695580099998));
#241477=CARTESIAN_POINT('Ctrl Pts',(-6.98069953300006,11.6,8.56695580099998));
#241478=CARTESIAN_POINT('Ctrl Pts',(-6.97969957100006,15.2,8.56396453399999));
#241479=CARTESIAN_POINT('Ctrl Pts',(-6.97969957100006,11.6,8.56396453399999));
#241480=CARTESIAN_POINT('Ctrl Pts',(-6.97869884300006,15.2,8.56097899899999));
#241481=CARTESIAN_POINT('Ctrl Pts',(-6.97869884300006,11.6,8.56097899899999));
#241482=CARTESIAN_POINT('Ctrl Pts',(-6.97769735700006,15.2,8.55799920099999));
#241483=CARTESIAN_POINT('Ctrl Pts',(-6.97769735700006,11.6,8.55799920099999));
#241484=CARTESIAN_POINT('Ctrl Pts',(-6.97669512400005,15.2,8.55502514799999));
#241485=CARTESIAN_POINT('Ctrl Pts',(-6.97669512400005,11.6,8.55502514799999));
#241486=CARTESIAN_POINT('Ctrl Pts',(-6.97569215400006,15.2,8.55205684399999));
#241487=CARTESIAN_POINT('Ctrl Pts',(-6.97569215400006,11.6,8.55205684399999));
#241488=CARTESIAN_POINT('Ctrl Pts',(-6.97468845400006,15.2,8.54909429699998));
#241489=CARTESIAN_POINT('Ctrl Pts',(-6.97468845400006,11.6,8.54909429699998));
#241490=CARTESIAN_POINT('Ctrl Pts',(-6.97368403800006,15.2,8.54613751299999));
#241491=CARTESIAN_POINT('Ctrl Pts',(-6.97368403800006,11.6,8.54613751299999));
#241492=CARTESIAN_POINT('Ctrl Pts',(-6.97267891300006,15.2,8.54318649699999));
#241493=CARTESIAN_POINT('Ctrl Pts',(-6.97267891300006,11.6,8.54318649699999));
#241494=CARTESIAN_POINT('Ctrl Pts',(-6.97167308800006,15.2,8.54024125799998));
#241495=CARTESIAN_POINT('Ctrl Pts',(-6.97167308800006,11.6,8.54024125799998));
#241496=CARTESIAN_POINT('Ctrl Pts',(-6.97066657500006,15.2,8.53730179799999));
#241497=CARTESIAN_POINT('Ctrl Pts',(-6.97066657500006,11.6,8.53730179799999));
#241498=CARTESIAN_POINT('Ctrl Pts',(-6.96965938300006,15.2,8.53436812799998));
#241499=CARTESIAN_POINT('Ctrl Pts',(-6.96965938300006,11.6,8.53436812799998));
#241500=CARTESIAN_POINT('Ctrl Pts',(-6.96865152100006,15.2,8.53144025099999));
#241501=CARTESIAN_POINT('Ctrl Pts',(-6.96865152100006,11.6,8.53144025099999));
#241502=CARTESIAN_POINT('Ctrl Pts',(-6.96764300000006,15.2,8.52851817499998));
#241503=CARTESIAN_POINT('Ctrl Pts',(-6.96764300000006,11.6,8.52851817499998));
#241504=CARTESIAN_POINT('Ctrl Pts',(-6.96663383000006,15.2,8.52560190499998));
#241505=CARTESIAN_POINT('Ctrl Pts',(-6.96663383000006,11.6,8.52560190499998));
#241506=CARTESIAN_POINT('Ctrl Pts',(-6.96562402000006,15.2,8.52269144799998));
#241507=CARTESIAN_POINT('Ctrl Pts',(-6.96562402000006,11.6,8.52269144799998));
#241508=CARTESIAN_POINT('Ctrl Pts',(-6.96461358100006,15.2,8.51978681099999));
#241509=CARTESIAN_POINT('Ctrl Pts',(-6.96461358100006,11.6,8.51978681099999));
#241510=CARTESIAN_POINT('Ctrl Pts',(-6.96360252100006,15.2,8.51688799899998));
#241511=CARTESIAN_POINT('Ctrl Pts',(-6.96360252100006,11.6,8.51688799899998));
#241512=CARTESIAN_POINT('Ctrl Pts',(-6.96259085300006,15.2,8.51399501999998));
#241513=CARTESIAN_POINT('Ctrl Pts',(-6.96259085300006,11.6,8.51399501999998));
#241514=CARTESIAN_POINT('Ctrl Pts',(-6.96157858500006,15.2,8.51110787899999));
#241515=CARTESIAN_POINT('Ctrl Pts',(-6.96157858500006,11.6,8.51110787899999));
#241516=CARTESIAN_POINT('Ctrl Pts',(-6.96056572800006,15.2,8.50822658299998));
#241517=CARTESIAN_POINT('Ctrl Pts',(-6.96056572800006,11.6,8.50822658299998));
#241518=CARTESIAN_POINT('Ctrl Pts',(-6.95955229200006,15.2,8.50535113899999));
#241519=CARTESIAN_POINT('Ctrl Pts',(-6.95955229200006,11.6,8.50535113899999));
#241520=CARTESIAN_POINT('Ctrl Pts',(-6.95853828500006,15.2,8.50248155199999));
#241521=CARTESIAN_POINT('Ctrl Pts',(-6.95853828500006,11.6,8.50248155199999));
#241522=CARTESIAN_POINT('Ctrl Pts',(-6.95752372100006,15.2,8.49961782899998));
#241523=CARTESIAN_POINT('Ctrl Pts',(-6.95752372100006,11.6,8.49961782899998));
#241524=CARTESIAN_POINT('Ctrl Pts',(-6.95650860700006,15.2,8.49675997499999));
#241525=CARTESIAN_POINT('Ctrl Pts',(-6.95650860700006,11.6,8.49675997499999));
#241526=CARTESIAN_POINT('Ctrl Pts',(-6.95549295500006,15.2,8.49390799999998));
#241527=CARTESIAN_POINT('Ctrl Pts',(-6.95549295500006,11.6,8.49390799999998));
#241528=CARTESIAN_POINT('Ctrl Pts',(-6.95447677300006,15.2,8.49106190699998));
#241529=CARTESIAN_POINT('Ctrl Pts',(-6.95447677300006,11.6,8.49106190699998));
#241530=CARTESIAN_POINT('Ctrl Pts',(-6.95346007500006,15.2,8.48822170299999));
#241531=CARTESIAN_POINT('Ctrl Pts',(-6.95346007500006,11.6,8.48822170299999));
#241532=CARTESIAN_POINT('Ctrl Pts',(-6.95244286800006,15.2,8.48538739599999));
#241533=CARTESIAN_POINT('Ctrl Pts',(-6.95244286800006,11.6,8.48538739599999));
#241534=CARTESIAN_POINT('Ctrl Pts',(-6.95142516400006,15.2,8.48255898999999));
#241535=CARTESIAN_POINT('Ctrl Pts',(-6.95142516400006,11.6,8.48255898999999));
#241536=CARTESIAN_POINT('Ctrl Pts',(-6.95040697200006,15.2,8.47973649399999));
#241537=CARTESIAN_POINT('Ctrl Pts',(-6.95040697200006,11.6,8.47973649399999));
#241538=CARTESIAN_POINT('Ctrl Pts',(-6.94938830500006,15.2,8.47691991299998));
#241539=CARTESIAN_POINT('Ctrl Pts',(-6.94938830500006,11.6,8.47691991299998));
#241540=CARTESIAN_POINT('Ctrl Pts',(-6.94836917000006,15.2,8.47410925299998));
#241541=CARTESIAN_POINT('Ctrl Pts',(-6.94836917000006,11.6,8.47410925299998));
#241542=CARTESIAN_POINT('Ctrl Pts',(-6.94734957900006,15.2,8.47130452199998));
#241543=CARTESIAN_POINT('Ctrl Pts',(-6.94734957900006,11.6,8.47130452199998));
#241544=CARTESIAN_POINT('Ctrl Pts',(-6.94632954300006,15.2,8.46850572499999));
#241545=CARTESIAN_POINT('Ctrl Pts',(-6.94632954300006,11.6,8.46850572499999));
#241546=CARTESIAN_POINT('Ctrl Pts',(-6.94530907200006,15.2,8.46571286899999));
#241547=CARTESIAN_POINT('Ctrl Pts',(-6.94530907200006,11.6,8.46571286899999));
#241548=CARTESIAN_POINT('Ctrl Pts',(-6.94428817600006,15.2,8.46292595999999));
#241549=CARTESIAN_POINT('Ctrl Pts',(-6.94428817600006,11.6,8.46292595999999));
#241550=CARTESIAN_POINT('Ctrl Pts',(-6.94326686700006,15.2,8.46014500499999));
#241551=CARTESIAN_POINT('Ctrl Pts',(-6.94326686700006,11.6,8.46014500499999));
#241552=CARTESIAN_POINT('Ctrl Pts',(-6.94224515500006,15.2,8.45737001099998));
#241553=CARTESIAN_POINT('Ctrl Pts',(-6.94224515500006,11.6,8.45737001099998));
#241554=CARTESIAN_POINT('Ctrl Pts',(-6.94122304900006,15.2,8.45460098399998));
#241555=CARTESIAN_POINT('Ctrl Pts',(-6.94122304900006,11.6,8.45460098399998));
#241556=CARTESIAN_POINT('Ctrl Pts',(-6.94020056100006,15.2,8.45183792999999));
#241557=CARTESIAN_POINT('Ctrl Pts',(-6.94020056100006,11.6,8.45183792999999));
#241558=CARTESIAN_POINT('Ctrl Pts',(-6.93917770200006,15.2,8.44908085699998));
#241559=CARTESIAN_POINT('Ctrl Pts',(-6.93917770200006,11.6,8.44908085699998));
#241560=CARTESIAN_POINT('Ctrl Pts',(-6.93815448200006,15.2,8.44632976799998));
#241561=CARTESIAN_POINT('Ctrl Pts',(-6.93815448200006,11.6,8.44632976799998));
#241562=CARTESIAN_POINT('Ctrl Pts',(-6.93713091200006,15.2,8.44358467399999));
#241563=CARTESIAN_POINT('Ctrl Pts',(-6.93713091200006,11.6,8.44358467399999));
#241564=CARTESIAN_POINT('Ctrl Pts',(-6.93610700300006,15.2,8.44084557799999));
#241565=CARTESIAN_POINT('Ctrl Pts',(-6.93610700300006,11.6,8.44084557799999));
#241566=CARTESIAN_POINT('Ctrl Pts',(-6.93508276600006,15.2,8.43811248899998));
#241567=CARTESIAN_POINT('Ctrl Pts',(-6.93508276600006,11.6,8.43811248899998));
#241568=CARTESIAN_POINT('Ctrl Pts',(-6.93405821100006,15.2,8.43538541199998));
#241569=CARTESIAN_POINT('Ctrl Pts',(-6.93405821100006,11.6,8.43538541199998));
#241570=CARTESIAN_POINT('Ctrl Pts',(-6.93303334800006,15.2,8.43266435399999));
#241571=CARTESIAN_POINT('Ctrl Pts',(-6.93303334800006,11.6,8.43266435399999));
#241572=CARTESIAN_POINT('Ctrl Pts',(-6.93200819100006,15.2,8.42994932099998));
#241573=CARTESIAN_POINT('Ctrl Pts',(-6.93200819100006,11.6,8.42994932099998));
#241574=CARTESIAN_POINT('Ctrl Pts',(-6.93098274800006,15.2,8.42724032099999));
#241575=CARTESIAN_POINT('Ctrl Pts',(-6.93098274800006,11.6,8.42724032099999));
#241576=CARTESIAN_POINT('Ctrl Pts',(-6.92995703100006,15.2,8.42453735999998));
#241577=CARTESIAN_POINT('Ctrl Pts',(-6.92995703100006,11.6,8.42453735999998));
#241578=CARTESIAN_POINT('Ctrl Pts',(-6.92893105100006,15.2,8.42184044299999));
#241579=CARTESIAN_POINT('Ctrl Pts',(-6.92893105100006,11.6,8.42184044299999));
#241580=CARTESIAN_POINT('Ctrl Pts',(-6.92790481800006,15.2,8.41914957799998));
#241581=CARTESIAN_POINT('Ctrl Pts',(-6.92790481800006,11.6,8.41914957799998));
#241582=CARTESIAN_POINT('Ctrl Pts',(-6.92687834600005,15.2,8.41646477099999));
#241583=CARTESIAN_POINT('Ctrl Pts',(-6.92687834600005,11.6,8.41646477099999));
#241584=CARTESIAN_POINT('Ctrl Pts',(-6.92585164200006,15.2,8.41378602999999));
#241585=CARTESIAN_POINT('Ctrl Pts',(-6.92585164200006,11.6,8.41378602999999));
#241586=CARTESIAN_POINT('Ctrl Pts',(-6.92482471900006,15.2,8.41111335999998));
#241587=CARTESIAN_POINT('Ctrl Pts',(-6.92482471900006,11.6,8.41111335999998));
#241588=CARTESIAN_POINT('Ctrl Pts',(-6.92379759000006,15.2,8.40844676899999));
#241589=CARTESIAN_POINT('Ctrl Pts',(-6.92379759000006,11.6,8.40844676899999));
#241590=CARTESIAN_POINT('Ctrl Pts',(-6.92277026400006,15.2,8.40578626199999));
#241591=CARTESIAN_POINT('Ctrl Pts',(-6.92277026400006,11.6,8.40578626199999));
#241592=CARTESIAN_POINT('Ctrl Pts',(-6.92174275100006,15.2,8.40313184599999));
#241593=CARTESIAN_POINT('Ctrl Pts',(-6.92174275100006,11.6,8.40313184599999));
#241594=CARTESIAN_POINT('Ctrl Pts',(-6.92071506500006,15.2,8.40048352999998));
#241595=CARTESIAN_POINT('Ctrl Pts',(-6.92071506500006,11.6,8.40048352999998));
#241596=CARTESIAN_POINT('Ctrl Pts',(-6.91968721600006,15.2,8.39784131699999));
#241597=CARTESIAN_POINT('Ctrl Pts',(-6.91968721600006,11.6,8.39784131699999));
#241598=CARTESIAN_POINT('Ctrl Pts',(-6.91865921500006,15.2,8.39520521599999));
#241599=CARTESIAN_POINT('Ctrl Pts',(-6.91865921500006,11.6,8.39520521599999));
#241600=CARTESIAN_POINT('Ctrl Pts',(-6.91763107300006,15.2,8.39257523199999));
#241601=CARTESIAN_POINT('Ctrl Pts',(-6.91763107300006,11.6,8.39257523199999));
#241602=CARTESIAN_POINT('Ctrl Pts',(-6.91660280300006,15.2,8.38995137299998));
#241603=CARTESIAN_POINT('Ctrl Pts',(-6.91660280300006,11.6,8.38995137299998));
#241604=CARTESIAN_POINT('Ctrl Pts',(-6.91557441500006,15.2,8.38733364499999));
#241605=CARTESIAN_POINT('Ctrl Pts',(-6.91557441500006,11.6,8.38733364499999));
#241606=CARTESIAN_POINT('Ctrl Pts',(-6.91454592100006,15.2,8.38472205599999));
#241607=CARTESIAN_POINT('Ctrl Pts',(-6.91454592100006,11.6,8.38472205599999));
#241608=CARTESIAN_POINT('Ctrl Pts',(-6.91351733200006,15.2,8.38211661099999));
#241609=CARTESIAN_POINT('Ctrl Pts',(-6.91351733200006,11.6,8.38211661099999));
#241610=CARTESIAN_POINT('Ctrl Pts',(-6.91248866000006,15.2,8.37951731799999));
#241611=CARTESIAN_POINT('Ctrl Pts',(-6.91248866000006,11.6,8.37951731799999));
#241612=CARTESIAN_POINT('Ctrl Pts',(-6.91145991600006,15.2,8.37692418199998));
#241613=CARTESIAN_POINT('Ctrl Pts',(-6.91145991600006,11.6,8.37692418199998));
#241614=CARTESIAN_POINT('Ctrl Pts',(-6.91043111200006,15.2,8.37433721099998));
#241615=CARTESIAN_POINT('Ctrl Pts',(-6.91043111200006,11.6,8.37433721099998));
#241616=CARTESIAN_POINT('Ctrl Pts',(-6.90940225900006,15.2,8.37175641099999));
#241617=CARTESIAN_POINT('Ctrl Pts',(-6.90940225900006,11.6,8.37175641099999));
#241618=CARTESIAN_POINT('Ctrl Pts',(-6.90837336900006,15.2,8.36918178999999));
#241619=CARTESIAN_POINT('Ctrl Pts',(-6.90837336900006,11.6,8.36918178999999));
#241620=CARTESIAN_POINT('Ctrl Pts',(-6.90734445400006,15.2,8.36661335399998));
#241621=CARTESIAN_POINT('Ctrl Pts',(-6.90734445400006,11.6,8.36661335399998));
#241622=CARTESIAN_POINT('Ctrl Pts',(-6.90631552400006,15.2,8.36405110899998));
#241623=CARTESIAN_POINT('Ctrl Pts',(-6.90631552400006,11.6,8.36405110899998));
#241624=CARTESIAN_POINT('Ctrl Pts',(-6.90528659400006,15.2,8.36149506199998));
#241625=CARTESIAN_POINT('Ctrl Pts',(-6.90528659400006,11.6,8.36149506199998));
#241626=CARTESIAN_POINT('Ctrl Pts',(-6.90425767200006,15.2,8.35894522099998));
#241627=CARTESIAN_POINT('Ctrl Pts',(-6.90425767200006,11.6,8.35894522099998));
#241628=CARTESIAN_POINT('Ctrl Pts',(-6.90322877200006,15.2,8.35640159099999));
#241629=CARTESIAN_POINT('Ctrl Pts',(-6.90322877200006,11.6,8.35640159099999));
#241630=CARTESIAN_POINT('Ctrl Pts',(-6.90219990600006,15.2,8.35386418099999));
#241631=CARTESIAN_POINT('Ctrl Pts',(-6.90219990600006,11.6,8.35386418099999));
#241632=CARTESIAN_POINT('Ctrl Pts',(-6.90117108500006,15.2,8.35133299499999));
#241633=CARTESIAN_POINT('Ctrl Pts',(-6.90117108500006,11.6,8.35133299499999));
#241634=CARTESIAN_POINT('Ctrl Pts',(-6.90014232100006,15.2,8.34880804199998));
#241635=CARTESIAN_POINT('Ctrl Pts',(-6.90014232100006,11.6,8.34880804199998));
#241636=CARTESIAN_POINT('Ctrl Pts',(-6.89911362600006,15.2,8.34628932799999));
#241637=CARTESIAN_POINT('Ctrl Pts',(-6.89911362600006,11.6,8.34628932799999));
#241638=CARTESIAN_POINT('Ctrl Pts',(-6.89808501200006,15.2,8.34377685899998));
#241639=CARTESIAN_POINT('Ctrl Pts',(-6.89808501200006,11.6,8.34377685899998));
#241640=CARTESIAN_POINT('Ctrl Pts',(-6.89705649000006,15.2,8.34127064299999));
#241641=CARTESIAN_POINT('Ctrl Pts',(-6.89705649000006,11.6,8.34127064299999));
#241642=CARTESIAN_POINT('Ctrl Pts',(-6.89602807500005,15.2,8.33877068699999));
#241643=CARTESIAN_POINT('Ctrl Pts',(-6.89602807500005,11.6,8.33877068699999));
#241644=CARTESIAN_POINT('Ctrl Pts',(-6.89499977500006,15.2,8.33627699599998));
#241645=CARTESIAN_POINT('Ctrl Pts',(-6.89499977500006,11.6,8.33627699599998));
#241646=CARTESIAN_POINT('Ctrl Pts',(-6.89397160500006,15.2,8.33378957899999));
#241647=CARTESIAN_POINT('Ctrl Pts',(-6.89397160500006,11.6,8.33378957899999));
#241648=CARTESIAN_POINT('Ctrl Pts',(-6.89294357700006,15.2,8.33130844199999));
#241649=CARTESIAN_POINT('Ctrl Pts',(-6.89294357700006,11.6,8.33130844199999));
#241650=CARTESIAN_POINT('Ctrl Pts',(-6.89191570200006,15.2,8.32883359199998));
#241651=CARTESIAN_POINT('Ctrl Pts',(-6.89191570200006,11.6,8.32883359199998));
#241652=CARTESIAN_POINT('Ctrl Pts',(-6.89088799300006,15.2,8.32636503499998));
#241653=CARTESIAN_POINT('Ctrl Pts',(-6.89088799300006,11.6,8.32636503499998));
#241654=CARTESIAN_POINT('Ctrl Pts',(-6.88986046100006,15.2,8.32390277899999));
#241655=CARTESIAN_POINT('Ctrl Pts',(-6.88986046100006,11.6,8.32390277899999));
#241656=CARTESIAN_POINT('Ctrl Pts',(-6.88883312000006,15.2,8.32144682999999));
#241657=CARTESIAN_POINT('Ctrl Pts',(-6.88883312000006,11.6,8.32144682999999));
#241658=CARTESIAN_POINT('Ctrl Pts',(-6.88780598100006,15.2,8.31899719499999));
#241659=CARTESIAN_POINT('Ctrl Pts',(-6.88780598100006,11.6,8.31899719499999));
#241660=CARTESIAN_POINT('Ctrl Pts',(-6.88677905700006,15.2,8.31655388199999));
#241661=CARTESIAN_POINT('Ctrl Pts',(-6.88677905700006,11.6,8.31655388199999));
#241662=CARTESIAN_POINT('Ctrl Pts',(-6.88575236000006,15.2,8.31411689699999));
#241663=CARTESIAN_POINT('Ctrl Pts',(-6.88575236000006,11.6,8.31411689699999));
#241664=CARTESIAN_POINT('Ctrl Pts',(-6.88472590400006,15.2,8.31168624599999));
#241665=CARTESIAN_POINT('Ctrl Pts',(-6.88472590400006,11.6,8.31168624599999));
#241666=CARTESIAN_POINT('Ctrl Pts',(-6.88369969900006,15.2,8.30926193799998));
#241667=CARTESIAN_POINT('Ctrl Pts',(-6.88369969900006,11.6,8.30926193799998));
#241668=CARTESIAN_POINT('Ctrl Pts',(-6.88267376000006,15.2,8.30684397899999));
#241669=CARTESIAN_POINT('Ctrl Pts',(-6.88267376000006,11.6,8.30684397899999));
#241670=CARTESIAN_POINT('Ctrl Pts',(-6.88164809600006,15.2,8.30443237499999));
#241671=CARTESIAN_POINT('Ctrl Pts',(-6.88164809600006,11.6,8.30443237499999));
#241672=CARTESIAN_POINT('Ctrl Pts',(-6.88062272400006,15.2,8.30202713399999));
#241673=CARTESIAN_POINT('Ctrl Pts',(-6.88062272400006,11.6,8.30202713399999));
#241674=CARTESIAN_POINT('Ctrl Pts',(-6.87959765300006,15.2,8.29962826199999));
#241675=CARTESIAN_POINT('Ctrl Pts',(-6.87959765300006,11.6,8.29962826199999));
#241676=CARTESIAN_POINT('Ctrl Pts',(-6.87857289800006,15.2,8.29723576799999));
#241677=CARTESIAN_POINT('Ctrl Pts',(-6.87857289800006,11.6,8.29723576799999));
#241678=CARTESIAN_POINT('Ctrl Pts',(-6.87754847000006,15.2,8.29484965699999));
#241679=CARTESIAN_POINT('Ctrl Pts',(-6.87754847000006,11.6,8.29484965699999));
#241680=CARTESIAN_POINT('Ctrl Pts',(-6.87652438300006,15.2,8.29246993699999));
#241681=CARTESIAN_POINT('Ctrl Pts',(-6.87652438300006,11.6,8.29246993699999));
#241682=CARTESIAN_POINT('Ctrl Pts',(-6.87550064900006,15.2,8.29009661299999));
#241683=CARTESIAN_POINT('Ctrl Pts',(-6.87550064900006,11.6,8.29009661299999));
#241684=CARTESIAN_POINT('Ctrl Pts',(-6.87447728200006,15.2,8.28772969599999));
#241685=CARTESIAN_POINT('Ctrl Pts',(-6.87447728200006,11.6,8.28772969599999));
#241686=CARTESIAN_POINT('Ctrl Pts',(-6.87345429300006,15.2,8.28536918899999));
#241687=CARTESIAN_POINT('Ctrl Pts',(-6.87345429300006,11.6,8.28536918899999));
#241688=CARTESIAN_POINT('Ctrl Pts',(-6.87243169600006,15.2,8.28301510199999));
#241689=CARTESIAN_POINT('Ctrl Pts',(-6.87243169600006,11.6,8.28301510199999));
#241690=CARTESIAN_POINT('Ctrl Pts',(-6.87140950400006,15.2,8.28066743899999));
#241691=CARTESIAN_POINT('Ctrl Pts',(-6.87140950400006,11.6,8.28066743899999));
#241692=CARTESIAN_POINT('Ctrl Pts',(-6.87038772900006,15.2,8.27832621099999));
#241693=CARTESIAN_POINT('Ctrl Pts',(-6.87038772900006,11.6,8.27832621099999));
#241694=CARTESIAN_POINT('Ctrl Pts',(-6.86936638600006,15.2,8.27599142099999));
#241695=CARTESIAN_POINT('Ctrl Pts',(-6.86936638600006,11.6,8.27599142099999));
#241696=CARTESIAN_POINT('Ctrl Pts',(-6.86834548600006,15.2,8.27366307899998));
#241697=CARTESIAN_POINT('Ctrl Pts',(-6.86834548600006,11.6,8.27366307899998));
#241698=CARTESIAN_POINT('Ctrl Pts',(-6.86732504300006,15.2,8.27134118999999));
#241699=CARTESIAN_POINT('Ctrl Pts',(-6.86732504300006,11.6,8.27134118999999));
#241700=CARTESIAN_POINT('Ctrl Pts',(-6.86630507000006,15.2,8.26902576299998));
#241701=CARTESIAN_POINT('Ctrl Pts',(-6.86630507000006,11.6,8.26902576299998));
#241702=CARTESIAN_POINT('Ctrl Pts',(-6.86528558100005,15.2,8.26671680299999));
#241703=CARTESIAN_POINT('Ctrl Pts',(-6.86528558100005,11.6,8.26671680299999));
#241704=CARTESIAN_POINT('Ctrl Pts',(-6.86426658700006,15.2,8.26441431899998));
#241705=CARTESIAN_POINT('Ctrl Pts',(-6.86426658700006,11.6,8.26441431899998));
#241706=CARTESIAN_POINT('Ctrl Pts',(-6.86324810300006,15.2,8.26211831699998));
#241707=CARTESIAN_POINT('Ctrl Pts',(-6.86324810300006,11.6,8.26211831699998));
#241708=CARTESIAN_POINT('Ctrl Pts',(-6.86223014300006,15.2,8.25982880399999));
#241709=CARTESIAN_POINT('Ctrl Pts',(-6.86223014300006,11.6,8.25982880399999));
#241710=CARTESIAN_POINT('Ctrl Pts',(-6.86121271900006,15.2,8.25754578899998));
#241711=CARTESIAN_POINT('Ctrl Pts',(-6.86121271900006,11.6,8.25754578899998));
#241712=CARTESIAN_POINT('Ctrl Pts',(-6.86019584400006,15.2,8.25526927799999));
#241713=CARTESIAN_POINT('Ctrl Pts',(-6.86019584400006,11.6,8.25526927799999));
#241714=CARTESIAN_POINT('Ctrl Pts',(-6.85917953300006,15.2,8.25299927699999));
#241715=CARTESIAN_POINT('Ctrl Pts',(-6.85917953300006,11.6,8.25299927699999));
#241716=CARTESIAN_POINT('Ctrl Pts',(-6.85816379800006,15.2,8.25073579399999));
#241717=CARTESIAN_POINT('Ctrl Pts',(-6.85816379800006,11.6,8.25073579399999));
#241718=CARTESIAN_POINT('Ctrl Pts',(-6.85714865300006,15.2,8.24847883599999));
#241719=CARTESIAN_POINT('Ctrl Pts',(-6.85714865300006,11.6,8.24847883599999));
#241720=CARTESIAN_POINT('Ctrl Pts',(-6.85613411100006,15.2,8.24622841099998));
#241721=CARTESIAN_POINT('Ctrl Pts',(-6.85613411100006,11.6,8.24622841099998));
#241722=CARTESIAN_POINT('Ctrl Pts',(-6.85512018700006,15.2,8.24398452599999));
#241723=CARTESIAN_POINT('Ctrl Pts',(-6.85512018700006,11.6,8.24398452599999));
#241724=CARTESIAN_POINT('Ctrl Pts',(-6.85410689400006,15.2,8.24174718599998));
#241725=CARTESIAN_POINT('Ctrl Pts',(-6.85410689400006,11.6,8.24174718599998));
#241726=CARTESIAN_POINT('Ctrl Pts',(-6.85309424500006,15.2,8.23951640199999));
#241727=CARTESIAN_POINT('Ctrl Pts',(-6.85309424500006,11.6,8.23951640199999));
#241728=CARTESIAN_POINT('Ctrl Pts',(-6.85208225500006,15.2,8.23729217899999));
#241729=CARTESIAN_POINT('Ctrl Pts',(-6.85208225500006,11.6,8.23729217899999));
#241730=CARTESIAN_POINT('Ctrl Pts',(-6.85107093700006,15.2,8.23507452399999));
#241731=CARTESIAN_POINT('Ctrl Pts',(-6.85107093700006,11.6,8.23507452399999));
#241732=CARTESIAN_POINT('Ctrl Pts',(-6.85006030400006,15.2,8.23286344499999));
#241733=CARTESIAN_POINT('Ctrl Pts',(-6.85006030400006,11.6,8.23286344499999));
#241734=CARTESIAN_POINT('Ctrl Pts',(-6.84905037200005,15.2,8.23065894899998));
#241735=CARTESIAN_POINT('Ctrl Pts',(-6.84905037200005,11.6,8.23065894899998));
#241736=CARTESIAN_POINT('Ctrl Pts',(-6.84804115200006,15.2,8.22846104399999));
#241737=CARTESIAN_POINT('Ctrl Pts',(-6.84804115200006,11.6,8.22846104399999));
#241738=CARTESIAN_POINT('Ctrl Pts',(-6.84703266000006,15.2,8.22626973599998));
#241739=CARTESIAN_POINT('Ctrl Pts',(-6.84703266000006,11.6,8.22626973599998));
#241740=CARTESIAN_POINT('Ctrl Pts',(-6.84602491000006,15.2,8.22408503299998));
#241741=CARTESIAN_POINT('Ctrl Pts',(-6.84602491000006,11.6,8.22408503299998));
#241742=CARTESIAN_POINT('Ctrl Pts',(-6.84501791600006,15.2,8.22190694199998));
#241743=CARTESIAN_POINT('Ctrl Pts',(-6.84501791600006,11.6,8.22190694199998));
#241744=CARTESIAN_POINT('Ctrl Pts',(-6.84401169000005,15.2,8.21973546999999));
#241745=CARTESIAN_POINT('Ctrl Pts',(-6.84401169000005,11.6,8.21973546999999));
#241746=CARTESIAN_POINT('Ctrl Pts',(-6.84300624900006,15.2,8.21757062599998));
#241747=CARTESIAN_POINT('Ctrl Pts',(-6.84300624900006,11.6,8.21757062599998));
#241748=CARTESIAN_POINT('Ctrl Pts',(-6.84200160600006,15.2,8.21541241499999));
#241749=CARTESIAN_POINT('Ctrl Pts',(-6.84200160600006,11.6,8.21541241499999));
#241750=CARTESIAN_POINT('Ctrl Pts',(-6.84099777500006,15.2,8.21326084699999));
#241751=CARTESIAN_POINT('Ctrl Pts',(-6.84099777500006,11.6,8.21326084699999));
#241752=CARTESIAN_POINT('Ctrl Pts',(-6.83999477000006,15.2,8.21111592799999));
#241753=CARTESIAN_POINT('Ctrl Pts',(-6.83999477000006,11.6,8.21111592799999));
#241754=CARTESIAN_POINT('Ctrl Pts',(-6.83899260600006,15.2,8.20897766399998));
#241755=CARTESIAN_POINT('Ctrl Pts',(-6.83899260600006,11.6,8.20897766399998));
#241756=CARTESIAN_POINT('Ctrl Pts',(-6.83799129700006,15.2,8.20684606399999));
#241757=CARTESIAN_POINT('Ctrl Pts',(-6.83799129700006,11.6,8.20684606399999));
#241758=CARTESIAN_POINT('Ctrl Pts',(-6.83699085800006,15.2,8.20472113499999));
#241759=CARTESIAN_POINT('Ctrl Pts',(-6.83699085800006,11.6,8.20472113499999));
#241760=CARTESIAN_POINT('Ctrl Pts',(-6.83599130200006,15.2,8.20260288499998));
#241761=CARTESIAN_POINT('Ctrl Pts',(-6.83599130200006,11.6,8.20260288499998));
#241762=CARTESIAN_POINT('Ctrl Pts',(-6.83499264500006,15.2,8.20049131999999));
#241763=CARTESIAN_POINT('Ctrl Pts',(-6.83499264500006,11.6,8.20049131999999));
#241764=CARTESIAN_POINT('Ctrl Pts',(-6.83399490100006,15.2,8.19838644999999));
#241765=CARTESIAN_POINT('Ctrl Pts',(-6.83399490100006,11.6,8.19838644999999));
#241766=CARTESIAN_POINT('Ctrl Pts',(-6.83299808500006,15.2,8.19628827899999));
#241767=CARTESIAN_POINT('Ctrl Pts',(-6.83299808500006,11.6,8.19628827899999));
#241768=CARTESIAN_POINT('Ctrl Pts',(-6.83200221000006,15.2,8.19419681699999));
#241769=CARTESIAN_POINT('Ctrl Pts',(-6.83200221000006,11.6,8.19419681699999));
#241770=CARTESIAN_POINT('Ctrl Pts',(-6.83100729300006,15.2,8.19211206999999));
#241771=CARTESIAN_POINT('Ctrl Pts',(-6.83100729300006,11.6,8.19211206999999));
#241772=CARTESIAN_POINT('Ctrl Pts',(-6.83001334700006,15.2,8.19003404699998));
#241773=CARTESIAN_POINT('Ctrl Pts',(-6.83001334700006,11.6,8.19003404699998));
#241774=CARTESIAN_POINT('Ctrl Pts',(-6.82902038700006,15.2,8.18796275499999));
#241775=CARTESIAN_POINT('Ctrl Pts',(-6.82902038700006,11.6,8.18796275499999));
#241776=CARTESIAN_POINT('Ctrl Pts',(-6.82802842900006,15.2,8.18589820099999));
#241777=CARTESIAN_POINT('Ctrl Pts',(-6.82802842900006,11.6,8.18589820099999));
#241778=CARTESIAN_POINT('Ctrl Pts',(-6.82703748600006,15.2,8.18384039199999));
#241779=CARTESIAN_POINT('Ctrl Pts',(-6.82703748600006,11.6,8.18384039199999));
#241780=CARTESIAN_POINT('Ctrl Pts',(-6.82604757500005,15.2,8.18178933699999));
#241781=CARTESIAN_POINT('Ctrl Pts',(-6.82604757500005,11.6,8.18178933699999));
#241782=CARTESIAN_POINT('Ctrl Pts',(-6.82505871000005,15.2,8.17974504099999));
#241783=CARTESIAN_POINT('Ctrl Pts',(-6.82505871000005,11.6,8.17974504099999));
#241784=CARTESIAN_POINT('Ctrl Pts',(-6.82407090600006,15.2,8.17770751499998));
#241785=CARTESIAN_POINT('Ctrl Pts',(-6.82407090600006,11.6,8.17770751499998));
#241786=CARTESIAN_POINT('Ctrl Pts',(-6.82308417900006,15.2,8.17567676499999));
#241787=CARTESIAN_POINT('Ctrl Pts',(-6.82308417900006,11.6,8.17567676499999));
#241788=CARTESIAN_POINT('Ctrl Pts',(-6.82209854200006,15.2,8.17365279799999));
#241789=CARTESIAN_POINT('Ctrl Pts',(-6.82209854200006,11.6,8.17365279799999));
#241790=CARTESIAN_POINT('Ctrl Pts',(-6.82111401300006,15.2,8.17163562099999));
#241791=CARTESIAN_POINT('Ctrl Pts',(-6.82111401300006,11.6,8.17163562099999));
#241792=CARTESIAN_POINT('Ctrl Pts',(-6.82013060500006,15.2,8.16962524399998));
#241793=CARTESIAN_POINT('Ctrl Pts',(-6.82013060500006,11.6,8.16962524399998));
#241794=CARTESIAN_POINT('Ctrl Pts',(-6.81914833400006,15.2,8.16762167299999));
#241795=CARTESIAN_POINT('Ctrl Pts',(-6.81914833400006,11.6,8.16762167299999));
#241796=CARTESIAN_POINT('Ctrl Pts',(-6.81816721500006,15.2,8.16562491699998));
#241797=CARTESIAN_POINT('Ctrl Pts',(-6.81816721500006,11.6,8.16562491699998));
#241798=CARTESIAN_POINT('Ctrl Pts',(-6.81718726400006,15.2,8.16363498099999));
#241799=CARTESIAN_POINT('Ctrl Pts',(-6.81718726400006,11.6,8.16363498099999));
#241800=CARTESIAN_POINT('Ctrl Pts',(-6.81620849600006,15.2,8.16165187399999));
#241801=CARTESIAN_POINT('Ctrl Pts',(-6.81620849600006,11.6,8.16165187399999));
#241802=CARTESIAN_POINT('Ctrl Pts',(-6.81523092700006,15.2,8.15967560499999));
#241803=CARTESIAN_POINT('Ctrl Pts',(-6.81523092700006,11.6,8.15967560499999));
#241804=CARTESIAN_POINT('Ctrl Pts',(-6.81425457300006,15.2,8.15770617999998));
#241805=CARTESIAN_POINT('Ctrl Pts',(-6.81425457300006,11.6,8.15770617999998));
#241806=CARTESIAN_POINT('Ctrl Pts',(-6.81327944800006,15.2,8.15574360799998));
#241807=CARTESIAN_POINT('Ctrl Pts',(-6.81327944800006,11.6,8.15574360799998));
#241808=CARTESIAN_POINT('Ctrl Pts',(-6.81230556900006,15.2,8.15378789499999));
#241809=CARTESIAN_POINT('Ctrl Pts',(-6.81230556900006,11.6,8.15378789499999));
#241810=CARTESIAN_POINT('Ctrl Pts',(-6.81133295100006,15.2,8.15183904999999));
#241811=CARTESIAN_POINT('Ctrl Pts',(-6.81133295100006,11.6,8.15183904999999));
#241812=CARTESIAN_POINT('Ctrl Pts',(-6.81036161000006,15.2,8.14989708099999));
#241813=CARTESIAN_POINT('Ctrl Pts',(-6.81036161000006,11.6,8.14989708099999));
#241814=CARTESIAN_POINT('Ctrl Pts',(-6.80939156200006,15.2,8.14796199499998));
#241815=CARTESIAN_POINT('Ctrl Pts',(-6.80939156200006,11.6,8.14796199499998));
#241816=CARTESIAN_POINT('Ctrl Pts',(-6.80842282200006,15.2,8.14603380099998));
#241817=CARTESIAN_POINT('Ctrl Pts',(-6.80842282200006,11.6,8.14603380099998));
#241818=CARTESIAN_POINT('Ctrl Pts',(-6.80745540800006,15.2,8.14411250399999));
#241819=CARTESIAN_POINT('Ctrl Pts',(-6.80745540800006,11.6,8.14411250399999));
#241820=CARTESIAN_POINT('Ctrl Pts',(-6.80648933300006,15.2,8.14219811399998));
#241821=CARTESIAN_POINT('Ctrl Pts',(-6.80648933300006,11.6,8.14219811399998));
#241822=CARTESIAN_POINT('Ctrl Pts',(-6.80552461600006,15.2,8.14029063899999));
#241823=CARTESIAN_POINT('Ctrl Pts',(-6.80552461600006,11.6,8.14029063899999));
#241824=CARTESIAN_POINT('Ctrl Pts',(-6.80456127200006,15.2,8.13839008599999));
#241825=CARTESIAN_POINT('Ctrl Pts',(-6.80456127200006,11.6,8.13839008599999));
#241826=CARTESIAN_POINT('Ctrl Pts',(-6.80359931600006,15.2,8.13649646299999));
#241827=CARTESIAN_POINT('Ctrl Pts',(-6.80359931600006,11.6,8.13649646299999));
#241828=CARTESIAN_POINT('Ctrl Pts',(-6.80263876600006,15.2,8.13460977699999));
#241829=CARTESIAN_POINT('Ctrl Pts',(-6.80263876600006,11.6,8.13460977699999));
#241830=CARTESIAN_POINT('Ctrl Pts',(-6.80167963800006,15.2,8.13273003799999));
#241831=CARTESIAN_POINT('Ctrl Pts',(-6.80167963800006,11.6,8.13273003799999));
#241832=CARTESIAN_POINT('Ctrl Pts',(-6.80072194600006,15.2,8.13085725199999));
#241833=CARTESIAN_POINT('Ctrl Pts',(-6.80072194600006,11.6,8.13085725199999));
#241834=CARTESIAN_POINT('Ctrl Pts',(-6.79976571000006,15.2,8.12899142899998));
#241835=CARTESIAN_POINT('Ctrl Pts',(-6.79976571000006,11.6,8.12899142899998));
#241836=CARTESIAN_POINT('Ctrl Pts',(-6.79881094300006,15.2,8.12713257299999));
#241837=CARTESIAN_POINT('Ctrl Pts',(-6.79881094300006,11.6,8.12713257299999));
#241838=CARTESIAN_POINT('Ctrl Pts',(-6.79785766400006,15.2,8.12528069599999));
#241839=CARTESIAN_POINT('Ctrl Pts',(-6.79785766400006,11.6,8.12528069599999));
#241840=CARTESIAN_POINT('Ctrl Pts',(-6.79690588900006,15.2,8.12343580499999));
#241841=CARTESIAN_POINT('Ctrl Pts',(-6.79690588900006,11.6,8.12343580499999));
#241842=CARTESIAN_POINT('Ctrl Pts',(-6.79595563300006,15.2,8.12159790499998));
#241843=CARTESIAN_POINT('Ctrl Pts',(-6.79595563300006,11.6,8.12159790499998));
#241844=CARTESIAN_POINT('Ctrl Pts',(-6.79500691600006,15.2,8.11976700799999));
#241845=CARTESIAN_POINT('Ctrl Pts',(-6.79500691600006,11.6,8.11976700799999));
#241846=CARTESIAN_POINT('Ctrl Pts',(-6.79405975100006,15.2,8.11794311999999));
#241847=CARTESIAN_POINT('Ctrl Pts',(-6.79405975100006,11.6,8.11794311999999));
#241848=CARTESIAN_POINT('Ctrl Pts',(-6.79311415800006,15.2,8.11612624899999));
#241849=CARTESIAN_POINT('Ctrl Pts',(-6.79311415800006,11.6,8.11612624899999));
#241850=CARTESIAN_POINT('Ctrl Pts',(-6.79217015000006,15.2,8.11431640399999));
#241851=CARTESIAN_POINT('Ctrl Pts',(-6.79217015000006,11.6,8.11431640399999));
#241852=CARTESIAN_POINT('Ctrl Pts',(-6.79122774800006,15.2,8.11251359099998));
#241853=CARTESIAN_POINT('Ctrl Pts',(-6.79122774800006,11.6,8.11251359099998));
#241854=CARTESIAN_POINT('Ctrl Pts',(-6.79028696800006,15.2,8.11071782099998));
#241855=CARTESIAN_POINT('Ctrl Pts',(-6.79028696800006,11.6,8.11071782099998));
#241856=CARTESIAN_POINT('Ctrl Pts',(-6.78934782500006,15.2,8.10892909799998));
#241857=CARTESIAN_POINT('Ctrl Pts',(-6.78934782500006,11.6,8.10892909799998));
#241858=CARTESIAN_POINT('Ctrl Pts',(-6.78841033800006,15.2,8.10714743499998));
#241859=CARTESIAN_POINT('Ctrl Pts',(-6.78841033800006,11.6,8.10714743499998));
#241860=CARTESIAN_POINT('Ctrl Pts',(-6.78747452300006,15.2,8.10537283699999));
#241861=CARTESIAN_POINT('Ctrl Pts',(-6.78747452300006,11.6,8.10537283699999));
#241862=CARTESIAN_POINT('Ctrl Pts',(-6.78654039900006,15.2,8.10360531199999));
#241863=CARTESIAN_POINT('Ctrl Pts',(-6.78654039900006,11.6,8.10360531199999));
#241864=CARTESIAN_POINT('Ctrl Pts',(-6.78560798200006,15.2,8.10184486899999));
#241865=CARTESIAN_POINT('Ctrl Pts',(-6.78560798200006,11.6,8.10184486899999));
#241866=CARTESIAN_POINT('Ctrl Pts',(-6.78467728900006,15.2,8.10009151699998));
#241867=CARTESIAN_POINT('Ctrl Pts',(-6.78467728900006,11.6,8.10009151699998));
#241868=CARTESIAN_POINT('Ctrl Pts',(-6.78374833800006,15.2,8.09834526099999));
#241869=CARTESIAN_POINT('Ctrl Pts',(-6.78374833800006,11.6,8.09834526099999));
#241870=CARTESIAN_POINT('Ctrl Pts',(-6.78282114600006,15.2,8.09660611299999));
#241871=CARTESIAN_POINT('Ctrl Pts',(-6.78282114600006,11.6,8.09660611299999));
#241872=CARTESIAN_POINT('Ctrl Pts',(-6.78189573200005,15.2,8.09487407999999));
#241873=CARTESIAN_POINT('Ctrl Pts',(-6.78189573200005,11.6,8.09487407999999));
#241874=CARTESIAN_POINT('Ctrl Pts',(-6.78097211100006,15.2,8.09314916899999));
#241875=CARTESIAN_POINT('Ctrl Pts',(-6.78097211100006,11.6,8.09314916899999));
#241876=CARTESIAN_POINT('Ctrl Pts',(-6.78005030300006,15.2,8.09143138899999));
#241877=CARTESIAN_POINT('Ctrl Pts',(-6.78005030300006,11.6,8.09143138899999));
#241878=CARTESIAN_POINT('Ctrl Pts',(-6.77913032500006,15.2,8.08972074899999));
#241879=CARTESIAN_POINT('Ctrl Pts',(-6.77913032500006,11.6,8.08972074899999));
#241880=CARTESIAN_POINT('Ctrl Pts',(-6.77821219500006,15.2,8.08801725599999));
#241881=CARTESIAN_POINT('Ctrl Pts',(-6.77821219500006,11.6,8.08801725599999));
#241882=CARTESIAN_POINT('Ctrl Pts',(-6.77729593100006,15.2,8.08632091799998));
#241883=CARTESIAN_POINT('Ctrl Pts',(-6.77729593100006,11.6,8.08632091799998));
#241884=CARTESIAN_POINT('Ctrl Pts',(-6.77638155000006,15.2,8.08463174499998));
#241885=CARTESIAN_POINT('Ctrl Pts',(-6.77638155000006,11.6,8.08463174499998));
#241886=CARTESIAN_POINT('Ctrl Pts',(-6.77546907200006,15.2,8.08294974399999));
#241887=CARTESIAN_POINT('Ctrl Pts',(-6.77546907200006,11.6,8.08294974399999));
#241888=CARTESIAN_POINT('Ctrl Pts',(-6.77455851200006,15.2,8.08127492399999));
#241889=CARTESIAN_POINT('Ctrl Pts',(-6.77455851200006,11.6,8.08127492399999));
#241890=CARTESIAN_POINT('Ctrl Pts',(-6.77364989000006,15.2,8.07960729299998));
#241891=CARTESIAN_POINT('Ctrl Pts',(-6.77364989000006,11.6,8.07960729299998));
#241892=CARTESIAN_POINT('Ctrl Pts',(-6.77274322500006,15.2,8.07794685999998));
#241893=CARTESIAN_POINT('Ctrl Pts',(-6.77274322500006,11.6,8.07794685999998));
#241894=CARTESIAN_POINT('Ctrl Pts',(-6.77183853400006,15.2,8.07629363199998));
#241895=CARTESIAN_POINT('Ctrl Pts',(-6.77183853400006,11.6,8.07629363199998));
#241896=CARTESIAN_POINT('Ctrl Pts',(-6.77093583500006,15.2,8.07464761899999));
#241897=CARTESIAN_POINT('Ctrl Pts',(-6.77093583500006,11.6,8.07464761899999));
#241898=CARTESIAN_POINT('Ctrl Pts',(-6.77003514900006,15.2,8.07300882799998));
#241899=CARTESIAN_POINT('Ctrl Pts',(-6.77003514900006,11.6,8.07300882799998));
#241900=CARTESIAN_POINT('Ctrl Pts',(-6.76913649100006,15.2,8.07137726799999));
#241901=CARTESIAN_POINT('Ctrl Pts',(-6.76913649100006,11.6,8.07137726799999));
#241902=CARTESIAN_POINT('Ctrl Pts',(-6.76823988100006,15.2,8.06975294799999));
#241903=CARTESIAN_POINT('Ctrl Pts',(-6.76823988100006,11.6,8.06975294799999));
#241904=CARTESIAN_POINT('Ctrl Pts',(-6.76734533900006,15.2,8.06813587699999));
#241905=CARTESIAN_POINT('Ctrl Pts',(-6.76734533900006,11.6,8.06813587699999));
#241906=CARTESIAN_POINT('Ctrl Pts',(-6.76645288200006,15.2,8.06652606199999));
#241907=CARTESIAN_POINT('Ctrl Pts',(-6.76645288200006,11.6,8.06652606199999));
#241908=CARTESIAN_POINT('Ctrl Pts',(-6.76556252900006,15.2,8.06492351199999));
#241909=CARTESIAN_POINT('Ctrl Pts',(-6.76556252900006,11.6,8.06492351199999));
#241910=CARTESIAN_POINT('Ctrl Pts',(-6.76467429900006,15.2,8.06332823599998));
#241911=CARTESIAN_POINT('Ctrl Pts',(-6.76467429900006,11.6,8.06332823599998));
#241912=CARTESIAN_POINT('Ctrl Pts',(-6.76378821300006,15.2,8.06174024099998));
#241913=CARTESIAN_POINT('Ctrl Pts',(-6.76378821300006,11.6,8.06174024099998));
#241914=CARTESIAN_POINT('Ctrl Pts',(-6.76290428600006,15.2,8.06015953799999));
#241915=CARTESIAN_POINT('Ctrl Pts',(-6.76290428600006,11.6,8.06015953799999));
#241916=CARTESIAN_POINT('Ctrl Pts',(-6.76202253900006,15.2,8.05858613399998));
#241917=CARTESIAN_POINT('Ctrl Pts',(-6.76202253900006,11.6,8.05858613399998));
#241918=CARTESIAN_POINT('Ctrl Pts',(-6.76114299300006,15.2,8.05702003799999));
#241919=CARTESIAN_POINT('Ctrl Pts',(-6.76114299300006,11.6,8.05702003799999));
#241920=CARTESIAN_POINT('Ctrl Pts',(-6.76026566400005,15.2,8.05546125899999));
#241921=CARTESIAN_POINT('Ctrl Pts',(-6.76026566400005,11.6,8.05546125899999));
#241922=CARTESIAN_POINT('Ctrl Pts',(-6.75939057400006,15.2,8.05390980499999));
#241923=CARTESIAN_POINT('Ctrl Pts',(-6.75939057400006,11.6,8.05390980499999));
#241924=CARTESIAN_POINT('Ctrl Pts',(-6.75851774100006,15.2,8.05236568499998));
#241925=CARTESIAN_POINT('Ctrl Pts',(-6.75851774100006,11.6,8.05236568499998));
#241926=CARTESIAN_POINT('Ctrl Pts',(-6.75764718400006,15.2,8.05082890799999));
#241927=CARTESIAN_POINT('Ctrl Pts',(-6.75764718400006,11.6,8.05082890799999));
#241928=CARTESIAN_POINT('Ctrl Pts',(-6.75677892300006,15.2,8.04929948199998));
#241929=CARTESIAN_POINT('Ctrl Pts',(-6.75677892300006,11.6,8.04929948199998));
#241930=CARTESIAN_POINT('Ctrl Pts',(-6.75591297800006,15.2,8.04777741599998));
#241931=CARTESIAN_POINT('Ctrl Pts',(-6.75591297800006,11.6,8.04777741599998));
#241932=CARTESIAN_POINT('Ctrl Pts',(-6.75504936900006,15.2,8.04626271899998));
#241933=CARTESIAN_POINT('Ctrl Pts',(-6.75504936900006,11.6,8.04626271899998));
#241934=CARTESIAN_POINT('Ctrl Pts',(-6.75418811500006,15.2,8.04475539999999));
#241935=CARTESIAN_POINT('Ctrl Pts',(-6.75418811500006,11.6,8.04475539999999));
#241936=CARTESIAN_POINT('Ctrl Pts',(-6.75332923600005,15.2,8.04325546699998));
#241937=CARTESIAN_POINT('Ctrl Pts',(-6.75332923600005,11.6,8.04325546699998));
#241938=CARTESIAN_POINT('Ctrl Pts',(-6.75247275200006,15.2,8.04176292999998));
#241939=CARTESIAN_POINT('Ctrl Pts',(-6.75247275200006,11.6,8.04176292999998));
#241940=CARTESIAN_POINT('Ctrl Pts',(-6.75161868200005,15.2,8.04027779599998));
#241941=CARTESIAN_POINT('Ctrl Pts',(-6.75161868200005,11.6,8.04027779599998));
#241942=CARTESIAN_POINT('Ctrl Pts',(-6.75076704800006,15.2,8.03880007599999));
#241943=CARTESIAN_POINT('Ctrl Pts',(-6.75076704800006,11.6,8.03880007599999));
#241944=CARTESIAN_POINT('Ctrl Pts',(-6.74991786900006,15.2,8.03732977699998));
#241945=CARTESIAN_POINT('Ctrl Pts',(-6.74991786900006,11.6,8.03732977699998));
#241946=CARTESIAN_POINT('Ctrl Pts',(-6.74907116500005,15.2,8.03586690899999));
#241947=CARTESIAN_POINT('Ctrl Pts',(-6.74907116500005,11.6,8.03586690899999));
#241948=CARTESIAN_POINT('Ctrl Pts',(-6.74822695800006,15.2,8.03441148099999));
#241949=CARTESIAN_POINT('Ctrl Pts',(-6.74822695800006,11.6,8.03441148099999));
#241950=CARTESIAN_POINT('Ctrl Pts',(-6.74738526500006,15.2,8.03296350199999));
#241951=CARTESIAN_POINT('Ctrl Pts',(-6.74738526500006,11.6,8.03296350199999));
#241952=CARTESIAN_POINT('Ctrl Pts',(-6.74654611000006,15.2,8.03152297999999));
#241953=CARTESIAN_POINT('Ctrl Pts',(-6.74654611000006,11.6,8.03152297999999));
#241954=CARTESIAN_POINT('Ctrl Pts',(-6.74570951200006,15.2,8.03008992499999));
#241955=CARTESIAN_POINT('Ctrl Pts',(-6.74570951200006,11.6,8.03008992499999));
#241956=CARTESIAN_POINT('Ctrl Pts',(-6.74487549200006,15.2,8.02866434499999));
#241957=CARTESIAN_POINT('Ctrl Pts',(-6.74487549200006,11.6,8.02866434499999));
#241958=CARTESIAN_POINT('Ctrl Pts',(-6.74404407000006,15.2,8.02724625099999));
#241959=CARTESIAN_POINT('Ctrl Pts',(-6.74404407000006,11.6,8.02724625099999));
#241960=CARTESIAN_POINT('Ctrl Pts',(-6.74321526700006,15.2,8.02583564899999));
#241961=CARTESIAN_POINT('Ctrl Pts',(-6.74321526700006,11.6,8.02583564899999));
#241962=CARTESIAN_POINT('Ctrl Pts',(-6.74238910500006,15.2,8.02443255099998));
#241963=CARTESIAN_POINT('Ctrl Pts',(-6.74238910500006,11.6,8.02443255099998));
#241964=CARTESIAN_POINT('Ctrl Pts',(-6.74156560400006,15.2,8.02303696499998));
#241965=CARTESIAN_POINT('Ctrl Pts',(-6.74156560400006,11.6,8.02303696499998));
#241966=CARTESIAN_POINT('Ctrl Pts',(-6.74074478500006,15.2,8.02164889999998));
#241967=CARTESIAN_POINT('Ctrl Pts',(-6.74074478500006,11.6,8.02164889999998));
#241968=CARTESIAN_POINT('Ctrl Pts',(-6.73992667000006,15.2,8.02026836499999));
#241969=CARTESIAN_POINT('Ctrl Pts',(-6.73992667000006,11.6,8.02026836499999));
#241970=CARTESIAN_POINT('Ctrl Pts',(-6.73911127900006,15.2,8.01889536999998));
#241971=CARTESIAN_POINT('Ctrl Pts',(-6.73911127900006,11.6,8.01889536999998));
#241972=CARTESIAN_POINT('Ctrl Pts',(-6.73829863500006,15.2,8.01752992299999));
#241973=CARTESIAN_POINT('Ctrl Pts',(-6.73829863500006,11.6,8.01752992299999));
#241974=CARTESIAN_POINT('Ctrl Pts',(-6.73748875900006,15.2,8.01617203399999));
#241975=CARTESIAN_POINT('Ctrl Pts',(-6.73748875900006,11.6,8.01617203399999));
#241976=CARTESIAN_POINT('Ctrl Pts',(-6.73668167000006,15.2,8.01482171199999));
#241977=CARTESIAN_POINT('Ctrl Pts',(-6.73668167000006,11.6,8.01482171199999));
#241978=CARTESIAN_POINT('Ctrl Pts',(-6.73587739300006,15.2,8.01347896699999));
#241979=CARTESIAN_POINT('Ctrl Pts',(-6.73587739300006,11.6,8.01347896699999));
#241980=CARTESIAN_POINT('Ctrl Pts',(-6.73507594800006,15.2,8.01214380699999));
#241981=CARTESIAN_POINT('Ctrl Pts',(-6.73507594800006,11.6,8.01214380699999));
#241982=CARTESIAN_POINT('Ctrl Pts',(-6.73427735700006,15.2,8.01081624299999));
#241983=CARTESIAN_POINT('Ctrl Pts',(-6.73427735700006,11.6,8.01081624299999));
#241984=CARTESIAN_POINT('Ctrl Pts',(-6.73348164200006,15.2,8.00949628199999));
#241985=CARTESIAN_POINT('Ctrl Pts',(-6.73348164200006,11.6,8.00949628199999));
#241986=CARTESIAN_POINT('Ctrl Pts',(-6.73268882400006,15.2,8.00818393499998));
#241987=CARTESIAN_POINT('Ctrl Pts',(-6.73268882400006,11.6,8.00818393499998));
#241988=CARTESIAN_POINT('Ctrl Pts',(-6.73189892800006,15.2,8.00687921199999));
#241989=CARTESIAN_POINT('Ctrl Pts',(-6.73189892800006,11.6,8.00687921199999));
#241990=CARTESIAN_POINT('Ctrl Pts',(-6.73111197300006,15.2,8.00558212099999));
#241991=CARTESIAN_POINT('Ctrl Pts',(-6.73111197300006,11.6,8.00558212099999));
#241992=CARTESIAN_POINT('Ctrl Pts',(-6.73032798300006,15.2,8.00429267199998));
#241993=CARTESIAN_POINT('Ctrl Pts',(-6.73032798300006,11.6,8.00429267199998));
#241994=CARTESIAN_POINT('Ctrl Pts',(-6.72954697900006,15.2,8.00301087499999));
#241995=CARTESIAN_POINT('Ctrl Pts',(-6.72954697900006,11.6,8.00301087499999));
#241996=CARTESIAN_POINT('Ctrl Pts',(-6.72876898500006,15.2,8.00173673899998));
#241997=CARTESIAN_POINT('Ctrl Pts',(-6.72876898500006,11.6,8.00173673899998));
#241998=CARTESIAN_POINT('Ctrl Pts',(-6.72799402200006,15.2,8.00047027299998));
#241999=CARTESIAN_POINT('Ctrl Pts',(-6.72799402200006,11.6,8.00047027299998));
#242000=CARTESIAN_POINT('Ctrl Pts',(-6.72722211500006,15.2,7.99921148699998));
#242001=CARTESIAN_POINT('Ctrl Pts',(-6.72722211500006,11.6,7.99921148699998));
#242002=CARTESIAN_POINT('Ctrl Pts',(-6.72645328300006,15.2,7.99796039199999));
#242003=CARTESIAN_POINT('Ctrl Pts',(-6.72645328300006,11.6,7.99796039199999));
#242004=CARTESIAN_POINT('Ctrl Pts',(-6.72568755300006,15.2,7.99671699499999));
#242005=CARTESIAN_POINT('Ctrl Pts',(-6.72568755300006,11.6,7.99671699499999));
#242006=CARTESIAN_POINT('Ctrl Pts',(-6.72492494500006,15.2,7.99548130699999));
#242007=CARTESIAN_POINT('Ctrl Pts',(-6.72492494500006,11.6,7.99548130699999));
#242008=CARTESIAN_POINT('Ctrl Pts',(-6.72416548300006,15.2,7.99425333899999));
#242009=CARTESIAN_POINT('Ctrl Pts',(-6.72416548300006,11.6,7.99425333899999));
#242010=CARTESIAN_POINT('Ctrl Pts',(-6.72340919000006,15.2,7.99303309799999));
#242011=CARTESIAN_POINT('Ctrl Pts',(-6.72340919000006,11.6,7.99303309799999));
#242012=CARTESIAN_POINT('Ctrl Pts',(-6.72265609000006,15.2,7.99182059499999));
#242013=CARTESIAN_POINT('Ctrl Pts',(-6.72265609000006,11.6,7.99182059499999));
#242014=CARTESIAN_POINT('Ctrl Pts',(-6.72190620500006,15.2,7.99061584099999));
#242015=CARTESIAN_POINT('Ctrl Pts',(-6.72190620500006,11.6,7.99061584099999));
#242016=CARTESIAN_POINT('Ctrl Pts',(-6.72115955900006,15.2,7.98941884399999));
#242017=CARTESIAN_POINT('Ctrl Pts',(-6.72115955900006,11.6,7.98941884399999));
#242018=CARTESIAN_POINT('Ctrl Pts',(-6.72041617600006,15.2,7.98822961399999));
#242019=CARTESIAN_POINT('Ctrl Pts',(-6.72041617600006,11.6,7.98822961399999));
#242020=CARTESIAN_POINT('Ctrl Pts',(-6.71967608100006,15.2,7.98704816199999));
#242021=CARTESIAN_POINT('Ctrl Pts',(-6.71967608100006,11.6,7.98704816199999));
#242022=CARTESIAN_POINT('Ctrl Pts',(-6.71893929400006,15.2,7.98587449599999));
#242023=CARTESIAN_POINT('Ctrl Pts',(-6.71893929400006,11.6,7.98587449599999));
#242024=CARTESIAN_POINT('Ctrl Pts',(-6.71820584200006,15.2,7.98470862799999));
#242025=CARTESIAN_POINT('Ctrl Pts',(-6.71820584200006,11.6,7.98470862799999));
#242026=CARTESIAN_POINT('Ctrl Pts',(-6.71747574700006,15.2,7.98355056599998));
#242027=CARTESIAN_POINT('Ctrl Pts',(-6.71747574700006,11.6,7.98355056599998));
#242028=CARTESIAN_POINT('Ctrl Pts',(-6.71674903500006,15.2,7.98240032199999));
#242029=CARTESIAN_POINT('Ctrl Pts',(-6.71674903500006,11.6,7.98240032199999));
#242030=CARTESIAN_POINT('Ctrl Pts',(-6.71602572900006,15.2,7.98125790399999));
#242031=CARTESIAN_POINT('Ctrl Pts',(-6.71602572900006,11.6,7.98125790399999));
#242032=CARTESIAN_POINT('Ctrl Pts',(-6.71530585400006,15.2,7.98012332299999));
#242033=CARTESIAN_POINT('Ctrl Pts',(-6.71530585400006,11.6,7.98012332299999));
#242034=CARTESIAN_POINT('Ctrl Pts',(-6.71458943400006,15.2,7.97899658999999));
#242035=CARTESIAN_POINT('Ctrl Pts',(-6.71458943400006,11.6,7.97899658999999));
#242036=CARTESIAN_POINT('Ctrl Pts',(-6.71387649200006,15.2,7.97787771299999));
#242037=CARTESIAN_POINT('Ctrl Pts',(-6.71387649200006,11.6,7.97787771299999));
#242038=CARTESIAN_POINT('Ctrl Pts',(-6.71316705500006,15.2,7.97676670399999));
#242039=CARTESIAN_POINT('Ctrl Pts',(-6.71316705500006,11.6,7.97676670399999));
#242040=CARTESIAN_POINT('Ctrl Pts',(-6.71246114700006,15.2,7.97566357099999));
#242041=CARTESIAN_POINT('Ctrl Pts',(-6.71246114700006,11.6,7.97566357099999));
#242042=CARTESIAN_POINT('Ctrl Pts',(-6.71175879300006,15.2,7.97456832599998));
#242043=CARTESIAN_POINT('Ctrl Pts',(-6.71175879300006,11.6,7.97456832599998));
#242044=CARTESIAN_POINT('Ctrl Pts',(-6.71106001700006,15.2,7.97348097999999));
#242045=CARTESIAN_POINT('Ctrl Pts',(-6.71106001700006,11.6,7.97348097999999));
#242046=CARTESIAN_POINT('Ctrl Pts',(-6.71036484500006,15.2,7.97240153999999));
#242047=CARTESIAN_POINT('Ctrl Pts',(-6.71036484500006,11.6,7.97240153999999));
#242048=CARTESIAN_POINT('Ctrl Pts',(-6.70967330200006,15.2,7.97133001899999));
#242049=CARTESIAN_POINT('Ctrl Pts',(-6.70967330200006,11.6,7.97133001899999));
#242050=CARTESIAN_POINT('Ctrl Pts',(-6.70898541300006,15.2,7.97026642699999));
#242051=CARTESIAN_POINT('Ctrl Pts',(-6.70898541300006,11.6,7.97026642699999));
#242052=CARTESIAN_POINT('Ctrl Pts',(-6.70830120400006,15.2,7.96921077299999));
#242053=CARTESIAN_POINT('Ctrl Pts',(-6.70830120400006,11.6,7.96921077299999));
#242054=CARTESIAN_POINT('Ctrl Pts',(-6.70762070000006,15.2,7.96816306899998));
#242055=CARTESIAN_POINT('Ctrl Pts',(-6.70762070000006,11.6,7.96816306899998));
#242056=CARTESIAN_POINT('Ctrl Pts',(-6.70694392700006,15.2,7.96712332499999));
#242057=CARTESIAN_POINT('Ctrl Pts',(-6.70694392700006,11.6,7.96712332499999));
#242058=CARTESIAN_POINT('Ctrl Pts',(-6.70627091100005,15.2,7.96609154899999));
#242059=CARTESIAN_POINT('Ctrl Pts',(-6.70627091100005,11.6,7.96609154899999));
#242060=CARTESIAN_POINT('Ctrl Pts',(-6.70560167800006,15.2,7.96506775499999));
#242061=CARTESIAN_POINT('Ctrl Pts',(-6.70560167800006,11.6,7.96506775499999));
#242062=CARTESIAN_POINT('Ctrl Pts',(-6.70493625300006,15.2,7.96405195199998));
#242063=CARTESIAN_POINT('Ctrl Pts',(-6.70493625300006,11.6,7.96405195199998));
#242064=CARTESIAN_POINT('Ctrl Pts',(-6.70427466300006,15.2,7.96304415099998));
#242065=CARTESIAN_POINT('Ctrl Pts',(-6.70427466300006,11.6,7.96304415099998));
#242066=CARTESIAN_POINT('Ctrl Pts',(-6.70361693400006,15.2,7.96204436099998));
#242067=CARTESIAN_POINT('Ctrl Pts',(-6.70361693400006,11.6,7.96204436099998));
#242068=CARTESIAN_POINT('Ctrl Pts',(-6.70296309400006,15.2,7.96105259399998));
#242069=CARTESIAN_POINT('Ctrl Pts',(-6.70296309400006,11.6,7.96105259399998));
#242070=CARTESIAN_POINT('Ctrl Pts',(-6.70231316700006,15.2,7.96006886099998));
#242071=CARTESIAN_POINT('Ctrl Pts',(-6.70231316700006,11.6,7.96006886099998));
#242072=CARTESIAN_POINT('Ctrl Pts',(-6.70166718000006,15.2,7.95909317099999));
#242073=CARTESIAN_POINT('Ctrl Pts',(-6.70166718000006,11.6,7.95909317099999));
#242074=CARTESIAN_POINT('Ctrl Pts',(-6.70102516100005,15.2,7.95812553699999));
#242075=CARTESIAN_POINT('Ctrl Pts',(-6.70102516100005,11.6,7.95812553699999));
#242076=CARTESIAN_POINT('Ctrl Pts',(-6.70038713700006,15.2,7.95716596799998));
#242077=CARTESIAN_POINT('Ctrl Pts',(-6.70038713700006,11.6,7.95716596799998));
#242078=CARTESIAN_POINT('Ctrl Pts',(-6.69975313400006,15.2,7.95621447499999));
#242079=CARTESIAN_POINT('Ctrl Pts',(-6.69975313400006,11.6,7.95621447499999));
#242080=CARTESIAN_POINT('Ctrl Pts',(-6.69912317900006,15.2,7.95527106999998));
#242081=CARTESIAN_POINT('Ctrl Pts',(-6.69912317900006,11.6,7.95527106999998));
#242082=CARTESIAN_POINT('Ctrl Pts',(-6.69849730200006,15.2,7.95433576299998));
#242083=CARTESIAN_POINT('Ctrl Pts',(-6.69849730200006,11.6,7.95433576299998));
#242084=CARTESIAN_POINT('Ctrl Pts',(-6.69787552700006,15.2,7.95340856399999));
#242085=CARTESIAN_POINT('Ctrl Pts',(-6.69787552700006,11.6,7.95340856399999));
#242086=CARTESIAN_POINT('Ctrl Pts',(-6.69725788400005,15.2,7.95248948499999));
#242087=CARTESIAN_POINT('Ctrl Pts',(-6.69725788400005,11.6,7.95248948499999));
#242088=CARTESIAN_POINT('Ctrl Pts',(-6.69664439800005,15.2,7.95157853799999));
#242089=CARTESIAN_POINT('Ctrl Pts',(-6.69664439800005,11.6,7.95157853799999));
#242090=CARTESIAN_POINT('Ctrl Pts',(-6.69603510100006,15.2,7.95067573199999));
#242091=CARTESIAN_POINT('Ctrl Pts',(-6.69603510100006,11.6,7.95067573199999));
#242092=CARTESIAN_POINT('Ctrl Pts',(-6.69543001600006,15.2,7.94978107899999));
#242093=CARTESIAN_POINT('Ctrl Pts',(-6.69543001600006,11.6,7.94978107899999));
#242094=CARTESIAN_POINT('Ctrl Pts',(-6.69482917600006,15.2,7.94889459099998));
#242095=CARTESIAN_POINT('Ctrl Pts',(-6.69482917600006,11.6,7.94889459099998));
#242096=CARTESIAN_POINT('Ctrl Pts',(-6.69423260600006,15.2,7.94801627699999));
#242097=CARTESIAN_POINT('Ctrl Pts',(-6.69423260600006,11.6,7.94801627699999));
#242098=CARTESIAN_POINT('Ctrl Pts',(-6.69364033500006,15.2,7.94714614999998));
#242099=CARTESIAN_POINT('Ctrl Pts',(-6.69364033500006,11.6,7.94714614999998));
#242100=CARTESIAN_POINT('Ctrl Pts',(-6.69305239300006,15.2,7.94628422099999));
#242101=CARTESIAN_POINT('Ctrl Pts',(-6.69305239300006,11.6,7.94628422099999));
#242102=CARTESIAN_POINT('Ctrl Pts',(-6.69246880700006,15.2,7.94543049999999));
#242103=CARTESIAN_POINT('Ctrl Pts',(-6.69246880700006,11.6,7.94543049999999));
#242104=CARTESIAN_POINT('Ctrl Pts',(-6.69188960600006,15.2,7.94458499899999));
#242105=CARTESIAN_POINT('Ctrl Pts',(-6.69188960600006,11.6,7.94458499899999));
#242106=CARTESIAN_POINT('Ctrl Pts',(-6.69131482100005,15.2,7.94374772999999));
#242107=CARTESIAN_POINT('Ctrl Pts',(-6.69131482100005,11.6,7.94374772999999));
#242108=CARTESIAN_POINT('Ctrl Pts',(-6.69074447800006,15.2,7.94291870399999));
#242109=CARTESIAN_POINT('Ctrl Pts',(-6.69074447800006,11.6,7.94291870399999));
#242110=CARTESIAN_POINT('Ctrl Pts',(-6.69017860900006,15.2,7.94209793299999));
#242111=CARTESIAN_POINT('Ctrl Pts',(-6.69017860900006,11.6,7.94209793299999));
#242112=CARTESIAN_POINT('Ctrl Pts',(-6.68961724200006,15.2,7.94128542699998));
#242113=CARTESIAN_POINT('Ctrl Pts',(-6.68961724200006,11.6,7.94128542699998));
#242114=CARTESIAN_POINT('Ctrl Pts',(-6.68906040700006,15.2,7.94048119799999));
#242115=CARTESIAN_POINT('Ctrl Pts',(-6.68906040700006,11.6,7.94048119799999));
#242116=CARTESIAN_POINT('Ctrl Pts',(-6.68850813400006,15.2,7.93968525899999));
#242117=CARTESIAN_POINT('Ctrl Pts',(-6.68850813400006,11.6,7.93968525899999));
#242118=CARTESIAN_POINT('Ctrl Pts',(-6.68796045100006,15.2,7.93889761999999));
#242119=CARTESIAN_POINT('Ctrl Pts',(-6.68796045100006,11.6,7.93889761999999));
#242120=CARTESIAN_POINT('Ctrl Pts',(-6.68741739100006,15.2,7.93811829299998));
#242121=CARTESIAN_POINT('Ctrl Pts',(-6.68741739100006,11.6,7.93811829299998));
#242122=CARTESIAN_POINT('Ctrl Pts',(-6.68687898200006,15.2,7.93734728999999));
#242123=CARTESIAN_POINT('Ctrl Pts',(-6.68687898200006,11.6,7.93734728999999));
#242124=CARTESIAN_POINT('Ctrl Pts',(-6.68634525600006,15.2,7.93658462199998));
#242125=CARTESIAN_POINT('Ctrl Pts',(-6.68634525600006,11.6,7.93658462199998));
#242126=CARTESIAN_POINT('Ctrl Pts',(-6.68581928800006,15.2,7.93583464699999));
#242127=CARTESIAN_POINT('Ctrl Pts',(-6.68581928800006,11.6,7.93583464699999));
#242128=CARTESIAN_POINT('Ctrl Pts',(-6.68540286400006,15.2,7.93524212599999));
#242129=CARTESIAN_POINT('Ctrl Pts',(-6.68540286400006,11.6,7.93524212599999));
#242130=CARTESIAN_POINT('Ctrl Pts',(-6.68509340700006,15.2,7.93480250499999));
#242131=CARTESIAN_POINT('Ctrl Pts',(-6.68509340700006,11.6,7.93480250499999));
#242132=CARTESIAN_POINT('Ctrl Pts',(-6.68488903500006,15.2,7.93451247199998));
#242133=CARTESIAN_POINT('Ctrl Pts',(-6.68488903500006,11.6,7.93451247199998));
#242134=CARTESIAN_POINT('Ctrl Pts',(-6.68478856800006,15.2,7.93436996999999));
#242135=CARTESIAN_POINT('Ctrl Pts',(-6.68478856800006,11.6,7.93436996999999));
#242136=CARTESIAN_POINT('',(-6.68478856800006,12.2,7.93436996999999));
#242137=CARTESIAN_POINT('',(-6.68478856800006,15.2,7.93436996999999));
#242138=CARTESIAN_POINT('',(-6.68478856800006,12.2,7.93436996999999));
#242139=CARTESIAN_POINT('Ctrl Pts',(-7.10901226900006,12.2,9.03946594399999));
#242140=CARTESIAN_POINT('Ctrl Pts',(-7.10820510876447,12.2,9.03572920290932));
#242141=CARTESIAN_POINT('Ctrl Pts',(-7.10739512190664,12.2,9.03199984245684));
#242142=CARTESIAN_POINT('Ctrl Pts',(-7.10658231406325,12.2,9.0282778601728));
#242143=CARTESIAN_POINT('Ctrl Pts',(-7.10576950621987,12.2,9.02455587788876));
#242144=CARTESIAN_POINT('Ctrl Pts',(-7.10495387608589,12.2,9.02084127356863));
#242145=CARTESIAN_POINT('Ctrl Pts',(-7.10413543695006,12.2,9.01713406172559));
#242146=CARTESIAN_POINT('Ctrl Pts',(-7.10331699781423,12.2,9.01342684988256));
#242147=CARTESIAN_POINT('Ctrl Pts',(-7.10249574876606,12.2,9.00972702820508));
#242148=CARTESIAN_POINT('Ctrl Pts',(-7.10167172592138,12.2,9.00603462587988));
#242149=CARTESIAN_POINT('Ctrl Pts',(-7.100847702927,12.2,9.0023422228839));
#242150=CARTESIAN_POINT('Ctrl Pts',(-7.10002090567351,12.2,8.99865723969837));
#242151=CARTESIAN_POINT('Ctrl Pts',(-7.09919137359424,12.2,8.99497970670658));
#242152=CARTESIAN_POINT('Ctrl Pts',(-7.09780882032972,12.2,8.98885048594438));
#242153=CARTESIAN_POINT('Ctrl Pts',(-7.09641866681232,12.2,8.9827419607242));
#242154=CARTESIAN_POINT('Ctrl Pts',(-7.0950210550756,12.2,8.97665424392032));
#242155=CARTESIAN_POINT('Ctrl Pts',(-7.09362344349122,12.2,8.97056652778002));
#242156=CARTESIAN_POINT('Ctrl Pts',(-7.09221836699138,12.2,8.96449961652235));
#242157=CARTESIAN_POINT('Ctrl Pts',(-7.09080597665981,12.2,8.95845362974909));
#242158=CARTESIAN_POINT('Ctrl Pts',(-7.08995854224534,12.2,8.95482603676251));
#242159=CARTESIAN_POINT('Ctrl Pts',(-7.0891084765218,12.2,8.95120597821974));
#242160=CARTESIAN_POINT('Ctrl Pts',(-7.08825581056419,12.2,8.94759347819574));
#242161=CARTESIAN_POINT('Ctrl Pts',(-7.08740314476148,12.2,8.94398097882802));
#242162=CARTESIAN_POINT('Ctrl Pts',(-7.08654787997558,12.2,8.94037603907659));
#242163=CARTESIAN_POINT('Ctrl Pts',(-7.08569004713153,12.2,8.93677868462462));
#242164=CARTESIAN_POINT('Ctrl Pts',(-7.08454627005807,12.2,8.93198221223983));
#242165=CARTESIAN_POINT('Ctrl Pts',(-7.08339792922195,12.2,8.92719922369441));
#242166=CARTESIAN_POINT('Ctrl Pts',(-7.08224510142567,12.2,8.92242977923376));
#242167=CARTESIAN_POINT('Ctrl Pts',(-7.08138048053918,12.2,8.9188526957258));
#242168=CARTESIAN_POINT('Ctrl Pts',(-7.08051333552438,12.2,8.9152832313314));
#242169=CARTESIAN_POINT('Ctrl Pts',(-7.07964370018132,12.2,8.91172141245974));
#242170=CARTESIAN_POINT('Ctrl Pts',(-7.07877406468027,12.2,8.90815959294103));
#242171=CARTESIAN_POINT('Ctrl Pts',(-7.07790193908686,12.2,8.90460541902451));
#242172=CARTESIAN_POINT('Ctrl Pts',(-7.07702735608441,12.2,8.90105891551013));
#242173=CARTESIAN_POINT('Ctrl Pts',(-7.07615277324085,12.2,8.89751241264003));
#242174=CARTESIAN_POINT('Ctrl Pts',(-7.07527573325576,12.2,8.89397358151954));
#242175=CARTESIAN_POINT('Ctrl Pts',(-7.0743962699125,12.2,8.8904424471485));
#242176=CARTESIAN_POINT('Ctrl Pts',(-7.07351680656924,12.2,8.88691131277746));
#242177=CARTESIAN_POINT('Ctrl Pts',(-7.0726349195545,12.2,8.88338787511826));
#242178=CARTESIAN_POINT('Ctrl Pts',(-7.07175064274927,12.2,8.87987216023008));
#242179=CARTESIAN_POINT('Ctrl Pts',(-7.07086636594404,12.2,8.8763564453419));
#242180=CARTESIAN_POINT('Ctrl Pts',(-7.06997969982261,12.2,8.8728484526252));
#242181=CARTESIAN_POINT('Ctrl Pts',(-7.06909067747588,12.2,8.86934820973645));
#242182=CARTESIAN_POINT('Ctrl Pts',(-7.06820165512916,12.2,8.8658479668477));
#242183=CARTESIAN_POINT('Ctrl Pts',(-7.06731027678143,12.2,8.86235547373728));
#242184=CARTESIAN_POINT('Ctrl Pts',(-7.06641657789745,12.2,8.85887075536323));
#242185=CARTESIAN_POINT('Ctrl Pts',(-7.06552287901346,12.2,8.85538603698917));
#242186=CARTESIAN_POINT('Ctrl Pts',(-7.06462685867962,12.2,8.85190909388126));
#242187=CARTESIAN_POINT('Ctrl Pts',(-7.06372855096257,12.2,8.8484399520062));
#242188=CARTESIAN_POINT('Ctrl Pts',(-7.06283024308231,12.2,8.84497080950092));
#242189=CARTESIAN_POINT('Ctrl Pts',(-7.06192964918477,12.2,8.84150946848127));
#242190=CARTESIAN_POINT('Ctrl Pts',(-7.06102680276158,12.2,8.83805595498041));
#242191=CARTESIAN_POINT('Ctrl Pts',(-7.06012395650241,12.2,8.83460244210694));
#242192=CARTESIAN_POINT('Ctrl Pts',(-7.05921885898503,12.2,8.83115675699975));
#242193=CARTESIAN_POINT('Ctrl Pts',(-7.05831154418447,12.2,8.82771892562534));
#242194=CARTESIAN_POINT('Ctrl Pts',(-7.05740422938391,12.2,8.82428109425093));
#242195=CARTESIAN_POINT('Ctrl Pts',(-7.05649469778694,12.2,8.82085111663799));
#242196=CARTESIAN_POINT('Ctrl Pts',(-7.05558298448258,12.2,8.81742901970516));
#242197=CARTESIAN_POINT('Ctrl Pts',(-7.05467127117822,12.2,8.81400692277234));
#242198=CARTESIAN_POINT('Ctrl Pts',(-7.05375737607178,12.2,8.81059270517812));
#242199=CARTESIAN_POINT('Ctrl Pts',(-7.05284133526757,12.2,8.80718639520303));
#242200=CARTESIAN_POINT('Ctrl Pts',(-7.05192529446337,12.2,8.80378008522795));
#242201=CARTESIAN_POINT('Ctrl Pts',(-7.05100710835006,12.2,8.80038168184715));
#242202=CARTESIAN_POINT('Ctrl Pts',(-7.05008681113368,12.2,8.79699121138628));
#242203=CARTESIAN_POINT('Ctrl Pts',(-7.04885974806704,12.2,8.7924705836945));
#242204=CARTESIAN_POINT('Ctrl Pts',(-7.04762893401108,12.2,8.78796405849062));
#242205=CARTESIAN_POINT('Ctrl Pts',(-7.04639445416578,12.2,8.78347170085781));
#242206=CARTESIAN_POINT('Ctrl Pts',(-7.0454685943659,12.2,8.78010243293924));
#242207=CARTESIAN_POINT('Ctrl Pts',(-7.044540672753,12.2,8.77674113294025));
#242208=CARTESIAN_POINT('Ctrl Pts',(-7.04361072549089,12.2,8.77338782850523));
#242209=CARTESIAN_POINT('Ctrl Pts',(-7.04237079586439,12.2,8.76891675612827));
#242210=CARTESIAN_POINT('Ctrl Pts',(-7.04112726599888,12.2,8.76445989729794));
#242211=CARTESIAN_POINT('Ctrl Pts',(-7.03988022171229,12.2,8.76001731499296));
#242212=CARTESIAN_POINT('Ctrl Pts',(-7.03894493828496,12.2,8.7566853775076));
#242213=CARTESIAN_POINT('Ctrl Pts',(-7.03800767816541,12.2,8.75336147084121));
#242214=CARTESIAN_POINT('Ctrl Pts',(-7.03706847877865,12.2,8.75004562181874));
#242215=CARTESIAN_POINT('Ctrl Pts',(-7.03612927956251,12.2,8.74672977339866));
#242216=CARTESIAN_POINT('Ctrl Pts',(-7.03518814159647,12.2,8.74342198123646));
#242217=CARTESIAN_POINT('Ctrl Pts',(-7.03424510133891,12.2,8.74012227435707));
#242218=CARTESIAN_POINT('Ctrl Pts',(-7.03330206108135,12.2,8.73682256747767));
#242219=CARTESIAN_POINT('Ctrl Pts',(-7.03235711881911,12.2,8.73353094505917));
#242220=CARTESIAN_POINT('Ctrl Pts',(-7.03141031247421,12.2,8.73024743320529));
#242221=CARTESIAN_POINT('Ctrl Pts',(-7.03046350612931,12.2,8.7269639213514));
#242222=CARTESIAN_POINT('Ctrl Pts',(-7.02951483450403,12.2,8.72368852088237));
#242223=CARTESIAN_POINT('Ctrl Pts',(-7.0285643367426,12.2,8.72042125848624));
#242224=CARTESIAN_POINT('Ctrl Pts',(-7.02761383898117,12.2,8.71715399609011));
#242225=CARTESIAN_POINT('Ctrl Pts',(-7.02666151566921,12.2,8.71389487227034));
#242226=CARTESIAN_POINT('Ctrl Pts',(-7.0257074038707,12.2,8.71064391288775));
#242227=CARTESIAN_POINT('Ctrl Pts',(-7.0247532920722,12.2,8.70739295350516));
#242228=CARTESIAN_POINT('Ctrl Pts',(-7.0237973912738,12.2,8.70415015888866));
#242229=CARTESIAN_POINT('Ctrl Pts',(-7.0228397414755,12.2,8.70091555696341));
#242230=CARTESIAN_POINT('Ctrl Pts',(-7.02188209150322,12.2,8.69768095445053));
#242231=CARTESIAN_POINT('Ctrl Pts',(-7.02092269168046,12.2,8.69445454353162));
#242232=CARTESIAN_POINT('Ctrl Pts',(-7.01996158033221,12.2,8.69123635206505));
#242233=CARTESIAN_POINT('Ctrl Pts',(-7.01900046915858,12.2,8.68801816118312));
#242234=CARTESIAN_POINT('Ctrl Pts',(-7.01803764759345,12.2,8.68480818968989));
#242235=CARTESIAN_POINT('Ctrl Pts',(-7.01707315428845,12.2,8.68160646464722));
#242236=CARTESIAN_POINT('Ctrl Pts',(-7.01578716327352,12.2,8.67733749811756));
#242237=CARTESIAN_POINT('Ctrl Pts',(-7.01449819990541,12.2,8.67308319145381));
#242238=CARTESIAN_POINT('Ctrl Pts',(-7.01320635712231,12.2,8.66884360985499));
#242239=CARTESIAN_POINT('Ctrl Pts',(-7.01191451416321,12.2,8.66460402767853));
#242240=CARTESIAN_POINT('Ctrl Pts',(-7.01061979363152,12.2,8.66037917167046));
#242241=CARTESIAN_POINT('Ctrl Pts',(-7.00932228789397,12.2,8.65616910416423));
#242242=CARTESIAN_POINT('Ctrl Pts',(-7.00802478233321,12.2,8.65195903723164));
#242243=CARTESIAN_POINT('Ctrl Pts',(-7.00672449235858,12.2,8.64776376044167));
#242244=CARTESIAN_POINT('Ctrl Pts',(-7.00542151395579,12.2,8.64358333857328));
#242245=CARTESIAN_POINT('Ctrl Pts',(-7.00411853537546,12.2,8.63940291613529));
#242246=CARTESIAN_POINT('Ctrl Pts',(-7.00281286668399,12.2,8.63523734875263));
#242247=CARTESIAN_POINT('Ctrl Pts',(-7.00150460633476,12.2,8.63108670119408));
#242248=CARTESIAN_POINT('Ctrl Pts',(-7.00019634616377,12.2,8.62693605420107));
#242249=CARTESIAN_POINT('Ctrl Pts',(-6.99888549384329,12.2,8.62280032821055));
#242250=CARTESIAN_POINT('Ctrl Pts',(-6.99757214500646,12.2,8.61867958665701));
#242251=CARTESIAN_POINT('Ctrl Pts',(-6.9962587959907,12.2,8.61455884454202));
#242252=CARTESIAN_POINT('Ctrl Pts',(-6.99494295321589,12.2,8.61045308979414));
#242253=CARTESIAN_POINT('Ctrl Pts',(-6.99362471224917,12.2,8.60636238499715));
#242254=CARTESIAN_POINT('Ctrl Pts',(-6.99230647146207,12.2,8.60227168075752));
#242255=CARTESIAN_POINT('Ctrl Pts',(-6.99098583494687,12.2,8.59819602863621));
#242256=CARTESIAN_POINT('Ctrl Pts',(-6.9896628994997,12.2,8.59413549368883));
#242257=CARTESIAN_POINT('Ctrl Pts',(-6.98833996387227,12.2,8.5900749581882));
#242258=CARTESIAN_POINT('Ctrl Pts',(-6.9870147311252,12.2,8.58602954099459));
#242259=CARTESIAN_POINT('Ctrl Pts',(-6.98568730144173,12.2,8.58199930627492));
#242260=CARTESIAN_POINT('Ctrl Pts',(-6.98402801442784,12.2,8.57696151314989));
#242261=CARTESIAN_POINT('Ctrl Pts',(-6.9823652933734,12.2,8.57194744614203));
#242262=CARTESIAN_POINT('Ctrl Pts',(-6.98069933878249,12.2,8.5669572320222));
#242263=CARTESIAN_POINT('Ctrl Pts',(-6.97936657521871,12.2,8.56296506105269));
#242264=CARTESIAN_POINT('Ctrl Pts',(-6.9780317408897,12.2,8.55898815627535));
#242265=CARTESIAN_POINT('Ctrl Pts',(-6.97669493994363,12.2,8.55502658593098));
#242266=CARTESIAN_POINT('Ctrl Pts',(-6.97535813881543,12.2,8.55106501504685));
#242267=CARTESIAN_POINT('Ctrl Pts',(-6.97401937026479,12.2,8.54711877746137));
#242268=CARTESIAN_POINT('Ctrl Pts',(-6.97267873802507,12.2,8.5431879411916));
#242269=CARTESIAN_POINT('Ctrl Pts',(-6.97133810578533,12.2,8.53925710492183));
#242270=CARTESIAN_POINT('Ctrl Pts',(-6.96999561026206,12.2,8.53534166874273));
#242271=CARTESIAN_POINT('Ctrl Pts',(-6.96865135602194,12.2,8.53144170058729));
#242272=CARTESIAN_POINT('Ctrl Pts',(-6.96730710196498,12.2,8.52754173296322));
#242273=CARTESIAN_POINT('Ctrl Pts',(-6.96596109052192,12.2,8.52365723225668));
#242274=CARTESIAN_POINT('Ctrl Pts',(-6.96461342579265,12.2,8.51978826727756));
#242275=CARTESIAN_POINT('Ctrl Pts',(-6.96326576087975,12.2,8.5159193017713));
#242276=CARTESIAN_POINT('Ctrl Pts',(-6.96191644408631,12.2,8.51206587156335));
#242277=CARTESIAN_POINT('Ctrl Pts',(-6.96056558301253,12.2,8.50822804535579));
#242278=CARTESIAN_POINT('Ctrl Pts',(-6.95921472212282,12.2,8.50439021967113));
#242279=CARTESIAN_POINT('Ctrl Pts',(-6.95786231535552,12.2,8.50056799663723));
#242280=CARTESIAN_POINT('Ctrl Pts',(-6.95650847257739,12.2,8.49676144500292));
#242281=CARTESIAN_POINT('Ctrl Pts',(-6.9551546296148,12.2,8.49295489284995));
#242282=CARTESIAN_POINT('Ctrl Pts',(-6.95379934985484,12.2,8.48916401246561));
#242283=CARTESIAN_POINT('Ctrl Pts',(-6.95244274361415,12.2,8.48538887098312));
#242284=CARTESIAN_POINT('Ctrl Pts',(-6.9510861375583,12.2,8.481613730015));
#242285=CARTESIAN_POINT('Ctrl Pts',(-6.94972820553451,12.2,8.47785432892837));
#242286=CARTESIAN_POINT('Ctrl Pts',(-6.94836905618894,12.2,8.47411073576822));
#242287=CARTESIAN_POINT('Ctrl Pts',(-6.94700990665817,12.2,8.470367142098));
#242288=CARTESIAN_POINT('Ctrl Pts',(-6.94564954147412,12.2,8.46663935695341));
#242289=CARTESIAN_POINT('Ctrl Pts',(-6.94428807262208,12.2,8.46292744819661));
#242290=CARTESIAN_POINT('Ctrl Pts',(-6.94292660395554,12.2,8.45921553994557));
#242291=CARTESIAN_POINT('Ctrl Pts',(-6.9415640318531,12.2,8.45551950956632));
#242292=CARTESIAN_POINT('Ctrl Pts',(-6.94020046846467,12.2,8.45183942580995));
#242293=CARTESIAN_POINT('Ctrl Pts',(-6.93883690489044,12.2,8.44815934155217));
#242294=CARTESIAN_POINT('Ctrl Pts',(-6.93747235057141,12.2,8.444495202485));
#242295=CARTESIAN_POINT('Ctrl Pts',(-6.9361069209908,12.2,8.44084707971411));
#242296=CARTESIAN_POINT('Ctrl Pts',(-6.93474149159622,12.2,8.43719895744027));
#242297=CARTESIAN_POINT('Ctrl Pts',(-6.93337518520063,12.2,8.43356685075275));
#242298=CARTESIAN_POINT('Ctrl Pts',(-6.93200811975691,12.2,8.42995082982447));
#242299=CARTESIAN_POINT('Ctrl Pts',(-6.93064105412692,12.2,8.42633480840351));
#242300=CARTESIAN_POINT('Ctrl Pts',(-6.92927322709964,12.2,8.42273487326746));
#242301=CARTESIAN_POINT('Ctrl Pts',(-6.92790475819173,12.2,8.41915109251658));
#242302=CARTESIAN_POINT('Ctrl Pts',(-6.92653628928381,12.2,8.41556731176571));
#242303=CARTESIAN_POINT('Ctrl Pts',(-6.92516717622027,12.2,8.41199968762786));
#242304=CARTESIAN_POINT('Ctrl Pts',(-6.92379754053446,12.2,8.40844828943595));
#242305=CARTESIAN_POINT('Ctrl Pts',(-6.92242790503526,12.2,8.40489689172791));
#242306=CARTESIAN_POINT('Ctrl Pts',(-6.92105774333963,12.2,8.4013617199196));
#242307=CARTESIAN_POINT('Ctrl Pts',(-6.91968717800099,12.2,8.39784284496899));
#242308=CARTESIAN_POINT('Ctrl Pts',(-6.91831661247562,12.2,8.39432396953894));
#242309=CARTESIAN_POINT('Ctrl Pts',(-6.91694564173117,12.2,8.39082138995437));
#242310=CARTESIAN_POINT('Ctrl Pts',(-6.91557438826753,12.2,8.38733517915494));
#242311=CARTESIAN_POINT('Ctrl Pts',(-6.91420313499071,12.2,8.3838489688305));
#242312=CARTESIAN_POINT('Ctrl Pts',(-6.9128315983806,12.2,8.38037912712338));
#242313=CARTESIAN_POINT('Ctrl Pts',(-6.91145990110386,12.2,8.37692572351573));
#242314=CARTESIAN_POINT('Ctrl Pts',(-6.91008820364023,12.2,8.37347231943755));
#242315=CARTESIAN_POINT('Ctrl Pts',(-6.90871634551375,12.2,8.37003535489566));
#242316=CARTESIAN_POINT('Ctrl Pts',(-6.90734445009265,12.2,8.36661490126201));
#242317=CARTESIAN_POINT('Ctrl Pts',(-6.90597255485848,12.2,8.3631944480944));
#242318=CARTESIAN_POINT('Ctrl Pts',(-6.90460062321396,12.2,8.35979050523729));
#242319=CARTESIAN_POINT('Ctrl Pts',(-6.90322878060387,12.2,8.35640314623532));
#242320=CARTESIAN_POINT('Ctrl Pts',(-6.90151397720106,12.2,8.35216894713671));
#242321=CARTESIAN_POINT('Ctrl Pts',(-6.89979931333997,12.2,8.34796065897496));
#242322=CARTESIAN_POINT('Ctrl Pts',(-6.89808503514551,12.2,8.34377842251527));
#242323=CARTESIAN_POINT('Ctrl Pts',(-6.89671361251519,12.2,8.34043263316517));
#242324=CARTESIAN_POINT('Ctrl Pts',(-6.89534243782485,12.2,8.33710351748334));
#242325=CARTESIAN_POINT('Ctrl Pts',(-6.89397164029282,12.2,8.33379114852771));
#242326=CARTESIAN_POINT('Ctrl Pts',(-6.89260084294755,12.2,8.33047878002339));
#242327=CARTESIAN_POINT('Ctrl Pts',(-6.89123042266955,12.2,8.32718315837063));
#242328=CARTESIAN_POINT('Ctrl Pts',(-6.88986050883705,12.2,8.32390435602645));
#242329=CARTESIAN_POINT('Ctrl Pts',(-6.88849059481791,12.2,8.32062555323553));
#242330=CARTESIAN_POINT('Ctrl Pts',(-6.88712118751272,12.2,8.31736357026887));
#242331=CARTESIAN_POINT('Ctrl Pts',(-6.88575242010483,12.2,8.31411848025979));
#242332=CARTESIAN_POINT('Ctrl Pts',(-6.88438365288343,12.2,8.31087339069285));
#242333=CARTESIAN_POINT('Ctrl Pts',(-6.8830155249773,12.2,8.30764519532095));
#242334=CARTESIAN_POINT('Ctrl Pts',(-6.88164816913181,12.2,8.30443396619933));
#242335=CARTESIAN_POINT('Ctrl Pts',(-6.8802808131,12.2,8.30122273664016));
#242336=CARTESIAN_POINT('Ctrl Pts',(-6.87891423041834,12.2,8.29802847458182));
#242337=CARTESIAN_POINT('Ctrl Pts',(-6.87754855512175,12.2,8.29485125446535));
#242338=CARTESIAN_POINT('Ctrl Pts',(-6.87618288001124,12.2,8.29167403478178));
#242339=CARTESIAN_POINT('Ctrl Pts',(-6.87481811360331,12.2,8.2885138560975));
#242340=CARTESIAN_POINT('Ctrl Pts',(-6.87345439121469,12.2,8.28537079446382));
#242341=CARTESIAN_POINT('Ctrl Pts',(-6.87209066864026,12.2,8.28222773240188));
#242342=CARTESIAN_POINT('Ctrl Pts',(-6.87072799079894,12.2,8.27910178697295));
#242343=CARTESIAN_POINT('Ctrl Pts',(-6.86936649677413,12.2,8.27599303295615));
#242344=CARTESIAN_POINT('Ctrl Pts',(-6.86800500293482,12.2,8.27288427936291));
#242345=CARTESIAN_POINT('Ctrl Pts',(-6.86664469211685,12.2,8.26979271739471));
#242346=CARTESIAN_POINT('Ctrl Pts',(-6.86528570500558,12.2,8.26671842247757));
#242347=CARTESIAN_POINT('Ctrl Pts',(-6.86392671770914,12.2,8.26364412714155));
#242348=CARTESIAN_POINT('Ctrl Pts',(-6.86256905411841,12.2,8.26058709849891));
#242349=CARTESIAN_POINT('Ctrl Pts',(-6.86121285626672,12.2,8.25754741499992));
#242350=CARTESIAN_POINT('Ctrl Pts',(-6.85951760904449,12.2,8.25374781083325));
#242351=CARTESIAN_POINT('Ctrl Pts',(-6.85782465187901,12.2,8.24997530349814));
#242352=CARTESIAN_POINT('Ctrl Pts',(-6.85613426548246,12.2,8.24623004598121));
#242353=CARTESIAN_POINT('Ctrl Pts',(-6.85444387908591,12.2,8.2424847884643));
#242354=CARTESIAN_POINT('Ctrl Pts',(-6.8527560653175,12.2,8.23876677837395));
#242355=CARTESIAN_POINT('Ctrl Pts',(-6.85107110816487,12.2,8.23507616775038));
#242356=CARTESIAN_POINT('Ctrl Pts',(-6.84938615101224,12.2,8.23138555712683));
#242357=CARTESIAN_POINT('Ctrl Pts',(-6.84770405040121,12.2,8.22772234645532));
#242358=CARTESIAN_POINT('Ctrl Pts',(-6.8460250988736,12.2,8.22408668576231));
#242359=CARTESIAN_POINT('Ctrl Pts',(-6.84434614734597,12.2,8.22045102506929));
#242360=CARTESIAN_POINT('Ctrl Pts',(-6.84267034271829,12.2,8.21684291401446));
#242361=CARTESIAN_POINT('Ctrl Pts',(-6.84099798139903,12.2,8.21326250901593));
#242362=CARTESIAN_POINT('Ctrl Pts',(-6.83899114788885,12.2,8.20896602317379));
#242363=CARTESIAN_POINT('Ctrl Pts',(-6.83698927177916,12.2,8.2047094274012));
#242364=CARTESIAN_POINT('Ctrl Pts',(-6.83499287325929,12.2,8.20049299370184));
#242365=CARTESIAN_POINT('Ctrl Pts',(-6.83332920776563,12.2,8.19697929882472));
#242366=CARTESIAN_POINT('Ctrl Pts',(-6.8316693463556,12.2,8.19349349127769));
#242367=CARTESIAN_POINT('Ctrl Pts',(-6.83001359350838,12.2,8.1900357297499));
#242368=CARTESIAN_POINT('Ctrl Pts',(-6.82835784066115,12.2,8.18657796822211));
#242369=CARTESIAN_POINT('Ctrl Pts',(-6.82670619727883,12.2,8.18314825062453));
#242370=CARTESIAN_POINT('Ctrl Pts',(-6.82505897525748,12.2,8.1797467334564));
#242371=CARTESIAN_POINT('Ctrl Pts',(-6.82341175323613,12.2,8.17634521628825));
#242372=CARTESIAN_POINT('Ctrl Pts',(-6.82176895281494,12.2,8.17297190092988));
#242373=CARTESIAN_POINT('Ctrl Pts',(-6.82013088913461,12.2,8.16962694530632));
#242374=CARTESIAN_POINT('Ctrl Pts',(-6.81849282545428,12.2,8.16628198968278));
#242375=CARTESIAN_POINT('Ctrl Pts',(-6.81685949770997,12.2,8.16296539310019));
#242376=CARTESIAN_POINT('Ctrl Pts',(-6.81523123062692,12.2,8.15967731581005));
#242377=CARTESIAN_POINT('Ctrl Pts',(-6.81360296354386,12.2,8.1563892385199));
#242378=CARTESIAN_POINT('Ctrl Pts',(-6.81197975514824,12.2,8.15312967960656));
#242379=CARTESIAN_POINT('Ctrl Pts',(-6.81036193305392,12.2,8.14989880139163));
#242380=CARTESIAN_POINT('Ctrl Pts',(-6.80874411095961,12.2,8.14666792317669));
#242381=CARTESIAN_POINT('Ctrl Pts',(-6.80713167445608,12.2,8.14346572471582));
#242382=CARTESIAN_POINT('Ctrl Pts',(-6.80552495903989,12.2,8.14029236909318));
#242383=CARTESIAN_POINT('Ctrl Pts',(-6.80391824362369,12.2,8.13711901347056));
#242384=CARTESIAN_POINT('Ctrl Pts',(-6.80231724744094,12.2,8.13397449881783));
#242385=CARTESIAN_POINT('Ctrl Pts',(-6.80072230973309,12.2,8.13085899229242));
#242386=CARTESIAN_POINT('Ctrl Pts',(-6.79912737219911,12.2,8.12774348610661));
#242387=CARTESIAN_POINT('Ctrl Pts',(-6.79753849293507,12.2,8.1246569853523));
#242388=CARTESIAN_POINT('Ctrl Pts',(-6.79595601789869,12.2,8.12159965609981));
#242389=CARTESIAN_POINT('Ctrl Pts',(-6.79437354268982,12.2,8.11854232651406));
#242390=CARTESIAN_POINT('Ctrl Pts',(-6.79279746987807,12.2,8.11551417021121));
#242391=CARTESIAN_POINT('Ctrl Pts',(-6.79122815369698,12.2,8.11251535208383));
#242392=CARTESIAN_POINT('Ctrl Pts',(-6.78965883751588,12.2,8.10951653395645));
#242393=CARTESIAN_POINT('Ctrl Pts',(-6.78809627455882,12.2,8.10654705507356));
#242394=CARTESIAN_POINT('Ctrl Pts',(-6.78654082593896,12.2,8.10360708284131));
#242395=CARTESIAN_POINT('Ctrl Pts',(-6.7846742874934,12.2,8.10007911597033));
#242396=CARTESIAN_POINT('Ctrl Pts',(-6.7828179900404,12.2,8.09659364105941));
#242397=CARTESIAN_POINT('Ctrl Pts',(-6.78097256402388,12.2,8.09315095137466));
#242398=CARTESIAN_POINT('Ctrl Pts',(-6.779127138175,12.2,8.08970826200263));
#242399=CARTESIAN_POINT('Ctrl Pts',(-6.77729258656622,12.2,8.08630835871654));
#242400=CARTESIAN_POINT('Ctrl Pts',(-6.77546955154088,12.2,8.08295153924006));
#242401=CARTESIAN_POINT('Ctrl Pts',(-6.77364651651555,12.2,8.07959471976359));
#242402=CARTESIAN_POINT('Ctrl Pts',(-6.77183499715831,12.2,8.0762809853114));
#242403=CARTESIAN_POINT('Ctrl Pts',(-6.77003565613982,12.2,8.07301063592833));
#242404=CARTESIAN_POINT('Ctrl Pts',(-6.7682363149579,12.2,8.0697402862482));
#242405=CARTESIAN_POINT('Ctrl Pts',(-6.76644914785245,12.2,8.06651332560679));
#242406=CARTESIAN_POINT('Ctrl Pts',(-6.76467483475664,12.2,8.06333005593628));
#242407=CARTESIAN_POINT('Ctrl Pts',(-6.76290052182198,12.2,8.06014678655492));
#242408=CARTESIAN_POINT('Ctrl Pts',(-6.76113905801572,12.2,8.05700721071698));
#242409=CARTESIAN_POINT('Ctrl Pts',(-6.75939113816316,12.2,8.05391163833139));
#242410=CARTESIAN_POINT('Ctrl Pts',(-6.7576432183106,12.2,8.05081606594578));
#242411=CARTESIAN_POINT('Ctrl Pts',(-6.75590883844864,12.2,8.04776449707332));
#242412=CARTESIAN_POINT('Ctrl Pts',(-6.75418870884384,12.2,8.04475724668065));
#242413=CARTESIAN_POINT('Ctrl Pts',(-6.75218189086742,12.2,8.0412487877071));
#242414=CARTESIAN_POINT('Ctrl Pts',(-6.75019446584363,12.2,8.03780064964788));
#242415=CARTESIAN_POINT('Ctrl Pts',(-6.74822758646655,12.2,8.03441334308353));
#242416=CARTESIAN_POINT('Ctrl Pts',(-6.74654168994513,12.2,8.03150993760765));
#242417=CARTESIAN_POINT('Ctrl Pts',(-6.74487088876418,12.2,8.02865122335319));
#242418=CARTESIAN_POINT('Ctrl Pts',(-6.74321592732362,12.2,8.02583752512011));
#242419=CARTESIAN_POINT('Ctrl Pts',(-6.74156096573273,12.2,8.02302382663146));
#242420=CARTESIAN_POINT('Ctrl Pts',(-6.73992184356047,12.2,8.02025514675672));
#242421=CARTESIAN_POINT('Ctrl Pts',(-6.73829932680651,12.2,8.01753181219474));
#242422=CARTESIAN_POINT('Ctrl Pts',(-6.73667681019993,12.2,8.01480847788012));
#242423=CARTESIAN_POINT('Ctrl Pts',(-6.73507089530507,12.2,8.0121304915007));
#242424=CARTESIAN_POINT('Ctrl Pts',(-6.73348236619686,12.2,8.00949818534832));
#242425=CARTESIAN_POINT('Ctrl Pts',(-6.73189383708866,12.2,8.00686587919593));
#242426=CARTESIAN_POINT('Ctrl Pts',(-6.73032269597908,12.2,8.00427925697325));
#242427=CARTESIAN_POINT('Ctrl Pts',(-6.72876974286807,12.2,8.00173865664689));
#242428=CARTESIAN_POINT('Ctrl Pts',(-6.72721678975705,12.2,7.99919805632055));
#242429=CARTESIAN_POINT('Ctrl Pts',(-6.72568202645312,12.2,7.99670347846429));
#242430=CARTESIAN_POINT('Ctrl Pts',(-6.72416627542358,12.2,7.99425527105011));
#242431=CARTESIAN_POINT('Ctrl Pts',(-6.72265052425637,12.2,7.99180706341354));
#242432=CARTESIAN_POINT('Ctrl Pts',(-6.72115378614092,12.2,7.98940522486475));
#242433=CARTESIAN_POINT('Ctrl Pts',(-6.71967690797795,12.2,7.98705010840508));
#242434=CARTESIAN_POINT('Ctrl Pts',(-6.71820002994913,12.2,7.98469499215934));
#242435=CARTESIAN_POINT('Ctrl Pts',(-6.71674300878007,12.2,7.98238659732083));
#242436=CARTESIAN_POINT('Ctrl Pts',(-6.71530671774234,12.2,7.98012528497593));
#242437=CARTESIAN_POINT('Ctrl Pts',(-6.71387042670461,12.2,7.97786397263103));
#242438=CARTESIAN_POINT('Ctrl Pts',(-6.71245486184446,12.2,7.97564974104394));
#242439=CARTESIAN_POINT('Ctrl Pts',(-6.71106091814363,12.2,7.9734829567861));
#242440=CARTESIAN_POINT('Ctrl Pts',(-6.70966697431618,12.2,7.97131617233144));
#242441=CARTESIAN_POINT('Ctrl Pts',(-6.70829465092583,12.2,7.96919683522989));
#242442=CARTESIAN_POINT('Ctrl Pts',(-6.7069448661195,12.2,7.96712531684963));
#242443=CARTESIAN_POINT('Ctrl Pts',(-6.70537011736268,12.2,7.96470854568825));
#242444=CARTESIAN_POINT('Ctrl Pts',(-6.70382604637675,12.2,7.96235686321937));
#242445=CARTESIAN_POINT('Ctrl Pts',(-6.70231415214961,12.2,7.96007087199682));
#242446=CARTESIAN_POINT('Ctrl Pts',(-6.70101824266072,12.2,7.95811145072011));
#242447=CARTESIAN_POINT('Ctrl Pts',(-6.69974597505825,12.2,7.95620029419487));
#242448=CARTESIAN_POINT('Ctrl Pts',(-6.69849832742938,12.2,7.95433778983651));
#242449=CARTESIAN_POINT('Ctrl Pts',(-6.69725067991383,12.2,7.95247528564732));
#242450=CARTESIAN_POINT('Ctrl Pts',(-6.69602764898984,12.2,7.95066143463579));
#242451=CARTESIAN_POINT('Ctrl Pts',(-6.69483024353334,12.2,7.94889663453322));
#242452=CARTESIAN_POINT('Ctrl Pts',(-6.69363283807683,12.2,7.94713183443065));
#242453=CARTESIAN_POINT('Ctrl Pts',(-6.69246105484464,12.2,7.94541608402843));
#242454=CARTESIAN_POINT('Ctrl Pts',(-6.69131593166085,12.2,7.94374979091955));
#242455=CARTESIAN_POINT('Ctrl Pts',(-6.69017080837305,12.2,7.94208349765932));
#242456=CARTESIAN_POINT('Ctrl Pts',(-6.68905234456365,12.2,7.94046666191108));
#242457=CARTESIAN_POINT('Ctrl Pts',(-6.68796160658946,12.2,7.93889969782912));
#242458=CARTESIAN_POINT('Ctrl Pts',(-6.68687610346005,12.2,7.93734025417272));
#242459=CARTESIAN_POINT('Ctrl Pts',(-6.68581806471473,12.2,7.93583020411499));
#242460=CARTESIAN_POINT('Ctrl Pts',(-6.68478856800006,12.2,7.93436996999999));
#242461=CARTESIAN_POINT('Ctrl Pts',(-6.68478856800006,15.2,7.93436996999999));
#242462=CARTESIAN_POINT('Ctrl Pts',(-6.68581806471473,15.2,7.93583020411499));
#242463=CARTESIAN_POINT('Ctrl Pts',(-6.68687610346001,15.2,7.93734025417266));
#242464=CARTESIAN_POINT('Ctrl Pts',(-6.68796160658946,15.2,7.93889969782911));
#242465=CARTESIAN_POINT('Ctrl Pts',(-6.68905234456369,15.2,7.94046666191113));
#242466=CARTESIAN_POINT('Ctrl Pts',(-6.69017080837302,15.2,7.94208349765928));
#242467=CARTESIAN_POINT('Ctrl Pts',(-6.69131593166085,15.2,7.94374979091955));
#242468=CARTESIAN_POINT('Ctrl Pts',(-6.69246105484467,15.2,7.94541608402847));
#242469=CARTESIAN_POINT('Ctrl Pts',(-6.69363283807684,15.2,7.94713183443067));
#242470=CARTESIAN_POINT('Ctrl Pts',(-6.69483024353334,15.2,7.94889663453323));
#242471=CARTESIAN_POINT('Ctrl Pts',(-6.69602764898984,15.2,7.95066143463578));
#242472=CARTESIAN_POINT('Ctrl Pts',(-6.69725067991382,15.2,7.9524752856473));
#242473=CARTESIAN_POINT('Ctrl Pts',(-6.69849832742937,15.2,7.9543377898365));
#242474=CARTESIAN_POINT('Ctrl Pts',(-6.69974597505826,15.2,7.95620029419488));
#242475=CARTESIAN_POINT('Ctrl Pts',(-6.70101824266071,15.2,7.95811145072009));
#242476=CARTESIAN_POINT('Ctrl Pts',(-6.70231415214961,15.2,7.96007087199682));
#242477=CARTESIAN_POINT('Ctrl Pts',(-6.7036100615208,15.2,7.96203029309558));
#242478=CARTESIAN_POINT('Ctrl Pts',(-6.70492961203493,15.2,7.9640379764411));
#242479=CARTESIAN_POINT('Ctrl Pts',(-6.7062718567423,15.2,7.96609354445918));
#242480=CARTESIAN_POINT('Ctrl Pts',(-6.70761410144967,15.2,7.96814911247727));
#242481=CARTESIAN_POINT('Ctrl Pts',(-6.70897904139254,15.2,7.97025256060477));
#242482=CARTESIAN_POINT('Ctrl Pts',(-6.71036575217453,15.2,7.97240351960788));
#242483=CARTESIAN_POINT('Ctrl Pts',(-6.71175246308249,15.2,7.97455447880635));
#242484=CARTESIAN_POINT('Ctrl Pts',(-6.71316094577651,15.2,7.97675294581909));
#242485=CARTESIAN_POINT('Ctrl Pts',(-6.71459030368916,15.2,7.97899855427803));
#242486=CARTESIAN_POINT('Ctrl Pts',(-6.71601966147198,15.2,7.98124416253299));
#242487=CARTESIAN_POINT('Ctrl Pts',(-6.71746989292446,15.2,7.98353691334393));
#242488=CARTESIAN_POINT('Ctrl Pts',(-6.71894012778856,15.2,7.98587644559427));
#242489=CARTESIAN_POINT('Ctrl Pts',(-6.72041036265266,15.2,7.9882159778446));
#242490=CARTESIAN_POINT('Ctrl Pts',(-6.72190059904019,15.2,7.99060229029125));
#242491=CARTESIAN_POINT('Ctrl Pts',(-6.72340998815117,15.2,7.99303503236752));
#242492=CARTESIAN_POINT('Ctrl Pts',(-6.72491937726217,15.2,7.99546777444376));
#242493=CARTESIAN_POINT('Ctrl Pts',(-6.72644791950553,15.2,7.99794694257784));
#242494=CARTESIAN_POINT('Ctrl Pts',(-6.72799478578142,15.2,8.000472192733));
#242495=CARTESIAN_POINT('Ctrl Pts',(-6.72954165219784,15.2,8.00299744311753));
#242496=CARTESIAN_POINT('Ctrl Pts',(-6.73110684411601,15.2,8.00556877248147));
#242497=CARTESIAN_POINT('Ctrl Pts',(-6.73268955453636,15.2,8.00818584112606));
#242498=CARTESIAN_POINT('Ctrl Pts',(-6.73427226481293,15.2,8.01080290953295));
#242499=CARTESIAN_POINT('Ctrl Pts',(-6.73587249451741,15.2,8.01346571642655));
#242500=CARTESIAN_POINT('Ctrl Pts',(-6.73748945579929,15.2,8.01617392575701));
#242501=CARTESIAN_POINT('Ctrl Pts',(-6.73910641708119,15.2,8.01888213508748));
#242502=CARTESIAN_POINT('Ctrl Pts',(-6.74074011055623,15.2,8.02163574622458));
#242503=CARTESIAN_POINT('Ctrl Pts',(-6.74238977007855,15.2,8.0244344287032));
#242504=CARTESIAN_POINT('Ctrl Pts',(-6.74403942975074,15.2,8.02723311143604));
#242505=CARTESIAN_POINT('Ctrl Pts',(-6.74570505504111,15.2,8.03007686676484));
#242506=CARTESIAN_POINT('Ctrl Pts',(-6.74738589955004,15.2,8.03296536642419));
#242507=CARTESIAN_POINT('Ctrl Pts',(-6.74906674390628,15.2,8.03585386582117));
#242508=CARTESIAN_POINT('Ctrl Pts',(-6.75076280499531,15.2,8.03878711137662));
#242509=CARTESIAN_POINT('Ctrl Pts',(-6.75247335552426,15.2,8.04176478078189));
#242510=CARTESIAN_POINT('Ctrl Pts',(-6.7541839060532,15.2,8.04474245018717));
#242511=CARTESIAN_POINT('Ctrl Pts',(-6.75590894320798,15.2,8.04776454395514));
#242512=CARTESIAN_POINT('Ctrl Pts',(-6.7576477578105,15.2,8.05083074542404));
#242513=CARTESIAN_POINT('Ctrl Pts',(-6.75938657257097,15.2,8.05389694717145));
#242514=CARTESIAN_POINT('Ctrl Pts',(-6.76113916048569,15.2,8.05700725707316));
#242515=CARTESIAN_POINT('Ctrl Pts',(-6.76290483117087,15.2,8.0601613630718));
#242516=CARTESIAN_POINT('Ctrl Pts',(-6.76467050169567,15.2,8.06331546878394));
#242517=CARTESIAN_POINT('Ctrl Pts',(-6.76644924912344,15.2,8.06651337068433));
#242518=CARTESIAN_POINT('Ctrl Pts',(-6.76824039797503,15.2,8.06975476023324));
#242519=CARTESIAN_POINT('Ctrl Pts',(-6.77003154682663,15.2,8.07299614978215));
#242520=CARTESIAN_POINT('Ctrl Pts',(-6.77183509503376,15.2,8.07628102945192));
#242521=CARTESIAN_POINT('Ctrl Pts',(-6.77365037905779,15.2,8.0796090921614));
#242522=CARTESIAN_POINT('Ctrl Pts',(-6.77546566324672,15.2,8.08293715517317));
#242523=CARTESIAN_POINT('Ctrl Pts',(-6.77729268209943,15.2,8.08630840419134));
#242524=CARTESIAN_POINT('Ctrl Pts',(-6.77913078720039,15.2,8.08972253613039));
#242525=CARTESIAN_POINT('Ctrl Pts',(-6.78096889213439,15.2,8.09313666775932));
#242526=CARTESIAN_POINT('Ctrl Pts',(-6.78281808346832,15.2,8.09659368458767));
#242527=CARTESIAN_POINT('Ctrl Pts',(-6.78467772449255,15.2,8.10009329105984));
#242528=CARTESIAN_POINT('Ctrl Pts',(-6.78653736551678,15.2,8.10359289753202));
#242529=CARTESIAN_POINT('Ctrl Pts',(-6.78840745708302,15.2,8.10713509117849));
#242530=CARTESIAN_POINT('Ctrl Pts',(-6.79028737718096,15.2,8.11071958262974));
#242531=CARTESIAN_POINT('Ctrl Pts',(-6.79185397731949,15.2,8.11370665894764));
#242532=CARTESIAN_POINT('Ctrl Pts',(-6.79342740458042,15.2,8.11672310687465));
#242533=CARTESIAN_POINT('Ctrl Pts',(-6.79500730395509,15.2,8.11976876006757));
#242534=CARTESIAN_POINT('Ctrl Pts',(-6.79658720332974,15.2,8.12281441326048));
#242535=CARTESIAN_POINT('Ctrl Pts',(-6.79817357701418,15.2,8.12588927274531));
#242536=CARTESIAN_POINT('Ctrl Pts',(-6.79976607729917,15.2,8.12899317081489));
#242537=CARTESIAN_POINT('Ctrl Pts',(-6.80167707757174,15.2,8.13271784836305));
#242538=CARTESIAN_POINT('Ctrl Pts',(-6.80359690061049,15.2,8.13648434248437));
#242539=CARTESIAN_POINT('Ctrl Pts',(-6.80552495903989,15.2,8.14029236909319));
#242540=CARTESIAN_POINT('Ctrl Pts',(-6.8071316744561,15.2,8.14346572471585));
#242541=CARTESIAN_POINT('Ctrl Pts',(-6.8087441109596,15.2,8.14666792317666));
#242542=CARTESIAN_POINT('Ctrl Pts',(-6.81036193305392,15.2,8.14989880139162));
#242543=CARTESIAN_POINT('Ctrl Pts',(-6.81197975514825,15.2,8.15312967960658));
#242544=CARTESIAN_POINT('Ctrl Pts',(-6.81360296354384,15.2,8.15638923851985));
#242545=CARTESIAN_POINT('Ctrl Pts',(-6.81523123062692,15.2,8.15967731581005));
#242546=CARTESIAN_POINT('Ctrl Pts',(-6.81718515123309,15.2,8.16362300877331));
#242547=CARTESIAN_POINT('Ctrl Pts',(-6.81914635879852,15.2,8.16760976851666));
#242548=CARTESIAN_POINT('Ctrl Pts',(-6.82111429348955,15.2,8.17163732140559));
#242549=CARTESIAN_POINT('Ctrl Pts',(-6.82275423879728,15.2,8.17499361493095));
#242550=CARTESIAN_POINT('Ctrl Pts',(-6.82439885848668,15.2,8.17837823533896));
#242551=CARTESIAN_POINT('Ctrl Pts',(-6.82604783629269,15.2,8.18179102635353));
#242552=CARTESIAN_POINT('Ctrl Pts',(-6.82769681427845,15.2,8.18520381774011));
#242553=CARTESIAN_POINT('Ctrl Pts',(-6.82935015166137,15.2,8.18864477664291));
#242554=CARTESIAN_POINT('Ctrl Pts',(-6.83100753554992,15.2,8.1921137505295));
#242555=CARTESIAN_POINT('Ctrl Pts',(-6.83299639632458,15.2,8.19627651942028));
#242556=CARTESIAN_POINT('Ctrl Pts',(-6.83499108617596,15.2,8.2004796268649));
#242557=CARTESIAN_POINT('Ctrl Pts',(-6.83699107896854,15.2,8.20472280514382));
#242558=CARTESIAN_POINT('Ctrl Pts',(-6.83899107157944,15.2,8.20896598303733));
#242559=CARTESIAN_POINT('Ctrl Pts',(-6.8409963668314,15.2,8.21324923069861));
#242560=CARTESIAN_POINT('Ctrl Pts',(-6.84300644850838,15.2,8.21757228429157));
#242561=CARTESIAN_POINT('Ctrl Pts',(-6.84501653018537,15.2,8.22189533788455));
#242562=CARTESIAN_POINT('Ctrl Pts',(-6.84703140014528,15.2,8.22625819658269));
#242563=CARTESIAN_POINT('Ctrl Pts',(-6.84905054982163,15.2,8.23066059625339));
#242564=CARTESIAN_POINT('Ctrl Pts',(-6.85073317461305,15.2,8.23432926277894));
#242565=CARTESIAN_POINT('Ctrl Pts',(-6.85241877168104,15.2,8.23802538877811));
#242566=CARTESIAN_POINT('Ctrl Pts',(-6.85410705482074,15.2,8.24174882451777));
#242567=CARTESIAN_POINT('Ctrl Pts',(-6.85579533796045,15.2,8.24547226025744));
#242568=CARTESIAN_POINT('Ctrl Pts',(-6.85748630704498,15.2,8.24922300395439));
#242569=CARTESIAN_POINT('Ctrl Pts',(-6.85917967690599,15.2,8.25300090624468));
#242570=CARTESIAN_POINT('Ctrl Pts',(-6.860873046767,15.2,8.25677880853496));
#242571=CARTESIAN_POINT('Ctrl Pts',(-6.86256881806138,15.2,8.26058386849535));
#242572=CARTESIAN_POINT('Ctrl Pts',(-6.86426671438068,15.2,8.26441593925778));
#242573=CARTESIAN_POINT('Ctrl Pts',(-6.86562503151016,15.2,8.26748159603481));
#242574=CARTESIAN_POINT('Ctrl Pts',(-6.8669847064636,15.2,8.27056453918565));
#242575=CARTESIAN_POINT('Ctrl Pts',(-6.8683456004392,15.2,8.2736646927332));
#242576=CARTESIAN_POINT('Ctrl Pts',(-6.86970649422937,15.2,8.27676484585836));
#242577=CARTESIAN_POINT('Ctrl Pts',(-6.87106860596401,15.2,8.27988220889283));
#242578=CARTESIAN_POINT('Ctrl Pts',(-6.87243179713029,15.2,8.28301670780217));
#242579=CARTESIAN_POINT('Ctrl Pts',(-6.8737949884823,15.2,8.28615120713857));
#242580=CARTESIAN_POINT('Ctrl Pts',(-6.87515925874831,15.2,8.28930284102418));
#242581=CARTESIAN_POINT('Ctrl Pts',(-6.87652447137834,15.2,8.29247153630913));
#242582=CARTESIAN_POINT('Ctrl Pts',(-6.87788968382236,15.2,8.29564023116235));
#242583=CARTESIAN_POINT('Ctrl Pts',(-6.87925583847857,15.2,8.2988259847469));
#242584=CARTESIAN_POINT('Ctrl Pts',(-6.8806227991017,15.2,8.30202872581028));
#242585=CARTESIAN_POINT('Ctrl Pts',(-6.88233150002033,15.2,8.30603215246679));
#242586=CARTESIAN_POINT('Ctrl Pts',(-6.88404146093822,15.2,8.31006211796952));
#242587=CARTESIAN_POINT('Ctrl Pts',(-6.88575242010483,15.2,8.31411848025978));
#242588=CARTESIAN_POINT('Ctrl Pts',(-6.88712118751271,15.2,8.31736357026885));
#242589=CARTESIAN_POINT('Ctrl Pts',(-6.88849059481791,15.2,8.32062555323554));
#242590=CARTESIAN_POINT('Ctrl Pts',(-6.88986050883705,15.2,8.32390435602645));
#242591=CARTESIAN_POINT('Ctrl Pts',(-6.89123042266954,15.2,8.32718315837062));
#242592=CARTESIAN_POINT('Ctrl Pts',(-6.89260084294753,15.2,8.33047878002334));
#242593=CARTESIAN_POINT('Ctrl Pts',(-6.89397164029281,15.2,8.33379114852769));
#242594=CARTESIAN_POINT('Ctrl Pts',(-6.89534243782485,15.2,8.33710351748335));
#242595=CARTESIAN_POINT('Ctrl Pts',(-6.8967136125152,15.2,8.34043263316519));
#242596=CARTESIAN_POINT('Ctrl Pts',(-6.89808503514551,15.2,8.34377842251527));
#242597=CARTESIAN_POINT('Ctrl Pts',(-6.89945645758896,15.2,8.34712421140948));
#242598=CARTESIAN_POINT('Ctrl Pts',(-6.9008281270907,15.2,8.35048667348928));
#242599=CARTESIAN_POINT('Ctrl Pts',(-6.9021999170341,15.2,8.35386573648912));
#242600=CARTESIAN_POINT('Ctrl Pts',(-6.9035717071644,15.2,8.35724479994934));
#242601=CARTESIAN_POINT('Ctrl Pts',(-6.90494361847277,15.2,8.36064046447572));
#242602=CARTESIAN_POINT('Ctrl Pts',(-6.90631552394266,15.2,8.36405265851058));
#242603=CARTESIAN_POINT('Ctrl Pts',(-6.90768742922563,15.2,8.36746485208053));
#242604=CARTESIAN_POINT('Ctrl Pts',(-6.90905932959068,15.2,8.37089357359774));
#242605=CARTESIAN_POINT('Ctrl Pts',(-6.91043109953411,15.2,8.37433875320331));
#242606=CARTESIAN_POINT('Ctrl Pts',(-6.91180286966444,15.2,8.37778393327828));
#242607=CARTESIAN_POINT('Ctrl Pts',(-6.91317450979477,15.2,8.38124556989093));
#242608=CARTESIAN_POINT('Ctrl Pts',(-6.91454589725839,15.2,8.38472359202492));
#242609=CARTESIAN_POINT('Ctrl Pts',(-6.91591728472202,15.2,8.3882016141589));
#242610=CARTESIAN_POINT('Ctrl Pts',(-6.91728841924951,15.2,8.39169602304481));
#242611=CARTESIAN_POINT('Ctrl Pts',(-6.91865917999085,15.2,8.39520674584895));
#242612=CARTESIAN_POINT('Ctrl Pts',(-6.92037263063738,15.2,8.39959514863663));
#242613=CARTESIAN_POINT('Ctrl Pts',(-6.92208549620712,15.2,8.40400904242189));
#242614=CARTESIAN_POINT('Ctrl Pts',(-6.92379754053445,15.2,8.40844828943594));
#242615=CARTESIAN_POINT('Ctrl Pts',(-6.92516717622026,15.2,8.41199968762783));
#242616=CARTESIAN_POINT('Ctrl Pts',(-6.92653628928382,15.2,8.41556731176574));
#242617=CARTESIAN_POINT('Ctrl Pts',(-6.92790475819172,15.2,8.41915109251658));
#242618=CARTESIAN_POINT('Ctrl Pts',(-6.92995746136712,15.2,8.42452676315456));
#242619=CARTESIAN_POINT('Ctrl Pts',(-6.93200871780712,15.2,8.42993878222585));
#242620=CARTESIAN_POINT('Ctrl Pts',(-6.93405813383513,15.2,8.43538691621463));
#242621=CARTESIAN_POINT('Ctrl Pts',(-6.93610755004931,15.2,8.44083505069828));
#242622=CARTESIAN_POINT('Ctrl Pts',(-6.93815512310335,15.2,8.44631929942333));
#242623=CARTESIAN_POINT('Ctrl Pts',(-6.94020046846467,15.2,8.45183942580996));
#242624=CARTESIAN_POINT('Ctrl Pts',(-6.94156403185309,15.2,8.45551950956629));
#242625=CARTESIAN_POINT('Ctrl Pts',(-6.94292660395554,15.2,8.45921553994557));
#242626=CARTESIAN_POINT('Ctrl Pts',(-6.94428807262208,15.2,8.46292744819662));
#242627=CARTESIAN_POINT('Ctrl Pts',(-6.94564954147413,15.2,8.46663935695343));
#242628=CARTESIAN_POINT('Ctrl Pts',(-6.94700990665818,15.2,8.47036714209802));
#242629=CARTESIAN_POINT('Ctrl Pts',(-6.94836905618895,15.2,8.47411073576823));
#242630=CARTESIAN_POINT('Ctrl Pts',(-6.9500679930098,15.2,8.47879022760096));
#242631=CARTESIAN_POINT('Ctrl Pts',(-6.9517650284997,15.2,8.48349441949977));
#242632=CARTESIAN_POINT('Ctrl Pts',(-6.95345994801342,15.2,8.48822317783513));
#242633=CARTESIAN_POINT('Ctrl Pts',(-6.95481588351355,15.2,8.49200618419414));
#242634=CARTESIAN_POINT('Ctrl Pts',(-6.95617046593052,15.2,8.49580491245943));
#242635=CARTESIAN_POINT('Ctrl Pts',(-6.9575235834311,15.2,8.4996192959799));
#242636=CARTESIAN_POINT('Ctrl Pts',(-6.95887670111603,15.2,8.50343368002008));
#242637=CARTESIAN_POINT('Ctrl Pts',(-6.96022835561194,15.2,8.50726371646497));
#242638=CARTESIAN_POINT('Ctrl Pts',(-6.96157843785209,15.2,8.51110934056446));
#242639=CARTESIAN_POINT('Ctrl Pts',(-6.96292851990828,15.2,8.51495496413997));
#242640=CARTESIAN_POINT('Ctrl Pts',(-6.96427703096119,15.2,8.51881617387873));
#242641=CARTESIAN_POINT('Ctrl Pts',(-6.96562386252962,15.2,8.5226929024208));
#242642=CARTESIAN_POINT('Ctrl Pts',(-6.96697069428156,15.2,8.52656963149107));
#242643=CARTESIAN_POINT('Ctrl Pts',(-6.96831584733122,15.2,8.53046187900832));
#242644=CARTESIAN_POINT('Ctrl Pts',(-6.96965921562653,15.2,8.53436957661119));
#242645=CARTESIAN_POINT('Ctrl Pts',(-6.9710025837388,15.2,8.53827727368162));
#242646=CARTESIAN_POINT('Ctrl Pts',(-6.9723441675459,15.2,8.54220042215731));
#242647=CARTESIAN_POINT('Ctrl Pts',(-6.97368386054769,15.2,8.54613895438931));
#242648=CARTESIAN_POINT('Ctrl Pts',(-6.975023553732,15.2,8.55007748715793));
#242649=CARTESIAN_POINT('Ctrl Pts',(-6.97636135866378,15.2,8.55403140365157));
#242650=CARTESIAN_POINT('Ctrl Pts',(-6.97769717024264,15.2,8.5580006372193));
#242651=CARTESIAN_POINT('Ctrl Pts',(-6.97903298163949,15.2,8.56196987024621));
#242652=CARTESIAN_POINT('Ctrl Pts',(-6.98036679895209,15.2,8.56595442136061));
#242653=CARTESIAN_POINT('Ctrl Pts',(-6.98169852173233,15.2,8.56995422108763));
#242654=CARTESIAN_POINT('Ctrl Pts',(-6.98303024469401,15.2,8.57395402135962));
#242655=CARTESIAN_POINT('Ctrl Pts',(-6.98435987175828,15.2,8.57796907155528));
#242656=CARTESIAN_POINT('Ctrl Pts',(-6.98568730144173,15.2,8.58199930627493));
#242657=CARTESIAN_POINT('Ctrl Pts',(-6.98701473112519,15.2,8.58602954099457));
#242658=CARTESIAN_POINT('Ctrl Pts',(-6.98833996387227,15.2,8.59007495818822));
#242659=CARTESIAN_POINT('Ctrl Pts',(-6.9896628994997,15.2,8.59413549368883));
#242660=CARTESIAN_POINT('Ctrl Pts',(-6.99098583494687,15.2,8.5981960286362));
#242661=CARTESIAN_POINT('Ctrl Pts',(-6.99230647146206,15.2,8.6022716807575));
#242662=CARTESIAN_POINT('Ctrl Pts',(-6.99362471224917,15.2,8.60636238499714));
#242663=CARTESIAN_POINT('Ctrl Pts',(-6.99494295321589,15.2,8.61045308979415));
#242664=CARTESIAN_POINT('Ctrl Pts',(-6.9962587959907,15.2,8.61455884454201));
#242665=CARTESIAN_POINT('Ctrl Pts',(-6.99757214500647,15.2,8.61867958665702));
#242666=CARTESIAN_POINT('Ctrl Pts',(-6.99888549384329,15.2,8.62280032821057));
#242667=CARTESIAN_POINT('Ctrl Pts',(-7.00019634616376,15.2,8.62693605420104));
#242668=CARTESIAN_POINT('Ctrl Pts',(-7.00150460633476,15.2,8.63108670119409));
#242669=CARTESIAN_POINT('Ctrl Pts',(-7.002812866684,15.2,8.63523734875266));
#242670=CARTESIAN_POINT('Ctrl Pts',(-7.00411853537548,15.2,8.63940291613535));
#242671=CARTESIAN_POINT('Ctrl Pts',(-7.00542151395579,15.2,8.64358333857328));
#242672=CARTESIAN_POINT('Ctrl Pts',(-7.00672449235856,15.2,8.64776376044163));
#242673=CARTESIAN_POINT('Ctrl Pts',(-7.0080247823332,15.2,8.65195903723162));
#242674=CARTESIAN_POINT('Ctrl Pts',(-7.00932228789397,15.2,8.65616910416422));
#242675=CARTESIAN_POINT('Ctrl Pts',(-7.01126854650029,15.2,8.66248420542356));
#242676=CARTESIAN_POINT('Ctrl Pts',(-7.01320853957256,15.2,8.66883258261215));
#242677=CARTESIAN_POINT('Ctrl Pts',(-7.01514195017748,15.2,8.67521401896219));
#242678=CARTESIAN_POINT('Ctrl Pts',(-7.01643089040514,15.2,8.67946830928259));
#242679=CARTESIAN_POINT('Ctrl Pts',(-7.0177169042149,15.2,8.68373729154168));
#242680=CARTESIAN_POINT('Ctrl Pts',(-7.01899990044919,15.2,8.68802090248868));
#242681=CARTESIAN_POINT('Ctrl Pts',(-7.01996214766861,15.2,8.69123361084483));
#242682=CARTESIAN_POINT('Ctrl Pts',(-7.02092269718022,15.2,8.69445454756615));
#242683=CARTESIAN_POINT('Ctrl Pts',(-7.02188150939553,15.2,8.69768368540642));
#242684=CARTESIAN_POINT('Ctrl Pts',(-7.02284032161084,15.2,8.70091282324669));
#242685=CARTESIAN_POINT('Ctrl Pts',(-7.02379739662628,15.2,8.7041501614781));
#242686=CARTESIAN_POINT('Ctrl Pts',(-7.02475269680015,15.2,8.70739567477574));
#242687=CARTESIAN_POINT('Ctrl Pts',(-7.02570799714756,15.2,8.71064118866297));
#242688=CARTESIAN_POINT('Ctrl Pts',(-7.02666152103614,15.2,8.71389487600254));
#242689=CARTESIAN_POINT('Ctrl Pts',(-7.02761323196587,15.2,8.71715671047769));
#242690=CARTESIAN_POINT('Ctrl Pts',(-7.02919941644535,15.2,8.72259309988696));
#242691=CARTESIAN_POINT('Ctrl Pts',(-7.03078056335973,15.2,8.72805212055449));
#242692=CARTESIAN_POINT('Ctrl Pts',(-7.0323564960356,15.2,8.73353364731628));
#242693=CARTESIAN_POINT('Ctrl Pts',(-7.03330205588161,15.2,8.73682256420984));
#242694=CARTESIAN_POINT('Ctrl Pts',(-7.03424573836877,15.2,8.74011958205567));
#242695=CARTESIAN_POINT('Ctrl Pts',(-7.03518750675538,15.2,8.74342467649546));
#242696=CARTESIAN_POINT('Ctrl Pts',(-7.03612927497089,15.2,8.74672977033481));
#242697=CARTESIAN_POINT('Ctrl Pts',(-7.03706912836985,15.2,8.75004293911539));
#242698=CARTESIAN_POINT('Ctrl Pts',(-7.03800703062727,15.2,8.75336415607875));
#242699=CARTESIAN_POINT('Ctrl Pts',(-7.0392575669137,15.2,8.7577924451621));
#242700=CARTESIAN_POINT('Ctrl Pts',(-7.04050463291439,15.2,8.76223504366289));
#242701=CARTESIAN_POINT('Ctrl Pts',(-7.04174814131961,15.2,8.7666918868533));
#242702=CARTESIAN_POINT('Ctrl Pts',(-7.04268077266588,15.2,8.77003451939792));
#242703=CARTESIAN_POINT('Ctrl Pts',(-7.04361140326443,15.2,8.77338516465752));
#242704=CARTESIAN_POINT('Ctrl Pts',(-7.0445399960643,15.2,8.77674379649274));
#242705=CARTESIAN_POINT('Ctrl Pts',(-7.04577811990992,15.2,8.78122197267979));
#242706=CARTESIAN_POINT('Ctrl Pts',(-7.04701262147466,15.2,8.78571434555435));
#242707=CARTESIAN_POINT('Ctrl Pts',(-7.04824341404174,15.2,8.7902208544666));
#242708=CARTESIAN_POINT('Ctrl Pts',(-7.0491665083832,15.2,8.79360073584377));
#242709=CARTESIAN_POINT('Ctrl Pts',(-7.05008751726641,15.2,8.796988568254));
#242710=CARTESIAN_POINT('Ctrl Pts',(-7.05100640314988,15.2,8.80038432458826));
#242711=CARTESIAN_POINT('Ctrl Pts',(-7.05192528903334,15.2,8.80378008092251));
#242712=CARTESIAN_POINT('Ctrl Pts',(-7.05284205296039,15.2,8.80718376067771));
#242713=CARTESIAN_POINT('Ctrl Pts',(-7.05375665930643,15.2,8.81059533959828));
#242714=CARTESIAN_POINT('Ctrl Pts',(-7.05528100327188,15.2,8.81628130467248));
#242715=CARTESIAN_POINT('Ctrl Pts',(-7.05679935279526,15.2,8.8219892064598));
#242716=CARTESIAN_POINT('Ctrl Pts',(-7.05831154418447,15.2,8.82771892562533));
#242717=CARTESIAN_POINT('Ctrl Pts',(-7.05921885898503,15.2,8.83115675699974));
#242718=CARTESIAN_POINT('Ctrl Pts',(-7.06012395650242,15.2,8.83460244210696));
#242719=CARTESIAN_POINT('Ctrl Pts',(-7.06102680276158,15.2,8.8380559549804));
#242720=CARTESIAN_POINT('Ctrl Pts',(-7.06192964918476,15.2,8.84150946848124));
#242721=CARTESIAN_POINT('Ctrl Pts',(-7.06283024308232,15.2,8.84497080950095));
#242722=CARTESIAN_POINT('Ctrl Pts',(-7.06372855096257,15.2,8.8484399520062));
#242723=CARTESIAN_POINT('Ctrl Pts',(-7.06462685867962,15.2,8.85190909388123));
#242724=CARTESIAN_POINT('Ctrl Pts',(-7.06552287901346,15.2,8.85538603698917));
#242725=CARTESIAN_POINT('Ctrl Pts',(-7.06641657789745,15.2,8.85887075536323));
#242726=CARTESIAN_POINT('Ctrl Pts',(-7.06760817635531,15.2,8.86351704631761));
#242727=CARTESIAN_POINT('Ctrl Pts',(-7.06879564930727,15.2,8.86817715920215));
#242728=CARTESIAN_POINT('Ctrl Pts',(-7.06997891310335,15.2,8.87285103433012));
#242729=CARTESIAN_POINT('Ctrl Pts',(-7.07086636099071,15.2,8.87635644083529));
#242730=CARTESIAN_POINT('Ctrl Pts',(-7.07175144172273,15.2,8.8798695873447));
#242731=CARTESIAN_POINT('Ctrl Pts',(-7.07263412156598,15.2,8.88339044775738));
#242732=CARTESIAN_POINT('Ctrl Pts',(-7.07381102813055,15.2,8.88808492873404));
#242733=CARTESIAN_POINT('Ctrl Pts',(-7.07498366564195,15.2,8.89279312302312));
#242734=CARTESIAN_POINT('Ctrl Pts',(-7.07615195548341,15.2,8.89751497122494));
#242735=CARTESIAN_POINT('Ctrl Pts',(-7.07702817278492,15.2,8.90105635705463));
#242736=CARTESIAN_POINT('Ctrl Pts',(-7.07790194381983,15.2,8.90460542295895));
#242737=CARTESIAN_POINT('Ctrl Pts',(-7.07877323566339,15.2,8.90816214191238));
#242738=CARTESIAN_POINT('Ctrl Pts',(-7.07964452750695,15.2,8.9117188608658));
#242739=CARTESIAN_POINT('Ctrl Pts',(-7.080513340187,15.2,8.9152832339111));
#242740=CARTESIAN_POINT('Ctrl Pts',(-7.08137964007411,15.2,8.91885523500058));
#242741=CARTESIAN_POINT('Ctrl Pts',(-7.08224593996121,15.2,8.92242723609006));
#242742=CARTESIAN_POINT('Ctrl Pts',(-7.08310972644326,15.2,8.92600686484928));
#242743=CARTESIAN_POINT('Ctrl Pts',(-7.08397096778732,15.2,8.92959409521793));
#242744=CARTESIAN_POINT('Ctrl Pts',(-7.0851192896837,15.2,8.93437706947724));
#242745=CARTESIAN_POINT('Ctrl Pts',(-7.08626308638521,15.2,8.93917355733779));
#242746=CARTESIAN_POINT('Ctrl Pts',(-7.08740227972508,15.2,8.9439835002666));
#242747=CARTESIAN_POINT('Ctrl Pts',(-7.08825667465236,15.2,8.94759095713553));
#242748=CARTESIAN_POINT('Ctrl Pts',(-7.08910848122144,15.2,8.95120598212082));
#242749=CARTESIAN_POINT('Ctrl Pts',(-7.08995766614914,15.2,8.95482854861353));
#242750=CARTESIAN_POINT('Ctrl Pts',(-7.09080685107684,15.2,8.95845111510624));
#242751=CARTESIAN_POINT('Ctrl Pts',(-7.09165341559164,15.2,8.96208122516421));
#242752=CARTESIAN_POINT('Ctrl Pts',(-7.09249732456177,15.2,8.96571884979622));
#242753=CARTESIAN_POINT('Ctrl Pts',(-7.09334123353191,15.2,8.96935647442823));
#242754=CARTESIAN_POINT('Ctrl Pts',(-7.09418248806403,15.2,8.97300161397071));
#242755=CARTESIAN_POINT('Ctrl Pts',(-7.0950210550756,15.2,8.97665424392033));
#242756=CARTESIAN_POINT('Ctrl Pts',(-7.0958596222395,15.2,8.98030687453351));
#242757=CARTESIAN_POINT('Ctrl Pts',(-7.09669550409432,15.2,8.98396699618209));
#242758=CARTESIAN_POINT('Ctrl Pts',(-7.09752867067337,15.2,8.98763458429948));
#242759=CARTESIAN_POINT('Ctrl Pts',(-7.09863955919318,15.2,8.99252470067887));
#242760=CARTESIAN_POINT('Ctrl Pts',(-7.09974562193026,15.2,8.99742809292313));
#242761=CARTESIAN_POINT('Ctrl Pts',(-7.10084677945168,15.2,9.00234469629812));
#242762=CARTESIAN_POINT('Ctrl Pts',(-7.10222322646597,15.2,9.00849045101926));
#242763=CARTESIAN_POINT('Ctrl Pts',(-7.10359199720425,15.2,9.01465683859633));
#242764=CARTESIAN_POINT('Ctrl Pts',(-7.10495293922433,15.2,9.02084373647156));
#242765=CARTESIAN_POINT('Ctrl Pts',(-7.10631388124442,15.2,9.02703063434678));
#242766=CARTESIAN_POINT('Ctrl Pts',(-7.10766700189186,15.2,9.03323804195593));
#242767=CARTESIAN_POINT('Ctrl Pts',(-7.10901226900006,15.2,9.03946594399999));
#242768=CARTESIAN_POINT('Origin',(-5.66257110645729E-14,15.2,-1.77635683940025E-14));
#242769=CARTESIAN_POINT('',(-7.01216898600006,15.2,7.64657512399998));
#242770=CARTESIAN_POINT('',(-7.01216898600006,12.2,7.64657512399998));
#242771=CARTESIAN_POINT('',(-7.01216898600006,15.2,7.64657512399998));
#242772=CARTESIAN_POINT('Origin',(-5.66257110645729E-14,12.2,-1.77635683940025E-14));
#242773=CARTESIAN_POINT('Origin',(-5.66257110645729E-14,15.2,-1.77635683940025E-14));
#242774=CARTESIAN_POINT('Origin',(-5.66257110645729E-14,15.2,-1.77635683940025E-14));
#242775=CARTESIAN_POINT('',(-8.05377977200006,15.2,8.20893606999999));
#242776=CARTESIAN_POINT('',(-8.32310290947582,15.2,7.93573928281797));
#242777=CARTESIAN_POINT('Origin',(-5.66257110645729E-14,15.2,-1.77635683940025E-14));
#242778=CARTESIAN_POINT('',(-8.32310290947582,12.2,7.93573928281797));
#242779=CARTESIAN_POINT('',(-8.32310291000006,15.2,7.93573928299999));
#242780=CARTESIAN_POINT('',(-8.05377977200006,12.2,8.20893606999999));
#242781=CARTESIAN_POINT('Origin',(-5.66257110645729E-14,12.2,-1.77635683940025E-14));
#242782=CARTESIAN_POINT('',(-8.05377977200006,15.2,8.20893606999999));
#242783=CARTESIAN_POINT('Ctrl Pts',(-8.32310290900006,15.2,7.93573928299999));
#242784=CARTESIAN_POINT('Ctrl Pts',(-8.32310290900006,11.6,7.93573928299999));
#242785=CARTESIAN_POINT('Ctrl Pts',(-8.32283676100005,15.2,7.93502251699999));
#242786=CARTESIAN_POINT('Ctrl Pts',(-8.32283676100005,11.6,7.93502251699999));
#242787=CARTESIAN_POINT('Ctrl Pts',(-8.32230434900006,15.2,7.93358949599998));
#242788=CARTESIAN_POINT('Ctrl Pts',(-8.32230434900006,11.6,7.93358949599998));
#242789=CARTESIAN_POINT('Ctrl Pts',(-8.32150538200005,15.2,7.93144150699998));
#242790=CARTESIAN_POINT('Ctrl Pts',(-8.32150538200005,11.6,7.93144150699998));
#242791=CARTESIAN_POINT('Ctrl Pts',(-8.32043939300006,15.2,7.92858060399999));
#242792=CARTESIAN_POINT('Ctrl Pts',(-8.32043939300006,11.6,7.92858060399999));
#242793=CARTESIAN_POINT('Ctrl Pts',(-8.31910574600006,15.2,7.92500961199998));
#242794=CARTESIAN_POINT('Ctrl Pts',(-8.31910574600006,11.6,7.92500961199998));
#242795=CARTESIAN_POINT('Ctrl Pts',(-8.31777093800006,15.2,7.92144375699999));
#242796=CARTESIAN_POINT('Ctrl Pts',(-8.31777093800006,11.6,7.92144375699999));
#242797=CARTESIAN_POINT('Ctrl Pts',(-8.31643496900006,15.2,7.91788304099998));
#242798=CARTESIAN_POINT('Ctrl Pts',(-8.31643496900006,11.6,7.91788304099998));
#242799=CARTESIAN_POINT('Ctrl Pts',(-8.31509784400006,15.2,7.91432746599998));
#242800=CARTESIAN_POINT('Ctrl Pts',(-8.31509784400006,11.6,7.91432746599998));
#242801=CARTESIAN_POINT('Ctrl Pts',(-8.31375956800006,15.2,7.91077703599999));
#242802=CARTESIAN_POINT('Ctrl Pts',(-8.31375956800006,11.6,7.91077703599999));
#242803=CARTESIAN_POINT('Ctrl Pts',(-8.31242014800005,15.2,7.90723175399999));
#242804=CARTESIAN_POINT('Ctrl Pts',(-8.31242014800005,11.6,7.90723175399999));
#242805=CARTESIAN_POINT('Ctrl Pts',(-8.31107959100006,15.2,7.90369162599998));
#242806=CARTESIAN_POINT('Ctrl Pts',(-8.31107959100006,11.6,7.90369162599998));
#242807=CARTESIAN_POINT('Ctrl Pts',(-8.30973790700006,15.2,7.90015665599999));
#242808=CARTESIAN_POINT('Ctrl Pts',(-8.30973790700006,11.6,7.90015665599999));
#242809=CARTESIAN_POINT('Ctrl Pts',(-8.30839510700006,15.2,7.89662685099999));
#242810=CARTESIAN_POINT('Ctrl Pts',(-8.30839510700006,11.6,7.89662685099999));
#242811=CARTESIAN_POINT('Ctrl Pts',(-8.30705119900006,15.2,7.89310221799998));
#242812=CARTESIAN_POINT('Ctrl Pts',(-8.30705119900006,11.6,7.89310221799998));
#242813=CARTESIAN_POINT('Ctrl Pts',(-8.30570619200006,15.2,7.88958275899999));
#242814=CARTESIAN_POINT('Ctrl Pts',(-8.30570619200006,11.6,7.88958275899999));
#242815=CARTESIAN_POINT('Ctrl Pts',(-8.30436009500006,15.2,7.88606848099998));
#242816=CARTESIAN_POINT('Ctrl Pts',(-8.30436009500006,11.6,7.88606848099998));
#242817=CARTESIAN_POINT('Ctrl Pts',(-8.30301291400006,15.2,7.88255938899999));
#242818=CARTESIAN_POINT('Ctrl Pts',(-8.30301291400006,11.6,7.88255938899999));
#242819=CARTESIAN_POINT('Ctrl Pts',(-8.30166465900006,15.2,7.87905548499998));
#242820=CARTESIAN_POINT('Ctrl Pts',(-8.30166465900006,11.6,7.87905548499998));
#242821=CARTESIAN_POINT('Ctrl Pts',(-8.30031533400006,15.2,7.87555677499999));
#242822=CARTESIAN_POINT('Ctrl Pts',(-8.30031533400006,11.6,7.87555677499999));
#242823=CARTESIAN_POINT('Ctrl Pts',(-8.29896494600005,15.2,7.87206326199998));
#242824=CARTESIAN_POINT('Ctrl Pts',(-8.29896494600005,11.6,7.87206326199998));
#242825=CARTESIAN_POINT('Ctrl Pts',(-8.29761350500006,15.2,7.86857495199998));
#242826=CARTESIAN_POINT('Ctrl Pts',(-8.29761350500006,11.6,7.86857495199998));
#242827=CARTESIAN_POINT('Ctrl Pts',(-8.29626101600006,15.2,7.86509184699998));
#242828=CARTESIAN_POINT('Ctrl Pts',(-8.29626101600006,11.6,7.86509184699998));
#242829=CARTESIAN_POINT('Ctrl Pts',(-8.29490748900006,15.2,7.86161395399999));
#242830=CARTESIAN_POINT('Ctrl Pts',(-8.29490748900006,11.6,7.86161395399999));
#242831=CARTESIAN_POINT('Ctrl Pts',(-8.29355293100006,15.2,7.85814127699999));
#242832=CARTESIAN_POINT('Ctrl Pts',(-8.29355293100006,11.6,7.85814127699999));
#242833=CARTESIAN_POINT('Ctrl Pts',(-8.29219735000006,15.2,7.85467382099998));
#242834=CARTESIAN_POINT('Ctrl Pts',(-8.29219735000006,11.6,7.85467382099998));
#242835=CARTESIAN_POINT('Ctrl Pts',(-8.29084075600005,15.2,7.85121158999999));
#242836=CARTESIAN_POINT('Ctrl Pts',(-8.29084075600005,11.6,7.85121158999999));
#242837=CARTESIAN_POINT('Ctrl Pts',(-8.28948315500006,15.2,7.84775459099999));
#242838=CARTESIAN_POINT('Ctrl Pts',(-8.28948315500006,11.6,7.84775459099999));
#242839=CARTESIAN_POINT('Ctrl Pts',(-8.28812455600006,15.2,7.84430282599998));
#242840=CARTESIAN_POINT('Ctrl Pts',(-8.28812455600006,11.6,7.84430282599998));
#242841=CARTESIAN_POINT('Ctrl Pts',(-8.28676496700006,15.2,7.84085629999999));
#242842=CARTESIAN_POINT('Ctrl Pts',(-8.28676496700006,11.6,7.84085629999999));
#242843=CARTESIAN_POINT('Ctrl Pts',(-8.28540439600006,15.2,7.83741501799998));
#242844=CARTESIAN_POINT('Ctrl Pts',(-8.28540439600006,11.6,7.83741501799998));
#242845=CARTESIAN_POINT('Ctrl Pts',(-8.28404285000006,15.2,7.83397898599999));
#242846=CARTESIAN_POINT('Ctrl Pts',(-8.28404285000006,11.6,7.83397898599999));
#242847=CARTESIAN_POINT('Ctrl Pts',(-8.28268033800006,15.2,7.83054820599999));
#242848=CARTESIAN_POINT('Ctrl Pts',(-8.28268033800006,11.6,7.83054820599999));
#242849=CARTESIAN_POINT('Ctrl Pts',(-8.28131686600006,15.2,7.82712268499999));
#242850=CARTESIAN_POINT('Ctrl Pts',(-8.28131686600006,11.6,7.82712268499999));
#242851=CARTESIAN_POINT('Ctrl Pts',(-8.27995244500006,15.2,7.82370242499999));
#242852=CARTESIAN_POINT('Ctrl Pts',(-8.27995244500006,11.6,7.82370242499999));
#242853=CARTESIAN_POINT('Ctrl Pts',(-8.27858708000005,15.2,7.82028743299998));
#242854=CARTESIAN_POINT('Ctrl Pts',(-8.27858708000005,11.6,7.82028743299998));
#242855=CARTESIAN_POINT('Ctrl Pts',(-8.27722078100006,15.2,7.81687771299998));
#242856=CARTESIAN_POINT('Ctrl Pts',(-8.27722078100006,11.6,7.81687771299998));
#242857=CARTESIAN_POINT('Ctrl Pts',(-8.27585355600006,15.2,7.81347326899999));
#242858=CARTESIAN_POINT('Ctrl Pts',(-8.27585355600006,11.6,7.81347326899999));
#242859=CARTESIAN_POINT('Ctrl Pts',(-8.27448541300006,15.2,7.81007410599998));
#242860=CARTESIAN_POINT('Ctrl Pts',(-8.27448541300006,11.6,7.81007410599998));
#242861=CARTESIAN_POINT('Ctrl Pts',(-8.27311636000006,15.2,7.80668022899999));
#242862=CARTESIAN_POINT('Ctrl Pts',(-8.27311636000006,11.6,7.80668022899999));
#242863=CARTESIAN_POINT('Ctrl Pts',(-8.27174640600006,15.2,7.80329164399999));
#242864=CARTESIAN_POINT('Ctrl Pts',(-8.27174640600006,11.6,7.80329164399999));
#242865=CARTESIAN_POINT('Ctrl Pts',(-8.27037555700005,15.2,7.79990835199998));
#242866=CARTESIAN_POINT('Ctrl Pts',(-8.27037555700005,11.6,7.79990835199998));
#242867=CARTESIAN_POINT('Ctrl Pts',(-8.26900382400006,15.2,7.79653036099998));
#242868=CARTESIAN_POINT('Ctrl Pts',(-8.26900382400006,11.6,7.79653036099998));
#242869=CARTESIAN_POINT('Ctrl Pts',(-8.26763121300005,15.2,7.79315767299998));
#242870=CARTESIAN_POINT('Ctrl Pts',(-8.26763121300005,11.6,7.79315767299998));
#242871=CARTESIAN_POINT('Ctrl Pts',(-8.26625773300006,15.2,7.78979029499999));
#242872=CARTESIAN_POINT('Ctrl Pts',(-8.26625773300006,11.6,7.78979029499999));
#242873=CARTESIAN_POINT('Ctrl Pts',(-8.26488339300005,15.2,7.78642823099998));
#242874=CARTESIAN_POINT('Ctrl Pts',(-8.26488339300005,11.6,7.78642823099998));
#242875=CARTESIAN_POINT('Ctrl Pts',(-8.26350820000006,15.2,7.78307148499999));
#242876=CARTESIAN_POINT('Ctrl Pts',(-8.26350820000006,11.6,7.78307148499999));
#242877=CARTESIAN_POINT('Ctrl Pts',(-8.26213216200006,15.2,7.77972006199998));
#242878=CARTESIAN_POINT('Ctrl Pts',(-8.26213216200006,11.6,7.77972006199998));
#242879=CARTESIAN_POINT('Ctrl Pts',(-8.26075528800006,15.2,7.77637396599999));
#242880=CARTESIAN_POINT('Ctrl Pts',(-8.26075528800006,11.6,7.77637396599999));
#242881=CARTESIAN_POINT('Ctrl Pts',(-8.25937758800006,15.2,7.77303320299998));
#242882=CARTESIAN_POINT('Ctrl Pts',(-8.25937758800006,11.6,7.77303320299998));
#242883=CARTESIAN_POINT('Ctrl Pts',(-8.25799906800006,15.2,7.76969777699998));
#242884=CARTESIAN_POINT('Ctrl Pts',(-8.25799906800006,11.6,7.76969777699998));
#242885=CARTESIAN_POINT('Ctrl Pts',(-8.25661973700005,15.2,7.76636769199998));
#242886=CARTESIAN_POINT('Ctrl Pts',(-8.25661973700005,11.6,7.76636769199998));
#242887=CARTESIAN_POINT('Ctrl Pts',(-8.25523960300006,15.2,7.76304295399999));
#242888=CARTESIAN_POINT('Ctrl Pts',(-8.25523960300006,11.6,7.76304295399999));
#242889=CARTESIAN_POINT('Ctrl Pts',(-8.25385867600006,15.2,7.75972356699998));
#242890=CARTESIAN_POINT('Ctrl Pts',(-8.25385867600006,11.6,7.75972356699998));
#242891=CARTESIAN_POINT('Ctrl Pts',(-8.25247696300006,15.2,7.75640953499998));
#242892=CARTESIAN_POINT('Ctrl Pts',(-8.25247696300006,11.6,7.75640953499998));
#242893=CARTESIAN_POINT('Ctrl Pts',(-8.25109447200006,15.2,7.75310086299999));
#242894=CARTESIAN_POINT('Ctrl Pts',(-8.25109447200006,11.6,7.75310086299999));
#242895=CARTESIAN_POINT('Ctrl Pts',(-8.24971121300005,15.2,7.74979755699999));
#242896=CARTESIAN_POINT('Ctrl Pts',(-8.24971121300005,11.6,7.74979755699999));
#242897=CARTESIAN_POINT('Ctrl Pts',(-8.24832719300005,15.2,7.74649961999998));
#242898=CARTESIAN_POINT('Ctrl Pts',(-8.24832719300005,11.6,7.74649961999998));
#242899=CARTESIAN_POINT('Ctrl Pts',(-8.24694242100006,15.2,7.74320705699999));
#242900=CARTESIAN_POINT('Ctrl Pts',(-8.24694242100006,11.6,7.74320705699999));
#242901=CARTESIAN_POINT('Ctrl Pts',(-8.24555690700005,15.2,7.73991987299999));
#242902=CARTESIAN_POINT('Ctrl Pts',(-8.24555690700005,11.6,7.73991987299999));
#242903=CARTESIAN_POINT('Ctrl Pts',(-8.24417065700005,15.2,7.73663807299998));
#242904=CARTESIAN_POINT('Ctrl Pts',(-8.24417065700005,11.6,7.73663807299998));
#242905=CARTESIAN_POINT('Ctrl Pts',(-8.24278368100006,15.2,7.73336166199999));
#242906=CARTESIAN_POINT('Ctrl Pts',(-8.24278368100006,11.6,7.73336166199999));
#242907=CARTESIAN_POINT('Ctrl Pts',(-8.24139598700006,15.2,7.73009064299998));
#242908=CARTESIAN_POINT('Ctrl Pts',(-8.24139598700006,11.6,7.73009064299998));
#242909=CARTESIAN_POINT('Ctrl Pts',(-8.24000758500006,15.2,7.72682502199999));
#242910=CARTESIAN_POINT('Ctrl Pts',(-8.24000758500006,11.6,7.72682502199999));
#242911=CARTESIAN_POINT('Ctrl Pts',(-8.23861848100006,15.2,7.72356480299998));
#242912=CARTESIAN_POINT('Ctrl Pts',(-8.23861848100006,11.6,7.72356480299998));
#242913=CARTESIAN_POINT('Ctrl Pts',(-8.23722868600005,15.2,7.72030999099999));
#242914=CARTESIAN_POINT('Ctrl Pts',(-8.23722868600005,11.6,7.72030999099999));
#242915=CARTESIAN_POINT('Ctrl Pts',(-8.23583820700006,15.2,7.71706059099999));
#242916=CARTESIAN_POINT('Ctrl Pts',(-8.23583820700006,11.6,7.71706059099999));
#242917=CARTESIAN_POINT('Ctrl Pts',(-8.23444705400006,15.2,7.71381660699999));
#242918=CARTESIAN_POINT('Ctrl Pts',(-8.23444705400006,11.6,7.71381660699999));
#242919=CARTESIAN_POINT('Ctrl Pts',(-8.23305523500006,15.2,7.71057804499999));
#242920=CARTESIAN_POINT('Ctrl Pts',(-8.23305523500006,11.6,7.71057804499999));
#242921=CARTESIAN_POINT('Ctrl Pts',(-8.23166275900006,15.2,7.70734490799998));
#242922=CARTESIAN_POINT('Ctrl Pts',(-8.23166275900006,11.6,7.70734490799998));
#242923=CARTESIAN_POINT('Ctrl Pts',(-8.23026963300006,15.2,7.70411720099998));
#242924=CARTESIAN_POINT('Ctrl Pts',(-8.23026963300006,11.6,7.70411720099998));
#242925=CARTESIAN_POINT('Ctrl Pts',(-8.22887586900006,15.2,7.70089492999999));
#242926=CARTESIAN_POINT('Ctrl Pts',(-8.22887586900006,11.6,7.70089492999999));
#242927=CARTESIAN_POINT('Ctrl Pts',(-8.22748147400005,15.2,7.69767809899999));
#242928=CARTESIAN_POINT('Ctrl Pts',(-8.22748147400005,11.6,7.69767809899999));
#242929=CARTESIAN_POINT('Ctrl Pts',(-8.22608645600006,15.2,7.69446671199999));
#242930=CARTESIAN_POINT('Ctrl Pts',(-8.22608645600006,11.6,7.69446671199999));
#242931=CARTESIAN_POINT('Ctrl Pts',(-8.22469082500006,15.2,7.69126077399999));
#242932=CARTESIAN_POINT('Ctrl Pts',(-8.22469082500006,11.6,7.69126077399999));
#242933=CARTESIAN_POINT('Ctrl Pts',(-8.22329458800005,15.2,7.68806028999999));
#242934=CARTESIAN_POINT('Ctrl Pts',(-8.22329458800005,11.6,7.68806028999999));
#242935=CARTESIAN_POINT('Ctrl Pts',(-8.22189775700006,15.2,7.68486526499998));
#242936=CARTESIAN_POINT('Ctrl Pts',(-8.22189775700006,11.6,7.68486526499998));
#242937=CARTESIAN_POINT('Ctrl Pts',(-8.22050033900006,15.2,7.68167570299998));
#242938=CARTESIAN_POINT('Ctrl Pts',(-8.22050033900006,11.6,7.68167570299998));
#242939=CARTESIAN_POINT('Ctrl Pts',(-8.21910234200006,15.2,7.67849160899999));
#242940=CARTESIAN_POINT('Ctrl Pts',(-8.21910234200006,11.6,7.67849160899999));
#242941=CARTESIAN_POINT('Ctrl Pts',(-8.21770377700006,15.2,7.67531298799998));
#242942=CARTESIAN_POINT('Ctrl Pts',(-8.21770377700006,11.6,7.67531298799998));
#242943=CARTESIAN_POINT('Ctrl Pts',(-8.21630465100006,15.2,7.67213984399999));
#242944=CARTESIAN_POINT('Ctrl Pts',(-8.21630465100006,11.6,7.67213984399999));
#242945=CARTESIAN_POINT('Ctrl Pts',(-8.21490497400006,15.2,7.66897218199999));
#242946=CARTESIAN_POINT('Ctrl Pts',(-8.21490497400006,11.6,7.66897218199999));
#242947=CARTESIAN_POINT('Ctrl Pts',(-8.21350475500006,15.2,7.66581000699999));
#242948=CARTESIAN_POINT('Ctrl Pts',(-8.21350475500006,11.6,7.66581000699999));
#242949=CARTESIAN_POINT('Ctrl Pts',(-8.21210400200006,15.2,7.66265332299999));
#242950=CARTESIAN_POINT('Ctrl Pts',(-8.21210400200006,11.6,7.66265332299999));
#242951=CARTESIAN_POINT('Ctrl Pts',(-8.21070272500006,15.2,7.65950213599999));
#242952=CARTESIAN_POINT('Ctrl Pts',(-8.21070272500006,11.6,7.65950213599999));
#242953=CARTESIAN_POINT('Ctrl Pts',(-8.20930093300005,15.2,7.65635645099999));
#242954=CARTESIAN_POINT('Ctrl Pts',(-8.20930093300005,11.6,7.65635645099999));
#242955=CARTESIAN_POINT('Ctrl Pts',(-8.20789863500006,15.2,7.65321626999998));
#242956=CARTESIAN_POINT('Ctrl Pts',(-8.20789863500006,11.6,7.65321626999998));
#242957=CARTESIAN_POINT('Ctrl Pts',(-8.20649583900006,15.2,7.65008159999999));
#242958=CARTESIAN_POINT('Ctrl Pts',(-8.20649583900006,11.6,7.65008159999999));
#242959=CARTESIAN_POINT('Ctrl Pts',(-8.20509255500006,15.2,7.64695244499999));
#242960=CARTESIAN_POINT('Ctrl Pts',(-8.20509255500006,11.6,7.64695244499999));
#242961=CARTESIAN_POINT('Ctrl Pts',(-8.20368879300006,15.2,7.64382880899999));
#242962=CARTESIAN_POINT('Ctrl Pts',(-8.20368879300006,11.6,7.64382880899999));
#242963=CARTESIAN_POINT('Ctrl Pts',(-8.20228456100006,15.2,7.64071069899998));
#242964=CARTESIAN_POINT('Ctrl Pts',(-8.20228456100006,11.6,7.64071069899998));
#242965=CARTESIAN_POINT('Ctrl Pts',(-8.20087986700005,15.2,7.63759811799999));
#242966=CARTESIAN_POINT('Ctrl Pts',(-8.20087986700005,11.6,7.63759811799999));
#242967=CARTESIAN_POINT('Ctrl Pts',(-8.19947472300005,15.2,7.63449107099999));
#242968=CARTESIAN_POINT('Ctrl Pts',(-8.19947472300005,11.6,7.63449107099999));
#242969=CARTESIAN_POINT('Ctrl Pts',(-8.19806913600006,15.2,7.63138956199998));
#242970=CARTESIAN_POINT('Ctrl Pts',(-8.19806913600006,11.6,7.63138956199998));
#242971=CARTESIAN_POINT('Ctrl Pts',(-8.19666311600006,15.2,7.62829359599999));
#242972=CARTESIAN_POINT('Ctrl Pts',(-8.19666311600006,11.6,7.62829359599999));
#242973=CARTESIAN_POINT('Ctrl Pts',(-8.19525667200006,15.2,7.62520317899998));
#242974=CARTESIAN_POINT('Ctrl Pts',(-8.19525667200006,11.6,7.62520317899998));
#242975=CARTESIAN_POINT('Ctrl Pts',(-8.19384981300006,15.2,7.62211831499998));
#242976=CARTESIAN_POINT('Ctrl Pts',(-8.19384981300006,11.6,7.62211831499998));
#242977=CARTESIAN_POINT('Ctrl Pts',(-8.19244254900006,15.2,7.61903900799999));
#242978=CARTESIAN_POINT('Ctrl Pts',(-8.19244254900006,11.6,7.61903900799999));
#242979=CARTESIAN_POINT('Ctrl Pts',(-8.19103488900006,15.2,7.61596526399998));
#242980=CARTESIAN_POINT('Ctrl Pts',(-8.19103488900006,11.6,7.61596526399998));
#242981=CARTESIAN_POINT('Ctrl Pts',(-8.18962684300006,15.2,7.61289708599998));
#242982=CARTESIAN_POINT('Ctrl Pts',(-8.18962684300006,11.6,7.61289708599998));
#242983=CARTESIAN_POINT('Ctrl Pts',(-8.18821841900006,15.2,7.60983448099999));
#242984=CARTESIAN_POINT('Ctrl Pts',(-8.18821841900006,11.6,7.60983448099999));
#242985=CARTESIAN_POINT('Ctrl Pts',(-8.18680962700006,15.2,7.60677745299999));
#242986=CARTESIAN_POINT('Ctrl Pts',(-8.18680962700006,11.6,7.60677745299999));
#242987=CARTESIAN_POINT('Ctrl Pts',(-8.18540047700006,15.2,7.60372600499998));
#242988=CARTESIAN_POINT('Ctrl Pts',(-8.18540047700006,11.6,7.60372600499998));
#242989=CARTESIAN_POINT('Ctrl Pts',(-8.18399097600006,15.2,7.60068014299998));
#242990=CARTESIAN_POINT('Ctrl Pts',(-8.18399097600006,11.6,7.60068014299998));
#242991=CARTESIAN_POINT('Ctrl Pts',(-8.18258113700006,15.2,7.59763987299999));
#242992=CARTESIAN_POINT('Ctrl Pts',(-8.18258113700006,11.6,7.59763987299999));
#242993=CARTESIAN_POINT('Ctrl Pts',(-8.18117096700006,15.2,7.59460519799998));
#242994=CARTESIAN_POINT('Ctrl Pts',(-8.18117096700006,11.6,7.59460519799998));
#242995=CARTESIAN_POINT('Ctrl Pts',(-8.17976047700006,15.2,7.59157612299998));
#242996=CARTESIAN_POINT('Ctrl Pts',(-8.17976047700006,11.6,7.59157612299998));
#242997=CARTESIAN_POINT('Ctrl Pts',(-8.17834967600006,15.2,7.58855265399998));
#242998=CARTESIAN_POINT('Ctrl Pts',(-8.17834967600006,11.6,7.58855265399998));
#242999=CARTESIAN_POINT('Ctrl Pts',(-8.17693857200006,15.2,7.58553479399998));
#243000=CARTESIAN_POINT('Ctrl Pts',(-8.17693857200006,11.6,7.58553479399998));
#243001=CARTESIAN_POINT('Ctrl Pts',(-8.17552717500006,15.2,7.58252254799999));
#243002=CARTESIAN_POINT('Ctrl Pts',(-8.17552717500006,11.6,7.58252254799999));
#243003=CARTESIAN_POINT('Ctrl Pts',(-8.17411549700006,15.2,7.57951592199999));
#243004=CARTESIAN_POINT('Ctrl Pts',(-8.17411549700006,11.6,7.57951592199999));
#243005=CARTESIAN_POINT('Ctrl Pts',(-8.17270354500006,15.2,7.57651491999999));
#243006=CARTESIAN_POINT('Ctrl Pts',(-8.17270354500006,11.6,7.57651491999999));
#243007=CARTESIAN_POINT('Ctrl Pts',(-8.17129133000006,15.2,7.57351954699998));
#243008=CARTESIAN_POINT('Ctrl Pts',(-8.17129133000006,11.6,7.57351954699998));
#243009=CARTESIAN_POINT('Ctrl Pts',(-8.16987886100006,15.2,7.57052980599998));
#243010=CARTESIAN_POINT('Ctrl Pts',(-8.16987886100006,11.6,7.57052980599998));
#243011=CARTESIAN_POINT('Ctrl Pts',(-8.16846614700006,15.2,7.56754570599998));
#243012=CARTESIAN_POINT('Ctrl Pts',(-8.16846614700006,11.6,7.56754570599998));
#243013=CARTESIAN_POINT('Ctrl Pts',(-8.16705320000005,15.2,7.56456724699999));
#243014=CARTESIAN_POINT('Ctrl Pts',(-8.16705320000005,11.6,7.56456724699999));
#243015=CARTESIAN_POINT('Ctrl Pts',(-8.16564002800006,15.2,7.56159443599999));
#243016=CARTESIAN_POINT('Ctrl Pts',(-8.16564002800006,11.6,7.56159443599999));
#243017=CARTESIAN_POINT('Ctrl Pts',(-8.16422664000006,15.2,7.55862727799999));
#243018=CARTESIAN_POINT('Ctrl Pts',(-8.16422664000006,11.6,7.55862727799999));
#243019=CARTESIAN_POINT('Ctrl Pts',(-8.16281304700006,15.2,7.55566577799998));
#243020=CARTESIAN_POINT('Ctrl Pts',(-8.16281304700006,11.6,7.55566577799998));
#243021=CARTESIAN_POINT('Ctrl Pts',(-8.16139925900006,15.2,7.55270993999999));
#243022=CARTESIAN_POINT('Ctrl Pts',(-8.16139925900006,11.6,7.55270993999999));
#243023=CARTESIAN_POINT('Ctrl Pts',(-8.15998528500005,15.2,7.54975976799999));
#243024=CARTESIAN_POINT('Ctrl Pts',(-8.15998528500005,11.6,7.54975976799999));
#243025=CARTESIAN_POINT('Ctrl Pts',(-8.15857113400006,15.2,7.54681526899999));
#243026=CARTESIAN_POINT('Ctrl Pts',(-8.15857113400006,11.6,7.54681526899999));
#243027=CARTESIAN_POINT('Ctrl Pts',(-8.15715681900006,15.2,7.54387644599999));
#243028=CARTESIAN_POINT('Ctrl Pts',(-8.15715681900006,11.6,7.54387644599999));
#243029=CARTESIAN_POINT('Ctrl Pts',(-8.15574234600006,15.2,7.54094330399998));
#243030=CARTESIAN_POINT('Ctrl Pts',(-8.15574234600006,11.6,7.54094330399998));
#243031=CARTESIAN_POINT('Ctrl Pts',(-8.15432772800006,15.2,7.53801584699998));
#243032=CARTESIAN_POINT('Ctrl Pts',(-8.15432772800006,11.6,7.53801584699998));
#243033=CARTESIAN_POINT('Ctrl Pts',(-8.15291297300006,15.2,7.53509408299998));
#243034=CARTESIAN_POINT('Ctrl Pts',(-8.15291297300006,11.6,7.53509408299998));
#243035=CARTESIAN_POINT('Ctrl Pts',(-8.15149809100006,15.2,7.53217801399998));
#243036=CARTESIAN_POINT('Ctrl Pts',(-8.15149809100006,11.6,7.53217801399998));
#243037=CARTESIAN_POINT('Ctrl Pts',(-8.15008309400006,15.2,7.52926764499998));
#243038=CARTESIAN_POINT('Ctrl Pts',(-8.15008309400006,11.6,7.52926764499998));
#243039=CARTESIAN_POINT('Ctrl Pts',(-8.14866799000006,15.2,7.52636298099999));
#243040=CARTESIAN_POINT('Ctrl Pts',(-8.14866799000006,11.6,7.52636298099999));
#243041=CARTESIAN_POINT('Ctrl Pts',(-8.14725278900006,15.2,7.52346402699998));
#243042=CARTESIAN_POINT('Ctrl Pts',(-8.14725278900006,11.6,7.52346402699998));
#243043=CARTESIAN_POINT('Ctrl Pts',(-8.14583750200006,15.2,7.52057078799999));
#243044=CARTESIAN_POINT('Ctrl Pts',(-8.14583750200006,11.6,7.52057078799999));
#243045=CARTESIAN_POINT('Ctrl Pts',(-8.14442213800006,15.2,7.51768326799999));
#243046=CARTESIAN_POINT('Ctrl Pts',(-8.14442213800006,11.6,7.51768326799999));
#243047=CARTESIAN_POINT('Ctrl Pts',(-8.14300670900005,15.2,7.51480147299999));
#243048=CARTESIAN_POINT('Ctrl Pts',(-8.14300670900005,11.6,7.51480147299999));
#243049=CARTESIAN_POINT('Ctrl Pts',(-8.14159122400006,15.2,7.51192540699999));
#243050=CARTESIAN_POINT('Ctrl Pts',(-8.14159122400006,11.6,7.51192540699999));
#243051=CARTESIAN_POINT('Ctrl Pts',(-8.14017569100006,15.2,7.50905507499999));
#243052=CARTESIAN_POINT('Ctrl Pts',(-8.14017569100006,11.6,7.50905507499999));
#243053=CARTESIAN_POINT('Ctrl Pts',(-8.13876012400006,15.2,7.50619048199999));
#243054=CARTESIAN_POINT('Ctrl Pts',(-8.13876012400006,11.6,7.50619048199999));
#243055=CARTESIAN_POINT('Ctrl Pts',(-8.13734453100006,15.2,7.50333163199999));
#243056=CARTESIAN_POINT('Ctrl Pts',(-8.13734453100006,11.6,7.50333163199999));
#243057=CARTESIAN_POINT('Ctrl Pts',(-8.13592892200005,15.2,7.50047853099999));
#243058=CARTESIAN_POINT('Ctrl Pts',(-8.13592892200005,11.6,7.50047853099999));
#243059=CARTESIAN_POINT('Ctrl Pts',(-8.13451330900006,15.2,7.49763118299998));
#243060=CARTESIAN_POINT('Ctrl Pts',(-8.13451330900006,11.6,7.49763118299998));
#243061=CARTESIAN_POINT('Ctrl Pts',(-8.13309770000006,15.2,7.49478959299999));
#243062=CARTESIAN_POINT('Ctrl Pts',(-8.13309770000006,11.6,7.49478959299999));
#243063=CARTESIAN_POINT('Ctrl Pts',(-8.13168210600006,15.2,7.49195376499999));
#243064=CARTESIAN_POINT('Ctrl Pts',(-8.13168210600006,11.6,7.49195376499999));
#243065=CARTESIAN_POINT('Ctrl Pts',(-8.13026653800006,15.2,7.48912370499998));
#243066=CARTESIAN_POINT('Ctrl Pts',(-8.13026653800006,11.6,7.48912370499998));
#243067=CARTESIAN_POINT('Ctrl Pts',(-8.12885100600005,15.2,7.48629941799998));
#243068=CARTESIAN_POINT('Ctrl Pts',(-8.12885100600005,11.6,7.48629941799998));
#243069=CARTESIAN_POINT('Ctrl Pts',(-8.12743552100006,15.2,7.48348090799999));
#243070=CARTESIAN_POINT('Ctrl Pts',(-8.12743552100006,11.6,7.48348090799999));
#243071=CARTESIAN_POINT('Ctrl Pts',(-8.12602009300005,15.2,7.48066817999998));
#243072=CARTESIAN_POINT('Ctrl Pts',(-8.12602009300005,11.6,7.48066817999998));
#243073=CARTESIAN_POINT('Ctrl Pts',(-8.12460473100005,15.2,7.47786123899999));
#243074=CARTESIAN_POINT('Ctrl Pts',(-8.12460473100005,11.6,7.47786123899999));
#243075=CARTESIAN_POINT('Ctrl Pts',(-8.12318944800005,15.2,7.47506008999999));
#243076=CARTESIAN_POINT('Ctrl Pts',(-8.12318944800005,11.6,7.47506008999999));
#243077=CARTESIAN_POINT('Ctrl Pts',(-8.12177425200005,15.2,7.47226473699998));
#243078=CARTESIAN_POINT('Ctrl Pts',(-8.12177425200005,11.6,7.47226473699998));
#243079=CARTESIAN_POINT('Ctrl Pts',(-8.12035915500006,15.2,7.46947518499999));
#243080=CARTESIAN_POINT('Ctrl Pts',(-8.12035915500006,11.6,7.46947518499999));
#243081=CARTESIAN_POINT('Ctrl Pts',(-8.11894416700006,15.2,7.46669143999998));
#243082=CARTESIAN_POINT('Ctrl Pts',(-8.11894416700006,11.6,7.46669143999998));
#243083=CARTESIAN_POINT('Ctrl Pts',(-8.11752930000005,15.2,7.46391350499999));
#243084=CARTESIAN_POINT('Ctrl Pts',(-8.11752930000005,11.6,7.46391350499999));
#243085=CARTESIAN_POINT('Ctrl Pts',(-8.11611456200006,15.2,7.46114138799998));
#243086=CARTESIAN_POINT('Ctrl Pts',(-8.11611456200006,11.6,7.46114138799998));
#243087=CARTESIAN_POINT('Ctrl Pts',(-8.11469996500006,15.2,7.45837508899999));
#243088=CARTESIAN_POINT('Ctrl Pts',(-8.11469996500006,11.6,7.45837508899999));
#243089=CARTESIAN_POINT('Ctrl Pts',(-8.11328552000005,15.2,7.45561461699998));
#243090=CARTESIAN_POINT('Ctrl Pts',(-8.11328552000005,11.6,7.45561461699998));
#243091=CARTESIAN_POINT('Ctrl Pts',(-8.11187123600006,15.2,7.45285997599999));
#243092=CARTESIAN_POINT('Ctrl Pts',(-8.11187123600006,11.6,7.45285997599999));
#243093=CARTESIAN_POINT('Ctrl Pts',(-8.11045712500006,15.2,7.45011116899998));
#243094=CARTESIAN_POINT('Ctrl Pts',(-8.11045712500006,11.6,7.45011116899998));
#243095=CARTESIAN_POINT('Ctrl Pts',(-8.10904319900006,15.2,7.44736820399999));
#243096=CARTESIAN_POINT('Ctrl Pts',(-8.10904319900006,11.6,7.44736820399999));
#243097=CARTESIAN_POINT('Ctrl Pts',(-8.10762946700006,15.2,7.44463108199999));
#243098=CARTESIAN_POINT('Ctrl Pts',(-8.10762946700006,11.6,7.44463108199999));
#243099=CARTESIAN_POINT('Ctrl Pts',(-8.10621593800006,15.2,7.44189980999998));
#243100=CARTESIAN_POINT('Ctrl Pts',(-8.10621593800006,11.6,7.44189980999998));
#243101=CARTESIAN_POINT('Ctrl Pts',(-8.10480262700005,15.2,7.43917439399999));
#243102=CARTESIAN_POINT('Ctrl Pts',(-8.10480262700005,11.6,7.43917439399999));
#243103=CARTESIAN_POINT('Ctrl Pts',(-8.10338954200006,15.2,7.43645483599998));
#243104=CARTESIAN_POINT('Ctrl Pts',(-8.10338954200006,11.6,7.43645483599998));
#243105=CARTESIAN_POINT('Ctrl Pts',(-8.10197669400005,15.2,7.43374114299999));
#243106=CARTESIAN_POINT('Ctrl Pts',(-8.10197669400005,11.6,7.43374114299999));
#243107=CARTESIAN_POINT('Ctrl Pts',(-8.10056409600006,15.2,7.43103331899999));
#243108=CARTESIAN_POINT('Ctrl Pts',(-8.10056409600006,11.6,7.43103331899999));
#243109=CARTESIAN_POINT('Ctrl Pts',(-8.09915175600005,15.2,7.42833136899999));
#243110=CARTESIAN_POINT('Ctrl Pts',(-8.09915175600005,11.6,7.42833136899999));
#243111=CARTESIAN_POINT('Ctrl Pts',(-8.09773968600006,15.2,7.42563529799998));
#243112=CARTESIAN_POINT('Ctrl Pts',(-8.09773968600006,11.6,7.42563529799998));
#243113=CARTESIAN_POINT('Ctrl Pts',(-8.09632789800006,15.2,7.42294511099999));
#243114=CARTESIAN_POINT('Ctrl Pts',(-8.09632789800006,11.6,7.42294511099999));
#243115=CARTESIAN_POINT('Ctrl Pts',(-8.09491640200006,15.2,7.42026081299999));
#243116=CARTESIAN_POINT('Ctrl Pts',(-8.09491640200006,11.6,7.42026081299999));
#243117=CARTESIAN_POINT('Ctrl Pts',(-8.09350520800006,15.2,7.41758240799999));
#243118=CARTESIAN_POINT('Ctrl Pts',(-8.09350520800006,11.6,7.41758240799999));
#243119=CARTESIAN_POINT('Ctrl Pts',(-8.09209433000006,15.2,7.41490990199999));
#243120=CARTESIAN_POINT('Ctrl Pts',(-8.09209433000006,11.6,7.41490990199999));
#243121=CARTESIAN_POINT('Ctrl Pts',(-8.09068377600006,15.2,7.41224329899998));
#243122=CARTESIAN_POINT('Ctrl Pts',(-8.09068377600006,11.6,7.41224329899998));
#243123=CARTESIAN_POINT('Ctrl Pts',(-8.08927355900006,15.2,7.40958260399999));
#243124=CARTESIAN_POINT('Ctrl Pts',(-8.08927355900006,11.6,7.40958260399999));
#243125=CARTESIAN_POINT('Ctrl Pts',(-8.08786369000006,15.2,7.40692782299998));
#243126=CARTESIAN_POINT('Ctrl Pts',(-8.08786369000006,11.6,7.40692782299998));
#243127=CARTESIAN_POINT('Ctrl Pts',(-8.08645417900006,15.2,7.40427895899998));
#243128=CARTESIAN_POINT('Ctrl Pts',(-8.08645417900006,11.6,7.40427895899998));
#243129=CARTESIAN_POINT('Ctrl Pts',(-8.08504503800006,15.2,7.40163601799999));
#243130=CARTESIAN_POINT('Ctrl Pts',(-8.08504503800006,11.6,7.40163601799999));
#243131=CARTESIAN_POINT('Ctrl Pts',(-8.08363627800006,15.2,7.39899900499999));
#243132=CARTESIAN_POINT('Ctrl Pts',(-8.08363627800006,11.6,7.39899900499999));
#243133=CARTESIAN_POINT('Ctrl Pts',(-8.08222791000006,15.2,7.39636792399998));
#243134=CARTESIAN_POINT('Ctrl Pts',(-8.08222791000006,11.6,7.39636792399998));
#243135=CARTESIAN_POINT('Ctrl Pts',(-8.08081994700006,15.2,7.39374278199998));
#243136=CARTESIAN_POINT('Ctrl Pts',(-8.08081994700006,11.6,7.39374278199998));
#243137=CARTESIAN_POINT('Ctrl Pts',(-8.07941239800006,15.2,7.39112358099998));
#243138=CARTESIAN_POINT('Ctrl Pts',(-8.07941239800006,11.6,7.39112358099998));
#243139=CARTESIAN_POINT('Ctrl Pts',(-8.07800527500006,15.2,7.38851032799998));
#243140=CARTESIAN_POINT('Ctrl Pts',(-8.07800527500006,11.6,7.38851032799998));
#243141=CARTESIAN_POINT('Ctrl Pts',(-8.07659859000006,15.2,7.38590302699999));
#243142=CARTESIAN_POINT('Ctrl Pts',(-8.07659859000006,11.6,7.38590302699999));
#243143=CARTESIAN_POINT('Ctrl Pts',(-8.07519235300006,15.2,7.38330168299999));
#243144=CARTESIAN_POINT('Ctrl Pts',(-8.07519235300006,11.6,7.38330168299999));
#243145=CARTESIAN_POINT('Ctrl Pts',(-8.07378657800006,15.2,7.38070630199999));
#243146=CARTESIAN_POINT('Ctrl Pts',(-8.07378657800006,11.6,7.38070630199999));
#243147=CARTESIAN_POINT('Ctrl Pts',(-8.07238127500005,15.2,7.37811688599999));
#243148=CARTESIAN_POINT('Ctrl Pts',(-8.07238127500005,11.6,7.37811688599999));
#243149=CARTESIAN_POINT('Ctrl Pts',(-8.07097645400006,15.2,7.37553344299998));
#243150=CARTESIAN_POINT('Ctrl Pts',(-8.07097645400006,11.6,7.37553344299998));
#243151=CARTESIAN_POINT('Ctrl Pts',(-8.06957212900006,15.2,7.37295597699998));
#243152=CARTESIAN_POINT('Ctrl Pts',(-8.06957212900006,11.6,7.37295597699998));
#243153=CARTESIAN_POINT('Ctrl Pts',(-8.06816830900006,15.2,7.37038449199999));
#243154=CARTESIAN_POINT('Ctrl Pts',(-8.06816830900006,11.6,7.37038449199999));
#243155=CARTESIAN_POINT('Ctrl Pts',(-8.06676500800006,15.2,7.36781899399999));
#243156=CARTESIAN_POINT('Ctrl Pts',(-8.06676500800006,11.6,7.36781899399999));
#243157=CARTESIAN_POINT('Ctrl Pts',(-8.06536223700006,15.2,7.36525948799999));
#243158=CARTESIAN_POINT('Ctrl Pts',(-8.06536223700006,11.6,7.36525948799999));
#243159=CARTESIAN_POINT('Ctrl Pts',(-8.06396000700006,15.2,7.36270597899999));
#243160=CARTESIAN_POINT('Ctrl Pts',(-8.06396000700006,11.6,7.36270597899999));
#243161=CARTESIAN_POINT('Ctrl Pts',(-8.06255832900005,15.2,7.36015846999998));
#243162=CARTESIAN_POINT('Ctrl Pts',(-8.06255832900005,11.6,7.36015846999998));
#243163=CARTESIAN_POINT('Ctrl Pts',(-8.06115721700005,15.2,7.35761696699999));
#243164=CARTESIAN_POINT('Ctrl Pts',(-8.06115721700005,11.6,7.35761696699999));
#243165=CARTESIAN_POINT('Ctrl Pts',(-8.05975668100006,15.2,7.35508147699999));
#243166=CARTESIAN_POINT('Ctrl Pts',(-8.05975668100006,11.6,7.35508147699999));
#243167=CARTESIAN_POINT('Ctrl Pts',(-8.05835673200006,15.2,7.35255200199998));
#243168=CARTESIAN_POINT('Ctrl Pts',(-8.05835673200006,11.6,7.35255200199998));
#243169=CARTESIAN_POINT('Ctrl Pts',(-8.05695738400006,15.2,7.35002854799998));
#243170=CARTESIAN_POINT('Ctrl Pts',(-8.05695738400006,11.6,7.35002854799998));
#243171=CARTESIAN_POINT('Ctrl Pts',(-8.05555864800005,15.2,7.34751112099998));
#243172=CARTESIAN_POINT('Ctrl Pts',(-8.05555864800005,11.6,7.34751112099998));
#243173=CARTESIAN_POINT('Ctrl Pts',(-8.05416053400006,15.2,7.34499972499999));
#243174=CARTESIAN_POINT('Ctrl Pts',(-8.05416053400006,11.6,7.34499972499999));
#243175=CARTESIAN_POINT('Ctrl Pts',(-8.05276305700006,15.2,7.34249436299999));
#243176=CARTESIAN_POINT('Ctrl Pts',(-8.05276305700006,11.6,7.34249436299999));
#243177=CARTESIAN_POINT('Ctrl Pts',(-8.05136622600006,15.2,7.33999504399999));
#243178=CARTESIAN_POINT('Ctrl Pts',(-8.05136622600006,11.6,7.33999504399999));
#243179=CARTESIAN_POINT('Ctrl Pts',(-8.04997005600006,15.2,7.33750177099999));
#243180=CARTESIAN_POINT('Ctrl Pts',(-8.04997005600006,11.6,7.33750177099999));
#243181=CARTESIAN_POINT('Ctrl Pts',(-8.04857455600006,15.2,7.33501454799999));
#243182=CARTESIAN_POINT('Ctrl Pts',(-8.04857455600006,11.6,7.33501454799999));
#243183=CARTESIAN_POINT('Ctrl Pts',(-8.04717974000006,15.2,7.33253338099999));
#243184=CARTESIAN_POINT('Ctrl Pts',(-8.04717974000006,11.6,7.33253338099999));
#243185=CARTESIAN_POINT('Ctrl Pts',(-8.04578561900006,15.2,7.33005827499999));
#243186=CARTESIAN_POINT('Ctrl Pts',(-8.04578561900006,11.6,7.33005827499999));
#243187=CARTESIAN_POINT('Ctrl Pts',(-8.04439220600005,15.2,7.32758923399999));
#243188=CARTESIAN_POINT('Ctrl Pts',(-8.04439220600005,11.6,7.32758923399999));
#243189=CARTESIAN_POINT('Ctrl Pts',(-8.04299951200005,15.2,7.32512626399998));
#243190=CARTESIAN_POINT('Ctrl Pts',(-8.04299951200005,11.6,7.32512626399998));
#243191=CARTESIAN_POINT('Ctrl Pts',(-8.04160755100006,15.2,7.32266936999999));
#243192=CARTESIAN_POINT('Ctrl Pts',(-8.04160755100006,11.6,7.32266936999999));
#243193=CARTESIAN_POINT('Ctrl Pts',(-8.04021633200006,15.2,7.32021855699998));
#243194=CARTESIAN_POINT('Ctrl Pts',(-8.04021633200006,11.6,7.32021855699998));
#243195=CARTESIAN_POINT('Ctrl Pts',(-8.03882587100006,15.2,7.31777382799999));
#243196=CARTESIAN_POINT('Ctrl Pts',(-8.03882587100006,11.6,7.31777382799999));
#243197=CARTESIAN_POINT('Ctrl Pts',(-8.03743617700006,15.2,7.31533519099998));
#243198=CARTESIAN_POINT('Ctrl Pts',(-8.03743617700006,11.6,7.31533519099998));
#243199=CARTESIAN_POINT('Ctrl Pts',(-8.03604726400006,15.2,7.31290264899998));
#243200=CARTESIAN_POINT('Ctrl Pts',(-8.03604726400006,11.6,7.31290264899998));
#243201=CARTESIAN_POINT('Ctrl Pts',(-8.03465914400006,15.2,7.31047620699999));
#243202=CARTESIAN_POINT('Ctrl Pts',(-8.03465914400006,11.6,7.31047620699999));
#243203=CARTESIAN_POINT('Ctrl Pts',(-8.03327182900006,15.2,7.30805587199999));
#243204=CARTESIAN_POINT('Ctrl Pts',(-8.03327182900006,11.6,7.30805587199999));
#243205=CARTESIAN_POINT('Ctrl Pts',(-8.03188533300006,15.2,7.30564164699998));
#243206=CARTESIAN_POINT('Ctrl Pts',(-8.03188533300006,11.6,7.30564164699998));
#243207=CARTESIAN_POINT('Ctrl Pts',(-8.03049966600006,15.2,7.30323353699998));
#243208=CARTESIAN_POINT('Ctrl Pts',(-8.03049966600006,11.6,7.30323353699998));
#243209=CARTESIAN_POINT('Ctrl Pts',(-8.02911484200006,15.2,7.30083154799999));
#243210=CARTESIAN_POINT('Ctrl Pts',(-8.02911484200006,11.6,7.30083154799999));
#243211=CARTESIAN_POINT('Ctrl Pts',(-8.02773087300006,15.2,7.29843568399998));
#243212=CARTESIAN_POINT('Ctrl Pts',(-8.02773087300006,11.6,7.29843568399998));
#243213=CARTESIAN_POINT('Ctrl Pts',(-8.02634777100005,15.2,7.29604595099998));
#243214=CARTESIAN_POINT('Ctrl Pts',(-8.02634777100005,11.6,7.29604595099998));
#243215=CARTESIAN_POINT('Ctrl Pts',(-8.02496555000005,15.2,7.29366235399999));
#243216=CARTESIAN_POINT('Ctrl Pts',(-8.02496555000005,11.6,7.29366235399999));
#243217=CARTESIAN_POINT('Ctrl Pts',(-8.02358422100006,15.2,7.29128489699999));
#243218=CARTESIAN_POINT('Ctrl Pts',(-8.02358422100006,11.6,7.29128489699999));
#243219=CARTESIAN_POINT('Ctrl Pts',(-8.02220379800006,15.2,7.28891358499999));
#243220=CARTESIAN_POINT('Ctrl Pts',(-8.02220379800006,11.6,7.28891358499999));
#243221=CARTESIAN_POINT('Ctrl Pts',(-8.02082429300006,15.2,7.28654842499999));
#243222=CARTESIAN_POINT('Ctrl Pts',(-8.02082429300006,11.6,7.28654842499999));
#243223=CARTESIAN_POINT('Ctrl Pts',(-8.01944571900006,15.2,7.28418941999998));
#243224=CARTESIAN_POINT('Ctrl Pts',(-8.01944571900006,11.6,7.28418941999998));
#243225=CARTESIAN_POINT('Ctrl Pts',(-8.01806808700006,15.2,7.28183657599998));
#243226=CARTESIAN_POINT('Ctrl Pts',(-8.01806808700006,11.6,7.28183657599998));
#243227=CARTESIAN_POINT('Ctrl Pts',(-8.01669141300006,15.2,7.27948989599999));
#243228=CARTESIAN_POINT('Ctrl Pts',(-8.01669141300006,11.6,7.27948989599999));
#243229=CARTESIAN_POINT('Ctrl Pts',(-8.01531570700006,15.2,7.27714938799998));
#243230=CARTESIAN_POINT('Ctrl Pts',(-8.01531570700006,11.6,7.27714938799998));
#243231=CARTESIAN_POINT('Ctrl Pts',(-8.01394098300005,15.2,7.27481505599999));
#243232=CARTESIAN_POINT('Ctrl Pts',(-8.01394098300005,11.6,7.27481505599999));
#243233=CARTESIAN_POINT('Ctrl Pts',(-8.01256725300006,15.2,7.27248690499999));
#243234=CARTESIAN_POINT('Ctrl Pts',(-8.01256725300006,11.6,7.27248690499999));
#243235=CARTESIAN_POINT('Ctrl Pts',(-8.01119453200006,15.2,7.27016493799999));
#243236=CARTESIAN_POINT('Ctrl Pts',(-8.01119453200006,11.6,7.27016493799999));
#243237=CARTESIAN_POINT('Ctrl Pts',(-8.00982283100005,15.2,7.26784916399998));
#243238=CARTESIAN_POINT('Ctrl Pts',(-8.00982283100005,11.6,7.26784916399998));
#243239=CARTESIAN_POINT('Ctrl Pts',(-8.00845216400005,15.2,7.26553958499998));
#243240=CARTESIAN_POINT('Ctrl Pts',(-8.00845216400005,11.6,7.26553958499998));
#243241=CARTESIAN_POINT('Ctrl Pts',(-8.00708254300006,15.2,7.26323620699999));
#243242=CARTESIAN_POINT('Ctrl Pts',(-8.00708254300006,11.6,7.26323620699999));
#243243=CARTESIAN_POINT('Ctrl Pts',(-8.00571398200006,15.2,7.26093903499999));
#243244=CARTESIAN_POINT('Ctrl Pts',(-8.00571398200006,11.6,7.26093903499999));
#243245=CARTESIAN_POINT('Ctrl Pts',(-8.00434649400006,15.2,7.25864807299998));
#243246=CARTESIAN_POINT('Ctrl Pts',(-8.00434649400006,11.6,7.25864807299998));
#243247=CARTESIAN_POINT('Ctrl Pts',(-8.00298009200005,15.2,7.25636332799999));
#243248=CARTESIAN_POINT('Ctrl Pts',(-8.00298009200005,11.6,7.25636332799999));
#243249=CARTESIAN_POINT('Ctrl Pts',(-8.00161478800005,15.2,7.25408480499999));
#243250=CARTESIAN_POINT('Ctrl Pts',(-8.00161478800005,11.6,7.25408480499999));
#243251=CARTESIAN_POINT('Ctrl Pts',(-8.00025059700006,15.2,7.25181250799999));
#243252=CARTESIAN_POINT('Ctrl Pts',(-8.00025059700006,11.6,7.25181250799999));
#243253=CARTESIAN_POINT('Ctrl Pts',(-7.99888753100006,15.2,7.24954644099999));
#243254=CARTESIAN_POINT('Ctrl Pts',(-7.99888753100006,11.6,7.24954644099999));
#243255=CARTESIAN_POINT('Ctrl Pts',(-7.99752560500006,15.2,7.24728661199999));
#243256=CARTESIAN_POINT('Ctrl Pts',(-7.99752560500006,11.6,7.24728661199999));
#243257=CARTESIAN_POINT('Ctrl Pts',(-7.99616483100006,15.2,7.24503302299999));
#243258=CARTESIAN_POINT('Ctrl Pts',(-7.99616483100006,11.6,7.24503302299999));
#243259=CARTESIAN_POINT('Ctrl Pts',(-7.99480522200006,15.2,7.24278568099999));
#243260=CARTESIAN_POINT('Ctrl Pts',(-7.99480522200006,11.6,7.24278568099999));
#243261=CARTESIAN_POINT('Ctrl Pts',(-7.99344679200006,15.2,7.24054459099998));
#243262=CARTESIAN_POINT('Ctrl Pts',(-7.99344679200006,11.6,7.24054459099998));
#243263=CARTESIAN_POINT('Ctrl Pts',(-7.99208955400006,15.2,7.23830975799999));
#243264=CARTESIAN_POINT('Ctrl Pts',(-7.99208955400006,11.6,7.23830975799999));
#243265=CARTESIAN_POINT('Ctrl Pts',(-7.99073352200006,15.2,7.23608118599999));
#243266=CARTESIAN_POINT('Ctrl Pts',(-7.99073352200006,11.6,7.23608118599999));
#243267=CARTESIAN_POINT('Ctrl Pts',(-7.98937871000006,15.2,7.23385888199999));
#243268=CARTESIAN_POINT('Ctrl Pts',(-7.98937871000006,11.6,7.23385888199999));
#243269=CARTESIAN_POINT('Ctrl Pts',(-7.98802513000006,15.2,7.23164284899998));
#243270=CARTESIAN_POINT('Ctrl Pts',(-7.98802513000006,11.6,7.23164284899998));
#243271=CARTESIAN_POINT('Ctrl Pts',(-7.98667279800006,15.2,7.22943309299998));
#243272=CARTESIAN_POINT('Ctrl Pts',(-7.98667279800006,11.6,7.22943309299998));
#243273=CARTESIAN_POINT('Ctrl Pts',(-7.98532172500006,15.2,7.22722962099999));
#243274=CARTESIAN_POINT('Ctrl Pts',(-7.98532172500006,11.6,7.22722962099999));
#243275=CARTESIAN_POINT('Ctrl Pts',(-7.98397192700006,15.2,7.22503243499999));
#243276=CARTESIAN_POINT('Ctrl Pts',(-7.98397192700006,11.6,7.22503243499999));
#243277=CARTESIAN_POINT('Ctrl Pts',(-7.98262341500006,15.2,7.22284154199999));
#243278=CARTESIAN_POINT('Ctrl Pts',(-7.98262341500006,11.6,7.22284154199999));
#243279=CARTESIAN_POINT('Ctrl Pts',(-7.98127620500006,15.2,7.22065694499998));
#243280=CARTESIAN_POINT('Ctrl Pts',(-7.98127620500006,11.6,7.22065694499998));
#243281=CARTESIAN_POINT('Ctrl Pts',(-7.97993031100006,15.2,7.21847865199998));
#243282=CARTESIAN_POINT('Ctrl Pts',(-7.97993031100006,11.6,7.21847865199998));
#243283=CARTESIAN_POINT('Ctrl Pts',(-7.97858574500006,15.2,7.21630666699999));
#243284=CARTESIAN_POINT('Ctrl Pts',(-7.97858574500006,11.6,7.21630666699999));
#243285=CARTESIAN_POINT('Ctrl Pts',(-7.97724252100006,15.2,7.21414099499999));
#243286=CARTESIAN_POINT('Ctrl Pts',(-7.97724252100006,11.6,7.21414099499999));
#243287=CARTESIAN_POINT('Ctrl Pts',(-7.97590065500006,15.2,7.21198164099999));
#243288=CARTESIAN_POINT('Ctrl Pts',(-7.97590065500006,11.6,7.21198164099999));
#243289=CARTESIAN_POINT('Ctrl Pts',(-7.97456015900006,15.2,7.20982860999998));
#243290=CARTESIAN_POINT('Ctrl Pts',(-7.97456015900006,11.6,7.20982860999998));
#243291=CARTESIAN_POINT('Ctrl Pts',(-7.97322104900006,15.2,7.20768190799999));
#243292=CARTESIAN_POINT('Ctrl Pts',(-7.97322104900006,11.6,7.20768190799999));
#243293=CARTESIAN_POINT('Ctrl Pts',(-7.97188333700006,15.2,7.20554153799998));
#243294=CARTESIAN_POINT('Ctrl Pts',(-7.97188333700006,11.6,7.20554153799998));
#243295=CARTESIAN_POINT('Ctrl Pts',(-7.97054703800006,15.2,7.20340750799998));
#243296=CARTESIAN_POINT('Ctrl Pts',(-7.97054703800006,11.6,7.20340750799998));
#243297=CARTESIAN_POINT('Ctrl Pts',(-7.96921216600006,15.2,7.20127982099999));
#243298=CARTESIAN_POINT('Ctrl Pts',(-7.96921216600006,11.6,7.20127982099999));
#243299=CARTESIAN_POINT('Ctrl Pts',(-7.96787873500006,15.2,7.19915848399998));
#243300=CARTESIAN_POINT('Ctrl Pts',(-7.96787873500006,11.6,7.19915848399998));
#243301=CARTESIAN_POINT('Ctrl Pts',(-7.96654675900006,15.2,7.19704350199999));
#243302=CARTESIAN_POINT('Ctrl Pts',(-7.96654675900006,11.6,7.19704350199999));
#243303=CARTESIAN_POINT('Ctrl Pts',(-7.96521625400005,15.2,7.19493487699999));
#243304=CARTESIAN_POINT('Ctrl Pts',(-7.96521625400005,11.6,7.19493487699999));
#243305=CARTESIAN_POINT('Ctrl Pts',(-7.96388723200005,15.2,7.19283261799998));
#243306=CARTESIAN_POINT('Ctrl Pts',(-7.96388723200005,11.6,7.19283261799998));
#243307=CARTESIAN_POINT('Ctrl Pts',(-7.96255970800006,15.2,7.19073672799999));
#243308=CARTESIAN_POINT('Ctrl Pts',(-7.96255970800006,11.6,7.19073672799999));
#243309=CARTESIAN_POINT('Ctrl Pts',(-7.96123369800006,15.2,7.18864721399999));
#243310=CARTESIAN_POINT('Ctrl Pts',(-7.96123369800006,11.6,7.18864721399999));
#243311=CARTESIAN_POINT('Ctrl Pts',(-7.95990921500006,15.2,7.18656407799998));
#243312=CARTESIAN_POINT('Ctrl Pts',(-7.95990921500006,11.6,7.18656407799998));
#243313=CARTESIAN_POINT('Ctrl Pts',(-7.95858627200006,15.2,7.18448732899999));
#243314=CARTESIAN_POINT('Ctrl Pts',(-7.95858627200006,11.6,7.18448732899999));
#243315=CARTESIAN_POINT('Ctrl Pts',(-7.95726488600006,15.2,7.18241696899998));
#243316=CARTESIAN_POINT('Ctrl Pts',(-7.95726488600006,11.6,7.18241696899998));
#243317=CARTESIAN_POINT('Ctrl Pts',(-7.95594507200006,15.2,7.18035300599999));
#243318=CARTESIAN_POINT('Ctrl Pts',(-7.95594507200006,11.6,7.18035300599999));
#243319=CARTESIAN_POINT('Ctrl Pts',(-7.95462684200006,15.2,7.17829544299998));
#243320=CARTESIAN_POINT('Ctrl Pts',(-7.95462684200006,11.6,7.17829544299998));
#243321=CARTESIAN_POINT('Ctrl Pts',(-7.95331021200005,15.2,7.17624428699998));
#243322=CARTESIAN_POINT('Ctrl Pts',(-7.95331021200005,11.6,7.17624428699998));
#243323=CARTESIAN_POINT('Ctrl Pts',(-7.95199519600006,15.2,7.17419954199999));
#243324=CARTESIAN_POINT('Ctrl Pts',(-7.95199519600006,11.6,7.17419954199999));
#243325=CARTESIAN_POINT('Ctrl Pts',(-7.95068181100006,15.2,7.17216121299998));
#243326=CARTESIAN_POINT('Ctrl Pts',(-7.95068181100006,11.6,7.17216121299998));
#243327=CARTESIAN_POINT('Ctrl Pts',(-7.94937007000006,15.2,7.17012930599999));
#243328=CARTESIAN_POINT('Ctrl Pts',(-7.94937007000006,11.6,7.17012930599999));
#243329=CARTESIAN_POINT('Ctrl Pts',(-7.94805998700006,15.2,7.16810382499999));
#243330=CARTESIAN_POINT('Ctrl Pts',(-7.94805998700006,11.6,7.16810382499999));
#243331=CARTESIAN_POINT('Ctrl Pts',(-7.94675157900006,15.2,7.16608477799999));
#243332=CARTESIAN_POINT('Ctrl Pts',(-7.94675157900006,11.6,7.16608477799999));
#243333=CARTESIAN_POINT('Ctrl Pts',(-7.94544485900006,15.2,7.16407216699999));
#243334=CARTESIAN_POINT('Ctrl Pts',(-7.94544485900006,11.6,7.16407216699999));
#243335=CARTESIAN_POINT('Ctrl Pts',(-7.94413984400006,15.2,7.16206599799998));
#243336=CARTESIAN_POINT('Ctrl Pts',(-7.94413984400006,11.6,7.16206599799998));
#243337=CARTESIAN_POINT('Ctrl Pts',(-7.94283654700005,15.2,7.16006627799998));
#243338=CARTESIAN_POINT('Ctrl Pts',(-7.94283654700005,11.6,7.16006627799998));
#243339=CARTESIAN_POINT('Ctrl Pts',(-7.94153498400006,15.2,7.15807301099999));
#243340=CARTESIAN_POINT('Ctrl Pts',(-7.94153498400006,11.6,7.15807301099999));
#243341=CARTESIAN_POINT('Ctrl Pts',(-7.94023517100006,15.2,7.15608620199998));
#243342=CARTESIAN_POINT('Ctrl Pts',(-7.94023517100006,11.6,7.15608620199998));
#243343=CARTESIAN_POINT('Ctrl Pts',(-7.93893712100005,15.2,7.15410585699999));
#243344=CARTESIAN_POINT('Ctrl Pts',(-7.93893712100005,11.6,7.15410585699999));
#243345=CARTESIAN_POINT('Ctrl Pts',(-7.93764085100006,15.2,7.15213197999999));
#243346=CARTESIAN_POINT('Ctrl Pts',(-7.93764085100006,11.6,7.15213197999999));
#243347=CARTESIAN_POINT('Ctrl Pts',(-7.93634637600006,15.2,7.15016457899999));
#243348=CARTESIAN_POINT('Ctrl Pts',(-7.93634637600006,11.6,7.15016457899999));
#243349=CARTESIAN_POINT('Ctrl Pts',(-7.93505371000006,15.2,7.14820365599999));
#243350=CARTESIAN_POINT('Ctrl Pts',(-7.93505371000006,11.6,7.14820365599999));
#243351=CARTESIAN_POINT('Ctrl Pts',(-7.93376287100005,15.2,7.14624921799999));
#243352=CARTESIAN_POINT('Ctrl Pts',(-7.93376287100005,11.6,7.14624921799999));
#243353=CARTESIAN_POINT('Ctrl Pts',(-7.93247387100006,15.2,7.14430126999999));
#243354=CARTESIAN_POINT('Ctrl Pts',(-7.93247387100006,11.6,7.14430126999999));
#243355=CARTESIAN_POINT('Ctrl Pts',(-7.93118672800006,15.2,7.14235981699999));
#243356=CARTESIAN_POINT('Ctrl Pts',(-7.93118672800006,11.6,7.14235981699999));
#243357=CARTESIAN_POINT('Ctrl Pts',(-7.92990145700006,15.2,7.14042486499999));
#243358=CARTESIAN_POINT('Ctrl Pts',(-7.92990145700006,11.6,7.14042486499999));
#243359=CARTESIAN_POINT('Ctrl Pts',(-7.92861807300006,15.2,7.13849641899999));
#243360=CARTESIAN_POINT('Ctrl Pts',(-7.92861807300006,11.6,7.13849641899999));
#243361=CARTESIAN_POINT('Ctrl Pts',(-7.92733659200006,15.2,7.13657448399999));
#243362=CARTESIAN_POINT('Ctrl Pts',(-7.92733659200006,11.6,7.13657448399999));
#243363=CARTESIAN_POINT('Ctrl Pts',(-7.92605703000006,15.2,7.13465906499999));
#243364=CARTESIAN_POINT('Ctrl Pts',(-7.92605703000006,11.6,7.13465906499999));
#243365=CARTESIAN_POINT('Ctrl Pts',(-7.92477940100006,15.2,7.13275016799999));
#243366=CARTESIAN_POINT('Ctrl Pts',(-7.92477940100006,11.6,7.13275016799999));
#243367=CARTESIAN_POINT('Ctrl Pts',(-7.92350372300006,15.2,7.13084779799999));
#243368=CARTESIAN_POINT('Ctrl Pts',(-7.92350372300006,11.6,7.13084779799999));
#243369=CARTESIAN_POINT('Ctrl Pts',(-7.92223001100006,15.2,7.12895196099999));
#243370=CARTESIAN_POINT('Ctrl Pts',(-7.92223001100006,11.6,7.12895196099999));
#243371=CARTESIAN_POINT('Ctrl Pts',(-7.92095828000006,15.2,7.12706266099998));
#243372=CARTESIAN_POINT('Ctrl Pts',(-7.92095828000006,11.6,7.12706266099998));
#243373=CARTESIAN_POINT('Ctrl Pts',(-7.91968854700006,15.2,7.12517990399999));
#243374=CARTESIAN_POINT('Ctrl Pts',(-7.91968854700006,11.6,7.12517990399999));
#243375=CARTESIAN_POINT('Ctrl Pts',(-7.91842082700006,15.2,7.12330369699998));
#243376=CARTESIAN_POINT('Ctrl Pts',(-7.91842082700006,11.6,7.12330369699998));
#243377=CARTESIAN_POINT('Ctrl Pts',(-7.91715513700006,15.2,7.12143404199999));
#243378=CARTESIAN_POINT('Ctrl Pts',(-7.91715513700006,11.6,7.12143404199999));
#243379=CARTESIAN_POINT('Ctrl Pts',(-7.91589149200006,15.2,7.11957094699999));
#243380=CARTESIAN_POINT('Ctrl Pts',(-7.91589149200006,11.6,7.11957094699999));
#243381=CARTESIAN_POINT('Ctrl Pts',(-7.91462990900006,15.2,7.11771441599999));
#243382=CARTESIAN_POINT('Ctrl Pts',(-7.91462990900006,11.6,7.11771441599999));
#243383=CARTESIAN_POINT('Ctrl Pts',(-7.91337040500006,15.2,7.11586445499999));
#243384=CARTESIAN_POINT('Ctrl Pts',(-7.91337040500006,11.6,7.11586445499999));
#243385=CARTESIAN_POINT('Ctrl Pts',(-7.91211299300006,15.2,7.11402106899998));
#243386=CARTESIAN_POINT('Ctrl Pts',(-7.91211299300006,11.6,7.11402106899998));
#243387=CARTESIAN_POINT('Ctrl Pts',(-7.91085769300006,15.2,7.11218426399999));
#243388=CARTESIAN_POINT('Ctrl Pts',(-7.91085769300006,11.6,7.11218426399999));
#243389=CARTESIAN_POINT('Ctrl Pts',(-7.90960451900006,15.2,7.11035404499999));
#243390=CARTESIAN_POINT('Ctrl Pts',(-7.90960451900006,11.6,7.11035404499999));
#243391=CARTESIAN_POINT('Ctrl Pts',(-7.90835348900006,15.2,7.10853041599999));
#243392=CARTESIAN_POINT('Ctrl Pts',(-7.90835348900006,11.6,7.10853041599999));
#243393=CARTESIAN_POINT('Ctrl Pts',(-7.90710461800006,15.2,7.10671338599998));
#243394=CARTESIAN_POINT('Ctrl Pts',(-7.90710461800006,11.6,7.10671338599998));
#243395=CARTESIAN_POINT('Ctrl Pts',(-7.90585792200006,15.2,7.10490295699999));
#243396=CARTESIAN_POINT('Ctrl Pts',(-7.90585792200006,11.6,7.10490295699999));
#243397=CARTESIAN_POINT('Ctrl Pts',(-7.90461341900006,15.2,7.10309913499999));
#243398=CARTESIAN_POINT('Ctrl Pts',(-7.90461341900006,11.6,7.10309913499999));
#243399=CARTESIAN_POINT('Ctrl Pts',(-7.90337112600006,15.2,7.10130192599999));
#243400=CARTESIAN_POINT('Ctrl Pts',(-7.90337112600006,11.6,7.10130192599999));
#243401=CARTESIAN_POINT('Ctrl Pts',(-7.90213105800006,15.2,7.09951133599999));
#243402=CARTESIAN_POINT('Ctrl Pts',(-7.90213105800006,11.6,7.09951133599999));
#243403=CARTESIAN_POINT('Ctrl Pts',(-7.90089323400006,15.2,7.09772736899998));
#243404=CARTESIAN_POINT('Ctrl Pts',(-7.90089323400006,11.6,7.09772736899998));
#243405=CARTESIAN_POINT('Ctrl Pts',(-7.89965766800006,15.2,7.09595003199999));
#243406=CARTESIAN_POINT('Ctrl Pts',(-7.89965766800006,11.6,7.09595003199999));
#243407=CARTESIAN_POINT('Ctrl Pts',(-7.89842437800005,15.2,7.09417932899999));
#243408=CARTESIAN_POINT('Ctrl Pts',(-7.89842437800005,11.6,7.09417932899999));
#243409=CARTESIAN_POINT('Ctrl Pts',(-7.89719338100006,15.2,7.09241526599998));
#243410=CARTESIAN_POINT('Ctrl Pts',(-7.89719338100006,11.6,7.09241526599998));
#243411=CARTESIAN_POINT('Ctrl Pts',(-7.89596469400006,15.2,7.09065784899998));
#243412=CARTESIAN_POINT('Ctrl Pts',(-7.89596469400006,11.6,7.09065784899998));
#243413=CARTESIAN_POINT('Ctrl Pts',(-7.89473833400006,15.2,7.08890708299998));
#243414=CARTESIAN_POINT('Ctrl Pts',(-7.89473833400006,11.6,7.08890708299998));
#243415=CARTESIAN_POINT('Ctrl Pts',(-7.89351431800006,15.2,7.08716297299999));
#243416=CARTESIAN_POINT('Ctrl Pts',(-7.89351431800006,11.6,7.08716297299999));
#243417=CARTESIAN_POINT('Ctrl Pts',(-7.89229266400006,15.2,7.08542552399998));
#243418=CARTESIAN_POINT('Ctrl Pts',(-7.89229266400006,11.6,7.08542552399998));
#243419=CARTESIAN_POINT('Ctrl Pts',(-7.89107338700005,15.2,7.08369474399999));
#243420=CARTESIAN_POINT('Ctrl Pts',(-7.89107338700005,11.6,7.08369474399999));
#243421=CARTESIAN_POINT('Ctrl Pts',(-7.88985650600005,15.2,7.08197063499998));
#243422=CARTESIAN_POINT('Ctrl Pts',(-7.88985650600005,11.6,7.08197063499998));
#243423=CARTESIAN_POINT('Ctrl Pts',(-7.88864203800006,15.2,7.08025320599998));
#243424=CARTESIAN_POINT('Ctrl Pts',(-7.88864203800006,11.6,7.08025320599998));
#243425=CARTESIAN_POINT('Ctrl Pts',(-7.88743000000006,15.2,7.07854245999999));
#243426=CARTESIAN_POINT('Ctrl Pts',(-7.88743000000006,11.6,7.07854245999999));
#243427=CARTESIAN_POINT('Ctrl Pts',(-7.88622040900006,15.2,7.07683840299998));
#243428=CARTESIAN_POINT('Ctrl Pts',(-7.88622040900006,11.6,7.07683840299998));
#243429=CARTESIAN_POINT('Ctrl Pts',(-7.88501328300006,15.2,7.07514104099998));
#243430=CARTESIAN_POINT('Ctrl Pts',(-7.88501328300006,11.6,7.07514104099998));
#243431=CARTESIAN_POINT('Ctrl Pts',(-7.88380864000005,15.2,7.07345037899999));
#243432=CARTESIAN_POINT('Ctrl Pts',(-7.88380864000005,11.6,7.07345037899999));
#243433=CARTESIAN_POINT('Ctrl Pts',(-7.88260649600005,15.2,7.07176642199999));
#243434=CARTESIAN_POINT('Ctrl Pts',(-7.88260649600005,11.6,7.07176642199999));
#243435=CARTESIAN_POINT('Ctrl Pts',(-7.88140687100006,15.2,7.07008917799998));
#243436=CARTESIAN_POINT('Ctrl Pts',(-7.88140687100006,11.6,7.07008917799998));
#243437=CARTESIAN_POINT('Ctrl Pts',(-7.88020978100005,15.2,7.06841864999999));
#243438=CARTESIAN_POINT('Ctrl Pts',(-7.88020978100005,11.6,7.06841864999999));
#243439=CARTESIAN_POINT('Ctrl Pts',(-7.87901524500005,15.2,7.06675484299998));
#243440=CARTESIAN_POINT('Ctrl Pts',(-7.87901524500005,11.6,7.06675484299998));
#243441=CARTESIAN_POINT('Ctrl Pts',(-7.87782327800005,15.2,7.06509776599999));
#243442=CARTESIAN_POINT('Ctrl Pts',(-7.87782327800005,11.6,7.06509776599999));
#243443=CARTESIAN_POINT('Ctrl Pts',(-7.87663390200006,15.2,7.06344742199998));
#243444=CARTESIAN_POINT('Ctrl Pts',(-7.87663390200006,11.6,7.06344742199998));
#243445=CARTESIAN_POINT('Ctrl Pts',(-7.87544713200005,15.2,7.06180381599999));
#243446=CARTESIAN_POINT('Ctrl Pts',(-7.87544713200005,11.6,7.06180381599999));
#243447=CARTESIAN_POINT('Ctrl Pts',(-7.87426298700005,15.2,7.06016695499999));
#243448=CARTESIAN_POINT('Ctrl Pts',(-7.87426298700005,11.6,7.06016695499999));
#243449=CARTESIAN_POINT('Ctrl Pts',(-7.87308148500006,15.2,7.05853684399998));
#243450=CARTESIAN_POINT('Ctrl Pts',(-7.87308148500006,11.6,7.05853684399998));
#243451=CARTESIAN_POINT('Ctrl Pts',(-7.87190264400006,15.2,7.05691348899999));
#243452=CARTESIAN_POINT('Ctrl Pts',(-7.87190264400006,11.6,7.05691348899999));
#243453=CARTESIAN_POINT('Ctrl Pts',(-7.87072648300006,15.2,7.05529689499999));
#243454=CARTESIAN_POINT('Ctrl Pts',(-7.87072648300006,11.6,7.05529689499999));
#243455=CARTESIAN_POINT('Ctrl Pts',(-7.86955301900005,15.2,7.05368706799998));
#243456=CARTESIAN_POINT('Ctrl Pts',(-7.86955301900005,11.6,7.05368706799998));
#243457=CARTESIAN_POINT('Ctrl Pts',(-7.86838227000005,15.2,7.05208401299998));
#243458=CARTESIAN_POINT('Ctrl Pts',(-7.86838227000005,11.6,7.05208401299998));
#243459=CARTESIAN_POINT('Ctrl Pts',(-7.86721425700006,15.2,7.05048773599999));
#243460=CARTESIAN_POINT('Ctrl Pts',(-7.86721425700006,11.6,7.05048773599999));
#243461=CARTESIAN_POINT('Ctrl Pts',(-7.86604899600006,15.2,7.04889824399999));
#243462=CARTESIAN_POINT('Ctrl Pts',(-7.86604899600006,11.6,7.04889824399999));
#243463=CARTESIAN_POINT('Ctrl Pts',(-7.86488650700005,15.2,7.04731553999999));
#243464=CARTESIAN_POINT('Ctrl Pts',(-7.86488650700005,11.6,7.04731553999999));
#243465=CARTESIAN_POINT('Ctrl Pts',(-7.86372680800006,15.2,7.04573962999999));
#243466=CARTESIAN_POINT('Ctrl Pts',(-7.86372680800006,11.6,7.04573962999999));
#243467=CARTESIAN_POINT('Ctrl Pts',(-7.86256991700006,15.2,7.04417052199998));
#243468=CARTESIAN_POINT('Ctrl Pts',(-7.86256991700006,11.6,7.04417052199998));
#243469=CARTESIAN_POINT('Ctrl Pts',(-7.86141585400006,15.2,7.04260821999998));
#243470=CARTESIAN_POINT('Ctrl Pts',(-7.86141585400006,11.6,7.04260821999998));
#243471=CARTESIAN_POINT('Ctrl Pts',(-7.86026463600006,15.2,7.04105272899999));
#243472=CARTESIAN_POINT('Ctrl Pts',(-7.86026463600006,11.6,7.04105272899999));
#243473=CARTESIAN_POINT('Ctrl Pts',(-7.85911628400005,15.2,7.03950405599999));
#243474=CARTESIAN_POINT('Ctrl Pts',(-7.85911628400005,11.6,7.03950405599999));
#243475=CARTESIAN_POINT('Ctrl Pts',(-7.85797081600006,15.2,7.03796220599998));
#243476=CARTESIAN_POINT('Ctrl Pts',(-7.85797081600006,11.6,7.03796220599998));
#243477=CARTESIAN_POINT('Ctrl Pts',(-7.85682825100006,15.2,7.03642718499999));
#243478=CARTESIAN_POINT('Ctrl Pts',(-7.85682825100006,11.6,7.03642718499999));
#243479=CARTESIAN_POINT('Ctrl Pts',(-7.85568860800005,15.2,7.03489899899999));
#243480=CARTESIAN_POINT('Ctrl Pts',(-7.85568860800005,11.6,7.03489899899999));
#243481=CARTESIAN_POINT('Ctrl Pts',(-7.85455190600005,15.2,7.03337765199999));
#243482=CARTESIAN_POINT('Ctrl Pts',(-7.85455190600005,11.6,7.03337765199999));
#243483=CARTESIAN_POINT('Ctrl Pts',(-7.85341816500006,15.2,7.03186315199999));
#243484=CARTESIAN_POINT('Ctrl Pts',(-7.85341816500006,11.6,7.03186315199999));
#243485=CARTESIAN_POINT('Ctrl Pts',(-7.85228740400005,15.2,7.03035550199999));
#243486=CARTESIAN_POINT('Ctrl Pts',(-7.85228740400005,11.6,7.03035550199999));
#243487=CARTESIAN_POINT('Ctrl Pts',(-7.85115964100005,15.2,7.02885470999998));
#243488=CARTESIAN_POINT('Ctrl Pts',(-7.85115964100005,11.6,7.02885470999998));
#243489=CARTESIAN_POINT('Ctrl Pts',(-7.85003489800006,15.2,7.02736078099999));
#243490=CARTESIAN_POINT('Ctrl Pts',(-7.85003489800006,11.6,7.02736078099999));
#243491=CARTESIAN_POINT('Ctrl Pts',(-7.84891319200005,15.2,7.02587372099998));
#243492=CARTESIAN_POINT('Ctrl Pts',(-7.84891319200005,11.6,7.02587372099998));
#243493=CARTESIAN_POINT('Ctrl Pts',(-7.84779454400006,15.2,7.02439353499998));
#243494=CARTESIAN_POINT('Ctrl Pts',(-7.84779454400006,11.6,7.02439353499998));
#243495=CARTESIAN_POINT('Ctrl Pts',(-7.84667897300006,15.2,7.02292022999998));
#243496=CARTESIAN_POINT('Ctrl Pts',(-7.84667897300006,11.6,7.02292022999998));
#243497=CARTESIAN_POINT('Ctrl Pts',(-7.84556650000006,15.2,7.02145380999998));
#243498=CARTESIAN_POINT('Ctrl Pts',(-7.84556650000006,11.6,7.02145380999998));
#243499=CARTESIAN_POINT('Ctrl Pts',(-7.84445714300006,15.2,7.01999428199999));
#243500=CARTESIAN_POINT('Ctrl Pts',(-7.84445714300006,11.6,7.01999428199999));
#243501=CARTESIAN_POINT('Ctrl Pts',(-7.84335092300006,15.2,7.01854165199999));
#243502=CARTESIAN_POINT('Ctrl Pts',(-7.84335092300006,11.6,7.01854165199999));
#243503=CARTESIAN_POINT('Ctrl Pts',(-7.84224785900006,15.2,7.01709592399999));
#243504=CARTESIAN_POINT('Ctrl Pts',(-7.84224785900006,11.6,7.01709592399999));
#243505=CARTESIAN_POINT('Ctrl Pts',(-7.84114797200005,15.2,7.01565710699998));
#243506=CARTESIAN_POINT('Ctrl Pts',(-7.84114797200005,11.6,7.01565710699998));
#243507=CARTESIAN_POINT('Ctrl Pts',(-7.84005128300005,15.2,7.01422520199999));
#243508=CARTESIAN_POINT('Ctrl Pts',(-7.84005128300005,11.6,7.01422520199999));
#243509=CARTESIAN_POINT('Ctrl Pts',(-7.83895781000006,15.2,7.01280021999998));
#243510=CARTESIAN_POINT('Ctrl Pts',(-7.83895781000006,11.6,7.01280021999998));
#243511=CARTESIAN_POINT('Ctrl Pts',(-7.83786757400006,15.2,7.01138216399999));
#243512=CARTESIAN_POINT('Ctrl Pts',(-7.83786757400006,11.6,7.01138216399999));
#243513=CARTESIAN_POINT('Ctrl Pts',(-7.83678059600006,15.2,7.00997103999998));
#243514=CARTESIAN_POINT('Ctrl Pts',(-7.83678059600006,11.6,7.00997103999998));
#243515=CARTESIAN_POINT('Ctrl Pts',(-7.83569689500006,15.2,7.00856685299998));
#243516=CARTESIAN_POINT('Ctrl Pts',(-7.83569689500006,11.6,7.00856685299998));
#243517=CARTESIAN_POINT('Ctrl Pts',(-7.83461649300006,15.2,7.00716961199999));
#243518=CARTESIAN_POINT('Ctrl Pts',(-7.83461649300006,11.6,7.00716961199999));
#243519=CARTESIAN_POINT('Ctrl Pts',(-7.83353941100006,15.2,7.00577931999998));
#243520=CARTESIAN_POINT('Ctrl Pts',(-7.83353941100006,11.6,7.00577931999998));
#243521=CARTESIAN_POINT('Ctrl Pts',(-7.83246566700005,15.2,7.00439598299998));
#243522=CARTESIAN_POINT('Ctrl Pts',(-7.83246566700005,11.6,7.00439598299998));
#243523=CARTESIAN_POINT('Ctrl Pts',(-7.83139528400006,15.2,7.00301960799998));
#243524=CARTESIAN_POINT('Ctrl Pts',(-7.83139528400006,11.6,7.00301960799998));
#243525=CARTESIAN_POINT('Ctrl Pts',(-7.83032828200006,15.2,7.00165019999999));
#243526=CARTESIAN_POINT('Ctrl Pts',(-7.83032828200006,11.6,7.00165019999999));
#243527=CARTESIAN_POINT('Ctrl Pts',(-7.82926468300006,15.2,7.00028776499998));
#243528=CARTESIAN_POINT('Ctrl Pts',(-7.82926468300006,11.6,7.00028776499998));
#243529=CARTESIAN_POINT('Ctrl Pts',(-7.82820450700005,15.2,6.99893230999999));
#243530=CARTESIAN_POINT('Ctrl Pts',(-7.82820450700005,11.6,6.99893230999999));
#243531=CARTESIAN_POINT('Ctrl Pts',(-7.82714777400006,15.2,6.99758383999999));
#243532=CARTESIAN_POINT('Ctrl Pts',(-7.82714777400006,11.6,6.99758383999999));
#243533=CARTESIAN_POINT('Ctrl Pts',(-7.82609450600006,15.2,6.99624236099999));
#243534=CARTESIAN_POINT('Ctrl Pts',(-7.82609450600006,11.6,6.99624236099999));
#243535=CARTESIAN_POINT('Ctrl Pts',(-7.82504472500006,15.2,6.99490787899999));
#243536=CARTESIAN_POINT('Ctrl Pts',(-7.82504472500006,11.6,6.99490787899999));
#243537=CARTESIAN_POINT('Ctrl Pts',(-7.82399845200005,15.2,6.99358039999999));
#243538=CARTESIAN_POINT('Ctrl Pts',(-7.82399845200005,11.6,6.99358039999999));
#243539=CARTESIAN_POINT('Ctrl Pts',(-7.82295570800006,15.2,6.99225992899999));
#243540=CARTESIAN_POINT('Ctrl Pts',(-7.82295570800006,11.6,6.99225992899999));
#243541=CARTESIAN_POINT('Ctrl Pts',(-7.82191651400005,15.2,6.99094647299999));
#243542=CARTESIAN_POINT('Ctrl Pts',(-7.82191651400005,11.6,6.99094647299999));
#243543=CARTESIAN_POINT('Ctrl Pts',(-7.82088089200006,15.2,6.98964003799999));
#243544=CARTESIAN_POINT('Ctrl Pts',(-7.82088089200006,11.6,6.98964003799999));
#243545=CARTESIAN_POINT('Ctrl Pts',(-7.81984886500006,15.2,6.98834062899999));
#243546=CARTESIAN_POINT('Ctrl Pts',(-7.81984886500006,11.6,6.98834062899999));
#243547=CARTESIAN_POINT('Ctrl Pts',(-7.81882045200006,15.2,6.98704825399999));
#243548=CARTESIAN_POINT('Ctrl Pts',(-7.81882045200006,11.6,6.98704825399999));
#243549=CARTESIAN_POINT('Ctrl Pts',(-7.81779567800006,15.2,6.98576291699998));
#243550=CARTESIAN_POINT('Ctrl Pts',(-7.81779567800006,11.6,6.98576291699998));
#243551=CARTESIAN_POINT('Ctrl Pts',(-7.81677456100006,15.2,6.98448462499999));
#243552=CARTESIAN_POINT('Ctrl Pts',(-7.81677456100006,11.6,6.98448462499999));
#243553=CARTESIAN_POINT('Ctrl Pts',(-7.81575712600005,15.2,6.98321338399998));
#243554=CARTESIAN_POINT('Ctrl Pts',(-7.81575712600005,11.6,6.98321338399998));
#243555=CARTESIAN_POINT('Ctrl Pts',(-7.81474339500006,15.2,6.98194919799998));
#243556=CARTESIAN_POINT('Ctrl Pts',(-7.81474339500006,11.6,6.98194919799998));
#243557=CARTESIAN_POINT('Ctrl Pts',(-7.81373338800006,15.2,6.98069207599998));
#243558=CARTESIAN_POINT('Ctrl Pts',(-7.81373338800006,11.6,6.98069207599998));
#243559=CARTESIAN_POINT('Ctrl Pts',(-7.81272713000006,15.2,6.97944202399999));
#243560=CARTESIAN_POINT('Ctrl Pts',(-7.81272713000006,11.6,6.97944202399999));
#243561=CARTESIAN_POINT('Ctrl Pts',(-7.81172464100005,15.2,6.97819904499998));
#243562=CARTESIAN_POINT('Ctrl Pts',(-7.81172464100005,11.6,6.97819904499998));
#243563=CARTESIAN_POINT('Ctrl Pts',(-7.81072594600006,15.2,6.97696314799998));
#243564=CARTESIAN_POINT('Ctrl Pts',(-7.81072594600006,11.6,6.97696314799998));
#243565=CARTESIAN_POINT('Ctrl Pts',(-7.80973106400006,15.2,6.97573433799998));
#243566=CARTESIAN_POINT('Ctrl Pts',(-7.80973106400006,11.6,6.97573433799998));
#243567=CARTESIAN_POINT('Ctrl Pts',(-7.80874002000005,15.2,6.97451262099998));
#243568=CARTESIAN_POINT('Ctrl Pts',(-7.80874002000005,11.6,6.97451262099998));
#243569=CARTESIAN_POINT('Ctrl Pts',(-7.80775283700006,15.2,6.97329800299999));
#243570=CARTESIAN_POINT('Ctrl Pts',(-7.80775283700006,11.6,6.97329800299999));
#243571=CARTESIAN_POINT('Ctrl Pts',(-7.80676953600006,15.2,6.97209049099998));
#243572=CARTESIAN_POINT('Ctrl Pts',(-7.80676953600006,11.6,6.97209049099998));
#243573=CARTESIAN_POINT('Ctrl Pts',(-7.80579014100006,15.2,6.97089009099999));
#243574=CARTESIAN_POINT('Ctrl Pts',(-7.80579014100006,11.6,6.97089009099999));
#243575=CARTESIAN_POINT('Ctrl Pts',(-7.80481467600006,15.2,6.96969680799998));
#243576=CARTESIAN_POINT('Ctrl Pts',(-7.80481467600006,11.6,6.96969680799998));
#243577=CARTESIAN_POINT('Ctrl Pts',(-7.80384316200006,15.2,6.96851064799999));
#243578=CARTESIAN_POINT('Ctrl Pts',(-7.80384316200006,11.6,6.96851064799999));
#243579=CARTESIAN_POINT('Ctrl Pts',(-7.80287562300006,15.2,6.96733161899999));
#243580=CARTESIAN_POINT('Ctrl Pts',(-7.80287562300006,11.6,6.96733161899999));
#243581=CARTESIAN_POINT('Ctrl Pts',(-7.80191208300005,15.2,6.96615972599999));
#243582=CARTESIAN_POINT('Ctrl Pts',(-7.80191208300005,11.6,6.96615972599999));
#243583=CARTESIAN_POINT('Ctrl Pts',(-7.80095256500006,15.2,6.96499497499998));
#243584=CARTESIAN_POINT('Ctrl Pts',(-7.80095256500006,11.6,6.96499497499998));
#243585=CARTESIAN_POINT('Ctrl Pts',(-7.79999709200006,15.2,6.96383737299998));
#243586=CARTESIAN_POINT('Ctrl Pts',(-7.79999709200006,11.6,6.96383737299998));
#243587=CARTESIAN_POINT('Ctrl Pts',(-7.79904568800006,15.2,6.96268692599999));
#243588=CARTESIAN_POINT('Ctrl Pts',(-7.79904568800006,11.6,6.96268692599999));
#243589=CARTESIAN_POINT('Ctrl Pts',(-7.79809837800006,15.2,6.96154363999998));
#243590=CARTESIAN_POINT('Ctrl Pts',(-7.79809837800006,11.6,6.96154363999998));
#243591=CARTESIAN_POINT('Ctrl Pts',(-7.79715518200006,15.2,6.96040752099999));
#243592=CARTESIAN_POINT('Ctrl Pts',(-7.79715518200006,11.6,6.96040752099999));
#243593=CARTESIAN_POINT('Ctrl Pts',(-7.79621612700005,15.2,6.95927857499999));
#243594=CARTESIAN_POINT('Ctrl Pts',(-7.79621612700005,11.6,6.95927857499999));
#243595=CARTESIAN_POINT('Ctrl Pts',(-7.79528123700005,15.2,6.95815680999999));
#243596=CARTESIAN_POINT('Ctrl Pts',(-7.79528123700005,11.6,6.95815680999999));
#243597=CARTESIAN_POINT('Ctrl Pts',(-7.79435053400006,15.2,6.95704223099998));
#243598=CARTESIAN_POINT('Ctrl Pts',(-7.79435053400006,11.6,6.95704223099998));
#243599=CARTESIAN_POINT('Ctrl Pts',(-7.79342404400006,15.2,6.95593484299999));
#243600=CARTESIAN_POINT('Ctrl Pts',(-7.79342404400006,11.6,6.95593484299999));
#243601=CARTESIAN_POINT('Ctrl Pts',(-7.79250179200006,15.2,6.95483465499999));
#243602=CARTESIAN_POINT('Ctrl Pts',(-7.79250179200006,11.6,6.95483465499999));
#243603=CARTESIAN_POINT('Ctrl Pts',(-7.79158380000006,15.2,6.95374166999999));
#243604=CARTESIAN_POINT('Ctrl Pts',(-7.79158380000006,11.6,6.95374166999999));
#243605=CARTESIAN_POINT('Ctrl Pts',(-7.79067009400006,15.2,6.95265589799998));
#243606=CARTESIAN_POINT('Ctrl Pts',(-7.79067009400006,11.6,6.95265589799998));
#243607=CARTESIAN_POINT('Ctrl Pts',(-7.78976069700006,15.2,6.95157734299999));
#243608=CARTESIAN_POINT('Ctrl Pts',(-7.78976069700006,11.6,6.95157734299999));
#243609=CARTESIAN_POINT('Ctrl Pts',(-7.78885563500006,15.2,6.95050601399998));
#243610=CARTESIAN_POINT('Ctrl Pts',(-7.78885563500006,11.6,6.95050601399998));
#243611=CARTESIAN_POINT('Ctrl Pts',(-7.78795493400006,15.2,6.94944191199999));
#243612=CARTESIAN_POINT('Ctrl Pts',(-7.78795493400006,11.6,6.94944191199999));
#243613=CARTESIAN_POINT('Ctrl Pts',(-7.78705861700006,15.2,6.94838504899998));
#243614=CARTESIAN_POINT('Ctrl Pts',(-7.78705861700006,11.6,6.94838504899998));
#243615=CARTESIAN_POINT('Ctrl Pts',(-7.78616671000006,15.2,6.94733542799998));
#243616=CARTESIAN_POINT('Ctrl Pts',(-7.78616671000006,11.6,6.94733542799998));
#243617=CARTESIAN_POINT('Ctrl Pts',(-7.78527923800005,15.2,6.94629305799998));
#243618=CARTESIAN_POINT('Ctrl Pts',(-7.78527923800005,11.6,6.94629305799998));
#243619=CARTESIAN_POINT('Ctrl Pts',(-7.78439622500006,15.2,6.94525794299999));
#243620=CARTESIAN_POINT('Ctrl Pts',(-7.78439622500006,11.6,6.94525794299999));
#243621=CARTESIAN_POINT('Ctrl Pts',(-7.78351769900006,15.2,6.94423009099999));
#243622=CARTESIAN_POINT('Ctrl Pts',(-7.78351769900006,11.6,6.94423009099999));
#243623=CARTESIAN_POINT('Ctrl Pts',(-7.78264368300006,15.2,6.94320950799998));
#243624=CARTESIAN_POINT('Ctrl Pts',(-7.78264368300006,11.6,6.94320950799998));
#243625=CARTESIAN_POINT('Ctrl Pts',(-7.78177420300005,15.2,6.94219619999998));
#243626=CARTESIAN_POINT('Ctrl Pts',(-7.78177420300005,11.6,6.94219619999998));
#243627=CARTESIAN_POINT('Ctrl Pts',(-7.78090928600006,15.2,6.94119017399998));
#243628=CARTESIAN_POINT('Ctrl Pts',(-7.78090928600006,11.6,6.94119017399998));
#243629=CARTESIAN_POINT('Ctrl Pts',(-7.78004895800006,15.2,6.94019143699999));
#243630=CARTESIAN_POINT('Ctrl Pts',(-7.78004895800006,11.6,6.94019143699999));
#243631=CARTESIAN_POINT('Ctrl Pts',(-7.77919324200005,15.2,6.93919999399998));
#243632=CARTESIAN_POINT('Ctrl Pts',(-7.77919324200005,11.6,6.93919999399998));
#243633=CARTESIAN_POINT('Ctrl Pts',(-7.77834216700005,15.2,6.93821585299998));
#243634=CARTESIAN_POINT('Ctrl Pts',(-7.77834216700005,11.6,6.93821585299998));
#243635=CARTESIAN_POINT('Ctrl Pts',(-7.77749575900006,15.2,6.93723901999999));
#243636=CARTESIAN_POINT('Ctrl Pts',(-7.77749575900006,11.6,6.93723901999999));
#243637=CARTESIAN_POINT('Ctrl Pts',(-7.77665404200006,15.2,6.93626949999998));
#243638=CARTESIAN_POINT('Ctrl Pts',(-7.77665404200006,11.6,6.93626949999998));
#243639=CARTESIAN_POINT('Ctrl Pts',(-7.77581704500006,15.2,6.93530730299998));
#243640=CARTESIAN_POINT('Ctrl Pts',(-7.77581704500006,11.6,6.93530730299998));
#243641=CARTESIAN_POINT('Ctrl Pts',(-7.77498479200006,15.2,6.93435243299999));
#243642=CARTESIAN_POINT('Ctrl Pts',(-7.77498479200006,11.6,6.93435243299999));
#243643=CARTESIAN_POINT('Ctrl Pts',(-7.77415731300006,15.2,6.93340489699998));
#243644=CARTESIAN_POINT('Ctrl Pts',(-7.77415731300006,11.6,6.93340489699998));
#243645=CARTESIAN_POINT('Ctrl Pts',(-7.77333463200006,15.2,6.93246470299999));
#243646=CARTESIAN_POINT('Ctrl Pts',(-7.77333463200006,11.6,6.93246470299999));
#243647=CARTESIAN_POINT('Ctrl Pts',(-7.77251677700006,15.2,6.93153185599999));
#243648=CARTESIAN_POINT('Ctrl Pts',(-7.77251677700006,11.6,6.93153185599999));
#243649=CARTESIAN_POINT('Ctrl Pts',(-7.77170377400005,15.2,6.93060636399998));
#243650=CARTESIAN_POINT('Ctrl Pts',(-7.77170377400005,11.6,6.93060636399998));
#243651=CARTESIAN_POINT('Ctrl Pts',(-7.77089565100006,15.2,6.92968823199998));
#243652=CARTESIAN_POINT('Ctrl Pts',(-7.77089565100006,11.6,6.92968823199998));
#243653=CARTESIAN_POINT('Ctrl Pts',(-7.77009243600006,15.2,6.92877746799999));
#243654=CARTESIAN_POINT('Ctrl Pts',(-7.77009243600006,11.6,6.92877746799999));
#243655=CARTESIAN_POINT('Ctrl Pts',(-7.76929415400006,15.2,6.92787407899999));
#243656=CARTESIAN_POINT('Ctrl Pts',(-7.76929415400006,11.6,6.92787407899999));
#243657=CARTESIAN_POINT('Ctrl Pts',(-7.76850083500006,15.2,6.92697806999998));
#243658=CARTESIAN_POINT('Ctrl Pts',(-7.76850083500006,11.6,6.92697806999998));
#243659=CARTESIAN_POINT('Ctrl Pts',(-7.76771250600006,15.2,6.92608944899998));
#243660=CARTESIAN_POINT('Ctrl Pts',(-7.76771250600006,11.6,6.92608944899998));
#243661=CARTESIAN_POINT('Ctrl Pts',(-7.76692919400006,15.2,6.92520822299999));
#243662=CARTESIAN_POINT('Ctrl Pts',(-7.76692919400006,11.6,6.92520822299999));
#243663=CARTESIAN_POINT('Ctrl Pts',(-7.76615092800006,15.2,6.92433439799998));
#243664=CARTESIAN_POINT('Ctrl Pts',(-7.76615092800006,11.6,6.92433439799998));
#243665=CARTESIAN_POINT('Ctrl Pts',(-7.76537773500006,15.2,6.92346798199999));
#243666=CARTESIAN_POINT('Ctrl Pts',(-7.76537773500006,11.6,6.92346798199999));
#243667=CARTESIAN_POINT('Ctrl Pts',(-7.76460964500006,15.2,6.92260897999999));
#243668=CARTESIAN_POINT('Ctrl Pts',(-7.76460964500006,11.6,6.92260897999999));
#243669=CARTESIAN_POINT('Ctrl Pts',(-7.76384668300006,15.2,6.92175739999998));
#243670=CARTESIAN_POINT('Ctrl Pts',(-7.76384668300006,11.6,6.92175739999998));
#243671=CARTESIAN_POINT('Ctrl Pts',(-7.76308888000005,15.2,6.92091324899998));
#243672=CARTESIAN_POINT('Ctrl Pts',(-7.76308888000005,11.6,6.92091324899998));
#243673=CARTESIAN_POINT('Ctrl Pts',(-7.76233626500006,15.2,6.92007653299999));
#243674=CARTESIAN_POINT('Ctrl Pts',(-7.76233626500006,11.6,6.92007653299999));
#243675=CARTESIAN_POINT('Ctrl Pts',(-7.76158886500006,15.2,6.91924725999999));
#243676=CARTESIAN_POINT('Ctrl Pts',(-7.76158886500006,11.6,6.91924725999999));
#243677=CARTESIAN_POINT('Ctrl Pts',(-7.76084671000006,15.2,6.91842543699998));
#243678=CARTESIAN_POINT('Ctrl Pts',(-7.76084671000006,11.6,6.91842543699998));
#243679=CARTESIAN_POINT('Ctrl Pts',(-7.76010982700006,15.2,6.91761106899998));
#243680=CARTESIAN_POINT('Ctrl Pts',(-7.76010982700006,11.6,6.91761106899998));
#243681=CARTESIAN_POINT('Ctrl Pts',(-7.75937824900006,15.2,6.91680416399999));
#243682=CARTESIAN_POINT('Ctrl Pts',(-7.75937824900006,11.6,6.91680416399999));
#243683=CARTESIAN_POINT('Ctrl Pts',(-7.75865200200006,15.2,6.91600473099999));
#243684=CARTESIAN_POINT('Ctrl Pts',(-7.75865200200006,11.6,6.91600473099999));
#243685=CARTESIAN_POINT('Ctrl Pts',(-7.75793111600006,15.2,6.91521277299999));
#243686=CARTESIAN_POINT('Ctrl Pts',(-7.75793111600006,11.6,6.91521277299999));
#243687=CARTESIAN_POINT('Ctrl Pts',(-7.75721562100006,15.2,6.91442829999998));
#243688=CARTESIAN_POINT('Ctrl Pts',(-7.75721562100006,11.6,6.91442829999998));
#243689=CARTESIAN_POINT('Ctrl Pts',(-7.75650554800006,15.2,6.91365131899998));
#243690=CARTESIAN_POINT('Ctrl Pts',(-7.75650554800006,11.6,6.91365131899998));
#243691=CARTESIAN_POINT('Ctrl Pts',(-7.75580092400006,15.2,6.91288183599998));
#243692=CARTESIAN_POINT('Ctrl Pts',(-7.75580092400006,11.6,6.91288183599998));
#243693=CARTESIAN_POINT('Ctrl Pts',(-7.75510178000006,15.2,6.91211985699999));
#243694=CARTESIAN_POINT('Ctrl Pts',(-7.75510178000006,11.6,6.91211985699999));
#243695=CARTESIAN_POINT('Ctrl Pts',(-7.75440814900006,15.2,6.91136539199999));
#243696=CARTESIAN_POINT('Ctrl Pts',(-7.75440814900006,11.6,6.91136539199999));
#243697=CARTESIAN_POINT('Ctrl Pts',(-7.75372005700006,15.2,6.91061844599999));
#243698=CARTESIAN_POINT('Ctrl Pts',(-7.75372005700006,11.6,6.91061844599999));
#243699=CARTESIAN_POINT('Ctrl Pts',(-7.75303753800006,15.2,6.90987902599999));
#243700=CARTESIAN_POINT('Ctrl Pts',(-7.75303753800006,11.6,6.90987902599999));
#243701=CARTESIAN_POINT('Ctrl Pts',(-7.75236062000006,15.2,6.90914714099998));
#243702=CARTESIAN_POINT('Ctrl Pts',(-7.75236062000006,11.6,6.90914714099998));
#243703=CARTESIAN_POINT('Ctrl Pts',(-7.75168933500006,15.2,6.90842279499999));
#243704=CARTESIAN_POINT('Ctrl Pts',(-7.75168933500006,11.6,6.90842279499999));
#243705=CARTESIAN_POINT('Ctrl Pts',(-7.75102371400005,15.2,6.90770599899999));
#243706=CARTESIAN_POINT('Ctrl Pts',(-7.75102371400005,11.6,6.90770599899999));
#243707=CARTESIAN_POINT('Ctrl Pts',(-7.75036378800006,15.2,6.90699675799999));
#243708=CARTESIAN_POINT('Ctrl Pts',(-7.75036378800006,11.6,6.90699675799999));
#243709=CARTESIAN_POINT('Ctrl Pts',(-7.74970958800005,15.2,6.90629507899998));
#243710=CARTESIAN_POINT('Ctrl Pts',(-7.74970958800005,11.6,6.90629507899998));
#243711=CARTESIAN_POINT('Ctrl Pts',(-7.74906114600006,15.2,6.90560096999998));
#243712=CARTESIAN_POINT('Ctrl Pts',(-7.74906114600006,11.6,6.90560096999998));
#243713=CARTESIAN_POINT('Ctrl Pts',(-7.74841849100006,15.2,6.90491443799999));
#243714=CARTESIAN_POINT('Ctrl Pts',(-7.74841849100006,11.6,6.90491443799999));
#243715=CARTESIAN_POINT('Ctrl Pts',(-7.74778165900005,15.2,6.90423549099999));
#243716=CARTESIAN_POINT('Ctrl Pts',(-7.74778165900005,11.6,6.90423549099999));
#243717=CARTESIAN_POINT('Ctrl Pts',(-7.74715431200006,15.2,6.90356800199999));
#243718=CARTESIAN_POINT('Ctrl Pts',(-7.74715431200006,11.6,6.90356800199999));
#243719=CARTESIAN_POINT('Ctrl Pts',(-7.74665780200006,15.2,6.90304077499999));
#243720=CARTESIAN_POINT('Ctrl Pts',(-7.74665780200006,11.6,6.90304077499999));
#243721=CARTESIAN_POINT('Ctrl Pts',(-7.74628893100005,15.2,6.90264966899999));
#243722=CARTESIAN_POINT('Ctrl Pts',(-7.74628893100005,11.6,6.90264966899999));
#243723=CARTESIAN_POINT('Ctrl Pts',(-7.74604536300006,15.2,6.90239167399999));
#243724=CARTESIAN_POINT('Ctrl Pts',(-7.74604536300006,11.6,6.90239167399999));
#243725=CARTESIAN_POINT('Ctrl Pts',(-7.74592563800006,15.2,6.90226491999999));
#243726=CARTESIAN_POINT('Ctrl Pts',(-7.74592563800006,11.6,6.90226491999999));
#243727=CARTESIAN_POINT('',(-7.74592563733583,12.2,6.90226492000216));
#243728=CARTESIAN_POINT('',(-7.74592563733583,15.2,6.90226492000216));
#243729=CARTESIAN_POINT('',(-7.74592563700006,12.2,6.90226491999999));
#243730=CARTESIAN_POINT('Ctrl Pts',(-8.32310290900006,12.2,7.93573928299999));
#243731=CARTESIAN_POINT('Ctrl Pts',(-8.3217721687583,12.2,7.93215545234894));
#243732=CARTESIAN_POINT('Ctrl Pts',(-8.32043968335571,12.2,7.92857931992112));
#243733=CARTESIAN_POINT('Ctrl Pts',(-8.31910545589695,12.2,7.92501089665198));
#243734=CARTESIAN_POINT('Ctrl Pts',(-8.31777122843819,12.2,7.92144247338284));
#243735=CARTESIAN_POINT('Ctrl Pts',(-8.31643525654356,12.2,7.91788175518672));
#243736=CARTESIAN_POINT('Ctrl Pts',(-8.31509755652553,12.2,7.91432875292909));
#243737=CARTESIAN_POINT('Ctrl Pts',(-8.31375985650751,12.2,7.91077575067146));
#243738=CARTESIAN_POINT('Ctrl Pts',(-8.31242042912681,12.2,7.90723046471033));
#243739=CARTESIAN_POINT('Ctrl Pts',(-8.31107930955076,12.2,7.90369291629612));
#243740=CARTESIAN_POINT('Ctrl Pts',(-8.30973818973107,12.2,7.90015536723925));
#243741=CARTESIAN_POINT('Ctrl Pts',(-8.3083953809026,12.2,7.89662555690962));
#243742=CARTESIAN_POINT('Ctrl Pts',(-8.30705092395697,12.2,7.89310351077379));
#243743=CARTESIAN_POINT('Ctrl Pts',(-8.30570646725559,12.2,7.88958146527781));
#243744=CARTESIAN_POINT('Ctrl Pts',(-8.30436036267098,12.2,7.88606718318977));
#243745=CARTESIAN_POINT('Ctrl Pts',(-8.30301264530314,12.2,7.88256068565118));
#243746=CARTESIAN_POINT('Ctrl Pts',(-8.3016649279353,12.2,7.8790541881126));
#243747=CARTESIAN_POINT('Ctrl Pts',(-8.30031559653923,12.2,7.87555547376907));
#243748=CARTESIAN_POINT('Ctrl Pts',(-8.29896468270717,12.2,7.87206456271343));
#243749=CARTESIAN_POINT('Ctrl Pts',(-8.29761376887511,12.2,7.86857365165778));
#243750=CARTESIAN_POINT('Ctrl Pts',(-8.29626127309158,12.2,7.86509054252597));
#243751=CARTESIAN_POINT('Ctrl Pts',(-8.29490723125963,12.2,7.86161525801142));
#243752=CARTESIAN_POINT('Ctrl Pts',(-8.29355318942768,12.2,7.85813997349687));
#243753=CARTESIAN_POINT('Ctrl Pts',(-8.29219760124853,12.2,7.85467251283548));
#243754=CARTESIAN_POINT('Ctrl Pts',(-8.29084050442296,12.2,7.85121289833549));
#243755=CARTESIAN_POINT('Ctrl Pts',(-8.2894834075974,12.2,7.8477532838355));
#243756=CARTESIAN_POINT('Ctrl Pts',(-8.28812480111361,12.2,7.84430151517664));
#243757=CARTESIAN_POINT('Ctrl Pts',(-8.28676472178823,12.2,7.84085761175903));
#243758=CARTESIAN_POINT('Ctrl Pts',(-8.28540464221577,12.2,7.83741370771578));
#243759=CARTESIAN_POINT('Ctrl Pts',(-8.28404308923455,12.2,7.83397767058309));
#243760=CARTESIAN_POINT('Ctrl Pts',(-8.2826800977446,12.2,7.83054951996093));
#243761=CARTESIAN_POINT('Ctrl Pts',(-8.28131710650225,12.2,7.82712136996156));
#243762=CARTESIAN_POINT('Ctrl Pts',(-8.2799526774879,12.2,7.82370110605206));
#243763=CARTESIAN_POINT('Ctrl Pts',(-8.27858684621913,12.2,7.8202887503398));
#243764=CARTESIAN_POINT('Ctrl Pts',(-8.27722101495035,12.2,7.81687639462754));
#243765=CARTESIAN_POINT('Ctrl Pts',(-8.27585378260126,12.2,7.81347194655575));
#243766=CARTESIAN_POINT('Ctrl Pts',(-8.2744851853592,12.2,7.81007542713818));
#243767=CARTESIAN_POINT('Ctrl Pts',(-8.27266038911933,12.2,7.80554673478709));
#243768=CARTESIAN_POINT('Ctrl Pts',(-8.27083316650773,12.2,7.80103213932765));
#243769=CARTESIAN_POINT('Ctrl Pts',(-8.2690036048242,12.2,7.79653168752742));
#243770=CARTESIAN_POINT('Ctrl Pts',(-8.26717404289138,12.2,7.79203123511401));
#243771=CARTESIAN_POINT('Ctrl Pts',(-8.26534214192101,12.2,7.78754492816924));
#243772=CARTESIAN_POINT('Ctrl Pts',(-8.26350798875715,12.2,7.78307281573856));
#243773=CARTESIAN_POINT('Ctrl Pts',(-8.2621323740092,12.2,7.77971873172021));
#243774=CARTESIAN_POINT('Ctrl Pts',(-8.2607554923575,12.2,7.77637263131356));
#243775=CARTESIAN_POINT('Ctrl Pts',(-8.25937738302632,12.2,7.77303453725297));
#243776=CARTESIAN_POINT('Ctrl Pts',(-8.25799927369513,12.2,7.76969644319238));
#243777=CARTESIAN_POINT('Ctrl Pts',(-8.25661993461692,12.2,7.76636635415884));
#243778=CARTESIAN_POINT('Ctrl Pts',(-8.25523940487552,12.2,7.76304429211217));
#243779=CARTESIAN_POINT('Ctrl Pts',(-8.25385887513412,12.2,7.7597222300655));
#243780=CARTESIAN_POINT('Ctrl Pts',(-8.25247715451779,12.2,7.75640819370163));
#243781=CARTESIAN_POINT('Ctrl Pts',(-8.25109428027653,12.2,7.75310220519564));
#243782=CARTESIAN_POINT('Ctrl Pts',(-8.24971140578403,12.2,7.74979621608907));
#243783=CARTESIAN_POINT('Ctrl Pts',(-8.24832737769956,12.2,7.74649827459311));
#243784=CARTESIAN_POINT('Ctrl Pts',(-8.24694223516477,12.2,7.74320840103276));
#243785=CARTESIAN_POINT('Ctrl Pts',(-8.24555709288163,12.2,7.73991852807006));
#243786=CARTESIAN_POINT('Ctrl Pts',(-8.24417083556518,12.2,7.7366367241736));
#243787=CARTESIAN_POINT('Ctrl Pts',(-8.24278350136549,12.2,7.73336300966823));
#243788=CARTESIAN_POINT('Ctrl Pts',(-8.2413961671658,12.2,7.73008929516287));
#243789=CARTESIAN_POINT('Ctrl Pts',(-8.24000775692131,12.2,7.72682366972671));
#243790=CARTESIAN_POINT('Ctrl Pts',(-8.23861830821548,12.2,7.72356615474699));
#243791=CARTESIAN_POINT('Ctrl Pts',(-8.23722885950965,12.2,7.72030863976728));
#243792=CARTESIAN_POINT('Ctrl Pts',(-8.23583837275708,12.2,7.71705923499986));
#243793=CARTESIAN_POINT('Ctrl Pts',(-8.23444688750966,12.2,7.71381796247788));
#243794=CARTESIAN_POINT('Ctrl Pts',(-8.23305540226224,12.2,7.7105766899559));
#243795=CARTESIAN_POINT('Ctrl Pts',(-8.23166291776788,12.2,7.70734354880179));
#243796=CARTESIAN_POINT('Ctrl Pts',(-8.23026947361026,12.2,7.70411856033491));
#243797=CARTESIAN_POINT('Ctrl Pts',(-8.22887602945264,12.2,7.70089357186803));
#243798=CARTESIAN_POINT('Ctrl Pts',(-8.2274816267701,12.2,7.6976767369173));
#243799=CARTESIAN_POINT('Ctrl Pts',(-8.22608630302924,12.2,7.69446807494942));
#243800=CARTESIAN_POINT('Ctrl Pts',(-8.22469097903491,12.2,7.69125941239863));
#243801=CARTESIAN_POINT('Ctrl Pts',(-8.223294734032,12.2,7.68805892365019));
#243802=CARTESIAN_POINT('Ctrl Pts',(-8.22189760995382,12.2,7.68486663006234));
#243803=CARTESIAN_POINT('Ctrl Pts',(-8.22050048612946,12.2,7.68167433705444));
#243804=CARTESIAN_POINT('Ctrl Pts',(-8.21910248131524,12.2,7.6784902388112));
#243805=CARTESIAN_POINT('Ctrl Pts',(-8.21770363650441,12.2,7.67531435664389));
#243806=CARTESIAN_POINT('Ctrl Pts',(-8.21583851017469,12.2,7.67107984727978));
#243807=CARTESIAN_POINT('Ctrl Pts',(-8.21397188993607,12.2,7.66685994396491));
#243808=CARTESIAN_POINT('Ctrl Pts',(-8.21210387114443,12.2,7.66265469758552));
#243809=CARTESIAN_POINT('Ctrl Pts',(-8.21070285698707,12.2,7.65950076265773));
#243810=CARTESIAN_POINT('Ctrl Pts',(-8.20930105702143,12.2,7.65635507333771));
#243811=CARTESIAN_POINT('Ctrl Pts',(-8.20789851082248,12.2,7.6532176484089));
#243812=CARTESIAN_POINT('Ctrl Pts',(-8.20649596436875,12.2,7.65008022291012));
#243813=CARTESIAN_POINT('Ctrl Pts',(-8.20509267173139,12.2,7.64695106282185));
#243814=CARTESIAN_POINT('Ctrl Pts',(-8.20368867519391,12.2,7.64383018978608));
#243815=CARTESIAN_POINT('Ctrl Pts',(-8.20228467891149,12.2,7.64070931731727));
#243816=CARTESIAN_POINT('Ctrl Pts',(-8.20087997681404,12.2,7.63759673257408));
#243817=CARTESIAN_POINT('Ctrl Pts',(-8.19947461200315,12.2,7.63449245490774));
#243818=CARTESIAN_POINT('Ctrl Pts',(-8.19806924719226,12.2,7.6313881772414));
#243819=CARTESIAN_POINT('Ctrl Pts',(-8.19666321876234,12.2,7.62829220696728));
#243820=CARTESIAN_POINT('Ctrl Pts',(-8.19525656810506,12.2,7.62520456691351));
#243821=CARTESIAN_POINT('Ctrl Pts',(-8.19384991744778,12.2,7.62211692685975));
#243822=CARTESIAN_POINT('Ctrl Pts',(-8.19244264468225,12.2,7.61903761600502));
#243823=CARTESIAN_POINT('Ctrl Pts',(-8.19103479248339,12.2,7.61596665553325));
#243824=CARTESIAN_POINT('Ctrl Pts',(-8.18962694028454,12.2,7.61289569506149));
#243825=CARTESIAN_POINT('Ctrl Pts',(-8.18821850786906,12.2,7.60983308587275));
#243826=CARTESIAN_POINT('Ctrl Pts',(-8.18680953762863,12.2,7.60677884835798));
#243827=CARTESIAN_POINT('Ctrl Pts',(-8.18540056738819,12.2,7.6037246108432));
#243828=CARTESIAN_POINT('Ctrl Pts',(-8.18399105832535,12.2,7.60067874456338));
#243829=CARTESIAN_POINT('Ctrl Pts',(-8.18258105455619,12.2,7.59764127235435));
#243830=CARTESIAN_POINT('Ctrl Pts',(-8.18117105078703,12.2,7.59460380014533));
#243831=CARTESIAN_POINT('Ctrl Pts',(-8.17976055227297,12.2,7.59157472098313));
#243832=CARTESIAN_POINT('Ctrl Pts',(-8.17834960057431,12.2,7.5885540569251));
#243833=CARTESIAN_POINT('Ctrl Pts',(-8.17646833147189,12.2,7.58452650448189));
#243834=CARTESIAN_POINT('Ctrl Pts',(-8.17458625622489,12.2,7.58051391034001));
#243835=CARTESIAN_POINT('Ctrl Pts',(-8.1727034792334,12.2,7.57651632723326));
#243836=CARTESIAN_POINT('Ctrl Pts',(-8.17082070224191,12.2,7.57251874412652));
#243837=CARTESIAN_POINT('Ctrl Pts',(-8.16893722194197,12.2,7.56853617121593));
#243838=CARTESIAN_POINT('Ctrl Pts',(-8.16705314345035,12.2,7.56456865833459));
#243839=CARTESIAN_POINT('Ctrl Pts',(-8.16516906521542,12.2,7.56060114599381));
#243840=CARTESIAN_POINT('Ctrl Pts',(-8.16328438602245,12.2,7.55664869561255));
#243841=CARTESIAN_POINT('Ctrl Pts',(-8.16139921250134,12.2,7.55271135652761));
#243842=CARTESIAN_POINT('Ctrl Pts',(-8.15951403872337,12.2,7.5487740169062));
#243843=CARTESIAN_POINT('Ctrl Pts',(-8.15762836900285,12.2,7.54485179018918));
#243844=CARTESIAN_POINT('Ctrl Pts',(-8.15574230940002,12.2,7.54094472464446));
#243845=CARTESIAN_POINT('Ctrl Pts',(-8.15385625005417,12.2,7.53703765963208));
#243846=CARTESIAN_POINT('Ctrl Pts',(-8.15196980026671,12.2,7.53314575936217));
#243847=CARTESIAN_POINT('Ctrl Pts',(-8.15008306742096,12.2,7.52926907156699));
#243848=CARTESIAN_POINT('Ctrl Pts',(-8.14819633431816,12.2,7.52539238324361));
#243849=CARTESIAN_POINT('Ctrl Pts',(-8.14630931581502,12.2,7.5215309085201));
#243850=CARTESIAN_POINT('Ctrl Pts',(-8.14442212145121,12.2,7.51768469867524));
#243851=CARTESIAN_POINT('Ctrl Pts',(-8.14253492734454,12.2,7.51383848935443));
#243852=CARTESIAN_POINT('Ctrl Pts',(-8.14064755651672,12.2,7.51000754587886));
#243853=CARTESIAN_POINT('Ctrl Pts',(-8.13876011767102,12.2,7.50619191807866));
#243854=CARTESIAN_POINT('Ctrl Pts',(-8.13687267856815,12.2,7.50237628975859));
#243855=CARTESIAN_POINT('Ctrl Pts',(-8.13498517114307,12.2,7.49857597819037));
#243856=CARTESIAN_POINT('Ctrl Pts',(-8.13309770359576,12.2,7.49479103320733));
#243857=CARTESIAN_POINT('Ctrl Pts',(-8.13121023630563,12.2,7.49100608873999));
#243858=CARTESIAN_POINT('Ctrl Pts',(-8.12932280973336,12.2,7.48723651203785));
#243859=CARTESIAN_POINT('Ctrl Pts',(-8.12743553551558,12.2,7.48348235404476));
#243860=CARTESIAN_POINT('Ctrl Pts',(-8.1250764425505,12.2,7.47878965616977));
#243861=CARTESIAN_POINT('Ctrl Pts',(-8.12271758505987,12.2,7.47412105057175));
#243862=CARTESIAN_POINT('Ctrl Pts',(-8.12035918242096,12.2,7.46947663702881));
#243863=CARTESIAN_POINT('Ctrl Pts',(-8.118472460207,12.2,7.46576110599196));
#243864=CARTESIAN_POINT('Ctrl Pts',(-8.11658602982086,12.2,7.46206105888477));
#243865=CARTESIAN_POINT('Ctrl Pts',(-8.11470000282921,12.2,7.45837654540719));
#243866=CARTESIAN_POINT('Ctrl Pts',(-8.11281397609452,12.2,7.45469203243164));
#243867=CARTESIAN_POINT('Ctrl Pts',(-8.11092835204705,12.2,7.45102305610424));
#243868=CARTESIAN_POINT('Ctrl Pts',(-8.10904324777359,12.2,7.44736966533013));
#243869=CARTESIAN_POINT('Ctrl Pts',(-8.10668686723912,12.2,7.44280292648915));
#243870=CARTESIAN_POINT('Ctrl Pts',(-8.10433129348742,12.2,7.43826054076349));
#243871=CARTESIAN_POINT('Ctrl Pts',(-8.10197675661237,12.2,7.43374261055386));
#243872=CARTESIAN_POINT('Ctrl Pts',(-8.10009312700967,12.2,7.43012826618918));
#243873=CARTESIAN_POINT('Ctrl Pts',(-8.09821015917093,12.2,7.42652957264305));
#243874=CARTESIAN_POINT('Ctrl Pts',(-8.0963279708462,12.2,7.42294658294883));
#243875=CARTESIAN_POINT('Ctrl Pts',(-8.0944457827779,12.2,7.41936359374279));
#243876=CARTESIAN_POINT('Ctrl Pts',(-8.09256437305387,12.2,7.41579630768909));
#243877=CARTESIAN_POINT('Ctrl Pts',(-8.09068386054085,12.2,7.41224477658894));
#243878=CARTESIAN_POINT('Ctrl Pts',(-8.08880334777161,12.2,7.4086932450049));
#243879=CARTESIAN_POINT('Ctrl Pts',(-8.08692373280415,12.2,7.40515746903032));
#243880=CARTESIAN_POINT('Ctrl Pts',(-8.08504513324877,12.2,7.40163749998919));
#243881=CARTESIAN_POINT('Ctrl Pts',(-8.08269688393254,12.2,7.39723753892757));
#243882=CARTESIAN_POINT('Ctrl Pts',(-8.08035022280215,12.2,7.39286227676422));
#243883=CARTESIAN_POINT('Ctrl Pts',(-8.07800538433004,12.2,7.38851181572388));
#243884=CARTESIAN_POINT('Ctrl Pts',(-8.0761295137057,12.2,7.38503144717613));
#243885=CARTESIAN_POINT('Ctrl Pts',(-8.07425481035335,12.2,7.38156695150017));
#243886=CARTESIAN_POINT('Ctrl Pts',(-8.07238139583969,12.2,7.37811837978044));
#243887=CARTESIAN_POINT('Ctrl Pts',(-8.07050798107078,12.2,7.37466980759083));
#243888=CARTESIAN_POINT('Ctrl Pts',(-8.06863585405367,12.2,7.37123716097705));
#243889=CARTESIAN_POINT('Ctrl Pts',(-8.06676514049878,12.2,7.3678204919976));
#243890=CARTESIAN_POINT('Ctrl Pts',(-8.06489442719877,12.2,7.36440382348368));
#243891=CARTESIAN_POINT('Ctrl Pts',(-8.06302512532789,12.2,7.36100313198659));
#243892=CARTESIAN_POINT('Ctrl Pts',(-8.06115736131376,12.2,7.35761847076166));
#243893=CARTESIAN_POINT('Ctrl Pts',(-8.05928959704514,12.2,7.35423380907556));
#243894=CARTESIAN_POINT('Ctrl Pts',(-8.05742336892112,12.2,7.35086517720208));
#243895=CARTESIAN_POINT('Ctrl Pts',(-8.05555880354172,12.2,7.34751262874158));
#243896=CARTESIAN_POINT('Ctrl Pts',(-8.05369423816231,12.2,7.34416008028108));
#243897=CARTESIAN_POINT('Ctrl Pts',(-8.05183133539423,12.2,7.34082361326415));
#243898=CARTESIAN_POINT('Ctrl Pts',(-8.04997022323743,12.2,7.33750328297372));
#243899=CARTESIAN_POINT('Ctrl Pts',(-8.0481091113342,12.2,7.3341829531357));
#243900=CARTESIAN_POINT('Ctrl Pts',(-8.04624978891069,12.2,7.33087875821226));
#243901=CARTESIAN_POINT('Ctrl Pts',(-8.04439238577632,12.2,7.32759075174384));
#243902=CARTESIAN_POINT('Ctrl Pts',(-8.04253498238886,12.2,7.32430274482742));
#243903=CARTESIAN_POINT('Ctrl Pts',(-8.04067949797838,12.2,7.32103092732398));
#243904=CARTESIAN_POINT('Ctrl Pts',(-8.03882606248868,12.2,7.31777535042598));
#243905=CARTESIAN_POINT('Ctrl Pts',(-8.03697262725152,12.2,7.31451977397156));
#243906=CARTESIAN_POINT('Ctrl Pts',(-8.03512123971688,12.2,7.31128043907337));
#243907=CARTESIAN_POINT('Ctrl Pts',(-8.03327203386791,12.2,7.30805739978022));
#243908=CARTESIAN_POINT('Ctrl Pts',(-8.03142282776697,12.2,7.30483436004793));
#243909=CARTESIAN_POINT('Ctrl Pts',(-8.02957580224709,12.2,7.30162761399944));
#243910=CARTESIAN_POINT('Ctrl Pts',(-8.02773108949905,12.2,7.29843721627873));
#243911=CARTESIAN_POINT('Ctrl Pts',(-8.02588637700236,12.2,7.29524681899272));
#243912=CARTESIAN_POINT('Ctrl Pts',(-8.02404397811968,12.2,7.29207277041229));
#243913=CARTESIAN_POINT('Ctrl Pts',(-8.02220402765882,12.2,7.28891512322488));
#243914=CARTESIAN_POINT('Ctrl Pts',(-8.02036407694725,12.2,7.28575747560723));
#243915=CARTESIAN_POINT('Ctrl Pts',(-8.01852657364991,12.2,7.28261623021387));
#243916=CARTESIAN_POINT('Ctrl Pts',(-8.0166916548834,12.2,7.2794914387113));
#243917=CARTESIAN_POINT('Ctrl Pts',(-8.01485673636691,12.2,7.27636664763448));
#243918=CARTESIAN_POINT('Ctrl Pts',(-8.0130244005104,12.2,7.27325831326569));
#243919=CARTESIAN_POINT('Ctrl Pts',(-8.01119478729054,12.2,7.27016648664032));
#243920=CARTESIAN_POINT('Ctrl Pts',(-8.0093651738214,12.2,7.26707465959368));
#243921=CARTESIAN_POINT('Ctrl Pts',(-8.0075382814224,12.2,7.26399934282954));
#243922=CARTESIAN_POINT('Ctrl Pts',(-8.00571425010096,12.2,7.26094058727503));
#243923=CARTESIAN_POINT('Ctrl Pts',(-8.00389021902804,12.2,7.25788183213727));
#243924=CARTESIAN_POINT('Ctrl Pts',(-8.00206904825732,12.2,7.25483964111564));
#243925=CARTESIAN_POINT('Ctrl Pts',(-8.00025087857232,12.2,7.25181406602794));
#243926=CARTESIAN_POINT('Ctrl Pts',(-7.99843270863958,12.2,7.248788490528));
#243927=CARTESIAN_POINT('Ctrl Pts',(-7.99661754134745,12.2,7.24577953161895));
#243928=CARTESIAN_POINT('Ctrl Pts',(-7.99480551674048,12.2,7.24278724399789));
#243929=CARTESIAN_POINT('Ctrl Pts',(-7.99299349238039,12.2,7.23979495678451));
#243930=CARTESIAN_POINT('Ctrl Pts',(-7.99118461129244,12.2,7.23681934085188));
#243931=CARTESIAN_POINT('Ctrl Pts',(-7.9893790183286,12.2,7.23386045025871));
#243932=CARTESIAN_POINT('Ctrl Pts',(-7.98757342511873,12.2,7.23090155926239));
#243933=CARTESIAN_POINT('Ctrl Pts',(-7.98577112047308,12.2,7.22795939382046));
#243934=CARTESIAN_POINT('Ctrl Pts',(-7.98397224854171,12.2,7.2250340082166));
#243935=CARTESIAN_POINT('Ctrl Pts',(-7.98217337661035,12.2,7.22210862261273));
#243936=CARTESIAN_POINT('Ctrl Pts',(-7.98037793865436,12.2,7.21920001571076));
#243937=CARTESIAN_POINT('Ctrl Pts',(-7.97858608022374,12.2,7.21630824477712));
#243938=CARTESIAN_POINT('Ctrl Pts',(-7.97679422203727,12.2,7.21341647423748));
#243939=CARTESIAN_POINT('Ctrl Pts',(-7.97500594488848,12.2,7.2105415382118));
#243940=CARTESIAN_POINT('Ctrl Pts',(-7.97322139852626,12.2,7.20768349104354));
#243941=CARTESIAN_POINT('Ctrl Pts',(-7.9714368519209,12.2,7.20482544348586));
#243942=CARTESIAN_POINT('Ctrl Pts',(-7.96965603490598,12.2,7.20198428469316));
#243943=CARTESIAN_POINT('Ctrl Pts',(-7.96787909847618,12.2,7.19916007226317));
#243944=CARTESIAN_POINT('Ctrl Pts',(-7.96565792805999,12.2,7.19562980691809));
#243945=CARTESIAN_POINT('Ctrl Pts',(-7.96344282182177,12.2,7.19212601567076));
#243946=CARTESIAN_POINT('Ctrl Pts',(-7.96123407946114,12.2,7.18864880810345));
#243947=CARTESIAN_POINT('Ctrl Pts',(-7.95902533734128,12.2,7.18517160091515));
#243948=CARTESIAN_POINT('Ctrl Pts',(-7.9568229566151,12.2,7.18172097653783));
#243949=CARTESIAN_POINT('Ctrl Pts',(-7.95462724227057,12.2,7.17829704517277));
#243950=CARTESIAN_POINT('Ctrl Pts',(-7.95243152768672,12.2,7.17487311343451));
#243951=CARTESIAN_POINT('Ctrl Pts',(-7.95024247975272,12.2,7.17147587319856));
#243952=CARTESIAN_POINT('Ctrl Pts',(-7.94806040600212,12.2,7.16810543389078));
#243953=CARTESIAN_POINT('Ctrl Pts',(-7.94587833225154,12.2,7.164734994583));
#243954=CARTESIAN_POINT('Ctrl Pts',(-7.94370323307863,12.2,7.1613913551804));
#243955=CARTESIAN_POINT('Ctrl Pts',(-7.94153542175859,12.2,7.15807462594209));
#243956=CARTESIAN_POINT('Ctrl Pts',(-7.93806692369378,12.2,7.15276785923307));
#243957=CARTESIAN_POINT('Ctrl Pts',(-7.93461707823475,12.2,7.14752998137508));
#243958=CARTESIAN_POINT('Ctrl Pts',(-7.93118719628043,12.2,7.14236144266412));
#243959=CARTESIAN_POINT('Ctrl Pts',(-7.92904352002977,12.2,7.13913110592575));
#243960=CARTESIAN_POINT('Ctrl Pts',(-7.92690764254568,12.2,7.13592785524537));
#243961=CARTESIAN_POINT('Ctrl Pts',(-7.92477988900335,12.2,7.13275180017369));
#243962=CARTESIAN_POINT('Ctrl Pts',(-7.922652135461,12.2,7.129575745102));
#243963=CARTESIAN_POINT('Ctrl Pts',(-7.92053250761231,12.2,7.12642688654244));
#243964=CARTESIAN_POINT('Ctrl Pts',(-7.91842133472847,12.2,7.12330533541238));
#243965=CARTESIAN_POINT('Ctrl Pts',(-7.91631016184464,12.2,7.12018378428232));
#243966=CARTESIAN_POINT('Ctrl Pts',(-7.91420744539304,12.2,7.11708953951319));
#243967=CARTESIAN_POINT('Ctrl Pts',(-7.91211352108703,12.2,7.11402271444232));
#243968=CARTESIAN_POINT('Ctrl Pts',(-7.91001959678102,12.2,7.11095588937146));
#243969=CARTESIAN_POINT('Ctrl Pts',(-7.90793446711411,12.2,7.10791648394849));
#243970=CARTESIAN_POINT('Ctrl Pts',(-7.90585847037751,12.2,7.10490460894705));
#243971=CARTESIAN_POINT('Ctrl Pts',(-7.90378247364092,12.2,7.1018927339456));
#243972=CARTESIAN_POINT('Ctrl Pts',(-7.90171561457166,12.2,7.09890838983727));
#243973=CARTESIAN_POINT('Ctrl Pts',(-7.89965823699282,12.2,7.0959516905182));
#243974=CARTESIAN_POINT('Ctrl Pts',(-7.897600859414,12.2,7.09299499119913));
#243975=CARTESIAN_POINT('Ctrl Pts',(-7.89555296451672,12.2,7.09006593653882));
#243976=CARTESIAN_POINT('Ctrl Pts',(-7.89351490847503,12.2,7.08716463827492));
#243977=CARTESIAN_POINT('Ctrl Pts',(-7.89147685243335,12.2,7.08426334001101));
#243978=CARTESIAN_POINT('Ctrl Pts',(-7.88944863350252,12.2,7.08138980059456));
#243979=CARTESIAN_POINT('Ctrl Pts',(-7.88743061175726,12.2,7.07854413224837));
#243980=CARTESIAN_POINT('Ctrl Pts',(-7.88541259001201,12.2,7.07569846390218));
#243981=CARTESIAN_POINT('Ctrl Pts',(-7.88340476471337,12.2,7.07288066627728));
#243982=CARTESIAN_POINT('Ctrl Pts',(-7.88140750464447,12.2,7.0700908568343));
#243983=CARTESIAN_POINT('Ctrl Pts',(-7.87941024457558,12.2,7.06730104739132));
#243984=CARTESIAN_POINT('Ctrl Pts',(-7.87742354804253,12.2,7.06453922371985));
#243985=CARTESIAN_POINT('Ctrl Pts',(-7.87544778811255,12.2,7.06180550205463));
#243986=CARTESIAN_POINT('Ctrl Pts',(-7.87347202818255,12.2,7.05907178038943));
#243987=CARTESIAN_POINT('Ctrl Pts',(-7.8715072057701,12.2,7.05636616173211));
#243988=CARTESIAN_POINT('Ctrl Pts',(-7.86955369754829,12.2,7.05368876069754));
#243989=CARTESIAN_POINT('Ctrl Pts',(-7.8672094877673,12.2,7.05047587957279));
#243990=CARTESIAN_POINT('Ctrl Pts',(-7.86488157480772,12.2,7.04730363264447));
#243991=CARTESIAN_POINT('Ctrl Pts',(-7.86257062397502,12.2,7.04417222350824));
#243992=CARTESIAN_POINT('Ctrl Pts',(-7.86025967314232,12.2,7.04104081437201));
#243993=CARTESIAN_POINT('Ctrl Pts',(-7.85796568526065,12.2,7.03795024112229));
#243994=CARTESIAN_POINT('Ctrl Pts',(-7.85568934347861,12.2,7.03490070907836));
#243995=CARTESIAN_POINT('Ctrl Pts',(-7.85341300148981,12.2,7.03185117675743));
#243996=CARTESIAN_POINT('Ctrl Pts',(-7.85115430702667,12.2,7.02884268435205));
#243997=CARTESIAN_POINT('Ctrl Pts',(-7.84891395623916,12.2,7.02587543919316));
#243998=CARTESIAN_POINT('Ctrl Pts',(-7.84667360565515,12.2,7.02290819430378));
#243999=CARTESIAN_POINT('Ctrl Pts',(-7.84445160067892,12.2,7.01998219575677));
#244000=CARTESIAN_POINT('Ctrl Pts',(-7.84224865324902,12.2,7.01709765168194));
#244001=CARTESIAN_POINT('Ctrl Pts',(-7.84004570581913,12.2,7.0142131076071));
#244002=CARTESIAN_POINT('Ctrl Pts',(-7.83786181919861,12.2,7.01137001650279));
#244003=CARTESIAN_POINT('Ctrl Pts',(-7.83569771985971,12.2,7.00856858960276));
#244004=CARTESIAN_POINT('Ctrl Pts',(-7.83353362032424,12.2,7.00576716244827));
#244005=CARTESIAN_POINT('Ctrl Pts',(-7.83138931029956,12.2,7.00300739883229));
#244006=CARTESIAN_POINT('Ctrl Pts',(-7.82926553851853,12.2,7.000289509687));
#244007=CARTESIAN_POINT('Ctrl Pts',(-7.82714176693041,12.2,6.9975716207886));
#244008=CARTESIAN_POINT('Ctrl Pts',(-7.82503852973505,12.2,6.99489560841732));
#244009=CARTESIAN_POINT('Ctrl Pts',(-7.82295659539498,12.2,6.99226168259821));
#244010=CARTESIAN_POINT('Ctrl Pts',(-7.82087466105491,12.2,6.98962775677911));
#244011=CARTESIAN_POINT('Ctrl Pts',(-7.81881402959643,12.2,6.98703591994823));
#244012=CARTESIAN_POINT('Ctrl Pts',(-7.81677548158621,12.2,6.98448638787237));
#244013=CARTESIAN_POINT('Ctrl Pts',(-7.81473693339083,12.2,6.98193685556494));
#244014=CARTESIAN_POINT('Ctrl Pts',(-7.81272047252316,12.2,6.97942962570439));
#244015=CARTESIAN_POINT('Ctrl Pts',(-7.81072689908272,12.2,6.9769649194896));
#244016=CARTESIAN_POINT('Ctrl Pts',(-7.80873332582335,12.2,6.97450021349869));
#244017=CARTESIAN_POINT('Ctrl Pts',(-7.80676263884723,12.2,6.97207803038208));
#244018=CARTESIAN_POINT('Ctrl Pts',(-7.80481566366901,12.2,6.96969858863709));
#244019=CARTESIAN_POINT('Ctrl Pts',(-7.80286868849079,12.2,6.96731914689208));
#244020=CARTESIAN_POINT('Ctrl Pts',(-7.800945421744,12.2,6.96498244829361));
#244021=CARTESIAN_POINT('Ctrl Pts',(-7.79904671156193,12.2,6.9626887163751));
#244022=CARTESIAN_POINT('Ctrl Pts',(-7.79714800137986,12.2,6.96039498445658));
#244023=CARTESIAN_POINT('Ctrl Pts',(-7.79527384169444,12.2,6.95814421811329));
#244024=CARTESIAN_POINT('Ctrl Pts',(-7.79342510367653,12.2,6.95593664319055));
#244025=CARTESIAN_POINT('Ctrl Pts',(-7.79157636549069,12.2,6.95372906806728));
#244026=CARTESIAN_POINT('Ctrl Pts',(-7.78975304394064,12.2,6.95156468542317));
#244027=CARTESIAN_POINT('Ctrl Pts',(-7.78795602992718,12.2,6.9494437215595));
#244028=CARTESIAN_POINT('Ctrl Pts',(-7.78615901607696,12.2,6.94732275788846));
#244029=CARTESIAN_POINT('Ctrl Pts',(-7.78438830853713,12.2,6.9452452166113));
#244030=CARTESIAN_POINT('Ctrl Pts',(-7.78264481700914,12.2,6.94321132675917));
#244031=CARTESIAN_POINT('Ctrl Pts',(-7.78090132548115,12.2,6.94117743690704));
#244032=CARTESIAN_POINT('Ctrl Pts',(-7.77918505249957,12.2,6.93918720018598));
#244033=CARTESIAN_POINT('Ctrl Pts',(-7.77749693197569,12.2,6.93724084850374));
#244034=CARTESIAN_POINT('Ctrl Pts',(-7.77580881129846,12.2,6.93529449664471));
#244035=CARTESIAN_POINT('Ctrl Pts',(-7.77414884352764,12.2,6.93339203265347));
#244036=CARTESIAN_POINT('Ctrl Pts',(-7.77251798985898,12.2,6.93153369454525));
#244037=CARTESIAN_POINT('Ctrl Pts',(-7.77088713633846,12.2,6.92967535660584));
#244038=CARTESIAN_POINT('Ctrl Pts',(-7.7692853965429,12.2,6.92786114359393));
#244039=CARTESIAN_POINT('Ctrl Pts',(-7.76771376026667,12.2,6.92609129774157));
#244040=CARTESIAN_POINT('Ctrl Pts',(-7.76614212399044,12.2,6.92432145188921));
#244041=CARTESIAN_POINT('Ctrl Pts',(-7.76460059048524,12.2,6.92259597378809));
#244042=CARTESIAN_POINT('Ctrl Pts',(-7.76309017712953,12.2,6.92091510792929));
#244043=CARTESIAN_POINT('Ctrl Pts',(-7.76157976363662,12.2,6.91923424191781));
#244044=CARTESIAN_POINT('Ctrl Pts',(-7.76010047016895,12.2,6.91759798963515));
#244045=CARTESIAN_POINT('Ctrl Pts',(-7.75865334209226,12.2,6.91600659963478));
#244046=CARTESIAN_POINT('Ctrl Pts',(-7.75720621414701,12.2,6.91441520977898));
#244047=CARTESIAN_POINT('Ctrl Pts',(-7.75579125177202,12.2,6.91286868171804));
#244048=CARTESIAN_POINT('Ctrl Pts',(-7.75440953381604,12.2,6.9113672717659));
#244049=CARTESIAN_POINT('Ctrl Pts',(-7.75302781586007,12.2,6.90986586181377));
#244050=CARTESIAN_POINT('Ctrl Pts',(-7.75167934028384,12.2,6.90840956728605));
#244051=CARTESIAN_POINT('Ctrl Pts',(-7.75036521958009,12.2,6.90699864858533));
#244052=CARTESIAN_POINT('Ctrl Pts',(-7.74883838549972,12.2,6.90535934806235));
#244053=CARTESIAN_POINT('Ctrl Pts',(-7.74735792437416,12.2,6.90378129525211));
#244054=CARTESIAN_POINT('Ctrl Pts',(-7.74592563800006,12.2,6.90226491999999));
#244055=CARTESIAN_POINT('Ctrl Pts',(-7.74592563800006,15.2,6.90226491999999));
#244056=CARTESIAN_POINT('Ctrl Pts',(-7.74715246678865,15.2,6.90356377534571));
#244057=CARTESIAN_POINT('Ctrl Pts',(-7.74841464217223,15.2,6.90490788340064));
#244058=CARTESIAN_POINT('Ctrl Pts',(-7.74971102733301,15.2,6.90629697133944));
#244059=CARTESIAN_POINT('Ctrl Pts',(-7.75101366431833,15.2,6.90769275816243));
#244060=CARTESIAN_POINT('Ctrl Pts',(-7.75235084435424,15.2,6.90913396283592));
#244061=CARTESIAN_POINT('Ctrl Pts',(-7.75372145033267,15.2,6.91062032766048));
#244062=CARTESIAN_POINT('Ctrl Pts',(-7.75532049045411,15.2,6.91235441975326));
#244063=CARTESIAN_POINT('Ctrl Pts',(-7.75696502619996,15.2,6.91414997818454));
#244064=CARTESIAN_POINT('Ctrl Pts',(-7.75865334209227,15.2,6.91600659963479));
#244065=CARTESIAN_POINT('Ctrl Pts',(-7.76010047016897,15.2,6.91759798963517));
#244066=CARTESIAN_POINT('Ctrl Pts',(-7.7615797636366,15.2,6.91923424191777));
#244067=CARTESIAN_POINT('Ctrl Pts',(-7.76309017712953,15.2,6.92091510792929));
#244068=CARTESIAN_POINT('Ctrl Pts',(-7.76460059048527,15.2,6.92259597378812));
#244069=CARTESIAN_POINT('Ctrl Pts',(-7.76614212399043,15.2,6.9243214518892));
#244070=CARTESIAN_POINT('Ctrl Pts',(-7.76771376026667,15.2,6.92609129774157));
#244071=CARTESIAN_POINT('Ctrl Pts',(-7.76928539654291,15.2,6.92786114359394));
#244072=CARTESIAN_POINT('Ctrl Pts',(-7.77088713633845,15.2,6.92967535660582));
#244073=CARTESIAN_POINT('Ctrl Pts',(-7.77251798985898,15.2,6.93153369454525));
#244074=CARTESIAN_POINT('Ctrl Pts',(-7.77414884352765,15.2,6.93339203265348));
#244075=CARTESIAN_POINT('Ctrl Pts',(-7.77580881129845,15.2,6.93529449664469));
#244076=CARTESIAN_POINT('Ctrl Pts',(-7.77749693197568,15.2,6.93724084850373));
#244077=CARTESIAN_POINT('Ctrl Pts',(-7.77918505249957,15.2,6.93918720018598));
#244078=CARTESIAN_POINT('Ctrl Pts',(-7.78090132548116,15.2,6.94117743690705));
#244079=CARTESIAN_POINT('Ctrl Pts',(-7.78264481700914,15.2,6.94321132675917));
#244080=CARTESIAN_POINT('Ctrl Pts',(-7.78438830853712,15.2,6.94524521661129));
#244081=CARTESIAN_POINT('Ctrl Pts',(-7.78615901607696,15.2,6.94732275788845));
#244082=CARTESIAN_POINT('Ctrl Pts',(-7.78795602992718,15.2,6.9494437215595));
#244083=CARTESIAN_POINT('Ctrl Pts',(-7.78975304394065,15.2,6.95156468542318));
#244084=CARTESIAN_POINT('Ctrl Pts',(-7.79157636549068,15.2,6.95372906806727));
#244085=CARTESIAN_POINT('Ctrl Pts',(-7.79342510367653,15.2,6.95593664319054));
#244086=CARTESIAN_POINT('Ctrl Pts',(-7.79527384169445,15.2,6.9581442181133));
#244087=CARTESIAN_POINT('Ctrl Pts',(-7.79714800137984,15.2,6.96039498445656));
#244088=CARTESIAN_POINT('Ctrl Pts',(-7.79904671156193,15.2,6.9626887163751));
#244089=CARTESIAN_POINT('Ctrl Pts',(-7.80094542174402,15.2,6.96498244829363));
#244090=CARTESIAN_POINT('Ctrl Pts',(-7.80286868849078,15.2,6.96731914689208));
#244091=CARTESIAN_POINT('Ctrl Pts',(-7.804815663669,15.2,6.96969858863707));
#244092=CARTESIAN_POINT('Ctrl Pts',(-7.80676263884721,15.2,6.97207803038206));
#244093=CARTESIAN_POINT('Ctrl Pts',(-7.80873332582338,15.2,6.97450021349873));
#244094=CARTESIAN_POINT('Ctrl Pts',(-7.81072689908272,15.2,6.9769649194896));
#244095=CARTESIAN_POINT('Ctrl Pts',(-7.81272047252313,15.2,6.97942962570435));
#244096=CARTESIAN_POINT('Ctrl Pts',(-7.81473693339078,15.2,6.98193685556488));
#244097=CARTESIAN_POINT('Ctrl Pts',(-7.81677548158621,15.2,6.98448638787237));
#244098=CARTESIAN_POINT('Ctrl Pts',(-7.81881402959647,15.2,6.98703591994829));
#244099=CARTESIAN_POINT('Ctrl Pts',(-7.82087466105487,15.2,6.98962775677906));
#244100=CARTESIAN_POINT('Ctrl Pts',(-7.82295659539498,15.2,6.99226168259821));
#244101=CARTESIAN_POINT('Ctrl Pts',(-7.82503852973509,15.2,6.99489560841737));
#244102=CARTESIAN_POINT('Ctrl Pts',(-7.82714176693043,15.2,6.99757162078863));
#244103=CARTESIAN_POINT('Ctrl Pts',(-7.82926553851854,15.2,7.00028950968701));
#244104=CARTESIAN_POINT('Ctrl Pts',(-7.83138931029955,15.2,7.00300739883227));
#244105=CARTESIAN_POINT('Ctrl Pts',(-7.83353362032421,15.2,7.00576716244823));
#244106=CARTESIAN_POINT('Ctrl Pts',(-7.83569771985971,15.2,7.00856858960276));
#244107=CARTESIAN_POINT('Ctrl Pts',(-7.83786181919864,15.2,7.01137001650283));
#244108=CARTESIAN_POINT('Ctrl Pts',(-7.84004570581912,15.2,7.0142131076071));
#244109=CARTESIAN_POINT('Ctrl Pts',(-7.84224865324903,15.2,7.01709765168194));
#244110=CARTESIAN_POINT('Ctrl Pts',(-7.84445160067893,15.2,7.01998219575679));
#244111=CARTESIAN_POINT('Ctrl Pts',(-7.84667360565514,15.2,7.02290819430377));
#244112=CARTESIAN_POINT('Ctrl Pts',(-7.84891395623916,15.2,7.02587543919316));
#244113=CARTESIAN_POINT('Ctrl Pts',(-7.85115430702668,15.2,7.02884268435206));
#244114=CARTESIAN_POINT('Ctrl Pts',(-7.8534130014898,15.2,7.03185117675742));
#244115=CARTESIAN_POINT('Ctrl Pts',(-7.85568934347861,15.2,7.03490070907836));
#244116=CARTESIAN_POINT('Ctrl Pts',(-7.85796568526066,15.2,7.0379502411223));
#244117=CARTESIAN_POINT('Ctrl Pts',(-7.86025967314234,15.2,7.04104081437204));
#244118=CARTESIAN_POINT('Ctrl Pts',(-7.86257062397502,15.2,7.04417222350824));
#244119=CARTESIAN_POINT('Ctrl Pts',(-7.8648815748077,15.2,7.04730363264444));
#244120=CARTESIAN_POINT('Ctrl Pts',(-7.86720948776729,15.2,7.05047587957277));
#244121=CARTESIAN_POINT('Ctrl Pts',(-7.86955369754829,15.2,7.05368876069754));
#244122=CARTESIAN_POINT('Ctrl Pts',(-7.87150720577011,15.2,7.05636616173213));
#244123=CARTESIAN_POINT('Ctrl Pts',(-7.87347202818256,15.2,7.05907178038944));
#244124=CARTESIAN_POINT('Ctrl Pts',(-7.87544778811255,15.2,7.06180550205465));
#244125=CARTESIAN_POINT('Ctrl Pts',(-7.87742354804254,15.2,7.06453922371986));
#244126=CARTESIAN_POINT('Ctrl Pts',(-7.87941024457559,15.2,7.06730104739134));
#244127=CARTESIAN_POINT('Ctrl Pts',(-7.88140750464447,15.2,7.07009085683429));
#244128=CARTESIAN_POINT('Ctrl Pts',(-7.88420366878443,15.2,7.07399659011525));
#244129=CARTESIAN_POINT('Ctrl Pts',(-7.88702053880993,15.2,7.0779571785731));
#244130=CARTESIAN_POINT('Ctrl Pts',(-7.8898571093826,15.2,7.08197230513765));
#244131=CARTESIAN_POINT('Ctrl Pts',(-7.89228845546155,15.2,7.08541384201434));
#244132=CARTESIAN_POINT('Ctrl Pts',(-7.89473427728936,15.2,7.08889544834617));
#244133=CARTESIAN_POINT('Ctrl Pts',(-7.89719395836603,15.2,7.09241692729982));
#244134=CARTESIAN_POINT('Ctrl Pts',(-7.89924369267107,15.2,7.09535149320116));
#244135=CARTESIAN_POINT('Ctrl Pts',(-7.90130305046732,15.2,7.09831374891258));
#244136=CARTESIAN_POINT('Ctrl Pts',(-7.90337168228224,15.2,7.10130358073163));
#244137=CARTESIAN_POINT('Ctrl Pts',(-7.90585404036996,15.2,7.10489137878413));
#244138=CARTESIAN_POINT('Ctrl Pts',(-7.90834975301863,15.2,7.10851888697784));
#244139=CARTESIAN_POINT('Ctrl Pts',(-7.91085822425995,15.2,7.11218591009188));
#244140=CARTESIAN_POINT('Ctrl Pts',(-7.91336669572912,15.2,7.11585293353903));
#244141=CARTESIAN_POINT('Ctrl Pts',(-7.91588792712977,15.2,7.11955947385212));
#244142=CARTESIAN_POINT('Ctrl Pts',(-7.91842133472847,15.2,7.12330533541238));
#244143=CARTESIAN_POINT('Ctrl Pts',(-7.92137697658178,15.2,7.12767550672231));
#244144=CARTESIAN_POINT('Ctrl Pts',(-7.9243491910579,15.2,7.13209920094139));
#244145=CARTESIAN_POINT('Ctrl Pts',(-7.92733707145422,15.2,7.13657611258999));
#244146=CARTESIAN_POINT('Ctrl Pts',(-7.93032495208318,15.2,7.14105302458716));
#244147=CARTESIAN_POINT('Ctrl Pts',(-7.93332850016596,15.2,7.14558315465606));
#244148=CARTESIAN_POINT('Ctrl Pts',(-7.9363468282822,15.2,7.1501661985398));
#244149=CARTESIAN_POINT('Ctrl Pts',(-7.93850277690308,15.2,7.15343980126294));
#244150=CARTESIAN_POINT('Ctrl Pts',(-7.94066626605559,15.2,7.15674040271658));
#244151=CARTESIAN_POINT('Ctrl Pts',(-7.94283698050004,15.2,7.16006789125824));
#244152=CARTESIAN_POINT('Ctrl Pts',(-7.94544183773873,15.2,7.16406087736317));
#244153=CARTESIAN_POINT('Ctrl Pts',(-7.94805709806829,15.2,7.16809258302344));
#244154=CARTESIAN_POINT('Ctrl Pts',(-7.95068222172223,15.2,7.1721628180396));
#244155=CARTESIAN_POINT('Ctrl Pts',(-7.95286982484666,15.2,7.1755546806763));
#244156=CARTESIAN_POINT('Ctrl Pts',(-7.95506428048505,15.2,7.17897329923534));
#244157=CARTESIAN_POINT('Ctrl Pts',(-7.95726527871956,15.2,7.1824185678084));
#244158=CARTESIAN_POINT('Ctrl Pts',(-7.95946627695407,15.2,7.18586383638145));
#244159=CARTESIAN_POINT('Ctrl Pts',(-7.9616738201834,15.2,7.18933575325045));
#244160=CARTESIAN_POINT('Ctrl Pts',(-7.96388760636363,15.2,7.19283421005461));
#244161=CARTESIAN_POINT('Ctrl Pts',(-7.96654414992467,15.2,7.1970323584484));
#244162=CARTESIAN_POINT('Ctrl Pts',(-7.96920968180351,15.2,7.20126872410527));
#244163=CARTESIAN_POINT('Ctrl Pts',(-7.97188369053318,15.2,7.20554312342417));
#244164=CARTESIAN_POINT('Ctrl Pts',(-7.97366636277674,15.2,7.20839272258186));
#244165=CARTESIAN_POINT('Ctrl Pts',(-7.97545280215928,15.2,7.21125922460953));
#244166=CARTESIAN_POINT('Ctrl Pts',(-7.97724286046549,15.2,7.21414257449796));
#244167=CARTESIAN_POINT('Ctrl Pts',(-7.97903291901561,15.2,7.21702592477925));
#244168=CARTESIAN_POINT('Ctrl Pts',(-7.9808265943456,15.2,7.21992612363562));
#244169=CARTESIAN_POINT('Ctrl Pts',(-7.98262374077721,15.2,7.22284311651852));
#244170=CARTESIAN_POINT('Ctrl Pts',(-7.98442088696397,15.2,7.22576010900398));
#244171=CARTESIAN_POINT('Ctrl Pts',(-7.98622150212531,15.2,7.22869389298174));
#244172=CARTESIAN_POINT('Ctrl Pts',(-7.98802544181093,15.2,7.2316444180172));
#244173=CARTESIAN_POINT('Ctrl Pts',(-7.98982938174235,15.2,7.23459494345466));
#244174=CARTESIAN_POINT('Ctrl Pts',(-7.99163664624837,15.2,7.23756220719483));
#244175=CARTESIAN_POINT('Ctrl Pts',(-7.9934470902711,15.2,7.24054615567467));
#244176=CARTESIAN_POINT('Ctrl Pts',(-7.99525753404717,15.2,7.24353010374794));
#244177=CARTESIAN_POINT('Ctrl Pts',(-7.99707115614192,15.2,7.24653073700669));
#244178=CARTESIAN_POINT('Ctrl Pts',(-7.99888781582656,15.2,7.2495480002034));
#244179=CARTESIAN_POINT('Ctrl Pts',(-8.00115864061799,15.2,7.25331957950761));
#244180=CARTESIAN_POINT('Ctrl Pts',(-8.00343421107341,15.2,7.25711714304025));
#244181=CARTESIAN_POINT('Ctrl Pts',(-8.00571425010096,15.2,7.26094058727502));
#244182=CARTESIAN_POINT('Ctrl Pts',(-8.0075382814224,15.2,7.26399934282954));
#244183=CARTESIAN_POINT('Ctrl Pts',(-8.00936517382141,15.2,7.2670746595937));
#244184=CARTESIAN_POINT('Ctrl Pts',(-8.01119478729055,15.2,7.27016648664033));
#244185=CARTESIAN_POINT('Ctrl Pts',(-8.0130244005104,15.2,7.27325831326569));
#244186=CARTESIAN_POINT('Ctrl Pts',(-8.01485673636691,15.2,7.27636664763449));
#244187=CARTESIAN_POINT('Ctrl Pts',(-8.0166916548834,15.2,7.27949143871129));
#244188=CARTESIAN_POINT('Ctrl Pts',(-8.01852657364989,15.2,7.28261623021384));
#244189=CARTESIAN_POINT('Ctrl Pts',(-8.02036407694727,15.2,7.28575747560727));
#244190=CARTESIAN_POINT('Ctrl Pts',(-8.02220402765882,15.2,7.28891512322488));
#244191=CARTESIAN_POINT('Ctrl Pts',(-8.02404397811966,15.2,7.29207277041225));
#244192=CARTESIAN_POINT('Ctrl Pts',(-8.02588637700234,15.2,7.2952468189927));
#244193=CARTESIAN_POINT('Ctrl Pts',(-8.02773108949904,15.2,7.29843721627872));
#244194=CARTESIAN_POINT('Ctrl Pts',(-8.02957580224709,15.2,7.30162761399944));
#244195=CARTESIAN_POINT('Ctrl Pts',(-8.03142282776698,15.2,7.30483436004793));
#244196=CARTESIAN_POINT('Ctrl Pts',(-8.03327203386791,15.2,7.30805739978023));
#244197=CARTESIAN_POINT('Ctrl Pts',(-8.03512123971688,15.2,7.31128043907338));
#244198=CARTESIAN_POINT('Ctrl Pts',(-8.03697262725151,15.2,7.31451977397155));
#244199=CARTESIAN_POINT('Ctrl Pts',(-8.03882606248868,15.2,7.31777535042597));
#244200=CARTESIAN_POINT('Ctrl Pts',(-8.04067949797837,15.2,7.32103092732396));
#244201=CARTESIAN_POINT('Ctrl Pts',(-8.04253498238887,15.2,7.32430274482745));
#244202=CARTESIAN_POINT('Ctrl Pts',(-8.04439238577631,15.2,7.32759075174384));
#244203=CARTESIAN_POINT('Ctrl Pts',(-8.04624978891068,15.2,7.33087875821224));
#244204=CARTESIAN_POINT('Ctrl Pts',(-8.0481091113342,15.2,7.3341829531357));
#244205=CARTESIAN_POINT('Ctrl Pts',(-8.04997022323742,15.2,7.33750328297372));
#244206=CARTESIAN_POINT('Ctrl Pts',(-8.05183133539422,15.2,7.34082361326413));
#244207=CARTESIAN_POINT('Ctrl Pts',(-8.05369423816233,15.2,7.34416008028111));
#244208=CARTESIAN_POINT('Ctrl Pts',(-8.05555880354172,15.2,7.34751262874159));
#244209=CARTESIAN_POINT('Ctrl Pts',(-8.05742336892111,15.2,7.35086517720206));
#244210=CARTESIAN_POINT('Ctrl Pts',(-8.05928959704515,15.2,7.35423380907557));
#244211=CARTESIAN_POINT('Ctrl Pts',(-8.06115736131377,15.2,7.35761847076166));
#244212=CARTESIAN_POINT('Ctrl Pts',(-8.06302512532789,15.2,7.3610031319866));
#244213=CARTESIAN_POINT('Ctrl Pts',(-8.06489442719878,15.2,7.36440382348369));
#244214=CARTESIAN_POINT('Ctrl Pts',(-8.06676514049877,15.2,7.36782049199759));
#244215=CARTESIAN_POINT('Ctrl Pts',(-8.06863585405365,15.2,7.37123716097702));
#244216=CARTESIAN_POINT('Ctrl Pts',(-8.07050798107081,15.2,7.37466980759088));
#244217=CARTESIAN_POINT('Ctrl Pts',(-8.07238139583969,15.2,7.37811837978044));
#244218=CARTESIAN_POINT('Ctrl Pts',(-8.07425481035332,15.2,7.38156695150012));
#244219=CARTESIAN_POINT('Ctrl Pts',(-8.07612951370569,15.2,7.3850314471761));
#244220=CARTESIAN_POINT('Ctrl Pts',(-8.07800538433004,15.2,7.38851181572388));
#244221=CARTESIAN_POINT('Ctrl Pts',(-8.07988125520997,15.2,7.39199218474584));
#244222=CARTESIAN_POINT('Ctrl Pts',(-8.08175829209296,15.2,7.39548842611083));
#244223=CARTESIAN_POINT('Ctrl Pts',(-8.08363637628925,15.2,7.39900048853464));
#244224=CARTESIAN_POINT('Ctrl Pts',(-8.08598398140665,15.2,7.40339056632514));
#244225=CARTESIAN_POINT('Ctrl Pts',(-8.08833321970741,15.2,7.40780536235083));
#244226=CARTESIAN_POINT('Ctrl Pts',(-8.09068386054085,15.2,7.41224477658895));
#244227=CARTESIAN_POINT('Ctrl Pts',(-8.09256437305388,15.2,7.4157963076891));
#244228=CARTESIAN_POINT('Ctrl Pts',(-8.09444578277789,15.2,7.41936359374276));
#244229=CARTESIAN_POINT('Ctrl Pts',(-8.09632797084619,15.2,7.42294658294883));
#244230=CARTESIAN_POINT('Ctrl Pts',(-8.09821015917094,15.2,7.42652957264307));
#244231=CARTESIAN_POINT('Ctrl Pts',(-8.10009312700966,15.2,7.43012826618917));
#244232=CARTESIAN_POINT('Ctrl Pts',(-8.10197675661238,15.2,7.43374261055389));
#244233=CARTESIAN_POINT('Ctrl Pts',(-8.10386038595845,15.2,7.43735695442614));
#244234=CARTESIAN_POINT('Ctrl Pts',(-8.10574467825319,15.2,7.44098694880214));
#244235=CARTESIAN_POINT('Ctrl Pts',(-8.10762951752655,15.2,7.44463254396267));
#244236=CARTESIAN_POINT('Ctrl Pts',(-8.10951435705672,15.2,7.44827813961991));
#244237=CARTESIAN_POINT('Ctrl Pts',(-8.11139974215976,15.2,7.45193933322982));
#244238=CARTESIAN_POINT('Ctrl Pts',(-8.11328556042922,15.2,7.4556160750423));
#244239=CARTESIAN_POINT('Ctrl Pts',(-8.11517137844174,15.2,7.45929281635384));
#244240=CARTESIAN_POINT('Ctrl Pts',(-8.11705762817364,15.2,7.46298510618451));
#244241=CARTESIAN_POINT('Ctrl Pts',(-8.11894419690827,15.2,7.46669289193537));
#244242=CARTESIAN_POINT('Ctrl Pts',(-8.12083076589994,15.2,7.47040067819143));
#244243=CARTESIAN_POINT('Ctrl Pts',(-8.12271765509825,15.2,7.47412396060668));
#244244=CARTESIAN_POINT('Ctrl Pts',(-8.12460475070967,15.2,7.47786268699414));
#244245=CARTESIAN_POINT('Ctrl Pts',(-8.12649184606397,15.2,7.48160141287219));
#244246=CARTESIAN_POINT('Ctrl Pts',(-8.12837914802076,15.2,7.48535558376832));
#244247=CARTESIAN_POINT('Ctrl Pts',(-8.1302665466998,15.2,7.48912514762527));
#244248=CARTESIAN_POINT('Ctrl Pts',(-8.13215394563599,15.2,7.49289471199582));
#244249=CARTESIAN_POINT('Ctrl Pts',(-8.13404144064164,15.2,7.49667967021783));
#244250=CARTESIAN_POINT('Ctrl Pts',(-8.13592892096672,15.2,7.50047996925826));
#244251=CARTESIAN_POINT('Ctrl Pts',(-8.13876014119718,15.2,7.50618041730114));
#244252=CARTESIAN_POINT('Ctrl Pts',(-8.14159133016264,15.2,7.51191538443199));
#244253=CARTESIAN_POINT('Ctrl Pts',(-8.14442212145121,15.2,7.51768469867524));
#244254=CARTESIAN_POINT('Ctrl Pts',(-8.14630931581501,15.2,7.52153090852009));
#244255=CARTESIAN_POINT('Ctrl Pts',(-8.14819633431816,15.2,7.52539238324361));
#244256=CARTESIAN_POINT('Ctrl Pts',(-8.15008306742097,15.2,7.52926907156699));
#244257=CARTESIAN_POINT('Ctrl Pts',(-8.15196980026671,15.2,7.53314575936217));
#244258=CARTESIAN_POINT('Ctrl Pts',(-8.15385625005416,15.2,7.53703765963207));
#244259=CARTESIAN_POINT('Ctrl Pts',(-8.15574230940002,15.2,7.54094472464445));
#244260=CARTESIAN_POINT('Ctrl Pts',(-8.15762836900285,15.2,7.54485179018917));
#244261=CARTESIAN_POINT('Ctrl Pts',(-8.15951403872337,15.2,7.54877401690621));
#244262=CARTESIAN_POINT('Ctrl Pts',(-8.16139921250134,15.2,7.55271135652762));
#244263=CARTESIAN_POINT('Ctrl Pts',(-8.16328438602246,15.2,7.55664869561256));
#244264=CARTESIAN_POINT('Ctrl Pts',(-8.16516906521542,15.2,7.56060114599382));
#244265=CARTESIAN_POINT('Ctrl Pts',(-8.16705314345034,15.2,7.56456865833458));
#244266=CARTESIAN_POINT('Ctrl Pts',(-8.16893722194196,15.2,7.56853617121591));
#244267=CARTESIAN_POINT('Ctrl Pts',(-8.1708207022419,15.2,7.57251874412651));
#244268=CARTESIAN_POINT('Ctrl Pts',(-8.17270347923339,15.2,7.57651632723326));
#244269=CARTESIAN_POINT('Ctrl Pts',(-8.17458625622489,15.2,7.58051391034001));
#244270=CARTESIAN_POINT('Ctrl Pts',(-8.17646833147188,15.2,7.58452650448186));
#244271=CARTESIAN_POINT('Ctrl Pts',(-8.17834960057431,15.2,7.5885540569251));
#244272=CARTESIAN_POINT('Ctrl Pts',(-8.17976055227298,15.2,7.59157472098315));
#244273=CARTESIAN_POINT('Ctrl Pts',(-8.18117105078704,15.2,7.59460380014535));
#244274=CARTESIAN_POINT('Ctrl Pts',(-8.18258105455619,15.2,7.59764127235435));
#244275=CARTESIAN_POINT('Ctrl Pts',(-8.18446105949633,15.2,7.60169123511575));
#244276=CARTESIAN_POINT('Ctrl Pts',(-8.1863401841111,15.2,7.60575612029827));
#244277=CARTESIAN_POINT('Ctrl Pts',(-8.18821832684651,15.2,7.60983587490822));
#244278=CARTESIAN_POINT('Ctrl Pts',(-8.18962693396205,15.2,7.61289569100464));
#244279=CARTESIAN_POINT('Ctrl Pts',(-8.19103498854429,15.2,7.61596387304216));
#244280=CARTESIAN_POINT('Ctrl Pts',(-8.19244244970157,15.2,7.61904039805425));
#244281=CARTESIAN_POINT('Ctrl Pts',(-8.19384991111453,15.2,7.62211692362523));
#244282=CARTESIAN_POINT('Ctrl Pts',(-8.19525677885234,15.2,7.62520179237357));
#244283=CARTESIAN_POINT('Ctrl Pts',(-8.19666301030662,15.2,7.62829498390759));
#244284=CARTESIAN_POINT('Ctrl Pts',(-8.19806924150545,15.2,7.63138817487968));
#244285=CARTESIAN_POINT('Ctrl Pts',(-8.19947483650281,15.2,7.63448968842502));
#244286=CARTESIAN_POINT('Ctrl Pts',(-8.2008797547302,15.2,7.63759950209335));
#244287=CARTESIAN_POINT('Ctrl Pts',(-8.2022846729576,15.2,7.64070931576167));
#244288=CARTESIAN_POINT('Ctrl Pts',(-8.20368891343743,15.2,7.64382743018705));
#244289=CARTESIAN_POINT('Ctrl Pts',(-8.20509243563637,15.2,7.64695382511584));
#244290=CARTESIAN_POINT('Ctrl Pts',(-8.20743163938625,15.2,7.65216448351981));
#244291=CARTESIAN_POINT('Ctrl Pts',(-8.20976884746398,15.2,7.65739813918152));
#244292=CARTESIAN_POINT('Ctrl Pts',(-8.21210387114443,15.2,7.66265469758551));
#244293=CARTESIAN_POINT('Ctrl Pts',(-8.21350488530179,15.2,7.66580863251331));
#244294=CARTESIAN_POINT('Ctrl Pts',(-8.21490511257916,15.2,7.66897081202024));
#244295=CARTESIAN_POINT('Ctrl Pts',(-8.216304513243,15.2,7.67214121450282));
#244296=CARTESIAN_POINT('Ctrl Pts',(-8.21817038071004,15.2,7.67636841762092));
#244297=CARTESIAN_POINT('Ctrl Pts',(-8.2200347782726,15.2,7.68061023957843));
#244298=CARTESIAN_POINT('Ctrl Pts',(-8.22189760995382,15.2,7.68486663006234));
#244299=CARTESIAN_POINT('Ctrl Pts',(-8.223294734032,15.2,7.6880589236502));
#244300=CARTESIAN_POINT('Ctrl Pts',(-8.22469097903492,15.2,7.69125941239865));
#244301=CARTESIAN_POINT('Ctrl Pts',(-8.22608630302924,15.2,7.69446807494943));
#244302=CARTESIAN_POINT('Ctrl Pts',(-8.22748162677009,15.2,7.69767673691729));
#244303=CARTESIAN_POINT('Ctrl Pts',(-8.22887602945265,15.2,7.70089357186806));
#244304=CARTESIAN_POINT('Ctrl Pts',(-8.23026947361027,15.2,7.70411856033493));
#244305=CARTESIAN_POINT('Ctrl Pts',(-8.23212739906937,15.2,7.70841854476211));
#244306=CARTESIAN_POINT('Ctrl Pts',(-8.23398361793977,15.2,7.71273302241631));
#244307=CARTESIAN_POINT('Ctrl Pts',(-8.2358380382143,15.2,7.71706194438852));
#244308=CARTESIAN_POINT('Ctrl Pts',(-8.23722885348336,15.2,7.72030863601513));
#244309=CARTESIAN_POINT('Ctrl Pts',(-8.23861865699762,15.2,7.7235634522916));
#244310=CARTESIAN_POINT('Ctrl Pts',(-8.24000740923898,15.2,7.72682637179695));
#244311=CARTESIAN_POINT('Ctrl Pts',(-8.242321996392,15.2,7.73226457117011));
#244312=CARTESIAN_POINT('Ctrl Pts',(-8.24463366460899,15.2,7.73772527922906));
#244313=CARTESIAN_POINT('Ctrl Pts',(-8.24694223516477,15.2,7.74320840103274));
#244314=CARTESIAN_POINT('Ctrl Pts',(-8.24832737769955,15.2,7.74649827459308));
#244315=CARTESIAN_POINT('Ctrl Pts',(-8.24971140578404,15.2,7.74979621608907));
#244316=CARTESIAN_POINT('Ctrl Pts',(-8.25109428027653,15.2,7.75310220519565));
#244317=CARTESIAN_POINT('Ctrl Pts',(-8.2524771545178,15.2,7.75640819370164));
#244318=CARTESIAN_POINT('Ctrl Pts',(-8.25385887513413,15.2,7.75972223006552));
#244319=CARTESIAN_POINT('Ctrl Pts',(-8.25523940487552,15.2,7.76304429211217));
#244320=CARTESIAN_POINT('Ctrl Pts',(-8.25708011111378,15.2,7.7674737079732));
#244321=CARTESIAN_POINT('Ctrl Pts',(-8.25891869948066,15.2,7.771917393285));
#244322=CARTESIAN_POINT('Ctrl Pts',(-8.26075508120025,15.2,7.77637529858647));
#244323=CARTESIAN_POINT('Ctrl Pts',(-8.26259146317004,15.2,7.78083320449532));
#244324=CARTESIAN_POINT('Ctrl Pts',(-8.26442563892233,15.2,7.78530532939918));
#244325=CARTESIAN_POINT('Ctrl Pts',(-8.26625751813313,15.2,7.78979162386682));
#244326=CARTESIAN_POINT('Ctrl Pts',(-8.26808939709433,15.2,7.79427791772318));
#244327=CARTESIAN_POINT('Ctrl Pts',(-8.26991898108655,15.2,7.79877838277397));
#244328=CARTESIAN_POINT('Ctrl Pts',(-8.27174618199298,15.2,7.80329296657013));
#244329=CARTESIAN_POINT('Ctrl Pts',(-8.27357338314836,15.2,7.8078075509814));
#244330=CARTESIAN_POINT('Ctrl Pts',(-8.27539820094928,15.2,7.8123362562431));
#244331=CARTESIAN_POINT('Ctrl Pts',(-8.2772205495013,15.2,7.81687903201136));
#244332=CARTESIAN_POINT('Ctrl Pts',(-8.27858731079118,15.2,7.82028611352807));
#244333=CARTESIAN_POINT('Ctrl Pts',(-8.27995268290886,15.2,7.82370111027236));
#244334=CARTESIAN_POINT('Ctrl Pts',(-8.28131662869883,15.2,7.82712400028849));
#244335=CARTESIAN_POINT('Ctrl Pts',(-8.28313522325065,15.2,7.83168785405788));
#244336=CARTESIAN_POINT('Ctrl Pts',(-8.284951282523,15.2,7.83626574011846));
#244337=CARTESIAN_POINT('Ctrl Pts',(-8.28676472178823,15.2,7.84085761175904));
#244338=CARTESIAN_POINT('Ctrl Pts',(-8.28812480111362,15.2,7.84430151517665));
#244339=CARTESIAN_POINT('Ctrl Pts',(-8.2894834075974,15.2,7.8477532838355));
#244340=CARTESIAN_POINT('Ctrl Pts',(-8.29084050442296,15.2,7.85121289833549));
#244341=CARTESIAN_POINT('Ctrl Pts',(-8.29219760124853,15.2,7.85467251283547));
#244342=CARTESIAN_POINT('Ctrl Pts',(-8.29355318942768,15.2,7.85813997349688));
#244343=CARTESIAN_POINT('Ctrl Pts',(-8.29490723125963,15.2,7.86161525801142));
#244344=CARTESIAN_POINT('Ctrl Pts',(-8.29626127309158,15.2,7.86509054252597));
#244345=CARTESIAN_POINT('Ctrl Pts',(-8.29761376887511,15.2,7.86857365165778));
#244346=CARTESIAN_POINT('Ctrl Pts',(-8.29896468270717,15.2,7.87206456271343));
#244347=CARTESIAN_POINT('Ctrl Pts',(-8.30031559653923,15.2,7.87555547376907));
#244348=CARTESIAN_POINT('Ctrl Pts',(-8.3016649279353,15.2,7.8790541881126));
#244349=CARTESIAN_POINT('Ctrl Pts',(-8.30301264530314,15.2,7.88256068565119));
#244350=CARTESIAN_POINT('Ctrl Pts',(-8.30436036267098,15.2,7.88606718318977));
#244351=CARTESIAN_POINT('Ctrl Pts',(-8.3057064672556,15.2,7.88958146527782));
#244352=CARTESIAN_POINT('Ctrl Pts',(-8.30705092395697,15.2,7.89310351077379));
#244353=CARTESIAN_POINT('Ctrl Pts',(-8.30839538090259,15.2,7.89662555690959));
#244354=CARTESIAN_POINT('Ctrl Pts',(-8.30973818973108,15.2,7.90015536723927));
#244355=CARTESIAN_POINT('Ctrl Pts',(-8.31107930955076,15.2,7.90369291629613));
#244356=CARTESIAN_POINT('Ctrl Pts',(-8.31331450868175,15.2,7.90958882989137));
#244357=CARTESIAN_POINT('Ctrl Pts',(-8.31554500059004,15.2,7.91550623273332));
#244358=CARTESIAN_POINT('Ctrl Pts',(-8.31777064750062,15.2,7.92144504097314));
#244359=CARTESIAN_POINT('Ctrl Pts',(-8.3195511653202,15.2,7.92619608834179));
#244360=CARTESIAN_POINT('Ctrl Pts',(-8.32132858851655,15.2,7.93096084169788));
#244361=CARTESIAN_POINT('Ctrl Pts',(-8.32310290900006,15.2,7.93573928299999));
#244362=CARTESIAN_POINT('Ctrl Pts',(-7.01216898600006,15.2,7.64657512399998));
#244363=CARTESIAN_POINT('Ctrl Pts',(-7.01216898600006,11.6,7.64657512399998));
#244364=CARTESIAN_POINT('Ctrl Pts',(-7.01229743800006,15.2,7.64669302599999));
#244365=CARTESIAN_POINT('Ctrl Pts',(-7.01229743800006,11.6,7.64669302599999));
#244366=CARTESIAN_POINT('Ctrl Pts',(-7.01255888500006,15.2,7.64693288599998));
#244367=CARTESIAN_POINT('Ctrl Pts',(-7.01255888500006,11.6,7.64693288599998));
#244368=CARTESIAN_POINT('Ctrl Pts',(-7.01295521800006,15.2,7.64729613499998));
#244369=CARTESIAN_POINT('Ctrl Pts',(-7.01295521800006,11.6,7.64729613499998));
#244370=CARTESIAN_POINT('Ctrl Pts',(-7.01348948000006,15.2,7.64778506499999));
#244371=CARTESIAN_POINT('Ctrl Pts',(-7.01348948000006,11.6,7.64778506499999));
#244372=CARTESIAN_POINT('Ctrl Pts',(-7.01416585900006,15.2,7.64840281599999));
#244373=CARTESIAN_POINT('Ctrl Pts',(-7.01416585900006,11.6,7.64840281599999));
#244374=CARTESIAN_POINT('Ctrl Pts',(-7.01485383100006,15.2,7.64902988999999));
#244375=CARTESIAN_POINT('Ctrl Pts',(-7.01485383100006,11.6,7.64902988999999));
#244376=CARTESIAN_POINT('Ctrl Pts',(-7.01554947000006,15.2,7.64966267399998));
#244377=CARTESIAN_POINT('Ctrl Pts',(-7.01554947000006,11.6,7.64966267399998));
#244378=CARTESIAN_POINT('Ctrl Pts',(-7.01625276700006,15.2,7.65030113899999));
#244379=CARTESIAN_POINT('Ctrl Pts',(-7.01625276700006,11.6,7.65030113899999));
#244380=CARTESIAN_POINT('Ctrl Pts',(-7.01696371600006,15.2,7.65094525299999));
#244381=CARTESIAN_POINT('Ctrl Pts',(-7.01696371600006,11.6,7.65094525299999));
#244382=CARTESIAN_POINT('Ctrl Pts',(-7.01768230900006,15.2,7.65159498499998));
#244383=CARTESIAN_POINT('Ctrl Pts',(-7.01768230900006,11.6,7.65159498499998));
#244384=CARTESIAN_POINT('Ctrl Pts',(-7.01840853600006,15.2,7.65225030299998));
#244385=CARTESIAN_POINT('Ctrl Pts',(-7.01840853600006,11.6,7.65225030299998));
#244386=CARTESIAN_POINT('Ctrl Pts',(-7.01914239300006,15.2,7.65291117499999));
#244387=CARTESIAN_POINT('Ctrl Pts',(-7.01914239300006,11.6,7.65291117499999));
#244388=CARTESIAN_POINT('Ctrl Pts',(-7.01988387000006,15.2,7.65357757299999));
#244389=CARTESIAN_POINT('Ctrl Pts',(-7.01988387000006,11.6,7.65357757299999));
#244390=CARTESIAN_POINT('Ctrl Pts',(-7.02063296000006,15.2,7.65424946399998));
#244391=CARTESIAN_POINT('Ctrl Pts',(-7.02063296000006,11.6,7.65424946399998));
#244392=CARTESIAN_POINT('Ctrl Pts',(-7.02138965700006,15.2,7.65492681899998));
#244393=CARTESIAN_POINT('Ctrl Pts',(-7.02138965700006,11.6,7.65492681899998));
#244394=CARTESIAN_POINT('Ctrl Pts',(-7.02215395000006,15.2,7.65560960799998));
#244395=CARTESIAN_POINT('Ctrl Pts',(-7.02215395000006,11.6,7.65560960799998));
#244396=CARTESIAN_POINT('Ctrl Pts',(-7.02292583400006,15.2,7.65629779899999));
#244397=CARTESIAN_POINT('Ctrl Pts',(-7.02292583400006,11.6,7.65629779899999));
#244398=CARTESIAN_POINT('Ctrl Pts',(-7.02370530000006,15.2,7.65699136299999));
#244399=CARTESIAN_POINT('Ctrl Pts',(-7.02370530000006,11.6,7.65699136299999));
#244400=CARTESIAN_POINT('Ctrl Pts',(-7.02449234200006,15.2,7.65769026899999));
#244401=CARTESIAN_POINT('Ctrl Pts',(-7.02449234200006,11.6,7.65769026899999));
#244402=CARTESIAN_POINT('Ctrl Pts',(-7.02528695100006,15.2,7.65839448899998));
#244403=CARTESIAN_POINT('Ctrl Pts',(-7.02528695100006,11.6,7.65839448899998));
#244404=CARTESIAN_POINT('Ctrl Pts',(-7.02608912200006,15.2,7.65910399299998));
#244405=CARTESIAN_POINT('Ctrl Pts',(-7.02608912200006,11.6,7.65910399299998));
#244406=CARTESIAN_POINT('Ctrl Pts',(-7.02689884500006,15.2,7.65981874999999));
#244407=CARTESIAN_POINT('Ctrl Pts',(-7.02689884500006,11.6,7.65981874999999));
#244408=CARTESIAN_POINT('Ctrl Pts',(-7.02771611300006,15.2,7.66053873299998));
#244409=CARTESIAN_POINT('Ctrl Pts',(-7.02771611300006,11.6,7.66053873299998));
#244410=CARTESIAN_POINT('Ctrl Pts',(-7.02854092000006,15.2,7.66126390999998));
#244411=CARTESIAN_POINT('Ctrl Pts',(-7.02854092000006,11.6,7.66126390999998));
#244412=CARTESIAN_POINT('Ctrl Pts',(-7.02937325800006,15.2,7.66199425499998));
#244413=CARTESIAN_POINT('Ctrl Pts',(-7.02937325800006,11.6,7.66199425499998));
#244414=CARTESIAN_POINT('Ctrl Pts',(-7.03021311900006,15.2,7.66272973699999));
#244415=CARTESIAN_POINT('Ctrl Pts',(-7.03021311900006,11.6,7.66272973699999));
#244416=CARTESIAN_POINT('Ctrl Pts',(-7.03106049600006,15.2,7.66347032799998));
#244417=CARTESIAN_POINT('Ctrl Pts',(-7.03106049600006,11.6,7.66347032799998));
#244418=CARTESIAN_POINT('Ctrl Pts',(-7.03191538200006,15.2,7.66421599899999));
#244419=CARTESIAN_POINT('Ctrl Pts',(-7.03191538200006,11.6,7.66421599899999));
#244420=CARTESIAN_POINT('Ctrl Pts',(-7.03277777000006,15.2,7.66496672199998));
#244421=CARTESIAN_POINT('Ctrl Pts',(-7.03277777000006,11.6,7.66496672199998));
#244422=CARTESIAN_POINT('Ctrl Pts',(-7.03364765200006,15.2,7.66572246899998));
#244423=CARTESIAN_POINT('Ctrl Pts',(-7.03364765200006,11.6,7.66572246899998));
#244424=CARTESIAN_POINT('Ctrl Pts',(-7.03452502100006,15.2,7.66648321099999));
#244425=CARTESIAN_POINT('Ctrl Pts',(-7.03452502100006,11.6,7.66648321099999));
#244426=CARTESIAN_POINT('Ctrl Pts',(-7.03540987000006,15.2,7.66724892099998));
#244427=CARTESIAN_POINT('Ctrl Pts',(-7.03540987000006,11.6,7.66724892099998));
#244428=CARTESIAN_POINT('Ctrl Pts',(-7.03630219100006,15.2,7.66801956799998));
#244429=CARTESIAN_POINT('Ctrl Pts',(-7.03630219100006,11.6,7.66801956799998));
#244430=CARTESIAN_POINT('Ctrl Pts',(-7.03720197800005,15.2,7.66879512799999));
#244431=CARTESIAN_POINT('Ctrl Pts',(-7.03720197800005,11.6,7.66879512799999));
#244432=CARTESIAN_POINT('Ctrl Pts',(-7.03810922400006,15.2,7.66957557299998));
#244433=CARTESIAN_POINT('Ctrl Pts',(-7.03810922400006,11.6,7.66957557299998));
#244434=CARTESIAN_POINT('Ctrl Pts',(-7.03902392100006,15.2,7.67036087199998));
#244435=CARTESIAN_POINT('Ctrl Pts',(-7.03902392100006,11.6,7.67036087199998));
#244436=CARTESIAN_POINT('Ctrl Pts',(-7.03994606100006,15.2,7.67115099999998));
#244437=CARTESIAN_POINT('Ctrl Pts',(-7.03994606100006,11.6,7.67115099999998));
#244438=CARTESIAN_POINT('Ctrl Pts',(-7.04087563900006,15.2,7.67194592999999));
#244439=CARTESIAN_POINT('Ctrl Pts',(-7.04087563900006,11.6,7.67194592999999));
#244440=CARTESIAN_POINT('Ctrl Pts',(-7.04181264600006,15.2,7.67274563399998));
#244441=CARTESIAN_POINT('Ctrl Pts',(-7.04181264600006,11.6,7.67274563399998));
#244442=CARTESIAN_POINT('Ctrl Pts',(-7.04275707700006,15.2,7.67355008599999));
#244443=CARTESIAN_POINT('Ctrl Pts',(-7.04275707700006,11.6,7.67355008599999));
#244444=CARTESIAN_POINT('Ctrl Pts',(-7.04370892200005,15.2,7.67435925699999));
#244445=CARTESIAN_POINT('Ctrl Pts',(-7.04370892200005,11.6,7.67435925699999));
#244446=CARTESIAN_POINT('Ctrl Pts',(-7.04466817800006,15.2,7.67517312299999));
#244447=CARTESIAN_POINT('Ctrl Pts',(-7.04466817800006,11.6,7.67517312299999));
#244448=CARTESIAN_POINT('Ctrl Pts',(-7.04563483400006,15.2,7.67599165499998));
#244449=CARTESIAN_POINT('Ctrl Pts',(-7.04563483400006,11.6,7.67599165499998));
#244450=CARTESIAN_POINT('Ctrl Pts',(-7.04660888600006,15.2,7.67681482699999));
#244451=CARTESIAN_POINT('Ctrl Pts',(-7.04660888600006,11.6,7.67681482699999));
#244452=CARTESIAN_POINT('Ctrl Pts',(-7.04759032400006,15.2,7.67764261299998));
#244453=CARTESIAN_POINT('Ctrl Pts',(-7.04759032400006,11.6,7.67764261299998));
#244454=CARTESIAN_POINT('Ctrl Pts',(-7.04857914400006,15.2,7.67847498699999));
#244455=CARTESIAN_POINT('Ctrl Pts',(-7.04857914400006,11.6,7.67847498699999));
#244456=CARTESIAN_POINT('Ctrl Pts',(-7.04957533900005,15.2,7.67931192299999));
#244457=CARTESIAN_POINT('Ctrl Pts',(-7.04957533900005,11.6,7.67931192299999));
#244458=CARTESIAN_POINT('Ctrl Pts',(-7.05057890000006,15.2,7.68015339299998));
#244459=CARTESIAN_POINT('Ctrl Pts',(-7.05057890000006,11.6,7.68015339299998));
#244460=CARTESIAN_POINT('Ctrl Pts',(-7.05158982000006,15.2,7.68099937399998));
#244461=CARTESIAN_POINT('Ctrl Pts',(-7.05158982000006,11.6,7.68099937399998));
#244462=CARTESIAN_POINT('Ctrl Pts',(-7.05260809400006,15.2,7.68184983699999));
#244463=CARTESIAN_POINT('Ctrl Pts',(-7.05260809400006,11.6,7.68184983699999));
#244464=CARTESIAN_POINT('Ctrl Pts',(-7.05363371500006,15.2,7.68270475799999));
#244465=CARTESIAN_POINT('Ctrl Pts',(-7.05363371500006,11.6,7.68270475799999));
#244466=CARTESIAN_POINT('Ctrl Pts',(-7.05466667400006,15.2,7.68356411099998));
#244467=CARTESIAN_POINT('Ctrl Pts',(-7.05466667400006,11.6,7.68356411099998));
#244468=CARTESIAN_POINT('Ctrl Pts',(-7.05570696700006,15.2,7.68442787099998));
#244469=CARTESIAN_POINT('Ctrl Pts',(-7.05570696700006,11.6,7.68442787099998));
#244470=CARTESIAN_POINT('Ctrl Pts',(-7.05675458400005,15.2,7.68529601199998));
#244471=CARTESIAN_POINT('Ctrl Pts',(-7.05675458400005,11.6,7.68529601199998));
#244472=CARTESIAN_POINT('Ctrl Pts',(-7.05780952100006,15.2,7.68616850899999));
#244473=CARTESIAN_POINT('Ctrl Pts',(-7.05780952100006,11.6,7.68616850899999));
#244474=CARTESIAN_POINT('Ctrl Pts',(-7.05887177100006,15.2,7.68704533799998));
#244475=CARTESIAN_POINT('Ctrl Pts',(-7.05887177100006,11.6,7.68704533799998));
#244476=CARTESIAN_POINT('Ctrl Pts',(-7.05994132500006,15.2,7.68792647199999));
#244477=CARTESIAN_POINT('Ctrl Pts',(-7.05994132500006,11.6,7.68792647199999));
#244478=CARTESIAN_POINT('Ctrl Pts',(-7.06101817900006,15.2,7.68881188699999));
#244479=CARTESIAN_POINT('Ctrl Pts',(-7.06101817900006,11.6,7.68881188699999));
#244480=CARTESIAN_POINT('Ctrl Pts',(-7.06210232400006,15.2,7.68970155699999));
#244481=CARTESIAN_POINT('Ctrl Pts',(-7.06210232400006,11.6,7.68970155699999));
#244482=CARTESIAN_POINT('Ctrl Pts',(-7.06319375500006,15.2,7.69059545999998));
#244483=CARTESIAN_POINT('Ctrl Pts',(-7.06319375500006,11.6,7.69059545999998));
#244484=CARTESIAN_POINT('Ctrl Pts',(-7.06429246300006,15.2,7.69149356899998));
#244485=CARTESIAN_POINT('Ctrl Pts',(-7.06429246300006,11.6,7.69149356899998));
#244486=CARTESIAN_POINT('Ctrl Pts',(-7.06539844400006,15.2,7.69239585999999));
#244487=CARTESIAN_POINT('Ctrl Pts',(-7.06539844400006,11.6,7.69239585999999));
#244488=CARTESIAN_POINT('Ctrl Pts',(-7.06651169000006,15.2,7.69330230899998));
#244489=CARTESIAN_POINT('Ctrl Pts',(-7.06651169000006,11.6,7.69330230899998));
#244490=CARTESIAN_POINT('Ctrl Pts',(-7.06763219400006,15.2,7.69421289099999));
#244491=CARTESIAN_POINT('Ctrl Pts',(-7.06763219400006,11.6,7.69421289099999));
#244492=CARTESIAN_POINT('Ctrl Pts',(-7.06875995000006,15.2,7.69512758399999));
#244493=CARTESIAN_POINT('Ctrl Pts',(-7.06875995000006,11.6,7.69512758399999));
#244494=CARTESIAN_POINT('Ctrl Pts',(-7.06989495100006,15.2,7.69604635999999));
#244495=CARTESIAN_POINT('Ctrl Pts',(-7.06989495100006,11.6,7.69604635999999));
#244496=CARTESIAN_POINT('Ctrl Pts',(-7.07103719100005,15.2,7.69696919799999));
#244497=CARTESIAN_POINT('Ctrl Pts',(-7.07103719100005,11.6,7.69696919799999));
#244498=CARTESIAN_POINT('Ctrl Pts',(-7.07218666200006,15.2,7.69789607499998));
#244499=CARTESIAN_POINT('Ctrl Pts',(-7.07218666200006,11.6,7.69789607499998));
#244500=CARTESIAN_POINT('Ctrl Pts',(-7.07334335900006,15.2,7.69882696299998));
#244501=CARTESIAN_POINT('Ctrl Pts',(-7.07334335900006,11.6,7.69882696299998));
#244502=CARTESIAN_POINT('Ctrl Pts',(-7.07450727400006,15.2,7.69976184299999));
#244503=CARTESIAN_POINT('Ctrl Pts',(-7.07450727400006,11.6,7.69976184299999));
#244504=CARTESIAN_POINT('Ctrl Pts',(-7.07567840200006,15.2,7.70070068799999));
#244505=CARTESIAN_POINT('Ctrl Pts',(-7.07567840200006,11.6,7.70070068799999));
#244506=CARTESIAN_POINT('Ctrl Pts',(-7.07685673500006,15.2,7.70164347599999));
#244507=CARTESIAN_POINT('Ctrl Pts',(-7.07685673500006,11.6,7.70164347599999));
#244508=CARTESIAN_POINT('Ctrl Pts',(-7.07804226800006,15.2,7.70259018399998));
#244509=CARTESIAN_POINT('Ctrl Pts',(-7.07804226800006,11.6,7.70259018399998));
#244510=CARTESIAN_POINT('Ctrl Pts',(-7.07923499300006,15.2,7.70354078799999));
#244511=CARTESIAN_POINT('Ctrl Pts',(-7.07923499300006,11.6,7.70354078799999));
#244512=CARTESIAN_POINT('Ctrl Pts',(-7.08043490300006,15.2,7.70449526499998));
#244513=CARTESIAN_POINT('Ctrl Pts',(-7.08043490300006,11.6,7.70449526499998));
#244514=CARTESIAN_POINT('Ctrl Pts',(-7.08164199400006,15.2,7.70545359099999));
#244515=CARTESIAN_POINT('Ctrl Pts',(-7.08164199400006,11.6,7.70545359099999));
#244516=CARTESIAN_POINT('Ctrl Pts',(-7.08285625800006,15.2,7.70641574499999));
#244517=CARTESIAN_POINT('Ctrl Pts',(-7.08285625800006,11.6,7.70641574499999));
#244518=CARTESIAN_POINT('Ctrl Pts',(-7.08407768800006,15.2,7.70738170199999));
#244519=CARTESIAN_POINT('Ctrl Pts',(-7.08407768800006,11.6,7.70738170199999));
#244520=CARTESIAN_POINT('Ctrl Pts',(-7.08530627800006,15.2,7.70835144099999));
#244521=CARTESIAN_POINT('Ctrl Pts',(-7.08530627800006,11.6,7.70835144099999));
#244522=CARTESIAN_POINT('Ctrl Pts',(-7.08654202200006,15.2,7.70932493899998));
#244523=CARTESIAN_POINT('Ctrl Pts',(-7.08654202200006,11.6,7.70932493899998));
#244524=CARTESIAN_POINT('Ctrl Pts',(-7.08778491400006,15.2,7.71030217199999));
#244525=CARTESIAN_POINT('Ctrl Pts',(-7.08778491400006,11.6,7.71030217199999));
#244526=CARTESIAN_POINT('Ctrl Pts',(-7.08903494500006,15.2,7.71128311899999));
#244527=CARTESIAN_POINT('Ctrl Pts',(-7.08903494500006,11.6,7.71128311899999));
#244528=CARTESIAN_POINT('Ctrl Pts',(-7.09029211200006,15.2,7.71226775599998));
#244529=CARTESIAN_POINT('Ctrl Pts',(-7.09029211200006,11.6,7.71226775599998));
#244530=CARTESIAN_POINT('Ctrl Pts',(-7.09155640600006,15.2,7.71325606199999));
#244531=CARTESIAN_POINT('Ctrl Pts',(-7.09155640600006,11.6,7.71325606199999));
#244532=CARTESIAN_POINT('Ctrl Pts',(-7.09282782300006,15.2,7.71424801399998));
#244533=CARTESIAN_POINT('Ctrl Pts',(-7.09282782300006,11.6,7.71424801399998));
#244534=CARTESIAN_POINT('Ctrl Pts',(-7.09410635400006,15.2,7.71524359099999));
#244535=CARTESIAN_POINT('Ctrl Pts',(-7.09410635400006,11.6,7.71524359099999));
#244536=CARTESIAN_POINT('Ctrl Pts',(-7.09539199400006,15.2,7.71624276799999));
#244537=CARTESIAN_POINT('Ctrl Pts',(-7.09539199400006,11.6,7.71624276799999));
#244538=CARTESIAN_POINT('Ctrl Pts',(-7.09668473700006,15.2,7.71724552699999));
#244539=CARTESIAN_POINT('Ctrl Pts',(-7.09668473700006,11.6,7.71724552699999));
#244540=CARTESIAN_POINT('Ctrl Pts',(-7.09798457700006,15.2,7.71825184399999));
#244541=CARTESIAN_POINT('Ctrl Pts',(-7.09798457700006,11.6,7.71825184399999));
#244542=CARTESIAN_POINT('Ctrl Pts',(-7.09929150500006,15.2,7.71926169699999));
#244543=CARTESIAN_POINT('Ctrl Pts',(-7.09929150500006,11.6,7.71926169699999));
#244544=CARTESIAN_POINT('Ctrl Pts',(-7.10060551800006,15.2,7.72027506499998));
#244545=CARTESIAN_POINT('Ctrl Pts',(-7.10060551800006,11.6,7.72027506499998));
#244546=CARTESIAN_POINT('Ctrl Pts',(-7.10192660800006,15.2,7.72129192499998));
#244547=CARTESIAN_POINT('Ctrl Pts',(-7.10192660800006,11.6,7.72129192499998));
#244548=CARTESIAN_POINT('Ctrl Pts',(-7.10325476900006,15.2,7.72231225799998));
#244549=CARTESIAN_POINT('Ctrl Pts',(-7.10325476900006,11.6,7.72231225799998));
#244550=CARTESIAN_POINT('Ctrl Pts',(-7.10458999400006,15.2,7.72333603999999));
#244551=CARTESIAN_POINT('Ctrl Pts',(-7.10458999400006,11.6,7.72333603999999));
#244552=CARTESIAN_POINT('Ctrl Pts',(-7.10593227900006,15.2,7.72436325099999));
#244553=CARTESIAN_POINT('Ctrl Pts',(-7.10593227900006,11.6,7.72436325099999));
#244554=CARTESIAN_POINT('Ctrl Pts',(-7.10728161500006,15.2,7.72539386899999));
#244555=CARTESIAN_POINT('Ctrl Pts',(-7.10728161500006,11.6,7.72539386899999));
#244556=CARTESIAN_POINT('Ctrl Pts',(-7.10863799800006,15.2,7.72642787299999));
#244557=CARTESIAN_POINT('Ctrl Pts',(-7.10863799800006,11.6,7.72642787299999));
#244558=CARTESIAN_POINT('Ctrl Pts',(-7.11000142000006,15.2,7.72746524299999));
#244559=CARTESIAN_POINT('Ctrl Pts',(-7.11000142000006,11.6,7.72746524299999));
#244560=CARTESIAN_POINT('Ctrl Pts',(-7.11137187600006,15.2,7.72850595599999));
#244561=CARTESIAN_POINT('Ctrl Pts',(-7.11137187600006,11.6,7.72850595599999));
#244562=CARTESIAN_POINT('Ctrl Pts',(-7.11274935900006,15.2,7.72954999299999));
#244563=CARTESIAN_POINT('Ctrl Pts',(-7.11274935900006,11.6,7.72954999299999));
#244564=CARTESIAN_POINT('Ctrl Pts',(-7.11413386400006,15.2,7.73059733099998));
#244565=CARTESIAN_POINT('Ctrl Pts',(-7.11413386400006,11.6,7.73059733099998));
#244566=CARTESIAN_POINT('Ctrl Pts',(-7.11552538300006,15.2,7.73164795099999));
#244567=CARTESIAN_POINT('Ctrl Pts',(-7.11552538300006,11.6,7.73164795099999));
#244568=CARTESIAN_POINT('Ctrl Pts',(-7.11692391100006,15.2,7.73270183099999));
#244569=CARTESIAN_POINT('Ctrl Pts',(-7.11692391100006,11.6,7.73270183099999));
#244570=CARTESIAN_POINT('Ctrl Pts',(-7.11832944100006,15.2,7.73375895199998));
#244571=CARTESIAN_POINT('Ctrl Pts',(-7.11832944100006,11.6,7.73375895199998));
#244572=CARTESIAN_POINT('Ctrl Pts',(-7.11974196900006,15.2,7.73481929199999));
#244573=CARTESIAN_POINT('Ctrl Pts',(-7.11974196900006,11.6,7.73481929199999));
#244574=CARTESIAN_POINT('Ctrl Pts',(-7.12116148600006,15.2,7.73588283099999));
#244575=CARTESIAN_POINT('Ctrl Pts',(-7.12116148600006,11.6,7.73588283099999));
#244576=CARTESIAN_POINT('Ctrl Pts',(-7.12258798800006,15.2,7.73694954699998));
#244577=CARTESIAN_POINT('Ctrl Pts',(-7.12258798800006,11.6,7.73694954699998));
#244578=CARTESIAN_POINT('Ctrl Pts',(-7.12402146800006,15.2,7.73801942399999));
#244579=CARTESIAN_POINT('Ctrl Pts',(-7.12402146800006,11.6,7.73801942399999));
#244580=CARTESIAN_POINT('Ctrl Pts',(-7.12546192000006,15.2,7.73909243699999));
#244581=CARTESIAN_POINT('Ctrl Pts',(-7.12546192000006,11.6,7.73909243699999));
#244582=CARTESIAN_POINT('Ctrl Pts',(-7.12690933700006,15.2,7.74016856899999));
#244583=CARTESIAN_POINT('Ctrl Pts',(-7.12690933700006,11.6,7.74016856899999));
#244584=CARTESIAN_POINT('Ctrl Pts',(-7.12836371400006,15.2,7.74124779699999));
#244585=CARTESIAN_POINT('Ctrl Pts',(-7.12836371400006,11.6,7.74124779699999));
#244586=CARTESIAN_POINT('Ctrl Pts',(-7.12982504600006,15.2,7.74233010399998));
#244587=CARTESIAN_POINT('Ctrl Pts',(-7.12982504600006,11.6,7.74233010399998));
#244588=CARTESIAN_POINT('Ctrl Pts',(-7.13129332400006,15.2,7.74341546899999));
#244589=CARTESIAN_POINT('Ctrl Pts',(-7.13129332400006,11.6,7.74341546899999));
#244590=CARTESIAN_POINT('Ctrl Pts',(-7.13276854400006,15.2,7.74450386999998));
#244591=CARTESIAN_POINT('Ctrl Pts',(-7.13276854400006,11.6,7.74450386999998));
#244592=CARTESIAN_POINT('Ctrl Pts',(-7.13425070000006,15.2,7.74559529099999));
#244593=CARTESIAN_POINT('Ctrl Pts',(-7.13425070000006,11.6,7.74559529099999));
#244594=CARTESIAN_POINT('Ctrl Pts',(-7.13573978500006,15.2,7.74668970999999));
#244595=CARTESIAN_POINT('Ctrl Pts',(-7.13573978500006,11.6,7.74668970999999));
#244596=CARTESIAN_POINT('Ctrl Pts',(-7.13723579400006,15.2,7.74778710799998));
#244597=CARTESIAN_POINT('Ctrl Pts',(-7.13723579400006,11.6,7.74778710799998));
#244598=CARTESIAN_POINT('Ctrl Pts',(-7.13873872000006,15.2,7.74888746499999));
#244599=CARTESIAN_POINT('Ctrl Pts',(-7.13873872000006,11.6,7.74888746499999));
#244600=CARTESIAN_POINT('Ctrl Pts',(-7.14024855600006,15.2,7.74999076199999));
#244601=CARTESIAN_POINT('Ctrl Pts',(-7.14024855600006,11.6,7.74999076199999));
#244602=CARTESIAN_POINT('Ctrl Pts',(-7.14176530000006,15.2,7.75109697799999));
#244603=CARTESIAN_POINT('Ctrl Pts',(-7.14176530000006,11.6,7.75109697799999));
#244604=CARTESIAN_POINT('Ctrl Pts',(-7.14328894200006,15.2,7.75220609499998));
#244605=CARTESIAN_POINT('Ctrl Pts',(-7.14328894200006,11.6,7.75220609499998));
#244606=CARTESIAN_POINT('Ctrl Pts',(-7.14481947700006,15.2,7.75331809499999));
#244607=CARTESIAN_POINT('Ctrl Pts',(-7.14481947700006,11.6,7.75331809499999));
#244608=CARTESIAN_POINT('Ctrl Pts',(-7.14635690000006,15.2,7.75443295699999));
#244609=CARTESIAN_POINT('Ctrl Pts',(-7.14635690000006,11.6,7.75443295699999));
#244610=CARTESIAN_POINT('Ctrl Pts',(-7.14790120500005,15.2,7.75555066199999));
#244611=CARTESIAN_POINT('Ctrl Pts',(-7.14790120500005,11.6,7.75555066199999));
#244612=CARTESIAN_POINT('Ctrl Pts',(-7.14945238500006,15.2,7.75667119099998));
#244613=CARTESIAN_POINT('Ctrl Pts',(-7.14945238500006,11.6,7.75667119099998));
#244614=CARTESIAN_POINT('Ctrl Pts',(-7.15101043300006,15.2,7.75779452499999));
#244615=CARTESIAN_POINT('Ctrl Pts',(-7.15101043300006,11.6,7.75779452499999));
#244616=CARTESIAN_POINT('Ctrl Pts',(-7.15257534700006,15.2,7.75892064699998));
#244617=CARTESIAN_POINT('Ctrl Pts',(-7.15257534700006,11.6,7.75892064699998));
#244618=CARTESIAN_POINT('Ctrl Pts',(-7.15414711700006,15.2,7.76004953499999));
#244619=CARTESIAN_POINT('Ctrl Pts',(-7.15414711700006,11.6,7.76004953499999));
#244620=CARTESIAN_POINT('Ctrl Pts',(-7.15572573900006,15.2,7.76118117199999));
#244621=CARTESIAN_POINT('Ctrl Pts',(-7.15572573900006,11.6,7.76118117199999));
#244622=CARTESIAN_POINT('Ctrl Pts',(-7.15731120800006,15.2,7.76231553799998));
#244623=CARTESIAN_POINT('Ctrl Pts',(-7.15731120800006,11.6,7.76231553799998));
#244624=CARTESIAN_POINT('Ctrl Pts',(-7.15890351700006,15.2,7.76345261699999));
#244625=CARTESIAN_POINT('Ctrl Pts',(-7.15890351700006,11.6,7.76345261699999));
#244626=CARTESIAN_POINT('Ctrl Pts',(-7.16050265800006,15.2,7.76459238699999));
#244627=CARTESIAN_POINT('Ctrl Pts',(-7.16050265800006,11.6,7.76459238699999));
#244628=CARTESIAN_POINT('Ctrl Pts',(-7.16210862800006,15.2,7.76573483199999));
#244629=CARTESIAN_POINT('Ctrl Pts',(-7.16210862800006,11.6,7.76573483199999));
#244630=CARTESIAN_POINT('Ctrl Pts',(-7.16372142100006,15.2,7.76687993299999));
#244631=CARTESIAN_POINT('Ctrl Pts',(-7.16372142100006,11.6,7.76687993299999));
#244632=CARTESIAN_POINT('Ctrl Pts',(-7.16534103000006,15.2,7.76802766999998));
#244633=CARTESIAN_POINT('Ctrl Pts',(-7.16534103000006,11.6,7.76802766999998));
#244634=CARTESIAN_POINT('Ctrl Pts',(-7.16696745000006,15.2,7.76917802599999));
#244635=CARTESIAN_POINT('Ctrl Pts',(-7.16696745000006,11.6,7.76917802599999));
#244636=CARTESIAN_POINT('Ctrl Pts',(-7.16860067400006,15.2,7.77033098499999));
#244637=CARTESIAN_POINT('Ctrl Pts',(-7.16860067400006,11.6,7.77033098499999));
#244638=CARTESIAN_POINT('Ctrl Pts',(-7.17024069700006,15.2,7.77148652499999));
#244639=CARTESIAN_POINT('Ctrl Pts',(-7.17024069700006,11.6,7.77148652499999));
#244640=CARTESIAN_POINT('Ctrl Pts',(-7.17188751300006,15.2,7.77264462899999));
#244641=CARTESIAN_POINT('Ctrl Pts',(-7.17188751300006,11.6,7.77264462899999));
#244642=CARTESIAN_POINT('Ctrl Pts',(-7.17354111600006,15.2,7.77380527999998));
#244643=CARTESIAN_POINT('Ctrl Pts',(-7.17354111600006,11.6,7.77380527999998));
#244644=CARTESIAN_POINT('Ctrl Pts',(-7.17520150000006,15.2,7.77496845799998));
#244645=CARTESIAN_POINT('Ctrl Pts',(-7.17520150000006,11.6,7.77496845799998));
#244646=CARTESIAN_POINT('Ctrl Pts',(-7.17686866000006,15.2,7.77613414899999));
#244647=CARTESIAN_POINT('Ctrl Pts',(-7.17686866000006,11.6,7.77613414899999));
#244648=CARTESIAN_POINT('Ctrl Pts',(-7.17854259000006,15.2,7.77730232999998));
#244649=CARTESIAN_POINT('Ctrl Pts',(-7.17854259000006,11.6,7.77730232999998));
#244650=CARTESIAN_POINT('Ctrl Pts',(-7.18022328300005,15.2,7.77847298699999));
#244651=CARTESIAN_POINT('Ctrl Pts',(-7.18022328300005,11.6,7.77847298699999));
#244652=CARTESIAN_POINT('Ctrl Pts',(-7.18191073400006,15.2,7.77964609999999));
#244653=CARTESIAN_POINT('Ctrl Pts',(-7.18191073400006,11.6,7.77964609999999));
#244654=CARTESIAN_POINT('Ctrl Pts',(-7.18360493800006,15.2,7.78082165399999));
#244655=CARTESIAN_POINT('Ctrl Pts',(-7.18360493800006,11.6,7.78082165399999));
#244656=CARTESIAN_POINT('Ctrl Pts',(-7.18530588900006,15.2,7.78199962799999));
#244657=CARTESIAN_POINT('Ctrl Pts',(-7.18530588900006,11.6,7.78199962799999));
#244658=CARTESIAN_POINT('Ctrl Pts',(-7.18701358000006,15.2,7.78318000699999));
#244659=CARTESIAN_POINT('Ctrl Pts',(-7.18701358000006,11.6,7.78318000699999));
#244660=CARTESIAN_POINT('Ctrl Pts',(-7.18872800700006,15.2,7.78436277199998));
#244661=CARTESIAN_POINT('Ctrl Pts',(-7.18872800700006,11.6,7.78436277199998));
#244662=CARTESIAN_POINT('Ctrl Pts',(-7.19044916200006,15.2,7.78554790599999));
#244663=CARTESIAN_POINT('Ctrl Pts',(-7.19044916200006,11.6,7.78554790599999));
#244664=CARTESIAN_POINT('Ctrl Pts',(-7.19217704100005,15.2,7.78673539199998));
#244665=CARTESIAN_POINT('Ctrl Pts',(-7.19217704100005,11.6,7.78673539199998));
#244666=CARTESIAN_POINT('Ctrl Pts',(-7.19391163700006,15.2,7.78792521199998));
#244667=CARTESIAN_POINT('Ctrl Pts',(-7.19391163700006,11.6,7.78792521199998));
#244668=CARTESIAN_POINT('Ctrl Pts',(-7.19565294600006,15.2,7.78911734999999));
#244669=CARTESIAN_POINT('Ctrl Pts',(-7.19565294600006,11.6,7.78911734999999));
#244670=CARTESIAN_POINT('Ctrl Pts',(-7.19740096200006,15.2,7.79031178799999));
#244671=CARTESIAN_POINT('Ctrl Pts',(-7.19740096200006,11.6,7.79031178799999));
#244672=CARTESIAN_POINT('Ctrl Pts',(-7.19915567700006,15.2,7.79150850799999));
#244673=CARTESIAN_POINT('Ctrl Pts',(-7.19915567700006,11.6,7.79150850799999));
#244674=CARTESIAN_POINT('Ctrl Pts',(-7.20091708800005,15.2,7.79270749399998));
#244675=CARTESIAN_POINT('Ctrl Pts',(-7.20091708800005,11.6,7.79270749399998));
#244676=CARTESIAN_POINT('Ctrl Pts',(-7.20268518700006,15.2,7.79390872899998));
#244677=CARTESIAN_POINT('Ctrl Pts',(-7.20268518700006,11.6,7.79390872899998));
#244678=CARTESIAN_POINT('Ctrl Pts',(-7.20445997000006,15.2,7.79511219599998));
#244679=CARTESIAN_POINT('Ctrl Pts',(-7.20445997000006,11.6,7.79511219599998));
#244680=CARTESIAN_POINT('Ctrl Pts',(-7.20624143100006,15.2,7.79631787699999));
#244681=CARTESIAN_POINT('Ctrl Pts',(-7.20624143100006,11.6,7.79631787699999));
#244682=CARTESIAN_POINT('Ctrl Pts',(-7.20802956400005,15.2,7.79752575699998));
#244683=CARTESIAN_POINT('Ctrl Pts',(-7.20802956400005,11.6,7.79752575699998));
#244684=CARTESIAN_POINT('Ctrl Pts',(-7.20982436400006,15.2,7.79873581599999));
#244685=CARTESIAN_POINT('Ctrl Pts',(-7.20982436400006,11.6,7.79873581599999));
#244686=CARTESIAN_POINT('Ctrl Pts',(-7.21162582400006,15.2,7.79994804199998));
#244687=CARTESIAN_POINT('Ctrl Pts',(-7.21162582400006,11.6,7.79994804199998));
#244688=CARTESIAN_POINT('Ctrl Pts',(-7.21343393900006,15.2,7.80116241399998));
#244689=CARTESIAN_POINT('Ctrl Pts',(-7.21343393900006,11.6,7.80116241399998));
#244690=CARTESIAN_POINT('Ctrl Pts',(-7.21524870400006,15.2,7.80237891799998));
#244691=CARTESIAN_POINT('Ctrl Pts',(-7.21524870400006,11.6,7.80237891799998));
#244692=CARTESIAN_POINT('Ctrl Pts',(-7.21707011300006,15.2,7.80359753599999));
#244693=CARTESIAN_POINT('Ctrl Pts',(-7.21707011300006,11.6,7.80359753599999));
#244694=CARTESIAN_POINT('Ctrl Pts',(-7.21889815900006,15.2,7.80481825199999));
#244695=CARTESIAN_POINT('Ctrl Pts',(-7.21889815900006,11.6,7.80481825199999));
#244696=CARTESIAN_POINT('Ctrl Pts',(-7.22073283800006,15.2,7.80604104899999));
#244697=CARTESIAN_POINT('Ctrl Pts',(-7.22073283800006,11.6,7.80604104899999));
#244698=CARTESIAN_POINT('Ctrl Pts',(-7.22257414400006,15.2,7.80726591199999));
#244699=CARTESIAN_POINT('Ctrl Pts',(-7.22257414400006,11.6,7.80726591199999));
#244700=CARTESIAN_POINT('Ctrl Pts',(-7.22442207200006,15.2,7.80849282399998));
#244701=CARTESIAN_POINT('Ctrl Pts',(-7.22442207200006,11.6,7.80849282399998));
#244702=CARTESIAN_POINT('Ctrl Pts',(-7.22627661400006,15.2,7.80972176699999));
#244703=CARTESIAN_POINT('Ctrl Pts',(-7.22627661400006,11.6,7.80972176699999));
#244704=CARTESIAN_POINT('Ctrl Pts',(-7.22813776800006,15.2,7.81095272699999));
#244705=CARTESIAN_POINT('Ctrl Pts',(-7.22813776800006,11.6,7.81095272699999));
#244706=CARTESIAN_POINT('Ctrl Pts',(-7.23000552500006,15.2,7.81218568699998));
#244707=CARTESIAN_POINT('Ctrl Pts',(-7.23000552500006,11.6,7.81218568699998));
#244708=CARTESIAN_POINT('Ctrl Pts',(-7.23187988200006,15.2,7.81342063099999));
#244709=CARTESIAN_POINT('Ctrl Pts',(-7.23187988200006,11.6,7.81342063099999));
#244710=CARTESIAN_POINT('Ctrl Pts',(-7.23376083100006,15.2,7.81465754299998));
#244711=CARTESIAN_POINT('Ctrl Pts',(-7.23376083100006,11.6,7.81465754299998));
#244712=CARTESIAN_POINT('Ctrl Pts',(-7.23564836800006,15.2,7.81589640599999));
#244713=CARTESIAN_POINT('Ctrl Pts',(-7.23564836800006,11.6,7.81589640599999));
#244714=CARTESIAN_POINT('Ctrl Pts',(-7.23754248700006,15.2,7.81713720599999));
#244715=CARTESIAN_POINT('Ctrl Pts',(-7.23754248700006,11.6,7.81713720599999));
#244716=CARTESIAN_POINT('Ctrl Pts',(-7.23944318300005,15.2,7.81837992399999));
#244717=CARTESIAN_POINT('Ctrl Pts',(-7.23944318300005,11.6,7.81837992399999));
#244718=CARTESIAN_POINT('Ctrl Pts',(-7.24135045000006,15.2,7.81962454799999));
#244719=CARTESIAN_POINT('Ctrl Pts',(-7.24135045000006,11.6,7.81962454799999));
#244720=CARTESIAN_POINT('Ctrl Pts',(-7.24326428200006,15.2,7.82087105799998));
#244721=CARTESIAN_POINT('Ctrl Pts',(-7.24326428200006,11.6,7.82087105799998));
#244722=CARTESIAN_POINT('Ctrl Pts',(-7.24518467300006,15.2,7.82211944199998));
#244723=CARTESIAN_POINT('Ctrl Pts',(-7.24518467300006,11.6,7.82211944199998));
#244724=CARTESIAN_POINT('Ctrl Pts',(-7.24711162000006,15.2,7.82336968199999));
#244725=CARTESIAN_POINT('Ctrl Pts',(-7.24711162000006,11.6,7.82336968199999));
#244726=CARTESIAN_POINT('Ctrl Pts',(-7.24904511400006,15.2,7.82462176199999));
#244727=CARTESIAN_POINT('Ctrl Pts',(-7.24904511400006,11.6,7.82462176199999));
#244728=CARTESIAN_POINT('Ctrl Pts',(-7.25098515300005,15.2,7.82587566899998));
#244729=CARTESIAN_POINT('Ctrl Pts',(-7.25098515300005,11.6,7.82587566899998));
#244730=CARTESIAN_POINT('Ctrl Pts',(-7.25293172800006,15.2,7.82713138499999));
#244731=CARTESIAN_POINT('Ctrl Pts',(-7.25293172800006,11.6,7.82713138499999));
#244732=CARTESIAN_POINT('Ctrl Pts',(-7.25488483700006,15.2,7.82838889399999));
#244733=CARTESIAN_POINT('Ctrl Pts',(-7.25488483700006,11.6,7.82838889399999));
#244734=CARTESIAN_POINT('Ctrl Pts',(-7.25684447100006,15.2,7.82964818299998));
#244735=CARTESIAN_POINT('Ctrl Pts',(-7.25684447100006,11.6,7.82964818299998));
#244736=CARTESIAN_POINT('Ctrl Pts',(-7.25881062600005,15.2,7.83090923599998));
#244737=CARTESIAN_POINT('Ctrl Pts',(-7.25881062600005,11.6,7.83090923599998));
#244738=CARTESIAN_POINT('Ctrl Pts',(-7.26078329800006,15.2,7.83217203499999));
#244739=CARTESIAN_POINT('Ctrl Pts',(-7.26078329800006,11.6,7.83217203499999));
#244740=CARTESIAN_POINT('Ctrl Pts',(-7.26276247900006,15.2,7.83343656799998));
#244741=CARTESIAN_POINT('Ctrl Pts',(-7.26276247900006,11.6,7.83343656799998));
#244742=CARTESIAN_POINT('Ctrl Pts',(-7.26474816500006,15.2,7.83470281899999));
#244743=CARTESIAN_POINT('Ctrl Pts',(-7.26474816500006,11.6,7.83470281899999));
#244744=CARTESIAN_POINT('Ctrl Pts',(-7.26674035000006,15.2,7.83597076999998));
#244745=CARTESIAN_POINT('Ctrl Pts',(-7.26674035000006,11.6,7.83597076999998));
#244746=CARTESIAN_POINT('Ctrl Pts',(-7.26873902900006,15.2,7.83724040899998));
#244747=CARTESIAN_POINT('Ctrl Pts',(-7.26873902900006,11.6,7.83724040899998));
#244748=CARTESIAN_POINT('Ctrl Pts',(-7.27074419600005,15.2,7.83851171899999));
#244749=CARTESIAN_POINT('Ctrl Pts',(-7.27074419600005,11.6,7.83851171899999));
#244750=CARTESIAN_POINT('Ctrl Pts',(-7.27275584500005,15.2,7.83978468699999));
#244751=CARTESIAN_POINT('Ctrl Pts',(-7.27275584500005,11.6,7.83978468699999));
#244752=CARTESIAN_POINT('Ctrl Pts',(-7.27477397200006,15.2,7.84105929599999));
#244753=CARTESIAN_POINT('Ctrl Pts',(-7.27477397200006,11.6,7.84105929599999));
#244754=CARTESIAN_POINT('Ctrl Pts',(-7.27679857000005,15.2,7.84233553099998));
#244755=CARTESIAN_POINT('Ctrl Pts',(-7.27679857000005,11.6,7.84233553099998));
#244756=CARTESIAN_POINT('Ctrl Pts',(-7.27882963600006,15.2,7.84361337899998));
#244757=CARTESIAN_POINT('Ctrl Pts',(-7.27882963600006,11.6,7.84361337899998));
#244758=CARTESIAN_POINT('Ctrl Pts',(-7.28086716200006,15.2,7.84489282299998));
#244759=CARTESIAN_POINT('Ctrl Pts',(-7.28086716200006,11.6,7.84489282299998));
#244760=CARTESIAN_POINT('Ctrl Pts',(-7.28291114200006,15.2,7.84617384799999));
#244761=CARTESIAN_POINT('Ctrl Pts',(-7.28291114200006,11.6,7.84617384799999));
#244762=CARTESIAN_POINT('Ctrl Pts',(-7.28496157300006,15.2,7.84745644199998));
#244763=CARTESIAN_POINT('Ctrl Pts',(-7.28496157300006,11.6,7.84745644199998));
#244764=CARTESIAN_POINT('Ctrl Pts',(-7.28701844900006,15.2,7.84874058699998));
#244765=CARTESIAN_POINT('Ctrl Pts',(-7.28701844900006,11.6,7.84874058699998));
#244766=CARTESIAN_POINT('Ctrl Pts',(-7.28908176300005,15.2,7.85002626999999));
#244767=CARTESIAN_POINT('Ctrl Pts',(-7.28908176300005,11.6,7.85002626999999));
#244768=CARTESIAN_POINT('Ctrl Pts',(-7.29115151200006,15.2,7.85131347699998));
#244769=CARTESIAN_POINT('Ctrl Pts',(-7.29115151200006,11.6,7.85131347699998));
#244770=CARTESIAN_POINT('Ctrl Pts',(-7.29322768800006,15.2,7.85260219099998));
#244771=CARTESIAN_POINT('Ctrl Pts',(-7.29322768800006,11.6,7.85260219099998));
#244772=CARTESIAN_POINT('Ctrl Pts',(-7.29531028700006,15.2,7.85389239899998));
#244773=CARTESIAN_POINT('Ctrl Pts',(-7.29531028700006,11.6,7.85389239899998));
#244774=CARTESIAN_POINT('Ctrl Pts',(-7.29739930400005,15.2,7.85518408599999));
#244775=CARTESIAN_POINT('Ctrl Pts',(-7.29739930400005,11.6,7.85518408599999));
#244776=CARTESIAN_POINT('Ctrl Pts',(-7.29949473300006,15.2,7.85647723899999));
#244777=CARTESIAN_POINT('Ctrl Pts',(-7.29949473300006,11.6,7.85647723899999));
#244778=CARTESIAN_POINT('Ctrl Pts',(-7.30159656800006,15.2,7.85777184099998));
#244779=CARTESIAN_POINT('Ctrl Pts',(-7.30159656800006,11.6,7.85777184099998));
#244780=CARTESIAN_POINT('Ctrl Pts',(-7.30370480500006,15.2,7.85906787899999));
#244781=CARTESIAN_POINT('Ctrl Pts',(-7.30370480500006,11.6,7.85906787899999));
#244782=CARTESIAN_POINT('Ctrl Pts',(-7.30581943700006,15.2,7.86036533899999));
#244783=CARTESIAN_POINT('Ctrl Pts',(-7.30581943700006,11.6,7.86036533899999));
#244784=CARTESIAN_POINT('Ctrl Pts',(-7.30794046000006,15.2,7.86166420599999));
#244785=CARTESIAN_POINT('Ctrl Pts',(-7.30794046000006,11.6,7.86166420599999));
#244786=CARTESIAN_POINT('Ctrl Pts',(-7.31006786800006,15.2,7.86296446599999));
#244787=CARTESIAN_POINT('Ctrl Pts',(-7.31006786800006,11.6,7.86296446599999));
#244788=CARTESIAN_POINT('Ctrl Pts',(-7.31220165500006,15.2,7.86426610399998));
#244789=CARTESIAN_POINT('Ctrl Pts',(-7.31220165500006,11.6,7.86426610399998));
#244790=CARTESIAN_POINT('Ctrl Pts',(-7.31434181800006,15.2,7.86556910899999));
#244791=CARTESIAN_POINT('Ctrl Pts',(-7.31434181800006,11.6,7.86556910899999));
#244792=CARTESIAN_POINT('Ctrl Pts',(-7.31648834800006,15.2,7.86687346199999));
#244793=CARTESIAN_POINT('Ctrl Pts',(-7.31648834800006,11.6,7.86687346199999));
#244794=CARTESIAN_POINT('Ctrl Pts',(-7.31864124200006,15.2,7.86817915199999));
#244795=CARTESIAN_POINT('Ctrl Pts',(-7.31864124200006,11.6,7.86817915199999));
#244796=CARTESIAN_POINT('Ctrl Pts',(-7.32080049400006,15.2,7.86948616399999));
#244797=CARTESIAN_POINT('Ctrl Pts',(-7.32080049400006,11.6,7.86948616399999));
#244798=CARTESIAN_POINT('Ctrl Pts',(-7.32296610000006,15.2,7.87079448499998));
#244799=CARTESIAN_POINT('Ctrl Pts',(-7.32296610000006,11.6,7.87079448499998));
#244800=CARTESIAN_POINT('Ctrl Pts',(-7.32513805400006,15.2,7.87210409899998));
#244801=CARTESIAN_POINT('Ctrl Pts',(-7.32513805400006,11.6,7.87210409899998));
#244802=CARTESIAN_POINT('Ctrl Pts',(-7.32731634900006,15.2,7.87341499399999));
#244803=CARTESIAN_POINT('Ctrl Pts',(-7.32731634900006,11.6,7.87341499399999));
#244804=CARTESIAN_POINT('Ctrl Pts',(-7.32950098000006,15.2,7.87472715499998));
#244805=CARTESIAN_POINT('Ctrl Pts',(-7.32950098000006,11.6,7.87472715499998));
#244806=CARTESIAN_POINT('Ctrl Pts',(-7.33169194400006,15.2,7.87604056899998));
#244807=CARTESIAN_POINT('Ctrl Pts',(-7.33169194400006,11.6,7.87604056899998));
#244808=CARTESIAN_POINT('Ctrl Pts',(-7.33388923300006,15.2,7.87735522199998));
#244809=CARTESIAN_POINT('Ctrl Pts',(-7.33388923300006,11.6,7.87735522199998));
#244810=CARTESIAN_POINT('Ctrl Pts',(-7.33609284400006,15.2,7.87867109999999));
#244811=CARTESIAN_POINT('Ctrl Pts',(-7.33609284400006,11.6,7.87867109999999));
#244812=CARTESIAN_POINT('Ctrl Pts',(-7.33830277000005,15.2,7.87998818899998));
#244813=CARTESIAN_POINT('Ctrl Pts',(-7.33830277000005,11.6,7.87998818899998));
#244814=CARTESIAN_POINT('Ctrl Pts',(-7.34051900600006,15.2,7.88130647499998));
#244815=CARTESIAN_POINT('Ctrl Pts',(-7.34051900600006,11.6,7.88130647499998));
#244816=CARTESIAN_POINT('Ctrl Pts',(-7.34274154700006,15.2,7.88262594599999));
#244817=CARTESIAN_POINT('Ctrl Pts',(-7.34274154700006,11.6,7.88262594599999));
#244818=CARTESIAN_POINT('Ctrl Pts',(-7.34497038800006,15.2,7.88394658699998));
#244819=CARTESIAN_POINT('Ctrl Pts',(-7.34497038800006,11.6,7.88394658699998));
#244820=CARTESIAN_POINT('Ctrl Pts',(-7.34720552300006,15.2,7.88526838399999));
#244821=CARTESIAN_POINT('Ctrl Pts',(-7.34720552300006,11.6,7.88526838399999));
#244822=CARTESIAN_POINT('Ctrl Pts',(-7.34944694700006,15.2,7.88659132499999));
#244823=CARTESIAN_POINT('Ctrl Pts',(-7.34944694700006,11.6,7.88659132499999));
#244824=CARTESIAN_POINT('Ctrl Pts',(-7.35169465500006,15.2,7.88791539599998));
#244825=CARTESIAN_POINT('Ctrl Pts',(-7.35169465500006,11.6,7.88791539599998));
#244826=CARTESIAN_POINT('Ctrl Pts',(-7.35394864100006,15.2,7.88924058299998));
#244827=CARTESIAN_POINT('Ctrl Pts',(-7.35394864100006,11.6,7.88924058299998));
#244828=CARTESIAN_POINT('Ctrl Pts',(-7.35620890000006,15.2,7.89056687299999));
#244829=CARTESIAN_POINT('Ctrl Pts',(-7.35620890000006,11.6,7.89056687299999));
#244830=CARTESIAN_POINT('Ctrl Pts',(-7.35847542700006,15.2,7.89189425299998));
#244831=CARTESIAN_POINT('Ctrl Pts',(-7.35847542700006,11.6,7.89189425299998));
#244832=CARTESIAN_POINT('Ctrl Pts',(-7.36074821700006,15.2,7.89322270699999));
#244833=CARTESIAN_POINT('Ctrl Pts',(-7.36074821700006,11.6,7.89322270699999));
#244834=CARTESIAN_POINT('Ctrl Pts',(-7.36302726400006,15.2,7.89455222599998));
#244835=CARTESIAN_POINT('Ctrl Pts',(-7.36302726400006,11.6,7.89455222599998));
#244836=CARTESIAN_POINT('Ctrl Pts',(-7.36531256300006,15.2,7.89588279499998));
#244837=CARTESIAN_POINT('Ctrl Pts',(-7.36531256300006,11.6,7.89588279499998));
#244838=CARTESIAN_POINT('Ctrl Pts',(-7.36760410800006,15.2,7.89721439899999));
#244839=CARTESIAN_POINT('Ctrl Pts',(-7.36760410800006,11.6,7.89721439899999));
#244840=CARTESIAN_POINT('Ctrl Pts',(-7.36990189600006,15.2,7.89854702799998));
#244841=CARTESIAN_POINT('Ctrl Pts',(-7.36990189600006,11.6,7.89854702799998));
#244842=CARTESIAN_POINT('Ctrl Pts',(-7.37220591900006,15.2,7.89988066499999));
#244843=CARTESIAN_POINT('Ctrl Pts',(-7.37220591900006,11.6,7.89988066499999));
#244844=CARTESIAN_POINT('Ctrl Pts',(-7.37451617400006,15.2,7.90121529999999));
#244845=CARTESIAN_POINT('Ctrl Pts',(-7.37451617400006,11.6,7.90121529999999));
#244846=CARTESIAN_POINT('Ctrl Pts',(-7.37683265400006,15.2,7.90255091899999));
#244847=CARTESIAN_POINT('Ctrl Pts',(-7.37683265400006,11.6,7.90255091899999));
#244848=CARTESIAN_POINT('Ctrl Pts',(-7.37915535500006,15.2,7.90388750999998));
#244849=CARTESIAN_POINT('Ctrl Pts',(-7.37915535500006,11.6,7.90388750999998));
#244850=CARTESIAN_POINT('Ctrl Pts',(-7.38148427100006,15.2,7.90522505699998));
#244851=CARTESIAN_POINT('Ctrl Pts',(-7.38148427100006,11.6,7.90522505699998));
#244852=CARTESIAN_POINT('Ctrl Pts',(-7.38381939700006,15.2,7.90656354999999));
#244853=CARTESIAN_POINT('Ctrl Pts',(-7.38381939700006,11.6,7.90656354999999));
#244854=CARTESIAN_POINT('Ctrl Pts',(-7.38616072800006,15.2,7.90790297499999));
#244855=CARTESIAN_POINT('Ctrl Pts',(-7.38616072800006,11.6,7.90790297499999));
#244856=CARTESIAN_POINT('Ctrl Pts',(-7.38850825800006,15.2,7.90924331999998));
#244857=CARTESIAN_POINT('Ctrl Pts',(-7.38850825800006,11.6,7.90924331999998));
#244858=CARTESIAN_POINT('Ctrl Pts',(-7.39086198300006,15.2,7.91058456999998));
#244859=CARTESIAN_POINT('Ctrl Pts',(-7.39086198300006,11.6,7.91058456999998));
#244860=CARTESIAN_POINT('Ctrl Pts',(-7.39322189600006,15.2,7.91192671399998));
#244861=CARTESIAN_POINT('Ctrl Pts',(-7.39322189600006,11.6,7.91192671399998));
#244862=CARTESIAN_POINT('Ctrl Pts',(-7.39558799400006,15.2,7.91326973999999));
#244863=CARTESIAN_POINT('Ctrl Pts',(-7.39558799400006,11.6,7.91326973999999));
#244864=CARTESIAN_POINT('Ctrl Pts',(-7.39796027100006,15.2,7.91461363299998));
#244865=CARTESIAN_POINT('Ctrl Pts',(-7.39796027100006,11.6,7.91461363299998));
#244866=CARTESIAN_POINT('Ctrl Pts',(-7.40033872100006,15.2,7.91595838099998));
#244867=CARTESIAN_POINT('Ctrl Pts',(-7.40033872100006,11.6,7.91595838099998));
#244868=CARTESIAN_POINT('Ctrl Pts',(-7.40272333900006,15.2,7.91730397299999));
#244869=CARTESIAN_POINT('Ctrl Pts',(-7.40272333900006,11.6,7.91730397299999));
#244870=CARTESIAN_POINT('Ctrl Pts',(-7.40511412000005,15.2,7.91865039499999));
#244871=CARTESIAN_POINT('Ctrl Pts',(-7.40511412000005,11.6,7.91865039499999));
#244872=CARTESIAN_POINT('Ctrl Pts',(-7.40751105900006,15.2,7.91999763299999));
#244873=CARTESIAN_POINT('Ctrl Pts',(-7.40751105900006,11.6,7.91999763299999));
#244874=CARTESIAN_POINT('Ctrl Pts',(-7.40991415200006,15.2,7.92134567699998));
#244875=CARTESIAN_POINT('Ctrl Pts',(-7.40991415200006,11.6,7.92134567699998));
#244876=CARTESIAN_POINT('Ctrl Pts',(-7.41232339100006,15.2,7.92269451299998));
#244877=CARTESIAN_POINT('Ctrl Pts',(-7.41232339100006,11.6,7.92269451299998));
#244878=CARTESIAN_POINT('Ctrl Pts',(-7.41473877300006,15.2,7.92404412999999));
#244879=CARTESIAN_POINT('Ctrl Pts',(-7.41473877300006,11.6,7.92404412999999));
#244880=CARTESIAN_POINT('Ctrl Pts',(-7.41716029100006,15.2,7.92539451399998));
#244881=CARTESIAN_POINT('Ctrl Pts',(-7.41716029100006,11.6,7.92539451399998));
#244882=CARTESIAN_POINT('Ctrl Pts',(-7.41958794200006,15.2,7.92674565199999));
#244883=CARTESIAN_POINT('Ctrl Pts',(-7.41958794200006,11.6,7.92674565199999));
#244884=CARTESIAN_POINT('Ctrl Pts',(-7.42202171900006,15.2,7.92809753399998));
#244885=CARTESIAN_POINT('Ctrl Pts',(-7.42202171900006,11.6,7.92809753399998));
#244886=CARTESIAN_POINT('Ctrl Pts',(-7.42446161900006,15.2,7.92945014599999));
#244887=CARTESIAN_POINT('Ctrl Pts',(-7.42446161900006,11.6,7.92945014599999));
#244888=CARTESIAN_POINT('Ctrl Pts',(-7.42690763400006,15.2,7.93080347599999));
#244889=CARTESIAN_POINT('Ctrl Pts',(-7.42690763400006,11.6,7.93080347599999));
#244890=CARTESIAN_POINT('Ctrl Pts',(-7.42935976100005,15.2,7.93215751199998));
#244891=CARTESIAN_POINT('Ctrl Pts',(-7.42935976100005,11.6,7.93215751199998));
#244892=CARTESIAN_POINT('Ctrl Pts',(-7.43181799400006,15.2,7.93351224099998));
#244893=CARTESIAN_POINT('Ctrl Pts',(-7.43181799400006,11.6,7.93351224099998));
#244894=CARTESIAN_POINT('Ctrl Pts',(-7.43428232700006,15.2,7.93486765199999));
#244895=CARTESIAN_POINT('Ctrl Pts',(-7.43428232700006,11.6,7.93486765199999));
#244896=CARTESIAN_POINT('Ctrl Pts',(-7.43675275700006,15.2,7.93622373199998));
#244897=CARTESIAN_POINT('Ctrl Pts',(-7.43675275700006,11.6,7.93622373199998));
#244898=CARTESIAN_POINT('Ctrl Pts',(-7.43922927800006,15.2,7.93758046899999));
#244899=CARTESIAN_POINT('Ctrl Pts',(-7.43922927800006,11.6,7.93758046899999));
#244900=CARTESIAN_POINT('Ctrl Pts',(-7.44171188300006,15.2,7.93893784999998));
#244901=CARTESIAN_POINT('Ctrl Pts',(-7.44171188300006,11.6,7.93893784999998));
#244902=CARTESIAN_POINT('Ctrl Pts',(-7.44420057000006,15.2,7.94029586499998));
#244903=CARTESIAN_POINT('Ctrl Pts',(-7.44420057000006,11.6,7.94029586499998));
#244904=CARTESIAN_POINT('Ctrl Pts',(-7.44669533100006,15.2,7.94165450099998));
#244905=CARTESIAN_POINT('Ctrl Pts',(-7.44669533100006,11.6,7.94165450099998));
#244906=CARTESIAN_POINT('Ctrl Pts',(-7.44919616200006,15.2,7.94301374399998));
#244907=CARTESIAN_POINT('Ctrl Pts',(-7.44919616200006,11.6,7.94301374399998));
#244908=CARTESIAN_POINT('Ctrl Pts',(-7.45170305800006,15.2,7.94437358599998));
#244909=CARTESIAN_POINT('Ctrl Pts',(-7.45170305800006,11.6,7.94437358599998));
#244910=CARTESIAN_POINT('Ctrl Pts',(-7.45421601400006,15.2,7.94573401099999));
#244911=CARTESIAN_POINT('Ctrl Pts',(-7.45421601400006,11.6,7.94573401099999));
#244912=CARTESIAN_POINT('Ctrl Pts',(-7.45673502500006,15.2,7.94709500999998));
#244913=CARTESIAN_POINT('Ctrl Pts',(-7.45673502500006,11.6,7.94709500999998));
#244914=CARTESIAN_POINT('Ctrl Pts',(-7.45926008500006,15.2,7.94845657099999));
#244915=CARTESIAN_POINT('Ctrl Pts',(-7.45926008500006,11.6,7.94845657099999));
#244916=CARTESIAN_POINT('Ctrl Pts',(-7.46179119000006,15.2,7.94981867899998));
#244917=CARTESIAN_POINT('Ctrl Pts',(-7.46179119000006,11.6,7.94981867899998));
#244918=CARTESIAN_POINT('Ctrl Pts',(-7.46432833400006,15.2,7.95118132499999));
#244919=CARTESIAN_POINT('Ctrl Pts',(-7.46432833400006,11.6,7.95118132499999));
#244920=CARTESIAN_POINT('Ctrl Pts',(-7.46687151300006,15.2,7.95254449699998));
#244921=CARTESIAN_POINT('Ctrl Pts',(-7.46687151300006,11.6,7.95254449699998));
#244922=CARTESIAN_POINT('Ctrl Pts',(-7.46942072000006,15.2,7.95390818299998));
#244923=CARTESIAN_POINT('Ctrl Pts',(-7.46942072000006,11.6,7.95390818299998));
#244924=CARTESIAN_POINT('Ctrl Pts',(-7.47197595100006,15.2,7.95527237099999));
#244925=CARTESIAN_POINT('Ctrl Pts',(-7.47197595100006,11.6,7.95527237099999));
#244926=CARTESIAN_POINT('Ctrl Pts',(-7.47453720200006,15.2,7.95663704999999));
#244927=CARTESIAN_POINT('Ctrl Pts',(-7.47453720200006,11.6,7.95663704999999));
#244928=CARTESIAN_POINT('Ctrl Pts',(-7.47710446500006,15.2,7.95800220799999));
#244929=CARTESIAN_POINT('Ctrl Pts',(-7.47710446500006,11.6,7.95800220799999));
#244930=CARTESIAN_POINT('Ctrl Pts',(-7.47967773800006,15.2,7.95936783099998));
#244931=CARTESIAN_POINT('Ctrl Pts',(-7.47967773800006,11.6,7.95936783099998));
#244932=CARTESIAN_POINT('Ctrl Pts',(-7.48225701500006,15.2,7.96073391199998));
#244933=CARTESIAN_POINT('Ctrl Pts',(-7.48225701500006,11.6,7.96073391199998));
#244934=CARTESIAN_POINT('Ctrl Pts',(-7.48484228800006,15.2,7.96210043599999));
#244935=CARTESIAN_POINT('Ctrl Pts',(-7.48484228800006,11.6,7.96210043599999));
#244936=CARTESIAN_POINT('Ctrl Pts',(-7.48743355700006,15.2,7.96346739199999));
#244937=CARTESIAN_POINT('Ctrl Pts',(-7.48743355700006,11.6,7.96346739199999));
#244938=CARTESIAN_POINT('Ctrl Pts',(-7.49003081300006,15.2,7.96483476999998));
#244939=CARTESIAN_POINT('Ctrl Pts',(-7.49003081300006,11.6,7.96483476999998));
#244940=CARTESIAN_POINT('Ctrl Pts',(-7.49263405300006,15.2,7.96620255599999));
#244941=CARTESIAN_POINT('Ctrl Pts',(-7.49263405300006,11.6,7.96620255599999));
#244942=CARTESIAN_POINT('Ctrl Pts',(-7.49524327100006,15.2,7.96757074199999));
#244943=CARTESIAN_POINT('Ctrl Pts',(-7.49524327100006,11.6,7.96757074199999));
#244944=CARTESIAN_POINT('Ctrl Pts',(-7.49785846200006,15.2,7.96893931299999));
#244945=CARTESIAN_POINT('Ctrl Pts',(-7.49785846200006,11.6,7.96893931299999));
#244946=CARTESIAN_POINT('Ctrl Pts',(-7.50047962100006,15.2,7.97030825999999));
#244947=CARTESIAN_POINT('Ctrl Pts',(-7.50047962100006,11.6,7.97030825999999));
#244948=CARTESIAN_POINT('Ctrl Pts',(-7.50310674300006,15.2,7.97167757099999));
#244949=CARTESIAN_POINT('Ctrl Pts',(-7.50310674300006,11.6,7.97167757099999));
#244950=CARTESIAN_POINT('Ctrl Pts',(-7.50573982300006,15.2,7.97304723499998));
#244951=CARTESIAN_POINT('Ctrl Pts',(-7.50573982300006,11.6,7.97304723499998));
#244952=CARTESIAN_POINT('Ctrl Pts',(-7.50837885500006,15.2,7.97441723899999));
#244953=CARTESIAN_POINT('Ctrl Pts',(-7.50837885500006,11.6,7.97441723899999));
#244954=CARTESIAN_POINT('Ctrl Pts',(-7.51102383600006,15.2,7.97578757299998));
#244955=CARTESIAN_POINT('Ctrl Pts',(-7.51102383600006,11.6,7.97578757299998));
#244956=CARTESIAN_POINT('Ctrl Pts',(-7.51367475900006,15.2,7.97715822699999));
#244957=CARTESIAN_POINT('Ctrl Pts',(-7.51367475900006,11.6,7.97715822699999));
#244958=CARTESIAN_POINT('Ctrl Pts',(-7.51633162000005,15.2,7.97852918799999));
#244959=CARTESIAN_POINT('Ctrl Pts',(-7.51633162000005,11.6,7.97852918799999));
#244960=CARTESIAN_POINT('Ctrl Pts',(-7.51899441200005,15.2,7.97990044499999));
#244961=CARTESIAN_POINT('Ctrl Pts',(-7.51899441200005,11.6,7.97990044499999));
#244962=CARTESIAN_POINT('Ctrl Pts',(-7.52166313300006,15.2,7.98127198799998));
#244963=CARTESIAN_POINT('Ctrl Pts',(-7.52166313300006,11.6,7.98127198799998));
#244964=CARTESIAN_POINT('Ctrl Pts',(-7.52433777600006,15.2,7.98264380499998));
#244965=CARTESIAN_POINT('Ctrl Pts',(-7.52433777600006,11.6,7.98264380499998));
#244966=CARTESIAN_POINT('Ctrl Pts',(-7.52701833700005,15.2,7.98401588399998));
#244967=CARTESIAN_POINT('Ctrl Pts',(-7.52701833700005,11.6,7.98401588399998));
#244968=CARTESIAN_POINT('Ctrl Pts',(-7.52970481000006,15.2,7.98538821699999));
#244969=CARTESIAN_POINT('Ctrl Pts',(-7.52970481000006,11.6,7.98538821699999));
#244970=CARTESIAN_POINT('Ctrl Pts',(-7.53239719100005,15.2,7.98676078899998));
#244971=CARTESIAN_POINT('Ctrl Pts',(-7.53239719100005,11.6,7.98676078899998));
#244972=CARTESIAN_POINT('Ctrl Pts',(-7.53509547300006,15.2,7.98813359199999));
#244973=CARTESIAN_POINT('Ctrl Pts',(-7.53509547300006,11.6,7.98813359199999));
#244974=CARTESIAN_POINT('Ctrl Pts',(-7.53779965400006,15.2,7.98950661499998));
#244975=CARTESIAN_POINT('Ctrl Pts',(-7.53779965400006,11.6,7.98950661499998));
#244976=CARTESIAN_POINT('Ctrl Pts',(-7.54050972500006,15.2,7.99087984499998));
#244977=CARTESIAN_POINT('Ctrl Pts',(-7.54050972500006,11.6,7.99087984499998));
#244978=CARTESIAN_POINT('Ctrl Pts',(-7.54322568500006,15.2,7.99225327099998));
#244979=CARTESIAN_POINT('Ctrl Pts',(-7.54322568500006,11.6,7.99225327099998));
#244980=CARTESIAN_POINT('Ctrl Pts',(-7.54594752700006,15.2,7.99362688499999));
#244981=CARTESIAN_POINT('Ctrl Pts',(-7.54594752700006,11.6,7.99362688499999));
#244982=CARTESIAN_POINT('Ctrl Pts',(-7.54867524600006,15.2,7.99500067299999));
#244983=CARTESIAN_POINT('Ctrl Pts',(-7.54867524600006,11.6,7.99500067299999));
#244984=CARTESIAN_POINT('Ctrl Pts',(-7.55140883700006,15.2,7.99637462699998));
#244985=CARTESIAN_POINT('Ctrl Pts',(-7.55140883700006,11.6,7.99637462699998));
#244986=CARTESIAN_POINT('Ctrl Pts',(-7.55414829500006,15.2,7.99774873399999));
#244987=CARTESIAN_POINT('Ctrl Pts',(-7.55414829500006,11.6,7.99774873399999));
#244988=CARTESIAN_POINT('Ctrl Pts',(-7.55689361600006,15.2,7.99912298399998));
#244989=CARTESIAN_POINT('Ctrl Pts',(-7.55689361600006,11.6,7.99912298399998));
#244990=CARTESIAN_POINT('Ctrl Pts',(-7.55964479300006,15.2,8.00049736599998));
#244991=CARTESIAN_POINT('Ctrl Pts',(-7.55964479300006,11.6,8.00049736599998));
#244992=CARTESIAN_POINT('Ctrl Pts',(-7.56240182300005,15.2,8.00187187099999));
#244993=CARTESIAN_POINT('Ctrl Pts',(-7.56240182300005,11.6,8.00187187099999));
#244994=CARTESIAN_POINT('Ctrl Pts',(-7.56516470000006,15.2,8.00324648399998));
#244995=CARTESIAN_POINT('Ctrl Pts',(-7.56516470000006,11.6,8.00324648399998));
#244996=CARTESIAN_POINT('Ctrl Pts',(-7.56793341800006,15.2,8.00462119899999));
#244997=CARTESIAN_POINT('Ctrl Pts',(-7.56793341800006,11.6,8.00462119899999));
#244998=CARTESIAN_POINT('Ctrl Pts',(-7.57070797500005,15.2,8.00599600399998));
#244999=CARTESIAN_POINT('Ctrl Pts',(-7.57070797500005,11.6,8.00599600399998));
#245000=CARTESIAN_POINT('Ctrl Pts',(-7.57348836300006,15.2,8.00737088699999));
#245001=CARTESIAN_POINT('Ctrl Pts',(-7.57348836300006,11.6,8.00737088699999));
#245002=CARTESIAN_POINT('Ctrl Pts',(-7.57627457800006,15.2,8.00874583799999));
#245003=CARTESIAN_POINT('Ctrl Pts',(-7.57627457800006,11.6,8.00874583799999));
#245004=CARTESIAN_POINT('Ctrl Pts',(-7.57906661600006,15.2,8.01012084699998));
#245005=CARTESIAN_POINT('Ctrl Pts',(-7.57906661600006,11.6,8.01012084699998));
#245006=CARTESIAN_POINT('Ctrl Pts',(-7.58186447000006,15.2,8.01149590299998));
#245007=CARTESIAN_POINT('Ctrl Pts',(-7.58186447000006,11.6,8.01149590299998));
#245008=CARTESIAN_POINT('Ctrl Pts',(-7.58466813600006,15.2,8.01287099699999));
#245009=CARTESIAN_POINT('Ctrl Pts',(-7.58466813600006,11.6,8.01287099699999));
#245010=CARTESIAN_POINT('Ctrl Pts',(-7.58747761100006,15.2,8.01424611599998));
#245011=CARTESIAN_POINT('Ctrl Pts',(-7.58747761100006,11.6,8.01424611599998));
#245012=CARTESIAN_POINT('Ctrl Pts',(-7.59029288700006,15.2,8.01562125099998));
#245013=CARTESIAN_POINT('Ctrl Pts',(-7.59029288700006,11.6,8.01562125099998));
#245014=CARTESIAN_POINT('Ctrl Pts',(-7.59311396000006,15.2,8.01699639099999));
#245015=CARTESIAN_POINT('Ctrl Pts',(-7.59311396000006,11.6,8.01699639099999));
#245016=CARTESIAN_POINT('Ctrl Pts',(-7.59594082600006,15.2,8.01837152699999));
#245017=CARTESIAN_POINT('Ctrl Pts',(-7.59594082600006,11.6,8.01837152699999));
#245018=CARTESIAN_POINT('Ctrl Pts',(-7.59877347800006,15.2,8.01974664699999));
#245019=CARTESIAN_POINT('Ctrl Pts',(-7.59877347800006,11.6,8.01974664699999));
#245020=CARTESIAN_POINT('Ctrl Pts',(-7.60161191400006,15.2,8.02112174099998));
#245021=CARTESIAN_POINT('Ctrl Pts',(-7.60161191400006,11.6,8.02112174099998));
#245022=CARTESIAN_POINT('Ctrl Pts',(-7.60445612600006,15.2,8.02249679899998));
#245023=CARTESIAN_POINT('Ctrl Pts',(-7.60445612600006,11.6,8.02249679899998));
#245024=CARTESIAN_POINT('Ctrl Pts',(-7.60730611100006,15.2,8.02387180999999));
#245025=CARTESIAN_POINT('Ctrl Pts',(-7.60730611100006,11.6,8.02387180999999));
#245026=CARTESIAN_POINT('Ctrl Pts',(-7.61016186300005,15.2,8.02524676499999));
#245027=CARTESIAN_POINT('Ctrl Pts',(-7.61016186300005,11.6,8.02524676499999));
#245028=CARTESIAN_POINT('Ctrl Pts',(-7.61302337700006,15.2,8.02662165399998));
#245029=CARTESIAN_POINT('Ctrl Pts',(-7.61302337700006,11.6,8.02662165399998));
#245030=CARTESIAN_POINT('Ctrl Pts',(-7.61589065000006,15.2,8.02799646399999));
#245031=CARTESIAN_POINT('Ctrl Pts',(-7.61589065000006,11.6,8.02799646399999));
#245032=CARTESIAN_POINT('Ctrl Pts',(-7.61876367500006,15.2,8.02937118799999));
#245033=CARTESIAN_POINT('Ctrl Pts',(-7.61876367500006,11.6,8.02937118799999));
#245034=CARTESIAN_POINT('Ctrl Pts',(-7.62164244700006,15.2,8.03074581399999));
#245035=CARTESIAN_POINT('Ctrl Pts',(-7.62164244700006,11.6,8.03074581399999));
#245036=CARTESIAN_POINT('Ctrl Pts',(-7.62452696100006,15.2,8.03212033199999));
#245037=CARTESIAN_POINT('Ctrl Pts',(-7.62452696100006,11.6,8.03212033199999));
#245038=CARTESIAN_POINT('Ctrl Pts',(-7.62741721300006,15.2,8.03349473299999));
#245039=CARTESIAN_POINT('Ctrl Pts',(-7.62741721300006,11.6,8.03349473299999));
#245040=CARTESIAN_POINT('Ctrl Pts',(-7.63031319900006,15.2,8.03486900599999));
#245041=CARTESIAN_POINT('Ctrl Pts',(-7.63031319900006,11.6,8.03486900599999));
#245042=CARTESIAN_POINT('Ctrl Pts',(-7.63321491200006,15.2,8.03624313999999));
#245043=CARTESIAN_POINT('Ctrl Pts',(-7.63321491200006,11.6,8.03624313999999));
#245044=CARTESIAN_POINT('Ctrl Pts',(-7.63612234700006,15.2,8.03761712699998));
#245045=CARTESIAN_POINT('Ctrl Pts',(-7.63612234700006,11.6,8.03761712699998));
#245046=CARTESIAN_POINT('Ctrl Pts',(-7.63903550100006,15.2,8.03899095599999));
#245047=CARTESIAN_POINT('Ctrl Pts',(-7.63903550100006,11.6,8.03899095599999));
#245048=CARTESIAN_POINT('Ctrl Pts',(-7.64195436800006,15.2,8.04036461599999));
#245049=CARTESIAN_POINT('Ctrl Pts',(-7.64195436800006,11.6,8.04036461599999));
#245050=CARTESIAN_POINT('Ctrl Pts',(-7.64487894200006,15.2,8.04173809899999));
#245051=CARTESIAN_POINT('Ctrl Pts',(-7.64487894200006,11.6,8.04173809899999));
#245052=CARTESIAN_POINT('Ctrl Pts',(-7.64780922000006,15.2,8.04311139499998));
#245053=CARTESIAN_POINT('Ctrl Pts',(-7.64780922000006,11.6,8.04311139499998));
#245054=CARTESIAN_POINT('Ctrl Pts',(-7.65074519600006,15.2,8.04448449199998));
#245055=CARTESIAN_POINT('Ctrl Pts',(-7.65074519600006,11.6,8.04448449199998));
#245056=CARTESIAN_POINT('Ctrl Pts',(-7.65368686500006,15.2,8.04585738099998));
#245057=CARTESIAN_POINT('Ctrl Pts',(-7.65368686500006,11.6,8.04585738099998));
#245058=CARTESIAN_POINT('Ctrl Pts',(-7.65663422300006,15.2,8.04723005299999));
#245059=CARTESIAN_POINT('Ctrl Pts',(-7.65663422300006,11.6,8.04723005299999));
#245060=CARTESIAN_POINT('Ctrl Pts',(-7.65958726300005,15.2,8.04860249699999));
#245061=CARTESIAN_POINT('Ctrl Pts',(-7.65958726300005,11.6,8.04860249699999));
#245062=CARTESIAN_POINT('Ctrl Pts',(-7.66254598200005,15.2,8.04997470299998));
#245063=CARTESIAN_POINT('Ctrl Pts',(-7.66254598200005,11.6,8.04997470299998));
#245064=CARTESIAN_POINT('Ctrl Pts',(-7.66551037500006,15.2,8.05134666399999));
#245065=CARTESIAN_POINT('Ctrl Pts',(-7.66551037500006,11.6,8.05134666399999));
#245066=CARTESIAN_POINT('Ctrl Pts',(-7.66848043700006,15.2,8.05271836699998));
#245067=CARTESIAN_POINT('Ctrl Pts',(-7.66848043700006,11.6,8.05271836699998));
#245068=CARTESIAN_POINT('Ctrl Pts',(-7.67145616200006,15.2,8.05408980299998));
#245069=CARTESIAN_POINT('Ctrl Pts',(-7.67145616200006,11.6,8.05408980299998));
#245070=CARTESIAN_POINT('Ctrl Pts',(-7.67443754600006,15.2,8.05546096299998));
#245071=CARTESIAN_POINT('Ctrl Pts',(-7.67443754600006,11.6,8.05546096299998));
#245072=CARTESIAN_POINT('Ctrl Pts',(-7.67742458300006,15.2,8.05683183699998));
#245073=CARTESIAN_POINT('Ctrl Pts',(-7.67742458300006,11.6,8.05683183699998));
#245074=CARTESIAN_POINT('Ctrl Pts',(-7.68041727000006,15.2,8.05820241499998));
#245075=CARTESIAN_POINT('Ctrl Pts',(-7.68041727000006,11.6,8.05820241499998));
#245076=CARTESIAN_POINT('Ctrl Pts',(-7.68341560100006,15.2,8.05957268799999));
#245077=CARTESIAN_POINT('Ctrl Pts',(-7.68341560100006,11.6,8.05957268799999));
#245078=CARTESIAN_POINT('Ctrl Pts',(-7.68641957100006,15.2,8.06094264599999));
#245079=CARTESIAN_POINT('Ctrl Pts',(-7.68641957100006,11.6,8.06094264599999));
#245080=CARTESIAN_POINT('Ctrl Pts',(-7.68942917500006,15.2,8.06231227899998));
#245081=CARTESIAN_POINT('Ctrl Pts',(-7.68942917500006,11.6,8.06231227899998));
#245082=CARTESIAN_POINT('Ctrl Pts',(-7.69244440900006,15.2,8.06368157799999));
#245083=CARTESIAN_POINT('Ctrl Pts',(-7.69244440900006,11.6,8.06368157799999));
#245084=CARTESIAN_POINT('Ctrl Pts',(-7.69546526600006,15.2,8.06505053299999));
#245085=CARTESIAN_POINT('Ctrl Pts',(-7.69546526600006,11.6,8.06505053299999));
#245086=CARTESIAN_POINT('Ctrl Pts',(-7.69849174400005,15.2,8.06641913399999));
#245087=CARTESIAN_POINT('Ctrl Pts',(-7.69849174400005,11.6,8.06641913399999));
#245088=CARTESIAN_POINT('Ctrl Pts',(-7.70152383600006,15.2,8.06778737399998));
#245089=CARTESIAN_POINT('Ctrl Pts',(-7.70152383600006,11.6,8.06778737399998));
#245090=CARTESIAN_POINT('Ctrl Pts',(-7.70456153900006,15.2,8.06915523999999));
#245091=CARTESIAN_POINT('Ctrl Pts',(-7.70456153900006,11.6,8.06915523999999));
#245092=CARTESIAN_POINT('Ctrl Pts',(-7.70760484600006,15.2,8.07052272399999));
#245093=CARTESIAN_POINT('Ctrl Pts',(-7.70760484600006,11.6,8.07052272399999));
#245094=CARTESIAN_POINT('Ctrl Pts',(-7.71065375300005,15.2,8.07188981699999));
#245095=CARTESIAN_POINT('Ctrl Pts',(-7.71065375300005,11.6,8.07188981699999));
#245096=CARTESIAN_POINT('Ctrl Pts',(-7.71370825500006,15.2,8.07325650899998));
#245097=CARTESIAN_POINT('Ctrl Pts',(-7.71370825500006,11.6,8.07325650899998));
#245098=CARTESIAN_POINT('Ctrl Pts',(-7.71676834800005,15.2,8.07462279199999));
#245099=CARTESIAN_POINT('Ctrl Pts',(-7.71676834800005,11.6,8.07462279199999));
#245100=CARTESIAN_POINT('Ctrl Pts',(-7.71983402500006,15.2,8.07598865399999));
#245101=CARTESIAN_POINT('Ctrl Pts',(-7.71983402500006,11.6,8.07598865399999));
#245102=CARTESIAN_POINT('Ctrl Pts',(-7.72290528400006,15.2,8.07735408899998));
#245103=CARTESIAN_POINT('Ctrl Pts',(-7.72290528400006,11.6,8.07735408899998));
#245104=CARTESIAN_POINT('Ctrl Pts',(-7.72598211700006,15.2,8.07871908399999));
#245105=CARTESIAN_POINT('Ctrl Pts',(-7.72598211700006,11.6,8.07871908399999));
#245106=CARTESIAN_POINT('Ctrl Pts',(-7.72906452200005,15.2,8.08008363199999));
#245107=CARTESIAN_POINT('Ctrl Pts',(-7.72906452200005,11.6,8.08008363199999));
#245108=CARTESIAN_POINT('Ctrl Pts',(-7.73215249300006,15.2,8.08144772299999));
#245109=CARTESIAN_POINT('Ctrl Pts',(-7.73215249300006,11.6,8.08144772299999));
#245110=CARTESIAN_POINT('Ctrl Pts',(-7.73524602400006,15.2,8.08281134799999));
#245111=CARTESIAN_POINT('Ctrl Pts',(-7.73524602400006,11.6,8.08281134799999));
#245112=CARTESIAN_POINT('Ctrl Pts',(-7.73834511100005,15.2,8.08417449699999));
#245113=CARTESIAN_POINT('Ctrl Pts',(-7.73834511100005,11.6,8.08417449699999));
#245114=CARTESIAN_POINT('Ctrl Pts',(-7.74144975100005,15.2,8.08553716199999));
#245115=CARTESIAN_POINT('Ctrl Pts',(-7.74144975100005,11.6,8.08553716199999));
#245116=CARTESIAN_POINT('Ctrl Pts',(-7.74455993600006,15.2,8.08689933299998));
#245117=CARTESIAN_POINT('Ctrl Pts',(-7.74455993600006,11.6,8.08689933299998));
#245118=CARTESIAN_POINT('Ctrl Pts',(-7.74767566300006,15.2,8.08826100099999));
#245119=CARTESIAN_POINT('Ctrl Pts',(-7.74767566300006,11.6,8.08826100099999));
#245120=CARTESIAN_POINT('Ctrl Pts',(-7.75079692700006,15.2,8.08962215699999));
#245121=CARTESIAN_POINT('Ctrl Pts',(-7.75079692700006,11.6,8.08962215699999));
#245122=CARTESIAN_POINT('Ctrl Pts',(-7.75392372200006,15.2,8.09098279099998));
#245123=CARTESIAN_POINT('Ctrl Pts',(-7.75392372200006,11.6,8.09098279099998));
#245124=CARTESIAN_POINT('Ctrl Pts',(-7.75705604400006,15.2,8.09234289499998));
#245125=CARTESIAN_POINT('Ctrl Pts',(-7.75705604400006,11.6,8.09234289499998));
#245126=CARTESIAN_POINT('Ctrl Pts',(-7.76019388900006,15.2,8.09370245899999));
#245127=CARTESIAN_POINT('Ctrl Pts',(-7.76019388900006,11.6,8.09370245899999));
#245128=CARTESIAN_POINT('Ctrl Pts',(-7.76333725000006,15.2,8.09506147499999));
#245129=CARTESIAN_POINT('Ctrl Pts',(-7.76333725000006,11.6,8.09506147499999));
#245130=CARTESIAN_POINT('Ctrl Pts',(-7.76648612500006,15.2,8.09641993199998));
#245131=CARTESIAN_POINT('Ctrl Pts',(-7.76648612500006,11.6,8.09641993199998));
#245132=CARTESIAN_POINT('Ctrl Pts',(-7.76964050600006,15.2,8.09777782399999));
#245133=CARTESIAN_POINT('Ctrl Pts',(-7.76964050600006,11.6,8.09777782399999));
#245134=CARTESIAN_POINT('Ctrl Pts',(-7.77280039100006,15.2,8.09913513899998));
#245135=CARTESIAN_POINT('Ctrl Pts',(-7.77280039100006,11.6,8.09913513899998));
#245136=CARTESIAN_POINT('Ctrl Pts',(-7.77596577300006,15.2,8.10049186899998));
#245137=CARTESIAN_POINT('Ctrl Pts',(-7.77596577300006,11.6,8.10049186899998));
#245138=CARTESIAN_POINT('Ctrl Pts',(-7.77913664800005,15.2,8.10184800599998));
#245139=CARTESIAN_POINT('Ctrl Pts',(-7.77913664800005,11.6,8.10184800599998));
#245140=CARTESIAN_POINT('Ctrl Pts',(-7.78231301200006,15.2,8.10320353899998));
#245141=CARTESIAN_POINT('Ctrl Pts',(-7.78231301200006,11.6,8.10320353899998));
#245142=CARTESIAN_POINT('Ctrl Pts',(-7.78549485900006,15.2,8.10455846299998));
#245143=CARTESIAN_POINT('Ctrl Pts',(-7.78549485900006,11.6,8.10455846299998));
#245144=CARTESIAN_POINT('Ctrl Pts',(-7.78868218500006,15.2,8.10591276399999));
#245145=CARTESIAN_POINT('Ctrl Pts',(-7.78868218500006,11.6,8.10591276399999));
#245146=CARTESIAN_POINT('Ctrl Pts',(-7.79187498300006,15.2,8.10726643599999));
#245147=CARTESIAN_POINT('Ctrl Pts',(-7.79187498300006,11.6,8.10726643599999));
#245148=CARTESIAN_POINT('Ctrl Pts',(-7.79507325100005,15.2,8.10861946999999));
#245149=CARTESIAN_POINT('Ctrl Pts',(-7.79507325100005,11.6,8.10861946999999));
#245150=CARTESIAN_POINT('Ctrl Pts',(-7.79827698300006,15.2,8.10997185699998));
#245151=CARTESIAN_POINT('Ctrl Pts',(-7.79827698300006,11.6,8.10997185699998));
#245152=CARTESIAN_POINT('Ctrl Pts',(-7.80148617400006,15.2,8.11132358799998));
#245153=CARTESIAN_POINT('Ctrl Pts',(-7.80148617400006,11.6,8.11132358799998));
#245154=CARTESIAN_POINT('Ctrl Pts',(-7.80470082000006,15.2,8.11267465299998));
#245155=CARTESIAN_POINT('Ctrl Pts',(-7.80470082000006,11.6,8.11267465299998));
#245156=CARTESIAN_POINT('Ctrl Pts',(-7.80792091500006,15.2,8.11402504599998));
#245157=CARTESIAN_POINT('Ctrl Pts',(-7.80792091500006,11.6,8.11402504599998));
#245158=CARTESIAN_POINT('Ctrl Pts',(-7.81114645400006,15.2,8.11537475499998));
#245159=CARTESIAN_POINT('Ctrl Pts',(-7.81114645400006,11.6,8.11537475499998));
#245160=CARTESIAN_POINT('Ctrl Pts',(-7.81437743500006,15.2,8.11672377399999));
#245161=CARTESIAN_POINT('Ctrl Pts',(-7.81437743500006,11.6,8.11672377399999));
#245162=CARTESIAN_POINT('Ctrl Pts',(-7.81761384900006,15.2,8.11807209299998));
#245163=CARTESIAN_POINT('Ctrl Pts',(-7.81761384900006,11.6,8.11807209299998));
#245164=CARTESIAN_POINT('Ctrl Pts',(-7.82085569500006,15.2,8.11941970299999));
#245165=CARTESIAN_POINT('Ctrl Pts',(-7.82085569500006,11.6,8.11941970299999));
#245166=CARTESIAN_POINT('Ctrl Pts',(-7.82410296500006,15.2,8.12076659599999));
#245167=CARTESIAN_POINT('Ctrl Pts',(-7.82410296500006,11.6,8.12076659599999));
#245168=CARTESIAN_POINT('Ctrl Pts',(-7.82735565600006,15.2,8.12211276299998));
#245169=CARTESIAN_POINT('Ctrl Pts',(-7.82735565600006,11.6,8.12211276299998));
#245170=CARTESIAN_POINT('Ctrl Pts',(-7.83061376200005,15.2,8.12345819399999));
#245171=CARTESIAN_POINT('Ctrl Pts',(-7.83061376200005,11.6,8.12345819399999));
#245172=CARTESIAN_POINT('Ctrl Pts',(-7.83387728100006,15.2,8.12480288399998));
#245173=CARTESIAN_POINT('Ctrl Pts',(-7.83387728100006,11.6,8.12480288399998));
#245174=CARTESIAN_POINT('Ctrl Pts',(-7.83714620400006,15.2,8.12614681999998));
#245175=CARTESIAN_POINT('Ctrl Pts',(-7.83714620400006,11.6,8.12614681999998));
#245176=CARTESIAN_POINT('Ctrl Pts',(-7.84042053000006,15.2,8.12748999699998));
#245177=CARTESIAN_POINT('Ctrl Pts',(-7.84042053000006,11.6,8.12748999699998));
#245178=CARTESIAN_POINT('Ctrl Pts',(-7.84370025300006,15.2,8.12883240399999));
#245179=CARTESIAN_POINT('Ctrl Pts',(-7.84370025300006,11.6,8.12883240399999));
#245180=CARTESIAN_POINT('Ctrl Pts',(-7.84698536600006,15.2,8.13017403499998));
#245181=CARTESIAN_POINT('Ctrl Pts',(-7.84698536600006,11.6,8.13017403499998));
#245182=CARTESIAN_POINT('Ctrl Pts',(-7.85027586700006,15.2,8.13151487799999));
#245183=CARTESIAN_POINT('Ctrl Pts',(-7.85027586700006,11.6,8.13151487799999));
#245184=CARTESIAN_POINT('Ctrl Pts',(-7.85357175000006,15.2,8.13285492699999));
#245185=CARTESIAN_POINT('Ctrl Pts',(-7.85357175000006,11.6,8.13285492699999));
#245186=CARTESIAN_POINT('Ctrl Pts',(-7.85687301000006,15.2,8.13419417299999));
#245187=CARTESIAN_POINT('Ctrl Pts',(-7.85687301000006,11.6,8.13419417299999));
#245188=CARTESIAN_POINT('Ctrl Pts',(-7.86017964300005,15.2,8.13553260699998));
#245189=CARTESIAN_POINT('Ctrl Pts',(-7.86017964300005,11.6,8.13553260699998));
#245190=CARTESIAN_POINT('Ctrl Pts',(-7.86349164400006,15.2,8.13687022099998));
#245191=CARTESIAN_POINT('Ctrl Pts',(-7.86349164400006,11.6,8.13687022099998));
#245192=CARTESIAN_POINT('Ctrl Pts',(-7.86680900800006,15.2,8.13820700699999));
#245193=CARTESIAN_POINT('Ctrl Pts',(-7.86680900800006,11.6,8.13820700699999));
#245194=CARTESIAN_POINT('Ctrl Pts',(-7.87013173000006,15.2,8.13954295599999));
#245195=CARTESIAN_POINT('Ctrl Pts',(-7.87013173000006,11.6,8.13954295599999));
#245196=CARTESIAN_POINT('Ctrl Pts',(-7.87345980500006,15.2,8.14087805999998));
#245197=CARTESIAN_POINT('Ctrl Pts',(-7.87345980500006,11.6,8.14087805999998));
#245198=CARTESIAN_POINT('Ctrl Pts',(-7.87679322900006,15.2,8.14221230999999));
#245199=CARTESIAN_POINT('Ctrl Pts',(-7.87679322900006,11.6,8.14221230999999));
#245200=CARTESIAN_POINT('Ctrl Pts',(-7.88013199700006,15.2,8.14354569699999));
#245201=CARTESIAN_POINT('Ctrl Pts',(-7.88013199700006,11.6,8.14354569699999));
#245202=CARTESIAN_POINT('Ctrl Pts',(-7.88347610400006,15.2,8.14487821399998));
#245203=CARTESIAN_POINT('Ctrl Pts',(-7.88347610400006,11.6,8.14487821399998));
#245204=CARTESIAN_POINT('Ctrl Pts',(-7.88682554500006,15.2,8.14620985299998));
#245205=CARTESIAN_POINT('Ctrl Pts',(-7.88682554500006,11.6,8.14620985299998));
#245206=CARTESIAN_POINT('Ctrl Pts',(-7.89018031600006,15.2,8.14754060399999));
#245207=CARTESIAN_POINT('Ctrl Pts',(-7.89018031600006,11.6,8.14754060399999));
#245208=CARTESIAN_POINT('Ctrl Pts',(-7.89354041200006,15.2,8.14887045999999));
#245209=CARTESIAN_POINT('Ctrl Pts',(-7.89354041200006,11.6,8.14887045999999));
#245210=CARTESIAN_POINT('Ctrl Pts',(-7.89690582700005,15.2,8.15019941199999));
#245211=CARTESIAN_POINT('Ctrl Pts',(-7.89690582700005,11.6,8.15019941199999));
#245212=CARTESIAN_POINT('Ctrl Pts',(-7.90027655700006,15.2,8.15152745299999));
#245213=CARTESIAN_POINT('Ctrl Pts',(-7.90027655700006,11.6,8.15152745299999));
#245214=CARTESIAN_POINT('Ctrl Pts',(-7.90365259800006,15.2,8.15285457299998));
#245215=CARTESIAN_POINT('Ctrl Pts',(-7.90365259800006,11.6,8.15285457299998));
#245216=CARTESIAN_POINT('Ctrl Pts',(-7.90703394500006,15.2,8.15418076499999));
#245217=CARTESIAN_POINT('Ctrl Pts',(-7.90703394500006,11.6,8.15418076499999));
#245218=CARTESIAN_POINT('Ctrl Pts',(-7.91042059300005,15.2,8.15550602099999));
#245219=CARTESIAN_POINT('Ctrl Pts',(-7.91042059300005,11.6,8.15550602099999));
#245220=CARTESIAN_POINT('Ctrl Pts',(-7.91381253600005,15.2,8.15683033199999));
#245221=CARTESIAN_POINT('Ctrl Pts',(-7.91381253600005,11.6,8.15683033199999));
#245222=CARTESIAN_POINT('Ctrl Pts',(-7.91720977000006,15.2,8.15815368899998));
#245223=CARTESIAN_POINT('Ctrl Pts',(-7.91720977000006,11.6,8.15815368899998));
#245224=CARTESIAN_POINT('Ctrl Pts',(-7.92061229100005,15.2,8.15947608599998));
#245225=CARTESIAN_POINT('Ctrl Pts',(-7.92061229100005,11.6,8.15947608599998));
#245226=CARTESIAN_POINT('Ctrl Pts',(-7.92402009400006,15.2,8.16079751399998));
#245227=CARTESIAN_POINT('Ctrl Pts',(-7.92402009400006,11.6,8.16079751399998));
#245228=CARTESIAN_POINT('Ctrl Pts',(-7.92743317500006,15.2,8.16211796399998));
#245229=CARTESIAN_POINT('Ctrl Pts',(-7.92743317500006,11.6,8.16211796399998));
#245230=CARTESIAN_POINT('Ctrl Pts',(-7.93085152700005,15.2,8.16343742899999));
#245231=CARTESIAN_POINT('Ctrl Pts',(-7.93085152700005,11.6,8.16343742899999));
#245232=CARTESIAN_POINT('Ctrl Pts',(-7.93427514700006,15.2,8.16475590099999));
#245233=CARTESIAN_POINT('Ctrl Pts',(-7.93427514700006,11.6,8.16475590099999));
#245234=CARTESIAN_POINT('Ctrl Pts',(-7.93770402900006,15.2,8.16607337199999));
#245235=CARTESIAN_POINT('Ctrl Pts',(-7.93770402900006,11.6,8.16607337199999));
#245236=CARTESIAN_POINT('Ctrl Pts',(-7.94113817000006,15.2,8.16738983299999));
#245237=CARTESIAN_POINT('Ctrl Pts',(-7.94113817000006,11.6,8.16738983299999));
#245238=CARTESIAN_POINT('Ctrl Pts',(-7.94457756400006,15.2,8.16870527599999));
#245239=CARTESIAN_POINT('Ctrl Pts',(-7.94457756400006,11.6,8.16870527599999));
#245240=CARTESIAN_POINT('Ctrl Pts',(-7.94802220600006,15.2,8.17001969299999));
#245241=CARTESIAN_POINT('Ctrl Pts',(-7.94802220600006,11.6,8.17001969299999));
#245242=CARTESIAN_POINT('Ctrl Pts',(-7.95147209200006,15.2,8.17133307699999));
#245243=CARTESIAN_POINT('Ctrl Pts',(-7.95147209200006,11.6,8.17133307699999));
#245244=CARTESIAN_POINT('Ctrl Pts',(-7.95492721600005,15.2,8.17264541999998));
#245245=CARTESIAN_POINT('Ctrl Pts',(-7.95492721600005,11.6,8.17264541999998));
#245246=CARTESIAN_POINT('Ctrl Pts',(-7.95838757500006,15.2,8.17395671299998));
#245247=CARTESIAN_POINT('Ctrl Pts',(-7.95838757500006,11.6,8.17395671299998));
#245248=CARTESIAN_POINT('Ctrl Pts',(-7.96185316300006,15.2,8.17526694799999));
#245249=CARTESIAN_POINT('Ctrl Pts',(-7.96185316300006,11.6,8.17526694799999));
#245250=CARTESIAN_POINT('Ctrl Pts',(-7.96532397700006,15.2,8.17657611899998));
#245251=CARTESIAN_POINT('Ctrl Pts',(-7.96532397700006,11.6,8.17657611899998));
#245252=CARTESIAN_POINT('Ctrl Pts',(-7.96880001000006,15.2,8.17788421699999));
#245253=CARTESIAN_POINT('Ctrl Pts',(-7.96880001000006,11.6,8.17788421699999));
#245254=CARTESIAN_POINT('Ctrl Pts',(-7.97228126000006,15.2,8.17919123499999));
#245255=CARTESIAN_POINT('Ctrl Pts',(-7.97228126000006,11.6,8.17919123499999));
#245256=CARTESIAN_POINT('Ctrl Pts',(-7.97576771900006,15.2,8.18049716399998));
#245257=CARTESIAN_POINT('Ctrl Pts',(-7.97576771900006,11.6,8.18049716399998));
#245258=CARTESIAN_POINT('Ctrl Pts',(-7.97925938500006,15.2,8.18180199599999));
#245259=CARTESIAN_POINT('Ctrl Pts',(-7.97925938500006,11.6,8.18180199599999));
#245260=CARTESIAN_POINT('Ctrl Pts',(-7.98275625000005,15.2,8.18310572199999));
#245261=CARTESIAN_POINT('Ctrl Pts',(-7.98275625000005,11.6,8.18310572199999));
#245262=CARTESIAN_POINT('Ctrl Pts',(-7.98625831300006,15.2,8.18440833599999));
#245263=CARTESIAN_POINT('Ctrl Pts',(-7.98625831300006,11.6,8.18440833599999));
#245264=CARTESIAN_POINT('Ctrl Pts',(-7.98976556600006,15.2,8.18570982799999));
#245265=CARTESIAN_POINT('Ctrl Pts',(-7.98976556600006,11.6,8.18570982799999));
#245266=CARTESIAN_POINT('Ctrl Pts',(-7.99327800400006,15.2,8.18701019299999));
#245267=CARTESIAN_POINT('Ctrl Pts',(-7.99327800400006,11.6,8.18701019299999));
#245268=CARTESIAN_POINT('Ctrl Pts',(-7.99679562600006,15.2,8.18830942099999));
#245269=CARTESIAN_POINT('Ctrl Pts',(-7.99679562600006,11.6,8.18830942099999));
#245270=CARTESIAN_POINT('Ctrl Pts',(-8.00031842500006,15.2,8.18960750499999));
#245271=CARTESIAN_POINT('Ctrl Pts',(-8.00031842500006,11.6,8.18960750499999));
#245272=CARTESIAN_POINT('Ctrl Pts',(-8.00384639600006,15.2,8.19090443999999));
#245273=CARTESIAN_POINT('Ctrl Pts',(-8.00384639600006,11.6,8.19090443999999));
#245274=CARTESIAN_POINT('Ctrl Pts',(-8.00737953700006,15.2,8.19220021799998));
#245275=CARTESIAN_POINT('Ctrl Pts',(-8.00737953700006,11.6,8.19220021799998));
#245276=CARTESIAN_POINT('Ctrl Pts',(-8.01091784300005,15.2,8.19349483199998));
#245277=CARTESIAN_POINT('Ctrl Pts',(-8.01091784300005,11.6,8.19349483199998));
#245278=CARTESIAN_POINT('Ctrl Pts',(-8.01446130800005,15.2,8.19478827199998));
#245279=CARTESIAN_POINT('Ctrl Pts',(-8.01446130800005,11.6,8.19478827199998));
#245280=CARTESIAN_POINT('Ctrl Pts',(-8.01800992700005,15.2,8.19608053199998));
#245281=CARTESIAN_POINT('Ctrl Pts',(-8.01800992700005,11.6,8.19608053199998));
#245282=CARTESIAN_POINT('Ctrl Pts',(-8.02156369500005,15.2,8.19737160199999));
#245283=CARTESIAN_POINT('Ctrl Pts',(-8.02156369500005,11.6,8.19737160199999));
#245284=CARTESIAN_POINT('Ctrl Pts',(-8.02512260400006,15.2,8.19866146999999));
#245285=CARTESIAN_POINT('Ctrl Pts',(-8.02512260400006,11.6,8.19866146999999));
#245286=CARTESIAN_POINT('Ctrl Pts',(-8.02868665100006,15.2,8.19995012899999));
#245287=CARTESIAN_POINT('Ctrl Pts',(-8.02868665100006,11.6,8.19995012899999));
#245288=CARTESIAN_POINT('Ctrl Pts',(-8.03225583000006,15.2,8.20123757099999));
#245289=CARTESIAN_POINT('Ctrl Pts',(-8.03225583000006,11.6,8.20123757099999));
#245290=CARTESIAN_POINT('Ctrl Pts',(-8.03583013500005,15.2,8.20252378799999));
#245291=CARTESIAN_POINT('Ctrl Pts',(-8.03583013500005,11.6,8.20252378799999));
#245292=CARTESIAN_POINT('Ctrl Pts',(-8.03940956400006,15.2,8.20380877499998));
#245293=CARTESIAN_POINT('Ctrl Pts',(-8.03940956400006,11.6,8.20380877499998));
#245294=CARTESIAN_POINT('Ctrl Pts',(-8.04299411600006,15.2,8.20509252899999));
#245295=CARTESIAN_POINT('Ctrl Pts',(-8.04299411600006,11.6,8.20509252899999));
#245296=CARTESIAN_POINT('Ctrl Pts',(-8.04658378800006,15.2,8.20637504799999));
#245297=CARTESIAN_POINT('Ctrl Pts',(-8.04658378800006,11.6,8.20637504799999));
#245298=CARTESIAN_POINT('Ctrl Pts',(-8.04945962200006,15.2,8.20740007499998));
#245299=CARTESIAN_POINT('Ctrl Pts',(-8.04945962200006,11.6,8.20740007499998));
#245300=CARTESIAN_POINT('Ctrl Pts',(-8.05161880100006,15.2,8.20816828899999));
#245301=CARTESIAN_POINT('Ctrl Pts',(-8.05161880100006,11.6,8.20816828899999));
#245302=CARTESIAN_POINT('Ctrl Pts',(-8.05305927800006,15.2,8.20868018399998));
#245303=CARTESIAN_POINT('Ctrl Pts',(-8.05305927800006,11.6,8.20868018399998));
#245304=CARTESIAN_POINT('Ctrl Pts',(-8.05377977200006,15.2,8.20893606999999));
#245305=CARTESIAN_POINT('Ctrl Pts',(-8.05377977200006,11.6,8.20893606999999));
#245306=CARTESIAN_POINT('Ctrl Pts',(-7.01216898600006,15.2,7.64657512399998));
#245307=CARTESIAN_POINT('Ctrl Pts',(-7.01229743700006,15.2,7.64669302599999));
#245308=CARTESIAN_POINT('Ctrl Pts',(-7.01255888300006,15.2,7.64693288499998));
#245309=CARTESIAN_POINT('Ctrl Pts',(-7.01295521800006,15.2,7.64729613499998));
#245310=CARTESIAN_POINT('Ctrl Pts',(-7.01348948000006,15.2,7.64778506499999));
#245311=CARTESIAN_POINT('Ctrl Pts',(-7.01416585900006,15.2,7.64840281599999));
#245312=CARTESIAN_POINT('Ctrl Pts',(-7.01485383100006,15.2,7.64902988999999));
#245313=CARTESIAN_POINT('Ctrl Pts',(-7.01554947000006,15.2,7.64966267399998));
#245314=CARTESIAN_POINT('Ctrl Pts',(-7.01625276700006,15.2,7.65030113899999));
#245315=CARTESIAN_POINT('Ctrl Pts',(-7.01696371600006,15.2,7.65094525299999));
#245316=CARTESIAN_POINT('Ctrl Pts',(-7.01768230900006,15.2,7.65159498499998));
#245317=CARTESIAN_POINT('Ctrl Pts',(-7.01840853600006,15.2,7.65225030299998));
#245318=CARTESIAN_POINT('Ctrl Pts',(-7.01914239300006,15.2,7.65291117499999));
#245319=CARTESIAN_POINT('Ctrl Pts',(-7.01988387000006,15.2,7.65357757299999));
#245320=CARTESIAN_POINT('Ctrl Pts',(-7.02063296000006,15.2,7.65424946399998));
#245321=CARTESIAN_POINT('Ctrl Pts',(-7.02138965700006,15.2,7.65492681899998));
#245322=CARTESIAN_POINT('Ctrl Pts',(-7.02215395000006,15.2,7.65560960799998));
#245323=CARTESIAN_POINT('Ctrl Pts',(-7.02292583400006,15.2,7.65629779899999));
#245324=CARTESIAN_POINT('Ctrl Pts',(-7.02370530000006,15.2,7.65699136299999));
#245325=CARTESIAN_POINT('Ctrl Pts',(-7.02449234200006,15.2,7.65769026899999));
#245326=CARTESIAN_POINT('Ctrl Pts',(-7.02528695100006,15.2,7.65839448899998));
#245327=CARTESIAN_POINT('Ctrl Pts',(-7.02608912200006,15.2,7.65910399299998));
#245328=CARTESIAN_POINT('Ctrl Pts',(-7.02689884500006,15.2,7.65981874999999));
#245329=CARTESIAN_POINT('Ctrl Pts',(-7.02771611300006,15.2,7.66053873299998));
#245330=CARTESIAN_POINT('Ctrl Pts',(-7.02854092000006,15.2,7.66126390999998));
#245331=CARTESIAN_POINT('Ctrl Pts',(-7.02937325800006,15.2,7.66199425499998));
#245332=CARTESIAN_POINT('Ctrl Pts',(-7.03021311900006,15.2,7.66272973699999));
#245333=CARTESIAN_POINT('Ctrl Pts',(-7.03106049600006,15.2,7.66347032799998));
#245334=CARTESIAN_POINT('Ctrl Pts',(-7.03191538200006,15.2,7.66421599899999));
#245335=CARTESIAN_POINT('Ctrl Pts',(-7.03277777000006,15.2,7.66496672199998));
#245336=CARTESIAN_POINT('Ctrl Pts',(-7.03364765200006,15.2,7.66572246899998));
#245337=CARTESIAN_POINT('Ctrl Pts',(-7.03452502100006,15.2,7.66648321099999));
#245338=CARTESIAN_POINT('Ctrl Pts',(-7.03540987000006,15.2,7.66724892099998));
#245339=CARTESIAN_POINT('Ctrl Pts',(-7.03630219100006,15.2,7.66801956799998));
#245340=CARTESIAN_POINT('Ctrl Pts',(-7.03720197800005,15.2,7.66879512799999));
#245341=CARTESIAN_POINT('Ctrl Pts',(-7.03810922400006,15.2,7.66957557299998));
#245342=CARTESIAN_POINT('Ctrl Pts',(-7.03902392100006,15.2,7.67036087199998));
#245343=CARTESIAN_POINT('Ctrl Pts',(-7.03994606100006,15.2,7.67115099999998));
#245344=CARTESIAN_POINT('Ctrl Pts',(-7.04087563900006,15.2,7.67194592999999));
#245345=CARTESIAN_POINT('Ctrl Pts',(-7.04181264600006,15.2,7.67274563399998));
#245346=CARTESIAN_POINT('Ctrl Pts',(-7.04275707700006,15.2,7.67355008599999));
#245347=CARTESIAN_POINT('Ctrl Pts',(-7.04370892200005,15.2,7.67435925699999));
#245348=CARTESIAN_POINT('Ctrl Pts',(-7.04466817800006,15.2,7.67517312299999));
#245349=CARTESIAN_POINT('Ctrl Pts',(-7.04563483400006,15.2,7.67599165499998));
#245350=CARTESIAN_POINT('Ctrl Pts',(-7.04660888600006,15.2,7.67681482699999));
#245351=CARTESIAN_POINT('Ctrl Pts',(-7.04759032400006,15.2,7.67764261299998));
#245352=CARTESIAN_POINT('Ctrl Pts',(-7.04857914400006,15.2,7.67847498699999));
#245353=CARTESIAN_POINT('Ctrl Pts',(-7.04957533900005,15.2,7.67931192299999));
#245354=CARTESIAN_POINT('Ctrl Pts',(-7.05057890000006,15.2,7.68015339299998));
#245355=CARTESIAN_POINT('Ctrl Pts',(-7.05158982000006,15.2,7.68099937399998));
#245356=CARTESIAN_POINT('Ctrl Pts',(-7.05260809400006,15.2,7.68184983699999));
#245357=CARTESIAN_POINT('Ctrl Pts',(-7.05363371500006,15.2,7.68270475799999));
#245358=CARTESIAN_POINT('Ctrl Pts',(-7.05466667400006,15.2,7.68356411099998));
#245359=CARTESIAN_POINT('Ctrl Pts',(-7.05570696700006,15.2,7.68442787099998));
#245360=CARTESIAN_POINT('Ctrl Pts',(-7.05675458400005,15.2,7.68529601199998));
#245361=CARTESIAN_POINT('Ctrl Pts',(-7.05780952100006,15.2,7.68616850899999));
#245362=CARTESIAN_POINT('Ctrl Pts',(-7.05887177100006,15.2,7.68704533799998));
#245363=CARTESIAN_POINT('Ctrl Pts',(-7.05994132500006,15.2,7.68792647199999));
#245364=CARTESIAN_POINT('Ctrl Pts',(-7.06101817900006,15.2,7.68881188699999));
#245365=CARTESIAN_POINT('Ctrl Pts',(-7.06210232400006,15.2,7.68970155699999));
#245366=CARTESIAN_POINT('Ctrl Pts',(-7.06319375500006,15.2,7.69059545999998));
#245367=CARTESIAN_POINT('Ctrl Pts',(-7.06429246300006,15.2,7.69149356899998));
#245368=CARTESIAN_POINT('Ctrl Pts',(-7.06539844400006,15.2,7.69239585999999));
#245369=CARTESIAN_POINT('Ctrl Pts',(-7.06651169000006,15.2,7.69330230899998));
#245370=CARTESIAN_POINT('Ctrl Pts',(-7.06763219400006,15.2,7.69421289099999));
#245371=CARTESIAN_POINT('Ctrl Pts',(-7.06875995000006,15.2,7.69512758399999));
#245372=CARTESIAN_POINT('Ctrl Pts',(-7.06989495100006,15.2,7.69604635999999));
#245373=CARTESIAN_POINT('Ctrl Pts',(-7.07103719100005,15.2,7.69696919799999));
#245374=CARTESIAN_POINT('Ctrl Pts',(-7.07218666200006,15.2,7.69789607499998));
#245375=CARTESIAN_POINT('Ctrl Pts',(-7.07334335900006,15.2,7.69882696299998));
#245376=CARTESIAN_POINT('Ctrl Pts',(-7.07450727400006,15.2,7.69976184299999));
#245377=CARTESIAN_POINT('Ctrl Pts',(-7.07567840200006,15.2,7.70070068799999));
#245378=CARTESIAN_POINT('Ctrl Pts',(-7.07685673500006,15.2,7.70164347599999));
#245379=CARTESIAN_POINT('Ctrl Pts',(-7.07804226800006,15.2,7.70259018399998));
#245380=CARTESIAN_POINT('Ctrl Pts',(-7.07923499300006,15.2,7.70354078799999));
#245381=CARTESIAN_POINT('Ctrl Pts',(-7.08043490300006,15.2,7.70449526499998));
#245382=CARTESIAN_POINT('Ctrl Pts',(-7.08164199400006,15.2,7.70545359099999));
#245383=CARTESIAN_POINT('Ctrl Pts',(-7.08285625800006,15.2,7.70641574499999));
#245384=CARTESIAN_POINT('Ctrl Pts',(-7.08407768800006,15.2,7.70738170199999));
#245385=CARTESIAN_POINT('Ctrl Pts',(-7.08530627800006,15.2,7.70835144099999));
#245386=CARTESIAN_POINT('Ctrl Pts',(-7.08654202200006,15.2,7.70932493899998));
#245387=CARTESIAN_POINT('Ctrl Pts',(-7.08778491400006,15.2,7.71030217199999));
#245388=CARTESIAN_POINT('Ctrl Pts',(-7.08903494500006,15.2,7.71128311899999));
#245389=CARTESIAN_POINT('Ctrl Pts',(-7.09029211200006,15.2,7.71226775599998));
#245390=CARTESIAN_POINT('Ctrl Pts',(-7.09155640600006,15.2,7.71325606199999));
#245391=CARTESIAN_POINT('Ctrl Pts',(-7.09282782300006,15.2,7.71424801399998));
#245392=CARTESIAN_POINT('Ctrl Pts',(-7.09410635400006,15.2,7.71524359099999));
#245393=CARTESIAN_POINT('Ctrl Pts',(-7.09539199400006,15.2,7.71624276799999));
#245394=CARTESIAN_POINT('Ctrl Pts',(-7.09668473700006,15.2,7.71724552699999));
#245395=CARTESIAN_POINT('Ctrl Pts',(-7.09798457700006,15.2,7.71825184399999));
#245396=CARTESIAN_POINT('Ctrl Pts',(-7.09929150500006,15.2,7.71926169699999));
#245397=CARTESIAN_POINT('Ctrl Pts',(-7.10060551800006,15.2,7.72027506499998));
#245398=CARTESIAN_POINT('Ctrl Pts',(-7.10192660800006,15.2,7.72129192499998));
#245399=CARTESIAN_POINT('Ctrl Pts',(-7.10325476900006,15.2,7.72231225799998));
#245400=CARTESIAN_POINT('Ctrl Pts',(-7.10458999400006,15.2,7.72333603999999));
#245401=CARTESIAN_POINT('Ctrl Pts',(-7.10593227900006,15.2,7.72436325099999));
#245402=CARTESIAN_POINT('Ctrl Pts',(-7.10728161500006,15.2,7.72539386899999));
#245403=CARTESIAN_POINT('Ctrl Pts',(-7.10863799800006,15.2,7.72642787299999));
#245404=CARTESIAN_POINT('Ctrl Pts',(-7.11000142000006,15.2,7.72746524299999));
#245405=CARTESIAN_POINT('Ctrl Pts',(-7.11137187600006,15.2,7.72850595599999));
#245406=CARTESIAN_POINT('Ctrl Pts',(-7.11274935900006,15.2,7.72954999299999));
#245407=CARTESIAN_POINT('Ctrl Pts',(-7.11413386400006,15.2,7.73059733099998));
#245408=CARTESIAN_POINT('Ctrl Pts',(-7.11552538300006,15.2,7.73164795099999));
#245409=CARTESIAN_POINT('Ctrl Pts',(-7.11692391100006,15.2,7.73270183099999));
#245410=CARTESIAN_POINT('Ctrl Pts',(-7.11832944100006,15.2,7.73375895199998));
#245411=CARTESIAN_POINT('Ctrl Pts',(-7.11974196900006,15.2,7.73481929199999));
#245412=CARTESIAN_POINT('Ctrl Pts',(-7.12116148600006,15.2,7.73588283099999));
#245413=CARTESIAN_POINT('Ctrl Pts',(-7.12258798800006,15.2,7.73694954699998));
#245414=CARTESIAN_POINT('Ctrl Pts',(-7.12402146800006,15.2,7.73801942399999));
#245415=CARTESIAN_POINT('Ctrl Pts',(-7.12546192000006,15.2,7.73909243699999));
#245416=CARTESIAN_POINT('Ctrl Pts',(-7.12690933700006,15.2,7.74016856899999));
#245417=CARTESIAN_POINT('Ctrl Pts',(-7.12836371400006,15.2,7.74124779699999));
#245418=CARTESIAN_POINT('Ctrl Pts',(-7.12982504600006,15.2,7.74233010399998));
#245419=CARTESIAN_POINT('Ctrl Pts',(-7.13129332400006,15.2,7.74341546899999));
#245420=CARTESIAN_POINT('Ctrl Pts',(-7.13276854400006,15.2,7.74450386999998));
#245421=CARTESIAN_POINT('Ctrl Pts',(-7.13425070000006,15.2,7.74559529099999));
#245422=CARTESIAN_POINT('Ctrl Pts',(-7.13573978500006,15.2,7.74668970999999));
#245423=CARTESIAN_POINT('Ctrl Pts',(-7.13723579400006,15.2,7.74778710799998));
#245424=CARTESIAN_POINT('Ctrl Pts',(-7.13873872000006,15.2,7.74888746499999));
#245425=CARTESIAN_POINT('Ctrl Pts',(-7.14024855600006,15.2,7.74999076199999));
#245426=CARTESIAN_POINT('Ctrl Pts',(-7.14176530000006,15.2,7.75109697799999));
#245427=CARTESIAN_POINT('Ctrl Pts',(-7.14328894200006,15.2,7.75220609499998));
#245428=CARTESIAN_POINT('Ctrl Pts',(-7.14481947700006,15.2,7.75331809499999));
#245429=CARTESIAN_POINT('Ctrl Pts',(-7.14635690000006,15.2,7.75443295699999));
#245430=CARTESIAN_POINT('Ctrl Pts',(-7.14790120500005,15.2,7.75555066199999));
#245431=CARTESIAN_POINT('Ctrl Pts',(-7.14945238500006,15.2,7.75667119099998));
#245432=CARTESIAN_POINT('Ctrl Pts',(-7.15101043300006,15.2,7.75779452499999));
#245433=CARTESIAN_POINT('Ctrl Pts',(-7.15257534700006,15.2,7.75892064699998));
#245434=CARTESIAN_POINT('Ctrl Pts',(-7.15414711700006,15.2,7.76004953499999));
#245435=CARTESIAN_POINT('Ctrl Pts',(-7.15572573900006,15.2,7.76118117199999));
#245436=CARTESIAN_POINT('Ctrl Pts',(-7.15731120800006,15.2,7.76231553799998));
#245437=CARTESIAN_POINT('Ctrl Pts',(-7.15890351700006,15.2,7.76345261699999));
#245438=CARTESIAN_POINT('Ctrl Pts',(-7.16050265800006,15.2,7.76459238699999));
#245439=CARTESIAN_POINT('Ctrl Pts',(-7.16210862800006,15.2,7.76573483199999));
#245440=CARTESIAN_POINT('Ctrl Pts',(-7.16372142100006,15.2,7.76687993299999));
#245441=CARTESIAN_POINT('Ctrl Pts',(-7.16534103000006,15.2,7.76802766999998));
#245442=CARTESIAN_POINT('Ctrl Pts',(-7.16696745000006,15.2,7.76917802599999));
#245443=CARTESIAN_POINT('Ctrl Pts',(-7.16860067400006,15.2,7.77033098499999));
#245444=CARTESIAN_POINT('Ctrl Pts',(-7.17024069700006,15.2,7.77148652499999));
#245445=CARTESIAN_POINT('Ctrl Pts',(-7.17188751300006,15.2,7.77264462899999));
#245446=CARTESIAN_POINT('Ctrl Pts',(-7.17354111600006,15.2,7.77380527999998));
#245447=CARTESIAN_POINT('Ctrl Pts',(-7.17520150000006,15.2,7.77496845799998));
#245448=CARTESIAN_POINT('Ctrl Pts',(-7.17686866000006,15.2,7.77613414899999));
#245449=CARTESIAN_POINT('Ctrl Pts',(-7.17854259000006,15.2,7.77730232999998));
#245450=CARTESIAN_POINT('Ctrl Pts',(-7.18022328300005,15.2,7.77847298699999));
#245451=CARTESIAN_POINT('Ctrl Pts',(-7.18191073400006,15.2,7.77964609999999));
#245452=CARTESIAN_POINT('Ctrl Pts',(-7.18360493800006,15.2,7.78082165399999));
#245453=CARTESIAN_POINT('Ctrl Pts',(-7.18530588900006,15.2,7.78199962799999));
#245454=CARTESIAN_POINT('Ctrl Pts',(-7.18701358000006,15.2,7.78318000699999));
#245455=CARTESIAN_POINT('Ctrl Pts',(-7.18872800700006,15.2,7.78436277199998));
#245456=CARTESIAN_POINT('Ctrl Pts',(-7.19044916200006,15.2,7.78554790599999));
#245457=CARTESIAN_POINT('Ctrl Pts',(-7.19217704100005,15.2,7.78673539199998));
#245458=CARTESIAN_POINT('Ctrl Pts',(-7.19391163700006,15.2,7.78792521199998));
#245459=CARTESIAN_POINT('Ctrl Pts',(-7.19565294600006,15.2,7.78911734999999));
#245460=CARTESIAN_POINT('Ctrl Pts',(-7.19740096200006,15.2,7.79031178799999));
#245461=CARTESIAN_POINT('Ctrl Pts',(-7.19915567700006,15.2,7.79150850799999));
#245462=CARTESIAN_POINT('Ctrl Pts',(-7.20091708800005,15.2,7.79270749399998));
#245463=CARTESIAN_POINT('Ctrl Pts',(-7.20268518700006,15.2,7.79390872899998));
#245464=CARTESIAN_POINT('Ctrl Pts',(-7.20445997000006,15.2,7.79511219599998));
#245465=CARTESIAN_POINT('Ctrl Pts',(-7.20624143100006,15.2,7.79631787699999));
#245466=CARTESIAN_POINT('Ctrl Pts',(-7.20802956400005,15.2,7.79752575699998));
#245467=CARTESIAN_POINT('Ctrl Pts',(-7.20982436400006,15.2,7.79873581599999));
#245468=CARTESIAN_POINT('Ctrl Pts',(-7.21162582400006,15.2,7.79994804199998));
#245469=CARTESIAN_POINT('Ctrl Pts',(-7.21343393900006,15.2,7.80116241399998));
#245470=CARTESIAN_POINT('Ctrl Pts',(-7.21524870400006,15.2,7.80237891799998));
#245471=CARTESIAN_POINT('Ctrl Pts',(-7.21707011300006,15.2,7.80359753599999));
#245472=CARTESIAN_POINT('Ctrl Pts',(-7.21889815900006,15.2,7.80481825199999));
#245473=CARTESIAN_POINT('Ctrl Pts',(-7.22073283800006,15.2,7.80604104899999));
#245474=CARTESIAN_POINT('Ctrl Pts',(-7.22257414400006,15.2,7.80726591199999));
#245475=CARTESIAN_POINT('Ctrl Pts',(-7.22442207200006,15.2,7.80849282399998));
#245476=CARTESIAN_POINT('Ctrl Pts',(-7.22627661400006,15.2,7.80972176699999));
#245477=CARTESIAN_POINT('Ctrl Pts',(-7.22813776800006,15.2,7.81095272699999));
#245478=CARTESIAN_POINT('Ctrl Pts',(-7.23000552500006,15.2,7.81218568699998));
#245479=CARTESIAN_POINT('Ctrl Pts',(-7.23187988200006,15.2,7.81342063099999));
#245480=CARTESIAN_POINT('Ctrl Pts',(-7.23376083100006,15.2,7.81465754299998));
#245481=CARTESIAN_POINT('Ctrl Pts',(-7.23564836800006,15.2,7.81589640599999));
#245482=CARTESIAN_POINT('Ctrl Pts',(-7.23754248700006,15.2,7.81713720599999));
#245483=CARTESIAN_POINT('Ctrl Pts',(-7.23944318300005,15.2,7.81837992399999));
#245484=CARTESIAN_POINT('Ctrl Pts',(-7.24135045000006,15.2,7.81962454799999));
#245485=CARTESIAN_POINT('Ctrl Pts',(-7.24326428200006,15.2,7.82087105799998));
#245486=CARTESIAN_POINT('Ctrl Pts',(-7.24518467300006,15.2,7.82211944199998));
#245487=CARTESIAN_POINT('Ctrl Pts',(-7.24711162000006,15.2,7.82336968199999));
#245488=CARTESIAN_POINT('Ctrl Pts',(-7.24904511400006,15.2,7.82462176199999));
#245489=CARTESIAN_POINT('Ctrl Pts',(-7.25098515300005,15.2,7.82587566899998));
#245490=CARTESIAN_POINT('Ctrl Pts',(-7.25293172800006,15.2,7.82713138499999));
#245491=CARTESIAN_POINT('Ctrl Pts',(-7.25488483700006,15.2,7.82838889399999));
#245492=CARTESIAN_POINT('Ctrl Pts',(-7.25684447100006,15.2,7.82964818299998));
#245493=CARTESIAN_POINT('Ctrl Pts',(-7.25881062600005,15.2,7.83090923599998));
#245494=CARTESIAN_POINT('Ctrl Pts',(-7.26078329800006,15.2,7.83217203499999));
#245495=CARTESIAN_POINT('Ctrl Pts',(-7.26276247900006,15.2,7.83343656799998));
#245496=CARTESIAN_POINT('Ctrl Pts',(-7.26474816500006,15.2,7.83470281899999));
#245497=CARTESIAN_POINT('Ctrl Pts',(-7.26674035000006,15.2,7.83597076999998));
#245498=CARTESIAN_POINT('Ctrl Pts',(-7.26873902900006,15.2,7.83724040899998));
#245499=CARTESIAN_POINT('Ctrl Pts',(-7.27074419600005,15.2,7.83851171899999));
#245500=CARTESIAN_POINT('Ctrl Pts',(-7.27275584500005,15.2,7.83978468699999));
#245501=CARTESIAN_POINT('Ctrl Pts',(-7.27477397200006,15.2,7.84105929599999));
#245502=CARTESIAN_POINT('Ctrl Pts',(-7.27679857000005,15.2,7.84233553099998));
#245503=CARTESIAN_POINT('Ctrl Pts',(-7.27882963600006,15.2,7.84361337899998));
#245504=CARTESIAN_POINT('Ctrl Pts',(-7.28086716200006,15.2,7.84489282299998));
#245505=CARTESIAN_POINT('Ctrl Pts',(-7.28291114200006,15.2,7.84617384799999));
#245506=CARTESIAN_POINT('Ctrl Pts',(-7.28496157300006,15.2,7.84745644199998));
#245507=CARTESIAN_POINT('Ctrl Pts',(-7.28701844900006,15.2,7.84874058699998));
#245508=CARTESIAN_POINT('Ctrl Pts',(-7.28908176300005,15.2,7.85002626999999));
#245509=CARTESIAN_POINT('Ctrl Pts',(-7.29115151200006,15.2,7.85131347699998));
#245510=CARTESIAN_POINT('Ctrl Pts',(-7.29322768800006,15.2,7.85260219099998));
#245511=CARTESIAN_POINT('Ctrl Pts',(-7.29531028700006,15.2,7.85389239899998));
#245512=CARTESIAN_POINT('Ctrl Pts',(-7.29739930400005,15.2,7.85518408599999));
#245513=CARTESIAN_POINT('Ctrl Pts',(-7.29949473300006,15.2,7.85647723899999));
#245514=CARTESIAN_POINT('Ctrl Pts',(-7.30159656800006,15.2,7.85777184099998));
#245515=CARTESIAN_POINT('Ctrl Pts',(-7.30370480500006,15.2,7.85906787899999));
#245516=CARTESIAN_POINT('Ctrl Pts',(-7.30581943700006,15.2,7.86036533899999));
#245517=CARTESIAN_POINT('Ctrl Pts',(-7.30794046000006,15.2,7.86166420599999));
#245518=CARTESIAN_POINT('Ctrl Pts',(-7.31006786800006,15.2,7.86296446599999));
#245519=CARTESIAN_POINT('Ctrl Pts',(-7.31220165500006,15.2,7.86426610399998));
#245520=CARTESIAN_POINT('Ctrl Pts',(-7.31434181800006,15.2,7.86556910899999));
#245521=CARTESIAN_POINT('Ctrl Pts',(-7.31648834800006,15.2,7.86687346199999));
#245522=CARTESIAN_POINT('Ctrl Pts',(-7.31864124200006,15.2,7.86817915199999));
#245523=CARTESIAN_POINT('Ctrl Pts',(-7.32080049400006,15.2,7.86948616399999));
#245524=CARTESIAN_POINT('Ctrl Pts',(-7.32296610000006,15.2,7.87079448499998));
#245525=CARTESIAN_POINT('Ctrl Pts',(-7.32513805400006,15.2,7.87210409899998));
#245526=CARTESIAN_POINT('Ctrl Pts',(-7.32731634900006,15.2,7.87341499399999));
#245527=CARTESIAN_POINT('Ctrl Pts',(-7.32950098000006,15.2,7.87472715499998));
#245528=CARTESIAN_POINT('Ctrl Pts',(-7.33169194400006,15.2,7.87604056899998));
#245529=CARTESIAN_POINT('Ctrl Pts',(-7.33388923300006,15.2,7.87735522199998));
#245530=CARTESIAN_POINT('Ctrl Pts',(-7.33609284400006,15.2,7.87867109999999));
#245531=CARTESIAN_POINT('Ctrl Pts',(-7.33830277000005,15.2,7.87998818899998));
#245532=CARTESIAN_POINT('Ctrl Pts',(-7.34051900600006,15.2,7.88130647499998));
#245533=CARTESIAN_POINT('Ctrl Pts',(-7.34274154700006,15.2,7.88262594599999));
#245534=CARTESIAN_POINT('Ctrl Pts',(-7.34497038800006,15.2,7.88394658699998));
#245535=CARTESIAN_POINT('Ctrl Pts',(-7.34720552300006,15.2,7.88526838399999));
#245536=CARTESIAN_POINT('Ctrl Pts',(-7.34944694700006,15.2,7.88659132499999));
#245537=CARTESIAN_POINT('Ctrl Pts',(-7.35169465500006,15.2,7.88791539599998));
#245538=CARTESIAN_POINT('Ctrl Pts',(-7.35394864100006,15.2,7.88924058299998));
#245539=CARTESIAN_POINT('Ctrl Pts',(-7.35620890000006,15.2,7.89056687299999));
#245540=CARTESIAN_POINT('Ctrl Pts',(-7.35847542700006,15.2,7.89189425299998));
#245541=CARTESIAN_POINT('Ctrl Pts',(-7.36074821700006,15.2,7.89322270699999));
#245542=CARTESIAN_POINT('Ctrl Pts',(-7.36302726400006,15.2,7.89455222599998));
#245543=CARTESIAN_POINT('Ctrl Pts',(-7.36531256300006,15.2,7.89588279499998));
#245544=CARTESIAN_POINT('Ctrl Pts',(-7.36760410800006,15.2,7.89721439899999));
#245545=CARTESIAN_POINT('Ctrl Pts',(-7.36990189600006,15.2,7.89854702799998));
#245546=CARTESIAN_POINT('Ctrl Pts',(-7.37220591900006,15.2,7.89988066499999));
#245547=CARTESIAN_POINT('Ctrl Pts',(-7.37451617400006,15.2,7.90121529999999));
#245548=CARTESIAN_POINT('Ctrl Pts',(-7.37683265400006,15.2,7.90255091899999));
#245549=CARTESIAN_POINT('Ctrl Pts',(-7.37915535500006,15.2,7.90388750999998));
#245550=CARTESIAN_POINT('Ctrl Pts',(-7.38148427100006,15.2,7.90522505699998));
#245551=CARTESIAN_POINT('Ctrl Pts',(-7.38381939700006,15.2,7.90656354999999));
#245552=CARTESIAN_POINT('Ctrl Pts',(-7.38616072800006,15.2,7.90790297499999));
#245553=CARTESIAN_POINT('Ctrl Pts',(-7.38850825800006,15.2,7.90924331999998));
#245554=CARTESIAN_POINT('Ctrl Pts',(-7.39086198300006,15.2,7.91058456999998));
#245555=CARTESIAN_POINT('Ctrl Pts',(-7.39322189600006,15.2,7.91192671399998));
#245556=CARTESIAN_POINT('Ctrl Pts',(-7.39558799400006,15.2,7.91326973999999));
#245557=CARTESIAN_POINT('Ctrl Pts',(-7.39796027100006,15.2,7.91461363299998));
#245558=CARTESIAN_POINT('Ctrl Pts',(-7.40033872100006,15.2,7.91595838099998));
#245559=CARTESIAN_POINT('Ctrl Pts',(-7.40272333900006,15.2,7.91730397299999));
#245560=CARTESIAN_POINT('Ctrl Pts',(-7.40511412000005,15.2,7.91865039499999));
#245561=CARTESIAN_POINT('Ctrl Pts',(-7.40751105900006,15.2,7.91999763299999));
#245562=CARTESIAN_POINT('Ctrl Pts',(-7.40991415200006,15.2,7.92134567699998));
#245563=CARTESIAN_POINT('Ctrl Pts',(-7.41232339100006,15.2,7.92269451299998));
#245564=CARTESIAN_POINT('Ctrl Pts',(-7.41473877300006,15.2,7.92404412999999));
#245565=CARTESIAN_POINT('Ctrl Pts',(-7.41716029100006,15.2,7.92539451399998));
#245566=CARTESIAN_POINT('Ctrl Pts',(-7.41958794200006,15.2,7.92674565199999));
#245567=CARTESIAN_POINT('Ctrl Pts',(-7.42202171900006,15.2,7.92809753399998));
#245568=CARTESIAN_POINT('Ctrl Pts',(-7.42446161900006,15.2,7.92945014599999));
#245569=CARTESIAN_POINT('Ctrl Pts',(-7.42690763400006,15.2,7.93080347599999));
#245570=CARTESIAN_POINT('Ctrl Pts',(-7.42935976100005,15.2,7.93215751199998));
#245571=CARTESIAN_POINT('Ctrl Pts',(-7.43181799400006,15.2,7.93351224099998));
#245572=CARTESIAN_POINT('Ctrl Pts',(-7.43428232700006,15.2,7.93486765199999));
#245573=CARTESIAN_POINT('Ctrl Pts',(-7.43675275700006,15.2,7.93622373199998));
#245574=CARTESIAN_POINT('Ctrl Pts',(-7.43922927800006,15.2,7.93758046899999));
#245575=CARTESIAN_POINT('Ctrl Pts',(-7.44171188300006,15.2,7.93893784999998));
#245576=CARTESIAN_POINT('Ctrl Pts',(-7.44420057000006,15.2,7.94029586499998));
#245577=CARTESIAN_POINT('Ctrl Pts',(-7.44669533100006,15.2,7.94165450099998));
#245578=CARTESIAN_POINT('Ctrl Pts',(-7.44919616200006,15.2,7.94301374399998));
#245579=CARTESIAN_POINT('Ctrl Pts',(-7.45170305800006,15.2,7.94437358599998));
#245580=CARTESIAN_POINT('Ctrl Pts',(-7.45421601400006,15.2,7.94573401099999));
#245581=CARTESIAN_POINT('Ctrl Pts',(-7.45673502500006,15.2,7.94709500999998));
#245582=CARTESIAN_POINT('Ctrl Pts',(-7.45926008500006,15.2,7.94845657099999));
#245583=CARTESIAN_POINT('Ctrl Pts',(-7.46179119000006,15.2,7.94981867899998));
#245584=CARTESIAN_POINT('Ctrl Pts',(-7.46432833400006,15.2,7.95118132499999));
#245585=CARTESIAN_POINT('Ctrl Pts',(-7.46687151300006,15.2,7.95254449699998));
#245586=CARTESIAN_POINT('Ctrl Pts',(-7.46942072000006,15.2,7.95390818299998));
#245587=CARTESIAN_POINT('Ctrl Pts',(-7.47197595100006,15.2,7.95527237099999));
#245588=CARTESIAN_POINT('Ctrl Pts',(-7.47453720200006,15.2,7.95663704999999));
#245589=CARTESIAN_POINT('Ctrl Pts',(-7.47710446500006,15.2,7.95800220799999));
#245590=CARTESIAN_POINT('Ctrl Pts',(-7.47967773800006,15.2,7.95936783099998));
#245591=CARTESIAN_POINT('Ctrl Pts',(-7.48225701500006,15.2,7.96073391199998));
#245592=CARTESIAN_POINT('Ctrl Pts',(-7.48484228800006,15.2,7.96210043599999));
#245593=CARTESIAN_POINT('Ctrl Pts',(-7.48743355700006,15.2,7.96346739199999));
#245594=CARTESIAN_POINT('Ctrl Pts',(-7.49003081300006,15.2,7.96483476999998));
#245595=CARTESIAN_POINT('Ctrl Pts',(-7.49263405300006,15.2,7.96620255599999));
#245596=CARTESIAN_POINT('Ctrl Pts',(-7.49524327100006,15.2,7.96757074199999));
#245597=CARTESIAN_POINT('Ctrl Pts',(-7.49785846200006,15.2,7.96893931299999));
#245598=CARTESIAN_POINT('Ctrl Pts',(-7.50047962100006,15.2,7.97030825999999));
#245599=CARTESIAN_POINT('Ctrl Pts',(-7.50310674300006,15.2,7.97167757099999));
#245600=CARTESIAN_POINT('Ctrl Pts',(-7.50573982300006,15.2,7.97304723499998));
#245601=CARTESIAN_POINT('Ctrl Pts',(-7.50837885500006,15.2,7.97441723899999));
#245602=CARTESIAN_POINT('Ctrl Pts',(-7.51102383600006,15.2,7.97578757299998));
#245603=CARTESIAN_POINT('Ctrl Pts',(-7.51367475900006,15.2,7.97715822699999));
#245604=CARTESIAN_POINT('Ctrl Pts',(-7.51633162000005,15.2,7.97852918799999));
#245605=CARTESIAN_POINT('Ctrl Pts',(-7.51899441200005,15.2,7.97990044499999));
#245606=CARTESIAN_POINT('Ctrl Pts',(-7.52166313300006,15.2,7.98127198799998));
#245607=CARTESIAN_POINT('Ctrl Pts',(-7.52433777600006,15.2,7.98264380499998));
#245608=CARTESIAN_POINT('Ctrl Pts',(-7.52701833700005,15.2,7.98401588399998));
#245609=CARTESIAN_POINT('Ctrl Pts',(-7.52970481000006,15.2,7.98538821699999));
#245610=CARTESIAN_POINT('Ctrl Pts',(-7.53239719100005,15.2,7.98676078899998));
#245611=CARTESIAN_POINT('Ctrl Pts',(-7.53509547300006,15.2,7.98813359199999));
#245612=CARTESIAN_POINT('Ctrl Pts',(-7.53779965400006,15.2,7.98950661499998));
#245613=CARTESIAN_POINT('Ctrl Pts',(-7.54050972500006,15.2,7.99087984499998));
#245614=CARTESIAN_POINT('Ctrl Pts',(-7.54322568500006,15.2,7.99225327099998));
#245615=CARTESIAN_POINT('Ctrl Pts',(-7.54594752700006,15.2,7.99362688499999));
#245616=CARTESIAN_POINT('Ctrl Pts',(-7.54867524600006,15.2,7.99500067299999));
#245617=CARTESIAN_POINT('Ctrl Pts',(-7.55140883700006,15.2,7.99637462699998));
#245618=CARTESIAN_POINT('Ctrl Pts',(-7.55414829500006,15.2,7.99774873399999));
#245619=CARTESIAN_POINT('Ctrl Pts',(-7.55689361600006,15.2,7.99912298399998));
#245620=CARTESIAN_POINT('Ctrl Pts',(-7.55964479300006,15.2,8.00049736599998));
#245621=CARTESIAN_POINT('Ctrl Pts',(-7.56240182300005,15.2,8.00187187099999));
#245622=CARTESIAN_POINT('Ctrl Pts',(-7.56516470000006,15.2,8.00324648399998));
#245623=CARTESIAN_POINT('Ctrl Pts',(-7.56793341800006,15.2,8.00462119899999));
#245624=CARTESIAN_POINT('Ctrl Pts',(-7.57070797500005,15.2,8.00599600399998));
#245625=CARTESIAN_POINT('Ctrl Pts',(-7.57348836300006,15.2,8.00737088699999));
#245626=CARTESIAN_POINT('Ctrl Pts',(-7.57627457800006,15.2,8.00874583799999));
#245627=CARTESIAN_POINT('Ctrl Pts',(-7.57906661600006,15.2,8.01012084699998));
#245628=CARTESIAN_POINT('Ctrl Pts',(-7.58186447000006,15.2,8.01149590299998));
#245629=CARTESIAN_POINT('Ctrl Pts',(-7.58466813600006,15.2,8.01287099699999));
#245630=CARTESIAN_POINT('Ctrl Pts',(-7.58747761100006,15.2,8.01424611599998));
#245631=CARTESIAN_POINT('Ctrl Pts',(-7.59029288700006,15.2,8.01562125099998));
#245632=CARTESIAN_POINT('Ctrl Pts',(-7.59311396000006,15.2,8.01699639099999));
#245633=CARTESIAN_POINT('Ctrl Pts',(-7.59594082600006,15.2,8.01837152699999));
#245634=CARTESIAN_POINT('Ctrl Pts',(-7.59877347800006,15.2,8.01974664699999));
#245635=CARTESIAN_POINT('Ctrl Pts',(-7.60161191400006,15.2,8.02112174099998));
#245636=CARTESIAN_POINT('Ctrl Pts',(-7.60445612600006,15.2,8.02249679899998));
#245637=CARTESIAN_POINT('Ctrl Pts',(-7.60730611100006,15.2,8.02387180999999));
#245638=CARTESIAN_POINT('Ctrl Pts',(-7.61016186300005,15.2,8.02524676499999));
#245639=CARTESIAN_POINT('Ctrl Pts',(-7.61302337700006,15.2,8.02662165399998));
#245640=CARTESIAN_POINT('Ctrl Pts',(-7.61589065000006,15.2,8.02799646399999));
#245641=CARTESIAN_POINT('Ctrl Pts',(-7.61876367500006,15.2,8.02937118799999));
#245642=CARTESIAN_POINT('Ctrl Pts',(-7.62164244700006,15.2,8.03074581399999));
#245643=CARTESIAN_POINT('Ctrl Pts',(-7.62452696100006,15.2,8.03212033199999));
#245644=CARTESIAN_POINT('Ctrl Pts',(-7.62741721300006,15.2,8.03349473299999));
#245645=CARTESIAN_POINT('Ctrl Pts',(-7.63031319900006,15.2,8.03486900599999));
#245646=CARTESIAN_POINT('Ctrl Pts',(-7.63321491200006,15.2,8.03624313999999));
#245647=CARTESIAN_POINT('Ctrl Pts',(-7.63612234700006,15.2,8.03761712699998));
#245648=CARTESIAN_POINT('Ctrl Pts',(-7.63903550100006,15.2,8.03899095599999));
#245649=CARTESIAN_POINT('Ctrl Pts',(-7.64195436800006,15.2,8.04036461599999));
#245650=CARTESIAN_POINT('Ctrl Pts',(-7.64487894200006,15.2,8.04173809899999));
#245651=CARTESIAN_POINT('Ctrl Pts',(-7.64780922000006,15.2,8.04311139499998));
#245652=CARTESIAN_POINT('Ctrl Pts',(-7.65074519600006,15.2,8.04448449199998));
#245653=CARTESIAN_POINT('Ctrl Pts',(-7.65368686500006,15.2,8.04585738099998));
#245654=CARTESIAN_POINT('Ctrl Pts',(-7.65663422300006,15.2,8.04723005299999));
#245655=CARTESIAN_POINT('Ctrl Pts',(-7.65958726300005,15.2,8.04860249699999));
#245656=CARTESIAN_POINT('Ctrl Pts',(-7.66254598200005,15.2,8.04997470299998));
#245657=CARTESIAN_POINT('Ctrl Pts',(-7.66551037500006,15.2,8.05134666399999));
#245658=CARTESIAN_POINT('Ctrl Pts',(-7.66848043700006,15.2,8.05271836699998));
#245659=CARTESIAN_POINT('Ctrl Pts',(-7.67145616200006,15.2,8.05408980299998));
#245660=CARTESIAN_POINT('Ctrl Pts',(-7.67443754600006,15.2,8.05546096299998));
#245661=CARTESIAN_POINT('Ctrl Pts',(-7.67742458300006,15.2,8.05683183699998));
#245662=CARTESIAN_POINT('Ctrl Pts',(-7.68041727000006,15.2,8.05820241499998));
#245663=CARTESIAN_POINT('Ctrl Pts',(-7.68341560100006,15.2,8.05957268799999));
#245664=CARTESIAN_POINT('Ctrl Pts',(-7.68641957100006,15.2,8.06094264599999));
#245665=CARTESIAN_POINT('Ctrl Pts',(-7.68942917500006,15.2,8.06231227899998));
#245666=CARTESIAN_POINT('Ctrl Pts',(-7.69244440900006,15.2,8.06368157799999));
#245667=CARTESIAN_POINT('Ctrl Pts',(-7.69546526600006,15.2,8.06505053299999));
#245668=CARTESIAN_POINT('Ctrl Pts',(-7.69849174400005,15.2,8.06641913399999));
#245669=CARTESIAN_POINT('Ctrl Pts',(-7.70152383600006,15.2,8.06778737399998));
#245670=CARTESIAN_POINT('Ctrl Pts',(-7.70456153900006,15.2,8.06915523999999));
#245671=CARTESIAN_POINT('Ctrl Pts',(-7.70760484600006,15.2,8.07052272399999));
#245672=CARTESIAN_POINT('Ctrl Pts',(-7.71065375300005,15.2,8.07188981699999));
#245673=CARTESIAN_POINT('Ctrl Pts',(-7.71370825500006,15.2,8.07325650899998));
#245674=CARTESIAN_POINT('Ctrl Pts',(-7.71676834800005,15.2,8.07462279199999));
#245675=CARTESIAN_POINT('Ctrl Pts',(-7.71983402500006,15.2,8.07598865399999));
#245676=CARTESIAN_POINT('Ctrl Pts',(-7.72290528400006,15.2,8.07735408899998));
#245677=CARTESIAN_POINT('Ctrl Pts',(-7.72598211700006,15.2,8.07871908399999));
#245678=CARTESIAN_POINT('Ctrl Pts',(-7.72906452200005,15.2,8.08008363199999));
#245679=CARTESIAN_POINT('Ctrl Pts',(-7.73215249300006,15.2,8.08144772299999));
#245680=CARTESIAN_POINT('Ctrl Pts',(-7.73524602400006,15.2,8.08281134799999));
#245681=CARTESIAN_POINT('Ctrl Pts',(-7.73834511100005,15.2,8.08417449699999));
#245682=CARTESIAN_POINT('Ctrl Pts',(-7.74144975100005,15.2,8.08553716199999));
#245683=CARTESIAN_POINT('Ctrl Pts',(-7.74455993600006,15.2,8.08689933299998));
#245684=CARTESIAN_POINT('Ctrl Pts',(-7.74767566300006,15.2,8.08826100099999));
#245685=CARTESIAN_POINT('Ctrl Pts',(-7.75079692700006,15.2,8.08962215699999));
#245686=CARTESIAN_POINT('Ctrl Pts',(-7.75392372200006,15.2,8.09098279099998));
#245687=CARTESIAN_POINT('Ctrl Pts',(-7.75705604400006,15.2,8.09234289499998));
#245688=CARTESIAN_POINT('Ctrl Pts',(-7.76019388900006,15.2,8.09370245899999));
#245689=CARTESIAN_POINT('Ctrl Pts',(-7.76333725000006,15.2,8.09506147499999));
#245690=CARTESIAN_POINT('Ctrl Pts',(-7.76648612500006,15.2,8.09641993199998));
#245691=CARTESIAN_POINT('Ctrl Pts',(-7.76964050600006,15.2,8.09777782399999));
#245692=CARTESIAN_POINT('Ctrl Pts',(-7.77280039100006,15.2,8.09913513899998));
#245693=CARTESIAN_POINT('Ctrl Pts',(-7.77596577300006,15.2,8.10049186899998));
#245694=CARTESIAN_POINT('Ctrl Pts',(-7.77913664800005,15.2,8.10184800599998));
#245695=CARTESIAN_POINT('Ctrl Pts',(-7.78231301200006,15.2,8.10320353899998));
#245696=CARTESIAN_POINT('Ctrl Pts',(-7.78549485900006,15.2,8.10455846299998));
#245697=CARTESIAN_POINT('Ctrl Pts',(-7.78868218500006,15.2,8.10591276399999));
#245698=CARTESIAN_POINT('Ctrl Pts',(-7.79187498300006,15.2,8.10726643599999));
#245699=CARTESIAN_POINT('Ctrl Pts',(-7.79507325100005,15.2,8.10861946999999));
#245700=CARTESIAN_POINT('Ctrl Pts',(-7.79827698300006,15.2,8.10997185699998));
#245701=CARTESIAN_POINT('Ctrl Pts',(-7.80148617400006,15.2,8.11132358799998));
#245702=CARTESIAN_POINT('Ctrl Pts',(-7.80470082000006,15.2,8.11267465299998));
#245703=CARTESIAN_POINT('Ctrl Pts',(-7.80792091500006,15.2,8.11402504599998));
#245704=CARTESIAN_POINT('Ctrl Pts',(-7.81114645400006,15.2,8.11537475499998));
#245705=CARTESIAN_POINT('Ctrl Pts',(-7.81437743500006,15.2,8.11672377399999));
#245706=CARTESIAN_POINT('Ctrl Pts',(-7.81761384900006,15.2,8.11807209299998));
#245707=CARTESIAN_POINT('Ctrl Pts',(-7.82085569500006,15.2,8.11941970299999));
#245708=CARTESIAN_POINT('Ctrl Pts',(-7.82410296500006,15.2,8.12076659599999));
#245709=CARTESIAN_POINT('Ctrl Pts',(-7.82735565600006,15.2,8.12211276299998));
#245710=CARTESIAN_POINT('Ctrl Pts',(-7.83061376200005,15.2,8.12345819399999));
#245711=CARTESIAN_POINT('Ctrl Pts',(-7.83387728100006,15.2,8.12480288399998));
#245712=CARTESIAN_POINT('Ctrl Pts',(-7.83714620400006,15.2,8.12614681999998));
#245713=CARTESIAN_POINT('Ctrl Pts',(-7.84042053000006,15.2,8.12748999699998));
#245714=CARTESIAN_POINT('Ctrl Pts',(-7.84370025300006,15.2,8.12883240399999));
#245715=CARTESIAN_POINT('Ctrl Pts',(-7.84698536600006,15.2,8.13017403499998));
#245716=CARTESIAN_POINT('Ctrl Pts',(-7.85027586700006,15.2,8.13151487799999));
#245717=CARTESIAN_POINT('Ctrl Pts',(-7.85357175000006,15.2,8.13285492699999));
#245718=CARTESIAN_POINT('Ctrl Pts',(-7.85687301000006,15.2,8.13419417299999));
#245719=CARTESIAN_POINT('Ctrl Pts',(-7.86017964300005,15.2,8.13553260699998));
#245720=CARTESIAN_POINT('Ctrl Pts',(-7.86349164400006,15.2,8.13687022099998));
#245721=CARTESIAN_POINT('Ctrl Pts',(-7.86680900800006,15.2,8.13820700699999));
#245722=CARTESIAN_POINT('Ctrl Pts',(-7.87013173000006,15.2,8.13954295599999));
#245723=CARTESIAN_POINT('Ctrl Pts',(-7.87345980500006,15.2,8.14087805999998));
#245724=CARTESIAN_POINT('Ctrl Pts',(-7.87679322900006,15.2,8.14221230999999));
#245725=CARTESIAN_POINT('Ctrl Pts',(-7.88013199700006,15.2,8.14354569699999));
#245726=CARTESIAN_POINT('Ctrl Pts',(-7.88347610400006,15.2,8.14487821399998));
#245727=CARTESIAN_POINT('Ctrl Pts',(-7.88682554500006,15.2,8.14620985299998));
#245728=CARTESIAN_POINT('Ctrl Pts',(-7.89018031600006,15.2,8.14754060399999));
#245729=CARTESIAN_POINT('Ctrl Pts',(-7.89354041200006,15.2,8.14887045999999));
#245730=CARTESIAN_POINT('Ctrl Pts',(-7.89690582700005,15.2,8.15019941199999));
#245731=CARTESIAN_POINT('Ctrl Pts',(-7.90027655700006,15.2,8.15152745299999));
#245732=CARTESIAN_POINT('Ctrl Pts',(-7.90365259800006,15.2,8.15285457299998));
#245733=CARTESIAN_POINT('Ctrl Pts',(-7.90703394500006,15.2,8.15418076499999));
#245734=CARTESIAN_POINT('Ctrl Pts',(-7.91042059300005,15.2,8.15550602099999));
#245735=CARTESIAN_POINT('Ctrl Pts',(-7.91381253600005,15.2,8.15683033199999));
#245736=CARTESIAN_POINT('Ctrl Pts',(-7.91720977000006,15.2,8.15815368899998));
#245737=CARTESIAN_POINT('Ctrl Pts',(-7.92061229100005,15.2,8.15947608599998));
#245738=CARTESIAN_POINT('Ctrl Pts',(-7.92402009400006,15.2,8.16079751399998));
#245739=CARTESIAN_POINT('Ctrl Pts',(-7.92743317500006,15.2,8.16211796399998));
#245740=CARTESIAN_POINT('Ctrl Pts',(-7.93085152700005,15.2,8.16343742899999));
#245741=CARTESIAN_POINT('Ctrl Pts',(-7.93427514700006,15.2,8.16475590099999));
#245742=CARTESIAN_POINT('Ctrl Pts',(-7.93770402900006,15.2,8.16607337199999));
#245743=CARTESIAN_POINT('Ctrl Pts',(-7.94113817000006,15.2,8.16738983299999));
#245744=CARTESIAN_POINT('Ctrl Pts',(-7.94457756400006,15.2,8.16870527599999));
#245745=CARTESIAN_POINT('Ctrl Pts',(-7.94802220600006,15.2,8.17001969299999));
#245746=CARTESIAN_POINT('Ctrl Pts',(-7.95147209200006,15.2,8.17133307699999));
#245747=CARTESIAN_POINT('Ctrl Pts',(-7.95492721600005,15.2,8.17264541999998));
#245748=CARTESIAN_POINT('Ctrl Pts',(-7.95838757500006,15.2,8.17395671299998));
#245749=CARTESIAN_POINT('Ctrl Pts',(-7.96185316300006,15.2,8.17526694799999));
#245750=CARTESIAN_POINT('Ctrl Pts',(-7.96532397700006,15.2,8.17657611899998));
#245751=CARTESIAN_POINT('Ctrl Pts',(-7.96880001000006,15.2,8.17788421699999));
#245752=CARTESIAN_POINT('Ctrl Pts',(-7.97228126000006,15.2,8.17919123499999));
#245753=CARTESIAN_POINT('Ctrl Pts',(-7.97576771900006,15.2,8.18049716399998));
#245754=CARTESIAN_POINT('Ctrl Pts',(-7.97925938500006,15.2,8.18180199599999));
#245755=CARTESIAN_POINT('Ctrl Pts',(-7.98275625000005,15.2,8.18310572199999));
#245756=CARTESIAN_POINT('Ctrl Pts',(-7.98625831300006,15.2,8.18440833599999));
#245757=CARTESIAN_POINT('Ctrl Pts',(-7.98976556600006,15.2,8.18570982799999));
#245758=CARTESIAN_POINT('Ctrl Pts',(-7.99327800400006,15.2,8.18701019299999));
#245759=CARTESIAN_POINT('Ctrl Pts',(-7.99679562600006,15.2,8.18830942099999));
#245760=CARTESIAN_POINT('Ctrl Pts',(-8.00031842500006,15.2,8.18960750499999));
#245761=CARTESIAN_POINT('Ctrl Pts',(-8.00384639600006,15.2,8.19090443999999));
#245762=CARTESIAN_POINT('Ctrl Pts',(-8.00737953700006,15.2,8.19220021799998));
#245763=CARTESIAN_POINT('Ctrl Pts',(-8.01091784300005,15.2,8.19349483199998));
#245764=CARTESIAN_POINT('Ctrl Pts',(-8.01446130800005,15.2,8.19478827199998));
#245765=CARTESIAN_POINT('Ctrl Pts',(-8.01800992700005,15.2,8.19608053199998));
#245766=CARTESIAN_POINT('Ctrl Pts',(-8.02156369500005,15.2,8.19737160199999));
#245767=CARTESIAN_POINT('Ctrl Pts',(-8.02512260400006,15.2,8.19866146999999));
#245768=CARTESIAN_POINT('Ctrl Pts',(-8.02868665100006,15.2,8.19995012899999));
#245769=CARTESIAN_POINT('Ctrl Pts',(-8.03225583000006,15.2,8.20123757099999));
#245770=CARTESIAN_POINT('Ctrl Pts',(-8.03583013500005,15.2,8.20252378799999));
#245771=CARTESIAN_POINT('Ctrl Pts',(-8.03940956400006,15.2,8.20380877499998));
#245772=CARTESIAN_POINT('Ctrl Pts',(-8.04299411600006,15.2,8.20509252899999));
#245773=CARTESIAN_POINT('Ctrl Pts',(-8.04658378800006,15.2,8.20637504799999));
#245774=CARTESIAN_POINT('Ctrl Pts',(-8.04945962200006,15.2,8.20740007499998));
#245775=CARTESIAN_POINT('Ctrl Pts',(-8.05161880100006,15.2,8.20816828899999));
#245776=CARTESIAN_POINT('Ctrl Pts',(-8.05305927800006,15.2,8.20868018399998));
#245777=CARTESIAN_POINT('Ctrl Pts',(-8.05377977200006,15.2,8.20893606999999));
#245778=CARTESIAN_POINT('Ctrl Pts',(-7.01216898600006,12.2,7.64657512399998));
#245779=CARTESIAN_POINT('Ctrl Pts',(-7.01229743700006,12.2,7.64669302599999));
#245780=CARTESIAN_POINT('Ctrl Pts',(-7.01255888300006,12.2,7.64693288499998));
#245781=CARTESIAN_POINT('Ctrl Pts',(-7.01295521800006,12.2,7.64729613499998));
#245782=CARTESIAN_POINT('Ctrl Pts',(-7.01348948000006,12.2,7.64778506499999));
#245783=CARTESIAN_POINT('Ctrl Pts',(-7.01416585900006,12.2,7.64840281599999));
#245784=CARTESIAN_POINT('Ctrl Pts',(-7.01485383100006,12.2,7.64902988999999));
#245785=CARTESIAN_POINT('Ctrl Pts',(-7.01554947000006,12.2,7.64966267399998));
#245786=CARTESIAN_POINT('Ctrl Pts',(-7.01625276700006,12.2,7.65030113899999));
#245787=CARTESIAN_POINT('Ctrl Pts',(-7.01696371600006,12.2,7.65094525299999));
#245788=CARTESIAN_POINT('Ctrl Pts',(-7.01768230900006,12.2,7.65159498499998));
#245789=CARTESIAN_POINT('Ctrl Pts',(-7.01840853600006,12.2,7.65225030299998));
#245790=CARTESIAN_POINT('Ctrl Pts',(-7.01914239300006,12.2,7.65291117499999));
#245791=CARTESIAN_POINT('Ctrl Pts',(-7.01988387000006,12.2,7.65357757299999));
#245792=CARTESIAN_POINT('Ctrl Pts',(-7.02063296000006,12.2,7.65424946399998));
#245793=CARTESIAN_POINT('Ctrl Pts',(-7.02138965700006,12.2,7.65492681899998));
#245794=CARTESIAN_POINT('Ctrl Pts',(-7.02215395000006,12.2,7.65560960799998));
#245795=CARTESIAN_POINT('Ctrl Pts',(-7.02292583400006,12.2,7.65629779899999));
#245796=CARTESIAN_POINT('Ctrl Pts',(-7.02370530000006,12.2,7.65699136299999));
#245797=CARTESIAN_POINT('Ctrl Pts',(-7.02449234200006,12.2,7.65769026899999));
#245798=CARTESIAN_POINT('Ctrl Pts',(-7.02528695100006,12.2,7.65839448899998));
#245799=CARTESIAN_POINT('Ctrl Pts',(-7.02608912200006,12.2,7.65910399299998));
#245800=CARTESIAN_POINT('Ctrl Pts',(-7.02689884500006,12.2,7.65981874999999));
#245801=CARTESIAN_POINT('Ctrl Pts',(-7.02771611300006,12.2,7.66053873299998));
#245802=CARTESIAN_POINT('Ctrl Pts',(-7.02854092000006,12.2,7.66126390999998));
#245803=CARTESIAN_POINT('Ctrl Pts',(-7.02937325800006,12.2,7.66199425499998));
#245804=CARTESIAN_POINT('Ctrl Pts',(-7.03021311900006,12.2,7.66272973699999));
#245805=CARTESIAN_POINT('Ctrl Pts',(-7.03106049600006,12.2,7.66347032799998));
#245806=CARTESIAN_POINT('Ctrl Pts',(-7.03191538200006,12.2,7.66421599899999));
#245807=CARTESIAN_POINT('Ctrl Pts',(-7.03277777000006,12.2,7.66496672199998));
#245808=CARTESIAN_POINT('Ctrl Pts',(-7.03364765200006,12.2,7.66572246899998));
#245809=CARTESIAN_POINT('Ctrl Pts',(-7.03452502100006,12.2,7.66648321099999));
#245810=CARTESIAN_POINT('Ctrl Pts',(-7.03540987000006,12.2,7.66724892099998));
#245811=CARTESIAN_POINT('Ctrl Pts',(-7.03630219100006,12.2,7.66801956799998));
#245812=CARTESIAN_POINT('Ctrl Pts',(-7.03720197800005,12.2,7.66879512799999));
#245813=CARTESIAN_POINT('Ctrl Pts',(-7.03810922400006,12.2,7.66957557299998));
#245814=CARTESIAN_POINT('Ctrl Pts',(-7.03902392100006,12.2,7.67036087199998));
#245815=CARTESIAN_POINT('Ctrl Pts',(-7.03994606100006,12.2,7.67115099999998));
#245816=CARTESIAN_POINT('Ctrl Pts',(-7.04087563900006,12.2,7.67194592999999));
#245817=CARTESIAN_POINT('Ctrl Pts',(-7.04181264600006,12.2,7.67274563399998));
#245818=CARTESIAN_POINT('Ctrl Pts',(-7.04275707700006,12.2,7.67355008599999));
#245819=CARTESIAN_POINT('Ctrl Pts',(-7.04370892200005,12.2,7.67435925699999));
#245820=CARTESIAN_POINT('Ctrl Pts',(-7.04466817800006,12.2,7.67517312299999));
#245821=CARTESIAN_POINT('Ctrl Pts',(-7.04563483400006,12.2,7.67599165499998));
#245822=CARTESIAN_POINT('Ctrl Pts',(-7.04660888600006,12.2,7.67681482699999));
#245823=CARTESIAN_POINT('Ctrl Pts',(-7.04759032400006,12.2,7.67764261299998));
#245824=CARTESIAN_POINT('Ctrl Pts',(-7.04857914400006,12.2,7.67847498699999));
#245825=CARTESIAN_POINT('Ctrl Pts',(-7.04957533900005,12.2,7.67931192299999));
#245826=CARTESIAN_POINT('Ctrl Pts',(-7.05057890000006,12.2,7.68015339299998));
#245827=CARTESIAN_POINT('Ctrl Pts',(-7.05158982000006,12.2,7.68099937399998));
#245828=CARTESIAN_POINT('Ctrl Pts',(-7.05260809400006,12.2,7.68184983699999));
#245829=CARTESIAN_POINT('Ctrl Pts',(-7.05363371500006,12.2,7.68270475799999));
#245830=CARTESIAN_POINT('Ctrl Pts',(-7.05466667400006,12.2,7.68356411099998));
#245831=CARTESIAN_POINT('Ctrl Pts',(-7.05570696700006,12.2,7.68442787099998));
#245832=CARTESIAN_POINT('Ctrl Pts',(-7.05675458400005,12.2,7.68529601199998));
#245833=CARTESIAN_POINT('Ctrl Pts',(-7.05780952100006,12.2,7.68616850899999));
#245834=CARTESIAN_POINT('Ctrl Pts',(-7.05887177100006,12.2,7.68704533799998));
#245835=CARTESIAN_POINT('Ctrl Pts',(-7.05994132500006,12.2,7.68792647199999));
#245836=CARTESIAN_POINT('Ctrl Pts',(-7.06101817900006,12.2,7.68881188699999));
#245837=CARTESIAN_POINT('Ctrl Pts',(-7.06210232400006,12.2,7.68970155699999));
#245838=CARTESIAN_POINT('Ctrl Pts',(-7.06319375500006,12.2,7.69059545999998));
#245839=CARTESIAN_POINT('Ctrl Pts',(-7.06429246300006,12.2,7.69149356899998));
#245840=CARTESIAN_POINT('Ctrl Pts',(-7.06539844400006,12.2,7.69239585999999));
#245841=CARTESIAN_POINT('Ctrl Pts',(-7.06651169000006,12.2,7.69330230899998));
#245842=CARTESIAN_POINT('Ctrl Pts',(-7.06763219400006,12.2,7.69421289099999));
#245843=CARTESIAN_POINT('Ctrl Pts',(-7.06875995000006,12.2,7.69512758399999));
#245844=CARTESIAN_POINT('Ctrl Pts',(-7.06989495100006,12.2,7.69604635999999));
#245845=CARTESIAN_POINT('Ctrl Pts',(-7.07103719100005,12.2,7.69696919799999));
#245846=CARTESIAN_POINT('Ctrl Pts',(-7.07218666200006,12.2,7.69789607499998));
#245847=CARTESIAN_POINT('Ctrl Pts',(-7.07334335900006,12.2,7.69882696299998));
#245848=CARTESIAN_POINT('Ctrl Pts',(-7.07450727400006,12.2,7.69976184299999));
#245849=CARTESIAN_POINT('Ctrl Pts',(-7.07567840200006,12.2,7.70070068799999));
#245850=CARTESIAN_POINT('Ctrl Pts',(-7.07685673500006,12.2,7.70164347599999));
#245851=CARTESIAN_POINT('Ctrl Pts',(-7.07804226800006,12.2,7.70259018399998));
#245852=CARTESIAN_POINT('Ctrl Pts',(-7.07923499300006,12.2,7.70354078799999));
#245853=CARTESIAN_POINT('Ctrl Pts',(-7.08043490300006,12.2,7.70449526499998));
#245854=CARTESIAN_POINT('Ctrl Pts',(-7.08164199400006,12.2,7.70545359099999));
#245855=CARTESIAN_POINT('Ctrl Pts',(-7.08285625800006,12.2,7.70641574499999));
#245856=CARTESIAN_POINT('Ctrl Pts',(-7.08407768800006,12.2,7.70738170199999));
#245857=CARTESIAN_POINT('Ctrl Pts',(-7.08530627800006,12.2,7.70835144099999));
#245858=CARTESIAN_POINT('Ctrl Pts',(-7.08654202200006,12.2,7.70932493899998));
#245859=CARTESIAN_POINT('Ctrl Pts',(-7.08778491400006,12.2,7.71030217199999));
#245860=CARTESIAN_POINT('Ctrl Pts',(-7.08903494500006,12.2,7.71128311899999));
#245861=CARTESIAN_POINT('Ctrl Pts',(-7.09029211200006,12.2,7.71226775599998));
#245862=CARTESIAN_POINT('Ctrl Pts',(-7.09155640600006,12.2,7.71325606199999));
#245863=CARTESIAN_POINT('Ctrl Pts',(-7.09282782300006,12.2,7.71424801399998));
#245864=CARTESIAN_POINT('Ctrl Pts',(-7.09410635400006,12.2,7.71524359099999));
#245865=CARTESIAN_POINT('Ctrl Pts',(-7.09539199400006,12.2,7.71624276799999));
#245866=CARTESIAN_POINT('Ctrl Pts',(-7.09668473700006,12.2,7.71724552699999));
#245867=CARTESIAN_POINT('Ctrl Pts',(-7.09798457700006,12.2,7.71825184399999));
#245868=CARTESIAN_POINT('Ctrl Pts',(-7.09929150500006,12.2,7.71926169699999));
#245869=CARTESIAN_POINT('Ctrl Pts',(-7.10060551800006,12.2,7.72027506499998));
#245870=CARTESIAN_POINT('Ctrl Pts',(-7.10192660800006,12.2,7.72129192499998));
#245871=CARTESIAN_POINT('Ctrl Pts',(-7.10325476900006,12.2,7.72231225799998));
#245872=CARTESIAN_POINT('Ctrl Pts',(-7.10458999400006,12.2,7.72333603999999));
#245873=CARTESIAN_POINT('Ctrl Pts',(-7.10593227900006,12.2,7.72436325099999));
#245874=CARTESIAN_POINT('Ctrl Pts',(-7.10728161500006,12.2,7.72539386899999));
#245875=CARTESIAN_POINT('Ctrl Pts',(-7.10863799800006,12.2,7.72642787299999));
#245876=CARTESIAN_POINT('Ctrl Pts',(-7.11000142000006,12.2,7.72746524299999));
#245877=CARTESIAN_POINT('Ctrl Pts',(-7.11137187600006,12.2,7.72850595599999));
#245878=CARTESIAN_POINT('Ctrl Pts',(-7.11274935900006,12.2,7.72954999299999));
#245879=CARTESIAN_POINT('Ctrl Pts',(-7.11413386400006,12.2,7.73059733099998));
#245880=CARTESIAN_POINT('Ctrl Pts',(-7.11552538300006,12.2,7.73164795099999));
#245881=CARTESIAN_POINT('Ctrl Pts',(-7.11692391100006,12.2,7.73270183099999));
#245882=CARTESIAN_POINT('Ctrl Pts',(-7.11832944100006,12.2,7.73375895199998));
#245883=CARTESIAN_POINT('Ctrl Pts',(-7.11974196900006,12.2,7.73481929199999));
#245884=CARTESIAN_POINT('Ctrl Pts',(-7.12116148600006,12.2,7.73588283099999));
#245885=CARTESIAN_POINT('Ctrl Pts',(-7.12258798800006,12.2,7.73694954699998));
#245886=CARTESIAN_POINT('Ctrl Pts',(-7.12402146800006,12.2,7.73801942399999));
#245887=CARTESIAN_POINT('Ctrl Pts',(-7.12546192000006,12.2,7.73909243699999));
#245888=CARTESIAN_POINT('Ctrl Pts',(-7.12690933700006,12.2,7.74016856899999));
#245889=CARTESIAN_POINT('Ctrl Pts',(-7.12836371400006,12.2,7.74124779699999));
#245890=CARTESIAN_POINT('Ctrl Pts',(-7.12982504600006,12.2,7.74233010399998));
#245891=CARTESIAN_POINT('Ctrl Pts',(-7.13129332400006,12.2,7.74341546899999));
#245892=CARTESIAN_POINT('Ctrl Pts',(-7.13276854400006,12.2,7.74450386999998));
#245893=CARTESIAN_POINT('Ctrl Pts',(-7.13425070000006,12.2,7.74559529099999));
#245894=CARTESIAN_POINT('Ctrl Pts',(-7.13573978500006,12.2,7.74668970999999));
#245895=CARTESIAN_POINT('Ctrl Pts',(-7.13723579400006,12.2,7.74778710799998));
#245896=CARTESIAN_POINT('Ctrl Pts',(-7.13873872000006,12.2,7.74888746499999));
#245897=CARTESIAN_POINT('Ctrl Pts',(-7.14024855600006,12.2,7.74999076199999));
#245898=CARTESIAN_POINT('Ctrl Pts',(-7.14176530000006,12.2,7.75109697799999));
#245899=CARTESIAN_POINT('Ctrl Pts',(-7.14328894200006,12.2,7.75220609499998));
#245900=CARTESIAN_POINT('Ctrl Pts',(-7.14481947700006,12.2,7.75331809499999));
#245901=CARTESIAN_POINT('Ctrl Pts',(-7.14635690000006,12.2,7.75443295699999));
#245902=CARTESIAN_POINT('Ctrl Pts',(-7.14790120500005,12.2,7.75555066199999));
#245903=CARTESIAN_POINT('Ctrl Pts',(-7.14945238500006,12.2,7.75667119099998));
#245904=CARTESIAN_POINT('Ctrl Pts',(-7.15101043300006,12.2,7.75779452499999));
#245905=CARTESIAN_POINT('Ctrl Pts',(-7.15257534700006,12.2,7.75892064699998));
#245906=CARTESIAN_POINT('Ctrl Pts',(-7.15414711700006,12.2,7.76004953499999));
#245907=CARTESIAN_POINT('Ctrl Pts',(-7.15572573900006,12.2,7.76118117199999));
#245908=CARTESIAN_POINT('Ctrl Pts',(-7.15731120800006,12.2,7.76231553799998));
#245909=CARTESIAN_POINT('Ctrl Pts',(-7.15890351700006,12.2,7.76345261699999));
#245910=CARTESIAN_POINT('Ctrl Pts',(-7.16050265800006,12.2,7.76459238699999));
#245911=CARTESIAN_POINT('Ctrl Pts',(-7.16210862800006,12.2,7.76573483199999));
#245912=CARTESIAN_POINT('Ctrl Pts',(-7.16372142100006,12.2,7.76687993299999));
#245913=CARTESIAN_POINT('Ctrl Pts',(-7.16534103000006,12.2,7.76802766999998));
#245914=CARTESIAN_POINT('Ctrl Pts',(-7.16696745000006,12.2,7.76917802599999));
#245915=CARTESIAN_POINT('Ctrl Pts',(-7.16860067400006,12.2,7.77033098499999));
#245916=CARTESIAN_POINT('Ctrl Pts',(-7.17024069700006,12.2,7.77148652499999));
#245917=CARTESIAN_POINT('Ctrl Pts',(-7.17188751300006,12.2,7.77264462899999));
#245918=CARTESIAN_POINT('Ctrl Pts',(-7.17354111600006,12.2,7.77380527999998));
#245919=CARTESIAN_POINT('Ctrl Pts',(-7.17520150000006,12.2,7.77496845799998));
#245920=CARTESIAN_POINT('Ctrl Pts',(-7.17686866000006,12.2,7.77613414899999));
#245921=CARTESIAN_POINT('Ctrl Pts',(-7.17854259000006,12.2,7.77730232999998));
#245922=CARTESIAN_POINT('Ctrl Pts',(-7.18022328300005,12.2,7.77847298699999));
#245923=CARTESIAN_POINT('Ctrl Pts',(-7.18191073400006,12.2,7.77964609999999));
#245924=CARTESIAN_POINT('Ctrl Pts',(-7.18360493800006,12.2,7.78082165399999));
#245925=CARTESIAN_POINT('Ctrl Pts',(-7.18530588900006,12.2,7.78199962799999));
#245926=CARTESIAN_POINT('Ctrl Pts',(-7.18701358000006,12.2,7.78318000699999));
#245927=CARTESIAN_POINT('Ctrl Pts',(-7.18872800700006,12.2,7.78436277199998));
#245928=CARTESIAN_POINT('Ctrl Pts',(-7.19044916200006,12.2,7.78554790599999));
#245929=CARTESIAN_POINT('Ctrl Pts',(-7.19217704100005,12.2,7.78673539199998));
#245930=CARTESIAN_POINT('Ctrl Pts',(-7.19391163700006,12.2,7.78792521199998));
#245931=CARTESIAN_POINT('Ctrl Pts',(-7.19565294600006,12.2,7.78911734999999));
#245932=CARTESIAN_POINT('Ctrl Pts',(-7.19740096200006,12.2,7.79031178799999));
#245933=CARTESIAN_POINT('Ctrl Pts',(-7.19915567700006,12.2,7.79150850799999));
#245934=CARTESIAN_POINT('Ctrl Pts',(-7.20091708800005,12.2,7.79270749399998));
#245935=CARTESIAN_POINT('Ctrl Pts',(-7.20268518700006,12.2,7.79390872899998));
#245936=CARTESIAN_POINT('Ctrl Pts',(-7.20445997000006,12.2,7.79511219599998));
#245937=CARTESIAN_POINT('Ctrl Pts',(-7.20624143100006,12.2,7.79631787699999));
#245938=CARTESIAN_POINT('Ctrl Pts',(-7.20802956400005,12.2,7.79752575699998));
#245939=CARTESIAN_POINT('Ctrl Pts',(-7.20982436400006,12.2,7.79873581599999));
#245940=CARTESIAN_POINT('Ctrl Pts',(-7.21162582400006,12.2,7.79994804199998));
#245941=CARTESIAN_POINT('Ctrl Pts',(-7.21343393900006,12.2,7.80116241399998));
#245942=CARTESIAN_POINT('Ctrl Pts',(-7.21524870400006,12.2,7.80237891799998));
#245943=CARTESIAN_POINT('Ctrl Pts',(-7.21707011300006,12.2,7.80359753599999));
#245944=CARTESIAN_POINT('Ctrl Pts',(-7.21889815900006,12.2,7.80481825199999));
#245945=CARTESIAN_POINT('Ctrl Pts',(-7.22073283800006,12.2,7.80604104899999));
#245946=CARTESIAN_POINT('Ctrl Pts',(-7.22257414400006,12.2,7.80726591199999));
#245947=CARTESIAN_POINT('Ctrl Pts',(-7.22442207200006,12.2,7.80849282399998));
#245948=CARTESIAN_POINT('Ctrl Pts',(-7.22627661400006,12.2,7.80972176699999));
#245949=CARTESIAN_POINT('Ctrl Pts',(-7.22813776800006,12.2,7.81095272699999));
#245950=CARTESIAN_POINT('Ctrl Pts',(-7.23000552500006,12.2,7.81218568699998));
#245951=CARTESIAN_POINT('Ctrl Pts',(-7.23187988200006,12.2,7.81342063099999));
#245952=CARTESIAN_POINT('Ctrl Pts',(-7.23376083100006,12.2,7.81465754299998));
#245953=CARTESIAN_POINT('Ctrl Pts',(-7.23564836800006,12.2,7.81589640599999));
#245954=CARTESIAN_POINT('Ctrl Pts',(-7.23754248700006,12.2,7.81713720599999));
#245955=CARTESIAN_POINT('Ctrl Pts',(-7.23944318300005,12.2,7.81837992399999));
#245956=CARTESIAN_POINT('Ctrl Pts',(-7.24135045000006,12.2,7.81962454799999));
#245957=CARTESIAN_POINT('Ctrl Pts',(-7.24326428200006,12.2,7.82087105799998));
#245958=CARTESIAN_POINT('Ctrl Pts',(-7.24518467300006,12.2,7.82211944199998));
#245959=CARTESIAN_POINT('Ctrl Pts',(-7.24711162000006,12.2,7.82336968199999));
#245960=CARTESIAN_POINT('Ctrl Pts',(-7.24904511400006,12.2,7.82462176199999));
#245961=CARTESIAN_POINT('Ctrl Pts',(-7.25098515300005,12.2,7.82587566899998));
#245962=CARTESIAN_POINT('Ctrl Pts',(-7.25293172800006,12.2,7.82713138499999));
#245963=CARTESIAN_POINT('Ctrl Pts',(-7.25488483700006,12.2,7.82838889399999));
#245964=CARTESIAN_POINT('Ctrl Pts',(-7.25684447100006,12.2,7.82964818299998));
#245965=CARTESIAN_POINT('Ctrl Pts',(-7.25881062600005,12.2,7.83090923599998));
#245966=CARTESIAN_POINT('Ctrl Pts',(-7.26078329800006,12.2,7.83217203499999));
#245967=CARTESIAN_POINT('Ctrl Pts',(-7.26276247900006,12.2,7.83343656799998));
#245968=CARTESIAN_POINT('Ctrl Pts',(-7.26474816500006,12.2,7.83470281899999));
#245969=CARTESIAN_POINT('Ctrl Pts',(-7.26674035000006,12.2,7.83597076999998));
#245970=CARTESIAN_POINT('Ctrl Pts',(-7.26873902900006,12.2,7.83724040899998));
#245971=CARTESIAN_POINT('Ctrl Pts',(-7.27074419600005,12.2,7.83851171899999));
#245972=CARTESIAN_POINT('Ctrl Pts',(-7.27275584500005,12.2,7.83978468699999));
#245973=CARTESIAN_POINT('Ctrl Pts',(-7.27477397200006,12.2,7.84105929599999));
#245974=CARTESIAN_POINT('Ctrl Pts',(-7.27679857000005,12.2,7.84233553099998));
#245975=CARTESIAN_POINT('Ctrl Pts',(-7.27882963600006,12.2,7.84361337899998));
#245976=CARTESIAN_POINT('Ctrl Pts',(-7.28086716200006,12.2,7.84489282299998));
#245977=CARTESIAN_POINT('Ctrl Pts',(-7.28291114200006,12.2,7.84617384799999));
#245978=CARTESIAN_POINT('Ctrl Pts',(-7.28496157300006,12.2,7.84745644199998));
#245979=CARTESIAN_POINT('Ctrl Pts',(-7.28701844900006,12.2,7.84874058699998));
#245980=CARTESIAN_POINT('Ctrl Pts',(-7.28908176300005,12.2,7.85002626999999));
#245981=CARTESIAN_POINT('Ctrl Pts',(-7.29115151200006,12.2,7.85131347699998));
#245982=CARTESIAN_POINT('Ctrl Pts',(-7.29322768800006,12.2,7.85260219099998));
#245983=CARTESIAN_POINT('Ctrl Pts',(-7.29531028700006,12.2,7.85389239899998));
#245984=CARTESIAN_POINT('Ctrl Pts',(-7.29739930400005,12.2,7.85518408599999));
#245985=CARTESIAN_POINT('Ctrl Pts',(-7.29949473300006,12.2,7.85647723899999));
#245986=CARTESIAN_POINT('Ctrl Pts',(-7.30159656800006,12.2,7.85777184099998));
#245987=CARTESIAN_POINT('Ctrl Pts',(-7.30370480500006,12.2,7.85906787899999));
#245988=CARTESIAN_POINT('Ctrl Pts',(-7.30581943700006,12.2,7.86036533899999));
#245989=CARTESIAN_POINT('Ctrl Pts',(-7.30794046000006,12.2,7.86166420599999));
#245990=CARTESIAN_POINT('Ctrl Pts',(-7.31006786800006,12.2,7.86296446599999));
#245991=CARTESIAN_POINT('Ctrl Pts',(-7.31220165500006,12.2,7.86426610399998));
#245992=CARTESIAN_POINT('Ctrl Pts',(-7.31434181800006,12.2,7.86556910899999));
#245993=CARTESIAN_POINT('Ctrl Pts',(-7.31648834800006,12.2,7.86687346199999));
#245994=CARTESIAN_POINT('Ctrl Pts',(-7.31864124200006,12.2,7.86817915199999));
#245995=CARTESIAN_POINT('Ctrl Pts',(-7.32080049400006,12.2,7.86948616399999));
#245996=CARTESIAN_POINT('Ctrl Pts',(-7.32296610000006,12.2,7.87079448499998));
#245997=CARTESIAN_POINT('Ctrl Pts',(-7.32513805400006,12.2,7.87210409899998));
#245998=CARTESIAN_POINT('Ctrl Pts',(-7.32731634900006,12.2,7.87341499399999));
#245999=CARTESIAN_POINT('Ctrl Pts',(-7.32950098000006,12.2,7.87472715499998));
#246000=CARTESIAN_POINT('Ctrl Pts',(-7.33169194400006,12.2,7.87604056899998));
#246001=CARTESIAN_POINT('Ctrl Pts',(-7.33388923300006,12.2,7.87735522199998));
#246002=CARTESIAN_POINT('Ctrl Pts',(-7.33609284400006,12.2,7.87867109999999));
#246003=CARTESIAN_POINT('Ctrl Pts',(-7.33830277000005,12.2,7.87998818899998));
#246004=CARTESIAN_POINT('Ctrl Pts',(-7.34051900600006,12.2,7.88130647499998));
#246005=CARTESIAN_POINT('Ctrl Pts',(-7.34274154700006,12.2,7.88262594599999));
#246006=CARTESIAN_POINT('Ctrl Pts',(-7.34497038800006,12.2,7.88394658699998));
#246007=CARTESIAN_POINT('Ctrl Pts',(-7.34720552300006,12.2,7.88526838399999));
#246008=CARTESIAN_POINT('Ctrl Pts',(-7.34944694700006,12.2,7.88659132499999));
#246009=CARTESIAN_POINT('Ctrl Pts',(-7.35169465500006,12.2,7.88791539599998));
#246010=CARTESIAN_POINT('Ctrl Pts',(-7.35394864100006,12.2,7.88924058299998));
#246011=CARTESIAN_POINT('Ctrl Pts',(-7.35620890000006,12.2,7.89056687299999));
#246012=CARTESIAN_POINT('Ctrl Pts',(-7.35847542700006,12.2,7.89189425299998));
#246013=CARTESIAN_POINT('Ctrl Pts',(-7.36074821700006,12.2,7.89322270699999));
#246014=CARTESIAN_POINT('Ctrl Pts',(-7.36302726400006,12.2,7.89455222599998));
#246015=CARTESIAN_POINT('Ctrl Pts',(-7.36531256300006,12.2,7.89588279499998));
#246016=CARTESIAN_POINT('Ctrl Pts',(-7.36760410800006,12.2,7.89721439899999));
#246017=CARTESIAN_POINT('Ctrl Pts',(-7.36990189600006,12.2,7.89854702799998));
#246018=CARTESIAN_POINT('Ctrl Pts',(-7.37220591900006,12.2,7.89988066499999));
#246019=CARTESIAN_POINT('Ctrl Pts',(-7.37451617400006,12.2,7.90121529999999));
#246020=CARTESIAN_POINT('Ctrl Pts',(-7.37683265400006,12.2,7.90255091899999));
#246021=CARTESIAN_POINT('Ctrl Pts',(-7.37915535500006,12.2,7.90388750999998));
#246022=CARTESIAN_POINT('Ctrl Pts',(-7.38148427100006,12.2,7.90522505699998));
#246023=CARTESIAN_POINT('Ctrl Pts',(-7.38381939700006,12.2,7.90656354999999));
#246024=CARTESIAN_POINT('Ctrl Pts',(-7.38616072800006,12.2,7.90790297499999));
#246025=CARTESIAN_POINT('Ctrl Pts',(-7.38850825800006,12.2,7.90924331999998));
#246026=CARTESIAN_POINT('Ctrl Pts',(-7.39086198300006,12.2,7.91058456999998));
#246027=CARTESIAN_POINT('Ctrl Pts',(-7.39322189600006,12.2,7.91192671399998));
#246028=CARTESIAN_POINT('Ctrl Pts',(-7.39558799400006,12.2,7.91326973999999));
#246029=CARTESIAN_POINT('Ctrl Pts',(-7.39796027100006,12.2,7.91461363299998));
#246030=CARTESIAN_POINT('Ctrl Pts',(-7.40033872100006,12.2,7.91595838099998));
#246031=CARTESIAN_POINT('Ctrl Pts',(-7.40272333900006,12.2,7.91730397299999));
#246032=CARTESIAN_POINT('Ctrl Pts',(-7.40511412000005,12.2,7.91865039499999));
#246033=CARTESIAN_POINT('Ctrl Pts',(-7.40751105900006,12.2,7.91999763299999));
#246034=CARTESIAN_POINT('Ctrl Pts',(-7.40991415200006,12.2,7.92134567699998));
#246035=CARTESIAN_POINT('Ctrl Pts',(-7.41232339100006,12.2,7.92269451299998));
#246036=CARTESIAN_POINT('Ctrl Pts',(-7.41473877300006,12.2,7.92404412999999));
#246037=CARTESIAN_POINT('Ctrl Pts',(-7.41716029100006,12.2,7.92539451399998));
#246038=CARTESIAN_POINT('Ctrl Pts',(-7.41958794200006,12.2,7.92674565199999));
#246039=CARTESIAN_POINT('Ctrl Pts',(-7.42202171900006,12.2,7.92809753399998));
#246040=CARTESIAN_POINT('Ctrl Pts',(-7.42446161900006,12.2,7.92945014599999));
#246041=CARTESIAN_POINT('Ctrl Pts',(-7.42690763400006,12.2,7.93080347599999));
#246042=CARTESIAN_POINT('Ctrl Pts',(-7.42935976100005,12.2,7.93215751199998));
#246043=CARTESIAN_POINT('Ctrl Pts',(-7.43181799400006,12.2,7.93351224099998));
#246044=CARTESIAN_POINT('Ctrl Pts',(-7.43428232700006,12.2,7.93486765199999));
#246045=CARTESIAN_POINT('Ctrl Pts',(-7.43675275700006,12.2,7.93622373199998));
#246046=CARTESIAN_POINT('Ctrl Pts',(-7.43922927800006,12.2,7.93758046899999));
#246047=CARTESIAN_POINT('Ctrl Pts',(-7.44171188300006,12.2,7.93893784999998));
#246048=CARTESIAN_POINT('Ctrl Pts',(-7.44420057000006,12.2,7.94029586499998));
#246049=CARTESIAN_POINT('Ctrl Pts',(-7.44669533100006,12.2,7.94165450099998));
#246050=CARTESIAN_POINT('Ctrl Pts',(-7.44919616200006,12.2,7.94301374399998));
#246051=CARTESIAN_POINT('Ctrl Pts',(-7.45170305800006,12.2,7.94437358599998));
#246052=CARTESIAN_POINT('Ctrl Pts',(-7.45421601400006,12.2,7.94573401099999));
#246053=CARTESIAN_POINT('Ctrl Pts',(-7.45673502500006,12.2,7.94709500999998));
#246054=CARTESIAN_POINT('Ctrl Pts',(-7.45926008500006,12.2,7.94845657099999));
#246055=CARTESIAN_POINT('Ctrl Pts',(-7.46179119000006,12.2,7.94981867899998));
#246056=CARTESIAN_POINT('Ctrl Pts',(-7.46432833400006,12.2,7.95118132499999));
#246057=CARTESIAN_POINT('Ctrl Pts',(-7.46687151300006,12.2,7.95254449699998));
#246058=CARTESIAN_POINT('Ctrl Pts',(-7.46942072000006,12.2,7.95390818299998));
#246059=CARTESIAN_POINT('Ctrl Pts',(-7.47197595100006,12.2,7.95527237099999));
#246060=CARTESIAN_POINT('Ctrl Pts',(-7.47453720200006,12.2,7.95663704999999));
#246061=CARTESIAN_POINT('Ctrl Pts',(-7.47710446500006,12.2,7.95800220799999));
#246062=CARTESIAN_POINT('Ctrl Pts',(-7.47967773800006,12.2,7.95936783099998));
#246063=CARTESIAN_POINT('Ctrl Pts',(-7.48225701500006,12.2,7.96073391199998));
#246064=CARTESIAN_POINT('Ctrl Pts',(-7.48484228800006,12.2,7.96210043599999));
#246065=CARTESIAN_POINT('Ctrl Pts',(-7.48743355700006,12.2,7.96346739199999));
#246066=CARTESIAN_POINT('Ctrl Pts',(-7.49003081300006,12.2,7.96483476999998));
#246067=CARTESIAN_POINT('Ctrl Pts',(-7.49263405300006,12.2,7.96620255599999));
#246068=CARTESIAN_POINT('Ctrl Pts',(-7.49524327100006,12.2,7.96757074199999));
#246069=CARTESIAN_POINT('Ctrl Pts',(-7.49785846200006,12.2,7.96893931299999));
#246070=CARTESIAN_POINT('Ctrl Pts',(-7.50047962100006,12.2,7.97030825999999));
#246071=CARTESIAN_POINT('Ctrl Pts',(-7.50310674300006,12.2,7.97167757099999));
#246072=CARTESIAN_POINT('Ctrl Pts',(-7.50573982300006,12.2,7.97304723499998));
#246073=CARTESIAN_POINT('Ctrl Pts',(-7.50837885500006,12.2,7.97441723899999));
#246074=CARTESIAN_POINT('Ctrl Pts',(-7.51102383600006,12.2,7.97578757299998));
#246075=CARTESIAN_POINT('Ctrl Pts',(-7.51367475900006,12.2,7.97715822699999));
#246076=CARTESIAN_POINT('Ctrl Pts',(-7.51633162000005,12.2,7.97852918799999));
#246077=CARTESIAN_POINT('Ctrl Pts',(-7.51899441200005,12.2,7.97990044499999));
#246078=CARTESIAN_POINT('Ctrl Pts',(-7.52166313300006,12.2,7.98127198799998));
#246079=CARTESIAN_POINT('Ctrl Pts',(-7.52433777600006,12.2,7.98264380499998));
#246080=CARTESIAN_POINT('Ctrl Pts',(-7.52701833700005,12.2,7.98401588399998));
#246081=CARTESIAN_POINT('Ctrl Pts',(-7.52970481000006,12.2,7.98538821699999));
#246082=CARTESIAN_POINT('Ctrl Pts',(-7.53239719100005,12.2,7.98676078899998));
#246083=CARTESIAN_POINT('Ctrl Pts',(-7.53509547300006,12.2,7.98813359199999));
#246084=CARTESIAN_POINT('Ctrl Pts',(-7.53779965400006,12.2,7.98950661499998));
#246085=CARTESIAN_POINT('Ctrl Pts',(-7.54050972500006,12.2,7.99087984499998));
#246086=CARTESIAN_POINT('Ctrl Pts',(-7.54322568500006,12.2,7.99225327099998));
#246087=CARTESIAN_POINT('Ctrl Pts',(-7.54594752700006,12.2,7.99362688499999));
#246088=CARTESIAN_POINT('Ctrl Pts',(-7.54867524600006,12.2,7.99500067299999));
#246089=CARTESIAN_POINT('Ctrl Pts',(-7.55140883700006,12.2,7.99637462699998));
#246090=CARTESIAN_POINT('Ctrl Pts',(-7.55414829500006,12.2,7.99774873399999));
#246091=CARTESIAN_POINT('Ctrl Pts',(-7.55689361600006,12.2,7.99912298399998));
#246092=CARTESIAN_POINT('Ctrl Pts',(-7.55964479300006,12.2,8.00049736599998));
#246093=CARTESIAN_POINT('Ctrl Pts',(-7.56240182300005,12.2,8.00187187099999));
#246094=CARTESIAN_POINT('Ctrl Pts',(-7.56516470000006,12.2,8.00324648399998));
#246095=CARTESIAN_POINT('Ctrl Pts',(-7.56793341800006,12.2,8.00462119899999));
#246096=CARTESIAN_POINT('Ctrl Pts',(-7.57070797500005,12.2,8.00599600399998));
#246097=CARTESIAN_POINT('Ctrl Pts',(-7.57348836300006,12.2,8.00737088699999));
#246098=CARTESIAN_POINT('Ctrl Pts',(-7.57627457800006,12.2,8.00874583799999));
#246099=CARTESIAN_POINT('Ctrl Pts',(-7.57906661600006,12.2,8.01012084699998));
#246100=CARTESIAN_POINT('Ctrl Pts',(-7.58186447000006,12.2,8.01149590299998));
#246101=CARTESIAN_POINT('Ctrl Pts',(-7.58466813600006,12.2,8.01287099699999));
#246102=CARTESIAN_POINT('Ctrl Pts',(-7.58747761100006,12.2,8.01424611599998));
#246103=CARTESIAN_POINT('Ctrl Pts',(-7.59029288700006,12.2,8.01562125099998));
#246104=CARTESIAN_POINT('Ctrl Pts',(-7.59311396000006,12.2,8.01699639099999));
#246105=CARTESIAN_POINT('Ctrl Pts',(-7.59594082600006,12.2,8.01837152699999));
#246106=CARTESIAN_POINT('Ctrl Pts',(-7.59877347800006,12.2,8.01974664699999));
#246107=CARTESIAN_POINT('Ctrl Pts',(-7.60161191400006,12.2,8.02112174099998));
#246108=CARTESIAN_POINT('Ctrl Pts',(-7.60445612600006,12.2,8.02249679899998));
#246109=CARTESIAN_POINT('Ctrl Pts',(-7.60730611100006,12.2,8.02387180999999));
#246110=CARTESIAN_POINT('Ctrl Pts',(-7.61016186300005,12.2,8.02524676499999));
#246111=CARTESIAN_POINT('Ctrl Pts',(-7.61302337700006,12.2,8.02662165399998));
#246112=CARTESIAN_POINT('Ctrl Pts',(-7.61589065000006,12.2,8.02799646399999));
#246113=CARTESIAN_POINT('Ctrl Pts',(-7.61876367500006,12.2,8.02937118799999));
#246114=CARTESIAN_POINT('Ctrl Pts',(-7.62164244700006,12.2,8.03074581399999));
#246115=CARTESIAN_POINT('Ctrl Pts',(-7.62452696100006,12.2,8.03212033199999));
#246116=CARTESIAN_POINT('Ctrl Pts',(-7.62741721300006,12.2,8.03349473299999));
#246117=CARTESIAN_POINT('Ctrl Pts',(-7.63031319900006,12.2,8.03486900599999));
#246118=CARTESIAN_POINT('Ctrl Pts',(-7.63321491200006,12.2,8.03624313999999));
#246119=CARTESIAN_POINT('Ctrl Pts',(-7.63612234700006,12.2,8.03761712699998));
#246120=CARTESIAN_POINT('Ctrl Pts',(-7.63903550100006,12.2,8.03899095599999));
#246121=CARTESIAN_POINT('Ctrl Pts',(-7.64195436800006,12.2,8.04036461599999));
#246122=CARTESIAN_POINT('Ctrl Pts',(-7.64487894200006,12.2,8.04173809899999));
#246123=CARTESIAN_POINT('Ctrl Pts',(-7.64780922000006,12.2,8.04311139499998));
#246124=CARTESIAN_POINT('Ctrl Pts',(-7.65074519600006,12.2,8.04448449199998));
#246125=CARTESIAN_POINT('Ctrl Pts',(-7.65368686500006,12.2,8.04585738099998));
#246126=CARTESIAN_POINT('Ctrl Pts',(-7.65663422300006,12.2,8.04723005299999));
#246127=CARTESIAN_POINT('Ctrl Pts',(-7.65958726300005,12.2,8.04860249699999));
#246128=CARTESIAN_POINT('Ctrl Pts',(-7.66254598200005,12.2,8.04997470299998));
#246129=CARTESIAN_POINT('Ctrl Pts',(-7.66551037500006,12.2,8.05134666399999));
#246130=CARTESIAN_POINT('Ctrl Pts',(-7.66848043700006,12.2,8.05271836699998));
#246131=CARTESIAN_POINT('Ctrl Pts',(-7.67145616200006,12.2,8.05408980299998));
#246132=CARTESIAN_POINT('Ctrl Pts',(-7.67443754600006,12.2,8.05546096299998));
#246133=CARTESIAN_POINT('Ctrl Pts',(-7.67742458300006,12.2,8.05683183699998));
#246134=CARTESIAN_POINT('Ctrl Pts',(-7.68041727000006,12.2,8.05820241499998));
#246135=CARTESIAN_POINT('Ctrl Pts',(-7.68341560100006,12.2,8.05957268799999));
#246136=CARTESIAN_POINT('Ctrl Pts',(-7.68641957100006,12.2,8.06094264599999));
#246137=CARTESIAN_POINT('Ctrl Pts',(-7.68942917500006,12.2,8.06231227899998));
#246138=CARTESIAN_POINT('Ctrl Pts',(-7.69244440900006,12.2,8.06368157799999));
#246139=CARTESIAN_POINT('Ctrl Pts',(-7.69546526600006,12.2,8.06505053299999));
#246140=CARTESIAN_POINT('Ctrl Pts',(-7.69849174400005,12.2,8.06641913399999));
#246141=CARTESIAN_POINT('Ctrl Pts',(-7.70152383600006,12.2,8.06778737399998));
#246142=CARTESIAN_POINT('Ctrl Pts',(-7.70456153900006,12.2,8.06915523999999));
#246143=CARTESIAN_POINT('Ctrl Pts',(-7.70760484600006,12.2,8.07052272399999));
#246144=CARTESIAN_POINT('Ctrl Pts',(-7.71065375300005,12.2,8.07188981699999));
#246145=CARTESIAN_POINT('Ctrl Pts',(-7.71370825500006,12.2,8.07325650899998));
#246146=CARTESIAN_POINT('Ctrl Pts',(-7.71676834800005,12.2,8.07462279199999));
#246147=CARTESIAN_POINT('Ctrl Pts',(-7.71983402500006,12.2,8.07598865399999));
#246148=CARTESIAN_POINT('Ctrl Pts',(-7.72290528400006,12.2,8.07735408899998));
#246149=CARTESIAN_POINT('Ctrl Pts',(-7.72598211700006,12.2,8.07871908399999));
#246150=CARTESIAN_POINT('Ctrl Pts',(-7.72906452200005,12.2,8.08008363199999));
#246151=CARTESIAN_POINT('Ctrl Pts',(-7.73215249300006,12.2,8.08144772299999));
#246152=CARTESIAN_POINT('Ctrl Pts',(-7.73524602400006,12.2,8.08281134799999));
#246153=CARTESIAN_POINT('Ctrl Pts',(-7.73834511100005,12.2,8.08417449699999));
#246154=CARTESIAN_POINT('Ctrl Pts',(-7.74144975100005,12.2,8.08553716199999));
#246155=CARTESIAN_POINT('Ctrl Pts',(-7.74455993600006,12.2,8.08689933299998));
#246156=CARTESIAN_POINT('Ctrl Pts',(-7.74767566300006,12.2,8.08826100099999));
#246157=CARTESIAN_POINT('Ctrl Pts',(-7.75079692700006,12.2,8.08962215699999));
#246158=CARTESIAN_POINT('Ctrl Pts',(-7.75392372200006,12.2,8.09098279099998));
#246159=CARTESIAN_POINT('Ctrl Pts',(-7.75705604400006,12.2,8.09234289499998));
#246160=CARTESIAN_POINT('Ctrl Pts',(-7.76019388900006,12.2,8.09370245899999));
#246161=CARTESIAN_POINT('Ctrl Pts',(-7.76333725000006,12.2,8.09506147499999));
#246162=CARTESIAN_POINT('Ctrl Pts',(-7.76648612500006,12.2,8.09641993199998));
#246163=CARTESIAN_POINT('Ctrl Pts',(-7.76964050600006,12.2,8.09777782399999));
#246164=CARTESIAN_POINT('Ctrl Pts',(-7.77280039100006,12.2,8.09913513899998));
#246165=CARTESIAN_POINT('Ctrl Pts',(-7.77596577300006,12.2,8.10049186899998));
#246166=CARTESIAN_POINT('Ctrl Pts',(-7.77913664800005,12.2,8.10184800599998));
#246167=CARTESIAN_POINT('Ctrl Pts',(-7.78231301200006,12.2,8.10320353899998));
#246168=CARTESIAN_POINT('Ctrl Pts',(-7.78549485900006,12.2,8.10455846299998));
#246169=CARTESIAN_POINT('Ctrl Pts',(-7.78868218500006,12.2,8.10591276399999));
#246170=CARTESIAN_POINT('Ctrl Pts',(-7.79187498300006,12.2,8.10726643599999));
#246171=CARTESIAN_POINT('Ctrl Pts',(-7.79507325100005,12.2,8.10861946999999));
#246172=CARTESIAN_POINT('Ctrl Pts',(-7.79827698300006,12.2,8.10997185699998));
#246173=CARTESIAN_POINT('Ctrl Pts',(-7.80148617400006,12.2,8.11132358799998));
#246174=CARTESIAN_POINT('Ctrl Pts',(-7.80470082000006,12.2,8.11267465299998));
#246175=CARTESIAN_POINT('Ctrl Pts',(-7.80792091500006,12.2,8.11402504599998));
#246176=CARTESIAN_POINT('Ctrl Pts',(-7.81114645400006,12.2,8.11537475499998));
#246177=CARTESIAN_POINT('Ctrl Pts',(-7.81437743500006,12.2,8.11672377399999));
#246178=CARTESIAN_POINT('Ctrl Pts',(-7.81761384900006,12.2,8.11807209299998));
#246179=CARTESIAN_POINT('Ctrl Pts',(-7.82085569500006,12.2,8.11941970299999));
#246180=CARTESIAN_POINT('Ctrl Pts',(-7.82410296500006,12.2,8.12076659599999));
#246181=CARTESIAN_POINT('Ctrl Pts',(-7.82735565600006,12.2,8.12211276299998));
#246182=CARTESIAN_POINT('Ctrl Pts',(-7.83061376200005,12.2,8.12345819399999));
#246183=CARTESIAN_POINT('Ctrl Pts',(-7.83387728100006,12.2,8.12480288399998));
#246184=CARTESIAN_POINT('Ctrl Pts',(-7.83714620400006,12.2,8.12614681999998));
#246185=CARTESIAN_POINT('Ctrl Pts',(-7.84042053000006,12.2,8.12748999699998));
#246186=CARTESIAN_POINT('Ctrl Pts',(-7.84370025300006,12.2,8.12883240399999));
#246187=CARTESIAN_POINT('Ctrl Pts',(-7.84698536600006,12.2,8.13017403499998));
#246188=CARTESIAN_POINT('Ctrl Pts',(-7.85027586700006,12.2,8.13151487799999));
#246189=CARTESIAN_POINT('Ctrl Pts',(-7.85357175000006,12.2,8.13285492699999));
#246190=CARTESIAN_POINT('Ctrl Pts',(-7.85687301000006,12.2,8.13419417299999));
#246191=CARTESIAN_POINT('Ctrl Pts',(-7.86017964300005,12.2,8.13553260699998));
#246192=CARTESIAN_POINT('Ctrl Pts',(-7.86349164400006,12.2,8.13687022099998));
#246193=CARTESIAN_POINT('Ctrl Pts',(-7.86680900800006,12.2,8.13820700699999));
#246194=CARTESIAN_POINT('Ctrl Pts',(-7.87013173000006,12.2,8.13954295599999));
#246195=CARTESIAN_POINT('Ctrl Pts',(-7.87345980500006,12.2,8.14087805999998));
#246196=CARTESIAN_POINT('Ctrl Pts',(-7.87679322900006,12.2,8.14221230999999));
#246197=CARTESIAN_POINT('Ctrl Pts',(-7.88013199700006,12.2,8.14354569699999));
#246198=CARTESIAN_POINT('Ctrl Pts',(-7.88347610400006,12.2,8.14487821399998));
#246199=CARTESIAN_POINT('Ctrl Pts',(-7.88682554500006,12.2,8.14620985299998));
#246200=CARTESIAN_POINT('Ctrl Pts',(-7.89018031600006,12.2,8.14754060399999));
#246201=CARTESIAN_POINT('Ctrl Pts',(-7.89354041200006,12.2,8.14887045999999));
#246202=CARTESIAN_POINT('Ctrl Pts',(-7.89690582700005,12.2,8.15019941199999));
#246203=CARTESIAN_POINT('Ctrl Pts',(-7.90027655700006,12.2,8.15152745299999));
#246204=CARTESIAN_POINT('Ctrl Pts',(-7.90365259800006,12.2,8.15285457299998));
#246205=CARTESIAN_POINT('Ctrl Pts',(-7.90703394500006,12.2,8.15418076499999));
#246206=CARTESIAN_POINT('Ctrl Pts',(-7.91042059300005,12.2,8.15550602099999));
#246207=CARTESIAN_POINT('Ctrl Pts',(-7.91381253600005,12.2,8.15683033199999));
#246208=CARTESIAN_POINT('Ctrl Pts',(-7.91720977000006,12.2,8.15815368899998));
#246209=CARTESIAN_POINT('Ctrl Pts',(-7.92061229100005,12.2,8.15947608599998));
#246210=CARTESIAN_POINT('Ctrl Pts',(-7.92402009400006,12.2,8.16079751399998));
#246211=CARTESIAN_POINT('Ctrl Pts',(-7.92743317500006,12.2,8.16211796399998));
#246212=CARTESIAN_POINT('Ctrl Pts',(-7.93085152700005,12.2,8.16343742899999));
#246213=CARTESIAN_POINT('Ctrl Pts',(-7.93427514700006,12.2,8.16475590099999));
#246214=CARTESIAN_POINT('Ctrl Pts',(-7.93770402900006,12.2,8.16607337199999));
#246215=CARTESIAN_POINT('Ctrl Pts',(-7.94113817000006,12.2,8.16738983299999));
#246216=CARTESIAN_POINT('Ctrl Pts',(-7.94457756400006,12.2,8.16870527599999));
#246217=CARTESIAN_POINT('Ctrl Pts',(-7.94802220600006,12.2,8.17001969299999));
#246218=CARTESIAN_POINT('Ctrl Pts',(-7.95147209200006,12.2,8.17133307699999));
#246219=CARTESIAN_POINT('Ctrl Pts',(-7.95492721600005,12.2,8.17264541999998));
#246220=CARTESIAN_POINT('Ctrl Pts',(-7.95838757500006,12.2,8.17395671299998));
#246221=CARTESIAN_POINT('Ctrl Pts',(-7.96185316300006,12.2,8.17526694799999));
#246222=CARTESIAN_POINT('Ctrl Pts',(-7.96532397700006,12.2,8.17657611899998));
#246223=CARTESIAN_POINT('Ctrl Pts',(-7.96880001000006,12.2,8.17788421699999));
#246224=CARTESIAN_POINT('Ctrl Pts',(-7.97228126000006,12.2,8.17919123499999));
#246225=CARTESIAN_POINT('Ctrl Pts',(-7.97576771900006,12.2,8.18049716399998));
#246226=CARTESIAN_POINT('Ctrl Pts',(-7.97925938500006,12.2,8.18180199599999));
#246227=CARTESIAN_POINT('Ctrl Pts',(-7.98275625000005,12.2,8.18310572199999));
#246228=CARTESIAN_POINT('Ctrl Pts',(-7.98625831300006,12.2,8.18440833599999));
#246229=CARTESIAN_POINT('Ctrl Pts',(-7.98976556600006,12.2,8.18570982799999));
#246230=CARTESIAN_POINT('Ctrl Pts',(-7.99327800400006,12.2,8.18701019299999));
#246231=CARTESIAN_POINT('Ctrl Pts',(-7.99679562600006,12.2,8.18830942099999));
#246232=CARTESIAN_POINT('Ctrl Pts',(-8.00031842500006,12.2,8.18960750499999));
#246233=CARTESIAN_POINT('Ctrl Pts',(-8.00384639600006,12.2,8.19090443999999));
#246234=CARTESIAN_POINT('Ctrl Pts',(-8.00737953700006,12.2,8.19220021799998));
#246235=CARTESIAN_POINT('Ctrl Pts',(-8.01091784300005,12.2,8.19349483199998));
#246236=CARTESIAN_POINT('Ctrl Pts',(-8.01446130800005,12.2,8.19478827199998));
#246237=CARTESIAN_POINT('Ctrl Pts',(-8.01800992700005,12.2,8.19608053199998));
#246238=CARTESIAN_POINT('Ctrl Pts',(-8.02156369500005,12.2,8.19737160199999));
#246239=CARTESIAN_POINT('Ctrl Pts',(-8.02512260400006,12.2,8.19866146999999));
#246240=CARTESIAN_POINT('Ctrl Pts',(-8.02868665100006,12.2,8.19995012899999));
#246241=CARTESIAN_POINT('Ctrl Pts',(-8.03225583000006,12.2,8.20123757099999));
#246242=CARTESIAN_POINT('Ctrl Pts',(-8.03583013500005,12.2,8.20252378799999));
#246243=CARTESIAN_POINT('Ctrl Pts',(-8.03940956400006,12.2,8.20380877499998));
#246244=CARTESIAN_POINT('Ctrl Pts',(-8.04299411600006,12.2,8.20509252899999));
#246245=CARTESIAN_POINT('Ctrl Pts',(-8.04658378800006,12.2,8.20637504799999));
#246246=CARTESIAN_POINT('Ctrl Pts',(-8.04945962200006,12.2,8.20740007499998));
#246247=CARTESIAN_POINT('Ctrl Pts',(-8.05161880100006,12.2,8.20816828899999));
#246248=CARTESIAN_POINT('Ctrl Pts',(-8.05305927800006,12.2,8.20868018399998));
#246249=CARTESIAN_POINT('Ctrl Pts',(-8.05377977200006,12.2,8.20893606999999));
#246250=CARTESIAN_POINT('Origin',(-5.66257110645729E-14,15.2,-1.77635683940025E-14));
#246251=CARTESIAN_POINT('',(-8.02901631900006,15.2,6.57080831899999));
#246252=CARTESIAN_POINT('',(-8.02901631900006,12.2,6.57080831899999));
#246253=CARTESIAN_POINT('',(-8.02901631900006,15.2,6.57080831899999));
#246254=CARTESIAN_POINT('Origin',(-5.66257110645729E-14,12.2,-1.77635683940025E-14));
#246255=CARTESIAN_POINT('Origin',(-5.66257110645729E-14,15.2,-1.77635683940025E-14));
#246256=CARTESIAN_POINT('Origin',(-5.66257110645729E-14,15.2,-1.77635683940025E-14));
#246257=CARTESIAN_POINT('',(-9.14005731500006,15.2,6.97920857099999));
#246258=CARTESIAN_POINT('',(-9.36775917500006,15.2,6.67046385499999));
#246259=CARTESIAN_POINT('Origin',(-5.66257110645729E-14,15.2,-1.77635683940025E-14));
#246260=CARTESIAN_POINT('',(-9.36775917500006,12.2,6.67046385499999));
#246261=CARTESIAN_POINT('',(-9.36775917500006,15.2,6.67046385499999));
#246262=CARTESIAN_POINT('',(-9.14005731500006,12.2,6.97920857099999));
#246263=CARTESIAN_POINT('Origin',(-5.66257110645729E-14,12.2,-1.77635683940025E-14));
#246264=CARTESIAN_POINT('',(-9.14005731500006,15.2,6.97920857099999));
#246265=CARTESIAN_POINT('Ctrl Pts',(-8.02901631900006,15.2,6.57080831899999));
#246266=CARTESIAN_POINT('Ctrl Pts',(-8.02901631900006,11.6,6.57080831899999));
#246267=CARTESIAN_POINT('Ctrl Pts',(-8.02916024200006,15.2,6.57090674099998));
#246268=CARTESIAN_POINT('Ctrl Pts',(-8.02916024200006,11.6,6.57090674099998));
#246269=CARTESIAN_POINT('Ctrl Pts',(-8.02945316300006,15.2,6.57110695199999));
#246270=CARTESIAN_POINT('Ctrl Pts',(-8.02945316300006,11.6,6.57110695199999));
#246271=CARTESIAN_POINT('Ctrl Pts',(-8.02989715800006,15.2,6.57141009799999));
#246272=CARTESIAN_POINT('Ctrl Pts',(-8.02989715800006,11.6,6.57141009799999));
#246273=CARTESIAN_POINT('Ctrl Pts',(-8.03049556400006,15.2,6.57181801999998));
#246274=CARTESIAN_POINT('Ctrl Pts',(-8.03049556400006,11.6,6.57181801999998));
#246275=CARTESIAN_POINT('Ctrl Pts',(-8.03125297400006,15.2,6.57233322399998));
#246276=CARTESIAN_POINT('Ctrl Pts',(-8.03125297400006,11.6,6.57233322399998));
#246277=CARTESIAN_POINT('Ctrl Pts',(-8.03202318500006,15.2,6.57285600599998));
#246278=CARTESIAN_POINT('Ctrl Pts',(-8.03202318500006,11.6,6.57285600599998));
#246279=CARTESIAN_POINT('Ctrl Pts',(-8.03280179800005,15.2,6.57338334999999));
#246280=CARTESIAN_POINT('Ctrl Pts',(-8.03280179800005,11.6,6.57338334999999));
#246281=CARTESIAN_POINT('Ctrl Pts',(-8.03358880000006,15.2,6.57391522699999));
#246282=CARTESIAN_POINT('Ctrl Pts',(-8.03358880000006,11.6,6.57391522699999));
#246283=CARTESIAN_POINT('Ctrl Pts',(-8.03438417900006,15.2,6.57445160599998));
#246284=CARTESIAN_POINT('Ctrl Pts',(-8.03438417900006,11.6,6.57445160599998));
#246285=CARTESIAN_POINT('Ctrl Pts',(-8.03518792400006,15.2,6.57499245799999));
#246286=CARTESIAN_POINT('Ctrl Pts',(-8.03518792400006,11.6,6.57499245799999));
#246287=CARTESIAN_POINT('Ctrl Pts',(-8.03600002200006,15.2,6.57553775199998));
#246288=CARTESIAN_POINT('Ctrl Pts',(-8.03600002200006,11.6,6.57553775199998));
#246289=CARTESIAN_POINT('Ctrl Pts',(-8.03682046100005,15.2,6.57608745999998));
#246290=CARTESIAN_POINT('Ctrl Pts',(-8.03682046100005,11.6,6.57608745999998));
#246291=CARTESIAN_POINT('Ctrl Pts',(-8.03764922900006,15.2,6.57664155099998));
#246292=CARTESIAN_POINT('Ctrl Pts',(-8.03764922900006,11.6,6.57664155099998));
#246293=CARTESIAN_POINT('Ctrl Pts',(-8.03848631400006,15.2,6.57719999799999));
#246294=CARTESIAN_POINT('Ctrl Pts',(-8.03848631400006,11.6,6.57719999799999));
#246295=CARTESIAN_POINT('Ctrl Pts',(-8.03933170600006,15.2,6.57776276899998));
#246296=CARTESIAN_POINT('Ctrl Pts',(-8.03933170600006,11.6,6.57776276899998));
#246297=CARTESIAN_POINT('Ctrl Pts',(-8.04018539100005,15.2,6.57832983699999));
#246298=CARTESIAN_POINT('Ctrl Pts',(-8.04018539100005,11.6,6.57832983699999));
#246299=CARTESIAN_POINT('Ctrl Pts',(-8.04104735700006,15.2,6.57890117299999));
#246300=CARTESIAN_POINT('Ctrl Pts',(-8.04104735700006,11.6,6.57890117299999));
#246301=CARTESIAN_POINT('Ctrl Pts',(-8.04191759500006,15.2,6.57947674699999));
#246302=CARTESIAN_POINT('Ctrl Pts',(-8.04191759500006,11.6,6.57947674699999));
#246303=CARTESIAN_POINT('Ctrl Pts',(-8.04279609000006,15.2,6.58005653299998));
#246304=CARTESIAN_POINT('Ctrl Pts',(-8.04279609000006,11.6,6.58005653299998));
#246305=CARTESIAN_POINT('Ctrl Pts',(-8.04368283300006,15.2,6.58064049899998));
#246306=CARTESIAN_POINT('Ctrl Pts',(-8.04368283300006,11.6,6.58064049899998));
#246307=CARTESIAN_POINT('Ctrl Pts',(-8.04457781100006,15.2,6.58122862099999));
#246308=CARTESIAN_POINT('Ctrl Pts',(-8.04457781100006,11.6,6.58122862099999));
#246309=CARTESIAN_POINT('Ctrl Pts',(-8.04548101300006,15.2,6.58182086699998));
#246310=CARTESIAN_POINT('Ctrl Pts',(-8.04548101300006,11.6,6.58182086699998));
#246311=CARTESIAN_POINT('Ctrl Pts',(-8.04639242800006,15.2,6.58241721199998));
#246312=CARTESIAN_POINT('Ctrl Pts',(-8.04639242800006,11.6,6.58241721199998));
#246313=CARTESIAN_POINT('Ctrl Pts',(-8.04731204200005,15.2,6.58301762599999));
#246314=CARTESIAN_POINT('Ctrl Pts',(-8.04731204200005,11.6,6.58301762599999));
#246315=CARTESIAN_POINT('Ctrl Pts',(-8.04823984700005,15.2,6.58362208299998));
#246316=CARTESIAN_POINT('Ctrl Pts',(-8.04823984700005,11.6,6.58362208299998));
#246317=CARTESIAN_POINT('Ctrl Pts',(-8.04917582900006,15.2,6.58423055499998));
#246318=CARTESIAN_POINT('Ctrl Pts',(-8.04917582900006,11.6,6.58423055499998));
#246319=CARTESIAN_POINT('Ctrl Pts',(-8.05011997800005,15.2,6.58484301199999));
#246320=CARTESIAN_POINT('Ctrl Pts',(-8.05011997800005,11.6,6.58484301199999));
#246321=CARTESIAN_POINT('Ctrl Pts',(-8.05107228300006,15.2,6.58545943199999));
#246322=CARTESIAN_POINT('Ctrl Pts',(-8.05107228300006,11.6,6.58545943199999));
#246323=CARTESIAN_POINT('Ctrl Pts',(-8.05203273200006,15.2,6.58607978299998));
#246324=CARTESIAN_POINT('Ctrl Pts',(-8.05203273200006,11.6,6.58607978299998));
#246325=CARTESIAN_POINT('Ctrl Pts',(-8.05300131400006,15.2,6.58670403999999));
#246326=CARTESIAN_POINT('Ctrl Pts',(-8.05300131400006,11.6,6.58670403999999));
#246327=CARTESIAN_POINT('Ctrl Pts',(-8.05397801800006,15.2,6.58733217599998));
#246328=CARTESIAN_POINT('Ctrl Pts',(-8.05397801800006,11.6,6.58733217599998));
#246329=CARTESIAN_POINT('Ctrl Pts',(-8.05496283200006,15.2,6.58796416399999));
#246330=CARTESIAN_POINT('Ctrl Pts',(-8.05496283200006,11.6,6.58796416399999));
#246331=CARTESIAN_POINT('Ctrl Pts',(-8.05595574600006,15.2,6.58859997699999));
#246332=CARTESIAN_POINT('Ctrl Pts',(-8.05595574600006,11.6,6.58859997699999));
#246333=CARTESIAN_POINT('Ctrl Pts',(-8.05695674700006,15.2,6.58923959099998));
#246334=CARTESIAN_POINT('Ctrl Pts',(-8.05695674700006,11.6,6.58923959099998));
#246335=CARTESIAN_POINT('Ctrl Pts',(-8.05796582700006,15.2,6.58988297599999));
#246336=CARTESIAN_POINT('Ctrl Pts',(-8.05796582700006,11.6,6.58988297599999));
#246337=CARTESIAN_POINT('Ctrl Pts',(-8.05898297300006,15.2,6.59053010699999));
#246338=CARTESIAN_POINT('Ctrl Pts',(-8.05898297300006,11.6,6.59053010699999));
#246339=CARTESIAN_POINT('Ctrl Pts',(-8.06000817500006,15.2,6.59118095899998));
#246340=CARTESIAN_POINT('Ctrl Pts',(-8.06000817500006,11.6,6.59118095899998));
#246341=CARTESIAN_POINT('Ctrl Pts',(-8.06104142100006,15.2,6.59183550499999));
#246342=CARTESIAN_POINT('Ctrl Pts',(-8.06104142100006,11.6,6.59183550499999));
#246343=CARTESIAN_POINT('Ctrl Pts',(-8.06208270100005,15.2,6.59249371899998));
#246344=CARTESIAN_POINT('Ctrl Pts',(-8.06208270100005,11.6,6.59249371899998));
#246345=CARTESIAN_POINT('Ctrl Pts',(-8.06313200300006,15.2,6.59315557599999));
#246346=CARTESIAN_POINT('Ctrl Pts',(-8.06313200300006,11.6,6.59315557599999));
#246347=CARTESIAN_POINT('Ctrl Pts',(-8.06418931900006,15.2,6.59382104899999));
#246348=CARTESIAN_POINT('Ctrl Pts',(-8.06418931900006,11.6,6.59382104899999));
#246349=CARTESIAN_POINT('Ctrl Pts',(-8.06525463500006,15.2,6.59449011399998));
#246350=CARTESIAN_POINT('Ctrl Pts',(-8.06525463500006,11.6,6.59449011399998));
#246351=CARTESIAN_POINT('Ctrl Pts',(-8.06632794200006,15.2,6.59516274499998));
#246352=CARTESIAN_POINT('Ctrl Pts',(-8.06632794200006,11.6,6.59516274499998));
#246353=CARTESIAN_POINT('Ctrl Pts',(-8.06740922800006,15.2,6.59583891799999));
#246354=CARTESIAN_POINT('Ctrl Pts',(-8.06740922800006,11.6,6.59583891799999));
#246355=CARTESIAN_POINT('Ctrl Pts',(-8.06849848300006,15.2,6.59651860499999));
#246356=CARTESIAN_POINT('Ctrl Pts',(-8.06849848300006,11.6,6.59651860499999));
#246357=CARTESIAN_POINT('Ctrl Pts',(-8.06959569800006,15.2,6.59720178299998));
#246358=CARTESIAN_POINT('Ctrl Pts',(-8.06959569800006,11.6,6.59720178299998));
#246359=CARTESIAN_POINT('Ctrl Pts',(-8.07070086000006,15.2,6.59788842599998));
#246360=CARTESIAN_POINT('Ctrl Pts',(-8.07070086000006,11.6,6.59788842599998));
#246361=CARTESIAN_POINT('Ctrl Pts',(-8.07181396000006,15.2,6.59857850899999));
#246362=CARTESIAN_POINT('Ctrl Pts',(-8.07181396000006,11.6,6.59857850899999));
#246363=CARTESIAN_POINT('Ctrl Pts',(-8.07293498600006,15.2,6.59927200999999));
#246364=CARTESIAN_POINT('Ctrl Pts',(-8.07293498600006,11.6,6.59927200999999));
#246365=CARTESIAN_POINT('Ctrl Pts',(-8.07406393000005,15.2,6.59996890099999));
#246366=CARTESIAN_POINT('Ctrl Pts',(-8.07406393000005,11.6,6.59996890099999));
#246367=CARTESIAN_POINT('Ctrl Pts',(-8.07520077900006,15.2,6.60066915999998));
#246368=CARTESIAN_POINT('Ctrl Pts',(-8.07520077900006,11.6,6.60066915999998));
#246369=CARTESIAN_POINT('Ctrl Pts',(-8.07634552300006,15.2,6.60137276099999));
#246370=CARTESIAN_POINT('Ctrl Pts',(-8.07634552300006,11.6,6.60137276099999));
#246371=CARTESIAN_POINT('Ctrl Pts',(-8.07749815200006,15.2,6.60207967899999));
#246372=CARTESIAN_POINT('Ctrl Pts',(-8.07749815200006,11.6,6.60207967899999));
#246373=CARTESIAN_POINT('Ctrl Pts',(-8.07865865700006,15.2,6.60278989299999));
#246374=CARTESIAN_POINT('Ctrl Pts',(-8.07865865700006,11.6,6.60278989299999));
#246375=CARTESIAN_POINT('Ctrl Pts',(-8.07982702600006,15.2,6.60350337599999));
#246376=CARTESIAN_POINT('Ctrl Pts',(-8.07982702600006,11.6,6.60350337599999));
#246377=CARTESIAN_POINT('Ctrl Pts',(-8.08100324800006,15.2,6.60422010599999));
#246378=CARTESIAN_POINT('Ctrl Pts',(-8.08100324800006,11.6,6.60422010599999));
#246379=CARTESIAN_POINT('Ctrl Pts',(-8.08218731400006,15.2,6.60494005799999));
#246380=CARTESIAN_POINT('Ctrl Pts',(-8.08218731400006,11.6,6.60494005799999));
#246381=CARTESIAN_POINT('Ctrl Pts',(-8.08337921500006,15.2,6.60566320799998));
#246382=CARTESIAN_POINT('Ctrl Pts',(-8.08337921500006,11.6,6.60566320799998));
#246383=CARTESIAN_POINT('Ctrl Pts',(-8.08457893900006,15.2,6.60638953299999));
#246384=CARTESIAN_POINT('Ctrl Pts',(-8.08457893900006,11.6,6.60638953299999));
#246385=CARTESIAN_POINT('Ctrl Pts',(-8.08578647500006,15.2,6.60711900999999));
#246386=CARTESIAN_POINT('Ctrl Pts',(-8.08578647500006,11.6,6.60711900999999));
#246387=CARTESIAN_POINT('Ctrl Pts',(-8.08700181600006,15.2,6.60785161499999));
#246388=CARTESIAN_POINT('Ctrl Pts',(-8.08700181600006,11.6,6.60785161499999));
#246389=CARTESIAN_POINT('Ctrl Pts',(-8.08822494800006,15.2,6.60858732499998));
#246390=CARTESIAN_POINT('Ctrl Pts',(-8.08822494800006,11.6,6.60858732499998));
#246391=CARTESIAN_POINT('Ctrl Pts',(-8.08945586400006,15.2,6.60932611599998));
#246392=CARTESIAN_POINT('Ctrl Pts',(-8.08945586400006,11.6,6.60932611599998));
#246393=CARTESIAN_POINT('Ctrl Pts',(-8.09069455200006,15.2,6.61006796499999));
#246394=CARTESIAN_POINT('Ctrl Pts',(-8.09069455200006,11.6,6.61006796499999));
#246395=CARTESIAN_POINT('Ctrl Pts',(-8.09194100400006,15.2,6.61081285099999));
#246396=CARTESIAN_POINT('Ctrl Pts',(-8.09194100400006,11.6,6.61081285099999));
#246397=CARTESIAN_POINT('Ctrl Pts',(-8.09319520700006,15.2,6.61156074899999));
#246398=CARTESIAN_POINT('Ctrl Pts',(-8.09319520700006,11.6,6.61156074899999));
#246399=CARTESIAN_POINT('Ctrl Pts',(-8.09445715400006,15.2,6.61231163599999));
#246400=CARTESIAN_POINT('Ctrl Pts',(-8.09445715400006,11.6,6.61231163599999));
#246401=CARTESIAN_POINT('Ctrl Pts',(-8.09572683400006,15.2,6.61306549099999));
#246402=CARTESIAN_POINT('Ctrl Pts',(-8.09572683400006,11.6,6.61306549099999));
#246403=CARTESIAN_POINT('Ctrl Pts',(-8.09700423700006,15.2,6.61382228999998));
#246404=CARTESIAN_POINT('Ctrl Pts',(-8.09700423700006,11.6,6.61382228999998));
#246405=CARTESIAN_POINT('Ctrl Pts',(-8.09828935300006,15.2,6.61458201099999));
#246406=CARTESIAN_POINT('Ctrl Pts',(-8.09828935300006,11.6,6.61458201099999));
#246407=CARTESIAN_POINT('Ctrl Pts',(-8.09958217100006,15.2,6.61534463099999));
#246408=CARTESIAN_POINT('Ctrl Pts',(-8.09958217100006,11.6,6.61534463099999));
#246409=CARTESIAN_POINT('Ctrl Pts',(-8.10088268300006,15.2,6.61611012799998));
#246410=CARTESIAN_POINT('Ctrl Pts',(-8.10088268300006,11.6,6.61611012799998));
#246411=CARTESIAN_POINT('Ctrl Pts',(-8.10219087900006,15.2,6.61687848099999));
#246412=CARTESIAN_POINT('Ctrl Pts',(-8.10219087900006,11.6,6.61687848099999));
#246413=CARTESIAN_POINT('Ctrl Pts',(-8.10350674900005,15.2,6.61764966799999));
#246414=CARTESIAN_POINT('Ctrl Pts',(-8.10350674900005,11.6,6.61764966799999));
#246415=CARTESIAN_POINT('Ctrl Pts',(-8.10483028300006,15.2,6.61842366399998));
#246416=CARTESIAN_POINT('Ctrl Pts',(-8.10483028300006,11.6,6.61842366399998));
#246417=CARTESIAN_POINT('Ctrl Pts',(-8.10616147100006,15.2,6.61920044899999));
#246418=CARTESIAN_POINT('Ctrl Pts',(-8.10616147100006,11.6,6.61920044899999));
#246419=CARTESIAN_POINT('Ctrl Pts',(-8.10750030400006,15.2,6.61998000199999));
#246420=CARTESIAN_POINT('Ctrl Pts',(-8.10750030400006,11.6,6.61998000199999));
#246421=CARTESIAN_POINT('Ctrl Pts',(-8.10884677200006,15.2,6.62076229999998));
#246422=CARTESIAN_POINT('Ctrl Pts',(-8.10884677200006,11.6,6.62076229999998));
#246423=CARTESIAN_POINT('Ctrl Pts',(-8.11020086500006,15.2,6.62154732099999));
#246424=CARTESIAN_POINT('Ctrl Pts',(-8.11020086500006,11.6,6.62154732099999));
#246425=CARTESIAN_POINT('Ctrl Pts',(-8.11156257400006,15.2,6.62233504499999));
#246426=CARTESIAN_POINT('Ctrl Pts',(-8.11156257400006,11.6,6.62233504499999));
#246427=CARTESIAN_POINT('Ctrl Pts',(-8.11293189000006,15.2,6.62312544999998));
#246428=CARTESIAN_POINT('Ctrl Pts',(-8.11293189000006,11.6,6.62312544999998));
#246429=CARTESIAN_POINT('Ctrl Pts',(-8.11430880100006,15.2,6.62391851299999));
#246430=CARTESIAN_POINT('Ctrl Pts',(-8.11430880100006,11.6,6.62391851299999));
#246431=CARTESIAN_POINT('Ctrl Pts',(-8.11569330000006,15.2,6.62471421499998));
#246432=CARTESIAN_POINT('Ctrl Pts',(-8.11569330000006,11.6,6.62471421499998));
#246433=CARTESIAN_POINT('Ctrl Pts',(-8.11708537600006,15.2,6.62551253399998));
#246434=CARTESIAN_POINT('Ctrl Pts',(-8.11708537600006,11.6,6.62551253399998));
#246435=CARTESIAN_POINT('Ctrl Pts',(-8.11848502100006,15.2,6.62631344799999));
#246436=CARTESIAN_POINT('Ctrl Pts',(-8.11848502100006,11.6,6.62631344799999));
#246437=CARTESIAN_POINT('Ctrl Pts',(-8.11989222400006,15.2,6.62711693599999));
#246438=CARTESIAN_POINT('Ctrl Pts',(-8.11989222400006,11.6,6.62711693599999));
#246439=CARTESIAN_POINT('Ctrl Pts',(-8.12130697600006,15.2,6.62792297899998));
#246440=CARTESIAN_POINT('Ctrl Pts',(-8.12130697600006,11.6,6.62792297899998));
#246441=CARTESIAN_POINT('Ctrl Pts',(-8.12272926800006,15.2,6.62873155499998));
#246442=CARTESIAN_POINT('Ctrl Pts',(-8.12272926800006,11.6,6.62873155499998));
#246443=CARTESIAN_POINT('Ctrl Pts',(-8.12415909100006,15.2,6.62954264199998));
#246444=CARTESIAN_POINT('Ctrl Pts',(-8.12415909100006,11.6,6.62954264199998));
#246445=CARTESIAN_POINT('Ctrl Pts',(-8.12559643300006,15.2,6.63035622099999));
#246446=CARTESIAN_POINT('Ctrl Pts',(-8.12559643300006,11.6,6.63035622099999));
#246447=CARTESIAN_POINT('Ctrl Pts',(-8.12704128900006,15.2,6.63117227099999));
#246448=CARTESIAN_POINT('Ctrl Pts',(-8.12704128900006,11.6,6.63117227099999));
#246449=CARTESIAN_POINT('Ctrl Pts',(-8.12849364700006,15.2,6.63199077099998));
#246450=CARTESIAN_POINT('Ctrl Pts',(-8.12849364700006,11.6,6.63199077099998));
#246451=CARTESIAN_POINT('Ctrl Pts',(-8.12995349700006,15.2,6.63281169999999));
#246452=CARTESIAN_POINT('Ctrl Pts',(-8.12995349700006,11.6,6.63281169999999));
#246453=CARTESIAN_POINT('Ctrl Pts',(-8.13142083200006,15.2,6.63363503899999));
#246454=CARTESIAN_POINT('Ctrl Pts',(-8.13142083200006,11.6,6.63363503899999));
#246455=CARTESIAN_POINT('Ctrl Pts',(-8.13289564100005,15.2,6.63446076699999));
#246456=CARTESIAN_POINT('Ctrl Pts',(-8.13289564100005,11.6,6.63446076699999));
#246457=CARTESIAN_POINT('Ctrl Pts',(-8.13437791500006,15.2,6.63528886499999));
#246458=CARTESIAN_POINT('Ctrl Pts',(-8.13437791500006,11.6,6.63528886499999));
#246459=CARTESIAN_POINT('Ctrl Pts',(-8.13586764600006,15.2,6.63611931099998));
#246460=CARTESIAN_POINT('Ctrl Pts',(-8.13586764600006,11.6,6.63611931099998));
#246461=CARTESIAN_POINT('Ctrl Pts',(-8.13736482400006,15.2,6.63695208599999));
#246462=CARTESIAN_POINT('Ctrl Pts',(-8.13736482400006,11.6,6.63695208599999));
#246463=CARTESIAN_POINT('Ctrl Pts',(-8.13886943900006,15.2,6.63778716999998));
#246464=CARTESIAN_POINT('Ctrl Pts',(-8.13886943900006,11.6,6.63778716999998));
#246465=CARTESIAN_POINT('Ctrl Pts',(-8.14038148300006,15.2,6.63862454399998));
#246466=CARTESIAN_POINT('Ctrl Pts',(-8.14038148300006,11.6,6.63862454399998));
#246467=CARTESIAN_POINT('Ctrl Pts',(-8.14190094800006,15.2,6.63946418699998));
#246468=CARTESIAN_POINT('Ctrl Pts',(-8.14190094800006,11.6,6.63946418699998));
#246469=CARTESIAN_POINT('Ctrl Pts',(-8.14342782200006,15.2,6.64030607899999));
#246470=CARTESIAN_POINT('Ctrl Pts',(-8.14342782200006,11.6,6.64030607899999));
#246471=CARTESIAN_POINT('Ctrl Pts',(-8.14496209800006,15.2,6.64115020099998));
#246472=CARTESIAN_POINT('Ctrl Pts',(-8.14496209800006,11.6,6.64115020099998));
#246473=CARTESIAN_POINT('Ctrl Pts',(-8.14650376600006,15.2,6.64199653299999));
#246474=CARTESIAN_POINT('Ctrl Pts',(-8.14650376600006,11.6,6.64199653299999));
#246475=CARTESIAN_POINT('Ctrl Pts',(-8.14805281800006,15.2,6.64284505699998));
#246476=CARTESIAN_POINT('Ctrl Pts',(-8.14805281800006,11.6,6.64284505699998));
#246477=CARTESIAN_POINT('Ctrl Pts',(-8.14960924300006,15.2,6.64369575199999));
#246478=CARTESIAN_POINT('Ctrl Pts',(-8.14960924300006,11.6,6.64369575199999));
#246479=CARTESIAN_POINT('Ctrl Pts',(-8.15117303600006,15.2,6.64454859999999));
#246480=CARTESIAN_POINT('Ctrl Pts',(-8.15117303600006,11.6,6.64454859999999));
#246481=CARTESIAN_POINT('Ctrl Pts',(-8.15274418400006,15.2,6.64540357999999));
#246482=CARTESIAN_POINT('Ctrl Pts',(-8.15274418400006,11.6,6.64540357999999));
#246483=CARTESIAN_POINT('Ctrl Pts',(-8.15432267900006,15.2,6.64626067399999));
#246484=CARTESIAN_POINT('Ctrl Pts',(-8.15432267900006,11.6,6.64626067399999));
#246485=CARTESIAN_POINT('Ctrl Pts',(-8.15590851400006,15.2,6.64711986299999));
#246486=CARTESIAN_POINT('Ctrl Pts',(-8.15590851400006,11.6,6.64711986299999));
#246487=CARTESIAN_POINT('Ctrl Pts',(-8.15750167800006,15.2,6.64798112699999));
#246488=CARTESIAN_POINT('Ctrl Pts',(-8.15750167800006,11.6,6.64798112699999));
#246489=CARTESIAN_POINT('Ctrl Pts',(-8.15910216400006,15.2,6.64884444899998));
#246490=CARTESIAN_POINT('Ctrl Pts',(-8.15910216400006,11.6,6.64884444899998));
#246491=CARTESIAN_POINT('Ctrl Pts',(-8.16070996000006,15.2,6.64970980799998));
#246492=CARTESIAN_POINT('Ctrl Pts',(-8.16070996000006,11.6,6.64970980799998));
#246493=CARTESIAN_POINT('Ctrl Pts',(-8.16232506100006,15.2,6.65057718599999));
#246494=CARTESIAN_POINT('Ctrl Pts',(-8.16232506100006,11.6,6.65057718599999));
#246495=CARTESIAN_POINT('Ctrl Pts',(-8.16394745600006,15.2,6.65144656499999));
#246496=CARTESIAN_POINT('Ctrl Pts',(-8.16394745600006,11.6,6.65144656499999));
#246497=CARTESIAN_POINT('Ctrl Pts',(-8.16557713600006,15.2,6.65231792599998));
#246498=CARTESIAN_POINT('Ctrl Pts',(-8.16557713600006,11.6,6.65231792599998));
#246499=CARTESIAN_POINT('Ctrl Pts',(-8.16721409300006,15.2,6.65319124899998));
#246500=CARTESIAN_POINT('Ctrl Pts',(-8.16721409300006,11.6,6.65319124899998));
#246501=CARTESIAN_POINT('Ctrl Pts',(-8.16885831800005,15.2,6.65406651699998));
#246502=CARTESIAN_POINT('Ctrl Pts',(-8.16885831800005,11.6,6.65406651699998));
#246503=CARTESIAN_POINT('Ctrl Pts',(-8.17050980300005,15.2,6.65494371199999));
#246504=CARTESIAN_POINT('Ctrl Pts',(-8.17050980300005,11.6,6.65494371199999));
#246505=CARTESIAN_POINT('Ctrl Pts',(-8.17216853900005,15.2,6.65582281399999));
#246506=CARTESIAN_POINT('Ctrl Pts',(-8.17216853900005,11.6,6.65582281399999));
#246507=CARTESIAN_POINT('Ctrl Pts',(-8.17383451600006,15.2,6.65670380499999));
#246508=CARTESIAN_POINT('Ctrl Pts',(-8.17383451600006,11.6,6.65670380499999));
#246509=CARTESIAN_POINT('Ctrl Pts',(-8.17550772700006,15.2,6.65758666799999));
#246510=CARTESIAN_POINT('Ctrl Pts',(-8.17550772700006,11.6,6.65758666799999));
#246511=CARTESIAN_POINT('Ctrl Pts',(-8.17718816300006,15.2,6.65847138399998));
#246512=CARTESIAN_POINT('Ctrl Pts',(-8.17718816300006,11.6,6.65847138399998));
#246513=CARTESIAN_POINT('Ctrl Pts',(-8.17887581500005,15.2,6.65935793499998));
#246514=CARTESIAN_POINT('Ctrl Pts',(-8.17887581500005,11.6,6.65935793499998));
#246515=CARTESIAN_POINT('Ctrl Pts',(-8.18057067400006,15.2,6.66024630299999));
#246516=CARTESIAN_POINT('Ctrl Pts',(-8.18057067400006,11.6,6.66024630299999));
#246517=CARTESIAN_POINT('Ctrl Pts',(-8.18227273200005,15.2,6.66113646999998));
#246518=CARTESIAN_POINT('Ctrl Pts',(-8.18227273200005,11.6,6.66113646999998));
#246519=CARTESIAN_POINT('Ctrl Pts',(-8.18398198000006,15.2,6.66202841799999));
#246520=CARTESIAN_POINT('Ctrl Pts',(-8.18398198000006,11.6,6.66202841799999));
#246521=CARTESIAN_POINT('Ctrl Pts',(-8.18569841000006,15.2,6.66292212999998));
#246522=CARTESIAN_POINT('Ctrl Pts',(-8.18569841000006,11.6,6.66292212999998));
#246523=CARTESIAN_POINT('Ctrl Pts',(-8.18742201200006,15.2,6.66381758699998));
#246524=CARTESIAN_POINT('Ctrl Pts',(-8.18742201200006,11.6,6.66381758699998));
#246525=CARTESIAN_POINT('Ctrl Pts',(-8.18915278100006,15.2,6.66471477199998));
#246526=CARTESIAN_POINT('Ctrl Pts',(-8.18915278100006,11.6,6.66471477199998));
#246527=CARTESIAN_POINT('Ctrl Pts',(-8.19089070500005,15.2,6.66561366699998));
#246528=CARTESIAN_POINT('Ctrl Pts',(-8.19089070500005,11.6,6.66561366699998));
#246529=CARTESIAN_POINT('Ctrl Pts',(-8.19263577500006,15.2,6.66651425499998));
#246530=CARTESIAN_POINT('Ctrl Pts',(-8.19263577500006,11.6,6.66651425499998));
#246531=CARTESIAN_POINT('Ctrl Pts',(-8.19438798700006,15.2,6.66741651699999));
#246532=CARTESIAN_POINT('Ctrl Pts',(-8.19438798700006,11.6,6.66741651699999));
#246533=CARTESIAN_POINT('Ctrl Pts',(-8.19614732800006,15.2,6.66832043799998));
#246534=CARTESIAN_POINT('Ctrl Pts',(-8.19614732800006,11.6,6.66832043799998));
#246535=CARTESIAN_POINT('Ctrl Pts',(-8.19791379200005,15.2,6.66922599899999));
#246536=CARTESIAN_POINT('Ctrl Pts',(-8.19791379200005,11.6,6.66922599899999));
#246537=CARTESIAN_POINT('Ctrl Pts',(-8.19968736900006,15.2,6.67013318399999));
#246538=CARTESIAN_POINT('Ctrl Pts',(-8.19968736900006,11.6,6.67013318399999));
#246539=CARTESIAN_POINT('Ctrl Pts',(-8.20146805300006,15.2,6.67104197399999));
#246540=CARTESIAN_POINT('Ctrl Pts',(-8.20146805300006,11.6,6.67104197399999));
#246541=CARTESIAN_POINT('Ctrl Pts',(-8.20325583300006,15.2,6.67195235199999));
#246542=CARTESIAN_POINT('Ctrl Pts',(-8.20325583300006,11.6,6.67195235199999));
#246543=CARTESIAN_POINT('Ctrl Pts',(-8.20505070200005,15.2,6.67286430199999));
#246544=CARTESIAN_POINT('Ctrl Pts',(-8.20505070200005,11.6,6.67286430199999));
#246545=CARTESIAN_POINT('Ctrl Pts',(-8.20685265200006,15.2,6.67377780699999));
#246546=CARTESIAN_POINT('Ctrl Pts',(-8.20685265200006,11.6,6.67377780699999));
#246547=CARTESIAN_POINT('Ctrl Pts',(-8.20866167300006,15.2,6.67469284899998));
#246548=CARTESIAN_POINT('Ctrl Pts',(-8.20866167300006,11.6,6.67469284899998));
#246549=CARTESIAN_POINT('Ctrl Pts',(-8.21047775900006,15.2,6.67560941199999));
#246550=CARTESIAN_POINT('Ctrl Pts',(-8.21047775900006,11.6,6.67560941199999));
#246551=CARTESIAN_POINT('Ctrl Pts',(-8.21230090000006,15.2,6.67652747899999));
#246552=CARTESIAN_POINT('Ctrl Pts',(-8.21230090000006,11.6,6.67652747899999));
#246553=CARTESIAN_POINT('Ctrl Pts',(-8.21413108800006,15.2,6.67744703199999));
#246554=CARTESIAN_POINT('Ctrl Pts',(-8.21413108800006,11.6,6.67744703199999));
#246555=CARTESIAN_POINT('Ctrl Pts',(-8.21596831500005,15.2,6.67836805599999));
#246556=CARTESIAN_POINT('Ctrl Pts',(-8.21596831500005,11.6,6.67836805599999));
#246557=CARTESIAN_POINT('Ctrl Pts',(-8.21781257400006,15.2,6.67929053299999));
#246558=CARTESIAN_POINT('Ctrl Pts',(-8.21781257400006,11.6,6.67929053299999));
#246559=CARTESIAN_POINT('Ctrl Pts',(-8.21966385400006,15.2,6.68021444699999));
#246560=CARTESIAN_POINT('Ctrl Pts',(-8.21966385400006,11.6,6.68021444699999));
#246561=CARTESIAN_POINT('Ctrl Pts',(-8.22152214900006,15.2,6.68113978099999));
#246562=CARTESIAN_POINT('Ctrl Pts',(-8.22152214900006,11.6,6.68113978099999));
#246563=CARTESIAN_POINT('Ctrl Pts',(-8.22338745000006,15.2,6.68206651899999));
#246564=CARTESIAN_POINT('Ctrl Pts',(-8.22338745000006,11.6,6.68206651899999));
#246565=CARTESIAN_POINT('Ctrl Pts',(-8.22525974800006,15.2,6.68299464499999));
#246566=CARTESIAN_POINT('Ctrl Pts',(-8.22525974800006,11.6,6.68299464499999));
#246567=CARTESIAN_POINT('Ctrl Pts',(-8.22713903600006,15.2,6.68392414099999));
#246568=CARTESIAN_POINT('Ctrl Pts',(-8.22713903600006,11.6,6.68392414099999));
#246569=CARTESIAN_POINT('Ctrl Pts',(-8.22902530700006,15.2,6.68485499099998));
#246570=CARTESIAN_POINT('Ctrl Pts',(-8.22902530700006,11.6,6.68485499099998));
#246571=CARTESIAN_POINT('Ctrl Pts',(-8.23091855000006,15.2,6.68578718099998));
#246572=CARTESIAN_POINT('Ctrl Pts',(-8.23091855000006,11.6,6.68578718099998));
#246573=CARTESIAN_POINT('Ctrl Pts',(-8.23281876000006,15.2,6.68672069299999));
#246574=CARTESIAN_POINT('Ctrl Pts',(-8.23281876000006,11.6,6.68672069299999));
#246575=CARTESIAN_POINT('Ctrl Pts',(-8.23472592500006,15.2,6.68765550999999));
#246576=CARTESIAN_POINT('Ctrl Pts',(-8.23472592500006,11.6,6.68765550999999));
#246577=CARTESIAN_POINT('Ctrl Pts',(-8.23664004100005,15.2,6.68859161699999));
#246578=CARTESIAN_POINT('Ctrl Pts',(-8.23664004100005,11.6,6.68859161699999));
#246579=CARTESIAN_POINT('Ctrl Pts',(-8.23856109700005,15.2,6.68952899899999));
#246580=CARTESIAN_POINT('Ctrl Pts',(-8.23856109700005,11.6,6.68952899899999));
#246581=CARTESIAN_POINT('Ctrl Pts',(-8.24048908700006,15.2,6.69046763799999));
#246582=CARTESIAN_POINT('Ctrl Pts',(-8.24048908700006,11.6,6.69046763799999));
#246583=CARTESIAN_POINT('Ctrl Pts',(-8.24242400200006,15.2,6.69140751899998));
#246584=CARTESIAN_POINT('Ctrl Pts',(-8.24242400200006,11.6,6.69140751899998));
#246585=CARTESIAN_POINT('Ctrl Pts',(-8.24436583300006,15.2,6.69234862599998));
#246586=CARTESIAN_POINT('Ctrl Pts',(-8.24436583300006,11.6,6.69234862599998));
#246587=CARTESIAN_POINT('Ctrl Pts',(-8.24631457400006,15.2,6.69329094299999));
#246588=CARTESIAN_POINT('Ctrl Pts',(-8.24631457400006,11.6,6.69329094299999));
#246589=CARTESIAN_POINT('Ctrl Pts',(-8.24827021500005,15.2,6.69423445399998));
#246590=CARTESIAN_POINT('Ctrl Pts',(-8.24827021500005,11.6,6.69423445399998));
#246591=CARTESIAN_POINT('Ctrl Pts',(-8.25023275000006,15.2,6.69517914499998));
#246592=CARTESIAN_POINT('Ctrl Pts',(-8.25023275000006,11.6,6.69517914499998));
#246593=CARTESIAN_POINT('Ctrl Pts',(-8.25220216900006,15.2,6.69612499799998));
#246594=CARTESIAN_POINT('Ctrl Pts',(-8.25220216900006,11.6,6.69612499799998));
#246595=CARTESIAN_POINT('Ctrl Pts',(-8.25417846600006,15.2,6.69707199899998));
#246596=CARTESIAN_POINT('Ctrl Pts',(-8.25417846600006,11.6,6.69707199899998));
#246597=CARTESIAN_POINT('Ctrl Pts',(-8.25616163200005,15.2,6.69802013199998));
#246598=CARTESIAN_POINT('Ctrl Pts',(-8.25616163200005,11.6,6.69802013199998));
#246599=CARTESIAN_POINT('Ctrl Pts',(-8.25815165800006,15.2,6.69896937999999));
#246600=CARTESIAN_POINT('Ctrl Pts',(-8.25815165800006,11.6,6.69896937999999));
#246601=CARTESIAN_POINT('Ctrl Pts',(-8.26014853900006,15.2,6.69991973099999));
#246602=CARTESIAN_POINT('Ctrl Pts',(-8.26014853900006,11.6,6.69991973099999));
#246603=CARTESIAN_POINT('Ctrl Pts',(-8.26215226500005,15.2,6.70087116699998));
#246604=CARTESIAN_POINT('Ctrl Pts',(-8.26215226500005,11.6,6.70087116699998));
#246605=CARTESIAN_POINT('Ctrl Pts',(-8.26416282900006,15.2,6.70182367299999));
#246606=CARTESIAN_POINT('Ctrl Pts',(-8.26416282900006,11.6,6.70182367299999));
#246607=CARTESIAN_POINT('Ctrl Pts',(-8.26618022200006,15.2,6.70277723399998));
#246608=CARTESIAN_POINT('Ctrl Pts',(-8.26618022200006,11.6,6.70277723399998));
#246609=CARTESIAN_POINT('Ctrl Pts',(-8.26820443600005,15.2,6.70373183399998));
#246610=CARTESIAN_POINT('Ctrl Pts',(-8.26820443600005,11.6,6.70373183399998));
#246611=CARTESIAN_POINT('Ctrl Pts',(-8.27023546500006,15.2,6.70468745899999));
#246612=CARTESIAN_POINT('Ctrl Pts',(-8.27023546500006,11.6,6.70468745899999));
#246613=CARTESIAN_POINT('Ctrl Pts',(-8.27227330000006,15.2,6.70564409399999));
#246614=CARTESIAN_POINT('Ctrl Pts',(-8.27227330000006,11.6,6.70564409399999));
#246615=CARTESIAN_POINT('Ctrl Pts',(-8.27431793400006,15.2,6.70660172299999));
#246616=CARTESIAN_POINT('Ctrl Pts',(-8.27431793400006,11.6,6.70660172299999));
#246617=CARTESIAN_POINT('Ctrl Pts',(-8.27636935800006,15.2,6.70756033199999));
#246618=CARTESIAN_POINT('Ctrl Pts',(-8.27636935800006,11.6,6.70756033199999));
#246619=CARTESIAN_POINT('Ctrl Pts',(-8.27842756500005,15.2,6.70851990399999));
#246620=CARTESIAN_POINT('Ctrl Pts',(-8.27842756500005,11.6,6.70851990399999));
#246621=CARTESIAN_POINT('Ctrl Pts',(-8.28049254600005,15.2,6.70948042599999));
#246622=CARTESIAN_POINT('Ctrl Pts',(-8.28049254600005,11.6,6.70948042599999));
#246623=CARTESIAN_POINT('Ctrl Pts',(-8.28256429600006,15.2,6.71044188299999));
#246624=CARTESIAN_POINT('Ctrl Pts',(-8.28256429600006,11.6,6.71044188299999));
#246625=CARTESIAN_POINT('Ctrl Pts',(-8.28464280400006,15.2,6.71140425899999));
#246626=CARTESIAN_POINT('Ctrl Pts',(-8.28464280400006,11.6,6.71140425899999));
#246627=CARTESIAN_POINT('Ctrl Pts',(-8.28672806400006,15.2,6.71236754099999));
#246628=CARTESIAN_POINT('Ctrl Pts',(-8.28672806400006,11.6,6.71236754099999));
#246629=CARTESIAN_POINT('Ctrl Pts',(-8.28882006800006,15.2,6.71333171199999));
#246630=CARTESIAN_POINT('Ctrl Pts',(-8.28882006800006,11.6,6.71333171199999));
#246631=CARTESIAN_POINT('Ctrl Pts',(-8.29091880900006,15.2,6.71429675899999));
#246632=CARTESIAN_POINT('Ctrl Pts',(-8.29091880900006,11.6,6.71429675899999));
#246633=CARTESIAN_POINT('Ctrl Pts',(-8.29302427900006,15.2,6.71526266699999));
#246634=CARTESIAN_POINT('Ctrl Pts',(-8.29302427900006,11.6,6.71526266699999));
#246635=CARTESIAN_POINT('Ctrl Pts',(-8.29513646900006,15.2,6.71622942099999));
#246636=CARTESIAN_POINT('Ctrl Pts',(-8.29513646900006,11.6,6.71622942099999));
#246637=CARTESIAN_POINT('Ctrl Pts',(-8.29725537200006,15.2,6.71719700699998));
#246638=CARTESIAN_POINT('Ctrl Pts',(-8.29725537200006,11.6,6.71719700699998));
#246639=CARTESIAN_POINT('Ctrl Pts',(-8.29938098200006,15.2,6.71816541099999));
#246640=CARTESIAN_POINT('Ctrl Pts',(-8.29938098200006,11.6,6.71816541099999));
#246641=CARTESIAN_POINT('Ctrl Pts',(-8.30151329000006,15.2,6.71913461699998));
#246642=CARTESIAN_POINT('Ctrl Pts',(-8.30151329000006,11.6,6.71913461699998));
#246643=CARTESIAN_POINT('Ctrl Pts',(-8.30365228800006,15.2,6.72010461099998));
#246644=CARTESIAN_POINT('Ctrl Pts',(-8.30365228800006,11.6,6.72010461099998));
#246645=CARTESIAN_POINT('Ctrl Pts',(-8.30579796800006,15.2,6.72107537999998));
#246646=CARTESIAN_POINT('Ctrl Pts',(-8.30579796800006,11.6,6.72107537999998));
#246647=CARTESIAN_POINT('Ctrl Pts',(-8.30795032400006,15.2,6.72204690899999));
#246648=CARTESIAN_POINT('Ctrl Pts',(-8.30795032400006,11.6,6.72204690899999));
#246649=CARTESIAN_POINT('Ctrl Pts',(-8.31010934700006,15.2,6.72301918299999));
#246650=CARTESIAN_POINT('Ctrl Pts',(-8.31010934700006,11.6,6.72301918299999));
#246651=CARTESIAN_POINT('Ctrl Pts',(-8.31227503200006,15.2,6.72399218899999));
#246652=CARTESIAN_POINT('Ctrl Pts',(-8.31227503200006,11.6,6.72399218899999));
#246653=CARTESIAN_POINT('Ctrl Pts',(-8.31444736700006,15.2,6.72496591099998));
#246654=CARTESIAN_POINT('Ctrl Pts',(-8.31444736700006,11.6,6.72496591099998));
#246655=CARTESIAN_POINT('Ctrl Pts',(-8.31662634800006,15.2,6.72594033599999));
#246656=CARTESIAN_POINT('Ctrl Pts',(-8.31662634800006,11.6,6.72594033599999));
#246657=CARTESIAN_POINT('Ctrl Pts',(-8.31881196700006,15.2,6.72691545099998));
#246658=CARTESIAN_POINT('Ctrl Pts',(-8.31881196700006,11.6,6.72691545099998));
#246659=CARTESIAN_POINT('Ctrl Pts',(-8.32100421400006,15.2,6.72789124199999));
#246660=CARTESIAN_POINT('Ctrl Pts',(-8.32100421400006,11.6,6.72789124199999));
#246661=CARTESIAN_POINT('Ctrl Pts',(-8.32320308600006,15.2,6.72886769299998));
#246662=CARTESIAN_POINT('Ctrl Pts',(-8.32320308600006,11.6,6.72886769299998));
#246663=CARTESIAN_POINT('Ctrl Pts',(-8.32540857100006,15.2,6.72984479099998));
#246664=CARTESIAN_POINT('Ctrl Pts',(-8.32540857100006,11.6,6.72984479099998));
#246665=CARTESIAN_POINT('Ctrl Pts',(-8.32762066300005,15.2,6.73082252199999));
#246666=CARTESIAN_POINT('Ctrl Pts',(-8.32762066300005,11.6,6.73082252199999));
#246667=CARTESIAN_POINT('Ctrl Pts',(-8.32983935500006,15.2,6.73180087299999));
#246668=CARTESIAN_POINT('Ctrl Pts',(-8.32983935500006,11.6,6.73180087299999));
#246669=CARTESIAN_POINT('Ctrl Pts',(-8.33206464000006,15.2,6.73277982899998));
#246670=CARTESIAN_POINT('Ctrl Pts',(-8.33206464000006,11.6,6.73277982899998));
#246671=CARTESIAN_POINT('Ctrl Pts',(-8.33429651000005,15.2,6.73375937799998));
#246672=CARTESIAN_POINT('Ctrl Pts',(-8.33429651000005,11.6,6.73375937799998));
#246673=CARTESIAN_POINT('Ctrl Pts',(-8.33653495700006,15.2,6.73473950399998));
#246674=CARTESIAN_POINT('Ctrl Pts',(-8.33653495700006,11.6,6.73473950399998));
#246675=CARTESIAN_POINT('Ctrl Pts',(-8.33877997400006,15.2,6.73572019399998));
#246676=CARTESIAN_POINT('Ctrl Pts',(-8.33877997400006,11.6,6.73572019399998));
#246677=CARTESIAN_POINT('Ctrl Pts',(-8.34103155400006,15.2,6.73670143699999));
#246678=CARTESIAN_POINT('Ctrl Pts',(-8.34103155400006,11.6,6.73670143699999));
#246679=CARTESIAN_POINT('Ctrl Pts',(-8.34328968900006,15.2,6.73768321599999));
#246680=CARTESIAN_POINT('Ctrl Pts',(-8.34328968900006,11.6,6.73768321599999));
#246681=CARTESIAN_POINT('Ctrl Pts',(-8.34555437200006,15.2,6.73866551899999));
#246682=CARTESIAN_POINT('Ctrl Pts',(-8.34555437200006,11.6,6.73866551899999));
#246683=CARTESIAN_POINT('Ctrl Pts',(-8.34782559500006,15.2,6.73964833199998));
#246684=CARTESIAN_POINT('Ctrl Pts',(-8.34782559500006,11.6,6.73964833199998));
#246685=CARTESIAN_POINT('Ctrl Pts',(-8.35010335200005,15.2,6.74063164199998));
#246686=CARTESIAN_POINT('Ctrl Pts',(-8.35010335200005,11.6,6.74063164199998));
#246687=CARTESIAN_POINT('Ctrl Pts',(-8.35238763300006,15.2,6.74161543599999));
#246688=CARTESIAN_POINT('Ctrl Pts',(-8.35238763300006,11.6,6.74161543599999));
#246689=CARTESIAN_POINT('Ctrl Pts',(-8.35467843300006,15.2,6.74259969899998));
#246690=CARTESIAN_POINT('Ctrl Pts',(-8.35467843300006,11.6,6.74259969899998));
#246691=CARTESIAN_POINT('Ctrl Pts',(-8.35697574500006,15.2,6.74358441899999));
#246692=CARTESIAN_POINT('Ctrl Pts',(-8.35697574500006,11.6,6.74358441899999));
#246693=CARTESIAN_POINT('Ctrl Pts',(-8.35927956000006,15.2,6.74456958299999));
#246694=CARTESIAN_POINT('Ctrl Pts',(-8.35927956000006,11.6,6.74456958299999));
#246695=CARTESIAN_POINT('Ctrl Pts',(-8.36158987100006,15.2,6.74555517699999));
#246696=CARTESIAN_POINT('Ctrl Pts',(-8.36158987100006,11.6,6.74555517699999));
#246697=CARTESIAN_POINT('Ctrl Pts',(-8.36390667000006,15.2,6.74654118799998));
#246698=CARTESIAN_POINT('Ctrl Pts',(-8.36390667000006,11.6,6.74654118799998));
#246699=CARTESIAN_POINT('Ctrl Pts',(-8.36622995200005,15.2,6.74752760299998));
#246700=CARTESIAN_POINT('Ctrl Pts',(-8.36622995200005,11.6,6.74752760299998));
#246701=CARTESIAN_POINT('Ctrl Pts',(-8.36855970800006,15.2,6.74851440899998));
#246702=CARTESIAN_POINT('Ctrl Pts',(-8.36855970800006,11.6,6.74851440899998));
#246703=CARTESIAN_POINT('Ctrl Pts',(-8.37089593200006,15.2,6.74950159299998));
#246704=CARTESIAN_POINT('Ctrl Pts',(-8.37089593200006,11.6,6.74950159299998));
#246705=CARTESIAN_POINT('Ctrl Pts',(-8.37323861500006,15.2,6.75048914099998));
#246706=CARTESIAN_POINT('Ctrl Pts',(-8.37323861500006,11.6,6.75048914099998));
#246707=CARTESIAN_POINT('Ctrl Pts',(-8.37558775000005,15.2,6.75147704099999));
#246708=CARTESIAN_POINT('Ctrl Pts',(-8.37558775000005,11.6,6.75147704099999));
#246709=CARTESIAN_POINT('Ctrl Pts',(-8.37794333100006,15.2,6.75246527999998));
#246710=CARTESIAN_POINT('Ctrl Pts',(-8.37794333100006,11.6,6.75246527999998));
#246711=CARTESIAN_POINT('Ctrl Pts',(-8.38030535100006,15.2,6.75345384399999));
#246712=CARTESIAN_POINT('Ctrl Pts',(-8.38030535100006,11.6,6.75345384399999));
#246713=CARTESIAN_POINT('Ctrl Pts',(-8.38267379900006,15.2,6.75444272199999));
#246714=CARTESIAN_POINT('Ctrl Pts',(-8.38267379900006,11.6,6.75444272199999));
#246715=CARTESIAN_POINT('Ctrl Pts',(-8.38504867400006,15.2,6.75543189999999));
#246716=CARTESIAN_POINT('Ctrl Pts',(-8.38504867400006,11.6,6.75543189999999));
#246717=CARTESIAN_POINT('Ctrl Pts',(-8.38742996300006,15.2,6.75642136499999));
#246718=CARTESIAN_POINT('Ctrl Pts',(-8.38742996300006,11.6,6.75642136499999));
#246719=CARTESIAN_POINT('Ctrl Pts',(-8.38981766300006,15.2,6.75741110399999));
#246720=CARTESIAN_POINT('Ctrl Pts',(-8.38981766300006,11.6,6.75741110399999));
#246721=CARTESIAN_POINT('Ctrl Pts',(-8.39221176300006,15.2,6.75840110599999));
#246722=CARTESIAN_POINT('Ctrl Pts',(-8.39221176300006,11.6,6.75840110599999));
#246723=CARTESIAN_POINT('Ctrl Pts',(-8.39461225900006,15.2,6.75939135599998));
#246724=CARTESIAN_POINT('Ctrl Pts',(-8.39461225900006,11.6,6.75939135599998));
#246725=CARTESIAN_POINT('Ctrl Pts',(-8.39701914300005,15.2,6.76038184399999));
#246726=CARTESIAN_POINT('Ctrl Pts',(-8.39701914300005,11.6,6.76038184399999));
#246727=CARTESIAN_POINT('Ctrl Pts',(-8.39943240800006,15.2,6.76137255499999));
#246728=CARTESIAN_POINT('Ctrl Pts',(-8.39943240800006,11.6,6.76137255499999));
#246729=CARTESIAN_POINT('Ctrl Pts',(-8.40185204500006,15.2,6.76236347699999));
#246730=CARTESIAN_POINT('Ctrl Pts',(-8.40185204500006,11.6,6.76236347699999));
#246731=CARTESIAN_POINT('Ctrl Pts',(-8.40427804900006,15.2,6.76335459899998));
#246732=CARTESIAN_POINT('Ctrl Pts',(-8.40427804900006,11.6,6.76335459899998));
#246733=CARTESIAN_POINT('Ctrl Pts',(-8.40671041200006,15.2,6.76434590699999));
#246734=CARTESIAN_POINT('Ctrl Pts',(-8.40671041200006,11.6,6.76434590699999));
#246735=CARTESIAN_POINT('Ctrl Pts',(-8.40914912700006,15.2,6.76533738899998));
#246736=CARTESIAN_POINT('Ctrl Pts',(-8.40914912700006,11.6,6.76533738899998));
#246737=CARTESIAN_POINT('Ctrl Pts',(-8.41159418600006,15.2,6.76632903299998));
#246738=CARTESIAN_POINT('Ctrl Pts',(-8.41159418600006,11.6,6.76632903299998));
#246739=CARTESIAN_POINT('Ctrl Pts',(-8.41404558400006,15.2,6.76732082599998));
#246740=CARTESIAN_POINT('Ctrl Pts',(-8.41404558400006,11.6,6.76732082599998));
#246741=CARTESIAN_POINT('Ctrl Pts',(-8.41650331200006,15.2,6.76831275599999));
#246742=CARTESIAN_POINT('Ctrl Pts',(-8.41650331200006,11.6,6.76831275599999));
#246743=CARTESIAN_POINT('Ctrl Pts',(-8.41896736400006,15.2,6.76930480999999));
#246744=CARTESIAN_POINT('Ctrl Pts',(-8.41896736400006,11.6,6.76930480999999));
#246745=CARTESIAN_POINT('Ctrl Pts',(-8.42143773200006,15.2,6.77029697699999));
#246746=CARTESIAN_POINT('Ctrl Pts',(-8.42143773200006,11.6,6.77029697699999));
#246747=CARTESIAN_POINT('Ctrl Pts',(-8.42391441000006,15.2,6.77128924499999));
#246748=CARTESIAN_POINT('Ctrl Pts',(-8.42391441000006,11.6,6.77128924499999));
#246749=CARTESIAN_POINT('Ctrl Pts',(-8.42639739000006,15.2,6.77228159899999));
#246750=CARTESIAN_POINT('Ctrl Pts',(-8.42639739000006,11.6,6.77228159899999));
#246751=CARTESIAN_POINT('Ctrl Pts',(-8.42888666600006,15.2,6.77327402999998));
#246752=CARTESIAN_POINT('Ctrl Pts',(-8.42888666600006,11.6,6.77327402999998));
#246753=CARTESIAN_POINT('Ctrl Pts',(-8.43138223000006,15.2,6.77426652399999));
#246754=CARTESIAN_POINT('Ctrl Pts',(-8.43138223000006,11.6,6.77426652399999));
#246755=CARTESIAN_POINT('Ctrl Pts',(-8.43388407600006,15.2,6.77525906999998));
#246756=CARTESIAN_POINT('Ctrl Pts',(-8.43388407600006,11.6,6.77525906999998));
#246757=CARTESIAN_POINT('Ctrl Pts',(-8.43639219500006,15.2,6.77625165599999));
#246758=CARTESIAN_POINT('Ctrl Pts',(-8.43639219500006,11.6,6.77625165599999));
#246759=CARTESIAN_POINT('Ctrl Pts',(-8.43890658200005,15.2,6.77724426899999));
#246760=CARTESIAN_POINT('Ctrl Pts',(-8.43890658200005,11.6,6.77724426899999));
#246761=CARTESIAN_POINT('Ctrl Pts',(-8.44142722800006,15.2,6.77823689799999));
#246762=CARTESIAN_POINT('Ctrl Pts',(-8.44142722800006,11.6,6.77823689799999));
#246763=CARTESIAN_POINT('Ctrl Pts',(-8.44395412900005,15.2,6.77922952999998));
#246764=CARTESIAN_POINT('Ctrl Pts',(-8.44395412900005,11.6,6.77922952999998));
#246765=CARTESIAN_POINT('Ctrl Pts',(-8.44648727500006,15.2,6.78022215499999));
#246766=CARTESIAN_POINT('Ctrl Pts',(-8.44648727500006,11.6,6.78022215499999));
#246767=CARTESIAN_POINT('Ctrl Pts',(-8.44902666200005,15.2,6.78121475899999));
#246768=CARTESIAN_POINT('Ctrl Pts',(-8.44902666200005,11.6,6.78121475899999));
#246769=CARTESIAN_POINT('Ctrl Pts',(-8.45157228000006,15.2,6.78220733099998));
#246770=CARTESIAN_POINT('Ctrl Pts',(-8.45157228000006,11.6,6.78220733099998));
#246771=CARTESIAN_POINT('Ctrl Pts',(-8.45412412400006,15.2,6.78319985899999));
#246772=CARTESIAN_POINT('Ctrl Pts',(-8.45412412400006,11.6,6.78319985899999));
#246773=CARTESIAN_POINT('Ctrl Pts',(-8.45668218700006,15.2,6.78419233299999));
#246774=CARTESIAN_POINT('Ctrl Pts',(-8.45668218700006,11.6,6.78419233299999));
#246775=CARTESIAN_POINT('Ctrl Pts',(-8.45924646000006,15.2,6.78518473899998));
#246776=CARTESIAN_POINT('Ctrl Pts',(-8.45924646000006,11.6,6.78518473899998));
#246777=CARTESIAN_POINT('Ctrl Pts',(-8.46181693900006,15.2,6.78617706599999));
#246778=CARTESIAN_POINT('Ctrl Pts',(-8.46181693900006,11.6,6.78617706599999));
#246779=CARTESIAN_POINT('Ctrl Pts',(-8.46439361500006,15.2,6.78716930199998));
#246780=CARTESIAN_POINT('Ctrl Pts',(-8.46439361500006,11.6,6.78716930199998));
#246781=CARTESIAN_POINT('Ctrl Pts',(-8.46697648200006,15.2,6.78816143599998));
#246782=CARTESIAN_POINT('Ctrl Pts',(-8.46697648200006,11.6,6.78816143599998));
#246783=CARTESIAN_POINT('Ctrl Pts',(-8.46956553300006,15.2,6.78915345699998));
#246784=CARTESIAN_POINT('Ctrl Pts',(-8.46956553300006,11.6,6.78915345699998));
#246785=CARTESIAN_POINT('Ctrl Pts',(-8.47216076100005,15.2,6.79014535399999));
#246786=CARTESIAN_POINT('Ctrl Pts',(-8.47216076100005,11.6,6.79014535399999));
#246787=CARTESIAN_POINT('Ctrl Pts',(-8.47476215800006,15.2,6.79113711099999));
#246788=CARTESIAN_POINT('Ctrl Pts',(-8.47476215800006,11.6,6.79113711099999));
#246789=CARTESIAN_POINT('Ctrl Pts',(-8.47736972000006,15.2,6.79212872199999));
#246790=CARTESIAN_POINT('Ctrl Pts',(-8.47736972000006,11.6,6.79212872199999));
#246791=CARTESIAN_POINT('Ctrl Pts',(-8.47998343700005,15.2,6.79312017299999));
#246792=CARTESIAN_POINT('Ctrl Pts',(-8.47998343700005,11.6,6.79312017299999));
#246793=CARTESIAN_POINT('Ctrl Pts',(-8.48260330400005,15.2,6.79411145299999));
#246794=CARTESIAN_POINT('Ctrl Pts',(-8.48260330400005,11.6,6.79411145299999));
#246795=CARTESIAN_POINT('Ctrl Pts',(-8.48522931400005,15.2,6.79510254999999));
#246796=CARTESIAN_POINT('Ctrl Pts',(-8.48522931400005,11.6,6.79510254999999));
#246797=CARTESIAN_POINT('Ctrl Pts',(-8.48786146000006,15.2,6.79609345399999));
#246798=CARTESIAN_POINT('Ctrl Pts',(-8.48786146000006,11.6,6.79609345399999));
#246799=CARTESIAN_POINT('Ctrl Pts',(-8.49049973400006,15.2,6.79708415199999));
#246800=CARTESIAN_POINT('Ctrl Pts',(-8.49049973400006,11.6,6.79708415199999));
#246801=CARTESIAN_POINT('Ctrl Pts',(-8.49314413000006,15.2,6.79807463399998));
#246802=CARTESIAN_POINT('Ctrl Pts',(-8.49314413000006,11.6,6.79807463399998));
#246803=CARTESIAN_POINT('Ctrl Pts',(-8.49579464300006,15.2,6.79906488799999));
#246804=CARTESIAN_POINT('Ctrl Pts',(-8.49579464300006,11.6,6.79906488799999));
#246805=CARTESIAN_POINT('Ctrl Pts',(-8.49845126200006,15.2,6.80005490199999));
#246806=CARTESIAN_POINT('Ctrl Pts',(-8.49845126200006,11.6,6.80005490199999));
#246807=CARTESIAN_POINT('Ctrl Pts',(-8.50111398500006,15.2,6.80104466699999));
#246808=CARTESIAN_POINT('Ctrl Pts',(-8.50111398500006,11.6,6.80104466699999));
#246809=CARTESIAN_POINT('Ctrl Pts',(-8.50378280200006,15.2,6.80203417099998));
#246810=CARTESIAN_POINT('Ctrl Pts',(-8.50378280200006,11.6,6.80203417099998));
#246811=CARTESIAN_POINT('Ctrl Pts',(-8.50645770800006,15.2,6.80302340199999));
#246812=CARTESIAN_POINT('Ctrl Pts',(-8.50645770800006,11.6,6.80302340199999));
#246813=CARTESIAN_POINT('Ctrl Pts',(-8.50913869400006,15.2,6.80401234999999));
#246814=CARTESIAN_POINT('Ctrl Pts',(-8.50913869400006,11.6,6.80401234999999));
#246815=CARTESIAN_POINT('Ctrl Pts',(-8.51182575500006,15.2,6.80500100299999));
#246816=CARTESIAN_POINT('Ctrl Pts',(-8.51182575500006,11.6,6.80500100299999));
#246817=CARTESIAN_POINT('Ctrl Pts',(-8.51451888400005,15.2,6.80598934999999));
#246818=CARTESIAN_POINT('Ctrl Pts',(-8.51451888400005,11.6,6.80598934999999));
#246819=CARTESIAN_POINT('Ctrl Pts',(-8.51721807400006,15.2,6.80697738099998));
#246820=CARTESIAN_POINT('Ctrl Pts',(-8.51721807400006,11.6,6.80697738099998));
#246821=CARTESIAN_POINT('Ctrl Pts',(-8.51992331900006,15.2,6.80796508499999));
#246822=CARTESIAN_POINT('Ctrl Pts',(-8.51992331900006,11.6,6.80796508499999));
#246823=CARTESIAN_POINT('Ctrl Pts',(-8.52263461100006,15.2,6.80895244999999));
#246824=CARTESIAN_POINT('Ctrl Pts',(-8.52263461100006,11.6,6.80895244999999));
#246825=CARTESIAN_POINT('Ctrl Pts',(-8.52535194400006,15.2,6.80993946599998));
#246826=CARTESIAN_POINT('Ctrl Pts',(-8.52535194400006,11.6,6.80993946599998));
#246827=CARTESIAN_POINT('Ctrl Pts',(-8.52807531100006,15.2,6.81092612099999));
#246828=CARTESIAN_POINT('Ctrl Pts',(-8.52807531100006,11.6,6.81092612099999));
#246829=CARTESIAN_POINT('Ctrl Pts',(-8.53080470500006,15.2,6.81191240399999));
#246830=CARTESIAN_POINT('Ctrl Pts',(-8.53080470500006,11.6,6.81191240399999));
#246831=CARTESIAN_POINT('Ctrl Pts',(-8.53354012000005,15.2,6.81289830599999));
#246832=CARTESIAN_POINT('Ctrl Pts',(-8.53354012000005,11.6,6.81289830599999));
#246833=CARTESIAN_POINT('Ctrl Pts',(-8.53628154900005,15.2,6.81388381599999));
#246834=CARTESIAN_POINT('Ctrl Pts',(-8.53628154900005,11.6,6.81388381599999));
#246835=CARTESIAN_POINT('Ctrl Pts',(-8.53902898600005,15.2,6.81486892199998));
#246836=CARTESIAN_POINT('Ctrl Pts',(-8.53902898600005,11.6,6.81486892199998));
#246837=CARTESIAN_POINT('Ctrl Pts',(-8.54178242300006,15.2,6.81585361399998));
#246838=CARTESIAN_POINT('Ctrl Pts',(-8.54178242300006,11.6,6.81585361399998));
#246839=CARTESIAN_POINT('Ctrl Pts',(-8.54454185400006,15.2,6.81683788099999));
#246840=CARTESIAN_POINT('Ctrl Pts',(-8.54454185400006,11.6,6.81683788099999));
#246841=CARTESIAN_POINT('Ctrl Pts',(-8.54730727200005,15.2,6.81782171199998));
#246842=CARTESIAN_POINT('Ctrl Pts',(-8.54730727200005,11.6,6.81782171199998));
#246843=CARTESIAN_POINT('Ctrl Pts',(-8.55007867000005,15.2,6.81880509699998));
#246844=CARTESIAN_POINT('Ctrl Pts',(-8.55007867000005,11.6,6.81880509699998));
#246845=CARTESIAN_POINT('Ctrl Pts',(-8.55285604400006,15.2,6.81978802599998));
#246846=CARTESIAN_POINT('Ctrl Pts',(-8.55285604400006,11.6,6.81978802599998));
#246847=CARTESIAN_POINT('Ctrl Pts',(-8.55563938300006,15.2,6.82077048699998));
#246848=CARTESIAN_POINT('Ctrl Pts',(-8.55563938300006,11.6,6.82077048699998));
#246849=CARTESIAN_POINT('Ctrl Pts',(-8.55842868500006,15.2,6.82175246999999));
#246850=CARTESIAN_POINT('Ctrl Pts',(-8.55842868500006,11.6,6.82175246999999));
#246851=CARTESIAN_POINT('Ctrl Pts',(-8.56122393900005,15.2,6.82273396399999));
#246852=CARTESIAN_POINT('Ctrl Pts',(-8.56122393900005,11.6,6.82273396399999));
#246853=CARTESIAN_POINT('Ctrl Pts',(-8.56402514200006,15.2,6.82371496099999));
#246854=CARTESIAN_POINT('Ctrl Pts',(-8.56402514200006,11.6,6.82371496099999));
#246855=CARTESIAN_POINT('Ctrl Pts',(-8.56683228400006,15.2,6.82469544699998));
#246856=CARTESIAN_POINT('Ctrl Pts',(-8.56683228400006,11.6,6.82469544699998));
#246857=CARTESIAN_POINT('Ctrl Pts',(-8.56964536200006,15.2,6.82567541399998));
#246858=CARTESIAN_POINT('Ctrl Pts',(-8.56964536200006,11.6,6.82567541399998));
#246859=CARTESIAN_POINT('Ctrl Pts',(-8.57246436700006,15.2,6.82665484999998));
#246860=CARTESIAN_POINT('Ctrl Pts',(-8.57246436700006,11.6,6.82665484999998));
#246861=CARTESIAN_POINT('Ctrl Pts',(-8.57528929200006,15.2,6.82763374599999));
#246862=CARTESIAN_POINT('Ctrl Pts',(-8.57528929200006,11.6,6.82763374599999));
#246863=CARTESIAN_POINT('Ctrl Pts',(-8.57812013200006,15.2,6.82861209099999));
#246864=CARTESIAN_POINT('Ctrl Pts',(-8.57812013200006,11.6,6.82861209099999));
#246865=CARTESIAN_POINT('Ctrl Pts',(-8.58095688000006,15.2,6.82958987499998));
#246866=CARTESIAN_POINT('Ctrl Pts',(-8.58095688000006,11.6,6.82958987499998));
#246867=CARTESIAN_POINT('Ctrl Pts',(-8.58379953000006,15.2,6.83056708799998));
#246868=CARTESIAN_POINT('Ctrl Pts',(-8.58379953000006,11.6,6.83056708799998));
#246869=CARTESIAN_POINT('Ctrl Pts',(-8.58664807300006,15.2,6.83154371699998));
#246870=CARTESIAN_POINT('Ctrl Pts',(-8.58664807300006,11.6,6.83154371699998));
#246871=CARTESIAN_POINT('Ctrl Pts',(-8.58950250400006,15.2,6.83251975699999));
#246872=CARTESIAN_POINT('Ctrl Pts',(-8.58950250400006,11.6,6.83251975699999));
#246873=CARTESIAN_POINT('Ctrl Pts',(-8.59236281800005,15.2,6.83349519299998));
#246874=CARTESIAN_POINT('Ctrl Pts',(-8.59236281800005,11.6,6.83349519299998));
#246875=CARTESIAN_POINT('Ctrl Pts',(-8.59522900700006,15.2,6.83447001699999));
#246876=CARTESIAN_POINT('Ctrl Pts',(-8.59522900700006,11.6,6.83447001699999));
#246877=CARTESIAN_POINT('Ctrl Pts',(-8.59810106400005,15.2,6.83544421899998));
#246878=CARTESIAN_POINT('Ctrl Pts',(-8.59810106400005,11.6,6.83544421899998));
#246879=CARTESIAN_POINT('Ctrl Pts',(-8.60097898200006,15.2,6.83641778699998));
#246880=CARTESIAN_POINT('Ctrl Pts',(-8.60097898200006,11.6,6.83641778699998));
#246881=CARTESIAN_POINT('Ctrl Pts',(-8.60386275600005,15.2,6.83739071399999));
#246882=CARTESIAN_POINT('Ctrl Pts',(-8.60386275600005,11.6,6.83739071399999));
#246883=CARTESIAN_POINT('Ctrl Pts',(-8.60675237900006,15.2,6.83836298699998));
#246884=CARTESIAN_POINT('Ctrl Pts',(-8.60675237900006,11.6,6.83836298699998));
#246885=CARTESIAN_POINT('Ctrl Pts',(-8.60964784400006,15.2,6.83933459799999));
#246886=CARTESIAN_POINT('Ctrl Pts',(-8.60964784400006,11.6,6.83933459799999));
#246887=CARTESIAN_POINT('Ctrl Pts',(-8.61254914500006,15.2,6.84030553499999));
#246888=CARTESIAN_POINT('Ctrl Pts',(-8.61254914500006,11.6,6.84030553499999));
#246889=CARTESIAN_POINT('Ctrl Pts',(-8.61545627500006,15.2,6.84127579099999));
#246890=CARTESIAN_POINT('Ctrl Pts',(-8.61545627500006,11.6,6.84127579099999));
#246891=CARTESIAN_POINT('Ctrl Pts',(-8.61836922900006,15.2,6.84224535299998));
#246892=CARTESIAN_POINT('Ctrl Pts',(-8.61836922900006,11.6,6.84224535299998));
#246893=CARTESIAN_POINT('Ctrl Pts',(-8.62128799900006,15.2,6.84321421299998));
#246894=CARTESIAN_POINT('Ctrl Pts',(-8.62128799900006,11.6,6.84321421299998));
#246895=CARTESIAN_POINT('Ctrl Pts',(-8.62421257700005,15.2,6.84418235999999));
#246896=CARTESIAN_POINT('Ctrl Pts',(-8.62421257700005,11.6,6.84418235999999));
#246897=CARTESIAN_POINT('Ctrl Pts',(-8.62714296000006,15.2,6.84514978399999));
#246898=CARTESIAN_POINT('Ctrl Pts',(-8.62714296000006,11.6,6.84514978399999));
#246899=CARTESIAN_POINT('Ctrl Pts',(-8.63007914000006,15.2,6.84611647699998));
#246900=CARTESIAN_POINT('Ctrl Pts',(-8.63007914000006,11.6,6.84611647699998));
#246901=CARTESIAN_POINT('Ctrl Pts',(-8.63302111000005,15.2,6.84708242699998));
#246902=CARTESIAN_POINT('Ctrl Pts',(-8.63302111000005,11.6,6.84708242699998));
#246903=CARTESIAN_POINT('Ctrl Pts',(-8.63596886400006,15.2,6.84804762499999));
#246904=CARTESIAN_POINT('Ctrl Pts',(-8.63596886400006,11.6,6.84804762499999));
#246905=CARTESIAN_POINT('Ctrl Pts',(-8.63892239600006,15.2,6.84901206199999));
#246906=CARTESIAN_POINT('Ctrl Pts',(-8.63892239600006,11.6,6.84901206199999));
#246907=CARTESIAN_POINT('Ctrl Pts',(-8.64188169900006,15.2,6.84997572699999));
#246908=CARTESIAN_POINT('Ctrl Pts',(-8.64188169900006,11.6,6.84997572699999));
#246909=CARTESIAN_POINT('Ctrl Pts',(-8.64484676600006,15.2,6.85093861099999));
#246910=CARTESIAN_POINT('Ctrl Pts',(-8.64484676600006,11.6,6.85093861099999));
#246911=CARTESIAN_POINT('Ctrl Pts',(-8.64781759100006,15.2,6.85190070499999));
#246912=CARTESIAN_POINT('Ctrl Pts',(-8.64781759100006,11.6,6.85190070499999));
#246913=CARTESIAN_POINT('Ctrl Pts',(-8.65079416900006,15.2,6.85286199699998));
#246914=CARTESIAN_POINT('Ctrl Pts',(-8.65079416900006,11.6,6.85286199699998));
#246915=CARTESIAN_POINT('Ctrl Pts',(-8.65377649100006,15.2,6.85382247999998));
#246916=CARTESIAN_POINT('Ctrl Pts',(-8.65377649100006,11.6,6.85382247999998));
#246917=CARTESIAN_POINT('Ctrl Pts',(-8.65676455400006,15.2,6.85478214199998));
#246918=CARTESIAN_POINT('Ctrl Pts',(-8.65676455400006,11.6,6.85478214199998));
#246919=CARTESIAN_POINT('Ctrl Pts',(-8.65975834800006,15.2,6.85574097599999));
#246920=CARTESIAN_POINT('Ctrl Pts',(-8.65975834800006,11.6,6.85574097599999));
#246921=CARTESIAN_POINT('Ctrl Pts',(-8.66275786800006,15.2,6.85669897099999));
#246922=CARTESIAN_POINT('Ctrl Pts',(-8.66275786800006,11.6,6.85669897099999));
#246923=CARTESIAN_POINT('Ctrl Pts',(-8.66576310800006,15.2,6.85765611699999));
#246924=CARTESIAN_POINT('Ctrl Pts',(-8.66576310800006,11.6,6.85765611699999));
#246925=CARTESIAN_POINT('Ctrl Pts',(-8.66877406100006,15.2,6.85861240499998));
#246926=CARTESIAN_POINT('Ctrl Pts',(-8.66877406100006,11.6,6.85861240499998));
#246927=CARTESIAN_POINT('Ctrl Pts',(-8.67179072300006,15.2,6.85956782599998));
#246928=CARTESIAN_POINT('Ctrl Pts',(-8.67179072300006,11.6,6.85956782599998));
#246929=CARTESIAN_POINT('Ctrl Pts',(-8.67481308300006,15.2,6.86052236899998));
#246930=CARTESIAN_POINT('Ctrl Pts',(-8.67481308300006,11.6,6.86052236899998));
#246931=CARTESIAN_POINT('Ctrl Pts',(-8.67784113900005,15.2,6.86147602699998));
#246932=CARTESIAN_POINT('Ctrl Pts',(-8.67784113900005,11.6,6.86147602699998));
#246933=CARTESIAN_POINT('Ctrl Pts',(-8.68087488300005,15.2,6.86242878899999));
#246934=CARTESIAN_POINT('Ctrl Pts',(-8.68087488300005,11.6,6.86242878899999));
#246935=CARTESIAN_POINT('Ctrl Pts',(-8.68391430700006,15.2,6.86338064599998));
#246936=CARTESIAN_POINT('Ctrl Pts',(-8.68391430700006,11.6,6.86338064599998));
#246937=CARTESIAN_POINT('Ctrl Pts',(-8.68695940700006,15.2,6.86433158899998));
#246938=CARTESIAN_POINT('Ctrl Pts',(-8.68695940700006,11.6,6.86433158899998));
#246939=CARTESIAN_POINT('Ctrl Pts',(-8.69001017600005,15.2,6.86528160699999));
#246940=CARTESIAN_POINT('Ctrl Pts',(-8.69001017600005,11.6,6.86528160699999));
#246941=CARTESIAN_POINT('Ctrl Pts',(-8.69306660800006,15.2,6.86623069199998));
#246942=CARTESIAN_POINT('Ctrl Pts',(-8.69306660800006,11.6,6.86623069199998));
#246943=CARTESIAN_POINT('Ctrl Pts',(-8.69612869600006,15.2,6.86717883599999));
#246944=CARTESIAN_POINT('Ctrl Pts',(-8.69612869600006,11.6,6.86717883599999));
#246945=CARTESIAN_POINT('Ctrl Pts',(-8.69919643300006,15.2,6.86812602599999));
#246946=CARTESIAN_POINT('Ctrl Pts',(-8.69919643300006,11.6,6.86812602599999));
#246947=CARTESIAN_POINT('Ctrl Pts',(-8.70226981400006,15.2,6.86907225699999));
#246948=CARTESIAN_POINT('Ctrl Pts',(-8.70226981400006,11.6,6.86907225699999));
#246949=CARTESIAN_POINT('Ctrl Pts',(-8.70534883200006,15.2,6.87001751699999));
#246950=CARTESIAN_POINT('Ctrl Pts',(-8.70534883200006,11.6,6.87001751699999));
#246951=CARTESIAN_POINT('Ctrl Pts',(-8.70843348100006,15.2,6.87096179799998));
#246952=CARTESIAN_POINT('Ctrl Pts',(-8.70843348100006,11.6,6.87096179799998));
#246953=CARTESIAN_POINT('Ctrl Pts',(-8.71152375500006,15.2,6.87190509099998));
#246954=CARTESIAN_POINT('Ctrl Pts',(-8.71152375500006,11.6,6.87190509099998));
#246955=CARTESIAN_POINT('Ctrl Pts',(-8.71461964700006,15.2,6.87284738499999));
#246956=CARTESIAN_POINT('Ctrl Pts',(-8.71461964700006,11.6,6.87284738499999));
#246957=CARTESIAN_POINT('Ctrl Pts',(-8.71772115100006,15.2,6.87378867299999));
#246958=CARTESIAN_POINT('Ctrl Pts',(-8.71772115100006,11.6,6.87378867299999));
#246959=CARTESIAN_POINT('Ctrl Pts',(-8.72082826000005,15.2,6.87472894499999));
#246960=CARTESIAN_POINT('Ctrl Pts',(-8.72082826000005,11.6,6.87472894499999));
#246961=CARTESIAN_POINT('Ctrl Pts',(-8.72394096900006,15.2,6.87566819299998));
#246962=CARTESIAN_POINT('Ctrl Pts',(-8.72394096900006,11.6,6.87566819299998));
#246963=CARTESIAN_POINT('Ctrl Pts',(-8.72705927100006,15.2,6.87660640599999));
#246964=CARTESIAN_POINT('Ctrl Pts',(-8.72705927100006,11.6,6.87660640599999));
#246965=CARTESIAN_POINT('Ctrl Pts',(-8.73018316100006,15.2,6.87754357599999));
#246966=CARTESIAN_POINT('Ctrl Pts',(-8.73018316100006,11.6,6.87754357599999));
#246967=CARTESIAN_POINT('Ctrl Pts',(-8.73331263100006,15.2,6.87847969399999));
#246968=CARTESIAN_POINT('Ctrl Pts',(-8.73331263100006,11.6,6.87847969399999));
#246969=CARTESIAN_POINT('Ctrl Pts',(-8.73644767400006,15.2,6.87941475199998));
#246970=CARTESIAN_POINT('Ctrl Pts',(-8.73644767400006,11.6,6.87941475199998));
#246971=CARTESIAN_POINT('Ctrl Pts',(-8.73958828700006,15.2,6.88034873899999));
#246972=CARTESIAN_POINT('Ctrl Pts',(-8.73958828700006,11.6,6.88034873899999));
#246973=CARTESIAN_POINT('Ctrl Pts',(-8.74273446100006,15.2,6.88128164799998));
#246974=CARTESIAN_POINT('Ctrl Pts',(-8.74273446100006,11.6,6.88128164799998));
#246975=CARTESIAN_POINT('Ctrl Pts',(-8.74588619100006,15.2,6.88221346799998));
#246976=CARTESIAN_POINT('Ctrl Pts',(-8.74588619100006,11.6,6.88221346799998));
#246977=CARTESIAN_POINT('Ctrl Pts',(-8.74904346900006,15.2,6.88314419199998));
#246978=CARTESIAN_POINT('Ctrl Pts',(-8.74904346900006,11.6,6.88314419199998));
#246979=CARTESIAN_POINT('Ctrl Pts',(-8.75220629200006,15.2,6.88407381099999));
#246980=CARTESIAN_POINT('Ctrl Pts',(-8.75220629200006,11.6,6.88407381099999));
#246981=CARTESIAN_POINT('Ctrl Pts',(-8.75537465200006,15.2,6.88500231499999));
#246982=CARTESIAN_POINT('Ctrl Pts',(-8.75537465200006,11.6,6.88500231499999));
#246983=CARTESIAN_POINT('Ctrl Pts',(-8.75854854200006,15.2,6.88592969499998));
#246984=CARTESIAN_POINT('Ctrl Pts',(-8.75854854200006,11.6,6.88592969499998));
#246985=CARTESIAN_POINT('Ctrl Pts',(-8.76172795600005,15.2,6.88685594399999));
#246986=CARTESIAN_POINT('Ctrl Pts',(-8.76172795600005,11.6,6.88685594399999));
#246987=CARTESIAN_POINT('Ctrl Pts',(-8.76491288800005,15.2,6.88778105199999));
#246988=CARTESIAN_POINT('Ctrl Pts',(-8.76491288800005,11.6,6.88778105199999));
#246989=CARTESIAN_POINT('Ctrl Pts',(-8.76810333300006,15.2,6.88870501099998));
#246990=CARTESIAN_POINT('Ctrl Pts',(-8.76810333300006,11.6,6.88870501099998));
#246991=CARTESIAN_POINT('Ctrl Pts',(-8.77129928400005,15.2,6.88962781099999));
#246992=CARTESIAN_POINT('Ctrl Pts',(-8.77129928400005,11.6,6.88962781099999));
#246993=CARTESIAN_POINT('Ctrl Pts',(-8.77450073400006,15.2,6.89054944399999));
#246994=CARTESIAN_POINT('Ctrl Pts',(-8.77450073400006,11.6,6.89054944399999));
#246995=CARTESIAN_POINT('Ctrl Pts',(-8.77770767800006,15.2,6.89146990199998));
#246996=CARTESIAN_POINT('Ctrl Pts',(-8.77770767800006,11.6,6.89146990199998));
#246997=CARTESIAN_POINT('Ctrl Pts',(-8.78092011000006,15.2,6.89238917599998));
#246998=CARTESIAN_POINT('Ctrl Pts',(-8.78092011000006,11.6,6.89238917599998));
#246999=CARTESIAN_POINT('Ctrl Pts',(-8.78413802200006,15.2,6.89330725599999));
#247000=CARTESIAN_POINT('Ctrl Pts',(-8.78413802200006,11.6,6.89330725599999));
#247001=CARTESIAN_POINT('Ctrl Pts',(-8.78736140900006,15.2,6.89422413499998));
#247002=CARTESIAN_POINT('Ctrl Pts',(-8.78736140900006,11.6,6.89422413499998));
#247003=CARTESIAN_POINT('Ctrl Pts',(-8.79059026600006,15.2,6.89513980399998));
#247004=CARTESIAN_POINT('Ctrl Pts',(-8.79059026600006,11.6,6.89513980399998));
#247005=CARTESIAN_POINT('Ctrl Pts',(-8.79382458400006,15.2,6.89605425399999));
#247006=CARTESIAN_POINT('Ctrl Pts',(-8.79382458400006,11.6,6.89605425399999));
#247007=CARTESIAN_POINT('Ctrl Pts',(-8.79706435900006,15.2,6.89696747699998));
#247008=CARTESIAN_POINT('Ctrl Pts',(-8.79706435900006,11.6,6.89696747699998));
#247009=CARTESIAN_POINT('Ctrl Pts',(-8.80030958500006,15.2,6.89787946299998));
#247010=CARTESIAN_POINT('Ctrl Pts',(-8.80030958500006,11.6,6.89787946299998));
#247011=CARTESIAN_POINT('Ctrl Pts',(-8.80356025500006,15.2,6.89879020499998));
#247012=CARTESIAN_POINT('Ctrl Pts',(-8.80356025500006,11.6,6.89879020499998));
#247013=CARTESIAN_POINT('Ctrl Pts',(-8.80681636300006,15.2,6.89969969599999));
#247014=CARTESIAN_POINT('Ctrl Pts',(-8.80681636300006,11.6,6.89969969599999));
#247015=CARTESIAN_POINT('Ctrl Pts',(-8.81007790200006,15.2,6.90060792399999));
#247016=CARTESIAN_POINT('Ctrl Pts',(-8.81007790200006,11.6,6.90060792399999));
#247017=CARTESIAN_POINT('Ctrl Pts',(-8.81334486800006,15.2,6.90151488299998));
#247018=CARTESIAN_POINT('Ctrl Pts',(-8.81334486800006,11.6,6.90151488299998));
#247019=CARTESIAN_POINT('Ctrl Pts',(-8.81661725300006,15.2,6.90242056299999));
#247020=CARTESIAN_POINT('Ctrl Pts',(-8.81661725300006,11.6,6.90242056299999));
#247021=CARTESIAN_POINT('Ctrl Pts',(-8.81989505200006,15.2,6.90332495799999));
#247022=CARTESIAN_POINT('Ctrl Pts',(-8.81989505200006,11.6,6.90332495799999));
#247023=CARTESIAN_POINT('Ctrl Pts',(-8.82317825900006,15.2,6.90422805599999));
#247024=CARTESIAN_POINT('Ctrl Pts',(-8.82317825900006,11.6,6.90422805599999));
#247025=CARTESIAN_POINT('Ctrl Pts',(-8.82646686600006,15.2,6.90512985099998));
#247026=CARTESIAN_POINT('Ctrl Pts',(-8.82646686600006,11.6,6.90512985099998));
#247027=CARTESIAN_POINT('Ctrl Pts',(-8.82976086800005,15.2,6.90603033599999));
#247028=CARTESIAN_POINT('Ctrl Pts',(-8.82976086800005,11.6,6.90603033599999));
#247029=CARTESIAN_POINT('Ctrl Pts',(-8.83306026000006,15.2,6.90692949999999));
#247030=CARTESIAN_POINT('Ctrl Pts',(-8.83306026000006,11.6,6.90692949999999));
#247031=CARTESIAN_POINT('Ctrl Pts',(-8.83636503500006,15.2,6.90782733499999));
#247032=CARTESIAN_POINT('Ctrl Pts',(-8.83636503500006,11.6,6.90782733499999));
#247033=CARTESIAN_POINT('Ctrl Pts',(-8.83967518800005,15.2,6.90872383499999));
#247034=CARTESIAN_POINT('Ctrl Pts',(-8.83967518800005,11.6,6.90872383499999));
#247035=CARTESIAN_POINT('Ctrl Pts',(-8.84299071000006,15.2,6.90961898899998));
#247036=CARTESIAN_POINT('Ctrl Pts',(-8.84299071000006,11.6,6.90961898899998));
#247037=CARTESIAN_POINT('Ctrl Pts',(-8.84631159700006,15.2,6.91051278999999));
#247038=CARTESIAN_POINT('Ctrl Pts',(-8.84631159700006,11.6,6.91051278999999));
#247039=CARTESIAN_POINT('Ctrl Pts',(-8.84963784400006,15.2,6.91140523099998));
#247040=CARTESIAN_POINT('Ctrl Pts',(-8.84963784400006,11.6,6.91140523099998));
#247041=CARTESIAN_POINT('Ctrl Pts',(-8.85296944200006,15.2,6.91229630099999));
#247042=CARTESIAN_POINT('Ctrl Pts',(-8.85296944200006,11.6,6.91229630099999));
#247043=CARTESIAN_POINT('Ctrl Pts',(-8.85630638700006,15.2,6.91318599399998));
#247044=CARTESIAN_POINT('Ctrl Pts',(-8.85630638700006,11.6,6.91318599399998));
#247045=CARTESIAN_POINT('Ctrl Pts',(-8.85964867400006,15.2,6.91407430099999));
#247046=CARTESIAN_POINT('Ctrl Pts',(-8.85964867400006,11.6,6.91407430099999));
#247047=CARTESIAN_POINT('Ctrl Pts',(-8.86299629400006,15.2,6.91496121399998));
#247048=CARTESIAN_POINT('Ctrl Pts',(-8.86299629400006,11.6,6.91496121399998));
#247049=CARTESIAN_POINT('Ctrl Pts',(-8.86634924200006,15.2,6.91584672599999));
#247050=CARTESIAN_POINT('Ctrl Pts',(-8.86634924200006,11.6,6.91584672599999));
#247051=CARTESIAN_POINT('Ctrl Pts',(-8.86970751300005,15.2,6.91673082599999));
#247052=CARTESIAN_POINT('Ctrl Pts',(-8.86970751300005,11.6,6.91673082599999));
#247053=CARTESIAN_POINT('Ctrl Pts',(-8.87307110100006,15.2,6.91761350899998));
#247054=CARTESIAN_POINT('Ctrl Pts',(-8.87307110100006,11.6,6.91761350899998));
#247055=CARTESIAN_POINT('Ctrl Pts',(-8.87643999800006,15.2,6.91849476499999));
#247056=CARTESIAN_POINT('Ctrl Pts',(-8.87643999800006,11.6,6.91849476499999));
#247057=CARTESIAN_POINT('Ctrl Pts',(-8.87981420000006,15.2,6.91937458799998));
#247058=CARTESIAN_POINT('Ctrl Pts',(-8.87981420000006,11.6,6.91937458799998));
#247059=CARTESIAN_POINT('Ctrl Pts',(-8.88319370000006,15.2,6.92025296799999));
#247060=CARTESIAN_POINT('Ctrl Pts',(-8.88319370000006,11.6,6.92025296799999));
#247061=CARTESIAN_POINT('Ctrl Pts',(-8.88657849200006,15.2,6.92112989699999));
#247062=CARTESIAN_POINT('Ctrl Pts',(-8.88657849200006,11.6,6.92112989699999));
#247063=CARTESIAN_POINT('Ctrl Pts',(-8.88996857100006,15.2,6.92200536799999));
#247064=CARTESIAN_POINT('Ctrl Pts',(-8.88996857100006,11.6,6.92200536799999));
#247065=CARTESIAN_POINT('Ctrl Pts',(-8.89336393000006,15.2,6.92287937299999));
#247066=CARTESIAN_POINT('Ctrl Pts',(-8.89336393000006,11.6,6.92287937299999));
#247067=CARTESIAN_POINT('Ctrl Pts',(-8.89676456200006,15.2,6.92375190499998));
#247068=CARTESIAN_POINT('Ctrl Pts',(-8.89676456200006,11.6,6.92375190499998));
#247069=CARTESIAN_POINT('Ctrl Pts',(-8.90017046300006,15.2,6.92462295199999));
#247070=CARTESIAN_POINT('Ctrl Pts',(-8.90017046300006,11.6,6.92462295199999));
#247071=CARTESIAN_POINT('Ctrl Pts',(-8.90358162600006,15.2,6.92549251099998));
#247072=CARTESIAN_POINT('Ctrl Pts',(-8.90358162600006,11.6,6.92549251099998));
#247073=CARTESIAN_POINT('Ctrl Pts',(-8.90699804400005,15.2,6.92636057199999));
#247074=CARTESIAN_POINT('Ctrl Pts',(-8.90699804400005,11.6,6.92636057199999));
#247075=CARTESIAN_POINT('Ctrl Pts',(-8.91041971400006,15.2,6.92722712699998));
#247076=CARTESIAN_POINT('Ctrl Pts',(-8.91041971400006,11.6,6.92722712699998));
#247077=CARTESIAN_POINT('Ctrl Pts',(-8.91384662700006,15.2,6.92809216799999));
#247078=CARTESIAN_POINT('Ctrl Pts',(-8.91384662700006,11.6,6.92809216799999));
#247079=CARTESIAN_POINT('Ctrl Pts',(-8.91727877800006,15.2,6.92895568799998));
#247080=CARTESIAN_POINT('Ctrl Pts',(-8.91727877800006,11.6,6.92895568799998));
#247081=CARTESIAN_POINT('Ctrl Pts',(-8.92071616200005,15.2,6.92981767899998));
#247082=CARTESIAN_POINT('Ctrl Pts',(-8.92071616200005,11.6,6.92981767899998));
#247083=CARTESIAN_POINT('Ctrl Pts',(-8.92415877200006,15.2,6.93067813199999));
#247084=CARTESIAN_POINT('Ctrl Pts',(-8.92415877200006,11.6,6.93067813199999));
#247085=CARTESIAN_POINT('Ctrl Pts',(-8.92760660200006,15.2,6.93153704099998));
#247086=CARTESIAN_POINT('Ctrl Pts',(-8.92760660200006,11.6,6.93153704099998));
#247087=CARTESIAN_POINT('Ctrl Pts',(-8.93105964700006,15.2,6.93239439799999));
#247088=CARTESIAN_POINT('Ctrl Pts',(-8.93105964700006,11.6,6.93239439799999));
#247089=CARTESIAN_POINT('Ctrl Pts',(-8.93451790000006,15.2,6.93325019299999));
#247090=CARTESIAN_POINT('Ctrl Pts',(-8.93451790000006,11.6,6.93325019299999));
#247091=CARTESIAN_POINT('Ctrl Pts',(-8.93798135500005,15.2,6.93410442099999));
#247092=CARTESIAN_POINT('Ctrl Pts',(-8.93798135500005,11.6,6.93410442099999));
#247093=CARTESIAN_POINT('Ctrl Pts',(-8.94145000700006,15.2,6.93495707399999));
#247094=CARTESIAN_POINT('Ctrl Pts',(-8.94145000700006,11.6,6.93495707399999));
#247095=CARTESIAN_POINT('Ctrl Pts',(-8.94492384900006,15.2,6.93580814299998));
#247096=CARTESIAN_POINT('Ctrl Pts',(-8.94492384900006,11.6,6.93580814299998));
#247097=CARTESIAN_POINT('Ctrl Pts',(-8.94840287600006,15.2,6.93665762099998));
#247098=CARTESIAN_POINT('Ctrl Pts',(-8.94840287600006,11.6,6.93665762099998));
#247099=CARTESIAN_POINT('Ctrl Pts',(-8.95188708200006,15.2,6.93750550099999));
#247100=CARTESIAN_POINT('Ctrl Pts',(-8.95188708200006,11.6,6.93750550099999));
#247101=CARTESIAN_POINT('Ctrl Pts',(-8.95537645900006,15.2,6.93835177399999));
#247102=CARTESIAN_POINT('Ctrl Pts',(-8.95537645900006,11.6,6.93835177399999));
#247103=CARTESIAN_POINT('Ctrl Pts',(-8.95887100500006,15.2,6.93919643299999));
#247104=CARTESIAN_POINT('Ctrl Pts',(-8.95887100500006,11.6,6.93919643299999));
#247105=CARTESIAN_POINT('Ctrl Pts',(-8.96237071000006,15.2,6.94003947099999));
#247106=CARTESIAN_POINT('Ctrl Pts',(-8.96237071000006,11.6,6.94003947099999));
#247107=CARTESIAN_POINT('Ctrl Pts',(-8.96587557000006,15.2,6.94088087999998));
#247108=CARTESIAN_POINT('Ctrl Pts',(-8.96587557000006,11.6,6.94088087999998));
#247109=CARTESIAN_POINT('Ctrl Pts',(-8.96938558000006,15.2,6.94172065299998));
#247110=CARTESIAN_POINT('Ctrl Pts',(-8.96938558000006,11.6,6.94172065299998));
#247111=CARTESIAN_POINT('Ctrl Pts',(-8.97290073400006,15.2,6.94255878199999));
#247112=CARTESIAN_POINT('Ctrl Pts',(-8.97290073400006,11.6,6.94255878199999));
#247113=CARTESIAN_POINT('Ctrl Pts',(-8.97642102300006,15.2,6.94339525799998));
#247114=CARTESIAN_POINT('Ctrl Pts',(-8.97642102300006,11.6,6.94339525799998));
#247115=CARTESIAN_POINT('Ctrl Pts',(-8.97994644400006,15.2,6.94423007599998));
#247116=CARTESIAN_POINT('Ctrl Pts',(-8.97994644400006,11.6,6.94423007599998));
#247117=CARTESIAN_POINT('Ctrl Pts',(-8.98347699100006,15.2,6.94506322799998));
#247118=CARTESIAN_POINT('Ctrl Pts',(-8.98347699100006,11.6,6.94506322799998));
#247119=CARTESIAN_POINT('Ctrl Pts',(-8.98701265700005,15.2,6.94589470499999));
#247120=CARTESIAN_POINT('Ctrl Pts',(-8.98701265700005,11.6,6.94589470499999));
#247121=CARTESIAN_POINT('Ctrl Pts',(-8.99055343700006,15.2,6.94672450099999));
#247122=CARTESIAN_POINT('Ctrl Pts',(-8.99055343700006,11.6,6.94672450099999));
#247123=CARTESIAN_POINT('Ctrl Pts',(-8.99409932400006,15.2,6.94755260799998));
#247124=CARTESIAN_POINT('Ctrl Pts',(-8.99409932400006,11.6,6.94755260799998));
#247125=CARTESIAN_POINT('Ctrl Pts',(-8.99765031400005,15.2,6.94837901999998));
#247126=CARTESIAN_POINT('Ctrl Pts',(-8.99765031400005,11.6,6.94837901999998));
#247127=CARTESIAN_POINT('Ctrl Pts',(-9.00120639900006,15.2,6.94920372699999));
#247128=CARTESIAN_POINT('Ctrl Pts',(-9.00120639900006,11.6,6.94920372699999));
#247129=CARTESIAN_POINT('Ctrl Pts',(-9.00476757400006,15.2,6.95002672299999));
#247130=CARTESIAN_POINT('Ctrl Pts',(-9.00476757400006,11.6,6.95002672299999));
#247131=CARTESIAN_POINT('Ctrl Pts',(-9.00833383300006,15.2,6.95084800199999));
#247132=CARTESIAN_POINT('Ctrl Pts',(-9.00833383300006,11.6,6.95084800199999));
#247133=CARTESIAN_POINT('Ctrl Pts',(-9.01190517100006,15.2,6.95166755499999));
#247134=CARTESIAN_POINT('Ctrl Pts',(-9.01190517100006,11.6,6.95166755499999));
#247135=CARTESIAN_POINT('Ctrl Pts',(-9.01548158200006,15.2,6.95248537499998));
#247136=CARTESIAN_POINT('Ctrl Pts',(-9.01548158200006,11.6,6.95248537499998));
#247137=CARTESIAN_POINT('Ctrl Pts',(-9.01906305900006,15.2,6.95330145399998));
#247138=CARTESIAN_POINT('Ctrl Pts',(-9.01906305900006,11.6,6.95330145399998));
#247139=CARTESIAN_POINT('Ctrl Pts',(-9.02264959700006,15.2,6.95411578599998));
#247140=CARTESIAN_POINT('Ctrl Pts',(-9.02264959700006,11.6,6.95411578599998));
#247141=CARTESIAN_POINT('Ctrl Pts',(-9.02624119000006,15.2,6.95492836299999));
#247142=CARTESIAN_POINT('Ctrl Pts',(-9.02624119000006,11.6,6.95492836299999));
#247143=CARTESIAN_POINT('Ctrl Pts',(-9.02983783100006,15.2,6.95573917899999));
#247144=CARTESIAN_POINT('Ctrl Pts',(-9.02983783100006,11.6,6.95573917899999));
#247145=CARTESIAN_POINT('Ctrl Pts',(-9.03343951600006,15.2,6.95654822399998));
#247146=CARTESIAN_POINT('Ctrl Pts',(-9.03343951600006,11.6,6.95654822399998));
#247147=CARTESIAN_POINT('Ctrl Pts',(-9.03704623800006,15.2,6.95735549299999));
#247148=CARTESIAN_POINT('Ctrl Pts',(-9.03704623800006,11.6,6.95735549299999));
#247149=CARTESIAN_POINT('Ctrl Pts',(-9.04065799200006,15.2,6.95816097899999));
#247150=CARTESIAN_POINT('Ctrl Pts',(-9.04065799200006,11.6,6.95816097899999));
#247151=CARTESIAN_POINT('Ctrl Pts',(-9.04427477200005,15.2,6.95896467299999));
#247152=CARTESIAN_POINT('Ctrl Pts',(-9.04427477200005,11.6,6.95896467299999));
#247153=CARTESIAN_POINT('Ctrl Pts',(-9.04789657200006,15.2,6.95976657099998));
#247154=CARTESIAN_POINT('Ctrl Pts',(-9.04789657200006,11.6,6.95976657099998));
#247155=CARTESIAN_POINT('Ctrl Pts',(-9.05152338600006,15.2,6.96056666299998));
#247156=CARTESIAN_POINT('Ctrl Pts',(-9.05152338600006,11.6,6.96056666299998));
#247157=CARTESIAN_POINT('Ctrl Pts',(-9.05515520900006,15.2,6.96136494399998));
#247158=CARTESIAN_POINT('Ctrl Pts',(-9.05515520900006,11.6,6.96136494399998));
#247159=CARTESIAN_POINT('Ctrl Pts',(-9.05879203500006,15.2,6.96216140399999));
#247160=CARTESIAN_POINT('Ctrl Pts',(-9.05879203500006,11.6,6.96216140399999));
#247161=CARTESIAN_POINT('Ctrl Pts',(-9.06243385700006,15.2,6.96295603899999));
#247162=CARTESIAN_POINT('Ctrl Pts',(-9.06243385700006,11.6,6.96295603899999));
#247163=CARTESIAN_POINT('Ctrl Pts',(-9.06608067000005,15.2,6.96374884099999));
#247164=CARTESIAN_POINT('Ctrl Pts',(-9.06608067000005,11.6,6.96374884099999));
#247165=CARTESIAN_POINT('Ctrl Pts',(-9.06973246700005,15.2,6.96453979999998));
#247166=CARTESIAN_POINT('Ctrl Pts',(-9.06973246700005,11.6,6.96453979999998));
#247167=CARTESIAN_POINT('Ctrl Pts',(-9.07338924200005,15.2,6.96532891099999));
#247168=CARTESIAN_POINT('Ctrl Pts',(-9.07338924200005,11.6,6.96532891099999));
#247169=CARTESIAN_POINT('Ctrl Pts',(-9.07705099100006,15.2,6.96611616699998));
#247170=CARTESIAN_POINT('Ctrl Pts',(-9.07705099100006,11.6,6.96611616699998));
#247171=CARTESIAN_POINT('Ctrl Pts',(-9.08071770800005,15.2,6.96690156099999));
#247172=CARTESIAN_POINT('Ctrl Pts',(-9.08071770800005,11.6,6.96690156099999));
#247173=CARTESIAN_POINT('Ctrl Pts',(-9.08438938600005,15.2,6.96768508699999));
#247174=CARTESIAN_POINT('Ctrl Pts',(-9.08438938600005,11.6,6.96768508699999));
#247175=CARTESIAN_POINT('Ctrl Pts',(-9.08806602100006,15.2,6.96846673699999));
#247176=CARTESIAN_POINT('Ctrl Pts',(-9.08806602100006,11.6,6.96846673699999));
#247177=CARTESIAN_POINT('Ctrl Pts',(-9.09174760800006,15.2,6.96924650799998));
#247178=CARTESIAN_POINT('Ctrl Pts',(-9.09174760800006,11.6,6.96924650799998));
#247179=CARTESIAN_POINT('Ctrl Pts',(-9.09543414200006,15.2,6.97002439099998));
#247180=CARTESIAN_POINT('Ctrl Pts',(-9.09543414200006,11.6,6.97002439099998));
#247181=CARTESIAN_POINT('Ctrl Pts',(-9.09912561600006,15.2,6.97080037899998));
#247182=CARTESIAN_POINT('Ctrl Pts',(-9.09912561600006,11.6,6.97080037899998));
#247183=CARTESIAN_POINT('Ctrl Pts',(-9.10282202200005,15.2,6.97157446399999));
#247184=CARTESIAN_POINT('Ctrl Pts',(-9.10282202200005,11.6,6.97157446399999));
#247185=CARTESIAN_POINT('Ctrl Pts',(-9.10652335600006,15.2,6.97234663799998));
#247186=CARTESIAN_POINT('Ctrl Pts',(-9.10652335600006,11.6,6.97234663799998));
#247187=CARTESIAN_POINT('Ctrl Pts',(-9.11022960900005,15.2,6.97311689299998));
#247188=CARTESIAN_POINT('Ctrl Pts',(-9.11022960900005,11.6,6.97311689299998));
#247189=CARTESIAN_POINT('Ctrl Pts',(-9.11394077400006,15.2,6.97388521799999));
#247190=CARTESIAN_POINT('Ctrl Pts',(-9.11394077400006,11.6,6.97388521799999));
#247191=CARTESIAN_POINT('Ctrl Pts',(-9.11765684500006,15.2,6.97465160799998));
#247192=CARTESIAN_POINT('Ctrl Pts',(-9.11765684500006,11.6,6.97465160799998));
#247193=CARTESIAN_POINT('Ctrl Pts',(-9.12137781700006,15.2,6.97541605599999));
#247194=CARTESIAN_POINT('Ctrl Pts',(-9.12137781700006,11.6,6.97541605599999));
#247195=CARTESIAN_POINT('Ctrl Pts',(-9.12510368600006,15.2,6.97617855899999));
#247196=CARTESIAN_POINT('Ctrl Pts',(-9.12510368600006,11.6,6.97617855899999));
#247197=CARTESIAN_POINT('Ctrl Pts',(-9.12883445000006,15.2,6.97693911099999));
#247198=CARTESIAN_POINT('Ctrl Pts',(-9.12883445000006,11.6,6.97693911099999));
#247199=CARTESIAN_POINT('Ctrl Pts',(-9.13257010500006,15.2,6.97769771199999));
#247200=CARTESIAN_POINT('Ctrl Pts',(-9.13257010500006,11.6,6.97769771199999));
#247201=CARTESIAN_POINT('Ctrl Pts',(-9.13556254400006,15.2,6.97830303199999));
#247202=CARTESIAN_POINT('Ctrl Pts',(-9.13556254400006,11.6,6.97830303199999));
#247203=CARTESIAN_POINT('Ctrl Pts',(-9.13780907400006,15.2,6.97875614399998));
#247204=CARTESIAN_POINT('Ctrl Pts',(-9.13780907400006,11.6,6.97875614399998));
#247205=CARTESIAN_POINT('Ctrl Pts',(-9.13930773800006,15.2,6.97905782699999));
#247206=CARTESIAN_POINT('Ctrl Pts',(-9.13930773800006,11.6,6.97905782699999));
#247207=CARTESIAN_POINT('Ctrl Pts',(-9.14005731500006,15.2,6.97920857099999));
#247208=CARTESIAN_POINT('Ctrl Pts',(-9.14005731500006,11.6,6.97920857099999));
#247209=CARTESIAN_POINT('Ctrl Pts',(-8.02901631900006,15.2,6.57080831899999));
#247210=CARTESIAN_POINT('Ctrl Pts',(-8.03049110446229,15.2,6.57181685366614));
#247211=CARTESIAN_POINT('Ctrl Pts',(-8.0320161093278,15.2,6.57285322826574));
#247212=CARTESIAN_POINT('Ctrl Pts',(-8.03359089408583,15.2,6.57391635240017));
#247213=CARTESIAN_POINT('Ctrl Pts',(-8.03517327325199,15.2,6.57498460345654));
#247214=CARTESIAN_POINT('Ctrl Pts',(-8.03680591570089,15.2,6.57607986594818));
#247215=CARTESIAN_POINT('Ctrl Pts',(-8.03848839087952,15.2,6.57720107915013));
#247216=CARTESIAN_POINT('Ctrl Pts',(-8.04017086590532,15.2,6.57832229225026));
#247217=CARTESIAN_POINT('Ctrl Pts',(-8.04190317283137,15.2,6.57946945464252));
#247218=CARTESIAN_POINT('Ctrl Pts',(-8.04368489176663,15.2,6.58064153793327));
#247219=CARTESIAN_POINT('Ctrl Pts',(-8.04546661070189,15.2,6.58181362122402));
#247220=CARTESIAN_POINT('Ctrl Pts',(-8.04729774128707,15.2,6.58301062651662));
#247221=CARTESIAN_POINT('Ctrl Pts',(-8.04917787055988,15.2,6.58423155119856));
#247222=CARTESIAN_POINT('Ctrl Pts',(-8.05105800000347,15.2,6.58545247599141));
#247223=CARTESIAN_POINT('Ctrl Pts',(-8.05298713099614,15.2,6.58669732359249));
#247224=CARTESIAN_POINT('Ctrl Pts',(-8.05496485719055,15.2,6.58796512041314));
#247225=CARTESIAN_POINT('Ctrl Pts',(-8.05694258320533,15.2,6.58923291711864));
#247226=CARTESIAN_POINT('Ctrl Pts',(-8.05896890538341,15.2,6.59052366630055));
#247227=CARTESIAN_POINT('Ctrl Pts',(-8.06104342948425,15.2,6.59183642200888));
#247228=CARTESIAN_POINT('Ctrl Pts',(-8.06311795358509,15.2,6.59314917771721));
#247229=CARTESIAN_POINT('Ctrl Pts',(-8.0652406808045,15.2,6.59448394076801));
#247230=CARTESIAN_POINT('Ctrl Pts',(-8.06741122014022,15.2,6.59583979646781));
#247231=CARTESIAN_POINT('Ctrl Pts',(-8.06958175967308,15.2,6.59719565229079));
#247232=CARTESIAN_POINT('Ctrl Pts',(-8.0718001153119,15.2,6.5985725970414));
#247233=CARTESIAN_POINT('Ctrl Pts',(-8.07406590652196,15.2,6.59996974311891));
#247234=CARTESIAN_POINT('Ctrl Pts',(-8.0763316975262,15.2,6.60136688906953));
#247235=CARTESIAN_POINT('Ctrl Pts',(-8.07864492271251,15.2,6.60278423372136));
#247236=CARTESIAN_POINT('Ctrl Pts',(-8.0810052091288,15.2,6.60422091158666));
#247237=CARTESIAN_POINT('Ctrl Pts',(-8.08336549554508,15.2,6.60565758945196));
#247238=CARTESIAN_POINT('Ctrl Pts',(-8.08577284749928,15.2,6.60711359814904));
#247239=CARTESIAN_POINT('Ctrl Pts',(-8.08822689382476,15.2,6.608588095178));
#247240=CARTESIAN_POINT('Ctrl Pts',(-8.09068094015023,15.2,6.61006259220696));
#247241=CARTESIAN_POINT('Ctrl Pts',(-8.09318168323473,15.2,6.6115555767414));
#247242=CARTESIAN_POINT('Ctrl Pts',(-8.09572876447236,15.2,6.61306622685197));
#247243=CARTESIAN_POINT('Ctrl Pts',(-8.09827584594135,15.2,6.61457687709976));
#247244=CARTESIAN_POINT('Ctrl Pts',(-8.10086926266481,15.2,6.61610519104097));
#247245=CARTESIAN_POINT('Ctrl Pts',(-8.10350866514402,15.2,6.61765037037591));
#247246=CARTESIAN_POINT('Ctrl Pts',(-8.10614806738348,15.2,6.61919554957051));
#247247=CARTESIAN_POINT('Ctrl Pts',(-8.10883345256066,15.2,6.62075759004112));
#247248=CARTESIAN_POINT('Ctrl Pts',(-8.11156447572374,15.2,6.62233571524091));
#247249=CARTESIAN_POINT('Ctrl Pts',(-8.11429549888682,15.2,6.6239138404407));
#247250=CARTESIAN_POINT('Ctrl Pts',(-8.11707215754802,15.2,6.62550804702571));
#247251=CARTESIAN_POINT('Ctrl Pts',(-8.1198941109424,15.2,6.62711757454952));
#247252=CARTESIAN_POINT('Ctrl Pts',(-8.1227160645931,15.2,6.62872710221953));
#247253=CARTESIAN_POINT('Ctrl Pts',(-8.12558331343989,15.2,6.63035195259939));
#247254=CARTESIAN_POINT('Ctrl Pts',(-8.12849552018388,15.2,6.63199137835604));
#247255=CARTESIAN_POINT('Ctrl Pts',(-8.13140772666334,15.2,6.63363080396376));
#247256=CARTESIAN_POINT('Ctrl Pts',(-8.13436489186082,15.2,6.63528480756059));
#247257=CARTESIAN_POINT('Ctrl Pts',(-8.13736668326528,15.2,6.63695266325754));
#247258=CARTESIAN_POINT('Ctrl Pts',(-8.14036847466976,15.2,6.63862051895448));
#247259=CARTESIAN_POINT('Ctrl Pts',(-8.14341489333673,15.2,6.6403022281027));
#247260=CARTESIAN_POINT('Ctrl Pts',(-8.14650561163811,15.2,6.64199708079023));
#247261=CARTESIAN_POINT('Ctrl Pts',(-8.14959633022023,15.2,6.64369193363172));
#247262=CARTESIAN_POINT('Ctrl Pts',(-8.15273134875635,15.2,6.64539993184433));
#247263=CARTESIAN_POINT('Ctrl Pts',(-8.15591034659095,15.2,6.64712038194143));
#247264=CARTESIAN_POINT('Ctrl Pts',(-8.15908934413678,15.2,6.64884083188225));
#247265=CARTESIAN_POINT('Ctrl Pts',(-8.16231231977699,15.2,6.65057373567169));
#247266=CARTESIAN_POINT('Ctrl Pts',(-8.16557895524164,15.2,6.65231841652496));
#247267=CARTESIAN_POINT('Ctrl Pts',(-8.16884559070628,15.2,6.65406309737823));
#247268=CARTESIAN_POINT('Ctrl Pts',(-8.17215588738246,15.2,6.65581955514721));
#247269=CARTESIAN_POINT('Ctrl Pts',(-8.17550953292566,15.2,6.65758713108734));
#247270=CARTESIAN_POINT('Ctrl Pts',(-8.17886317877349,15.2,6.65935470718801));
#247271=CARTESIAN_POINT('Ctrl Pts',(-8.18226017247622,15.2,6.66113340036345));
#247272=CARTESIAN_POINT('Ctrl Pts',(-8.18570020341662,15.2,6.66292256646165));
#247273=CARTESIAN_POINT('Ctrl Pts',(-8.18914023404455,15.2,6.66471173239735));
#247274=CARTESIAN_POINT('Ctrl Pts',(-8.19262330516359,15.2,6.66651136899997));
#247275=CARTESIAN_POINT('Ctrl Pts',(-8.19614910871825,15.2,6.66832084802579));
#247276=CARTESIAN_POINT('Ctrl Pts',(-8.19967491227291,15.2,6.67013032705162));
#247277=CARTESIAN_POINT('Ctrl Pts',(-8.20324345005307,15.2,6.6719496470672));
#247278=CARTESIAN_POINT('Ctrl Pts',(-8.2068544195867,15.2,6.67377819116702));
#247279=CARTESIAN_POINT('Ctrl Pts',(-8.20986356097405,15.2,6.67530197797224));
#247280=CARTESIAN_POINT('Ctrl Pts',(-8.21290216901772,15.2,6.6768321706943));
#247281=CARTESIAN_POINT('Ctrl Pts',(-8.21597007276618,15.2,6.6783684191662));
#247282=CARTESIAN_POINT('Ctrl Pts',(-8.21903797651465,15.2,6.6799046676381));
#247283=CARTESIAN_POINT('Ctrl Pts',(-8.22213517478973,15.2,6.68144697153657));
#247284=CARTESIAN_POINT('Ctrl Pts',(-8.22526149549829,15.2,6.6829949875158));
#247285=CARTESIAN_POINT('Ctrl Pts',(-8.22838781620684,15.2,6.68454300349504));
#247286=CARTESIAN_POINT('Ctrl Pts',(-8.23154326289995,15.2,6.68609673124996));
#247287=CARTESIAN_POINT('Ctrl Pts',(-8.23472766269164,15.2,6.68765583249997));
#247288=CARTESIAN_POINT('Ctrl Pts',(-8.23854894230283,15.2,6.68952675393201));
#247289=CARTESIAN_POINT('Ctrl Pts',(-8.24241191793825,15.2,6.69140541580895));
#247290=CARTESIAN_POINT('Ctrl Pts',(-8.24631629865572,15.2,6.69329124133423));
#247291=CARTESIAN_POINT('Ctrl Pts',(-8.24956994937182,15.2,6.69486276266239));
#247292=CARTESIAN_POINT('Ctrl Pts',(-8.25285235445733,15.2,6.69643926186906));
#247293=CARTESIAN_POINT('Ctrl Pts',(-8.25616334681695,15.2,6.69802041068826));
#247294=CARTESIAN_POINT('Ctrl Pts',(-8.25947433917657,15.2,6.69960155950747));
#247295=CARTESIAN_POINT('Ctrl Pts',(-8.26281392218693,15.2,6.70118736157957));
#247296=CARTESIAN_POINT('Ctrl Pts',(-8.26618192704656,15.2,6.70277749366267));
#247297=CARTESIAN_POINT('Ctrl Pts',(-8.26954993190617,15.2,6.70436762574578));
#247298=CARTESIAN_POINT('Ctrl Pts',(-8.27294636232709,15.2,6.70596209069186));
#247299=CARTESIAN_POINT('Ctrl Pts',(-8.27637105373145,15.2,6.70756057278244));
#247300=CARTESIAN_POINT('Ctrl Pts',(-8.27979574513583,15.2,6.70915905487303));
#247301=CARTESIAN_POINT('Ctrl Pts',(-8.28324869771664,15.2,6.71076155453331));
#247302=CARTESIAN_POINT('Ctrl Pts',(-8.28672975000832,15.2,6.71236776328331));
#247303=CARTESIAN_POINT('Ctrl Pts',(-8.29021080229998,15.2,6.71397397203331));
#247304=CARTESIAN_POINT('Ctrl Pts',(-8.29371995558578,15.2,6.71558388856019));
#247305=CARTESIAN_POINT('Ctrl Pts',(-8.29725704872691,15.2,6.71719721148419));
#247306=CARTESIAN_POINT('Ctrl Pts',(-8.30079414186805,15.2,6.71881053440819));
#247307=CARTESIAN_POINT('Ctrl Pts',(-8.30435917615591,15.2,6.72042726148355));
#247308=CARTESIAN_POINT('Ctrl Pts',(-8.30795199101846,15.2,6.7220470953726));
#247309=CARTESIAN_POINT('Ctrl Pts',(-8.31154480588101,15.2,6.72366692926165));
#247310=CARTESIAN_POINT('Ctrl Pts',(-8.31516540353176,15.2,6.72528986717284));
#247311=CARTESIAN_POINT('Ctrl Pts',(-8.31881362429708,15.2,6.72691562008965));
#247312=CARTESIAN_POINT('Ctrl Pts',(-8.3224618450624,15.2,6.72854137300647));
#247313=CARTESIAN_POINT('Ctrl Pts',(-8.32613769035757,15.2,6.73016993708987));
#247314=CARTESIAN_POINT('Ctrl Pts',(-8.32984100348402,15.2,6.73180102438167));
#247315=CARTESIAN_POINT('Ctrl Pts',(-8.33354431661046,15.2,6.73343211167347));
#247316=CARTESIAN_POINT('Ctrl Pts',(-8.33727509821339,15.2,6.7350657214969));
#247317=CARTESIAN_POINT('Ctrl Pts',(-8.34103319319468,15.2,6.73670157123155));
#247318=CARTESIAN_POINT('Ctrl Pts',(-8.34479128817596,15.2,6.73833742096621));
#247319=CARTESIAN_POINT('Ctrl Pts',(-8.34857669656313,15.2,6.73997550786434));
#247320=CARTESIAN_POINT('Ctrl Pts',(-8.35238926323202,15.2,6.7416155534895));
#247321=CARTESIAN_POINT('Ctrl Pts',(-8.35620182990089,15.2,6.74325559911466));
#247322=CARTESIAN_POINT('Ctrl Pts',(-8.36004155802578,15.2,6.74489760268706));
#247323=CARTESIAN_POINT('Ctrl Pts',(-8.36390829122243,15.2,6.74654128921497));
#247324=CARTESIAN_POINT('Ctrl Pts',(-8.36700167752687,15.2,6.7478562383298));
#247325=CARTESIAN_POINT('Ctrl Pts',(-8.37011235030333,15.2,6.74917226514799));
#247326=CARTESIAN_POINT('Ctrl Pts',(-8.37324022800619,15.2,6.75048922899075));
#247327=CARTESIAN_POINT('Ctrl Pts',(-8.37636810613523,15.2,6.75180619301294));
#247328=CARTESIAN_POINT('Ctrl Pts',(-8.37951319143738,15.2,6.75312409465198));
#247329=CARTESIAN_POINT('Ctrl Pts',(-8.38267540616702,15.2,6.75444279722393));
#247330=CARTESIAN_POINT('Ctrl Pts',(-8.38583762046581,15.2,6.75576149961619));
#247331=CARTESIAN_POINT('Ctrl Pts',(-8.38901696530126,15.2,6.75708100143059));
#247332=CARTESIAN_POINT('Ctrl Pts',(-8.39221336170551,15.2,6.75840116793373));
#247333=CARTESIAN_POINT('Ctrl Pts',(-8.39540975854526,15.2,6.75972133461675));
#247334=CARTESIAN_POINT('Ctrl Pts',(-8.39862321024381,15.2,6.76104216575087));
#247335=CARTESIAN_POINT('Ctrl Pts',(-8.40185363719384,15.2,6.76236352716673));
#247336=CARTESIAN_POINT('Ctrl Pts',(-8.40508406370374,15.2,6.76368488840255));
#247337=CARTESIAN_POINT('Ctrl Pts',(-8.40833146682903,15.2,6.76500678031389));
#247338=CARTESIAN_POINT('Ctrl Pts',(-8.41159577044996,15.2,6.76632907015022));
#247339=CARTESIAN_POINT('Ctrl Pts',(-8.41486007451564,15.2,6.76765136016671));
#247340=CARTESIAN_POINT('Ctrl Pts',(-8.41814127968336,15.2,6.76897404709436));
#247341=CARTESIAN_POINT('Ctrl Pts',(-8.4214393097531,15.2,6.77029700233314));
#247342=CARTESIAN_POINT('Ctrl Pts',(-8.42473733937348,15.2,6.77161995739168));
#247343=CARTESIAN_POINT('Ctrl Pts',(-8.42805219426569,15.2,6.77294317811949));
#247344=CARTESIAN_POINT('Ctrl Pts',(-8.43138379999164,15.2,6.77426653679962));
#247345=CARTESIAN_POINT('Ctrl Pts',(-8.43471540617151,15.2,6.77558989566006));
#247346=CARTESIAN_POINT('Ctrl Pts',(-8.4380637612352,15.2,6.77691339275549));
#247347=CARTESIAN_POINT('Ctrl Pts',(-8.44142879197524,15.2,6.77823689888318));
#247348=CARTESIAN_POINT('Ctrl Pts',(-8.44563508017105,15.2,6.77989128145262));
#247349=CARTESIAN_POINT('Ctrl Pts',(-8.4498674242884,15.2,6.78154567890817));
#247350=CARTESIAN_POINT('Ctrl Pts',(-8.45412567901197,15.2,6.78319984557483));
#247351=CARTESIAN_POINT('Ctrl Pts',(-8.45753228251232,15.2,6.78452317879997));
#247352=CARTESIAN_POINT('Ctrl Pts',(-8.46095546774228,15.2,6.78584636423894));
#247353=CARTESIAN_POINT('Ctrl Pts',(-8.46439516224262,15.2,6.78716927630802));
#247354=CARTESIAN_POINT('Ctrl Pts',(-8.46783485721161,15.2,6.78849218855734));
#247355=CARTESIAN_POINT('Ctrl Pts',(-8.47129106073814,15.2,6.78981483024714));
#247356=CARTESIAN_POINT('Ctrl Pts',(-8.47476369948404,15.2,6.79113707454141));
#247357=CARTESIAN_POINT('Ctrl Pts',(-8.47823633775679,15.2,6.79245931865553));
#247358=CARTESIAN_POINT('Ctrl Pts',(-8.48172541120677,15.2,6.79378116889469));
#247359=CARTESIAN_POINT('Ctrl Pts',(-8.48523084741852,15.2,6.79510250150895));
#247360=CARTESIAN_POINT('Ctrl Pts',(-8.48961264304142,15.2,6.79675416741179));
#247361=CARTESIAN_POINT('Ctrl Pts',(-8.49402000303247,15.2,6.79840502507597));
#247362=CARTESIAN_POINT('Ctrl Pts',(-8.49845278741884,15.2,6.80005483953347));
#247363=CARTESIAN_POINT('Ctrl Pts',(-8.5028855718052,15.2,6.80170465399096));
#247364=CARTESIAN_POINT('Ctrl Pts',(-8.50734378101378,15.2,6.80335342785883));
#247365=CARTESIAN_POINT('Ctrl Pts',(-8.51182727170693,15.2,6.80500092640057));
#247366=CARTESIAN_POINT('Ctrl Pts',(-8.51631076240006,15.2,6.8066484249423));
#247367=CARTESIAN_POINT('Ctrl Pts',(-8.52081953651052,15.2,6.80829465141456));
#247368=CARTESIAN_POINT('Ctrl Pts',(-8.52535345220363,15.2,6.80993937565075));
#247369=CARTESIAN_POINT('Ctrl Pts',(-8.52988736789674,15.2,6.81158409988694));
#247370=CARTESIAN_POINT('Ctrl Pts',(-8.534446425299,15.2,6.81322732160831));
#247371=CARTESIAN_POINT('Ctrl Pts',(-8.53903048601416,15.2,6.81486881849076));
#247372=CARTESIAN_POINT('Ctrl Pts',(-8.54269773478616,15.2,6.81618201606829));
#247373=CARTESIAN_POINT('Ctrl Pts',(-8.54638098384325,15.2,6.81749410834855));
#247374=CARTESIAN_POINT('Ctrl Pts',(-8.55008016454649,15.2,6.81880498319765));
#247375=CARTESIAN_POINT('Ctrl Pts',(-8.5537793447457,15.2,6.82011585786814));
#247376=CARTESIAN_POINT('Ctrl Pts',(-8.55749445558174,15.2,6.82142551358878));
#247377=CARTESIAN_POINT('Ctrl Pts',(-8.5612254258868,15.2,6.82273383959303));
#247378=CARTESIAN_POINT('Ctrl Pts',(-8.5649563967002,15.2,6.82404216577552));
#247379=CARTESIAN_POINT('Ctrl Pts',(-8.56870322783498,15.2,6.82534916148094));
#247380=CARTESIAN_POINT('Ctrl Pts',(-8.57246584756273,15.2,6.82665471517276));
#247381=CARTESIAN_POINT('Ctrl Pts',(-8.57622846677783,15.2,6.82796026868669));
#247382=CARTESIAN_POINT('Ctrl Pts',(-8.58000687539563,15.2,6.82926438173321));
#247383=CARTESIAN_POINT('Ctrl Pts',(-8.5838010029733,15.2,6.83056694196016));
#247384=CARTESIAN_POINT('Ctrl Pts',(-8.58949219511525,15.2,6.83252078256678));
#247385=CARTESIAN_POINT('Ctrl Pts',(-8.59521875529496,15.2,6.83447113347301));
#247386=CARTESIAN_POINT('Ctrl Pts',(-8.60098044661137,15.2,6.83641762691216));
#247387=CARTESIAN_POINT('Ctrl Pts',(-8.60482157363228,15.2,6.83771528902813));
#247388=CARTESIAN_POINT('Ctrl Pts',(-8.60867831560116,15.2,6.83901123714431));
#247389=CARTESIAN_POINT('Ctrl Pts',(-8.61255060195025,15.2,6.84030536459418));
#247390=CARTESIAN_POINT('Ctrl Pts',(-8.61642288882695,15.2,6.84159949222039));
#247391=CARTESIAN_POINT('Ctrl Pts',(-8.62031072164352,15.2,6.8428917996526));
#247392=CARTESIAN_POINT('Ctrl Pts',(-8.62421402877481,15.2,6.84418217945389));
#247393=CARTESIAN_POINT('Ctrl Pts',(-8.62909316242302,15.2,6.84579515411761));
#247394=CARTESIAN_POINT('Ctrl Pts',(-8.63399647786476,15.2,6.84740511894931));
#247395=CARTESIAN_POINT('Ctrl Pts',(-8.6389238393945,15.2,6.84901186922683));
#247396=CARTESIAN_POINT('Ctrl Pts',(-8.64286572829605,15.2,6.85029726934376));
#247397=CARTESIAN_POINT('Ctrl Pts',(-8.6468230057178,15.2,6.85158061243038));
#247398=CARTESIAN_POINT('Ctrl Pts',(-8.65079560472538,15.2,6.85286179460357));
#247399=CARTESIAN_POINT('Ctrl Pts',(-8.65476820427422,15.2,6.85414297695131));
#247400=CARTESIAN_POINT('Ctrl Pts',(-8.65875612554205,15.2,6.8554219991993));
#247401=CARTESIAN_POINT('Ctrl Pts',(-8.66275929857264,15.2,6.85669875894358));
#247402=CARTESIAN_POINT('Ctrl Pts',(-8.66876405757309,15.2,6.85861389838604));
#247403=CARTESIAN_POINT('Ctrl Pts',(-8.67480313625397,15.2,6.86052394531918));
#247404=CARTESIAN_POINT('Ctrl Pts',(-8.68087630303333,15.2,6.86242856275));
#247405=CARTESIAN_POINT('Ctrl Pts',(-8.684925081254,15.2,6.86369830781921));
#247406=CARTESIAN_POINT('Ctrl Pts',(-8.68898900988754,15.2,6.86496563867979));
#247407=CARTESIAN_POINT('Ctrl Pts',(-8.69306802266692,15.2,6.86623045691512));
#247408=CARTESIAN_POINT('Ctrl Pts',(-8.6981667878075,15.2,6.86781147945079));
#247409=CARTESIAN_POINT('Ctrl Pts',(-8.70328911886753,15.2,6.86938857400425));
#247410=CARTESIAN_POINT('Ctrl Pts',(-8.7084348865686,15.2,6.87096155077758));
#247411=CARTESIAN_POINT('Ctrl Pts',(-8.71460980881948,15.2,6.87284912321417));
#247412=CARTESIAN_POINT('Ctrl Pts',(-8.72081847705701,15.2,6.87473076365857));
#247413=CARTESIAN_POINT('Ctrl Pts',(-8.72706066831535,15.2,6.87660614534385));
#247414=CARTESIAN_POINT('Ctrl Pts',(-8.73122212858724,15.2,6.87785639963035));
#247415=CARTESIAN_POINT('Ctrl Pts',(-8.73539848625421,15.2,6.87910387299203));
#247416=CARTESIAN_POINT('Ctrl Pts',(-8.73958967667525,15.2,6.88034846928605));
#247417=CARTESIAN_POINT('Ctrl Pts',(-8.74378086766732,15.2,6.88159306574964));
#247418=CARTESIAN_POINT('Ctrl Pts',(-8.7479868885392,15.2,6.88283478468114));
#247419=CARTESIAN_POINT('Ctrl Pts',(-8.75220767660352,15.2,6.88407353235957));
#247420=CARTESIAN_POINT('Ctrl Pts',(-8.75642846409276,15.2,6.88531227986922));
#247421=CARTESIAN_POINT('Ctrl Pts',(-8.76066401522073,15.2,6.88654805429891));
#247422=CARTESIAN_POINT('Ctrl Pts',(-8.76491426553842,15.2,6.88778076453178));
#247423=CARTESIAN_POINT('Ctrl Pts',(-8.7691645164352,15.2,6.88901347493261));
#247424=CARTESIAN_POINT('Ctrl Pts',(-8.77342946651131,15.2,6.89024311897565));
#247425=CARTESIAN_POINT('Ctrl Pts',(-8.77770904998625,15.2,6.8914696059925));
#247426=CARTESIAN_POINT('Ctrl Pts',(-8.78091873730091,15.2,6.89238947117158));
#247427=CARTESIAN_POINT('Ctrl Pts',(-8.78413665514967,15.2,6.89330755927829));
#247428=CARTESIAN_POINT('Ctrl Pts',(-8.78736277646374,15.2,6.89422383249916));
#247429=CARTESIAN_POINT('Ctrl Pts',(-8.7905888977778,15.2,6.89514010572004));
#247430=CARTESIAN_POINT('Ctrl Pts',(-8.79382322154856,15.2,6.89605456391682));
#247431=CARTESIAN_POINT('Ctrl Pts',(-8.79706572138837,15.2,6.89696716767549));
#247432=CARTESIAN_POINT('Ctrl Pts',(-8.80138905490083,15.2,6.89818397279758));
#247433=CARTESIAN_POINT('Ctrl Pts',(-8.80572692283445,15.2,6.89939748297205));
#247434=CARTESIAN_POINT('Ctrl Pts',(-8.81007925907261,15.2,6.90060760681556));
#247435=CARTESIAN_POINT('Ctrl Pts',(-8.81334351095472,15.2,6.90151519961575));
#247436=CARTESIAN_POINT('Ctrl Pts',(-8.81661590167391,15.2,6.90242088807956));
#247437=CARTESIAN_POINT('Ctrl Pts',(-8.81989640398631,15.2,6.90332463380082));
#247438=CARTESIAN_POINT('Ctrl Pts',(-8.82427040687088,15.2,6.90452962804111));
#247439=CARTESIAN_POINT('Ctrl Pts',(-8.82865882807488,15.2,6.9057311691128));
#247440=CARTESIAN_POINT('Ctrl Pts',(-8.83306160504682,15.2,6.90692916757079));
#247441=CARTESIAN_POINT('Ctrl Pts',(-8.83636368852562,15.2,6.90782766661832));
#247442=CARTESIAN_POINT('Ctrl Pts',(-8.8396738473567,15.2,6.90872417389861));
#247443=CARTESIAN_POINT('Ctrl Pts',(-8.84299205196505,15.2,6.90961865094499));
#247444=CARTESIAN_POINT('Ctrl Pts',(-8.8463102559706,15.2,6.91051312782888));
#247445=CARTESIAN_POINT('Ctrl Pts',(-8.84963650810069,15.2,6.91140557597954));
#247446=CARTESIAN_POINT('Ctrl Pts',(-8.85297077910524,15.2,6.91229595682202));
#247447=CARTESIAN_POINT('Ctrl Pts',(-8.85630505010979,15.2,6.91318633766449));
#247448=CARTESIAN_POINT('Ctrl Pts',(-8.85964734252619,15.2,6.91407465199566));
#247449=CARTESIAN_POINT('Ctrl Pts',(-8.86299762600305,15.2,6.91496086371747));
#247450=CARTESIAN_POINT('Ctrl Pts',(-8.86634790947992,15.2,6.91584707543929));
#247451=CARTESIAN_POINT('Ctrl Pts',(-8.86970618638733,15.2,6.91673118347723));
#247452=CARTESIAN_POINT('Ctrl Pts',(-8.87307242828028,15.2,6.91761315228253));
#247453=CARTESIAN_POINT('Ctrl Pts',(-8.87643867017324,15.2,6.91849512108784));
#247454=CARTESIAN_POINT('Ctrl Pts',(-8.87981287722173,15.2,6.91937495131933));
#247455=CARTESIAN_POINT('Ctrl Pts',(-8.88319502263981,15.2,6.92025260516263));
#247456=CARTESIAN_POINT('Ctrl Pts',(-8.88657716805789,15.2,6.92113025900594));
#247457=CARTESIAN_POINT('Ctrl Pts',(-8.88996725261712,15.2,6.92200573684105));
#247458=CARTESIAN_POINT('Ctrl Pts',(-8.89336524753424,15.2,6.92287900451796));
#247459=CARTESIAN_POINT('Ctrl Pts',(-8.89676324306866,15.2,6.9237522723535));
#247460=CARTESIAN_POINT('Ctrl Pts',(-8.900169149947,15.2,6.9246233273301));
#247461=CARTESIAN_POINT('Ctrl Pts',(-8.90358294052755,15.2,6.92549213670606));
#247462=CARTESIAN_POINT('Ctrl Pts',(-8.90927259004805,15.2,6.92694015196439));
#247463=CARTESIAN_POINT('Ctrl Pts',(-8.91498414095459,15.2,6.92838192553484));
#247464=CARTESIAN_POINT('Ctrl Pts',(-8.92071746775842,15.2,6.92981729433725));
#247465=CARTESIAN_POINT('Ctrl Pts',(-8.9253041299514,15.2,6.93096558956692));
#247466=CARTESIAN_POINT('Ctrl Pts',(-8.92990472886795,15.2,6.93210978655176));
#247467=CARTESIAN_POINT('Ctrl Pts',(-8.93451920050833,15.2,6.93324980122501));
#247468=CARTESIAN_POINT('Ctrl Pts',(-8.93798005392426,15.2,6.93410481215228));
#247469=CARTESIAN_POINT('Ctrl Pts',(-8.94144871094819,15.2,6.9349574722713));
#247470=CARTESIAN_POINT('Ctrl Pts',(-8.94492514486286,15.2,6.93580774515728));
#247471=CARTESIAN_POINT('Ctrl Pts',(-8.94956039050346,15.2,6.93694144244157));
#247472=CARTESIAN_POINT('Ctrl Pts',(-8.95420946170408,15.2,6.93807089727257));
#247473=CARTESIAN_POINT('Ctrl Pts',(-8.95887229518132,15.2,6.93919602783361));
#247474=CARTESIAN_POINT('Ctrl Pts',(-8.96353512802323,15.2,6.94032115824135));
#247475=CARTESIAN_POINT('Ctrl Pts',(-8.96821172260313,15.2,6.94144196610087));
#247476=CARTESIAN_POINT('Ctrl Pts',(-8.97290201711949,15.2,6.94255836862131));
#247477=CARTESIAN_POINT('Ctrl Pts',(-8.97641973816652,15.2,6.94339567054968));
#247478=CARTESIAN_POINT('Ctrl Pts',(-8.97994516412586,15.2,6.94423049524845));
#247479=CARTESIAN_POINT('Ctrl Pts',(-8.98347826999646,15.2,6.94506280909356));
#247480=CARTESIAN_POINT('Ctrl Pts',(-8.9870113765089,15.2,6.94589512308986));
#247481=CARTESIAN_POINT('Ctrl Pts',(-8.99055216197349,15.2,6.9467249254438));
#247482=CARTESIAN_POINT('Ctrl Pts',(-8.99410060049023,15.2,6.94755218439701));
#247483=CARTESIAN_POINT('Ctrl Pts',(-8.9988318507715,15.2,6.94865519608415));
#247484=CARTESIAN_POINT('Ctrl Pts',(-9.00357670535378,15.2,6.94975368340521));
#247485=CARTESIAN_POINT('Ctrl Pts',(-9.0083351023528,15.2,6.95084757042721));
#247486=CARTESIAN_POINT('Ctrl Pts',(-9.01190390026415,15.2,6.95166798573096));
#247487=CARTESIAN_POINT('Ctrl Pts',(-9.01548031645871,15.2,6.95248581214751));
#247488=CARTESIAN_POINT('Ctrl Pts',(-9.01906432354832,15.2,6.95330101707559));
#247489=CARTESIAN_POINT('Ctrl Pts',(-9.02264833063795,15.2,6.95411622200366));
#247490=CARTESIAN_POINT('Ctrl Pts',(-9.02623992878052,15.2,6.95492880626917));
#247491=CARTESIAN_POINT('Ctrl Pts',(-9.02983909119039,15.2,6.9557387361151));
#247492=CARTESIAN_POINT('Ctrl Pts',(-9.0334382542541,15.2,6.95654866610817));
#247493=CARTESIAN_POINT('Ctrl Pts',(-9.03704498226163,15.2,6.95735594164217));
#247494=CARTESIAN_POINT('Ctrl Pts',(-9.04065924928792,15.2,6.95816053121707));
#247495=CARTESIAN_POINT('Ctrl Pts',(-9.04427351565762,15.2,6.9589651206458));
#247496=CARTESIAN_POINT('Ctrl Pts',(-9.04789532072694,15.2,6.95976702444967));
#247497=CARTESIAN_POINT('Ctrl Pts',(-9.05152463863739,15.2,6.9605662102954));
#247498=CARTESIAN_POINT('Ctrl Pts',(-9.05515395654783,15.2,6.96136539614112));
#247499=CARTESIAN_POINT('Ctrl Pts',(-9.05879078785248,15.2,6.96216186300931));
#247500=CARTESIAN_POINT('Ctrl Pts',(-9.06243510473666,15.2,6.96295558073406));
#247501=CARTESIAN_POINT('Ctrl Pts',(-9.06607942162084,15.2,6.96374929845882));
#247502=CARTESIAN_POINT('Ctrl Pts',(-9.06973122401306,15.2,6.96454026435767));
#247503=CARTESIAN_POINT('Ctrl Pts',(-9.07339048548002,15.2,6.96532844724929));
#247504=CARTESIAN_POINT('Ctrl Pts',(-9.07704974694698,15.2,6.96611663014091));
#247505=CARTESIAN_POINT('Ctrl Pts',(-9.08071646885045,15.2,6.96690203044285));
#247506=CARTESIAN_POINT('Ctrl Pts',(-9.08439062484131,15.2,6.96768461795632));
#247507=CARTESIAN_POINT('Ctrl Pts',(-9.08806478083216,15.2,6.9684672054698));
#247508=CARTESIAN_POINT('Ctrl Pts',(-9.09174637294751,15.2,6.96924698222514));
#247509=CARTESIAN_POINT('Ctrl Pts',(-9.09543537618747,15.2,6.9700239170723));
#247510=CARTESIAN_POINT('Ctrl Pts',(-9.09912438009759,15.2,6.97080085206061));
#247511=CARTESIAN_POINT('Ctrl Pts',(-9.10282079320149,15.2,6.9715749445731));
#247512=CARTESIAN_POINT('Ctrl Pts',(-9.10652458657411,15.2,6.97234615839313));
#247513=CARTESIAN_POINT('Ctrl Pts',(-9.11022837927387,15.2,6.97311737207304));
#247514=CARTESIAN_POINT('Ctrl Pts',(-9.11393954980134,15.2,6.97388570408798));
#247515=CARTESIAN_POINT('Ctrl Pts',(-9.11765807097785,15.2,6.9746511226814));
#247516=CARTESIAN_POINT('Ctrl Pts',(-9.12137659215437,15.2,6.97541654127482));
#247517=CARTESIAN_POINT('Ctrl Pts',(-9.12510246390719,15.2,6.97617904686198));
#247518=CARTESIAN_POINT('Ctrl Pts',(-9.1288356732116,15.2,6.97693862333241));
#247519=CARTESIAN_POINT('Ctrl Pts',(-9.13256888251601,15.2,6.97769819980284));
#247520=CARTESIAN_POINT('Ctrl Pts',(-9.13630942931919,15.2,6.97845485086305));
#247521=CARTESIAN_POINT('Ctrl Pts',(-9.14005731500006,15.2,6.97920857099999));
#247522=CARTESIAN_POINT('Ctrl Pts',(-8.02901631900006,12.2,6.57080831899999));
#247523=CARTESIAN_POINT('Ctrl Pts',(-8.03049110446229,12.2,6.57181685366614));
#247524=CARTESIAN_POINT('Ctrl Pts',(-8.0320161093278,12.2,6.57285322826574));
#247525=CARTESIAN_POINT('Ctrl Pts',(-8.03359089408583,12.2,6.57391635240017));
#247526=CARTESIAN_POINT('Ctrl Pts',(-8.03517327325199,12.2,6.57498460345654));
#247527=CARTESIAN_POINT('Ctrl Pts',(-8.03680591570089,12.2,6.57607986594818));
#247528=CARTESIAN_POINT('Ctrl Pts',(-8.03848839087952,12.2,6.57720107915013));
#247529=CARTESIAN_POINT('Ctrl Pts',(-8.04017086590532,12.2,6.57832229225026));
#247530=CARTESIAN_POINT('Ctrl Pts',(-8.04190317283137,12.2,6.57946945464252));
#247531=CARTESIAN_POINT('Ctrl Pts',(-8.04368489176663,12.2,6.58064153793327));
#247532=CARTESIAN_POINT('Ctrl Pts',(-8.04546661070189,12.2,6.58181362122402));
#247533=CARTESIAN_POINT('Ctrl Pts',(-8.04729774128707,12.2,6.58301062651662));
#247534=CARTESIAN_POINT('Ctrl Pts',(-8.04917787055988,12.2,6.58423155119856));
#247535=CARTESIAN_POINT('Ctrl Pts',(-8.05105800000347,12.2,6.58545247599141));
#247536=CARTESIAN_POINT('Ctrl Pts',(-8.05298713099614,12.2,6.58669732359249));
#247537=CARTESIAN_POINT('Ctrl Pts',(-8.05496485719055,12.2,6.58796512041314));
#247538=CARTESIAN_POINT('Ctrl Pts',(-8.05694258320533,12.2,6.58923291711864));
#247539=CARTESIAN_POINT('Ctrl Pts',(-8.05896890538341,12.2,6.59052366630055));
#247540=CARTESIAN_POINT('Ctrl Pts',(-8.06104342948425,12.2,6.59183642200888));
#247541=CARTESIAN_POINT('Ctrl Pts',(-8.06311795358509,12.2,6.59314917771721));
#247542=CARTESIAN_POINT('Ctrl Pts',(-8.0652406808045,12.2,6.59448394076801));
#247543=CARTESIAN_POINT('Ctrl Pts',(-8.06741122014022,12.2,6.59583979646781));
#247544=CARTESIAN_POINT('Ctrl Pts',(-8.06958175967308,12.2,6.59719565229079));
#247545=CARTESIAN_POINT('Ctrl Pts',(-8.0718001153119,12.2,6.5985725970414));
#247546=CARTESIAN_POINT('Ctrl Pts',(-8.07406590652196,12.2,6.59996974311891));
#247547=CARTESIAN_POINT('Ctrl Pts',(-8.0763316975262,12.2,6.60136688906953));
#247548=CARTESIAN_POINT('Ctrl Pts',(-8.07864492271251,12.2,6.60278423372136));
#247549=CARTESIAN_POINT('Ctrl Pts',(-8.0810052091288,12.2,6.60422091158666));
#247550=CARTESIAN_POINT('Ctrl Pts',(-8.08336549554508,12.2,6.60565758945196));
#247551=CARTESIAN_POINT('Ctrl Pts',(-8.08577284749928,12.2,6.60711359814904));
#247552=CARTESIAN_POINT('Ctrl Pts',(-8.08822689382476,12.2,6.608588095178));
#247553=CARTESIAN_POINT('Ctrl Pts',(-8.09068094015023,12.2,6.61006259220696));
#247554=CARTESIAN_POINT('Ctrl Pts',(-8.09318168323473,12.2,6.6115555767414));
#247555=CARTESIAN_POINT('Ctrl Pts',(-8.09572876447236,12.2,6.61306622685197));
#247556=CARTESIAN_POINT('Ctrl Pts',(-8.09827584594135,12.2,6.61457687709976));
#247557=CARTESIAN_POINT('Ctrl Pts',(-8.10086926266482,12.2,6.61610519104097));
#247558=CARTESIAN_POINT('Ctrl Pts',(-8.10350866514402,12.2,6.61765037037591));
#247559=CARTESIAN_POINT('Ctrl Pts',(-8.10614806738348,12.2,6.61919554957051));
#247560=CARTESIAN_POINT('Ctrl Pts',(-8.10883345256066,12.2,6.62075759004112));
#247561=CARTESIAN_POINT('Ctrl Pts',(-8.11156447572374,12.2,6.62233571524091));
#247562=CARTESIAN_POINT('Ctrl Pts',(-8.11429549888682,12.2,6.6239138404407));
#247563=CARTESIAN_POINT('Ctrl Pts',(-8.11707215754802,12.2,6.62550804702571));
#247564=CARTESIAN_POINT('Ctrl Pts',(-8.1198941109424,12.2,6.62711757454952));
#247565=CARTESIAN_POINT('Ctrl Pts',(-8.1227160645931,12.2,6.62872710221953));
#247566=CARTESIAN_POINT('Ctrl Pts',(-8.12558331343989,12.2,6.63035195259939));
#247567=CARTESIAN_POINT('Ctrl Pts',(-8.12849552018388,12.2,6.63199137835604));
#247568=CARTESIAN_POINT('Ctrl Pts',(-8.13140772666334,12.2,6.63363080396375));
#247569=CARTESIAN_POINT('Ctrl Pts',(-8.13436489186082,12.2,6.63528480756059));
#247570=CARTESIAN_POINT('Ctrl Pts',(-8.13736668326528,12.2,6.63695266325754));
#247571=CARTESIAN_POINT('Ctrl Pts',(-8.14036847466976,12.2,6.63862051895448));
#247572=CARTESIAN_POINT('Ctrl Pts',(-8.14341489333673,12.2,6.6403022281027));
#247573=CARTESIAN_POINT('Ctrl Pts',(-8.14650561163811,12.2,6.64199708079023));
#247574=CARTESIAN_POINT('Ctrl Pts',(-8.14959633022023,12.2,6.64369193363172));
#247575=CARTESIAN_POINT('Ctrl Pts',(-8.15273134875633,12.2,6.64539993184432));
#247576=CARTESIAN_POINT('Ctrl Pts',(-8.15591034659093,12.2,6.64712038194142));
#247577=CARTESIAN_POINT('Ctrl Pts',(-8.15908934413677,12.2,6.64884083188224));
#247578=CARTESIAN_POINT('Ctrl Pts',(-8.16231231977698,12.2,6.65057373567168));
#247579=CARTESIAN_POINT('Ctrl Pts',(-8.16557895524163,12.2,6.65231841652496));
#247580=CARTESIAN_POINT('Ctrl Pts',(-8.16884559070627,12.2,6.65406309737823));
#247581=CARTESIAN_POINT('Ctrl Pts',(-8.17215588738246,12.2,6.65581955514721));
#247582=CARTESIAN_POINT('Ctrl Pts',(-8.17550953292566,12.2,6.65758713108734));
#247583=CARTESIAN_POINT('Ctrl Pts',(-8.17886317877349,12.2,6.65935470718801));
#247584=CARTESIAN_POINT('Ctrl Pts',(-8.18226017247621,12.2,6.66113340036344));
#247585=CARTESIAN_POINT('Ctrl Pts',(-8.18570020341661,12.2,6.66292256646165));
#247586=CARTESIAN_POINT('Ctrl Pts',(-8.18914023404453,12.2,6.66471173239735));
#247587=CARTESIAN_POINT('Ctrl Pts',(-8.19262330516359,12.2,6.66651136899997));
#247588=CARTESIAN_POINT('Ctrl Pts',(-8.19614910871825,12.2,6.66832084802579));
#247589=CARTESIAN_POINT('Ctrl Pts',(-8.19967491227291,12.2,6.67013032705162));
#247590=CARTESIAN_POINT('Ctrl Pts',(-8.20324345005308,12.2,6.6719496470672));
#247591=CARTESIAN_POINT('Ctrl Pts',(-8.20685441958671,12.2,6.67377819116703));
#247592=CARTESIAN_POINT('Ctrl Pts',(-8.20986356097406,12.2,6.67530197797225));
#247593=CARTESIAN_POINT('Ctrl Pts',(-8.21290216901772,12.2,6.6768321706943));
#247594=CARTESIAN_POINT('Ctrl Pts',(-8.21597007276618,12.2,6.6783684191662));
#247595=CARTESIAN_POINT('Ctrl Pts',(-8.21903797651465,12.2,6.6799046676381));
#247596=CARTESIAN_POINT('Ctrl Pts',(-8.22213517478972,12.2,6.68144697153656));
#247597=CARTESIAN_POINT('Ctrl Pts',(-8.22526149549828,12.2,6.68299498751579));
#247598=CARTESIAN_POINT('Ctrl Pts',(-8.22838781620684,12.2,6.68454300349503));
#247599=CARTESIAN_POINT('Ctrl Pts',(-8.23154326289995,12.2,6.68609673124996));
#247600=CARTESIAN_POINT('Ctrl Pts',(-8.23472766269165,12.2,6.68765583249997));
#247601=CARTESIAN_POINT('Ctrl Pts',(-8.23791206248333,12.2,6.68921493374999));
#247602=CARTESIAN_POINT('Ctrl Pts',(-8.24112541823138,12.2,6.6907794107159));
#247603=CARTESIAN_POINT('Ctrl Pts',(-8.24436756046842,12.2,6.69234892850083));
#247604=CARTESIAN_POINT('Ctrl Pts',(-8.24760970270545,12.2,6.69391844628575));
#247605=CARTESIAN_POINT('Ctrl Pts',(-8.25088063221447,12.2,6.69549300605304));
#247606=CARTESIAN_POINT('Ctrl Pts',(-8.25418018346594,12.2,6.69707228209495));
#247607=CARTESIAN_POINT('Ctrl Pts',(-8.25747973471739,12.2,6.69865155813684));
#247608=CARTESIAN_POINT('Ctrl Pts',(-8.26080790682374,12.2,6.70023554983142));
#247609=CARTESIAN_POINT('Ctrl Pts',(-8.26416453647801,12.2,6.70182393684555));
#247610=CARTESIAN_POINT('Ctrl Pts',(-8.26752116613229,12.2,6.70341232385966));
#247611=CARTESIAN_POINT('Ctrl Pts',(-8.27090625118495,12.2,6.70500510523308));
#247612=CARTESIAN_POINT('Ctrl Pts',(-8.27431963191299,12.2,6.70660196816036));
#247613=CARTESIAN_POINT('Ctrl Pts',(-8.27773301264105,12.2,6.70819883108764));
#247614=CARTESIAN_POINT('Ctrl Pts',(-8.28117468674043,12.2,6.70979977275957));
#247615=CARTESIAN_POINT('Ctrl Pts',(-8.28464449243718,12.2,6.71140448567654));
#247616=CARTESIAN_POINT('Ctrl Pts',(-8.28811429813392,12.2,6.71300919859351));
#247617=CARTESIAN_POINT('Ctrl Pts',(-8.2916122377867,12.2,6.71461768115499));
#247618=CARTESIAN_POINT('Ctrl Pts',(-8.29513814771951,12.2,6.71622962921083));
#247619=CARTESIAN_POINT('Ctrl Pts',(-8.29866405726801,12.2,6.71784157709094));
#247620=CARTESIAN_POINT('Ctrl Pts',(-8.3022179412742,12.2,6.71945699038162));
#247621=CARTESIAN_POINT('Ctrl Pts',(-8.30579963650651,12.2,6.72107556978827));
#247622=CARTESIAN_POINT('Ctrl Pts',(-8.30938133212924,12.2,6.72269414937134));
#247623=CARTESIAN_POINT('Ctrl Pts',(-8.3129908415932,12.2,6.72431589348772));
#247624=CARTESIAN_POINT('Ctrl Pts',(-8.31662800700758,12.2,6.72594050827915));
#247625=CARTESIAN_POINT('Ctrl Pts',(-8.32099260574272,12.2,6.7278900461351));
#247626=CARTESIAN_POINT('Ctrl Pts',(-8.32539702749008,12.2,6.72984371952484));
#247627=CARTESIAN_POINT('Ctrl Pts',(-8.32984100348402,12.2,6.73180102438167));
#247628=CARTESIAN_POINT('Ctrl Pts',(-8.33354431661046,12.2,6.73343211167347));
#247629=CARTESIAN_POINT('Ctrl Pts',(-8.33727509821339,12.2,6.7350657214969));
#247630=CARTESIAN_POINT('Ctrl Pts',(-8.34103319319468,12.2,6.73670157123155));
#247631=CARTESIAN_POINT('Ctrl Pts',(-8.34479128817596,12.2,6.73833742096621));
#247632=CARTESIAN_POINT('Ctrl Pts',(-8.34857669656313,12.2,6.73997550786434));
#247633=CARTESIAN_POINT('Ctrl Pts',(-8.35238926323202,12.2,6.7416155534895));
#247634=CARTESIAN_POINT('Ctrl Pts',(-8.35543931631778,12.2,6.74292758988237));
#247635=CARTESIAN_POINT('Ctrl Pts',(-8.35850675374851,12.2,6.74424087936118));
#247636=CARTESIAN_POINT('Ctrl Pts',(-8.36159149277297,12.2,6.74555528114254));
#247637=CARTESIAN_POINT('Ctrl Pts',(-8.36467623221773,12.2,6.74686968310298));
#247638=CARTESIAN_POINT('Ctrl Pts',(-8.36777827644761,12.2,6.74818519751453));
#247639=CARTESIAN_POINT('Ctrl Pts',(-8.37089754721938,12.2,6.74950168420768));
#247640=CARTESIAN_POINT('Ctrl Pts',(-8.37401681756615,12.2,6.75081817072147));
#247641=CARTESIAN_POINT('Ctrl Pts',(-8.37715331341794,12.2,6.75213562919726));
#247642=CARTESIAN_POINT('Ctrl Pts',(-8.38030695782567,12.2,6.75345392236722));
#247643=CARTESIAN_POINT('Ctrl Pts',(-8.38346060266309,12.2,6.75477221571679));
#247644=CARTESIAN_POINT('Ctrl Pts',(-8.38663139731092,12.2,6.7560913438637));
#247645=CARTESIAN_POINT('Ctrl Pts',(-8.38981926331909,12.2,6.75741116982455));
#247646=CARTESIAN_POINT('Ctrl Pts',(-8.39300712889291,12.2,6.75873099560558));
#247647=CARTESIAN_POINT('Ctrl Pts',(-8.3962120667809,12.2,6.76005152021978));
#247648=CARTESIAN_POINT('Ctrl Pts',(-8.3994340005659,12.2,6.76137260756663));
#247649=CARTESIAN_POINT('Ctrl Pts',(-8.40265593478988,12.2,6.76269369509347));
#247650=CARTESIAN_POINT('Ctrl Pts',(-8.40589486450167,12.2,6.76401534691654));
#247651=CARTESIAN_POINT('Ctrl Pts',(-8.40915071329132,12.2,6.76533742959974));
#247652=CARTESIAN_POINT('Ctrl Pts',(-8.41240656163736,12.2,6.76665951210279));
#247653=CARTESIAN_POINT('Ctrl Pts',(-8.41567933019394,12.2,6.76798202541133));
#247654=CARTESIAN_POINT('Ctrl Pts',(-8.41896894247882,12.2,6.76930483802538));
#247655=CARTESIAN_POINT('Ctrl Pts',(-8.42225855521192,12.2,6.77062765081966));
#247656=CARTESIAN_POINT('Ctrl Pts',(-8.42556501193377,12.2,6.77195076375331));
#247657=CARTESIAN_POINT('Ctrl Pts',(-8.42888823801892,12.2,6.77327404577588));
#247658=CARTESIAN_POINT('Ctrl Pts',(-8.43221146365128,12.2,6.77459732761816));
#247659=CARTESIAN_POINT('Ctrl Pts',(-8.43555145857452,12.2,6.77592077954181));
#247660=CARTESIAN_POINT('Ctrl Pts',(-8.43890814624284,12.2,6.77724427276693));
#247661=CARTESIAN_POINT('Ctrl Pts',(-8.44226483436849,12.2,6.77856776617238));
#247662=CARTESIAN_POINT('Ctrl Pts',(-8.44563821710689,12.2,6.77989130153064));
#247663=CARTESIAN_POINT('Ctrl Pts',(-8.44902821979165,12.2,6.78121475099165));
#247664=CARTESIAN_POINT('Ctrl Pts',(-8.45241822247642,12.2,6.78253820045268));
#247665=CARTESIAN_POINT('Ctrl Pts',(-8.455824844552,12.2,6.78386156533035));
#247666=CARTESIAN_POINT('Ctrl Pts',(-8.45924801201803,12.2,6.78518471945799));
#247667=CARTESIAN_POINT('Ctrl Pts',(-8.46267117901766,12.2,6.78650787340536));
#247668=CARTESIAN_POINT('Ctrl Pts',(-8.46611089233953,12.2,6.78783081555953));
#247669=CARTESIAN_POINT('Ctrl Pts',(-8.46956707723931,12.2,6.78915342595742));
#247670=CARTESIAN_POINT('Ctrl Pts',(-8.47302326261,12.2,6.79047603653552));
#247671=CARTESIAN_POINT('Ctrl Pts',(-8.47649591952865,12.2,6.7917983109969));
#247672=CARTESIAN_POINT('Ctrl Pts',(-8.4799849750538,12.2,6.79312013045777));
#247673=CARTESIAN_POINT('Ctrl Pts',(-8.48347403010358,12.2,6.79444194973855));
#247674=CARTESIAN_POINT('Ctrl Pts',(-8.48697948512065,12.2,6.79576331253883));
#247675=CARTESIAN_POINT('Ctrl Pts',(-8.49050126422058,12.2,6.79708409787534));
#247676=CARTESIAN_POINT('Ctrl Pts',(-8.49402304380035,12.2,6.79840488339181));
#247677=CARTESIAN_POINT('Ctrl Pts',(-8.49756114951816,12.2,6.79972509047035));
#247678=CARTESIAN_POINT('Ctrl Pts',(-8.50111550905751,12.2,6.80104460194146));
#247679=CARTESIAN_POINT('Ctrl Pts',(-8.50466986811258,12.2,6.80236411323277));
#247680=CARTESIAN_POINT('Ctrl Pts',(-8.50824047944563,12.2,6.80368292767492));
#247681=CARTESIAN_POINT('Ctrl Pts',(-8.51182727170693,12.2,6.80500092640057));
#247682=CARTESIAN_POINT('Ctrl Pts',(-8.51541406445691,12.2,6.80631892530578));
#247683=CARTESIAN_POINT('Ctrl Pts',(-8.51901703872827,12.2,6.80763610999146));
#247684=CARTESIAN_POINT('Ctrl Pts',(-8.52263612153768,12.2,6.80895236284092));
#247685=CARTESIAN_POINT('Ctrl Pts',(-8.52625520385399,12.2,6.81026861551103));
#247686=CARTESIAN_POINT('Ctrl Pts',(-8.52989039448496,12.2,6.81158393445375));
#247687=CARTESIAN_POINT('Ctrl Pts',(-8.53354162297859,12.2,6.81289820780094));
#247688=CARTESIAN_POINT('Ctrl Pts',(-8.53810565896874,12.2,6.81454104961924));
#247689=CARTESIAN_POINT('Ctrl Pts',(-8.54269475415526,12.2,6.8161822551149));
#247690=CARTESIAN_POINT('Ctrl Pts',(-8.54730876672338,12.2,6.81782160039276));
#247691=CARTESIAN_POINT('Ctrl Pts',(-8.55099997697905,12.2,6.81913307668653));
#247692=CARTESIAN_POINT('Ctrl Pts',(-8.55470713661169,12.2,6.82044336419962));
#247693=CARTESIAN_POINT('Ctrl Pts',(-8.55843017337117,12.2,6.82175234788199));
#247694=CARTESIAN_POINT('Ctrl Pts',(-8.56215320962339,12.2,6.823061331386));
#247695=CARTESIAN_POINT('Ctrl Pts',(-8.56589212223155,12.2,6.82436901362683));
#247696=CARTESIAN_POINT('Ctrl Pts',(-8.56964684322191,12.2,6.82567528108543));
#247697=CARTESIAN_POINT('Ctrl Pts',(-8.57340156472385,12.2,6.826981548722));
#247698=CARTESIAN_POINT('Ctrl Pts',(-8.5771720910773,12.2,6.82828640220504));
#247699=CARTESIAN_POINT('Ctrl Pts',(-8.58095835578467,12.2,6.82958973233152));
#247700=CARTESIAN_POINT('Ctrl Pts',(-8.58474461997617,12.2,6.83089306228044));
#247701=CARTESIAN_POINT('Ctrl Pts',(-8.5885466186145,12.2,6.83219486754353));
#247702=CARTESIAN_POINT('Ctrl Pts',(-8.59236428613413,12.2,6.83349503977074));
#247703=CARTESIAN_POINT('Ctrl Pts',(-8.59618195417391,12.2,6.83479521217509));
#247704=CARTESIAN_POINT('Ctrl Pts',(-8.60001528748467,12.2,6.83609375163766));
#247705=CARTESIAN_POINT('Ctrl Pts',(-8.60386421824999,12.2,6.83739055054166));
#247706=CARTESIAN_POINT('Ctrl Pts',(-8.60771314901532,12.2,6.83868734944567));
#247707=CARTESIAN_POINT('Ctrl Pts',(-8.61157767611857,12.2,6.83998240684948));
#247708=CARTESIAN_POINT('Ctrl Pts',(-8.61545773160939,12.2,6.8412756177531));
#247709=CARTESIAN_POINT('Ctrl Pts',(-8.61933778657157,12.2,6.84256882848053));
#247710=CARTESIAN_POINT('Ctrl Pts',(-8.62323336839101,12.2,6.84386019109311));
#247711=CARTESIAN_POINT('Ctrl Pts',(-8.62714440925567,12.2,6.84514960121578));
#247712=CARTESIAN_POINT('Ctrl Pts',(-8.6310554506532,12.2,6.84643901151414));
#247713=CARTESIAN_POINT('Ctrl Pts',(-8.63498194995588,12.2,6.84772646893476));
#247714=CARTESIAN_POINT('Ctrl Pts',(-8.6389238393945,12.2,6.84901186922683));
#247715=CARTESIAN_POINT('Ctrl Pts',(-8.64286572829605,12.2,6.85029726934376));
#247716=CARTESIAN_POINT('Ctrl Pts',(-8.6468230057178,12.2,6.85158061243038));
#247717=CARTESIAN_POINT('Ctrl Pts',(-8.65079560472538,12.2,6.85286179460357));
#247718=CARTESIAN_POINT('Ctrl Pts',(-8.65675450350738,12.2,6.85478356795062));
#247719=CARTESIAN_POINT('Ctrl Pts',(-8.66274787400597,12.2,6.85670048076072));
#247720=CARTESIAN_POINT('Ctrl Pts',(-8.66877548753467,12.2,6.85861218802495));
#247721=CARTESIAN_POINT('Ctrl Pts',(-8.67279389691878,12.2,6.8598866596502));
#247722=CARTESIAN_POINT('Ctrl Pts',(-8.67682752481266,12.2,6.86115881768079));
#247723=CARTESIAN_POINT('Ctrl Pts',(-8.68087630303333,12.2,6.86242856275));
#247724=CARTESIAN_POINT('Ctrl Pts',(-8.684925081254,12.2,6.86369830781921));
#247725=CARTESIAN_POINT('Ctrl Pts',(-8.68898900988754,12.2,6.86496563867979));
#247726=CARTESIAN_POINT('Ctrl Pts',(-8.69306802266692,12.2,6.86623045691512));
#247727=CARTESIAN_POINT('Ctrl Pts',(-8.6981667878075,12.2,6.86781147945079));
#247728=CARTESIAN_POINT('Ctrl Pts',(-8.70328911886753,12.2,6.86938857400426));
#247729=CARTESIAN_POINT('Ctrl Pts',(-8.70843488656861,12.2,6.87096155077758));
#247730=CARTESIAN_POINT('Ctrl Pts',(-8.71255150140253,12.2,6.87221993240198));
#247731=CARTESIAN_POINT('Ctrl Pts',(-8.71668311509067,12.2,6.87347567662893));
#247732=CARTESIAN_POINT('Ctrl Pts',(-8.72082965998333,12.2,6.874728688975));
#247733=CARTESIAN_POINT('Ctrl Pts',(-8.72497620487598,12.2,6.87598170132107));
#247734=CARTESIAN_POINT('Ctrl Pts',(-8.72913768329261,12.2,6.87723197950015));
#247735=CARTESIAN_POINT('Ctrl Pts',(-8.73331402496617,12.2,6.87847942917895));
#247736=CARTESIAN_POINT('Ctrl Pts',(-8.7374903660707,12.2,6.87972687868779));
#247737=CARTESIAN_POINT('Ctrl Pts',(-8.74168157364137,12.2,6.88097149896723));
#247738=CARTESIAN_POINT('Ctrl Pts',(-8.7458875780388,12.2,6.88221319398248));
#247739=CARTESIAN_POINT('Ctrl Pts',(-8.75009358300931,12.2,6.88345488916692));
#247740=CARTESIAN_POINT('Ctrl Pts',(-8.75431438812685,12.2,6.88469366063778));
#247741=CARTESIAN_POINT('Ctrl Pts',(-8.75854992369252,12.2,6.88592941242704));
#247742=CARTESIAN_POINT('Ctrl Pts',(-8.7627854586811,12.2,6.88716516404793));
#247743=CARTESIAN_POINT('Ctrl Pts',(-8.76703572543441,12.2,6.88839789813865));
#247744=CARTESIAN_POINT('Ctrl Pts',(-8.77130065841814,12.2,6.88962751914945));
#247745=CARTESIAN_POINT('Ctrl Pts',(-8.77449935830122,12.2,6.89054973494943));
#247746=CARTESIAN_POINT('Ctrl Pts',(-8.77770630790183,12.2,6.89147020104284));
#247747=CARTESIAN_POINT('Ctrl Pts',(-8.78092147940302,12.2,6.89238887734724));
#247748=CARTESIAN_POINT('Ctrl Pts',(-8.78413665090421,12.2,6.89330755365163));
#247749=CARTESIAN_POINT('Ctrl Pts',(-8.7873600437474,12.2,6.89422444030018));
#247750=CARTESIAN_POINT('Ctrl Pts',(-8.79059163058719,12.2,6.89513949905885));
#247751=CARTESIAN_POINT('Ctrl Pts',(-8.79382321801404,12.2,6.89605455798375));
#247752=CARTESIAN_POINT('Ctrl Pts',(-8.79706299878493,12.2,6.89696778864981));
#247753=CARTESIAN_POINT('Ctrl Pts',(-8.8003109467164,12.2,6.89787915219867));
#247754=CARTESIAN_POINT('Ctrl Pts',(-8.80355889405783,12.2,6.89879051558197));
#247755=CARTESIAN_POINT('Ctrl Pts',(-8.80681500719049,12.2,6.89970001401537));
#247756=CARTESIAN_POINT('Ctrl Pts',(-8.81007925907261,12.2,6.90060760681556));
#247757=CARTESIAN_POINT('Ctrl Pts',(-8.81443159471776,12.2,6.90181773049419));
#247758=CARTESIAN_POINT('Ctrl Pts',(-8.81879839991876,12.2,6.90302446882722));
#247759=CARTESIAN_POINT('Ctrl Pts',(-8.82317960838934,12.2,6.90422773006705));
#247760=CARTESIAN_POINT('Ctrl Pts',(-8.82646551489151,12.2,6.9051301760379));
#247761=CARTESIAN_POINT('Ctrl Pts',(-8.82975952216789,12.2,6.90603066868649));
#247762=CARTESIAN_POINT('Ctrl Pts',(-8.83306160504682,12.2,6.90692916757079));
#247763=CARTESIAN_POINT('Ctrl Pts',(-8.83636368852561,12.2,6.90782766661832));
#247764=CARTESIAN_POINT('Ctrl Pts',(-8.8396738473567,12.2,6.90872417389861));
#247765=CARTESIAN_POINT('Ctrl Pts',(-8.84299205196505,12.2,6.90961865094499));
#247766=CARTESIAN_POINT('Ctrl Pts',(-8.8463102559706,12.2,6.91051312782888));
#247767=CARTESIAN_POINT('Ctrl Pts',(-8.84963650810069,12.2,6.91140557597954));
#247768=CARTESIAN_POINT('Ctrl Pts',(-8.85297077910524,12.2,6.91229595682202));
#247769=CARTESIAN_POINT('Ctrl Pts',(-8.85630505010979,12.2,6.91318633766449));
#247770=CARTESIAN_POINT('Ctrl Pts',(-8.85964734252618,12.2,6.91407465199566));
#247771=CARTESIAN_POINT('Ctrl Pts',(-8.86299762600305,12.2,6.91496086371747));
#247772=CARTESIAN_POINT('Ctrl Pts',(-8.86634790947992,12.2,6.91584707543929));
#247773=CARTESIAN_POINT('Ctrl Pts',(-8.86970618638733,12.2,6.91673118347723));
#247774=CARTESIAN_POINT('Ctrl Pts',(-8.87307242828028,12.2,6.91761315228253));
#247775=CARTESIAN_POINT('Ctrl Pts',(-8.87643867017324,12.2,6.91849512108784));
#247776=CARTESIAN_POINT('Ctrl Pts',(-8.87981287722173,12.2,6.91937495131933));
#247777=CARTESIAN_POINT('Ctrl Pts',(-8.88319502263981,12.2,6.92025260516263));
#247778=CARTESIAN_POINT('Ctrl Pts',(-8.88657716805789,12.2,6.92113025900594));
#247779=CARTESIAN_POINT('Ctrl Pts',(-8.88996725261712,12.2,6.92200573684105));
#247780=CARTESIAN_POINT('Ctrl Pts',(-8.89336524753424,12.2,6.92287900451796));
#247781=CARTESIAN_POINT('Ctrl Pts',(-8.89676324306866,12.2,6.9237522723535));
#247782=CARTESIAN_POINT('Ctrl Pts',(-8.900169149947,12.2,6.9246233273301));
#247783=CARTESIAN_POINT('Ctrl Pts',(-8.90358294052755,12.2,6.92549213670606));
#247784=CARTESIAN_POINT('Ctrl Pts',(-8.90927259004805,12.2,6.92694015196439));
#247785=CARTESIAN_POINT('Ctrl Pts',(-8.91498414095459,12.2,6.92838192553484));
#247786=CARTESIAN_POINT('Ctrl Pts',(-8.92071746775843,12.2,6.92981729433725));
#247787=CARTESIAN_POINT('Ctrl Pts',(-8.9253041299514,12.2,6.93096558956692));
#247788=CARTESIAN_POINT('Ctrl Pts',(-8.92990472886795,12.2,6.93210978655176));
#247789=CARTESIAN_POINT('Ctrl Pts',(-8.93451920050833,12.2,6.93324980122501));
#247790=CARTESIAN_POINT('Ctrl Pts',(-8.93798005392426,12.2,6.93410481215228));
#247791=CARTESIAN_POINT('Ctrl Pts',(-8.94144871094819,12.2,6.9349574722713));
#247792=CARTESIAN_POINT('Ctrl Pts',(-8.94492514486286,12.2,6.93580774515728));
#247793=CARTESIAN_POINT('Ctrl Pts',(-8.94840157877754,12.2,6.93665801804326));
#247794=CARTESIAN_POINT('Ctrl Pts',(-8.95188578955003,12.2,6.93750590492941));
#247795=CARTESIAN_POINT('Ctrl Pts',(-8.95537775042209,12.2,6.93835137031569));
#247796=CARTESIAN_POINT('Ctrl Pts',(-8.95886971192853,12.2,6.93919683585556));
#247797=CARTESIAN_POINT('Ctrl Pts',(-8.96236942320384,12.2,6.94003988067809));
#247798=CARTESIAN_POINT('Ctrl Pts',(-8.9658768582563,12.2,6.94088047117491));
#247799=CARTESIAN_POINT('Ctrl Pts',(-8.96938429267157,12.2,6.94172106151903));
#247800=CARTESIAN_POINT('Ctrl Pts',(-8.97289945198276,12.2,6.94255919716723));
#247801=CARTESIAN_POINT('Ctrl Pts',(-8.97642230665666,12.2,6.94339484363665));
#247802=CARTESIAN_POINT('Ctrl Pts',(-8.98111944600853,12.2,6.94450903887863));
#247803=CARTESIAN_POINT('Ctrl Pts',(-8.98583026972047,12.2,6.94561881087745));
#247804=CARTESIAN_POINT('Ctrl Pts',(-8.99055471338891,12.2,6.94672407867627));
#247805=CARTESIAN_POINT('Ctrl Pts',(-8.99409804630116,12.2,6.94755302956303));
#247806=CARTESIAN_POINT('Ctrl Pts',(-8.99764904130456,12.2,6.94837944809998));
#247807=CARTESIAN_POINT('Ctrl Pts',(-9.00120767071589,12.2,6.9492032990704));
#247808=CARTESIAN_POINT('Ctrl Pts',(-9.00476630077371,12.2,6.95002715019049));
#247809=CARTESIAN_POINT('Ctrl Pts',(-9.00833256554203,12.2,6.95084843592652));
#247810=CARTESIAN_POINT('Ctrl Pts',(-9.01190644002079,12.2,6.95166712192015));
#247811=CARTESIAN_POINT('Ctrl Pts',(-9.0154803138503,12.2,6.95248580776504));
#247812=CARTESIAN_POINT('Ctrl Pts',(-9.01906179642801,12.2,6.95330189349657));
#247813=CARTESIAN_POINT('Ctrl Pts',(-9.02265086143614,12.2,6.95411534742403));
#247814=CARTESIAN_POINT('Ctrl Pts',(-9.02623992644427,12.2,6.95492880135148));
#247815=CARTESIAN_POINT('Ctrl Pts',(-9.02983657278995,12.2,6.95573962360097));
#247816=CARTESIAN_POINT('Ctrl Pts',(-9.03344077565966,12.2,6.95654778007138));
#247817=CARTESIAN_POINT('Ctrl Pts',(-9.03704497852936,12.2,6.95735593654179));
#247818=CARTESIAN_POINT('Ctrl Pts',(-9.04065673763151,12.2,6.95816142856251));
#247819=CARTESIAN_POINT('Ctrl Pts',(-9.044276027,12.2,6.95896422395001));
#247820=CARTESIAN_POINT('Ctrl Pts',(-9.04789531636849,12.2,6.9597670193375));
#247821=CARTESIAN_POINT('Ctrl Pts',(-9.05152213552004,12.2,6.96056711882511));
#247822=CARTESIAN_POINT('Ctrl Pts',(-9.05515645934565,12.2,6.96136448871304));
#247823=CARTESIAN_POINT('Ctrl Pts',(-9.05879078317127,12.2,6.96216185860098));
#247824=CARTESIAN_POINT('Ctrl Pts',(-9.06243261079517,12.2,6.96295650025233));
#247825=CARTESIAN_POINT('Ctrl Pts',(-9.06608191530235,12.2,6.96374838013843));
#247826=CARTESIAN_POINT('Ctrl Pts',(-9.06973121980953,12.2,6.96454026002454));
#247827=CARTESIAN_POINT('Ctrl Pts',(-9.07338799986868,12.2,6.96532937690677));
#247828=CARTESIAN_POINT('Ctrl Pts',(-9.07705223219287,12.2,6.96611570133692));
#247829=CARTESIAN_POINT('Ctrl Pts',(-9.08071646518273,12.2,6.96690202590991));
#247830=CARTESIAN_POINT('Ctrl Pts',(-9.08438814868303,12.2,6.96768555725712));
#247831=CARTESIAN_POINT('Ctrl Pts',(-9.08806725980206,12.2,6.9684662673702));
#247832=CARTESIAN_POINT('Ctrl Pts',(-9.09174637025272,12.2,6.96924697734145));
#247833=CARTESIAN_POINT('Ctrl Pts',(-9.09543291006968,12.2,6.97002486752951));
#247834=CARTESIAN_POINT('Ctrl Pts',(-9.0991268494361,12.2,6.97079990333443));
#247835=CARTESIAN_POINT('Ctrl Pts',(-9.10282078880253,12.2,6.97157493913936));
#247836=CARTESIAN_POINT('Ctrl Pts',(-9.10652212867126,12.2,6.97234712124184));
#247837=CARTESIAN_POINT('Ctrl Pts',(-9.11023083701171,12.2,6.9731164105507));
#247838=CARTESIAN_POINT('Ctrl Pts',(-9.11641201780371,12.2,6.97439855944539));
#247839=CARTESIAN_POINT('Ctrl Pts',(-9.12261365747818,12.2,6.97567266250236));
#247840=CARTESIAN_POINT('Ctrl Pts',(-9.1288356732116,12.2,6.97693862333241));
#247841=CARTESIAN_POINT('Ctrl Pts',(-9.13256888251601,12.2,6.97769819980284));
#247842=CARTESIAN_POINT('Ctrl Pts',(-9.13630942931919,12.2,6.97845485086305));
#247843=CARTESIAN_POINT('Ctrl Pts',(-9.14005731500006,12.2,6.97920857099999));
#247844=CARTESIAN_POINT('Ctrl Pts',(-9.36775917500006,15.2,6.67046385499999));
#247845=CARTESIAN_POINT('Ctrl Pts',(-9.36775917500006,11.6,6.67046385499999));
#247846=CARTESIAN_POINT('Ctrl Pts',(-9.36739373000006,15.2,6.66979226099999));
#247847=CARTESIAN_POINT('Ctrl Pts',(-9.36739373000006,11.6,6.66979226099999));
#247848=CARTESIAN_POINT('Ctrl Pts',(-9.36666279600006,15.2,6.66844959699999));
#247849=CARTESIAN_POINT('Ctrl Pts',(-9.36666279600006,11.6,6.66844959699999));
#247850=CARTESIAN_POINT('Ctrl Pts',(-9.36556627000006,15.2,6.66643717599998));
#247851=CARTESIAN_POINT('Ctrl Pts',(-9.36556627000006,11.6,6.66643717599998));
#247852=CARTESIAN_POINT('Ctrl Pts',(-9.36410398400006,15.2,6.66375709899999));
#247853=CARTESIAN_POINT('Ctrl Pts',(-9.36410398400006,11.6,6.66375709899999));
#247854=CARTESIAN_POINT('Ctrl Pts',(-9.36227570600006,15.2,6.66041225199999));
#247855=CARTESIAN_POINT('Ctrl Pts',(-9.36227570600006,11.6,6.66041225199999));
#247856=CARTESIAN_POINT('Ctrl Pts',(-9.36044701000006,15.2,6.65707265499999));
#247857=CARTESIAN_POINT('Ctrl Pts',(-9.36044701000006,11.6,6.65707265499999));
#247858=CARTESIAN_POINT('Ctrl Pts',(-9.35861789700006,15.2,6.65373830999999));
#247859=CARTESIAN_POINT('Ctrl Pts',(-9.35861789700006,11.6,6.65373830999999));
#247860=CARTESIAN_POINT('Ctrl Pts',(-9.35678837100006,15.2,6.65040921899998));
#247861=CARTESIAN_POINT('Ctrl Pts',(-9.35678837100006,11.6,6.65040921899998));
#247862=CARTESIAN_POINT('Ctrl Pts',(-9.35495843800006,15.2,6.64708538399999));
#247863=CARTESIAN_POINT('Ctrl Pts',(-9.35495843800006,11.6,6.64708538399999));
#247864=CARTESIAN_POINT('Ctrl Pts',(-9.35312810400006,15.2,6.64376680699998));
#247865=CARTESIAN_POINT('Ctrl Pts',(-9.35312810400006,11.6,6.64376680699998));
#247866=CARTESIAN_POINT('Ctrl Pts',(-9.35129738000006,15.2,6.64045349299998));
#247867=CARTESIAN_POINT('Ctrl Pts',(-9.35129738000006,11.6,6.64045349299998));
#247868=CARTESIAN_POINT('Ctrl Pts',(-9.34946627400006,15.2,6.63714544599999));
#247869=CARTESIAN_POINT('Ctrl Pts',(-9.34946627400006,11.6,6.63714544599999));
#247870=CARTESIAN_POINT('Ctrl Pts',(-9.34763479800005,15.2,6.63384267099998));
#247871=CARTESIAN_POINT('Ctrl Pts',(-9.34763479800005,11.6,6.63384267099998));
#247872=CARTESIAN_POINT('Ctrl Pts',(-9.34580296100006,15.2,6.63054516999999));
#247873=CARTESIAN_POINT('Ctrl Pts',(-9.34580296100006,11.6,6.63054516999999));
#247874=CARTESIAN_POINT('Ctrl Pts',(-9.34397077300006,15.2,6.62725294899998));
#247875=CARTESIAN_POINT('Ctrl Pts',(-9.34397077300006,11.6,6.62725294899998));
#247876=CARTESIAN_POINT('Ctrl Pts',(-9.34213824300006,15.2,6.62396601199998));
#247877=CARTESIAN_POINT('Ctrl Pts',(-9.34213824300006,11.6,6.62396601199998));
#247878=CARTESIAN_POINT('Ctrl Pts',(-9.34030538000006,15.2,6.62068435999998));
#247879=CARTESIAN_POINT('Ctrl Pts',(-9.34030538000006,11.6,6.62068435999998));
#247880=CARTESIAN_POINT('Ctrl Pts',(-9.33847218900006,15.2,6.61740799699999));
#247881=CARTESIAN_POINT('Ctrl Pts',(-9.33847218900006,11.6,6.61740799699999));
#247882=CARTESIAN_POINT('Ctrl Pts',(-9.33663868100006,15.2,6.61413692899998));
#247883=CARTESIAN_POINT('Ctrl Pts',(-9.33663868100006,11.6,6.61413692899998));
#247884=CARTESIAN_POINT('Ctrl Pts',(-9.33480486000006,15.2,6.61087115499999));
#247885=CARTESIAN_POINT('Ctrl Pts',(-9.33480486000006,11.6,6.61087115499999));
#247886=CARTESIAN_POINT('Ctrl Pts',(-9.33297073500006,15.2,6.60761067999999));
#247887=CARTESIAN_POINT('Ctrl Pts',(-9.33297073500006,11.6,6.60761067999999));
#247888=CARTESIAN_POINT('Ctrl Pts',(-9.33113631600006,15.2,6.60435550799999));
#247889=CARTESIAN_POINT('Ctrl Pts',(-9.33113631600006,11.6,6.60435550799999));
#247890=CARTESIAN_POINT('Ctrl Pts',(-9.32930160900005,15.2,6.60110564199999));
#247891=CARTESIAN_POINT('Ctrl Pts',(-9.32930160900005,11.6,6.60110564199999));
#247892=CARTESIAN_POINT('Ctrl Pts',(-9.32746662500006,15.2,6.59786108599998));
#247893=CARTESIAN_POINT('Ctrl Pts',(-9.32746662500006,11.6,6.59786108599998));
#247894=CARTESIAN_POINT('Ctrl Pts',(-9.32563137200006,15.2,6.59462184199998));
#247895=CARTESIAN_POINT('Ctrl Pts',(-9.32563137200006,11.6,6.59462184199998));
#247896=CARTESIAN_POINT('Ctrl Pts',(-9.32379585900006,15.2,6.59138791599998));
#247897=CARTESIAN_POINT('Ctrl Pts',(-9.32379585900006,11.6,6.59138791599998));
#247898=CARTESIAN_POINT('Ctrl Pts',(-9.32196009400006,15.2,6.58815930999998));
#247899=CARTESIAN_POINT('Ctrl Pts',(-9.32196009400006,11.6,6.58815930999998));
#247900=CARTESIAN_POINT('Ctrl Pts',(-9.32012408700006,15.2,6.58493602799999));
#247901=CARTESIAN_POINT('Ctrl Pts',(-9.32012408700006,11.6,6.58493602799999));
#247902=CARTESIAN_POINT('Ctrl Pts',(-9.31828784500006,15.2,6.58171807199999));
#247903=CARTESIAN_POINT('Ctrl Pts',(-9.31828784500006,11.6,6.58171807199999));
#247904=CARTESIAN_POINT('Ctrl Pts',(-9.31645137600006,15.2,6.57850544799999));
#247905=CARTESIAN_POINT('Ctrl Pts',(-9.31645137600006,11.6,6.57850544799999));
#247906=CARTESIAN_POINT('Ctrl Pts',(-9.31461469100006,15.2,6.57529815699998));
#247907=CARTESIAN_POINT('Ctrl Pts',(-9.31461469100006,11.6,6.57529815699998));
#247908=CARTESIAN_POINT('Ctrl Pts',(-9.31277779500006,15.2,6.57209620299999));
#247909=CARTESIAN_POINT('Ctrl Pts',(-9.31277779500006,11.6,6.57209620299999));
#247910=CARTESIAN_POINT('Ctrl Pts',(-9.31094070000006,15.2,6.56889958999999));
#247911=CARTESIAN_POINT('Ctrl Pts',(-9.31094070000006,11.6,6.56889958999999));
#247912=CARTESIAN_POINT('Ctrl Pts',(-9.30910341200006,15.2,6.56570832299998));
#247913=CARTESIAN_POINT('Ctrl Pts',(-9.30910341200006,11.6,6.56570832299998));
#247914=CARTESIAN_POINT('Ctrl Pts',(-9.30726594100006,15.2,6.56252240099998));
#247915=CARTESIAN_POINT('Ctrl Pts',(-9.30726594100006,11.6,6.56252240099998));
#247916=CARTESIAN_POINT('Ctrl Pts',(-9.30542829600006,15.2,6.55934183199999));
#247917=CARTESIAN_POINT('Ctrl Pts',(-9.30542829600006,11.6,6.55934183199999));
#247918=CARTESIAN_POINT('Ctrl Pts',(-9.30359048400006,15.2,6.55616661699998));
#247919=CARTESIAN_POINT('Ctrl Pts',(-9.30359048400006,11.6,6.55616661699998));
#247920=CARTESIAN_POINT('Ctrl Pts',(-9.30175251500006,15.2,6.55299675999998));
#247921=CARTESIAN_POINT('Ctrl Pts',(-9.30175251500006,11.6,6.55299675999998));
#247922=CARTESIAN_POINT('Ctrl Pts',(-9.29991439900006,15.2,6.54983226399998));
#247923=CARTESIAN_POINT('Ctrl Pts',(-9.29991439900006,11.6,6.54983226399998));
#247924=CARTESIAN_POINT('Ctrl Pts',(-9.29807614200006,15.2,6.54667313399998));
#247925=CARTESIAN_POINT('Ctrl Pts',(-9.29807614200006,11.6,6.54667313399998));
#247926=CARTESIAN_POINT('Ctrl Pts',(-9.29623775500006,15.2,6.54351937099998));
#247927=CARTESIAN_POINT('Ctrl Pts',(-9.29623775500006,11.6,6.54351937099998));
#247928=CARTESIAN_POINT('Ctrl Pts',(-9.29439924500005,15.2,6.54037098099998));
#247929=CARTESIAN_POINT('Ctrl Pts',(-9.29439924500005,11.6,6.54037098099998));
#247930=CARTESIAN_POINT('Ctrl Pts',(-9.29256062200006,15.2,6.53722796599999));
#247931=CARTESIAN_POINT('Ctrl Pts',(-9.29256062200006,11.6,6.53722796599999));
#247932=CARTESIAN_POINT('Ctrl Pts',(-9.29072189500006,15.2,6.53409032999999));
#247933=CARTESIAN_POINT('Ctrl Pts',(-9.29072189500006,11.6,6.53409032999999));
#247934=CARTESIAN_POINT('Ctrl Pts',(-9.28888307100006,15.2,6.53095807499999));
#247935=CARTESIAN_POINT('Ctrl Pts',(-9.28888307100006,11.6,6.53095807499999));
#247936=CARTESIAN_POINT('Ctrl Pts',(-9.28704416000006,15.2,6.52783120699999));
#247937=CARTESIAN_POINT('Ctrl Pts',(-9.28704416000006,11.6,6.52783120699999));
#247938=CARTESIAN_POINT('Ctrl Pts',(-9.28520517200005,15.2,6.52470972599998));
#247939=CARTESIAN_POINT('Ctrl Pts',(-9.28520517200005,11.6,6.52470972599998));
#247940=CARTESIAN_POINT('Ctrl Pts',(-9.28336611400006,15.2,6.52159363899998));
#247941=CARTESIAN_POINT('Ctrl Pts',(-9.28336611400006,11.6,6.52159363899998));
#247942=CARTESIAN_POINT('Ctrl Pts',(-9.28152699600006,15.2,6.51848294699998));
#247943=CARTESIAN_POINT('Ctrl Pts',(-9.28152699600006,11.6,6.51848294699998));
#247944=CARTESIAN_POINT('Ctrl Pts',(-9.27968782700006,15.2,6.51537765499998));
#247945=CARTESIAN_POINT('Ctrl Pts',(-9.27968782700006,11.6,6.51537765499998));
#247946=CARTESIAN_POINT('Ctrl Pts',(-9.27784861500006,15.2,6.51227776499999));
#247947=CARTESIAN_POINT('Ctrl Pts',(-9.27784861500006,11.6,6.51227776499999));
#247948=CARTESIAN_POINT('Ctrl Pts',(-9.27600936900006,15.2,6.50918328099999));
#247949=CARTESIAN_POINT('Ctrl Pts',(-9.27600936900006,11.6,6.50918328099999));
#247950=CARTESIAN_POINT('Ctrl Pts',(-9.27417010000006,15.2,6.50609420699999));
#247951=CARTESIAN_POINT('Ctrl Pts',(-9.27417010000006,11.6,6.50609420699999));
#247952=CARTESIAN_POINT('Ctrl Pts',(-9.27233081400006,15.2,6.50301054499998));
#247953=CARTESIAN_POINT('Ctrl Pts',(-9.27233081400006,11.6,6.50301054499998));
#247954=CARTESIAN_POINT('Ctrl Pts',(-9.27049152300006,15.2,6.49993229999998));
#247955=CARTESIAN_POINT('Ctrl Pts',(-9.27049152300006,11.6,6.49993229999998));
#247956=CARTESIAN_POINT('Ctrl Pts',(-9.26865223400006,15.2,6.49685947499999));
#247957=CARTESIAN_POINT('Ctrl Pts',(-9.26865223400006,11.6,6.49685947499999));
#247958=CARTESIAN_POINT('Ctrl Pts',(-9.26681295600006,15.2,6.49379207299998));
#247959=CARTESIAN_POINT('Ctrl Pts',(-9.26681295600006,11.6,6.49379207299998));
#247960=CARTESIAN_POINT('Ctrl Pts',(-9.26497369900006,15.2,6.49073009799999));
#247961=CARTESIAN_POINT('Ctrl Pts',(-9.26497369900006,11.6,6.49073009799999));
#247962=CARTESIAN_POINT('Ctrl Pts',(-9.26313447100006,15.2,6.48767355199999));
#247963=CARTESIAN_POINT('Ctrl Pts',(-9.26313447100006,11.6,6.48767355199999));
#247964=CARTESIAN_POINT('Ctrl Pts',(-9.26129528300006,15.2,6.48462243999998));
#247965=CARTESIAN_POINT('Ctrl Pts',(-9.26129528300006,11.6,6.48462243999998));
#247966=CARTESIAN_POINT('Ctrl Pts',(-9.25945614200005,15.2,6.48157676499999));
#247967=CARTESIAN_POINT('Ctrl Pts',(-9.25945614200005,11.6,6.48157676499999));
#247968=CARTESIAN_POINT('Ctrl Pts',(-9.25761705900005,15.2,6.47853652899999));
#247969=CARTESIAN_POINT('Ctrl Pts',(-9.25761705900005,11.6,6.47853652899999));
#247970=CARTESIAN_POINT('Ctrl Pts',(-9.25577804200006,15.2,6.47550173699998));
#247971=CARTESIAN_POINT('Ctrl Pts',(-9.25577804200006,11.6,6.47550173699998));
#247972=CARTESIAN_POINT('Ctrl Pts',(-9.25393910000006,15.2,6.47247239299999));
#247973=CARTESIAN_POINT('Ctrl Pts',(-9.25393910000006,11.6,6.47247239299999));
#247974=CARTESIAN_POINT('Ctrl Pts',(-9.25210024300006,15.2,6.46944849899998));
#247975=CARTESIAN_POINT('Ctrl Pts',(-9.25210024300006,11.6,6.46944849899998));
#247976=CARTESIAN_POINT('Ctrl Pts',(-9.25026148000006,15.2,6.46643005899998));
#247977=CARTESIAN_POINT('Ctrl Pts',(-9.25026148000006,11.6,6.46643005899998));
#247978=CARTESIAN_POINT('Ctrl Pts',(-9.24842281900006,15.2,6.46341707599999));
#247979=CARTESIAN_POINT('Ctrl Pts',(-9.24842281900006,11.6,6.46341707599999));
#247980=CARTESIAN_POINT('Ctrl Pts',(-9.24658427100006,15.2,6.46040955399998));
#247981=CARTESIAN_POINT('Ctrl Pts',(-9.24658427100006,11.6,6.46040955399998));
#247982=CARTESIAN_POINT('Ctrl Pts',(-9.24474584400006,15.2,6.45740749499998));
#247983=CARTESIAN_POINT('Ctrl Pts',(-9.24474584400006,11.6,6.45740749499998));
#247984=CARTESIAN_POINT('Ctrl Pts',(-9.24290754900005,15.2,6.45441090499999));
#247985=CARTESIAN_POINT('Ctrl Pts',(-9.24290754900005,11.6,6.45441090499999));
#247986=CARTESIAN_POINT('Ctrl Pts',(-9.24106939500006,15.2,6.45141978499999));
#247987=CARTESIAN_POINT('Ctrl Pts',(-9.24106939500006,11.6,6.45141978499999));
#247988=CARTESIAN_POINT('Ctrl Pts',(-9.23923138900006,15.2,6.44843413999999));
#247989=CARTESIAN_POINT('Ctrl Pts',(-9.23923138900006,11.6,6.44843413999999));
#247990=CARTESIAN_POINT('Ctrl Pts',(-9.23739354200006,15.2,6.44545397099999));
#247991=CARTESIAN_POINT('Ctrl Pts',(-9.23739354200006,11.6,6.44545397099999));
#247992=CARTESIAN_POINT('Ctrl Pts',(-9.23555586400006,15.2,6.44247928399999));
#247993=CARTESIAN_POINT('Ctrl Pts',(-9.23555586400006,11.6,6.44247928399999));
#247994=CARTESIAN_POINT('Ctrl Pts',(-9.23371836400005,15.2,6.43951008199998));
#247995=CARTESIAN_POINT('Ctrl Pts',(-9.23371836400005,11.6,6.43951008199998));
#247996=CARTESIAN_POINT('Ctrl Pts',(-9.23188105000006,15.2,6.43654636699999));
#247997=CARTESIAN_POINT('Ctrl Pts',(-9.23188105000006,11.6,6.43654636699999));
#247998=CARTESIAN_POINT('Ctrl Pts',(-9.23004393400005,15.2,6.43358814399999));
#247999=CARTESIAN_POINT('Ctrl Pts',(-9.23004393400005,11.6,6.43358814399999));
#248000=CARTESIAN_POINT('Ctrl Pts',(-9.22820702300006,15.2,6.43063541499998));
#248001=CARTESIAN_POINT('Ctrl Pts',(-9.22820702300006,11.6,6.43063541499998));
#248002=CARTESIAN_POINT('Ctrl Pts',(-9.22637032800005,15.2,6.42768818399999));
#248003=CARTESIAN_POINT('Ctrl Pts',(-9.22637032800005,11.6,6.42768818399999));
#248004=CARTESIAN_POINT('Ctrl Pts',(-9.22453385800006,15.2,6.42474645499998));
#248005=CARTESIAN_POINT('Ctrl Pts',(-9.22453385800006,11.6,6.42474645499998));
#248006=CARTESIAN_POINT('Ctrl Pts',(-9.22269762200006,15.2,6.42181023099998));
#248007=CARTESIAN_POINT('Ctrl Pts',(-9.22269762200006,11.6,6.42181023099998));
#248008=CARTESIAN_POINT('Ctrl Pts',(-9.22086163000005,15.2,6.41887951399998));
#248009=CARTESIAN_POINT('Ctrl Pts',(-9.22086163000005,11.6,6.41887951399998));
#248010=CARTESIAN_POINT('Ctrl Pts',(-9.21902589300006,15.2,6.41595430899999));
#248011=CARTESIAN_POINT('Ctrl Pts',(-9.21902589300006,11.6,6.41595430899999));
#248012=CARTESIAN_POINT('Ctrl Pts',(-9.21719041800005,15.2,6.41303461799998));
#248013=CARTESIAN_POINT('Ctrl Pts',(-9.21719041800005,11.6,6.41303461799998));
#248014=CARTESIAN_POINT('Ctrl Pts',(-9.21535521700006,15.2,6.41012044699998));
#248015=CARTESIAN_POINT('Ctrl Pts',(-9.21535521700006,11.6,6.41012044699998));
#248016=CARTESIAN_POINT('Ctrl Pts',(-9.21352029700006,15.2,6.40721179599999));
#248017=CARTESIAN_POINT('Ctrl Pts',(-9.21352029700006,11.6,6.40721179599999));
#248018=CARTESIAN_POINT('Ctrl Pts',(-9.21168567000005,15.2,6.40430867199999));
#248019=CARTESIAN_POINT('Ctrl Pts',(-9.21168567000005,11.6,6.40430867199999));
#248020=CARTESIAN_POINT('Ctrl Pts',(-9.20985134500006,15.2,6.40141107499999));
#248021=CARTESIAN_POINT('Ctrl Pts',(-9.20985134500006,11.6,6.40141107499999));
#248022=CARTESIAN_POINT('Ctrl Pts',(-9.20801733100006,15.2,6.39851900999999));
#248023=CARTESIAN_POINT('Ctrl Pts',(-9.20801733100006,11.6,6.39851900999999));
#248024=CARTESIAN_POINT('Ctrl Pts',(-9.20618363700006,15.2,6.39563248099999));
#248025=CARTESIAN_POINT('Ctrl Pts',(-9.20618363700006,11.6,6.39563248099999));
#248026=CARTESIAN_POINT('Ctrl Pts',(-9.20435027600006,15.2,6.39275148899999));
#248027=CARTESIAN_POINT('Ctrl Pts',(-9.20435027600006,11.6,6.39275148899999));
#248028=CARTESIAN_POINT('Ctrl Pts',(-9.20251725500006,15.2,6.38987603999999));
#248029=CARTESIAN_POINT('Ctrl Pts',(-9.20251725500006,11.6,6.38987603999999));
#248030=CARTESIAN_POINT('Ctrl Pts',(-9.20068458400005,15.2,6.38700613599998));
#248031=CARTESIAN_POINT('Ctrl Pts',(-9.20068458400005,11.6,6.38700613599998));
#248032=CARTESIAN_POINT('Ctrl Pts',(-9.19885227300006,15.2,6.38414178099998));
#248033=CARTESIAN_POINT('Ctrl Pts',(-9.19885227300006,11.6,6.38414178099998));
#248034=CARTESIAN_POINT('Ctrl Pts',(-9.19702033200006,15.2,6.38128297799998));
#248035=CARTESIAN_POINT('Ctrl Pts',(-9.19702033200006,11.6,6.38128297799998));
#248036=CARTESIAN_POINT('Ctrl Pts',(-9.19518877100005,15.2,6.37842972899998));
#248037=CARTESIAN_POINT('Ctrl Pts',(-9.19518877100005,11.6,6.37842972899998));
#248038=CARTESIAN_POINT('Ctrl Pts',(-9.19335760100006,15.2,6.37558203999999));
#248039=CARTESIAN_POINT('Ctrl Pts',(-9.19335760100006,11.6,6.37558203999999));
#248040=CARTESIAN_POINT('Ctrl Pts',(-9.19152683000006,15.2,6.37273991299999));
#248041=CARTESIAN_POINT('Ctrl Pts',(-9.19152683000006,11.6,6.37273991299999));
#248042=CARTESIAN_POINT('Ctrl Pts',(-9.18969646800005,15.2,6.36990335099998));
#248043=CARTESIAN_POINT('Ctrl Pts',(-9.18969646800005,11.6,6.36990335099998));
#248044=CARTESIAN_POINT('Ctrl Pts',(-9.18786652500006,15.2,6.36707235899999));
#248045=CARTESIAN_POINT('Ctrl Pts',(-9.18786652500006,11.6,6.36707235899999));
#248046=CARTESIAN_POINT('Ctrl Pts',(-9.18603701300006,15.2,6.36424693799999));
#248047=CARTESIAN_POINT('Ctrl Pts',(-9.18603701300006,11.6,6.36424693799999));
#248048=CARTESIAN_POINT('Ctrl Pts',(-9.18420793900006,15.2,6.36142709299998));
#248049=CARTESIAN_POINT('Ctrl Pts',(-9.18420793900006,11.6,6.36142709299998));
#248050=CARTESIAN_POINT('Ctrl Pts',(-9.18237931500006,15.2,6.35861282699998));
#248051=CARTESIAN_POINT('Ctrl Pts',(-9.18237931500006,11.6,6.35861282699998));
#248052=CARTESIAN_POINT('Ctrl Pts',(-9.18055115000006,15.2,6.35580414299999));
#248053=CARTESIAN_POINT('Ctrl Pts',(-9.18055115000006,11.6,6.35580414299999));
#248054=CARTESIAN_POINT('Ctrl Pts',(-9.17872345400006,15.2,6.35300104399998));
#248055=CARTESIAN_POINT('Ctrl Pts',(-9.17872345400006,11.6,6.35300104399998));
#248056=CARTESIAN_POINT('Ctrl Pts',(-9.17689623800005,15.2,6.35020353599998));
#248057=CARTESIAN_POINT('Ctrl Pts',(-9.17689623800005,11.6,6.35020353599998));
#248058=CARTESIAN_POINT('Ctrl Pts',(-9.17506951200006,15.2,6.34741161799998));
#248059=CARTESIAN_POINT('Ctrl Pts',(-9.17506951200006,11.6,6.34741161799998));
#248060=CARTESIAN_POINT('Ctrl Pts',(-9.17324328500005,15.2,6.34462529599999));
#248061=CARTESIAN_POINT('Ctrl Pts',(-9.17324328500005,11.6,6.34462529599999));
#248062=CARTESIAN_POINT('Ctrl Pts',(-9.17141756700006,15.2,6.34184457399999));
#248063=CARTESIAN_POINT('Ctrl Pts',(-9.17141756700006,11.6,6.34184457399999));
#248064=CARTESIAN_POINT('Ctrl Pts',(-9.16959236900006,15.2,6.33906945299999));
#248065=CARTESIAN_POINT('Ctrl Pts',(-9.16959236900006,11.6,6.33906945299999));
#248066=CARTESIAN_POINT('Ctrl Pts',(-9.16776770300006,15.2,6.33629993899999));
#248067=CARTESIAN_POINT('Ctrl Pts',(-9.16776770300006,11.6,6.33629993899999));
#248068=CARTESIAN_POINT('Ctrl Pts',(-9.16594357600006,15.2,6.33353603299999));
#248069=CARTESIAN_POINT('Ctrl Pts',(-9.16594357600006,11.6,6.33353603299999));
#248070=CARTESIAN_POINT('Ctrl Pts',(-9.16411999900006,15.2,6.33077774099998));
#248071=CARTESIAN_POINT('Ctrl Pts',(-9.16411999900006,11.6,6.33077774099998));
#248072=CARTESIAN_POINT('Ctrl Pts',(-9.16229698400005,15.2,6.32802506299999));
#248073=CARTESIAN_POINT('Ctrl Pts',(-9.16229698400005,11.6,6.32802506299999));
#248074=CARTESIAN_POINT('Ctrl Pts',(-9.16047453800006,15.2,6.32527800399998));
#248075=CARTESIAN_POINT('Ctrl Pts',(-9.16047453800006,11.6,6.32527800399998));
#248076=CARTESIAN_POINT('Ctrl Pts',(-9.15865267500006,15.2,6.32253656799998));
#248077=CARTESIAN_POINT('Ctrl Pts',(-9.15865267500006,11.6,6.32253656799998));
#248078=CARTESIAN_POINT('Ctrl Pts',(-9.15683140400006,15.2,6.31980075699998));
#248079=CARTESIAN_POINT('Ctrl Pts',(-9.15683140400006,11.6,6.31980075699998));
#248080=CARTESIAN_POINT('Ctrl Pts',(-9.15501073300005,15.2,6.31707057599999));
#248081=CARTESIAN_POINT('Ctrl Pts',(-9.15501073300005,11.6,6.31707057599999));
#248082=CARTESIAN_POINT('Ctrl Pts',(-9.15319067500005,15.2,6.31434602699999));
#248083=CARTESIAN_POINT('Ctrl Pts',(-9.15319067500005,11.6,6.31434602699999));
#248084=CARTESIAN_POINT('Ctrl Pts',(-9.15137124100006,15.2,6.31162711399998));
#248085=CARTESIAN_POINT('Ctrl Pts',(-9.15137124100006,11.6,6.31162711399998));
#248086=CARTESIAN_POINT('Ctrl Pts',(-9.14955243800006,15.2,6.30891383999998));
#248087=CARTESIAN_POINT('Ctrl Pts',(-9.14955243800006,11.6,6.30891383999998));
#248088=CARTESIAN_POINT('Ctrl Pts',(-9.14773428000006,15.2,6.30620620699998));
#248089=CARTESIAN_POINT('Ctrl Pts',(-9.14773428000006,11.6,6.30620620699998));
#248090=CARTESIAN_POINT('Ctrl Pts',(-9.14591677600006,15.2,6.30350422099998));
#248091=CARTESIAN_POINT('Ctrl Pts',(-9.14591677600006,11.6,6.30350422099998));
#248092=CARTESIAN_POINT('Ctrl Pts',(-9.14409993600006,15.2,6.30080788299999));
#248093=CARTESIAN_POINT('Ctrl Pts',(-9.14409993600006,11.6,6.30080788299999));
#248094=CARTESIAN_POINT('Ctrl Pts',(-9.14228377000006,15.2,6.29811719799999));
#248095=CARTESIAN_POINT('Ctrl Pts',(-9.14228377000006,11.6,6.29811719799999));
#248096=CARTESIAN_POINT('Ctrl Pts',(-9.14046829000006,15.2,6.29543216899999));
#248097=CARTESIAN_POINT('Ctrl Pts',(-9.14046829000006,11.6,6.29543216899999));
#248098=CARTESIAN_POINT('Ctrl Pts',(-9.13865350700006,15.2,6.29275279899999));
#248099=CARTESIAN_POINT('Ctrl Pts',(-9.13865350700006,11.6,6.29275279899999));
#248100=CARTESIAN_POINT('Ctrl Pts',(-9.13683942900006,15.2,6.29007908999998));
#248101=CARTESIAN_POINT('Ctrl Pts',(-9.13683942900006,11.6,6.29007908999998));
#248102=CARTESIAN_POINT('Ctrl Pts',(-9.13502606900006,15.2,6.28741104799998));
#248103=CARTESIAN_POINT('Ctrl Pts',(-9.13502606900006,11.6,6.28741104799998));
#248104=CARTESIAN_POINT('Ctrl Pts',(-9.13321343700006,15.2,6.28474867399999));
#248105=CARTESIAN_POINT('Ctrl Pts',(-9.13321343700006,11.6,6.28474867399999));
#248106=CARTESIAN_POINT('Ctrl Pts',(-9.13140154400006,15.2,6.28209197299999));
#248107=CARTESIAN_POINT('Ctrl Pts',(-9.13140154400006,11.6,6.28209197299999));
#248108=CARTESIAN_POINT('Ctrl Pts',(-9.12959039800005,15.2,6.27944094699998));
#248109=CARTESIAN_POINT('Ctrl Pts',(-9.12959039800005,11.6,6.27944094699998));
#248110=CARTESIAN_POINT('Ctrl Pts',(-9.12778001300006,15.2,6.27679559999999));
#248111=CARTESIAN_POINT('Ctrl Pts',(-9.12778001300006,11.6,6.27679559999999));
#248112=CARTESIAN_POINT('Ctrl Pts',(-9.12597039900006,15.2,6.27415593499999));
#248113=CARTESIAN_POINT('Ctrl Pts',(-9.12597039900006,11.6,6.27415593499999));
#248114=CARTESIAN_POINT('Ctrl Pts',(-9.12416156500005,15.2,6.27152195499999));
#248115=CARTESIAN_POINT('Ctrl Pts',(-9.12416156500005,11.6,6.27152195499999));
#248116=CARTESIAN_POINT('Ctrl Pts',(-9.12235352400005,15.2,6.26889366399999));
#248117=CARTESIAN_POINT('Ctrl Pts',(-9.12235352400005,11.6,6.26889366399999));
#248118=CARTESIAN_POINT('Ctrl Pts',(-9.12054628500006,15.2,6.26627106499999));
#248119=CARTESIAN_POINT('Ctrl Pts',(-9.12054628500006,11.6,6.26627106499999));
#248120=CARTESIAN_POINT('Ctrl Pts',(-9.11873986100005,15.2,6.26365416199998));
#248121=CARTESIAN_POINT('Ctrl Pts',(-9.11873986100005,11.6,6.26365416199998));
#248122=CARTESIAN_POINT('Ctrl Pts',(-9.11693426000006,15.2,6.26104295699999));
#248123=CARTESIAN_POINT('Ctrl Pts',(-9.11693426000006,11.6,6.26104295699999));
#248124=CARTESIAN_POINT('Ctrl Pts',(-9.11512949500005,15.2,6.25843745499999));
#248125=CARTESIAN_POINT('Ctrl Pts',(-9.11512949500005,11.6,6.25843745499999));
#248126=CARTESIAN_POINT('Ctrl Pts',(-9.11332557600005,15.2,6.25583765599998));
#248127=CARTESIAN_POINT('Ctrl Pts',(-9.11332557600005,11.6,6.25583765599998));
#248128=CARTESIAN_POINT('Ctrl Pts',(-9.11152251500006,15.2,6.25324356799998));
#248129=CARTESIAN_POINT('Ctrl Pts',(-9.11152251500006,11.6,6.25324356799998));
#248130=CARTESIAN_POINT('Ctrl Pts',(-9.10972032100006,15.2,6.25065518999998));
#248131=CARTESIAN_POINT('Ctrl Pts',(-9.10972032100006,11.6,6.25065518999998));
#248132=CARTESIAN_POINT('Ctrl Pts',(-9.10791900700006,15.2,6.24807252899998));
#248133=CARTESIAN_POINT('Ctrl Pts',(-9.10791900700006,11.6,6.24807252899998));
#248134=CARTESIAN_POINT('Ctrl Pts',(-9.10611858300006,15.2,6.24549558499999));
#248135=CARTESIAN_POINT('Ctrl Pts',(-9.10611858300006,11.6,6.24549558499999));
#248136=CARTESIAN_POINT('Ctrl Pts',(-9.10431906000005,15.2,6.24292436399998));
#248137=CARTESIAN_POINT('Ctrl Pts',(-9.10431906000005,11.6,6.24292436399998));
#248138=CARTESIAN_POINT('Ctrl Pts',(-9.10252044900006,15.2,6.24035886699998));
#248139=CARTESIAN_POINT('Ctrl Pts',(-9.10252044900006,11.6,6.24035886699998));
#248140=CARTESIAN_POINT('Ctrl Pts',(-9.10072276000006,15.2,6.23779909799998));
#248141=CARTESIAN_POINT('Ctrl Pts',(-9.10072276000006,11.6,6.23779909799998));
#248142=CARTESIAN_POINT('Ctrl Pts',(-9.09892600800006,15.2,6.23524506099999));
#248143=CARTESIAN_POINT('Ctrl Pts',(-9.09892600800006,11.6,6.23524506099999));
#248144=CARTESIAN_POINT('Ctrl Pts',(-9.09713019900006,15.2,6.23269675899999));
#248145=CARTESIAN_POINT('Ctrl Pts',(-9.09713019900006,11.6,6.23269675899999));
#248146=CARTESIAN_POINT('Ctrl Pts',(-9.09533534800006,15.2,6.23015419499998));
#248147=CARTESIAN_POINT('Ctrl Pts',(-9.09533534800006,11.6,6.23015419499998));
#248148=CARTESIAN_POINT('Ctrl Pts',(-9.09354146400006,15.2,6.22761737199998));
#248149=CARTESIAN_POINT('Ctrl Pts',(-9.09354146400006,11.6,6.22761737199998));
#248150=CARTESIAN_POINT('Ctrl Pts',(-9.09174856000006,15.2,6.22508629499999));
#248151=CARTESIAN_POINT('Ctrl Pts',(-9.09174856000006,11.6,6.22508629499999));
#248152=CARTESIAN_POINT('Ctrl Pts',(-9.08995664500006,15.2,6.22256096499999));
#248153=CARTESIAN_POINT('Ctrl Pts',(-9.08995664500006,11.6,6.22256096499999));
#248154=CARTESIAN_POINT('Ctrl Pts',(-9.08816573200006,15.2,6.22004138599999));
#248155=CARTESIAN_POINT('Ctrl Pts',(-9.08816573200006,11.6,6.22004138599999));
#248156=CARTESIAN_POINT('Ctrl Pts',(-9.08637583300006,15.2,6.21752756199999));
#248157=CARTESIAN_POINT('Ctrl Pts',(-9.08637583300006,11.6,6.21752756199999));
#248158=CARTESIAN_POINT('Ctrl Pts',(-9.08458695700006,15.2,6.21501949599998));
#248159=CARTESIAN_POINT('Ctrl Pts',(-9.08458695700006,11.6,6.21501949599998));
#248160=CARTESIAN_POINT('Ctrl Pts',(-9.08279911700006,15.2,6.21251719099998));
#248161=CARTESIAN_POINT('Ctrl Pts',(-9.08279911700006,11.6,6.21251719099998));
#248162=CARTESIAN_POINT('Ctrl Pts',(-9.08101232300006,15.2,6.21002064899999));
#248163=CARTESIAN_POINT('Ctrl Pts',(-9.08101232300006,11.6,6.21002064899999));
#248164=CARTESIAN_POINT('Ctrl Pts',(-9.07922658800006,15.2,6.20752987599998));
#248165=CARTESIAN_POINT('Ctrl Pts',(-9.07922658800006,11.6,6.20752987599998));
#248166=CARTESIAN_POINT('Ctrl Pts',(-9.07744192200006,15.2,6.20504487299999));
#248167=CARTESIAN_POINT('Ctrl Pts',(-9.07744192200006,11.6,6.20504487299999));
#248168=CARTESIAN_POINT('Ctrl Pts',(-9.07565833800006,15.2,6.20256564499999));
#248169=CARTESIAN_POINT('Ctrl Pts',(-9.07565833800006,11.6,6.20256564499999));
#248170=CARTESIAN_POINT('Ctrl Pts',(-9.07387584700006,15.2,6.20009219399999));
#248171=CARTESIAN_POINT('Ctrl Pts',(-9.07387584700006,11.6,6.20009219399999));
#248172=CARTESIAN_POINT('Ctrl Pts',(-9.07209445900006,15.2,6.19762452499998));
#248173=CARTESIAN_POINT('Ctrl Pts',(-9.07209445900006,11.6,6.19762452499998));
#248174=CARTESIAN_POINT('Ctrl Pts',(-9.07031418700005,15.2,6.19516263799999));
#248175=CARTESIAN_POINT('Ctrl Pts',(-9.07031418700005,11.6,6.19516263799999));
#248176=CARTESIAN_POINT('Ctrl Pts',(-9.06853504200006,15.2,6.19270653899999));
#248177=CARTESIAN_POINT('Ctrl Pts',(-9.06853504200006,11.6,6.19270653899999));
#248178=CARTESIAN_POINT('Ctrl Pts',(-9.06675703600006,15.2,6.19025622999998));
#248179=CARTESIAN_POINT('Ctrl Pts',(-9.06675703600006,11.6,6.19025622999998));
#248180=CARTESIAN_POINT('Ctrl Pts',(-9.06498018100006,15.2,6.18781171499998));
#248181=CARTESIAN_POINT('Ctrl Pts',(-9.06498018100006,11.6,6.18781171499998));
#248182=CARTESIAN_POINT('Ctrl Pts',(-9.06320448800006,15.2,6.18537299699998));
#248183=CARTESIAN_POINT('Ctrl Pts',(-9.06320448800006,11.6,6.18537299699998));
#248184=CARTESIAN_POINT('Ctrl Pts',(-9.06142996800006,15.2,6.18294007899999));
#248185=CARTESIAN_POINT('Ctrl Pts',(-9.06142996800006,11.6,6.18294007899999));
#248186=CARTESIAN_POINT('Ctrl Pts',(-9.05965663400006,15.2,6.18051296499999));
#248187=CARTESIAN_POINT('Ctrl Pts',(-9.05965663400006,11.6,6.18051296499999));
#248188=CARTESIAN_POINT('Ctrl Pts',(-9.05788449700006,15.2,6.17809165699998));
#248189=CARTESIAN_POINT('Ctrl Pts',(-9.05788449700006,11.6,6.17809165699998));
#248190=CARTESIAN_POINT('Ctrl Pts',(-9.05611357000006,15.2,6.17567615899999));
#248191=CARTESIAN_POINT('Ctrl Pts',(-9.05611357000006,11.6,6.17567615899999));
#248192=CARTESIAN_POINT('Ctrl Pts',(-9.05434386300006,15.2,6.17326647399998));
#248193=CARTESIAN_POINT('Ctrl Pts',(-9.05434386300006,11.6,6.17326647399998));
#248194=CARTESIAN_POINT('Ctrl Pts',(-9.05257538900005,15.2,6.17086260599999));
#248195=CARTESIAN_POINT('Ctrl Pts',(-9.05257538900005,11.6,6.17086260599999));
#248196=CARTESIAN_POINT('Ctrl Pts',(-9.05080816000006,15.2,6.16846455799998));
#248197=CARTESIAN_POINT('Ctrl Pts',(-9.05080816000006,11.6,6.16846455799998));
#248198=CARTESIAN_POINT('Ctrl Pts',(-9.04904218600005,15.2,6.16607233099998));
#248199=CARTESIAN_POINT('Ctrl Pts',(-9.04904218600005,11.6,6.16607233099998));
#248200=CARTESIAN_POINT('Ctrl Pts',(-9.04727748100006,15.2,6.16368593199999));
#248201=CARTESIAN_POINT('Ctrl Pts',(-9.04727748100006,11.6,6.16368593199999));
#248202=CARTESIAN_POINT('Ctrl Pts',(-9.04551405600006,15.2,6.16130536099998));
#248203=CARTESIAN_POINT('Ctrl Pts',(-9.04551405600006,11.6,6.16130536099998));
#248204=CARTESIAN_POINT('Ctrl Pts',(-9.04375192500006,15.2,6.15893062399999));
#248205=CARTESIAN_POINT('Ctrl Pts',(-9.04375192500006,11.6,6.15893062399999));
#248206=CARTESIAN_POINT('Ctrl Pts',(-9.04199109600006,15.2,6.15656172199999));
#248207=CARTESIAN_POINT('Ctrl Pts',(-9.04199109600006,11.6,6.15656172199999));
#248208=CARTESIAN_POINT('Ctrl Pts',(-9.04023158400006,15.2,6.15419865999999));
#248209=CARTESIAN_POINT('Ctrl Pts',(-9.04023158400006,11.6,6.15419865999999));
#248210=CARTESIAN_POINT('Ctrl Pts',(-9.03847340100006,15.2,6.15184143899998));
#248211=CARTESIAN_POINT('Ctrl Pts',(-9.03847340100006,11.6,6.15184143899998));
#248212=CARTESIAN_POINT('Ctrl Pts',(-9.03671655700006,15.2,6.14949006399998));
#248213=CARTESIAN_POINT('Ctrl Pts',(-9.03671655700006,11.6,6.14949006399998));
#248214=CARTESIAN_POINT('Ctrl Pts',(-9.03496106600005,15.2,6.14714453699998));
#248215=CARTESIAN_POINT('Ctrl Pts',(-9.03496106600005,11.6,6.14714453699998));
#248216=CARTESIAN_POINT('Ctrl Pts',(-9.03320694100006,15.2,6.14480486299998));
#248217=CARTESIAN_POINT('Ctrl Pts',(-9.03320694100006,11.6,6.14480486299998));
#248218=CARTESIAN_POINT('Ctrl Pts',(-9.03145419200006,15.2,6.14247104399999));
#248219=CARTESIAN_POINT('Ctrl Pts',(-9.03145419200006,11.6,6.14247104399999));
#248220=CARTESIAN_POINT('Ctrl Pts',(-9.02970283100006,15.2,6.14014308299998));
#248221=CARTESIAN_POINT('Ctrl Pts',(-9.02970283100006,11.6,6.14014308299998));
#248222=CARTESIAN_POINT('Ctrl Pts',(-9.02795287300006,15.2,6.13782098399999));
#248223=CARTESIAN_POINT('Ctrl Pts',(-9.02795287300006,11.6,6.13782098399999));
#248224=CARTESIAN_POINT('Ctrl Pts',(-9.02620432800006,15.2,6.13550474999998));
#248225=CARTESIAN_POINT('Ctrl Pts',(-9.02620432800006,11.6,6.13550474999998));
#248226=CARTESIAN_POINT('Ctrl Pts',(-9.02445720900005,15.2,6.13319438399999));
#248227=CARTESIAN_POINT('Ctrl Pts',(-9.02445720900005,11.6,6.13319438399999));
#248228=CARTESIAN_POINT('Ctrl Pts',(-9.02271153000006,15.2,6.13088988899998));
#248229=CARTESIAN_POINT('Ctrl Pts',(-9.02271153000006,11.6,6.13088988899998));
#248230=CARTESIAN_POINT('Ctrl Pts',(-9.02096729900006,15.2,6.12859126899998));
#248231=CARTESIAN_POINT('Ctrl Pts',(-9.02096729900006,11.6,6.12859126899998));
#248232=CARTESIAN_POINT('Ctrl Pts',(-9.01922453200006,15.2,6.12629852599999));
#248233=CARTESIAN_POINT('Ctrl Pts',(-9.01922453200006,11.6,6.12629852599999));
#248234=CARTESIAN_POINT('Ctrl Pts',(-9.01748324100006,15.2,6.12401166399999));
#248235=CARTESIAN_POINT('Ctrl Pts',(-9.01748324100006,11.6,6.12401166399999));
#248236=CARTESIAN_POINT('Ctrl Pts',(-9.01574343800006,15.2,6.12173068599999));
#248237=CARTESIAN_POINT('Ctrl Pts',(-9.01574343800006,11.6,6.12173068599999));
#248238=CARTESIAN_POINT('Ctrl Pts',(-9.01400513500005,15.2,6.11945559499999));
#248239=CARTESIAN_POINT('Ctrl Pts',(-9.01400513500005,11.6,6.11945559499999));
#248240=CARTESIAN_POINT('Ctrl Pts',(-9.01226834600006,15.2,6.11718639599999));
#248241=CARTESIAN_POINT('Ctrl Pts',(-9.01226834600006,11.6,6.11718639599999));
#248242=CARTESIAN_POINT('Ctrl Pts',(-9.01053308100006,15.2,6.11492308999999));
#248243=CARTESIAN_POINT('Ctrl Pts',(-9.01053308100006,11.6,6.11492308999999));
#248244=CARTESIAN_POINT('Ctrl Pts',(-9.00879935600006,15.2,6.11266568099998));
#248245=CARTESIAN_POINT('Ctrl Pts',(-9.00879935600006,11.6,6.11266568099998));
#248246=CARTESIAN_POINT('Ctrl Pts',(-9.00706718100006,15.2,6.11041417099998));
#248247=CARTESIAN_POINT('Ctrl Pts',(-9.00706718100006,11.6,6.11041417099998));
#248248=CARTESIAN_POINT('Ctrl Pts',(-9.00533657000006,15.2,6.10816856499999));
#248249=CARTESIAN_POINT('Ctrl Pts',(-9.00533657000006,11.6,6.10816856499999));
#248250=CARTESIAN_POINT('Ctrl Pts',(-9.00360753400006,15.2,6.10592886599999));
#248251=CARTESIAN_POINT('Ctrl Pts',(-9.00360753400006,11.6,6.10592886599999));
#248252=CARTESIAN_POINT('Ctrl Pts',(-9.00188008800006,15.2,6.10369507599999));
#248253=CARTESIAN_POINT('Ctrl Pts',(-9.00188008800006,11.6,6.10369507599999));
#248254=CARTESIAN_POINT('Ctrl Pts',(-9.00015424300006,15.2,6.10146719899999));
#248255=CARTESIAN_POINT('Ctrl Pts',(-9.00015424300006,11.6,6.10146719899999));
#248256=CARTESIAN_POINT('Ctrl Pts',(-8.99843001300006,15.2,6.09924523799998));
#248257=CARTESIAN_POINT('Ctrl Pts',(-8.99843001300006,11.6,6.09924523799998));
#248258=CARTESIAN_POINT('Ctrl Pts',(-8.99670741000006,15.2,6.09702919599999));
#248259=CARTESIAN_POINT('Ctrl Pts',(-8.99670741000006,11.6,6.09702919599999));
#248260=CARTESIAN_POINT('Ctrl Pts',(-8.99498644700006,15.2,6.09481907799999));
#248261=CARTESIAN_POINT('Ctrl Pts',(-8.99498644700006,11.6,6.09481907799999));
#248262=CARTESIAN_POINT('Ctrl Pts',(-8.99326713900006,15.2,6.09261488399999));
#248263=CARTESIAN_POINT('Ctrl Pts',(-8.99326713900006,11.6,6.09261488399999));
#248264=CARTESIAN_POINT('Ctrl Pts',(-8.99154949500005,15.2,6.09041661899998));
#248265=CARTESIAN_POINT('Ctrl Pts',(-8.99154949500005,11.6,6.09041661899998));
#248266=CARTESIAN_POINT('Ctrl Pts',(-8.98983353100006,15.2,6.08822428699998));
#248267=CARTESIAN_POINT('Ctrl Pts',(-8.98983353100006,11.6,6.08822428699998));
#248268=CARTESIAN_POINT('Ctrl Pts',(-8.98811925800005,15.2,6.08603788899998));
#248269=CARTESIAN_POINT('Ctrl Pts',(-8.98811925800005,11.6,6.08603788899998));
#248270=CARTESIAN_POINT('Ctrl Pts',(-8.98640669100006,15.2,6.08385742899999));
#248271=CARTESIAN_POINT('Ctrl Pts',(-8.98640669100006,11.6,6.08385742899999));
#248272=CARTESIAN_POINT('Ctrl Pts',(-8.98469584100006,15.2,6.08168291199998));
#248273=CARTESIAN_POINT('Ctrl Pts',(-8.98469584100006,11.6,6.08168291199998));
#248274=CARTESIAN_POINT('Ctrl Pts',(-8.98298672300006,15.2,6.07951433899999));
#248275=CARTESIAN_POINT('Ctrl Pts',(-8.98298672300006,11.6,6.07951433899999));
#248276=CARTESIAN_POINT('Ctrl Pts',(-8.98127935000005,15.2,6.07735171299999));
#248277=CARTESIAN_POINT('Ctrl Pts',(-8.98127935000005,11.6,6.07735171299999));
#248278=CARTESIAN_POINT('Ctrl Pts',(-8.97957373300006,15.2,6.07519503899999));
#248279=CARTESIAN_POINT('Ctrl Pts',(-8.97957373300006,11.6,6.07519503899999));
#248280=CARTESIAN_POINT('Ctrl Pts',(-8.97786988800006,15.2,6.07304431899998));
#248281=CARTESIAN_POINT('Ctrl Pts',(-8.97786988800006,11.6,6.07304431899998));
#248282=CARTESIAN_POINT('Ctrl Pts',(-8.97616782700006,15.2,6.07089955599999));
#248283=CARTESIAN_POINT('Ctrl Pts',(-8.97616782700006,11.6,6.07089955599999));
#248284=CARTESIAN_POINT('Ctrl Pts',(-8.97446756400005,15.2,6.06876075399998));
#248285=CARTESIAN_POINT('Ctrl Pts',(-8.97446756400005,11.6,6.06876075399998));
#248286=CARTESIAN_POINT('Ctrl Pts',(-8.97276911000005,15.2,6.06662791599998));
#248287=CARTESIAN_POINT('Ctrl Pts',(-8.97276911000005,11.6,6.06662791599998));
#248288=CARTESIAN_POINT('Ctrl Pts',(-8.97107248000006,15.2,6.06450104399999));
#248289=CARTESIAN_POINT('Ctrl Pts',(-8.97107248000006,11.6,6.06450104399999));
#248290=CARTESIAN_POINT('Ctrl Pts',(-8.96937768800005,15.2,6.06238014199998));
#248291=CARTESIAN_POINT('Ctrl Pts',(-8.96937768800005,11.6,6.06238014199998));
#248292=CARTESIAN_POINT('Ctrl Pts',(-8.96768474700006,15.2,6.06026521299999));
#248293=CARTESIAN_POINT('Ctrl Pts',(-8.96768474700006,11.6,6.06026521299999));
#248294=CARTESIAN_POINT('Ctrl Pts',(-8.96599367000006,15.2,6.05815626099999));
#248295=CARTESIAN_POINT('Ctrl Pts',(-8.96599367000006,11.6,6.05815626099999));
#248296=CARTESIAN_POINT('Ctrl Pts',(-8.96430447100006,15.2,6.05605328799999));
#248297=CARTESIAN_POINT('Ctrl Pts',(-8.96430447100006,11.6,6.05605328799999));
#248298=CARTESIAN_POINT('Ctrl Pts',(-8.96261716200006,15.2,6.05395629799999));
#248299=CARTESIAN_POINT('Ctrl Pts',(-8.96261716200006,11.6,6.05395629799999));
#248300=CARTESIAN_POINT('Ctrl Pts',(-8.96093175900005,15.2,6.05186529299999));
#248301=CARTESIAN_POINT('Ctrl Pts',(-8.96093175900005,11.6,6.05186529299999));
#248302=CARTESIAN_POINT('Ctrl Pts',(-8.95924827400006,15.2,6.04978027699998));
#248303=CARTESIAN_POINT('Ctrl Pts',(-8.95924827400006,11.6,6.04978027699998));
#248304=CARTESIAN_POINT('Ctrl Pts',(-8.95756672200006,15.2,6.04770125299999));
#248305=CARTESIAN_POINT('Ctrl Pts',(-8.95756672200006,11.6,6.04770125299999));
#248306=CARTESIAN_POINT('Ctrl Pts',(-8.95588711400006,15.2,6.04562822499998));
#248307=CARTESIAN_POINT('Ctrl Pts',(-8.95588711400006,11.6,6.04562822499998));
#248308=CARTESIAN_POINT('Ctrl Pts',(-8.95420946700006,15.2,6.04356119499998));
#248309=CARTESIAN_POINT('Ctrl Pts',(-8.95420946700006,11.6,6.04356119499998));
#248310=CARTESIAN_POINT('Ctrl Pts',(-8.95253379300006,15.2,6.04150016599998));
#248311=CARTESIAN_POINT('Ctrl Pts',(-8.95253379300006,11.6,6.04150016599998));
#248312=CARTESIAN_POINT('Ctrl Pts',(-8.95086010600006,15.2,6.03944514299998));
#248313=CARTESIAN_POINT('Ctrl Pts',(-8.95086010600006,11.6,6.03944514299998));
#248314=CARTESIAN_POINT('Ctrl Pts',(-8.94918841900006,15.2,6.03739612599998));
#248315=CARTESIAN_POINT('Ctrl Pts',(-8.94918841900006,11.6,6.03739612599998));
#248316=CARTESIAN_POINT('Ctrl Pts',(-8.94751874800006,15.2,6.03535311999998));
#248317=CARTESIAN_POINT('Ctrl Pts',(-8.94751874800006,11.6,6.03535311999998));
#248318=CARTESIAN_POINT('Ctrl Pts',(-8.94585110500006,15.2,6.03331612899999));
#248319=CARTESIAN_POINT('Ctrl Pts',(-8.94585110500006,11.6,6.03331612899999));
#248320=CARTESIAN_POINT('Ctrl Pts',(-8.94418550500006,15.2,6.03128515399998));
#248321=CARTESIAN_POINT('Ctrl Pts',(-8.94418550500006,11.6,6.03128515399998));
#248322=CARTESIAN_POINT('Ctrl Pts',(-8.94252196200006,15.2,6.02926019999998));
#248323=CARTESIAN_POINT('Ctrl Pts',(-8.94252196200006,11.6,6.02926019999998));
#248324=CARTESIAN_POINT('Ctrl Pts',(-8.94086048900006,15.2,6.02724126799998));
#248325=CARTESIAN_POINT('Ctrl Pts',(-8.94086048900006,11.6,6.02724126799998));
#248326=CARTESIAN_POINT('Ctrl Pts',(-8.93920110100006,15.2,6.02522836499999));
#248327=CARTESIAN_POINT('Ctrl Pts',(-8.93920110100006,11.6,6.02522836499999));
#248328=CARTESIAN_POINT('Ctrl Pts',(-8.93754381200005,15.2,6.02322148899999));
#248329=CARTESIAN_POINT('Ctrl Pts',(-8.93754381200005,11.6,6.02322148899999));
#248330=CARTESIAN_POINT('Ctrl Pts',(-8.93588863500005,15.2,6.02122064799998));
#248331=CARTESIAN_POINT('Ctrl Pts',(-8.93588863500005,11.6,6.02122064799998));
#248332=CARTESIAN_POINT('Ctrl Pts',(-8.93423558600006,15.2,6.01922584099999));
#248333=CARTESIAN_POINT('Ctrl Pts',(-8.93423558600006,11.6,6.01922584099999));
#248334=CARTESIAN_POINT('Ctrl Pts',(-8.93258467900005,15.2,6.01723707299998));
#248335=CARTESIAN_POINT('Ctrl Pts',(-8.93258467900005,11.6,6.01723707299998));
#248336=CARTESIAN_POINT('Ctrl Pts',(-8.93093592600006,15.2,6.01525434899998));
#248337=CARTESIAN_POINT('Ctrl Pts',(-8.93093592600006,11.6,6.01525434899998));
#248338=CARTESIAN_POINT('Ctrl Pts',(-8.92928934500006,15.2,6.01327766899999));
#248339=CARTESIAN_POINT('Ctrl Pts',(-8.92928934500006,11.6,6.01327766899999));
#248340=CARTESIAN_POINT('Ctrl Pts',(-8.92764494700005,15.2,6.01130703699998));
#248341=CARTESIAN_POINT('Ctrl Pts',(-8.92764494700005,11.6,6.01130703699998));
#248342=CARTESIAN_POINT('Ctrl Pts',(-8.92600274800006,15.2,6.00934245699998));
#248343=CARTESIAN_POINT('Ctrl Pts',(-8.92600274800006,11.6,6.00934245699998));
#248344=CARTESIAN_POINT('Ctrl Pts',(-8.92436276200005,15.2,6.00738392999999));
#248345=CARTESIAN_POINT('Ctrl Pts',(-8.92436276200005,11.6,6.00738392999999));
#248346=CARTESIAN_POINT('Ctrl Pts',(-8.92272500400006,15.2,6.00543146199998));
#248347=CARTESIAN_POINT('Ctrl Pts',(-8.92272500400006,11.6,6.00543146199998));
#248348=CARTESIAN_POINT('Ctrl Pts',(-8.92108948800006,15.2,6.00348505499999));
#248349=CARTESIAN_POINT('Ctrl Pts',(-8.92108948800006,11.6,6.00348505499999));
#248350=CARTESIAN_POINT('Ctrl Pts',(-8.91945622800005,15.2,6.00154471099999));
#248351=CARTESIAN_POINT('Ctrl Pts',(-8.91945622800005,11.6,6.00154471099999));
#248352=CARTESIAN_POINT('Ctrl Pts',(-8.91782524000006,15.2,5.99961043399999));
#248353=CARTESIAN_POINT('Ctrl Pts',(-8.91782524000006,11.6,5.99961043399999));
#248354=CARTESIAN_POINT('Ctrl Pts',(-8.91619653800005,15.2,5.99768222699999));
#248355=CARTESIAN_POINT('Ctrl Pts',(-8.91619653800005,11.6,5.99768222699999));
#248356=CARTESIAN_POINT('Ctrl Pts',(-8.91457013600006,15.2,5.99576009299999));
#248357=CARTESIAN_POINT('Ctrl Pts',(-8.91457013600006,11.6,5.99576009299999));
#248358=CARTESIAN_POINT('Ctrl Pts',(-8.91294605000006,15.2,5.99384403599998));
#248359=CARTESIAN_POINT('Ctrl Pts',(-8.91294605000006,11.6,5.99384403599998));
#248360=CARTESIAN_POINT('Ctrl Pts',(-8.91132429400006,15.2,5.99193405799999));
#248361=CARTESIAN_POINT('Ctrl Pts',(-8.91132429400006,11.6,5.99193405799999));
#248362=CARTESIAN_POINT('Ctrl Pts',(-8.90970488300006,15.2,5.99003016199998));
#248363=CARTESIAN_POINT('Ctrl Pts',(-8.90970488300006,11.6,5.99003016199998));
#248364=CARTESIAN_POINT('Ctrl Pts',(-8.90808783100006,15.2,5.98813235099998));
#248365=CARTESIAN_POINT('Ctrl Pts',(-8.90808783100006,11.6,5.98813235099998));
#248366=CARTESIAN_POINT('Ctrl Pts',(-8.90647315400006,15.2,5.98624062899999));
#248367=CARTESIAN_POINT('Ctrl Pts',(-8.90647315400006,11.6,5.98624062899999));
#248368=CARTESIAN_POINT('Ctrl Pts',(-8.90486086700006,15.2,5.98435499899999));
#248369=CARTESIAN_POINT('Ctrl Pts',(-8.90486086700006,11.6,5.98435499899999));
#248370=CARTESIAN_POINT('Ctrl Pts',(-8.90325098400006,15.2,5.98247546299999));
#248371=CARTESIAN_POINT('Ctrl Pts',(-8.90325098400006,11.6,5.98247546299999));
#248372=CARTESIAN_POINT('Ctrl Pts',(-8.90164352100006,15.2,5.98060202599999));
#248373=CARTESIAN_POINT('Ctrl Pts',(-8.90164352100006,11.6,5.98060202599999));
#248374=CARTESIAN_POINT('Ctrl Pts',(-8.90003849200006,15.2,5.97873468899999));
#248375=CARTESIAN_POINT('Ctrl Pts',(-8.90003849200006,11.6,5.97873468899999));
#248376=CARTESIAN_POINT('Ctrl Pts',(-8.89843591300006,15.2,5.97687345599999));
#248377=CARTESIAN_POINT('Ctrl Pts',(-8.89843591300006,11.6,5.97687345599999));
#248378=CARTESIAN_POINT('Ctrl Pts',(-8.89683579900005,15.2,5.97501832999999));
#248379=CARTESIAN_POINT('Ctrl Pts',(-8.89683579900005,11.6,5.97501832999999));
#248380=CARTESIAN_POINT('Ctrl Pts',(-8.89523816500006,15.2,5.97316931399998));
#248381=CARTESIAN_POINT('Ctrl Pts',(-8.89523816500006,11.6,5.97316931399998));
#248382=CARTESIAN_POINT('Ctrl Pts',(-8.89364302700006,15.2,5.97132641099999));
#248383=CARTESIAN_POINT('Ctrl Pts',(-8.89364302700006,11.6,5.97132641099999));
#248384=CARTESIAN_POINT('Ctrl Pts',(-8.89205039900006,15.2,5.96948962399999));
#248385=CARTESIAN_POINT('Ctrl Pts',(-8.89205039900006,11.6,5.96948962399999));
#248386=CARTESIAN_POINT('Ctrl Pts',(-8.89046029700006,15.2,5.96765895699999));
#248387=CARTESIAN_POINT('Ctrl Pts',(-8.89046029700006,11.6,5.96765895699999));
#248388=CARTESIAN_POINT('Ctrl Pts',(-8.88887273700006,15.2,5.96583441199999));
#248389=CARTESIAN_POINT('Ctrl Pts',(-8.88887273700006,11.6,5.96583441199999));
#248390=CARTESIAN_POINT('Ctrl Pts',(-8.88728773400006,15.2,5.96401599199999));
#248391=CARTESIAN_POINT('Ctrl Pts',(-8.88728773400006,11.6,5.96401599199999));
#248392=CARTESIAN_POINT('Ctrl Pts',(-8.88570530300006,15.2,5.96220370099999));
#248393=CARTESIAN_POINT('Ctrl Pts',(-8.88570530300006,11.6,5.96220370099999));
#248394=CARTESIAN_POINT('Ctrl Pts',(-8.88412545900006,15.2,5.96039754099999));
#248395=CARTESIAN_POINT('Ctrl Pts',(-8.88412545900006,11.6,5.96039754099999));
#248396=CARTESIAN_POINT('Ctrl Pts',(-8.88254821900006,15.2,5.95859751599999));
#248397=CARTESIAN_POINT('Ctrl Pts',(-8.88254821900006,11.6,5.95859751599999));
#248398=CARTESIAN_POINT('Ctrl Pts',(-8.88097359900006,15.2,5.95680362899999));
#248399=CARTESIAN_POINT('Ctrl Pts',(-8.88097359900006,11.6,5.95680362899999));
#248400=CARTESIAN_POINT('Ctrl Pts',(-8.87940161200006,15.2,5.95501588299998));
#248401=CARTESIAN_POINT('Ctrl Pts',(-8.87940161200006,11.6,5.95501588299998));
#248402=CARTESIAN_POINT('Ctrl Pts',(-8.87783227600006,15.2,5.95323427899999));
#248403=CARTESIAN_POINT('Ctrl Pts',(-8.87783227600006,11.6,5.95323427899999));
#248404=CARTESIAN_POINT('Ctrl Pts',(-8.87626560700006,15.2,5.95145882299998));
#248405=CARTESIAN_POINT('Ctrl Pts',(-8.87626560700006,11.6,5.95145882299998));
#248406=CARTESIAN_POINT('Ctrl Pts',(-8.87470161900006,15.2,5.94968951599999));
#248407=CARTESIAN_POINT('Ctrl Pts',(-8.87470161900006,11.6,5.94968951599999));
#248408=CARTESIAN_POINT('Ctrl Pts',(-8.87314032900006,15.2,5.94792636199998));
#248409=CARTESIAN_POINT('Ctrl Pts',(-8.87314032900006,11.6,5.94792636199998));
#248410=CARTESIAN_POINT('Ctrl Pts',(-8.87158175200006,15.2,5.94616936499998));
#248411=CARTESIAN_POINT('Ctrl Pts',(-8.87158175200006,11.6,5.94616936499998));
#248412=CARTESIAN_POINT('Ctrl Pts',(-8.87002590600006,15.2,5.94441852499998));
#248413=CARTESIAN_POINT('Ctrl Pts',(-8.87002590600006,11.6,5.94441852499998));
#248414=CARTESIAN_POINT('Ctrl Pts',(-8.86847280500006,15.2,5.94267384799998));
#248415=CARTESIAN_POINT('Ctrl Pts',(-8.86847280500006,11.6,5.94267384799998));
#248416=CARTESIAN_POINT('Ctrl Pts',(-8.86692246600006,15.2,5.94093533599998));
#248417=CARTESIAN_POINT('Ctrl Pts',(-8.86692246600006,11.6,5.94093533599998));
#248418=CARTESIAN_POINT('Ctrl Pts',(-8.86537490400006,15.2,5.93920299199999));
#248419=CARTESIAN_POINT('Ctrl Pts',(-8.86537490400006,11.6,5.93920299199999));
#248420=CARTESIAN_POINT('Ctrl Pts',(-8.86383013600006,15.2,5.93747681899998));
#248421=CARTESIAN_POINT('Ctrl Pts',(-8.86383013600006,11.6,5.93747681899998));
#248422=CARTESIAN_POINT('Ctrl Pts',(-8.86228818000006,15.2,5.93575682099999));
#248423=CARTESIAN_POINT('Ctrl Pts',(-8.86228818000006,11.6,5.93575682099999));
#248424=CARTESIAN_POINT('Ctrl Pts',(-8.86074904800006,15.2,5.93404299899999));
#248425=CARTESIAN_POINT('Ctrl Pts',(-8.86074904800006,11.6,5.93404299899999));
#248426=CARTESIAN_POINT('Ctrl Pts',(-8.85921276100006,15.2,5.93233535699999));
#248427=CARTESIAN_POINT('Ctrl Pts',(-8.85921276100006,11.6,5.93233535699999));
#248428=CARTESIAN_POINT('Ctrl Pts',(-8.85767933100006,15.2,5.93063389799998));
#248429=CARTESIAN_POINT('Ctrl Pts',(-8.85767933100006,11.6,5.93063389799998));
#248430=CARTESIAN_POINT('Ctrl Pts',(-8.85614877800006,15.2,5.92893862599999));
#248431=CARTESIAN_POINT('Ctrl Pts',(-8.85614877800006,11.6,5.92893862599999));
#248432=CARTESIAN_POINT('Ctrl Pts',(-8.85462111600006,15.2,5.92724954299998));
#248433=CARTESIAN_POINT('Ctrl Pts',(-8.85462111600006,11.6,5.92724954299998));
#248434=CARTESIAN_POINT('Ctrl Pts',(-8.85309636200006,15.2,5.92556665199999));
#248435=CARTESIAN_POINT('Ctrl Pts',(-8.85309636200006,11.6,5.92556665199999));
#248436=CARTESIAN_POINT('Ctrl Pts',(-8.85157453400006,15.2,5.92388995699999));
#248437=CARTESIAN_POINT('Ctrl Pts',(-8.85157453400006,11.6,5.92388995699999));
#248438=CARTESIAN_POINT('Ctrl Pts',(-8.85005564700006,15.2,5.92221945899999));
#248439=CARTESIAN_POINT('Ctrl Pts',(-8.85005564700006,11.6,5.92221945899999));
#248440=CARTESIAN_POINT('Ctrl Pts',(-8.84853971900006,15.2,5.92055516299999));
#248441=CARTESIAN_POINT('Ctrl Pts',(-8.84853971900006,11.6,5.92055516299999));
#248442=CARTESIAN_POINT('Ctrl Pts',(-8.84702676400006,15.2,5.91889707099998));
#248443=CARTESIAN_POINT('Ctrl Pts',(-8.84702676400006,11.6,5.91889707099998));
#248444=CARTESIAN_POINT('Ctrl Pts',(-8.84551680300006,15.2,5.91724518599998));
#248445=CARTESIAN_POINT('Ctrl Pts',(-8.84551680300006,11.6,5.91724518599998));
#248446=CARTESIAN_POINT('Ctrl Pts',(-8.84400984900006,15.2,5.91559951099998));
#248447=CARTESIAN_POINT('Ctrl Pts',(-8.84400984900006,11.6,5.91559951099998));
#248448=CARTESIAN_POINT('Ctrl Pts',(-8.84250592200006,15.2,5.91396004999999));
#248449=CARTESIAN_POINT('Ctrl Pts',(-8.84250592200006,11.6,5.91396004999999));
#248450=CARTESIAN_POINT('Ctrl Pts',(-8.84100503600006,15.2,5.91232680499999));
#248451=CARTESIAN_POINT('Ctrl Pts',(-8.84100503600006,11.6,5.91232680499999));
#248452=CARTESIAN_POINT('Ctrl Pts',(-8.83950720900006,15.2,5.91069977899998));
#248453=CARTESIAN_POINT('Ctrl Pts',(-8.83950720900006,11.6,5.91069977899998));
#248454=CARTESIAN_POINT('Ctrl Pts',(-8.83801245900005,15.2,5.90907897599998));
#248455=CARTESIAN_POINT('Ctrl Pts',(-8.83801245900005,11.6,5.90907897599998));
#248456=CARTESIAN_POINT('Ctrl Pts',(-8.83652080300006,15.2,5.90746439799998));
#248457=CARTESIAN_POINT('Ctrl Pts',(-8.83652080300006,11.6,5.90746439799998));
#248458=CARTESIAN_POINT('Ctrl Pts',(-8.83503225700006,15.2,5.90585604699999));
#248459=CARTESIAN_POINT('Ctrl Pts',(-8.83503225700006,11.6,5.90585604699999));
#248460=CARTESIAN_POINT('Ctrl Pts',(-8.83354683900006,15.2,5.90425392799999));
#248461=CARTESIAN_POINT('Ctrl Pts',(-8.83354683900006,11.6,5.90425392799999));
#248462=CARTESIAN_POINT('Ctrl Pts',(-8.83206456600006,15.2,5.90265804399999));
#248463=CARTESIAN_POINT('Ctrl Pts',(-8.83206456600006,11.6,5.90265804399999));
#248464=CARTESIAN_POINT('Ctrl Pts',(-8.83058545500005,15.2,5.90106839599999));
#248465=CARTESIAN_POINT('Ctrl Pts',(-8.83058545500005,11.6,5.90106839599999));
#248466=CARTESIAN_POINT('Ctrl Pts',(-8.82910952400006,15.2,5.89948498899999));
#248467=CARTESIAN_POINT('Ctrl Pts',(-8.82910952400006,11.6,5.89948498899999));
#248468=CARTESIAN_POINT('Ctrl Pts',(-8.82763679000006,15.2,5.89790782499998));
#248469=CARTESIAN_POINT('Ctrl Pts',(-8.82763679000006,11.6,5.89790782499998));
#248470=CARTESIAN_POINT('Ctrl Pts',(-8.82616727000006,15.2,5.89633690599998));
#248471=CARTESIAN_POINT('Ctrl Pts',(-8.82616727000006,11.6,5.89633690599998));
#248472=CARTESIAN_POINT('Ctrl Pts',(-8.82470098300006,15.2,5.89477223799998));
#248473=CARTESIAN_POINT('Ctrl Pts',(-8.82470098300006,11.6,5.89477223799998));
#248474=CARTESIAN_POINT('Ctrl Pts',(-8.82323794700006,15.2,5.89321382099998));
#248475=CARTESIAN_POINT('Ctrl Pts',(-8.82323794700006,11.6,5.89321382099998));
#248476=CARTESIAN_POINT('Ctrl Pts',(-8.82177817700006,15.2,5.89166165899999));
#248477=CARTESIAN_POINT('Ctrl Pts',(-8.82177817700006,11.6,5.89166165899999));
#248478=CARTESIAN_POINT('Ctrl Pts',(-8.82032169200006,15.2,5.89011575499998));
#248479=CARTESIAN_POINT('Ctrl Pts',(-8.82032169200006,11.6,5.89011575499998));
#248480=CARTESIAN_POINT('Ctrl Pts',(-8.81886850900005,15.2,5.88857611299999));
#248481=CARTESIAN_POINT('Ctrl Pts',(-8.81886850900005,11.6,5.88857611299999));
#248482=CARTESIAN_POINT('Ctrl Pts',(-8.81741864900006,15.2,5.88704273299999));
#248483=CARTESIAN_POINT('Ctrl Pts',(-8.81741864900006,11.6,5.88704273299999));
#248484=CARTESIAN_POINT('Ctrl Pts',(-8.81597212600006,15.2,5.88551562099998));
#248485=CARTESIAN_POINT('Ctrl Pts',(-8.81597212600006,11.6,5.88551562099998));
#248486=CARTESIAN_POINT('Ctrl Pts',(-8.81452896000006,15.2,5.88399477899999));
#248487=CARTESIAN_POINT('Ctrl Pts',(-8.81452896000006,11.6,5.88399477899999));
#248488=CARTESIAN_POINT('Ctrl Pts',(-8.81308916900006,15.2,5.88248020899999));
#248489=CARTESIAN_POINT('Ctrl Pts',(-8.81308916900006,11.6,5.88248020899999));
#248490=CARTESIAN_POINT('Ctrl Pts',(-8.81165277000006,15.2,5.88097191699998));
#248491=CARTESIAN_POINT('Ctrl Pts',(-8.81165277000006,11.6,5.88097191699998));
#248492=CARTESIAN_POINT('Ctrl Pts',(-8.81021978200006,15.2,5.87946990199999));
#248493=CARTESIAN_POINT('Ctrl Pts',(-8.81021978200006,11.6,5.87946990199999));
#248494=CARTESIAN_POINT('Ctrl Pts',(-8.80879022300006,15.2,5.87797416799998));
#248495=CARTESIAN_POINT('Ctrl Pts',(-8.80879022300006,11.6,5.87797416799998));
#248496=CARTESIAN_POINT('Ctrl Pts',(-8.80736411200006,15.2,5.87648471999999));
#248497=CARTESIAN_POINT('Ctrl Pts',(-8.80736411200006,11.6,5.87648471999999));
#248498=CARTESIAN_POINT('Ctrl Pts',(-8.80594146500006,15.2,5.87500155999999));
#248499=CARTESIAN_POINT('Ctrl Pts',(-8.80594146500006,11.6,5.87500155999999));
#248500=CARTESIAN_POINT('Ctrl Pts',(-8.80452230200006,15.2,5.87352468799998));
#248501=CARTESIAN_POINT('Ctrl Pts',(-8.80452230200006,11.6,5.87352468799998));
#248502=CARTESIAN_POINT('Ctrl Pts',(-8.80310664300006,15.2,5.87205411199999));
#248503=CARTESIAN_POINT('Ctrl Pts',(-8.80310664300006,11.6,5.87205411199999));
#248504=CARTESIAN_POINT('Ctrl Pts',(-8.80169450400006,15.2,5.87058983199999));
#248505=CARTESIAN_POINT('Ctrl Pts',(-8.80169450400006,11.6,5.87058983199999));
#248506=CARTESIAN_POINT('Ctrl Pts',(-8.80028590400006,15.2,5.86913184999998));
#248507=CARTESIAN_POINT('Ctrl Pts',(-8.80028590400006,11.6,5.86913184999998));
#248508=CARTESIAN_POINT('Ctrl Pts',(-8.79888086200006,15.2,5.86768017199999));
#248509=CARTESIAN_POINT('Ctrl Pts',(-8.79888086200006,11.6,5.86768017199999));
#248510=CARTESIAN_POINT('Ctrl Pts',(-8.79747939700006,15.2,5.86623479899998));
#248511=CARTESIAN_POINT('Ctrl Pts',(-8.79747939700006,11.6,5.86623479899998));
#248512=CARTESIAN_POINT('Ctrl Pts',(-8.79608152800006,15.2,5.86479573299999));
#248513=CARTESIAN_POINT('Ctrl Pts',(-8.79608152800006,11.6,5.86479573299999));
#248514=CARTESIAN_POINT('Ctrl Pts',(-8.79468727200006,15.2,5.86336297899998));
#248515=CARTESIAN_POINT('Ctrl Pts',(-8.79468727200006,11.6,5.86336297899998));
#248516=CARTESIAN_POINT('Ctrl Pts',(-8.79329665000006,15.2,5.86193653899999));
#248517=CARTESIAN_POINT('Ctrl Pts',(-8.79329665000006,11.6,5.86193653899999));
#248518=CARTESIAN_POINT('Ctrl Pts',(-8.79190968000006,15.2,5.86051641499999));
#248519=CARTESIAN_POINT('Ctrl Pts',(-8.79190968000006,11.6,5.86051641499999));
#248520=CARTESIAN_POINT('Ctrl Pts',(-8.79052638100006,15.2,5.85910261299999));
#248521=CARTESIAN_POINT('Ctrl Pts',(-8.79052638100006,11.6,5.85910261299999));
#248522=CARTESIAN_POINT('Ctrl Pts',(-8.78914677300006,15.2,5.85769513199998));
#248523=CARTESIAN_POINT('Ctrl Pts',(-8.78914677300006,11.6,5.85769513199998));
#248524=CARTESIAN_POINT('Ctrl Pts',(-8.78777087400006,15.2,5.85629397699999));
#248525=CARTESIAN_POINT('Ctrl Pts',(-8.78777087400006,11.6,5.85629397699999));
#248526=CARTESIAN_POINT('Ctrl Pts',(-8.78639870300006,15.2,5.85489915099998));
#248527=CARTESIAN_POINT('Ctrl Pts',(-8.78639870300006,11.6,5.85489915099998));
#248528=CARTESIAN_POINT('Ctrl Pts',(-8.78503028000006,15.2,5.85351065699999));
#248529=CARTESIAN_POINT('Ctrl Pts',(-8.78503028000006,11.6,5.85351065699999));
#248530=CARTESIAN_POINT('Ctrl Pts',(-8.78366562500006,15.2,5.85212849699998));
#248531=CARTESIAN_POINT('Ctrl Pts',(-8.78366562500006,11.6,5.85212849699998));
#248532=CARTESIAN_POINT('Ctrl Pts',(-8.78230475700006,15.2,5.85075267399999));
#248533=CARTESIAN_POINT('Ctrl Pts',(-8.78230475700006,11.6,5.85075267399999));
#248534=CARTESIAN_POINT('Ctrl Pts',(-8.78094769300005,15.2,5.84938319199999));
#248535=CARTESIAN_POINT('Ctrl Pts',(-8.78094769300005,11.6,5.84938319199999));
#248536=CARTESIAN_POINT('Ctrl Pts',(-8.77959445700006,15.2,5.84802005299998));
#248537=CARTESIAN_POINT('Ctrl Pts',(-8.77959445700006,11.6,5.84802005299998));
#248538=CARTESIAN_POINT('Ctrl Pts',(-8.77824506500006,15.2,5.84666325999999));
#248539=CARTESIAN_POINT('Ctrl Pts',(-8.77824506500006,11.6,5.84666325999999));
#248540=CARTESIAN_POINT('Ctrl Pts',(-8.77689953800006,15.2,5.84531281599999));
#248541=CARTESIAN_POINT('Ctrl Pts',(-8.77689953800006,11.6,5.84531281599999));
#248542=CARTESIAN_POINT('Ctrl Pts',(-8.77555789700006,15.2,5.84396872499998));
#248543=CARTESIAN_POINT('Ctrl Pts',(-8.77555789700006,11.6,5.84396872499998));
#248544=CARTESIAN_POINT('Ctrl Pts',(-8.77422015900006,15.2,5.84263098799998));
#248545=CARTESIAN_POINT('Ctrl Pts',(-8.77422015900006,11.6,5.84263098799998));
#248546=CARTESIAN_POINT('Ctrl Pts',(-8.77288634600006,15.2,5.84129960899999));
#248547=CARTESIAN_POINT('Ctrl Pts',(-8.77288634600006,11.6,5.84129960899999));
#248548=CARTESIAN_POINT('Ctrl Pts',(-8.77155647800006,15.2,5.83997458999999));
#248549=CARTESIAN_POINT('Ctrl Pts',(-8.77155647800006,11.6,5.83997458999999));
#248550=CARTESIAN_POINT('Ctrl Pts',(-8.77023057400006,15.2,5.83865593399998));
#248551=CARTESIAN_POINT('Ctrl Pts',(-8.77023057400006,11.6,5.83865593399998));
#248552=CARTESIAN_POINT('Ctrl Pts',(-8.76890865500006,15.2,5.83734364499998));
#248553=CARTESIAN_POINT('Ctrl Pts',(-8.76890865500006,11.6,5.83734364499998));
#248554=CARTESIAN_POINT('Ctrl Pts',(-8.76759074100006,15.2,5.83603772599999));
#248555=CARTESIAN_POINT('Ctrl Pts',(-8.76759074100006,11.6,5.83603772599999));
#248556=CARTESIAN_POINT('Ctrl Pts',(-8.76627685200006,15.2,5.83473817899999));
#248557=CARTESIAN_POINT('Ctrl Pts',(-8.76627685200006,11.6,5.83473817899999));
#248558=CARTESIAN_POINT('Ctrl Pts',(-8.76496700900006,15.2,5.83344500699998));
#248559=CARTESIAN_POINT('Ctrl Pts',(-8.76496700900006,11.6,5.83344500699998));
#248560=CARTESIAN_POINT('Ctrl Pts',(-8.76366123100006,15.2,5.83215821299999));
#248561=CARTESIAN_POINT('Ctrl Pts',(-8.76366123100006,11.6,5.83215821299999));
#248562=CARTESIAN_POINT('Ctrl Pts',(-8.76235953900006,15.2,5.83087779999998));
#248563=CARTESIAN_POINT('Ctrl Pts',(-8.76235953900006,11.6,5.83087779999998));
#248564=CARTESIAN_POINT('Ctrl Pts',(-8.76106195600006,15.2,5.82960376999999));
#248565=CARTESIAN_POINT('Ctrl Pts',(-8.76106195600006,11.6,5.82960376999999));
#248566=CARTESIAN_POINT('Ctrl Pts',(-8.75976849800006,15.2,5.82833612699999));
#248567=CARTESIAN_POINT('Ctrl Pts',(-8.75976849800006,11.6,5.82833612699999));
#248568=CARTESIAN_POINT('Ctrl Pts',(-8.75847919000006,15.2,5.82707487399999));
#248569=CARTESIAN_POINT('Ctrl Pts',(-8.75847919000006,11.6,5.82707487399999));
#248570=CARTESIAN_POINT('Ctrl Pts',(-8.75719405100006,15.2,5.82582001299999));
#248571=CARTESIAN_POINT('Ctrl Pts',(-8.75719405100006,11.6,5.82582001299999));
#248572=CARTESIAN_POINT('Ctrl Pts',(-8.75591310200006,15.2,5.82457154599999));
#248573=CARTESIAN_POINT('Ctrl Pts',(-8.75591310200006,11.6,5.82457154599999));
#248574=CARTESIAN_POINT('Ctrl Pts',(-8.75463636300006,15.2,5.82332947899998));
#248575=CARTESIAN_POINT('Ctrl Pts',(-8.75463636300006,11.6,5.82332947899998));
#248576=CARTESIAN_POINT('Ctrl Pts',(-8.75336385700006,15.2,5.82209381199998));
#248577=CARTESIAN_POINT('Ctrl Pts',(-8.75336385700006,11.6,5.82209381199998));
#248578=CARTESIAN_POINT('Ctrl Pts',(-8.75209560400006,15.2,5.82086454899999));
#248579=CARTESIAN_POINT('Ctrl Pts',(-8.75209560400006,11.6,5.82086454899999));
#248580=CARTESIAN_POINT('Ctrl Pts',(-8.75083162500006,15.2,5.81964169299999));
#248581=CARTESIAN_POINT('Ctrl Pts',(-8.75083162500006,11.6,5.81964169299999));
#248582=CARTESIAN_POINT('Ctrl Pts',(-8.74957194200006,15.2,5.81842524699999));
#248583=CARTESIAN_POINT('Ctrl Pts',(-8.74957194200006,11.6,5.81842524699999));
#248584=CARTESIAN_POINT('Ctrl Pts',(-8.74831657500006,15.2,5.81721521199999));
#248585=CARTESIAN_POINT('Ctrl Pts',(-8.74831657500006,11.6,5.81721521199999));
#248586=CARTESIAN_POINT('Ctrl Pts',(-8.74706554700006,15.2,5.81601159299999));
#248587=CARTESIAN_POINT('Ctrl Pts',(-8.74706554700006,11.6,5.81601159299999));
#248588=CARTESIAN_POINT('Ctrl Pts',(-8.74581887900005,15.2,5.81481439299999));
#248589=CARTESIAN_POINT('Ctrl Pts',(-8.74581887900005,11.6,5.81481439299999));
#248590=CARTESIAN_POINT('Ctrl Pts',(-8.74457659200005,15.2,5.81362361299998));
#248591=CARTESIAN_POINT('Ctrl Pts',(-8.74457659200005,11.6,5.81362361299998));
#248592=CARTESIAN_POINT('Ctrl Pts',(-8.74333870800006,15.2,5.81243925699999));
#248593=CARTESIAN_POINT('Ctrl Pts',(-8.74333870800006,11.6,5.81243925699999));
#248594=CARTESIAN_POINT('Ctrl Pts',(-8.74210524900005,15.2,5.81126132799999));
#248595=CARTESIAN_POINT('Ctrl Pts',(-8.74210524900005,11.6,5.81126132799999));
#248596=CARTESIAN_POINT('Ctrl Pts',(-8.74087623700006,15.2,5.81008982799998));
#248597=CARTESIAN_POINT('Ctrl Pts',(-8.74087623700006,11.6,5.81008982799998));
#248598=CARTESIAN_POINT('Ctrl Pts',(-8.73965169200006,15.2,5.80892475999998));
#248599=CARTESIAN_POINT('Ctrl Pts',(-8.73965169200006,11.6,5.80892475999998));
#248600=CARTESIAN_POINT('Ctrl Pts',(-8.73843163900006,15.2,5.80776612799998));
#248601=CARTESIAN_POINT('Ctrl Pts',(-8.73843163900006,11.6,5.80776612799998));
#248602=CARTESIAN_POINT('Ctrl Pts',(-8.73721609900005,15.2,5.80661393499999));
#248603=CARTESIAN_POINT('Ctrl Pts',(-8.73721609900005,11.6,5.80661393499999));
#248604=CARTESIAN_POINT('Ctrl Pts',(-8.73600509400006,15.2,5.80546818099998));
#248605=CARTESIAN_POINT('Ctrl Pts',(-8.73600509400006,11.6,5.80546818099998));
#248606=CARTESIAN_POINT('Ctrl Pts',(-8.73479864500006,15.2,5.80432887199999));
#248607=CARTESIAN_POINT('Ctrl Pts',(-8.73479864500006,11.6,5.80432887199999));
#248608=CARTESIAN_POINT('Ctrl Pts',(-8.73359677600006,15.2,5.80319600899998));
#248609=CARTESIAN_POINT('Ctrl Pts',(-8.73359677600006,11.6,5.80319600899998));
#248610=CARTESIAN_POINT('Ctrl Pts',(-8.73239951000006,15.2,5.80206959599998));
#248611=CARTESIAN_POINT('Ctrl Pts',(-8.73239951000006,11.6,5.80206959599998));
#248612=CARTESIAN_POINT('Ctrl Pts',(-8.73120686700006,15.2,5.80094963499998));
#248613=CARTESIAN_POINT('Ctrl Pts',(-8.73120686700006,11.6,5.80094963499998));
#248614=CARTESIAN_POINT('Ctrl Pts',(-8.73001887200006,15.2,5.79983612899999));
#248615=CARTESIAN_POINT('Ctrl Pts',(-8.73001887200006,11.6,5.79983612899999));
#248616=CARTESIAN_POINT('Ctrl Pts',(-8.72883554600006,15.2,5.79872908099999));
#248617=CARTESIAN_POINT('Ctrl Pts',(-8.72883554600006,11.6,5.79872908099999));
#248618=CARTESIAN_POINT('Ctrl Pts',(-8.72765691300006,15.2,5.79762849299998));
#248619=CARTESIAN_POINT('Ctrl Pts',(-8.72765691300006,11.6,5.79762849299998));
#248620=CARTESIAN_POINT('Ctrl Pts',(-8.72648299600005,15.2,5.79653436899999));
#248621=CARTESIAN_POINT('Ctrl Pts',(-8.72648299600005,11.6,5.79653436899999));
#248622=CARTESIAN_POINT('Ctrl Pts',(-8.72531381600006,15.2,5.79544671199999));
#248623=CARTESIAN_POINT('Ctrl Pts',(-8.72531381600006,11.6,5.79544671199999));
#248624=CARTESIAN_POINT('Ctrl Pts',(-8.72414939900005,15.2,5.79436552399999));
#248625=CARTESIAN_POINT('Ctrl Pts',(-8.72414939900005,11.6,5.79436552399999));
#248626=CARTESIAN_POINT('Ctrl Pts',(-8.72298976600005,15.2,5.79329080799998));
#248627=CARTESIAN_POINT('Ctrl Pts',(-8.72298976600005,11.6,5.79329080799998));
#248628=CARTESIAN_POINT('Ctrl Pts',(-8.72183494200006,15.2,5.79222256599999));
#248629=CARTESIAN_POINT('Ctrl Pts',(-8.72183494200006,11.6,5.79222256599999));
#248630=CARTESIAN_POINT('Ctrl Pts',(-8.72068494800006,15.2,5.79116080199999));
#248631=CARTESIAN_POINT('Ctrl Pts',(-8.72068494800006,11.6,5.79116080199999));
#248632=CARTESIAN_POINT('Ctrl Pts',(-8.71953981000006,15.2,5.79010551899999));
#248633=CARTESIAN_POINT('Ctrl Pts',(-8.71953981000006,11.6,5.79010551899999));
#248634=CARTESIAN_POINT('Ctrl Pts',(-8.71839954900006,15.2,5.78905671899999));
#248635=CARTESIAN_POINT('Ctrl Pts',(-8.71839954900006,11.6,5.78905671899999));
#248636=CARTESIAN_POINT('Ctrl Pts',(-8.71726419000005,15.2,5.78801440599998));
#248637=CARTESIAN_POINT('Ctrl Pts',(-8.71726419000005,11.6,5.78801440599998));
#248638=CARTESIAN_POINT('Ctrl Pts',(-8.71613375600005,15.2,5.78697858099999));
#248639=CARTESIAN_POINT('Ctrl Pts',(-8.71613375600005,11.6,5.78697858099999));
#248640=CARTESIAN_POINT('Ctrl Pts',(-8.71500827300006,15.2,5.78594924699999));
#248641=CARTESIAN_POINT('Ctrl Pts',(-8.71500827300006,11.6,5.78594924699999));
#248642=CARTESIAN_POINT('Ctrl Pts',(-8.71388776300006,15.2,5.78492640799999));
#248643=CARTESIAN_POINT('Ctrl Pts',(-8.71388776300006,11.6,5.78492640799999));
#248644=CARTESIAN_POINT('Ctrl Pts',(-8.71277225000006,15.2,5.78391006599999));
#248645=CARTESIAN_POINT('Ctrl Pts',(-8.71277225000006,11.6,5.78391006599999));
#248646=CARTESIAN_POINT('Ctrl Pts',(-8.71166175800006,15.2,5.78290022499999));
#248647=CARTESIAN_POINT('Ctrl Pts',(-8.71166175800006,11.6,5.78290022499999));
#248648=CARTESIAN_POINT('Ctrl Pts',(-8.71055631300005,15.2,5.78189688699998));
#248649=CARTESIAN_POINT('Ctrl Pts',(-8.71055631300005,11.6,5.78189688699998));
#248650=CARTESIAN_POINT('Ctrl Pts',(-8.70945593700006,15.2,5.78090005399999));
#248651=CARTESIAN_POINT('Ctrl Pts',(-8.70945593700006,11.6,5.78090005399999));
#248652=CARTESIAN_POINT('Ctrl Pts',(-8.70836065600006,15.2,5.77990972999999));
#248653=CARTESIAN_POINT('Ctrl Pts',(-8.70836065600006,11.6,5.77990972999999));
#248654=CARTESIAN_POINT('Ctrl Pts',(-8.70727049400006,15.2,5.77892591699998));
#248655=CARTESIAN_POINT('Ctrl Pts',(-8.70727049400006,11.6,5.77892591699998));
#248656=CARTESIAN_POINT('Ctrl Pts',(-8.70618547400005,15.2,5.77794861799998));
#248657=CARTESIAN_POINT('Ctrl Pts',(-8.70618547400005,11.6,5.77794861799998));
#248658=CARTESIAN_POINT('Ctrl Pts',(-8.70510562500005,15.2,5.77697783599999));
#248659=CARTESIAN_POINT('Ctrl Pts',(-8.70510562500005,11.6,5.77697783599999));
#248660=CARTESIAN_POINT('Ctrl Pts',(-8.70403096800005,15.2,5.77601357299999));
#248661=CARTESIAN_POINT('Ctrl Pts',(-8.70403096800005,11.6,5.77601357299999));
#248662=CARTESIAN_POINT('Ctrl Pts',(-8.70296152800006,15.2,5.77505583299998));
#248663=CARTESIAN_POINT('Ctrl Pts',(-8.70296152800006,11.6,5.77505583299998));
#248664=CARTESIAN_POINT('Ctrl Pts',(-8.70189733300006,15.2,5.77410461799998));
#248665=CARTESIAN_POINT('Ctrl Pts',(-8.70189733300006,11.6,5.77410461799998));
#248666=CARTESIAN_POINT('Ctrl Pts',(-8.70083840400006,15.2,5.77315993199999));
#248667=CARTESIAN_POINT('Ctrl Pts',(-8.70083840400006,11.6,5.77315993199999));
#248668=CARTESIAN_POINT('Ctrl Pts',(-8.69978477000006,15.2,5.77222177599998));
#248669=CARTESIAN_POINT('Ctrl Pts',(-8.69978477000006,11.6,5.77222177599998));
#248670=CARTESIAN_POINT('Ctrl Pts',(-8.69873645500006,15.2,5.77129015299998));
#248671=CARTESIAN_POINT('Ctrl Pts',(-8.69873645500006,11.6,5.77129015299998));
#248672=CARTESIAN_POINT('Ctrl Pts',(-8.69769348400006,15.2,5.77036506799999));
#248673=CARTESIAN_POINT('Ctrl Pts',(-8.69769348400006,11.6,5.77036506799999));
#248674=CARTESIAN_POINT('Ctrl Pts',(-8.69665588300006,15.2,5.76944652099999));
#248675=CARTESIAN_POINT('Ctrl Pts',(-8.69665588300006,11.6,5.76944652099999));
#248676=CARTESIAN_POINT('Ctrl Pts',(-8.69562367700006,15.2,5.76853451599998));
#248677=CARTESIAN_POINT('Ctrl Pts',(-8.69562367700006,11.6,5.76853451599998));
#248678=CARTESIAN_POINT('Ctrl Pts',(-8.69459689400006,15.2,5.76762905499999));
#248679=CARTESIAN_POINT('Ctrl Pts',(-8.69459689400006,11.6,5.76762905499999));
#248680=CARTESIAN_POINT('Ctrl Pts',(-8.69357555800006,15.2,5.76673014199999));
#248681=CARTESIAN_POINT('Ctrl Pts',(-8.69357555800006,11.6,5.76673014199999));
#248682=CARTESIAN_POINT('Ctrl Pts',(-8.69255969400006,15.2,5.76583777999998));
#248683=CARTESIAN_POINT('Ctrl Pts',(-8.69255969400006,11.6,5.76583777999998));
#248684=CARTESIAN_POINT('Ctrl Pts',(-8.69154933000006,15.2,5.76495196899998));
#248685=CARTESIAN_POINT('Ctrl Pts',(-8.69154933000006,11.6,5.76495196899998));
#248686=CARTESIAN_POINT('Ctrl Pts',(-8.69054449300006,15.2,5.76407271599999));
#248687=CARTESIAN_POINT('Ctrl Pts',(-8.69054449300006,11.6,5.76407271599999));
#248688=CARTESIAN_POINT('Ctrl Pts',(-8.68954520600006,15.2,5.76320001999999));
#248689=CARTESIAN_POINT('Ctrl Pts',(-8.68954520600006,11.6,5.76320001999999));
#248690=CARTESIAN_POINT('Ctrl Pts',(-8.68855149800006,15.2,5.76233388499999));
#248691=CARTESIAN_POINT('Ctrl Pts',(-8.68855149800006,11.6,5.76233388499999));
#248692=CARTESIAN_POINT('Ctrl Pts',(-8.68756339700005,15.2,5.76147431599999));
#248693=CARTESIAN_POINT('Ctrl Pts',(-8.68756339700005,11.6,5.76147431599999));
#248694=CARTESIAN_POINT('Ctrl Pts',(-8.68658092700005,15.2,5.76062131199999));
#248695=CARTESIAN_POINT('Ctrl Pts',(-8.68658092700005,11.6,5.76062131199999));
#248696=CARTESIAN_POINT('Ctrl Pts',(-8.68560411500006,15.2,5.75977487799998));
#248697=CARTESIAN_POINT('Ctrl Pts',(-8.68560411500006,11.6,5.75977487799998));
#248698=CARTESIAN_POINT('Ctrl Pts',(-8.68463299000006,15.2,5.75893501599998));
#248699=CARTESIAN_POINT('Ctrl Pts',(-8.68463299000006,11.6,5.75893501599998));
#248700=CARTESIAN_POINT('Ctrl Pts',(-8.68366757600005,15.2,5.75810172899998));
#248701=CARTESIAN_POINT('Ctrl Pts',(-8.68366757600005,11.6,5.75810172899998));
#248702=CARTESIAN_POINT('Ctrl Pts',(-8.68270790300006,15.2,5.75727502099999));
#248703=CARTESIAN_POINT('Ctrl Pts',(-8.68270790300006,11.6,5.75727502099999));
#248704=CARTESIAN_POINT('Ctrl Pts',(-8.68175399700006,15.2,5.75645489199999));
#248705=CARTESIAN_POINT('Ctrl Pts',(-8.68175399700006,11.6,5.75645489199999));
#248706=CARTESIAN_POINT('Ctrl Pts',(-8.68080588600005,15.2,5.75564134699999));
#248707=CARTESIAN_POINT('Ctrl Pts',(-8.68080588600005,11.6,5.75564134699999));
#248708=CARTESIAN_POINT('Ctrl Pts',(-8.67986359800006,15.2,5.75483438799999));
#248709=CARTESIAN_POINT('Ctrl Pts',(-8.67986359800006,11.6,5.75483438799999));
#248710=CARTESIAN_POINT('Ctrl Pts',(-8.67892715900006,15.2,5.75403401799999));
#248711=CARTESIAN_POINT('Ctrl Pts',(-8.67892715900006,11.6,5.75403401799999));
#248712=CARTESIAN_POINT('Ctrl Pts',(-8.67799659800006,15.2,5.75324023999999));
#248713=CARTESIAN_POINT('Ctrl Pts',(-8.67799659800006,11.6,5.75324023999999));
#248714=CARTESIAN_POINT('Ctrl Pts',(-8.67707194300005,15.2,5.75245305599999));
#248715=CARTESIAN_POINT('Ctrl Pts',(-8.67707194300005,11.6,5.75245305599999));
#248716=CARTESIAN_POINT('Ctrl Pts',(-8.67615322100006,15.2,5.75167246799998));
#248717=CARTESIAN_POINT('Ctrl Pts',(-8.67615322100006,11.6,5.75167246799998));
#248718=CARTESIAN_POINT('Ctrl Pts',(-8.67524046200005,15.2,5.75089848099999));
#248719=CARTESIAN_POINT('Ctrl Pts',(-8.67524046200005,11.6,5.75089848099999));
#248720=CARTESIAN_POINT('Ctrl Pts',(-8.67433369300005,15.2,5.75013109599999));
#248721=CARTESIAN_POINT('Ctrl Pts',(-8.67433369300005,11.6,5.75013109599999));
#248722=CARTESIAN_POINT('Ctrl Pts',(-8.67343294200005,15.2,5.74937031599998));
#248723=CARTESIAN_POINT('Ctrl Pts',(-8.67343294200005,11.6,5.74937031599998));
#248724=CARTESIAN_POINT('Ctrl Pts',(-8.67253824000005,15.2,5.74861614399998));
#248725=CARTESIAN_POINT('Ctrl Pts',(-8.67253824000005,11.6,5.74861614399998));
#248726=CARTESIAN_POINT('Ctrl Pts',(-8.67164961300006,15.2,5.74786858299999));
#248727=CARTESIAN_POINT('Ctrl Pts',(-8.67164961300006,11.6,5.74786858299999));
#248728=CARTESIAN_POINT('Ctrl Pts',(-8.67076709100006,15.2,5.74712763599998));
#248729=CARTESIAN_POINT('Ctrl Pts',(-8.67076709100006,11.6,5.74712763599998));
#248730=CARTESIAN_POINT('Ctrl Pts',(-8.66989070400006,15.2,5.74639330399998));
#248731=CARTESIAN_POINT('Ctrl Pts',(-8.66989070400006,11.6,5.74639330399998));
#248732=CARTESIAN_POINT('Ctrl Pts',(-8.66902047900006,15.2,5.74566559199998));
#248733=CARTESIAN_POINT('Ctrl Pts',(-8.66902047900006,11.6,5.74566559199998));
#248734=CARTESIAN_POINT('Ctrl Pts',(-8.66815644700005,15.2,5.74494450199998));
#248735=CARTESIAN_POINT('Ctrl Pts',(-8.66815644700005,11.6,5.74494450199998));
#248736=CARTESIAN_POINT('Ctrl Pts',(-8.66729863700006,15.2,5.74423003599998));
#248737=CARTESIAN_POINT('Ctrl Pts',(-8.66729863700006,11.6,5.74423003599998));
#248738=CARTESIAN_POINT('Ctrl Pts',(-8.66644707700006,15.2,5.74352219699998));
#248739=CARTESIAN_POINT('Ctrl Pts',(-8.66644707700006,11.6,5.74352219699998));
#248740=CARTESIAN_POINT('Ctrl Pts',(-8.66560179900006,15.2,5.74282098699998));
#248741=CARTESIAN_POINT('Ctrl Pts',(-8.66560179900006,11.6,5.74282098699998));
#248742=CARTESIAN_POINT('Ctrl Pts',(-8.66476283200006,15.2,5.74212641099999));
#248743=CARTESIAN_POINT('Ctrl Pts',(-8.66476283200006,11.6,5.74212641099999));
#248744=CARTESIAN_POINT('Ctrl Pts',(-8.66393020600006,15.2,5.74143846999998));
#248745=CARTESIAN_POINT('Ctrl Pts',(-8.66393020600006,11.6,5.74143846999998));
#248746=CARTESIAN_POINT('Ctrl Pts',(-8.66310395100006,15.2,5.74075716599998));
#248747=CARTESIAN_POINT('Ctrl Pts',(-8.66310395100006,11.6,5.74075716599998));
#248748=CARTESIAN_POINT('Ctrl Pts',(-8.66228409600006,15.2,5.74008250399999));
#248749=CARTESIAN_POINT('Ctrl Pts',(-8.66228409600006,11.6,5.74008250399999));
#248750=CARTESIAN_POINT('Ctrl Pts',(-8.66147067400006,15.2,5.73941448499999));
#248751=CARTESIAN_POINT('Ctrl Pts',(-8.66147067400006,11.6,5.73941448499999));
#248752=CARTESIAN_POINT('Ctrl Pts',(-8.66066371400006,15.2,5.73875311199998));
#248753=CARTESIAN_POINT('Ctrl Pts',(-8.66066371400006,11.6,5.73875311199998));
#248754=CARTESIAN_POINT('Ctrl Pts',(-8.65986324600006,15.2,5.73809838799999));
#248755=CARTESIAN_POINT('Ctrl Pts',(-8.65986324600006,11.6,5.73809838799999));
#248756=CARTESIAN_POINT('Ctrl Pts',(-8.65906930300006,15.2,5.73745031599999));
#248757=CARTESIAN_POINT('Ctrl Pts',(-8.65906930300006,11.6,5.73745031599999));
#248758=CARTESIAN_POINT('Ctrl Pts',(-8.65828191300006,15.2,5.73680889799999));
#248759=CARTESIAN_POINT('Ctrl Pts',(-8.65828191300006,11.6,5.73680889799999));
#248760=CARTESIAN_POINT('Ctrl Pts',(-8.65750111000006,15.2,5.73617413799998));
#248761=CARTESIAN_POINT('Ctrl Pts',(-8.65750111000006,11.6,5.73617413799998));
#248762=CARTESIAN_POINT('Ctrl Pts',(-8.65672692500006,15.2,5.73554603699999));
#248763=CARTESIAN_POINT('Ctrl Pts',(-8.65672692500006,11.6,5.73554603699999));
#248764=CARTESIAN_POINT('Ctrl Pts',(-8.65595938700006,15.2,5.73492459899998));
#248765=CARTESIAN_POINT('Ctrl Pts',(-8.65595938700006,11.6,5.73492459899998));
#248766=CARTESIAN_POINT('Ctrl Pts',(-8.65519853100006,15.2,5.73430982499998));
#248767=CARTESIAN_POINT('Ctrl Pts',(-8.65519853100006,11.6,5.73430982499998));
#248768=CARTESIAN_POINT('Ctrl Pts',(-8.65444438600005,15.2,5.73370172099998));
#248769=CARTESIAN_POINT('Ctrl Pts',(-8.65444438600005,11.6,5.73370172099998));
#248770=CARTESIAN_POINT('Ctrl Pts',(-8.65369698500006,15.2,5.73310028599998));
#248771=CARTESIAN_POINT('Ctrl Pts',(-8.65369698500006,11.6,5.73310028599998));
#248772=CARTESIAN_POINT('Ctrl Pts',(-8.65295636100005,15.2,5.73250552499999));
#248773=CARTESIAN_POINT('Ctrl Pts',(-8.65295636100005,11.6,5.73250552499999));
#248774=CARTESIAN_POINT('Ctrl Pts',(-8.65222254500006,15.2,5.73191744099999));
#248775=CARTESIAN_POINT('Ctrl Pts',(-8.65222254500006,11.6,5.73191744099999));
#248776=CARTESIAN_POINT('Ctrl Pts',(-8.65149557000005,15.2,5.73133603499999));
#248777=CARTESIAN_POINT('Ctrl Pts',(-8.65149557000005,11.6,5.73133603499999));
#248778=CARTESIAN_POINT('Ctrl Pts',(-8.65077961600005,15.2,5.73076462099999));
#248779=CARTESIAN_POINT('Ctrl Pts',(-8.65077961600005,11.6,5.73076462099999));
#248780=CARTESIAN_POINT('Ctrl Pts',(-8.65021312700006,15.2,5.73031342099998));
#248781=CARTESIAN_POINT('Ctrl Pts',(-8.65021312700006,11.6,5.73031342099998));
#248782=CARTESIAN_POINT('Ctrl Pts',(-8.64979235000006,15.2,5.72997879199999));
#248783=CARTESIAN_POINT('Ctrl Pts',(-8.64979235000006,11.6,5.72997879199999));
#248784=CARTESIAN_POINT('Ctrl Pts',(-8.64951454400006,15.2,5.72975808599999));
#248785=CARTESIAN_POINT('Ctrl Pts',(-8.64951454400006,11.6,5.72975808599999));
#248786=CARTESIAN_POINT('Ctrl Pts',(-8.64937799900006,15.2,5.72964966099998));
#248787=CARTESIAN_POINT('Ctrl Pts',(-8.64937799900006,11.6,5.72964966099998));
#248788=CARTESIAN_POINT('',(-8.64937799900006,12.2,5.72964966099998));
#248789=CARTESIAN_POINT('',(-8.64937799900006,15.2,5.72964966099998));
#248790=CARTESIAN_POINT('',(-8.64937799900006,12.2,5.72964966099998));
#248791=CARTESIAN_POINT('Ctrl Pts',(-9.36775917500006,12.2,6.67046385499999));
#248792=CARTESIAN_POINT('Ctrl Pts',(-9.36593194966811,12.2,6.66710588438994));
#248793=CARTESIAN_POINT('Ctrl Pts',(-9.36410408846955,12.2,6.66375578663033));
#248794=CARTESIAN_POINT('Ctrl Pts',(-9.36227560168602,12.2,6.66041356487326));
#248795=CARTESIAN_POINT('Ctrl Pts',(-9.3604471149025,12.2,6.6570713431162));
#248796=CARTESIAN_POINT('Ctrl Pts',(-9.35861799862892,12.2,6.65373699652317));
#248797=CARTESIAN_POINT('Ctrl Pts',(-9.35678826960406,12.2,6.65041053364359));
#248798=CARTESIAN_POINT('Ctrl Pts',(-9.3549585405792,12.2,6.64708407076401));
#248799=CARTESIAN_POINT('Ctrl Pts',(-9.35312819903259,12.2,6.64376549048578));
#248800=CARTESIAN_POINT('Ctrl Pts',(-9.35129728493254,12.2,6.64045481048));
#248801=CARTESIAN_POINT('Ctrl Pts',(-9.34946637049987,12.2,6.63714412987279));
#248802=CARTESIAN_POINT('Ctrl Pts',(-9.34763488481701,12.2,6.6338413503261));
#248803=CARTESIAN_POINT('Ctrl Pts',(-9.34580287284235,12.2,6.63054648926499));
#248804=CARTESIAN_POINT('Ctrl Pts',(-9.34336019076417,12.2,6.62615334218112));
#248805=CARTESIAN_POINT('Ctrl Pts',(-9.34091657485832,12.2,6.62177427441485));
#248806=CARTESIAN_POINT('Ctrl Pts',(-9.33847210989155,12.2,6.61740932104856));
#248807=CARTESIAN_POINT('Ctrl Pts',(-9.33663876108321,12.2,6.61413560587517));
#248808=CARTESIAN_POINT('Ctrl Pts',(-9.33480493317988,12.2,6.61086982962563));
#248809=CARTESIAN_POINT('Ctrl Pts',(-9.33297066182161,12.2,6.60761200637198));
#248810=CARTESIAN_POINT('Ctrl Pts',(-9.33113639046334,12.2,6.60435418311835));
#248811=CARTESIAN_POINT('Ctrl Pts',(-9.32930167588341,12.2,6.60110431429001));
#248812=CARTESIAN_POINT('Ctrl Pts',(-9.32746655815845,12.2,6.59786241474));
#248813=CARTESIAN_POINT('Ctrl Pts',(-9.32563144010011,12.2,6.59462051460104));
#248814=CARTESIAN_POINT('Ctrl Pts',(-9.32379591863337,12.2,6.59138658449776));
#248815=CARTESIAN_POINT('Ctrl Pts',(-9.32196003307483,12.2,6.58816064028001));
#248816=CARTESIAN_POINT('Ctrl Pts',(-9.32012414784982,12.2,6.5849346966483));
#248817=CARTESIAN_POINT('Ctrl Pts',(-9.31828789801651,12.2,6.58171673809954));
#248818=CARTESIAN_POINT('Ctrl Pts',(-9.31645132174987,12.2,6.57850678092518));
#248819=CARTESIAN_POINT('Ctrl Pts',(-9.31461474548322,12.2,6.57529682375082));
#248820=CARTESIAN_POINT('Ctrl Pts',(-9.31277784255665,12.2,6.57209486617878));
#248821=CARTESIAN_POINT('Ctrl Pts',(-9.31094065178172,12.2,6.56890092644703));
#248822=CARTESIAN_POINT('Ctrl Pts',(-9.3091034610068,12.2,6.56570698671527));
#248823=CARTESIAN_POINT('Ctrl Pts',(-9.30726598200996,12.2,6.56252106221848));
#248824=CARTESIAN_POINT('Ctrl Pts',(-9.30542825427673,12.2,6.55934317052782));
#248825=CARTESIAN_POINT('Ctrl Pts',(-9.30359052654349,12.2,6.55616527883715));
#248826=CARTESIAN_POINT('Ctrl Pts',(-9.30175254971693,12.2,6.55299541844716));
#248827=CARTESIAN_POINT('Ctrl Pts',(-9.29991436399208,12.2,6.54983360581136));
#248828=CARTESIAN_POINT('Ctrl Pts',(-9.29807617826723,12.2,6.54667179317556));
#248829=CARTESIAN_POINT('Ctrl Pts',(-9.29623778278405,12.2,6.54351802758918));
#248830=CARTESIAN_POINT('Ctrl Pts',(-9.29439921714253,12.2,6.54037232545236));
#248831=CARTESIAN_POINT('Ctrl Pts',(-9.292560651167,12.2,6.53722662274407));
#248832=CARTESIAN_POINT('Ctrl Pts',(-9.29072191578313,12.2,6.53408898272142));
#248833=CARTESIAN_POINT('Ctrl Pts',(-9.28888304884919,12.2,6.5309594210177));
#248834=CARTESIAN_POINT('Ctrl Pts',(-9.28704418224932,12.2,6.52782985988251));
#248835=CARTESIAN_POINT('Ctrl Pts',(-9.28520518586931,12.2,6.52470837647246));
#248836=CARTESIAN_POINT('Ctrl Pts',(-9.2833660986359,12.2,6.52159498718097));
#248837=CARTESIAN_POINT('Ctrl Pts',(-9.2815270114025,12.2,6.51848159788949));
#248838=CARTESIAN_POINT('Ctrl Pts',(-9.2796878344161,12.2,6.5153763027159));
#248839=CARTESIAN_POINT('Ctrl Pts',(-9.27784860631625,12.2,6.51227911616247));
#248840=CARTESIAN_POINT('Ctrl Pts',(-9.2760093782164,12.2,6.50918192960904));
#248841=CARTESIAN_POINT('Ctrl Pts',(-9.27417010034989,12.2,6.50609285228798));
#248842=CARTESIAN_POINT('Ctrl Pts',(-9.27233081270839,12.2,6.50301189923325));
#248843=CARTESIAN_POINT('Ctrl Pts',(-9.27049152506689,12.2,6.49993094617853));
#248844=CARTESIAN_POINT('Ctrl Pts',(-9.26865222811705,12.2,6.49685811820683));
#248845=CARTESIAN_POINT('Ctrl Pts',(-9.26681296143387,12.2,6.49379343006745));
#248846=CARTESIAN_POINT('Ctrl Pts',(-9.26497369475068,12.2,6.49072874192807));
#248847=CARTESIAN_POINT('Ctrl Pts',(-9.26313445886751,12.2,6.48767219308817));
#248848=CARTESIAN_POINT('Ctrl Pts',(-9.26129529518433,12.2,6.48462379990615));
#248849=CARTESIAN_POINT('Ctrl Pts',(-9.25884307671734,12.2,6.48055927529426));
#248850=CARTESIAN_POINT('Ctrl Pts',(-9.25639098632924,12.2,6.47650924741871));
#248851=CARTESIAN_POINT('Ctrl Pts',(-9.25393912124005,12.2,6.47247375551385));
#248852=CARTESIAN_POINT('Ctrl Pts',(-9.25210022259019,12.2,6.46944713686012));
#248853=CARTESIAN_POINT('Ctrl Pts',(-9.25026145087661,12.2,6.46642869339033));
#248854=CARTESIAN_POINT('Ctrl Pts',(-9.24842284722673,12.2,6.463418441236));
#248855=CARTESIAN_POINT('Ctrl Pts',(-9.24658424357685,12.2,6.46040818908167));
#248856=CARTESIAN_POINT('Ctrl Pts',(-9.24474580820033,12.2,6.45740612750167));
#248857=CARTESIAN_POINT('Ctrl Pts',(-9.24290758443376,12.2,6.45441227285973));
#248858=CARTESIAN_POINT('Ctrl Pts',(-9.24106936066718,12.2,6.45141841821777));
#248859=CARTESIAN_POINT('Ctrl Pts',(-9.23923134628396,12.2,6.44843276964197));
#248860=CARTESIAN_POINT('Ctrl Pts',(-9.23739358464235,12.2,6.44545534212401));
#248861=CARTESIAN_POINT('Ctrl Pts',(-9.23555582266689,12.2,6.44247791406516));
#248862=CARTESIAN_POINT('Ctrl Pts',(-9.23371831353318,12.2,6.43950870846698));
#248863=CARTESIAN_POINT('Ctrl Pts',(-9.23188109905788,12.2,6.43654773932945));
#248864=CARTESIAN_POINT('Ctrl Pts',(-9.23004388491633,12.2,6.43358677072982));
#248865=CARTESIAN_POINT('Ctrl Pts',(-9.22820696566972,12.2,6.4306340386695));
#248866=CARTESIAN_POINT('Ctrl Pts',(-9.22637038389473,12.2,6.42768955892199));
#248867=CARTESIAN_POINT('Ctrl Pts',(-9.22453380211974,12.2,6.42474507917449));
#248868=CARTESIAN_POINT('Ctrl Pts',(-9.22269755719989,12.2,6.42180885225716));
#248869=CARTESIAN_POINT('Ctrl Pts',(-9.22086169351662,12.2,6.41888089165592));
#248870=CARTESIAN_POINT('Ctrl Pts',(-9.21902582983335,12.2,6.41595293105468));
#248871=CARTESIAN_POINT('Ctrl Pts',(-9.21719034693338,12.2,6.41303323766081));
#248872=CARTESIAN_POINT('Ctrl Pts',(-9.21535528729172,12.2,6.41012182705826));
#248873=CARTESIAN_POINT('Ctrl Pts',(-9.21352022765006,12.2,6.4072104164557));
#248874=CARTESIAN_POINT('Ctrl Pts',(-9.21168559163339,12.2,6.40430728882782));
#248875=CARTESIAN_POINT('Ctrl Pts',(-9.20985142294998,12.2,6.40141245830727));
#248876=CARTESIAN_POINT('Ctrl Pts',(-9.20801725426658,12.2,6.39851762778672));
#248877=CARTESIAN_POINT('Ctrl Pts',(-9.20618355169643,12.2,6.39563109548038));
#248878=CARTESIAN_POINT('Ctrl Pts',(-9.20435036137973,12.2,6.39275287527354));
#248879=CARTESIAN_POINT('Ctrl Pts',(-9.20251717106304,12.2,6.3898746550667));
#248880=CARTESIAN_POINT('Ctrl Pts',(-9.20068449099963,12.2,6.38700474830425));
#248881=CARTESIAN_POINT('Ctrl Pts',(-9.19885236589946,12.2,6.38414316961542));
#248882=CARTESIAN_POINT('Ctrl Pts',(-9.19702024046645,12.2,6.38128159040674));
#248883=CARTESIAN_POINT('Ctrl Pts',(-9.19518867038359,12.2,6.37842833809208));
#248884=CARTESIAN_POINT('Ctrl Pts',(-9.19335770036757,12.2,6.37558342988809));
#248885=CARTESIAN_POINT('Ctrl Pts',(-9.19091640756726,12.2,6.37179021981081));
#248886=CARTESIAN_POINT('Ctrl Pts',(-9.18847617881958,12.2,6.36801184220659));
#248887=CARTESIAN_POINT('Ctrl Pts',(-9.18603712274112,12.2,6.36424833229107));
#248888=CARTESIAN_POINT('Ctrl Pts',(-9.18420783059919,12.2,6.36142569972623));
#248889=CARTESIAN_POINT('Ctrl Pts',(-9.18237919726203,12.2,6.35861143098206));
#248890=CARTESIAN_POINT('Ctrl Pts',(-9.18055126761205,12.2,6.35580553981788));
#248891=CARTESIAN_POINT('Ctrl Pts',(-9.17872333796207,12.2,6.35299964865369));
#248892=CARTESIAN_POINT('Ctrl Pts',(-9.17689611279862,12.2,6.35020213707442));
#248893=CARTESIAN_POINT('Ctrl Pts',(-9.17506963715655,12.2,6.34741301759129));
#248894=CARTESIAN_POINT('Ctrl Pts',(-9.17263433607925,12.2,6.34369419127598));
#248895=CARTESIAN_POINT('Ctrl Pts',(-9.17020036558262,12.2,6.33999028752041));
#248896=CARTESIAN_POINT('Ctrl Pts',(-9.16776783778339,12.2,6.3363013410416));
#248897=CARTESIAN_POINT('Ctrl Pts',(-9.16533530998416,12.2,6.33261239456279));
#248898=CARTESIAN_POINT('Ctrl Pts',(-9.16290422149898,12.2,6.32893840566626));
#248899=CARTESIAN_POINT('Ctrl Pts',(-9.16047468331115,12.2,6.32527940913502));
#248900=CARTESIAN_POINT('Ctrl Pts',(-9.15804514545435,12.2,6.32162041310232));
#248901=CARTESIAN_POINT('Ctrl Pts',(-9.15561715778105,12.2,6.31797640999172));
#248902=CARTESIAN_POINT('Ctrl Pts',(-9.15319083096837,12.2,6.31434743599407));
#248903=CARTESIAN_POINT('Ctrl Pts',(-9.1507645038251,12.2,6.31071846150197));
#248904=CARTESIAN_POINT('Ctrl Pts',(-9.14833983662467,12.2,6.30710451497278));
#248905=CARTESIAN_POINT('Ctrl Pts',(-9.14591694160391,12.2,6.30350563244485));
#248906=CARTESIAN_POINT('Ctrl Pts',(-9.14349404691327,12.2,6.29990675040727));
#248907=CARTESIAN_POINT('Ctrl Pts',(-9.14107292279186,12.2,6.29632293317329));
#248908=CARTESIAN_POINT('Ctrl Pts',(-9.13865368348951,12.2,6.29275421457515));
#248909=CARTESIAN_POINT('Ctrl Pts',(-9.13623444385753,12.2,6.28918549549077));
#248910=CARTESIAN_POINT('Ctrl Pts',(-9.13381708881282,12.2,6.28563187595487));
#248911=CARTESIAN_POINT('Ctrl Pts',(-9.13140173044958,12.2,6.28209339125322));
#248912=CARTESIAN_POINT('Ctrl Pts',(-9.12898637241543,12.2,6.2785549070337));
#248913=CARTESIAN_POINT('Ctrl Pts',(-9.12657301199467,12.2,6.27503155752053));
#248914=CARTESIAN_POINT('Ctrl Pts',(-9.12416176341385,12.2,6.27152337752852));
#248915=CARTESIAN_POINT('Ctrl Pts',(-9.12175051450449,12.2,6.26801519705854));
#248916=CARTESIAN_POINT('Ctrl Pts',(-9.11934137829824,12.2,6.26452218700155));
#248917=CARTESIAN_POINT('Ctrl Pts',(-9.1169344687783,12.2,6.26104438242409));
#248918=CARTESIAN_POINT('Ctrl Pts',(-9.11452755958629,12.2,6.25756657832047));
#248919=CARTESIAN_POINT('Ctrl Pts',(-9.11212287863636,12.2,6.25410397852805));
#248920=CARTESIAN_POINT('Ctrl Pts',(-9.10972054132365,12.2,6.25065661969191));
#248921=CARTESIAN_POINT('Ctrl Pts',(-9.10731820368362,12.2,6.24720926038604));
#248922=CARTESIAN_POINT('Ctrl Pts',(-9.10491821142067,12.2,6.24377714246149));
#248923=CARTESIAN_POINT('Ctrl Pts',(-9.10252067934574,12.2,6.24036029872075));
#248924=CARTESIAN_POINT('Ctrl Pts',(-9.10012314759748,12.2,6.23694345544554));
#248925=CARTESIAN_POINT('Ctrl Pts',(-9.09772807875701,12.2,6.23354188810056));
#248926=CARTESIAN_POINT('Ctrl Pts',(-9.09533559017455,12.2,6.23015563082025));
#248927=CARTESIAN_POINT('Ctrl Pts',(-9.09294310126612,12.2,6.22676937307857));
#248928=CARTESIAN_POINT('Ctrl Pts',(-9.0905531924477,12.2,6.22339842654849));
#248929=CARTESIAN_POINT('Ctrl Pts',(-9.08816598547342,12.2,6.22004282473931));
#248930=CARTESIAN_POINT('Ctrl Pts',(-9.0851819769182,12.2,6.21584832270643));
#248931=CARTESIAN_POINT('Ctrl Pts',(-9.0822021876497,12.2,6.21167779784431));
#248932=CARTESIAN_POINT('Ctrl Pts',(-9.07922685508048,12.2,6.20753131826222));
#248933=CARTESIAN_POINT('Ctrl Pts',(-9.07684658921969,12.2,6.20421413486774));
#248934=CARTESIAN_POINT('Ctrl Pts',(-9.07446917684448,12.2,6.20091234115352));
#248935=CARTESIAN_POINT('Ctrl Pts',(-9.0720947383716,12.2,6.19762597108725));
#248936=CARTESIAN_POINT('Ctrl Pts',(-9.0697202995752,12.2,6.1943396005732));
#248937=CARTESIAN_POINT('Ctrl Pts',(-9.06734883574021,12.2,6.19106865276066));
#248938=CARTESIAN_POINT('Ctrl Pts',(-9.06498047150005,12.2,6.18781316424993));
#248939=CARTESIAN_POINT('Ctrl Pts',(-9.06261210725988,12.2,6.1845576757392));
#248940=CARTESIAN_POINT('Ctrl Pts',(-9.06024684060615,12.2,6.181317646083));
#248941=CARTESIAN_POINT('Ctrl Pts',(-9.05788479908885,12.2,6.17809310896439));
#248942=CARTESIAN_POINT('Ctrl Pts',(-9.05493224767497,12.2,6.17406243822514));
#248943=CARTESIAN_POINT('Ctrl Pts',(-9.05198473405351,12.2,6.17005597587762));
#248944=CARTESIAN_POINT('Ctrl Pts',(-9.04904250360988,12.2,6.16607378846246));
#248945=CARTESIAN_POINT('Ctrl Pts',(-9.04668871887013,12.2,6.16288803800946));
#248946=CARTESIAN_POINT('Ctrl Pts',(-9.04433831785295,12.2,6.15971782447184));
#248947=CARTESIAN_POINT('Ctrl Pts',(-9.04199142522504,12.2,6.15656318196659));
#248948=CARTESIAN_POINT('Ctrl Pts',(-9.03964453259714,12.2,6.15340853946133));
#248949=CARTESIAN_POINT('Ctrl Pts',(-9.03730114994188,12.2,6.15026946682734));
#248950=CARTESIAN_POINT('Ctrl Pts',(-9.03496140709249,12.2,6.14714599971424));
#248951=CARTESIAN_POINT('Ctrl Pts',(-9.0326216645619,12.2,6.14402253302672));
#248952=CARTESIAN_POINT('Ctrl Pts',(-9.03028556015212,12.2,6.14091467168001));
#248953=CARTESIAN_POINT('Ctrl Pts',(-9.02795322627664,12.2,6.13782245025204));
#248954=CARTESIAN_POINT('Ctrl Pts',(-9.02562089208336,12.2,6.13473022840276));
#248955=CARTESIAN_POINT('Ctrl Pts',(-9.02329232849071,12.2,6.1316536462647));
#248956=CARTESIAN_POINT('Ctrl Pts',(-9.02096766458663,12.2,6.12859273776614));
#248957=CARTESIAN_POINT('Ctrl Pts',(-9.01864300099929,12.2,6.12553182968462));
#248958=CARTESIAN_POINT('Ctrl Pts',(-9.01632224013369,12.2,6.12248659430111));
#248959=CARTESIAN_POINT('Ctrl Pts',(-9.01400551365613,12.2,6.1194570682144));
#248960=CARTESIAN_POINT('Ctrl Pts',(-9.01168878686293,12.2,6.11642754171491));
#248961=CARTESIAN_POINT('Ctrl Pts',(-9.00937609449197,12.2,6.11341372374899));
#248962=CARTESIAN_POINT('Ctrl Pts',(-9.00706757164009,12.2,6.11041564654831));
#248963=CARTESIAN_POINT('Ctrl Pts',(-9.00475904910274,12.2,6.10741756975611));
#248964=CARTESIAN_POINT('Ctrl Pts',(-9.00245469528924,12.2,6.10443523633443));
#248965=CARTESIAN_POINT('Ctrl Pts',(-9.00015464692144,12.2,6.10146867824259));
#248966=CARTESIAN_POINT('Ctrl Pts',(-8.99785459824026,12.2,6.09850211974656));
#248967=CARTESIAN_POINT('Ctrl Pts',(-8.99555885494013,12.2,6.0955513383274));
#248968=CARTESIAN_POINT('Ctrl Pts',(-8.99326755487111,12.2,6.09261636600182));
#248969=CARTESIAN_POINT('Ctrl Pts',(-8.99097625511427,12.2,6.08968139407612));
#248970=CARTESIAN_POINT('Ctrl Pts',(-8.98868939709794,12.2,6.08676223271368));
#248971=CARTESIAN_POINT('Ctrl Pts',(-8.98640712061457,12.2,6.08385891513796));
#248972=CARTESIAN_POINT('Ctrl Pts',(-8.98412484382023,12.2,6.08095559716666));
#248973=CARTESIAN_POINT('Ctrl Pts',(-8.9818471490156,12.2,6.07806812315132));
#248974=CARTESIAN_POINT('Ctrl Pts',(-8.97957417578094,12.2,6.07519652727366));
#248975=CARTESIAN_POINT('Ctrl Pts',(-8.97730120285597,12.2,6.07232493178725));
#248976=CARTESIAN_POINT('Ctrl Pts',(-8.97503295389946,12.2,6.06946921408372));
#248977=CARTESIAN_POINT('Ctrl Pts',(-8.97276956636176,12.2,6.0666294079809));
#248978=CARTESIAN_POINT('Ctrl Pts',(-8.97050617851567,12.2,6.06378960149115));
#248979=CARTESIAN_POINT('Ctrl Pts',(-8.96824765550376,12.2,6.06096570559707));
#248980=CARTESIAN_POINT('Ctrl Pts',(-8.96599413948184,12.2,6.05815775576469));
#248981=CARTESIAN_POINT('Ctrl Pts',(-8.96374062376698,12.2,6.0553498063149));
#248982=CARTESIAN_POINT('Ctrl Pts',(-8.96149211395618,12.2,6.05255780151461));
#248983=CARTESIAN_POINT('Ctrl Pts',(-8.95924875758349,12.2,6.04978177546214));
#248984=CARTESIAN_POINT('Ctrl Pts',(-8.95700540090515,12.2,6.04700574903145));
#248985=CARTESIAN_POINT('Ctrl Pts',(-8.95476719569672,12.2,6.04424570199668));
#248986=CARTESIAN_POINT('Ctrl Pts',(-8.9525342897417,12.2,6.04150166745825));
#248987=CARTESIAN_POINT('Ctrl Pts',(-8.95030138378669,12.2,6.03875763291983));
#248988=CARTESIAN_POINT('Ctrl Pts',(-8.94807377588782,12.2,6.03602960973602));
#248989=CARTESIAN_POINT('Ctrl Pts',(-8.94585161537839,12.2,6.03331763258986));
#248990=CARTESIAN_POINT('Ctrl Pts',(-8.94307391519575,12.2,6.02992766171141));
#248991=CARTESIAN_POINT('Ctrl Pts',(-8.9403047264054,12.2,6.02656276143039));
#248992=CARTESIAN_POINT('Ctrl Pts',(-8.93754434038609,12.2,6.02322299811177));
#248993=CARTESIAN_POINT('Ctrl Pts',(-8.93533603120957,12.2,6.02055118702003));
#248994=CARTESIAN_POINT('Ctrl Pts',(-8.93313335678365,12.2,6.01789546262155));
#248995=CARTESIAN_POINT('Ctrl Pts',(-8.9309364689417,12.2,6.01525586003325));
#248996=CARTESIAN_POINT('Ctrl Pts',(-8.92873958109975,12.2,6.01261625744496));
#248997=CARTESIAN_POINT('Ctrl Pts',(-8.92654847980845,12.2,6.00999277398628));
#248998=CARTESIAN_POINT('Ctrl Pts',(-8.92436331863442,12.2,6.00738544429029));
#248999=CARTESIAN_POINT('Ctrl Pts',(-8.92217815775812,12.2,6.00477811494955));
#249000=CARTESIAN_POINT('Ctrl Pts',(-8.91999893644484,12.2,6.00218694030291));
#249001=CARTESIAN_POINT('Ctrl Pts',(-8.91782581150152,12.2,5.99961195150169));
#249002=CARTESIAN_POINT('Ctrl Pts',(-8.9156526862621,12.2,5.99703696234962));
#249003=CARTESIAN_POINT('Ctrl Pts',(-8.91348565639443,12.2,5.99447816055447));
#249004=CARTESIAN_POINT('Ctrl Pts',(-8.91132487988841,12.2,5.99193557808421));
#249005=CARTESIAN_POINT('Ctrl Pts',(-8.90862390940309,12.2,5.9887573501696));
#249006=CARTESIAN_POINT('Ctrl Pts',(-8.90593270821518,12.2,5.98560446438877));
#249007=CARTESIAN_POINT('Ctrl Pts',(-8.90325158863268,12.2,5.98247698730753));
#249008=CARTESIAN_POINT('Ctrl Pts',(-8.90057046934242,12.2,5.97934951056718));
#249009=CARTESIAN_POINT('Ctrl Pts',(-8.89789943029222,12.2,5.97624744106908));
#249010=CARTESIAN_POINT('Ctrl Pts',(-8.89523878933137,12.2,5.97317084265234));
#249011=CARTESIAN_POINT('Ctrl Pts',(-8.89257814808052,12.2,5.97009424390025));
#249012=CARTESIAN_POINT('Ctrl Pts',(-8.88992790359616,12.2,5.96704311671443));
#249013=CARTESIAN_POINT('Ctrl Pts',(-8.88728837734528,12.2,5.96401752462901));
#249014=CARTESIAN_POINT('Ctrl Pts',(-8.88464885109441,12.2,5.96099193254359));
#249015=CARTESIAN_POINT('Ctrl Pts',(-8.88202004188223,12.2,5.95799187677997));
#249016=CARTESIAN_POINT('Ctrl Pts',(-8.87940227507577,12.2,5.95501741893065));
#249017=CARTESIAN_POINT('Ctrl Pts',(-8.8752138482425,12.2,5.95025828643659));
#249018=CARTESIAN_POINT('Ctrl Pts',(-8.87105369166071,12.2,5.94556468565188));
#249019=CARTESIAN_POINT('Ctrl Pts',(-8.86692316060437,12.2,5.94093687837826));
#249020=CARTESIAN_POINT('Ctrl Pts',(-8.864341578659,12.2,5.93804449879283));
#249021=CARTESIAN_POINT('Ctrl Pts',(-8.86177157093003,12.2,5.93517782014584));
#249022=CARTESIAN_POINT('Ctrl Pts',(-8.85921347565129,12.2,5.93233690312985));
#249023=CARTESIAN_POINT('Ctrl Pts',(-8.85665538037255,12.2,5.92949598611385));
#249024=CARTESIAN_POINT('Ctrl Pts',(-8.85410919657167,12.2,5.92668083383164));
#249025=CARTESIAN_POINT('Ctrl Pts',(-8.85157526956922,12.2,5.92389150660714));
#249026=CARTESIAN_POINT('Ctrl Pts',(-8.84904134256677,12.2,5.92110217938266));
#249027=CARTESIAN_POINT('Ctrl Pts',(-8.84651967100374,12.2,5.91833867758046));
#249028=CARTESIAN_POINT('Ctrl Pts',(-8.84401060586419,12.2,5.91560106466244));
#249029=CARTESIAN_POINT('Ctrl Pts',(-8.84150154072464,12.2,5.91286345174443));
#249030=CARTESIAN_POINT('Ctrl Pts',(-8.83900507998542,12.2,5.91015172863265));
#249031=CARTESIAN_POINT('Ctrl Pts',(-8.83652158067919,12.2,5.90746595495072));
#249032=CARTESIAN_POINT('Ctrl Pts',(-8.83403808137295,12.2,5.90478018126881));
#249033=CARTESIAN_POINT('Ctrl Pts',(-8.83156754173479,12.2,5.90212035865229));
#249034=CARTESIAN_POINT('Ctrl Pts',(-8.82911032325137,12.2,5.89948654975137));
#249035=CARTESIAN_POINT('Ctrl Pts',(-8.82665310476795,12.2,5.89685274085044));
#249036=CARTESIAN_POINT('Ctrl Pts',(-8.82420920823334,12.2,5.8942449446888));
#249037=CARTESIAN_POINT('Ctrl Pts',(-8.82177899823336,12.2,5.89166322350825));
#249038=CARTESIAN_POINT('Ctrl Pts',(-8.81934878823337,12.2,5.88908150232771));
#249039=CARTESIAN_POINT('Ctrl Pts',(-8.81693226548736,12.2,5.88652585648773));
#249040=CARTESIAN_POINT('Ctrl Pts',(-8.81452980374038,12.2,5.88399634703187));
#249041=CARTESIAN_POINT('Ctrl Pts',(-8.81212734199339,12.2,5.88146683757603));
#249042=CARTESIAN_POINT('Ctrl Pts',(-8.80973894037744,12.2,5.87896346501449));
#249043=CARTESIAN_POINT('Ctrl Pts',(-8.80736497787818,12.2,5.8764862918214));
#249044=CARTESIAN_POINT('Ctrl Pts',(-8.80499101537891,12.2,5.87400911862832));
#249045=CARTESIAN_POINT('Ctrl Pts',(-8.80263149237376,12.2,5.87155814197902));
#249046=CARTESIAN_POINT('Ctrl Pts',(-8.80028679334676,12.2,5.86913342579982));
#249047=CARTESIAN_POINT('Ctrl Pts',(-8.79794209431974,12.2,5.86670870962063));
#249048=CARTESIAN_POINT('Ctrl Pts',(-8.79561222028486,12.2,5.86431025398577));
#249049=CARTESIAN_POINT('Ctrl Pts',(-8.79329756273971,12.2,5.86193811775798));
#249050=CARTESIAN_POINT('Ctrl Pts',(-8.79005704237834,12.2,5.85861712724592));
#249051=CARTESIAN_POINT('Ctrl Pts',(-8.78684634516754,12.2,5.85534772751428));
#249052=CARTESIAN_POINT('Ctrl Pts',(-8.78366657203044,12.2,5.85213008155888));
#249053=CARTESIAN_POINT('Ctrl Pts',(-8.78094105188033,12.2,5.84937209898929));
#249054=CARTESIAN_POINT('Ctrl Pts',(-8.77823824856104,12.2,5.84665214112681));
#249055=CARTESIAN_POINT('Ctrl Pts',(-8.77555887253255,12.2,5.84397031326558));
#249056=CARTESIAN_POINT('Ctrl Pts',(-8.77287949674744,12.2,5.84128848564795));
#249057=CARTESIAN_POINT('Ctrl Pts',(-8.77022354674606,12.2,5.83864478449692));
#249058=CARTESIAN_POINT('Ctrl Pts',(-8.76759174725834,12.2,5.83603931900825));
#249059=CARTESIAN_POINT('Ctrl Pts',(-8.76495994777063,12.2,5.83343385351958));
#249060=CARTESIAN_POINT('Ctrl Pts',(-8.7623522980699,12.2,5.83086662035635));
#249061=CARTESIAN_POINT('Ctrl Pts',(-8.75976953569992,12.2,5.82833772473631));
#249062=CARTESIAN_POINT('Ctrl Pts',(-8.75718677309533,12.2,5.82580882888658));
#249063=CARTESIAN_POINT('Ctrl Pts',(-8.75462890078526,12.2,5.82331826911366));
#249064=CARTESIAN_POINT('Ctrl Pts',(-8.75209667223233,12.2,5.82086615048264));
#249065=CARTESIAN_POINT('Ctrl Pts',(-8.74956444390942,12.2,5.81841403207436));
#249066=CARTESIAN_POINT('Ctrl Pts',(-8.74705786000329,12.2,5.81600035433157));
#249067=CARTESIAN_POINT('Ctrl Pts',(-8.74457769274889,12.2,5.81362521899051));
#249068=CARTESIAN_POINT('Ctrl Pts',(-8.74209752549448,12.2,5.81125008364944));
#249069=CARTESIAN_POINT('Ctrl Pts',(-8.7396437742037,12.2,5.8089134913435));
#249070=CARTESIAN_POINT('Ctrl Pts',(-8.73721723287403,12.2,5.80661554492531));
#249071=CARTESIAN_POINT('Ctrl Pts',(-8.73479069132394,12.2,5.80431759829841));
#249072=CARTESIAN_POINT('Ctrl Pts',(-8.73239135639386,12.2,5.80205829695126));
#249073=CARTESIAN_POINT('Ctrl Pts',(-8.73002003901654,12.2,5.79983774324955));
#249074=CARTESIAN_POINT('Ctrl Pts',(-8.72764872185461,12.2,5.79761718974955));
#249075=CARTESIAN_POINT('Ctrl Pts',(-8.72530542130863,12.2,5.79543538394739));
#249076=CARTESIAN_POINT('Ctrl Pts',(-8.72299096821562,12.2,5.79329242651561));
#249077=CARTESIAN_POINT('Ctrl Pts',(-8.72067651512262,12.2,5.79114946908385));
#249078=CARTESIAN_POINT('Ctrl Pts',(-8.71839090675908,12.2,5.7890453622143));
#249079=CARTESIAN_POINT('Ctrl Pts',(-8.71613499383974,12.2,5.78698020387097));
#249080=CARTESIAN_POINT('Ctrl Pts',(-8.71387908071548,12.2,5.78491504534004));
#249081=CARTESIAN_POINT('Ctrl Pts',(-8.71165286344493,12.2,5.7828888376223));
#249082=CARTESIAN_POINT('Ctrl Pts',(-8.70945721049402,12.2,5.78090168101666));
#249083=CARTESIAN_POINT('Ctrl Pts',(-8.70726155774254,12.2,5.77891452459151));
#249084=CARTESIAN_POINT('Ctrl Pts',(-8.7050964699133,12.2,5.77696641859167));
#249085=CARTESIAN_POINT('Ctrl Pts',(-8.70296283907551,12.2,5.7750574641627));
#249086=CARTESIAN_POINT('Ctrl Pts',(-8.70082920823772,12.2,5.77314850973373));
#249087=CARTESIAN_POINT('Ctrl Pts',(-8.69872703439749,12.2,5.77127870801839));
#249088=CARTESIAN_POINT('Ctrl Pts',(-8.69665723188794,12.2,5.76944815658318));
#249089=CARTESIAN_POINT('Ctrl Pts',(-8.6945874293784,12.2,5.76761760514797));
#249090=CARTESIAN_POINT('Ctrl Pts',(-8.69255000036457,12.2,5.76582630417156));
#249091=CARTESIAN_POINT('Ctrl Pts',(-8.69054588076846,12.2,5.76407435548256));
#249092=CARTESIAN_POINT('Ctrl Pts',(-8.6885417609903,12.2,5.76232240663441));
#249093=CARTESIAN_POINT('Ctrl Pts',(-8.68657095229864,12.2,5.76060980817335));
#249094=CARTESIAN_POINT('Ctrl Pts',(-8.6846344176946,12.2,5.75893665966723));
#249095=CARTESIAN_POINT('Ctrl Pts',(-8.68269788326646,12.2,5.75726351131309));
#249096=CARTESIAN_POINT('Ctrl Pts',(-8.68079562368323,12.2,5.75562981352503));
#249097=CARTESIAN_POINT('Ctrl Pts',(-8.67892862849251,12.2,5.75403566599231));
#249098=CARTESIAN_POINT('Ctrl Pts',(-8.6770616333018,12.2,5.75244151845958));
#249099=CARTESIAN_POINT('Ctrl Pts',(-8.67522990259125,12.2,5.75088691961269));
#249100=CARTESIAN_POINT('Ctrl Pts',(-8.67343445440404,12.2,5.74937196816505));
#249101=CARTESIAN_POINT('Ctrl Pts',(-8.67163900605374,12.2,5.74785701657981));
#249102=CARTESIAN_POINT('Ctrl Pts',(-8.66987983975288,12.2,5.74638171360046));
#249103=CARTESIAN_POINT('Ctrl Pts',(-8.66815800232518,12.2,5.74494615786947));
#249104=CARTESIAN_POINT('Ctrl Pts',(-8.66643616505387,12.2,5.74351060226887));
#249105=CARTESIAN_POINT('Ctrl Pts',(-8.66475165580683,12.2,5.74211479191732));
#249106=CARTESIAN_POINT('Ctrl Pts',(-8.66310555103332,12.2,5.74075882646657));
#249107=CARTESIAN_POINT('Ctrl Pts',(-8.66145944625979,12.2,5.73940286101584));
#249108=CARTESIAN_POINT('Ctrl Pts',(-8.65985174748376,12.2,5.73808674020149));
#249109=CARTESIAN_POINT('Ctrl Pts',(-8.65828355987679,12.2,5.73681056259847));
#249110=CARTESIAN_POINT('Ctrl Pts',(-8.65671537212737,12.2,5.73553438487952));
#249111=CARTESIAN_POINT('Ctrl Pts',(-8.65518669881612,12.2,5.73429814974866));
#249112=CARTESIAN_POINT('Ctrl Pts',(-8.65369867907114,12.2,5.73310195435287));
#249113=CARTESIAN_POINT('Ctrl Pts',(-8.6522178008694,12.2,5.73191149993006));
#249114=CARTESIAN_POINT('Ctrl Pts',(-8.65077718857068,12.2,5.73076070226254));
#249115=CARTESIAN_POINT('Ctrl Pts',(-8.64937799900006,12.2,5.72964966099998));
#249116=CARTESIAN_POINT('Ctrl Pts',(-8.64937799900006,15.2,5.72964966099998));
#249117=CARTESIAN_POINT('Ctrl Pts',(-8.65077718857068,15.2,5.73076070226254));
#249118=CARTESIAN_POINT('Ctrl Pts',(-8.65221780086937,15.2,5.73191149993004));
#249119=CARTESIAN_POINT('Ctrl Pts',(-8.65369867907113,15.2,5.73310195435287));
#249120=CARTESIAN_POINT('Ctrl Pts',(-8.65518669881613,15.2,5.73429814974867));
#249121=CARTESIAN_POINT('Ctrl Pts',(-8.65671537212734,15.2,5.7355343848795));
#249122=CARTESIAN_POINT('Ctrl Pts',(-8.65828355987679,15.2,5.73681056259847));
#249123=CARTESIAN_POINT('Ctrl Pts',(-8.65985174748379,15.2,5.73808674020152));
#249124=CARTESIAN_POINT('Ctrl Pts',(-8.6614594462598,15.2,5.73940286101585));
#249125=CARTESIAN_POINT('Ctrl Pts',(-8.66310555103331,15.2,5.74075882646657));
#249126=CARTESIAN_POINT('Ctrl Pts',(-8.66475165580682,15.2,5.74211479191731));
#249127=CARTESIAN_POINT('Ctrl Pts',(-8.66643616505388,15.2,5.74351060226888));
#249128=CARTESIAN_POINT('Ctrl Pts',(-8.66815800232518,15.2,5.74494615786947));
#249129=CARTESIAN_POINT('Ctrl Pts',(-8.66987983975287,15.2,5.74638171360045));
#249130=CARTESIAN_POINT('Ctrl Pts',(-8.6716390060537,15.2,5.74785701657977));
#249131=CARTESIAN_POINT('Ctrl Pts',(-8.67343445440403,15.2,5.74937196816505));
#249132=CARTESIAN_POINT('Ctrl Pts',(-8.67522990259129,15.2,5.75088691961273));
#249133=CARTESIAN_POINT('Ctrl Pts',(-8.67706163330177,15.2,5.75244151845955));
#249134=CARTESIAN_POINT('Ctrl Pts',(-8.67892862849251,15.2,5.75403566599231));
#249135=CARTESIAN_POINT('Ctrl Pts',(-8.68079562368326,15.2,5.75562981352506));
#249136=CARTESIAN_POINT('Ctrl Pts',(-8.68269788326646,15.2,5.75726351131309));
#249137=CARTESIAN_POINT('Ctrl Pts',(-8.6846344176946,15.2,5.75893665966723));
#249138=CARTESIAN_POINT('Ctrl Pts',(-8.68657095229864,15.2,5.76060980817335));
#249139=CARTESIAN_POINT('Ctrl Pts',(-8.68854176099027,15.2,5.76232240663438));
#249140=CARTESIAN_POINT('Ctrl Pts',(-8.69054588076846,15.2,5.76407435548256));
#249141=CARTESIAN_POINT('Ctrl Pts',(-8.69255000036461,15.2,5.7658263041716));
#249142=CARTESIAN_POINT('Ctrl Pts',(-8.69458742937841,15.2,5.76761760514798));
#249143=CARTESIAN_POINT('Ctrl Pts',(-8.69665723188794,15.2,5.76944815658318));
#249144=CARTESIAN_POINT('Ctrl Pts',(-8.69872703439747,15.2,5.77127870801838));
#249145=CARTESIAN_POINT('Ctrl Pts',(-8.70082920823772,15.2,5.77314850973373));
#249146=CARTESIAN_POINT('Ctrl Pts',(-8.70296283907552,15.2,5.77505746416271));
#249147=CARTESIAN_POINT('Ctrl Pts',(-8.70509646991331,15.2,5.77696641859168));
#249148=CARTESIAN_POINT('Ctrl Pts',(-8.70726155774256,15.2,5.77891452459153));
#249149=CARTESIAN_POINT('Ctrl Pts',(-8.70945721049402,15.2,5.78090168101666));
#249150=CARTESIAN_POINT('Ctrl Pts',(-8.71165286344492,15.2,5.78288883762229));
#249151=CARTESIAN_POINT('Ctrl Pts',(-8.71387908071551,15.2,5.78491504534007));
#249152=CARTESIAN_POINT('Ctrl Pts',(-8.71613499383974,15.2,5.78698020387097));
#249153=CARTESIAN_POINT('Ctrl Pts',(-8.7187668921773,15.2,5.78938955520896));
#249154=CARTESIAN_POINT('Ctrl Pts',(-8.72143920775675,15.2,5.79185192106912));
#249155=CARTESIAN_POINT('Ctrl Pts',(-8.72415059478003,15.2,5.79436714175661));
#249156=CARTESIAN_POINT('Ctrl Pts',(-8.72647464107139,15.2,5.79652304545479));
#249157=CARTESIAN_POINT('Ctrl Pts',(-8.72882739479893,15.2,5.79871778224841));
#249158=CARTESIAN_POINT('Ctrl Pts',(-8.73120802909653,15.2,5.8009512488718));
#249159=CARTESIAN_POINT('Ctrl Pts',(-8.7335886631779,15.2,5.80318471529232));
#249160=CARTESIAN_POINT('Ctrl Pts',(-8.73599717779872,15.2,5.80545691293479));
#249161=CARTESIAN_POINT('Ctrl Pts',(-8.73843276712572,15.2,5.80776773759914));
#249162=CARTESIAN_POINT('Ctrl Pts',(-8.74127428815468,15.2,5.81046369984749));
#249163=CARTESIAN_POINT('Ctrl Pts',(-8.74415266250621,15.2,5.81321224270758));
#249164=CARTESIAN_POINT('Ctrl Pts',(-8.74706663713624,15.2,5.81601319786425));
#249165=CARTESIAN_POINT('Ctrl Pts',(-8.74956432954663,15.2,5.81841401644537));
#249166=CARTESIAN_POINT('Ctrl Pts',(-8.75208817976324,15.2,5.82085334532339));
#249167=CARTESIAN_POINT('Ctrl Pts',(-8.75463742108618,15.2,5.82333107889837));
#249168=CARTESIAN_POINT('Ctrl Pts',(-8.75718666240915,15.2,5.82580881247335));
#249169=CARTESIAN_POINT('Ctrl Pts',(-8.75976129425447,15.2,5.82832495308358));
#249170=CARTESIAN_POINT('Ctrl Pts',(-8.76236056590836,15.2,5.83087939548815));
#249171=CARTESIAN_POINT('Ctrl Pts',(-8.76495983779834,15.2,5.83343383812474));
#249172=CARTESIAN_POINT('Ctrl Pts',(-8.7675837506574,15.2,5.8360265813234));
#249173=CARTESIAN_POINT('Ctrl Pts',(-8.77023157038609,15.2,5.83865752588513));
#249174=CARTESIAN_POINT('Ctrl Pts',(-8.77332069304212,15.2,5.84172696084867));
#249175=CARTESIAN_POINT('Ctrl Pts',(-8.77644235554255,15.2,5.84484838598747));
#249176=CARTESIAN_POINT('Ctrl Pts',(-8.77959541774711,15.2,5.84802163920346));
#249177=CARTESIAN_POINT('Ctrl Pts',(-8.78229804280949,15.2,5.8507415708491));
#249178=CARTESIAN_POINT('Ctrl Pts',(-8.78502373925748,15.2,5.85349957874843));
#249179=CARTESIAN_POINT('Ctrl Pts',(-8.78777180615821,15.2,5.85629555940246));
#249180=CARTESIAN_POINT('Ctrl Pts',(-8.79143589510955,15.2,5.86002353335384));
#249181=CARTESIAN_POINT('Ctrl Pts',(-8.79513975134169,15.2,5.86381901413341));
#249182=CARTESIAN_POINT('Ctrl Pts',(-8.79888175640306,15.2,5.8676817484163));
#249183=CARTESIAN_POINT('Ctrl Pts',(-8.8012205095983,15.2,5.87009595737601));
#249184=CARTESIAN_POINT('Ctrl Pts',(-8.80357416393203,15.2,5.87253643944894));
#249185=CARTESIAN_POINT('Ctrl Pts',(-8.80594233615498,15.2,5.87500313222806));
#249186=CARTESIAN_POINT('Ctrl Pts',(-8.80831050837794,15.2,5.87746982500719));
#249187=CARTESIAN_POINT('Ctrl Pts',(-8.81069319467424,15.2,5.87996272728698));
#249188=CARTESIAN_POINT('Ctrl Pts',(-8.81309001729498,15.2,5.88248177873411));
#249189=CARTESIAN_POINT('Ctrl Pts',(-8.81548683991571,15.2,5.88500083018124));
#249190=CARTESIAN_POINT('Ctrl Pts',(-8.81789779715491,15.2,5.88754603274521));
#249191=CARTESIAN_POINT('Ctrl Pts',(-8.82032251785052,15.2,5.89011732080292));
#249192=CARTESIAN_POINT('Ctrl Pts',(-8.82323218257952,15.2,5.89320286636009));
#249193=CARTESIAN_POINT('Ctrl Pts',(-8.82616166117839,15.2,5.89632597918507));
#249194=CARTESIAN_POINT('Ctrl Pts',(-8.82911032325136,15.2,5.89948654975136));
#249195=CARTESIAN_POINT('Ctrl Pts',(-8.83156754173478,15.2,5.90212035865228));
#249196=CARTESIAN_POINT('Ctrl Pts',(-8.83403808137296,15.2,5.90478018126882));
#249197=CARTESIAN_POINT('Ctrl Pts',(-8.83652158067919,15.2,5.90746595495072));
#249198=CARTESIAN_POINT('Ctrl Pts',(-8.83900507998541,15.2,5.91015172863263));
#249199=CARTESIAN_POINT('Ctrl Pts',(-8.84150154072465,15.2,5.91286345174443));
#249200=CARTESIAN_POINT('Ctrl Pts',(-8.8440106058642,15.2,5.91560106466246));
#249201=CARTESIAN_POINT('Ctrl Pts',(-8.84702148392227,15.2,5.91888620004472));
#249202=CARTESIAN_POINT('Ctrl Pts',(-8.85005051432056,15.2,5.92220861549699));
#249203=CARTESIAN_POINT('Ctrl Pts',(-8.85309709347364,15.2,5.9255682009734));
#249204=CARTESIAN_POINT('Ctrl Pts',(-8.85563590952679,15.2,5.92836785563879));
#249205=CARTESIAN_POINT('Ctrl Pts',(-8.85818691230002,15.2,5.93119332447771));
#249206=CARTESIAN_POINT('Ctrl Pts',(-8.86074975917502,15.2,5.93404454399158));
#249207=CARTESIAN_POINT('Ctrl Pts',(-8.86485031411913,15.2,5.93860649515163));
#249208=CARTESIAN_POINT('Ctrl Pts',(-8.86898118831148,15.2,5.94323436703555));
#249209=CARTESIAN_POINT('Ctrl Pts',(-8.87314100727362,15.2,5.947927901215));
#249210=CARTESIAN_POINT('Ctrl Pts',(-8.87574089416037,15.2,5.95086136011712));
#249211=CARTESIAN_POINT('Ctrl Pts',(-8.87835208694446,15.2,5.95382047034435));
#249212=CARTESIAN_POINT('Ctrl Pts',(-8.88097425729169,15.2,5.95680516423325));
#249213=CARTESIAN_POINT('Ctrl Pts',(-8.88412086159406,15.2,5.9603867967698));
#249214=CARTESIAN_POINT('Ctrl Pts',(-8.88728327284515,15.2,5.9640052756618));
#249215=CARTESIAN_POINT('Ctrl Pts',(-8.89046093214533,15.2,5.96766048710984));
#249216=CARTESIAN_POINT('Ctrl Pts',(-8.89310898165836,15.2,5.97070649676054));
#249217=CARTESIAN_POINT('Ctrl Pts',(-8.8957676200576,15.2,5.97377801682086));
#249218=CARTESIAN_POINT('Ctrl Pts',(-8.89843652894025,15.2,5.9768749823905));
#249219=CARTESIAN_POINT('Ctrl Pts',(-8.9011054378229,15.2,5.97997194796015));
#249220=CARTESIAN_POINT('Ctrl Pts',(-8.90378461666361,15.2,5.98309435880108));
#249221=CARTESIAN_POINT('Ctrl Pts',(-8.90647375131589,15.2,5.98624215178588));
#249222=CARTESIAN_POINT('Ctrl Pts',(-8.90916288596816,15.2,5.98938994477068));
#249223=CARTESIAN_POINT('Ctrl Pts',(-8.9118619768901,15.2,5.9925631199422));
#249224=CARTESIAN_POINT('Ctrl Pts',(-8.91457071480627,15.2,5.99576161202423));
#249225=CARTESIAN_POINT('Ctrl Pts',(-8.91782120018757,15.2,5.9995998023832));
#249226=CARTESIAN_POINT('Ctrl Pts',(-8.92108557717114,15.2,6.00347445010159));
#249227=CARTESIAN_POINT('Ctrl Pts',(-8.92436331863443,15.2,6.00738544429029));
#249228=CARTESIAN_POINT('Ctrl Pts',(-8.92709476995307,15.2,6.01064460623263));
#249229=CARTESIAN_POINT('Ctrl Pts',(-8.92983550260778,15.2,6.01392900720799));
#249230=CARTESIAN_POINT('Ctrl Pts',(-8.93258521719037,15.2,6.01723858352537));
#249231=CARTESIAN_POINT('Ctrl Pts',(-8.93533493177299,15.2,6.02054815984277));
#249232=CARTESIAN_POINT('Ctrl Pts',(-8.93809362763003,15.2,6.02388291246607));
#249233=CARTESIAN_POINT('Ctrl Pts',(-8.94086100992048,15.2,6.02724277478498));
#249234=CARTESIAN_POINT('Ctrl Pts',(-8.9430749158735,15.2,6.0299306647866));
#249235=CARTESIAN_POINT('Ctrl Pts',(-8.94529438058538,15.2,6.03263462607594));
#249236=CARTESIAN_POINT('Ctrl Pts',(-8.94751925520697,15.2,6.03535462394743));
#249237=CARTESIAN_POINT('Ctrl Pts',(-8.94974412952543,15.2,6.03807462144833));
#249238=CARTESIAN_POINT('Ctrl Pts',(-8.95197441419562,15.2,6.04081065615439));
#249239=CARTESIAN_POINT('Ctrl Pts',(-8.95420995990119,15.2,6.04356269481663));
#249240=CARTESIAN_POINT('Ctrl Pts',(-8.95644550591134,15.2,6.04631473385383));
#249241=CARTESIAN_POINT('Ctrl Pts',(-8.95868631456062,15.2,6.04908277646797));
#249242=CARTESIAN_POINT('Ctrl Pts',(-8.96093223852656,15.2,6.05186679024349));
#249243=CARTESIAN_POINT('Ctrl Pts',(-8.9631781621865,15.2,6.05465080363969));
#249244=CARTESIAN_POINT('Ctrl Pts',(-8.96542920232445,15.2,6.05745078667136));
#249245=CARTESIAN_POINT('Ctrl Pts',(-8.96768521263951,15.2,6.06026670677285));
#249246=CARTESIAN_POINT('Ctrl Pts',(-8.96994122326194,15.2,6.06308262725801));
#249247=CARTESIAN_POINT('Ctrl Pts',(-8.97220220627099,15.2,6.06591448511415));
#249248=CARTESIAN_POINT('Ctrl Pts',(-8.97446801628337,15.2,6.06876224499158));
#249249=CARTESIAN_POINT('Ctrl Pts',(-8.97730027864447,15.2,6.07232194464437));
#249250=CARTESIAN_POINT('Ctrl Pts',(-8.98014008505528,15.2,6.07590649380763));
#249251=CARTESIAN_POINT('Ctrl Pts',(-8.98298715923492,15.2,6.07951582576856));
#249252=CARTESIAN_POINT('Ctrl Pts',(-8.98526481839244,15.2,6.08240329110125));
#249253=CARTESIAN_POINT('Ctrl Pts',(-8.98754713037465,15.2,6.08530661723234));
#249254=CARTESIAN_POINT('Ctrl Pts',(-8.98983395340948,15.2,6.08822577004764));
#249255=CARTESIAN_POINT('Ctrl Pts',(-8.99269248243668,15.2,6.09187471136507));
#249256=CARTESIAN_POINT('Ctrl Pts',(-8.99555806028602,15.2,6.09554838200711));
#249257=CARTESIAN_POINT('Ctrl Pts',(-8.99843041938266,15.2,6.09924671728285));
#249258=CARTESIAN_POINT('Ctrl Pts',(-9.0013027784793,15.2,6.10294505255858));
#249259=CARTESIAN_POINT('Ctrl Pts',(-9.00418191823247,15.2,6.10666805025166));
#249260=CARTESIAN_POINT('Ctrl Pts',(-9.00706757164008,15.2,6.1104156465483));
#249261=CARTESIAN_POINT('Ctrl Pts',(-9.0099532250477,15.2,6.11416324284494));
#249262=CARTESIAN_POINT('Ctrl Pts',(-9.0128453929664,15.2,6.1179354339086));
#249263=CARTESIAN_POINT('Ctrl Pts',(-9.01574381282718,15.2,6.12173215751843));
#249264=CARTESIAN_POINT('Ctrl Pts',(-9.01806254884218,15.2,6.12476953657183));
#249265=CARTESIAN_POINT('Ctrl Pts',(-9.02038528679656,15.2,6.12782261481601));
#249266=CARTESIAN_POINT('Ctrl Pts',(-9.02271189225695,15.2,6.13089135798428));
#249267=CARTESIAN_POINT('Ctrl Pts',(-9.02503849740031,15.2,6.13396010073441));
#249268=CARTESIAN_POINT('Ctrl Pts',(-9.02736897016642,15.2,6.13704450853063));
#249269=CARTESIAN_POINT('Ctrl Pts',(-9.02970318136968,15.2,6.14014454804183));
#249270=CARTESIAN_POINT('Ctrl Pts',(-9.03262094561227,15.2,6.14401959774762));
#249271=CARTESIAN_POINT('Ctrl Pts',(-9.03554454809213,15.2,6.14791907070584));
#249272=CARTESIAN_POINT('Ctrl Pts',(-9.03847373559184,15.2,6.15184290021845));
#249273=CARTESIAN_POINT('Ctrl Pts',(-9.04140292309154,15.2,6.15576672973106));
#249274=CARTESIAN_POINT('Ctrl Pts',(-9.04433769423584,15.2,6.15971491420819));
#249275=CARTESIAN_POINT('Ctrl Pts',(-9.04727780083279,15.2,6.16368738879028));
#249276=CARTESIAN_POINT('Ctrl Pts',(-9.04962988623855,15.2,6.16686536862914));
#249277=CARTESIAN_POINT('Ctrl Pts',(-9.05198538539287,15.2,6.17005889342631));
#249278=CARTESIAN_POINT('Ctrl Pts',(-9.054344171584,15.2,6.17326792870733));
#249279=CARTESIAN_POINT('Ctrl Pts',(-9.05670295745375,15.2,6.17647696355111));
#249280=CARTESIAN_POINT('Ctrl Pts',(-9.05906502981693,15.2,6.1797015089844));
#249281=CARTESIAN_POINT('Ctrl Pts',(-9.06143026429005,15.2,6.18294152971853));
#249282=CARTESIAN_POINT('Ctrl Pts',(-9.06379549908542,15.2,6.1861815508941));
#249283=CARTESIAN_POINT('Ctrl Pts',(-9.06616389414783,15.2,6.18943704827154));
#249284=CARTESIAN_POINT('Ctrl Pts',(-9.06853532694394,15.2,6.19270798678414));
#249285=CARTESIAN_POINT('Ctrl Pts',(-9.07090675941694,15.2,6.19597892485107));
#249286=CARTESIAN_POINT('Ctrl Pts',(-9.07328122888098,15.2,6.19926530339546));
#249287=CARTESIAN_POINT('Ctrl Pts',(-9.07565861085301,15.2,6.20256708873509));
#249288=CARTESIAN_POINT('Ctrl Pts',(-9.07863033856098,15.2,6.20669432074703));
#249289=CARTESIAN_POINT('Ctrl Pts',(-9.08160662041098,15.2,6.21084562673059));
#249290=CARTESIAN_POINT('Ctrl Pts',(-9.08458721562906,15.2,6.21502093575699));
#249291=CARTESIAN_POINT('Ctrl Pts',(-9.08756781084713,15.2,6.21919624478339));
#249292=CARTESIAN_POINT('Ctrl Pts',(-9.09055272029924,15.2,6.22339555860844));
#249293=CARTESIAN_POINT('Ctrl Pts',(-9.09354170877125,15.2,6.22761880819053));
#249294=CARTESIAN_POINT('Ctrl Pts',(-9.09653069724327,15.2,6.23184205777262));
#249295=CARTESIAN_POINT('Ctrl Pts',(-9.09952376441539,15.2,6.23608924427754));
#249296=CARTESIAN_POINT('Ctrl Pts',(-9.10252067934573,15.2,6.24036029872074));
#249297=CARTESIAN_POINT('Ctrl Pts',(-9.10491821142068,15.2,6.24377714246151));
#249298=CARTESIAN_POINT('Ctrl Pts',(-9.10731820368361,15.2,6.24720926038603));
#249299=CARTESIAN_POINT('Ctrl Pts',(-9.10972054132366,15.2,6.25065661969191));
#249300=CARTESIAN_POINT('Ctrl Pts',(-9.11212287863637,15.2,6.25410397852807));
#249301=CARTESIAN_POINT('Ctrl Pts',(-9.11452755958632,15.2,6.2575665783205));
#249302=CARTESIAN_POINT('Ctrl Pts',(-9.1169344687783,15.2,6.26104438242409));
#249303=CARTESIAN_POINT('Ctrl Pts',(-9.11934137829823,15.2,6.26452218700154));
#249304=CARTESIAN_POINT('Ctrl Pts',(-9.12175051450451,15.2,6.26801519705856));
#249305=CARTESIAN_POINT('Ctrl Pts',(-9.12416176341386,15.2,6.27152337752853));
#249306=CARTESIAN_POINT('Ctrl Pts',(-9.12657301199466,15.2,6.27503155752052));
#249307=CARTESIAN_POINT('Ctrl Pts',(-9.12898637241543,15.2,6.2785549070337));
#249308=CARTESIAN_POINT('Ctrl Pts',(-9.13140173044957,15.2,6.28209339125321));
#249309=CARTESIAN_POINT('Ctrl Pts',(-9.1338170888128,15.2,6.28563187595485));
#249310=CARTESIAN_POINT('Ctrl Pts',(-9.13623444385753,15.2,6.28918549549077));
#249311=CARTESIAN_POINT('Ctrl Pts',(-9.13865368348951,15.2,6.29275421457515));
#249312=CARTESIAN_POINT('Ctrl Pts',(-9.14107292279187,15.2,6.2963229331733));
#249313=CARTESIAN_POINT('Ctrl Pts',(-9.14349404691327,15.2,6.29990675040727));
#249314=CARTESIAN_POINT('Ctrl Pts',(-9.1459169416039,15.2,6.30350563244484));
#249315=CARTESIAN_POINT('Ctrl Pts',(-9.14833983662467,15.2,6.30710451497278));
#249316=CARTESIAN_POINT('Ctrl Pts',(-9.15076450382512,15.2,6.310718461502));
#249317=CARTESIAN_POINT('Ctrl Pts',(-9.15319083096837,15.2,6.31434743599407));
#249318=CARTESIAN_POINT('Ctrl Pts',(-9.15561715778103,15.2,6.31797640999169));
#249319=CARTESIAN_POINT('Ctrl Pts',(-9.15804514545436,15.2,6.32162041310233));
#249320=CARTESIAN_POINT('Ctrl Pts',(-9.16047468331115,15.2,6.32527940913501));
#249321=CARTESIAN_POINT('Ctrl Pts',(-9.16290422149896,15.2,6.32893840566623));
#249322=CARTESIAN_POINT('Ctrl Pts',(-9.16533530998415,15.2,6.33261239456278));
#249323=CARTESIAN_POINT('Ctrl Pts',(-9.16776783778338,15.2,6.33630134104159));
#249324=CARTESIAN_POINT('Ctrl Pts',(-9.17020036558262,15.2,6.33999028752041));
#249325=CARTESIAN_POINT('Ctrl Pts',(-9.17263433607927,15.2,6.34369419127602));
#249326=CARTESIAN_POINT('Ctrl Pts',(-9.17506963715656,15.2,6.3474130175913));
#249327=CARTESIAN_POINT('Ctrl Pts',(-9.17689611279862,15.2,6.35020213707441));
#249328=CARTESIAN_POINT('Ctrl Pts',(-9.17872333796206,15.2,6.35299964865368));
#249329=CARTESIAN_POINT('Ctrl Pts',(-9.18055126761205,15.2,6.35580553981788));
#249330=CARTESIAN_POINT('Ctrl Pts',(-9.18237919726203,15.2,6.35861143098207));
#249331=CARTESIAN_POINT('Ctrl Pts',(-9.18420783059919,15.2,6.36142569972623));
#249332=CARTESIAN_POINT('Ctrl Pts',(-9.18603712274112,15.2,6.36424833229107));
#249333=CARTESIAN_POINT('Ctrl Pts',(-9.18786641488304,15.2,6.3670709648559));
#249334=CARTESIAN_POINT('Ctrl Pts',(-9.1896963666499,15.2,6.36990196020309));
#249335=CARTESIAN_POINT('Ctrl Pts',(-9.19152693225005,15.2,6.37274130426659));
#249336=CARTESIAN_POINT('Ctrl Pts',(-9.19396768660528,15.2,6.37652709669512));
#249337=CARTESIAN_POINT('Ctrl Pts',(-9.19640953221067,15.2,6.3803277310171));
#249338=CARTESIAN_POINT('Ctrl Pts',(-9.19885236589946,15.2,6.38414316961543));
#249339=CARTESIAN_POINT('Ctrl Pts',(-9.20068449099963,15.2,6.38700474830425));
#249340=CARTESIAN_POINT('Ctrl Pts',(-9.20251717106304,15.2,6.38987465506671));
#249341=CARTESIAN_POINT('Ctrl Pts',(-9.20435036137973,15.2,6.39275287527354));
#249342=CARTESIAN_POINT('Ctrl Pts',(-9.20618355169643,15.2,6.39563109548038));
#249343=CARTESIAN_POINT('Ctrl Pts',(-9.20801725426658,15.2,6.39851762778671));
#249344=CARTESIAN_POINT('Ctrl Pts',(-9.20985142294998,15.2,6.40141245830726));
#249345=CARTESIAN_POINT('Ctrl Pts',(-9.21168559163339,15.2,6.40430728882783));
#249346=CARTESIAN_POINT('Ctrl Pts',(-9.21352022765006,15.2,6.4072104164557));
#249347=CARTESIAN_POINT('Ctrl Pts',(-9.21535528729172,15.2,6.41012182705825));
#249348=CARTESIAN_POINT('Ctrl Pts',(-9.21719034693338,15.2,6.41303323766081));
#249349=CARTESIAN_POINT('Ctrl Pts',(-9.21902582983335,15.2,6.41595293105468));
#249350=CARTESIAN_POINT('Ctrl Pts',(-9.22086169351662,15.2,6.41888089165592));
#249351=CARTESIAN_POINT('Ctrl Pts',(-9.22269755719989,15.2,6.42180885225716));
#249352=CARTESIAN_POINT('Ctrl Pts',(-9.22453380211974,15.2,6.42474507917449));
#249353=CARTESIAN_POINT('Ctrl Pts',(-9.22637038389473,15.2,6.42768955892199));
#249354=CARTESIAN_POINT('Ctrl Pts',(-9.22820696566971,15.2,6.43063403866949));
#249355=CARTESIAN_POINT('Ctrl Pts',(-9.23004388491633,15.2,6.43358677072982));
#249356=CARTESIAN_POINT('Ctrl Pts',(-9.23188109905787,15.2,6.43654773932944));
#249357=CARTESIAN_POINT('Ctrl Pts',(-9.23371831353317,15.2,6.43950870846697));
#249358=CARTESIAN_POINT('Ctrl Pts',(-9.23555582266689,15.2,6.44247791406516));
#249359=CARTESIAN_POINT('Ctrl Pts',(-9.23739358464236,15.2,6.44545534212402));
#249360=CARTESIAN_POINT('Ctrl Pts',(-9.23923134628397,15.2,6.44843276964198));
#249361=CARTESIAN_POINT('Ctrl Pts',(-9.24106936066719,15.2,6.45141841821779));
#249362=CARTESIAN_POINT('Ctrl Pts',(-9.24290758443376,15.2,6.45441227285973));
#249363=CARTESIAN_POINT('Ctrl Pts',(-9.24474580820032,15.2,6.45740612750166));
#249364=CARTESIAN_POINT('Ctrl Pts',(-9.24658424357686,15.2,6.46040818908168));
#249365=CARTESIAN_POINT('Ctrl Pts',(-9.24842284722673,15.2,6.463418441236));
#249366=CARTESIAN_POINT('Ctrl Pts',(-9.2502614508766,15.2,6.46642869339033));
#249367=CARTESIAN_POINT('Ctrl Pts',(-9.25210022259017,15.2,6.4694471368601));
#249368=CARTESIAN_POINT('Ctrl Pts',(-9.25393912124005,15.2,6.47247375551385));
#249369=CARTESIAN_POINT('Ctrl Pts',(-9.25639098632926,15.2,6.47650924741873));
#249370=CARTESIAN_POINT('Ctrl Pts',(-9.25884307671734,15.2,6.48055927529425));
#249371=CARTESIAN_POINT('Ctrl Pts',(-9.26129529518433,15.2,6.48462379990616));
#249372=CARTESIAN_POINT('Ctrl Pts',(-9.26313445886752,15.2,6.48767219308819));
#249373=CARTESIAN_POINT('Ctrl Pts',(-9.26497369475068,15.2,6.49072874192808));
#249374=CARTESIAN_POINT('Ctrl Pts',(-9.26681296143387,15.2,6.49379343006745));
#249375=CARTESIAN_POINT('Ctrl Pts',(-9.26926531690006,15.2,6.49787968073436));
#249376=CARTESIAN_POINT('Ctrl Pts',(-9.27171772659957,15.2,6.50198040274556));
#249377=CARTESIAN_POINT('Ctrl Pts',(-9.27417009539909,15.2,6.5060955593521));
#249378=CARTESIAN_POINT('Ctrl Pts',(-9.2760093724164,15.2,6.50918192750788));
#249379=CARTESIAN_POINT('Ctrl Pts',(-9.27784862660039,15.2,6.51227641499096));
#249380=CARTESIAN_POINT('Ctrl Pts',(-9.27968781665933,15.2,6.51537900619297));
#249381=CARTESIAN_POINT('Ctrl Pts',(-9.2821400695144,15.2,6.5195157935229));
#249382=CARTESIAN_POINT('Ctrl Pts',(-9.28459220919047,15.2,6.52366698851598));
#249383=CARTESIAN_POINT('Ctrl Pts',(-9.28704414072339,15.2,6.52783255380543));
#249384=CARTESIAN_POINT('Ctrl Pts',(-9.2888830894566,15.2,6.53095672791441));
#249385=CARTESIAN_POINT('Ctrl Pts',(-9.29072192151643,15.2,6.53408898525591));
#249386=CARTESIAN_POINT('Ctrl Pts',(-9.29256059578298,15.2,6.5372293103911));
#249387=CARTESIAN_POINT('Ctrl Pts',(-9.29439927004952,15.2,6.5403696355263));
#249388=CARTESIAN_POINT('Ctrl Pts',(-9.29623778788273,15.2,6.54351802901093));
#249389=CARTESIAN_POINT('Ctrl Pts',(-9.29807610906597,15.2,6.54667447510349));
#249390=CARTESIAN_POINT('Ctrl Pts',(-9.29991443058316,15.2,6.54983092176947));
#249391=CARTESIAN_POINT('Ctrl Pts',(-9.30175255521699,15.2,6.55299542101272));
#249392=CARTESIAN_POINT('Ctrl Pts',(-9.30359044515072,15.2,6.55616795718322));
#249393=CARTESIAN_POINT('Ctrl Pts',(-9.30604096450588,15.2,6.56039800444996));
#249394=CARTESIAN_POINT('Ctrl Pts',(-9.30849106419308,15.2,6.56464234033144));
#249395=CARTESIAN_POINT('Ctrl Pts',(-9.31094065178172,15.2,6.56890092644704));
#249396=CARTESIAN_POINT('Ctrl Pts',(-9.31277784255665,15.2,6.57209486617879));
#249397=CARTESIAN_POINT('Ctrl Pts',(-9.31461474548323,15.2,6.57529682375083));
#249398=CARTESIAN_POINT('Ctrl Pts',(-9.31645132174987,15.2,6.57850678092517));
#249399=CARTESIAN_POINT('Ctrl Pts',(-9.3189000903278,15.2,6.58278672421304));
#249400=CARTESIAN_POINT('Ctrl Pts',(-9.32134827841678,15.2,6.58708089179985));
#249401=CARTESIAN_POINT('Ctrl Pts',(-9.3237957962168,15.2,6.59138924636893));
#249402=CARTESIAN_POINT('Ctrl Pts',(-9.32624331368334,15.2,6.59569760035099));
#249403=CARTESIAN_POINT('Ctrl Pts',(-9.32869016070891,15.2,6.60002014240703));
#249404=CARTESIAN_POINT('Ctrl Pts',(-9.33113624368678,15.2,6.60435683387906));
#249405=CARTESIAN_POINT('Ctrl Pts',(-9.3329708060035,15.2,6.6076093526308));
#249406=CARTESIAN_POINT('Ctrl Pts',(-9.33480493850019,15.2,6.61086983112389));
#249407=CARTESIAN_POINT('Ctrl Pts',(-9.33663860239199,15.2,6.61413825183742));
#249408=CARTESIAN_POINT('Ctrl Pts',(-9.33908348780312,15.2,6.61849614651796));
#249409=CARTESIAN_POINT('Ctrl Pts',(-9.34152754303359,15.2,6.62286816468036));
#249410=CARTESIAN_POINT('Ctrl Pts',(-9.34397068750006,15.2,6.62725426997492));
#249411=CARTESIAN_POINT('Ctrl Pts',(-9.34580304568348,15.2,6.63054384864704));
#249412=CARTESIAN_POINT('Ctrl Pts',(-9.34763489121691,15.2,6.6338413530272));
#249413=CARTESIAN_POINT('Ctrl Pts',(-9.34946618127544,15.2,6.63714676361477));
#249414=CARTESIAN_POINT('Ctrl Pts',(-9.35190790157527,15.2,6.64155397813186));
#249415=CARTESIAN_POINT('Ctrl Pts',(-9.35434863068266,15.2,6.64597524940131));
#249416=CARTESIAN_POINT('Ctrl Pts',(-9.35678826960406,15.2,6.6504105336436));
#249417=CARTESIAN_POINT('Ctrl Pts',(-9.35861799862891,15.2,6.65373699652316));
#249418=CARTESIAN_POINT('Ctrl Pts',(-9.3604471149025,15.2,6.65707134311622));
#249419=CARTESIAN_POINT('Ctrl Pts',(-9.36227560168603,15.2,6.66041356487327));
#249420=CARTESIAN_POINT('Ctrl Pts',(-9.36410408846955,15.2,6.66375578663033));
#249421=CARTESIAN_POINT('Ctrl Pts',(-9.36593194966811,15.2,6.66710588438994));
#249422=CARTESIAN_POINT('Ctrl Pts',(-9.36775917500006,15.2,6.67046385499999));
#249423=CARTESIAN_POINT('Origin',(-5.66257110645729E-14,15.2,-1.77635683940025E-14));
#249424=CARTESIAN_POINT('',(-8.88241603300006,15.2,5.36127880599999));
#249425=CARTESIAN_POINT('',(-8.88241603300006,12.2,5.36127880599999));
#249426=CARTESIAN_POINT('',(-8.88241603300006,15.2,5.36127880599999));
#249427=CARTESIAN_POINT('Origin',(-5.66257110645729E-14,12.2,-1.77635683940025E-14));
#249428=CARTESIAN_POINT('Origin',(-5.66257110645729E-14,15.2,-1.77635683940025E-14));
#249429=CARTESIAN_POINT('Origin',(-5.66257110645729E-14,15.2,-1.77635683940025E-14));
#249430=CARTESIAN_POINT('',(-10.0402696494501,15.2,5.60740451254565));
#249431=CARTESIAN_POINT('',(-10.2217148785197,15.2,5.26939701892417));
#249432=CARTESIAN_POINT('Origin',(-5.66257110645729E-14,15.2,-1.77635683940025E-14));
#249433=CARTESIAN_POINT('',(-10.2217148785197,12.2,5.26939701892417));
#249434=CARTESIAN_POINT('',(-10.2217148790001,15.2,5.26939701899998));
#249435=CARTESIAN_POINT('',(-10.0402696494501,12.2,5.60740451254564));
#249436=CARTESIAN_POINT('Origin',(-5.66257110645729E-14,12.2,-1.77635683940025E-14));
#249437=CARTESIAN_POINT('',(-10.0402696500001,15.2,5.60740451299999));
#249438=CARTESIAN_POINT('Ctrl Pts',(-10.2217148780001,15.2,5.26939701899998));
#249439=CARTESIAN_POINT('Ctrl Pts',(-10.2217148780001,11.6,5.26939701899998));
#249440=CARTESIAN_POINT('Ctrl Pts',(-10.2212575740001,15.2,5.26878426899999));
#249441=CARTESIAN_POINT('Ctrl Pts',(-10.2212575740001,11.6,5.26878426899999));
#249442=CARTESIAN_POINT('Ctrl Pts',(-10.2203430010001,15.2,5.26755929399998));
#249443=CARTESIAN_POINT('Ctrl Pts',(-10.2203430010001,11.6,5.26755929399998));
#249444=CARTESIAN_POINT('Ctrl Pts',(-10.2189712390001,15.2,5.26572340899998));
#249445=CARTESIAN_POINT('Ctrl Pts',(-10.2189712390001,11.6,5.26572340899998));
#249446=CARTESIAN_POINT('Ctrl Pts',(-10.2171424210001,15.2,5.26327871599998));
#249447=CARTESIAN_POINT('Ctrl Pts',(-10.2171424210001,11.6,5.26327871599998));
#249448=CARTESIAN_POINT('Ctrl Pts',(-10.2148567310001,15.2,5.26022810499998));
#249449=CARTESIAN_POINT('Ctrl Pts',(-10.2148567310001,11.6,5.26022810499998));
#249450=CARTESIAN_POINT('Ctrl Pts',(-10.2125713740001,15.2,5.25718275199999));
#249451=CARTESIAN_POINT('Ctrl Pts',(-10.2125713740001,11.6,5.25718275199999));
#249452=CARTESIAN_POINT('Ctrl Pts',(-10.2102863520001,15.2,5.25414265499998));
#249453=CARTESIAN_POINT('Ctrl Pts',(-10.2102863520001,11.6,5.25414265499998));
#249454=CARTESIAN_POINT('Ctrl Pts',(-10.2080016700001,15.2,5.25110781899999));
#249455=CARTESIAN_POINT('Ctrl Pts',(-10.2080016700001,11.6,5.25110781899999));
#249456=CARTESIAN_POINT('Ctrl Pts',(-10.2057173310001,15.2,5.24807824199998));
#249457=CARTESIAN_POINT('Ctrl Pts',(-10.2057173310001,11.6,5.24807824199998));
#249458=CARTESIAN_POINT('Ctrl Pts',(-10.2034333450001,15.2,5.24505392699999));
#249459=CARTESIAN_POINT('Ctrl Pts',(-10.2034333450001,11.6,5.24505392699999));
#249460=CARTESIAN_POINT('Ctrl Pts',(-10.2011497210001,15.2,5.24203487699998));
#249461=CARTESIAN_POINT('Ctrl Pts',(-10.2011497210001,11.6,5.24203487699998));
#249462=CARTESIAN_POINT('Ctrl Pts',(-10.1988664690001,15.2,5.23902109499998));
#249463=CARTESIAN_POINT('Ctrl Pts',(-10.1988664690001,11.6,5.23902109499998));
#249464=CARTESIAN_POINT('Ctrl Pts',(-10.1965836000001,15.2,5.23601258299998));
#249465=CARTESIAN_POINT('Ctrl Pts',(-10.1965836000001,11.6,5.23601258299998));
#249466=CARTESIAN_POINT('Ctrl Pts',(-10.1943011260001,15.2,5.23300934399998));
#249467=CARTESIAN_POINT('Ctrl Pts',(-10.1943011260001,11.6,5.23300934399998));
#249468=CARTESIAN_POINT('Ctrl Pts',(-10.1920190550001,15.2,5.23001137999999));
#249469=CARTESIAN_POINT('Ctrl Pts',(-10.1920190550001,11.6,5.23001137999999));
#249470=CARTESIAN_POINT('Ctrl Pts',(-10.1897373990001,15.2,5.22701869499999));
#249471=CARTESIAN_POINT('Ctrl Pts',(-10.1897373990001,11.6,5.22701869499999));
#249472=CARTESIAN_POINT('Ctrl Pts',(-10.1874561630001,15.2,5.22403128999999));
#249473=CARTESIAN_POINT('Ctrl Pts',(-10.1874561630001,11.6,5.22403128999999));
#249474=CARTESIAN_POINT('Ctrl Pts',(-10.1851753570001,15.2,5.22104916599999));
#249475=CARTESIAN_POINT('Ctrl Pts',(-10.1851753570001,11.6,5.22104916599999));
#249476=CARTESIAN_POINT('Ctrl Pts',(-10.1828949880001,15.2,5.21807232799999));
#249477=CARTESIAN_POINT('Ctrl Pts',(-10.1828949880001,11.6,5.21807232799999));
#249478=CARTESIAN_POINT('Ctrl Pts',(-10.1806150650001,15.2,5.21510077499999));
#249479=CARTESIAN_POINT('Ctrl Pts',(-10.1806150650001,11.6,5.21510077499999));
#249480=CARTESIAN_POINT('Ctrl Pts',(-10.1783355960001,15.2,5.21213451099998));
#249481=CARTESIAN_POINT('Ctrl Pts',(-10.1783355960001,11.6,5.21213451099998));
#249482=CARTESIAN_POINT('Ctrl Pts',(-10.1760565880001,15.2,5.20917353699998));
#249483=CARTESIAN_POINT('Ctrl Pts',(-10.1760565880001,11.6,5.20917353699998));
#249484=CARTESIAN_POINT('Ctrl Pts',(-10.1737780520001,15.2,5.20621785499999));
#249485=CARTESIAN_POINT('Ctrl Pts',(-10.1737780520001,11.6,5.20621785499999));
#249486=CARTESIAN_POINT('Ctrl Pts',(-10.1714999970001,15.2,5.20326746899999));
#249487=CARTESIAN_POINT('Ctrl Pts',(-10.1714999970001,11.6,5.20326746899999));
#249488=CARTESIAN_POINT('Ctrl Pts',(-10.1692224320001,15.2,5.20032237999998));
#249489=CARTESIAN_POINT('Ctrl Pts',(-10.1692224320001,11.6,5.20032237999998));
#249490=CARTESIAN_POINT('Ctrl Pts',(-10.1669453660001,15.2,5.19738259099999));
#249491=CARTESIAN_POINT('Ctrl Pts',(-10.1669453660001,11.6,5.19738259099999));
#249492=CARTESIAN_POINT('Ctrl Pts',(-10.1646688090001,15.2,5.19444810399998));
#249493=CARTESIAN_POINT('Ctrl Pts',(-10.1646688090001,11.6,5.19444810399998));
#249494=CARTESIAN_POINT('Ctrl Pts',(-10.1623927680001,15.2,5.19151892199999));
#249495=CARTESIAN_POINT('Ctrl Pts',(-10.1623927680001,11.6,5.19151892199999));
#249496=CARTESIAN_POINT('Ctrl Pts',(-10.1601172530001,15.2,5.18859504499999));
#249497=CARTESIAN_POINT('Ctrl Pts',(-10.1601172530001,11.6,5.18859504499999));
#249498=CARTESIAN_POINT('Ctrl Pts',(-10.1578422740001,15.2,5.18567647699999));
#249499=CARTESIAN_POINT('Ctrl Pts',(-10.1578422740001,11.6,5.18567647699999));
#249500=CARTESIAN_POINT('Ctrl Pts',(-10.1555678380001,15.2,5.18276321899998));
#249501=CARTESIAN_POINT('Ctrl Pts',(-10.1555678380001,11.6,5.18276321899998));
#249502=CARTESIAN_POINT('Ctrl Pts',(-10.1532939540001,15.2,5.17985527399999));
#249503=CARTESIAN_POINT('Ctrl Pts',(-10.1532939540001,11.6,5.17985527399999));
#249504=CARTESIAN_POINT('Ctrl Pts',(-10.1510206320001,15.2,5.17695264399999));
#249505=CARTESIAN_POINT('Ctrl Pts',(-10.1510206320001,11.6,5.17695264399999));
#249506=CARTESIAN_POINT('Ctrl Pts',(-10.1487478800001,15.2,5.17405533199998));
#249507=CARTESIAN_POINT('Ctrl Pts',(-10.1487478800001,11.6,5.17405533199998));
#249508=CARTESIAN_POINT('Ctrl Pts',(-10.1464757090001,15.2,5.17116333899998));
#249509=CARTESIAN_POINT('Ctrl Pts',(-10.1464757090001,11.6,5.17116333899998));
#249510=CARTESIAN_POINT('Ctrl Pts',(-10.1442041250001,15.2,5.16827666599998));
#249511=CARTESIAN_POINT('Ctrl Pts',(-10.1442041250001,11.6,5.16827666599998));
#249512=CARTESIAN_POINT('Ctrl Pts',(-10.1419331390001,15.2,5.16539531899999));
#249513=CARTESIAN_POINT('Ctrl Pts',(-10.1419331390001,11.6,5.16539531899999));
#249514=CARTESIAN_POINT('Ctrl Pts',(-10.1396627610001,15.2,5.16251929699998));
#249515=CARTESIAN_POINT('Ctrl Pts',(-10.1396627610001,11.6,5.16251929699998));
#249516=CARTESIAN_POINT('Ctrl Pts',(-10.1373930000001,15.2,5.15964860299999));
#249517=CARTESIAN_POINT('Ctrl Pts',(-10.1373930000001,11.6,5.15964860299999));
#249518=CARTESIAN_POINT('Ctrl Pts',(-10.1351238630001,15.2,5.15678323899999));
#249519=CARTESIAN_POINT('Ctrl Pts',(-10.1351238630001,11.6,5.15678323899999));
#249520=CARTESIAN_POINT('Ctrl Pts',(-10.1328553600001,15.2,5.15392320699998));
#249521=CARTESIAN_POINT('Ctrl Pts',(-10.1328553600001,11.6,5.15392320699998));
#249522=CARTESIAN_POINT('Ctrl Pts',(-10.1305875000001,15.2,5.15106850999998));
#249523=CARTESIAN_POINT('Ctrl Pts',(-10.1305875000001,11.6,5.15106850999998));
#249524=CARTESIAN_POINT('Ctrl Pts',(-10.1283202940001,15.2,5.14821914899999));
#249525=CARTESIAN_POINT('Ctrl Pts',(-10.1283202940001,11.6,5.14821914899999));
#249526=CARTESIAN_POINT('Ctrl Pts',(-10.1260537500001,15.2,5.14537512799999));
#249527=CARTESIAN_POINT('Ctrl Pts',(-10.1260537500001,11.6,5.14537512799999));
#249528=CARTESIAN_POINT('Ctrl Pts',(-10.1237878770001,15.2,5.14253644699998));
#249529=CARTESIAN_POINT('Ctrl Pts',(-10.1237878770001,11.6,5.14253644699998));
#249530=CARTESIAN_POINT('Ctrl Pts',(-10.1215226840001,15.2,5.13970310999999));
#249531=CARTESIAN_POINT('Ctrl Pts',(-10.1215226840001,11.6,5.13970310999999));
#249532=CARTESIAN_POINT('Ctrl Pts',(-10.1192581800001,15.2,5.13687511699998));
#249533=CARTESIAN_POINT('Ctrl Pts',(-10.1192581800001,11.6,5.13687511699998));
#249534=CARTESIAN_POINT('Ctrl Pts',(-10.1169943770001,15.2,5.13405247199999));
#249535=CARTESIAN_POINT('Ctrl Pts',(-10.1169943770001,11.6,5.13405247199999));
#249536=CARTESIAN_POINT('Ctrl Pts',(-10.1147312810001,15.2,5.13123517699999));
#249537=CARTESIAN_POINT('Ctrl Pts',(-10.1147312810001,11.6,5.13123517699999));
#249538=CARTESIAN_POINT('Ctrl Pts',(-10.1124689020001,15.2,5.12842323299999));
#249539=CARTESIAN_POINT('Ctrl Pts',(-10.1124689020001,11.6,5.12842323299999));
#249540=CARTESIAN_POINT('Ctrl Pts',(-10.1102072500001,15.2,5.12561664199998));
#249541=CARTESIAN_POINT('Ctrl Pts',(-10.1102072500001,11.6,5.12561664199998));
#249542=CARTESIAN_POINT('Ctrl Pts',(-10.1079463350001,15.2,5.12281540799999));
#249543=CARTESIAN_POINT('Ctrl Pts',(-10.1079463350001,11.6,5.12281540799999));
#249544=CARTESIAN_POINT('Ctrl Pts',(-10.1056861660001,15.2,5.12001953099999));
#249545=CARTESIAN_POINT('Ctrl Pts',(-10.1056861660001,11.6,5.12001953099999));
#249546=CARTESIAN_POINT('Ctrl Pts',(-10.1034267510001,15.2,5.11722901499999));
#249547=CARTESIAN_POINT('Ctrl Pts',(-10.1034267510001,11.6,5.11722901499999));
#249548=CARTESIAN_POINT('Ctrl Pts',(-10.1011681000001,15.2,5.11444385899999));
#249549=CARTESIAN_POINT('Ctrl Pts',(-10.1011681000001,11.6,5.11444385899999));
#249550=CARTESIAN_POINT('Ctrl Pts',(-10.0989102230001,15.2,5.11166406999998));
#249551=CARTESIAN_POINT('Ctrl Pts',(-10.0989102230001,11.6,5.11166406999998));
#249552=CARTESIAN_POINT('Ctrl Pts',(-10.0966531300001,15.2,5.10888964599998));
#249553=CARTESIAN_POINT('Ctrl Pts',(-10.0966531300001,11.6,5.10888964599998));
#249554=CARTESIAN_POINT('Ctrl Pts',(-10.0943968300001,15.2,5.10612058999998));
#249555=CARTESIAN_POINT('Ctrl Pts',(-10.0943968300001,11.6,5.10612058999998));
#249556=CARTESIAN_POINT('Ctrl Pts',(-10.0921413310001,15.2,5.10335690499998));
#249557=CARTESIAN_POINT('Ctrl Pts',(-10.0921413310001,11.6,5.10335690499998));
#249558=CARTESIAN_POINT('Ctrl Pts',(-10.0898866440001,15.2,5.10059859299999));
#249559=CARTESIAN_POINT('Ctrl Pts',(-10.0898866440001,11.6,5.10059859299999));
#249560=CARTESIAN_POINT('Ctrl Pts',(-10.0876327790001,15.2,5.09784565499999));
#249561=CARTESIAN_POINT('Ctrl Pts',(-10.0876327790001,11.6,5.09784565499999));
#249562=CARTESIAN_POINT('Ctrl Pts',(-10.0853797440001,15.2,5.09509809399999));
#249563=CARTESIAN_POINT('Ctrl Pts',(-10.0853797440001,11.6,5.09509809399999));
#249564=CARTESIAN_POINT('Ctrl Pts',(-10.0831275500001,15.2,5.09235591199998));
#249565=CARTESIAN_POINT('Ctrl Pts',(-10.0831275500001,11.6,5.09235591199998));
#249566=CARTESIAN_POINT('Ctrl Pts',(-10.0808762050001,15.2,5.08961910999999));
#249567=CARTESIAN_POINT('Ctrl Pts',(-10.0808762050001,11.6,5.08961910999999));
#249568=CARTESIAN_POINT('Ctrl Pts',(-10.0786257200001,15.2,5.08688769099999));
#249569=CARTESIAN_POINT('Ctrl Pts',(-10.0786257200001,11.6,5.08688769099999));
#249570=CARTESIAN_POINT('Ctrl Pts',(-10.0763761030001,15.2,5.08416165899998));
#249571=CARTESIAN_POINT('Ctrl Pts',(-10.0763761030001,11.6,5.08416165899998));
#249572=CARTESIAN_POINT('Ctrl Pts',(-10.0741273660001,15.2,5.08144101199999));
#249573=CARTESIAN_POINT('Ctrl Pts',(-10.0741273660001,11.6,5.08144101199999));
#249574=CARTESIAN_POINT('Ctrl Pts',(-10.0718795170001,15.2,5.07872575499999));
#249575=CARTESIAN_POINT('Ctrl Pts',(-10.0718795170001,11.6,5.07872575499999));
#249576=CARTESIAN_POINT('Ctrl Pts',(-10.0696325650001,15.2,5.07601588799999));
#249577=CARTESIAN_POINT('Ctrl Pts',(-10.0696325650001,11.6,5.07601588799999));
#249578=CARTESIAN_POINT('Ctrl Pts',(-10.0673865220001,15.2,5.07331141599998));
#249579=CARTESIAN_POINT('Ctrl Pts',(-10.0673865220001,11.6,5.07331141599998));
#249580=CARTESIAN_POINT('Ctrl Pts',(-10.0651413960001,15.2,5.07061233799998));
#249581=CARTESIAN_POINT('Ctrl Pts',(-10.0651413960001,11.6,5.07061233799998));
#249582=CARTESIAN_POINT('Ctrl Pts',(-10.0628971970001,15.2,5.06791865699999));
#249583=CARTESIAN_POINT('Ctrl Pts',(-10.0628971970001,11.6,5.06791865699999));
#249584=CARTESIAN_POINT('Ctrl Pts',(-10.0606539350001,15.2,5.06523037599998));
#249585=CARTESIAN_POINT('Ctrl Pts',(-10.0606539350001,11.6,5.06523037599998));
#249586=CARTESIAN_POINT('Ctrl Pts',(-10.0584116200001,15.2,5.06254749499998));
#249587=CARTESIAN_POINT('Ctrl Pts',(-10.0584116200001,11.6,5.06254749499998));
#249588=CARTESIAN_POINT('Ctrl Pts',(-10.0561702600001,15.2,5.05987001899998));
#249589=CARTESIAN_POINT('Ctrl Pts',(-10.0561702600001,11.6,5.05987001899998));
#249590=CARTESIAN_POINT('Ctrl Pts',(-10.0539298680001,15.2,5.05719794699999));
#249591=CARTESIAN_POINT('Ctrl Pts',(-10.0539298680001,11.6,5.05719794699999));
#249592=CARTESIAN_POINT('Ctrl Pts',(-10.0516904520001,15.2,5.05453128299998));
#249593=CARTESIAN_POINT('Ctrl Pts',(-10.0516904520001,11.6,5.05453128299998));
#249594=CARTESIAN_POINT('Ctrl Pts',(-10.0494520200001,15.2,5.05187002899999));
#249595=CARTESIAN_POINT('Ctrl Pts',(-10.0494520200001,11.6,5.05187002899999));
#249596=CARTESIAN_POINT('Ctrl Pts',(-10.0472145860001,15.2,5.04921418599999));
#249597=CARTESIAN_POINT('Ctrl Pts',(-10.0472145860001,11.6,5.04921418599999));
#249598=CARTESIAN_POINT('Ctrl Pts',(-10.0449781570001,15.2,5.04656375599998));
#249599=CARTESIAN_POINT('Ctrl Pts',(-10.0449781570001,11.6,5.04656375599998));
#249600=CARTESIAN_POINT('Ctrl Pts',(-10.0427427430001,15.2,5.04391874099999));
#249601=CARTESIAN_POINT('Ctrl Pts',(-10.0427427430001,11.6,5.04391874099999));
#249602=CARTESIAN_POINT('Ctrl Pts',(-10.0405083540001,15.2,5.04127914399999));
#249603=CARTESIAN_POINT('Ctrl Pts',(-10.0405083540001,11.6,5.04127914399999));
#249604=CARTESIAN_POINT('Ctrl Pts',(-10.0382750020001,15.2,5.03864496599999));
#249605=CARTESIAN_POINT('Ctrl Pts',(-10.0382750020001,11.6,5.03864496599999));
#249606=CARTESIAN_POINT('Ctrl Pts',(-10.0360426940001,15.2,5.03601620899998));
#249607=CARTESIAN_POINT('Ctrl Pts',(-10.0360426940001,11.6,5.03601620899998));
#249608=CARTESIAN_POINT('Ctrl Pts',(-10.0338114420001,15.2,5.03339287599999));
#249609=CARTESIAN_POINT('Ctrl Pts',(-10.0338114420001,11.6,5.03339287599999));
#249610=CARTESIAN_POINT('Ctrl Pts',(-10.0315812560001,15.2,5.03077496799998));
#249611=CARTESIAN_POINT('Ctrl Pts',(-10.0315812560001,11.6,5.03077496799998));
#249612=CARTESIAN_POINT('Ctrl Pts',(-10.0293521450001,15.2,5.02816248699999));
#249613=CARTESIAN_POINT('Ctrl Pts',(-10.0293521450001,11.6,5.02816248699999));
#249614=CARTESIAN_POINT('Ctrl Pts',(-10.0271241190001,15.2,5.02555543599998));
#249615=CARTESIAN_POINT('Ctrl Pts',(-10.0271241190001,11.6,5.02555543599998));
#249616=CARTESIAN_POINT('Ctrl Pts',(-10.0248971890001,15.2,5.02295381499999));
#249617=CARTESIAN_POINT('Ctrl Pts',(-10.0248971890001,11.6,5.02295381499999));
#249618=CARTESIAN_POINT('Ctrl Pts',(-10.0226713640001,15.2,5.02035762799999));
#249619=CARTESIAN_POINT('Ctrl Pts',(-10.0226713640001,11.6,5.02035762799999));
#249620=CARTESIAN_POINT('Ctrl Pts',(-10.0204466560001,15.2,5.01776687599998));
#249621=CARTESIAN_POINT('Ctrl Pts',(-10.0204466560001,11.6,5.01776687599998));
#249622=CARTESIAN_POINT('Ctrl Pts',(-10.0182230730001,15.2,5.01518155999998));
#249623=CARTESIAN_POINT('Ctrl Pts',(-10.0182230730001,11.6,5.01518155999998));
#249624=CARTESIAN_POINT('Ctrl Pts',(-10.0160006270001,15.2,5.01260168399998));
#249625=CARTESIAN_POINT('Ctrl Pts',(-10.0160006270001,11.6,5.01260168399998));
#249626=CARTESIAN_POINT('Ctrl Pts',(-10.0137793260001,15.2,5.01002724899998));
#249627=CARTESIAN_POINT('Ctrl Pts',(-10.0137793260001,11.6,5.01002724899998));
#249628=CARTESIAN_POINT('Ctrl Pts',(-10.0115591820001,15.2,5.00745825599999));
#249629=CARTESIAN_POINT('Ctrl Pts',(-10.0115591820001,11.6,5.00745825599999));
#249630=CARTESIAN_POINT('Ctrl Pts',(-10.0093402040001,15.2,5.00489470899999));
#249631=CARTESIAN_POINT('Ctrl Pts',(-10.0093402040001,11.6,5.00489470899999));
#249632=CARTESIAN_POINT('Ctrl Pts',(-10.0071224030001,15.2,5.00233660799999));
#249633=CARTESIAN_POINT('Ctrl Pts',(-10.0071224030001,11.6,5.00233660799999));
#249634=CARTESIAN_POINT('Ctrl Pts',(-10.0049057900001,15.2,4.99978395499999));
#249635=CARTESIAN_POINT('Ctrl Pts',(-10.0049057900001,11.6,4.99978395499998));
#249636=CARTESIAN_POINT('Ctrl Pts',(-10.0026903730001,15.2,4.99723675299999));
#249637=CARTESIAN_POINT('Ctrl Pts',(-10.0026903730001,11.6,4.99723675299998));
#249638=CARTESIAN_POINT('Ctrl Pts',(-10.0004761650001,15.2,4.99469500399999));
#249639=CARTESIAN_POINT('Ctrl Pts',(-10.0004761650001,11.6,4.99469500399999));
#249640=CARTESIAN_POINT('Ctrl Pts',(-9.99826317500006,15.2,4.99215870899998));
#249641=CARTESIAN_POINT('Ctrl Pts',(-9.99826317500006,11.6,4.99215870899998));
#249642=CARTESIAN_POINT('Ctrl Pts',(-9.99605141300006,15.2,4.98962787099998));
#249643=CARTESIAN_POINT('Ctrl Pts',(-9.99605141300006,11.6,4.98962787099998));
#249644=CARTESIAN_POINT('Ctrl Pts',(-9.99384088900005,15.2,4.98710248899998));
#249645=CARTESIAN_POINT('Ctrl Pts',(-9.99384088900005,11.6,4.98710248899998));
#249646=CARTESIAN_POINT('Ctrl Pts',(-9.99163161400006,15.2,4.98458256899998));
#249647=CARTESIAN_POINT('Ctrl Pts',(-9.99163161400006,11.6,4.98458256899998));
#249648=CARTESIAN_POINT('Ctrl Pts',(-9.98942360000006,15.2,4.98206810999999));
#249649=CARTESIAN_POINT('Ctrl Pts',(-9.98942360000006,11.6,4.98206810999999));
#249650=CARTESIAN_POINT('Ctrl Pts',(-9.98721685500006,15.2,4.97955911499999));
#249651=CARTESIAN_POINT('Ctrl Pts',(-9.98721685500006,11.6,4.97955911499999));
#249652=CARTESIAN_POINT('Ctrl Pts',(-9.98501139000006,15.2,4.97705558599999));
#249653=CARTESIAN_POINT('Ctrl Pts',(-9.98501139000006,11.6,4.97705558599998));
#249654=CARTESIAN_POINT('Ctrl Pts',(-9.98280721700005,15.2,4.97455752399999));
#249655=CARTESIAN_POINT('Ctrl Pts',(-9.98280721700005,11.6,4.97455752399999));
#249656=CARTESIAN_POINT('Ctrl Pts',(-9.98060434500006,15.2,4.97206493199998));
#249657=CARTESIAN_POINT('Ctrl Pts',(-9.98060434500006,11.6,4.97206493199998));
#249658=CARTESIAN_POINT('Ctrl Pts',(-9.97840278500006,15.2,4.96957781099999));
#249659=CARTESIAN_POINT('Ctrl Pts',(-9.97840278500006,11.6,4.96957781099999));
#249660=CARTESIAN_POINT('Ctrl Pts',(-9.97620254700006,15.2,4.96709616399999));
#249661=CARTESIAN_POINT('Ctrl Pts',(-9.97620254700006,11.6,4.96709616399999));
#249662=CARTESIAN_POINT('Ctrl Pts',(-9.97400364300006,15.2,4.96461999099999));
#249663=CARTESIAN_POINT('Ctrl Pts',(-9.97400364300006,11.6,4.96461999099999));
#249664=CARTESIAN_POINT('Ctrl Pts',(-9.97180608100006,15.2,4.96214929599999));
#249665=CARTESIAN_POINT('Ctrl Pts',(-9.97180608100006,11.6,4.96214929599999));
#249666=CARTESIAN_POINT('Ctrl Pts',(-9.96960987500006,15.2,4.95968407899999));
#249667=CARTESIAN_POINT('Ctrl Pts',(-9.96960987500006,11.6,4.95968407899999));
#249668=CARTESIAN_POINT('Ctrl Pts',(-9.96741503200005,15.2,4.95722434199998));
#249669=CARTESIAN_POINT('Ctrl Pts',(-9.96741503200005,11.6,4.95722434199998));
#249670=CARTESIAN_POINT('Ctrl Pts',(-9.96522156600006,15.2,4.95477008799998));
#249671=CARTESIAN_POINT('Ctrl Pts',(-9.96522156600006,11.6,4.95477008799998));
#249672=CARTESIAN_POINT('Ctrl Pts',(-9.96302948600006,15.2,4.95232131899999));
#249673=CARTESIAN_POINT('Ctrl Pts',(-9.96302948600006,11.6,4.95232131899999));
#249674=CARTESIAN_POINT('Ctrl Pts',(-9.96083880200005,15.2,4.94987803499999));
#249675=CARTESIAN_POINT('Ctrl Pts',(-9.96083880200005,11.6,4.94987803499999));
#249676=CARTESIAN_POINT('Ctrl Pts',(-9.95864952600006,15.2,4.94744023899998));
#249677=CARTESIAN_POINT('Ctrl Pts',(-9.95864952600006,11.6,4.94744023899998));
#249678=CARTESIAN_POINT('Ctrl Pts',(-9.95646166800006,15.2,4.94500793199999));
#249679=CARTESIAN_POINT('Ctrl Pts',(-9.95646166800006,11.6,4.94500793199998));
#249680=CARTESIAN_POINT('Ctrl Pts',(-9.95427524000006,15.2,4.94258111799999));
#249681=CARTESIAN_POINT('Ctrl Pts',(-9.95427524000006,11.6,4.94258111799999));
#249682=CARTESIAN_POINT('Ctrl Pts',(-9.95209025100005,15.2,4.94015979599999));
#249683=CARTESIAN_POINT('Ctrl Pts',(-9.95209025100005,11.6,4.94015979599998));
#249684=CARTESIAN_POINT('Ctrl Pts',(-9.94990671400006,15.2,4.93774396999999));
#249685=CARTESIAN_POINT('Ctrl Pts',(-9.94990671400006,11.6,4.93774396999999));
#249686=CARTESIAN_POINT('Ctrl Pts',(-9.94772463800006,15.2,4.93533364199998));
#249687=CARTESIAN_POINT('Ctrl Pts',(-9.94772463800006,11.6,4.93533364199998));
#249688=CARTESIAN_POINT('Ctrl Pts',(-9.94554403500005,15.2,4.93292881099999));
#249689=CARTESIAN_POINT('Ctrl Pts',(-9.94554403500005,11.6,4.93292881099998));
#249690=CARTESIAN_POINT('Ctrl Pts',(-9.94336491400006,15.2,4.93052947999999));
#249691=CARTESIAN_POINT('Ctrl Pts',(-9.94336491400006,11.6,4.93052947999998));
#249692=CARTESIAN_POINT('Ctrl Pts',(-9.94118728800006,15.2,4.92813565299999));
#249693=CARTESIAN_POINT('Ctrl Pts',(-9.94118728800006,11.6,4.92813565299999));
#249694=CARTESIAN_POINT('Ctrl Pts',(-9.93901116700006,15.2,4.92574732999999));
#249695=CARTESIAN_POINT('Ctrl Pts',(-9.93901116700006,11.6,4.92574732999999));
#249696=CARTESIAN_POINT('Ctrl Pts',(-9.93683656200006,15.2,4.92336451199999));
#249697=CARTESIAN_POINT('Ctrl Pts',(-9.93683656200006,11.6,4.92336451199998));
#249698=CARTESIAN_POINT('Ctrl Pts',(-9.93466348400006,15.2,4.92098720199999));
#249699=CARTESIAN_POINT('Ctrl Pts',(-9.93466348400006,11.6,4.92098720199999));
#249700=CARTESIAN_POINT('Ctrl Pts',(-9.93249194500006,15.2,4.91861540099999));
#249701=CARTESIAN_POINT('Ctrl Pts',(-9.93249194500006,11.6,4.91861540099999));
#249702=CARTESIAN_POINT('Ctrl Pts',(-9.93032195400006,15.2,4.91624911099999));
#249703=CARTESIAN_POINT('Ctrl Pts',(-9.93032195400006,11.6,4.91624911099999));
#249704=CARTESIAN_POINT('Ctrl Pts',(-9.92815352500006,15.2,4.91388833399999));
#249705=CARTESIAN_POINT('Ctrl Pts',(-9.92815352500006,11.6,4.91388833399998));
#249706=CARTESIAN_POINT('Ctrl Pts',(-9.92598666500006,15.2,4.91153307199999));
#249707=CARTESIAN_POINT('Ctrl Pts',(-9.92598666500006,11.6,4.91153307199998));
#249708=CARTESIAN_POINT('Ctrl Pts',(-9.92382138900006,15.2,4.90918332699999));
#249709=CARTESIAN_POINT('Ctrl Pts',(-9.92382138900006,11.6,4.90918332699999));
#249710=CARTESIAN_POINT('Ctrl Pts',(-9.92165770700005,15.2,4.90683909899998));
#249711=CARTESIAN_POINT('Ctrl Pts',(-9.92165770700005,11.6,4.90683909899998));
#249712=CARTESIAN_POINT('Ctrl Pts',(-9.91949562900006,15.2,4.90450039199998));
#249713=CARTESIAN_POINT('Ctrl Pts',(-9.91949562900006,11.6,4.90450039199998));
#249714=CARTESIAN_POINT('Ctrl Pts',(-9.91733516600006,15.2,4.90216720499999));
#249715=CARTESIAN_POINT('Ctrl Pts',(-9.91733516600006,11.6,4.90216720499998));
#249716=CARTESIAN_POINT('Ctrl Pts',(-9.91517633100005,15.2,4.89983954299999));
#249717=CARTESIAN_POINT('Ctrl Pts',(-9.91517633100005,11.6,4.89983954299999));
#249718=CARTESIAN_POINT('Ctrl Pts',(-9.91301913400006,15.2,4.89751740499998));
#249719=CARTESIAN_POINT('Ctrl Pts',(-9.91301913400006,11.6,4.89751740499998));
#249720=CARTESIAN_POINT('Ctrl Pts',(-9.91086358700005,15.2,4.89520079499999));
#249721=CARTESIAN_POINT('Ctrl Pts',(-9.91086358700005,11.6,4.89520079499999));
#249722=CARTESIAN_POINT('Ctrl Pts',(-9.90870970100006,15.2,4.89288971199999));
#249723=CARTESIAN_POINT('Ctrl Pts',(-9.90870970100006,11.6,4.89288971199999));
#249724=CARTESIAN_POINT('Ctrl Pts',(-9.90655748600006,15.2,4.89058415999998));
#249725=CARTESIAN_POINT('Ctrl Pts',(-9.90655748600006,11.6,4.89058415999998));
#249726=CARTESIAN_POINT('Ctrl Pts',(-9.90440695600006,15.2,4.88828413899999));
#249727=CARTESIAN_POINT('Ctrl Pts',(-9.90440695600006,11.6,4.88828413899998));
#249728=CARTESIAN_POINT('Ctrl Pts',(-9.90225812000006,15.2,4.88598965199999));
#249729=CARTESIAN_POINT('Ctrl Pts',(-9.90225812000006,11.6,4.88598965199999));
#249730=CARTESIAN_POINT('Ctrl Pts',(-9.90011099000006,15.2,4.88370070099998));
#249731=CARTESIAN_POINT('Ctrl Pts',(-9.90011099000006,11.6,4.88370070099998));
#249732=CARTESIAN_POINT('Ctrl Pts',(-9.89796557800006,15.2,4.88141728499999));
#249733=CARTESIAN_POINT('Ctrl Pts',(-9.89796557800006,11.6,4.88141728499999));
#249734=CARTESIAN_POINT('Ctrl Pts',(-9.89582189500006,15.2,4.87913940899999));
#249735=CARTESIAN_POINT('Ctrl Pts',(-9.89582189500006,11.6,4.87913940899999));
#249736=CARTESIAN_POINT('Ctrl Pts',(-9.89367995200006,15.2,4.87686707399998));
#249737=CARTESIAN_POINT('Ctrl Pts',(-9.89367995200006,11.6,4.87686707399998));
#249738=CARTESIAN_POINT('Ctrl Pts',(-9.89153976200006,15.2,4.87460027999998));
#249739=CARTESIAN_POINT('Ctrl Pts',(-9.89153976200006,11.6,4.87460027999998));
#249740=CARTESIAN_POINT('Ctrl Pts',(-9.88940133500006,15.2,4.87233902899998));
#249741=CARTESIAN_POINT('Ctrl Pts',(-9.88940133500006,11.6,4.87233902899998));
#249742=CARTESIAN_POINT('Ctrl Pts',(-9.88726468300005,15.2,4.87008332399999));
#249743=CARTESIAN_POINT('Ctrl Pts',(-9.88726468300005,11.6,4.87008332399998));
#249744=CARTESIAN_POINT('Ctrl Pts',(-9.88512981800006,15.2,4.86783316599999));
#249745=CARTESIAN_POINT('Ctrl Pts',(-9.88512981800006,11.6,4.86783316599999));
#249746=CARTESIAN_POINT('Ctrl Pts',(-9.88299675000006,15.2,4.86558855699998));
#249747=CARTESIAN_POINT('Ctrl Pts',(-9.88299675000006,11.6,4.86558855699998));
#249748=CARTESIAN_POINT('Ctrl Pts',(-9.88086549300006,15.2,4.86334949699998));
#249749=CARTESIAN_POINT('Ctrl Pts',(-9.88086549300006,11.6,4.86334949699998));
#249750=CARTESIAN_POINT('Ctrl Pts',(-9.87873605800005,15.2,4.86111598899999));
#249751=CARTESIAN_POINT('Ctrl Pts',(-9.87873605800005,11.6,4.86111598899999));
#249752=CARTESIAN_POINT('Ctrl Pts',(-9.87660845500006,15.2,4.85888803499999));
#249753=CARTESIAN_POINT('Ctrl Pts',(-9.87660845500006,11.6,4.85888803499999));
#249754=CARTESIAN_POINT('Ctrl Pts',(-9.87448269700005,15.2,4.85666563499999));
#249755=CARTESIAN_POINT('Ctrl Pts',(-9.87448269700005,11.6,4.85666563499999));
#249756=CARTESIAN_POINT('Ctrl Pts',(-9.87235879600006,15.2,4.85444879299998));
#249757=CARTESIAN_POINT('Ctrl Pts',(-9.87235879600006,11.6,4.85444879299998));
#249758=CARTESIAN_POINT('Ctrl Pts',(-9.87023676300005,15.2,4.85223750899999));
#249759=CARTESIAN_POINT('Ctrl Pts',(-9.87023676300005,11.6,4.85223750899998));
#249760=CARTESIAN_POINT('Ctrl Pts',(-9.86811661000005,15.2,4.85003178499999));
#249761=CARTESIAN_POINT('Ctrl Pts',(-9.86811661000005,11.6,4.85003178499999));
#249762=CARTESIAN_POINT('Ctrl Pts',(-9.86599834900005,15.2,4.84783162199999));
#249763=CARTESIAN_POINT('Ctrl Pts',(-9.86599834900005,11.6,4.84783162199999));
#249764=CARTESIAN_POINT('Ctrl Pts',(-9.86388199200006,15.2,4.84563702199999));
#249765=CARTESIAN_POINT('Ctrl Pts',(-9.86388199200006,11.6,4.84563702199999));
#249766=CARTESIAN_POINT('Ctrl Pts',(-9.86176755000006,15.2,4.84344798699999));
#249767=CARTESIAN_POINT('Ctrl Pts',(-9.86176755000006,11.6,4.84344798699999));
#249768=CARTESIAN_POINT('Ctrl Pts',(-9.85965503600006,15.2,4.84126451799998));
#249769=CARTESIAN_POINT('Ctrl Pts',(-9.85965503600006,11.6,4.84126451799998));
#249770=CARTESIAN_POINT('Ctrl Pts',(-9.85754446100006,15.2,4.83908661799998));
#249771=CARTESIAN_POINT('Ctrl Pts',(-9.85754446100006,11.6,4.83908661799998));
#249772=CARTESIAN_POINT('Ctrl Pts',(-9.85543583700006,15.2,4.83691428599998));
#249773=CARTESIAN_POINT('Ctrl Pts',(-9.85543583700006,11.6,4.83691428599998));
#249774=CARTESIAN_POINT('Ctrl Pts',(-9.85332917700006,15.2,4.83474752599999));
#249775=CARTESIAN_POINT('Ctrl Pts',(-9.85332917700006,11.6,4.83474752599999));
#249776=CARTESIAN_POINT('Ctrl Pts',(-9.85122449200006,15.2,4.83258633799998));
#249777=CARTESIAN_POINT('Ctrl Pts',(-9.85122449200006,11.6,4.83258633799998));
#249778=CARTESIAN_POINT('Ctrl Pts',(-9.84912179500006,15.2,4.83043072399998));
#249779=CARTESIAN_POINT('Ctrl Pts',(-9.84912179500006,11.6,4.83043072399998));
#249780=CARTESIAN_POINT('Ctrl Pts',(-9.84702109500006,15.2,4.82828068499998));
#249781=CARTESIAN_POINT('Ctrl Pts',(-9.84702109500006,11.6,4.82828068499998));
#249782=CARTESIAN_POINT('Ctrl Pts',(-9.84492240900006,15.2,4.82613622399998));
#249783=CARTESIAN_POINT('Ctrl Pts',(-9.84492240900006,11.6,4.82613622399998));
#249784=CARTESIAN_POINT('Ctrl Pts',(-9.84282574500006,15.2,4.82399734199999));
#249785=CARTESIAN_POINT('Ctrl Pts',(-9.84282574500006,11.6,4.82399734199999));
#249786=CARTESIAN_POINT('Ctrl Pts',(-9.84073111800006,15.2,4.82186403999999));
#249787=CARTESIAN_POINT('Ctrl Pts',(-9.84073111800006,11.6,4.82186403999999));
#249788=CARTESIAN_POINT('Ctrl Pts',(-9.83863853800005,15.2,4.81973631899999));
#249789=CARTESIAN_POINT('Ctrl Pts',(-9.83863853800005,11.6,4.81973631899999));
#249790=CARTESIAN_POINT('Ctrl Pts',(-9.83654801900006,15.2,4.81761418299998));
#249791=CARTESIAN_POINT('Ctrl Pts',(-9.83654801900006,11.6,4.81761418299998));
#249792=CARTESIAN_POINT('Ctrl Pts',(-9.83445957100006,15.2,4.81549763099999));
#249793=CARTESIAN_POINT('Ctrl Pts',(-9.83445957100006,11.6,4.81549763099998));
#249794=CARTESIAN_POINT('Ctrl Pts',(-9.83237320800006,15.2,4.81338666499998));
#249795=CARTESIAN_POINT('Ctrl Pts',(-9.83237320800006,11.6,4.81338666499998));
#249796=CARTESIAN_POINT('Ctrl Pts',(-9.83028894200006,15.2,4.81128128699999));
#249797=CARTESIAN_POINT('Ctrl Pts',(-9.83028894200006,11.6,4.81128128699999));
#249798=CARTESIAN_POINT('Ctrl Pts',(-9.82820678500006,15.2,4.80918149899999));
#249799=CARTESIAN_POINT('Ctrl Pts',(-9.82820678500006,11.6,4.80918149899999));
#249800=CARTESIAN_POINT('Ctrl Pts',(-9.82612674900006,15.2,4.80708729999999));
#249801=CARTESIAN_POINT('Ctrl Pts',(-9.82612674900006,11.6,4.80708729999998));
#249802=CARTESIAN_POINT('Ctrl Pts',(-9.82404884900006,15.2,4.80499869499998));
#249803=CARTESIAN_POINT('Ctrl Pts',(-9.82404884900006,11.6,4.80499869499998));
#249804=CARTESIAN_POINT('Ctrl Pts',(-9.82197309300006,15.2,4.80291568299998));
#249805=CARTESIAN_POINT('Ctrl Pts',(-9.82197309300006,11.6,4.80291568299998));
#249806=CARTESIAN_POINT('Ctrl Pts',(-9.81989949700005,15.2,4.80083826599999));
#249807=CARTESIAN_POINT('Ctrl Pts',(-9.81989949700005,11.6,4.80083826599999));
#249808=CARTESIAN_POINT('Ctrl Pts',(-9.81782807000006,15.2,4.79876644699999));
#249809=CARTESIAN_POINT('Ctrl Pts',(-9.81782807000006,11.6,4.79876644699999));
#249810=CARTESIAN_POINT('Ctrl Pts',(-9.81575883000006,15.2,4.79670022499998));
#249811=CARTESIAN_POINT('Ctrl Pts',(-9.81575883000006,11.6,4.79670022499998));
#249812=CARTESIAN_POINT('Ctrl Pts',(-9.81369178300006,15.2,4.79463960299999));
#249813=CARTESIAN_POINT('Ctrl Pts',(-9.81369178300006,11.6,4.79463960299999));
#249814=CARTESIAN_POINT('Ctrl Pts',(-9.81162694700006,15.2,4.79258458199999));
#249815=CARTESIAN_POINT('Ctrl Pts',(-9.81162694700006,11.6,4.79258458199998));
#249816=CARTESIAN_POINT('Ctrl Pts',(-9.80956433100006,15.2,4.79053516399999));
#249817=CARTESIAN_POINT('Ctrl Pts',(-9.80956433100006,11.6,4.79053516399999));
#249818=CARTESIAN_POINT('Ctrl Pts',(-9.80750395000006,15.2,4.78849134999999));
#249819=CARTESIAN_POINT('Ctrl Pts',(-9.80750395000006,11.6,4.78849134999999));
#249820=CARTESIAN_POINT('Ctrl Pts',(-9.80544581400006,15.2,4.78645313999999));
#249821=CARTESIAN_POINT('Ctrl Pts',(-9.80544581400006,11.6,4.78645313999999));
#249822=CARTESIAN_POINT('Ctrl Pts',(-9.80338993900006,15.2,4.78442053799998));
#249823=CARTESIAN_POINT('Ctrl Pts',(-9.80338993900006,11.6,4.78442053799998));
#249824=CARTESIAN_POINT('Ctrl Pts',(-9.80133633400006,15.2,4.78239354399999));
#249825=CARTESIAN_POINT('Ctrl Pts',(-9.80133633400006,11.6,4.78239354399999));
#249826=CARTESIAN_POINT('Ctrl Pts',(-9.79928501600006,15.2,4.78037215999999));
#249827=CARTESIAN_POINT('Ctrl Pts',(-9.79928501600006,11.6,4.78037215999999));
#249828=CARTESIAN_POINT('Ctrl Pts',(-9.79723599400005,15.2,4.77835638599998));
#249829=CARTESIAN_POINT('Ctrl Pts',(-9.79723599400005,11.6,4.77835638599998));
#249830=CARTESIAN_POINT('Ctrl Pts',(-9.79518928200006,15.2,4.77634622499998));
#249831=CARTESIAN_POINT('Ctrl Pts',(-9.79518928200006,11.6,4.77634622499998));
#249832=CARTESIAN_POINT('Ctrl Pts',(-9.79314489400006,15.2,4.77434167799998));
#249833=CARTESIAN_POINT('Ctrl Pts',(-9.79314489400006,11.6,4.77434167799998));
#249834=CARTESIAN_POINT('Ctrl Pts',(-9.79110284100006,15.2,4.77234274599999));
#249835=CARTESIAN_POINT('Ctrl Pts',(-9.79110284100006,11.6,4.77234274599999));
#249836=CARTESIAN_POINT('Ctrl Pts',(-9.78906313700006,15.2,4.77034943099999));
#249837=CARTESIAN_POINT('Ctrl Pts',(-9.78906313700006,11.6,4.77034943099999));
#249838=CARTESIAN_POINT('Ctrl Pts',(-9.78702579600006,15.2,4.76836173399998));
#249839=CARTESIAN_POINT('Ctrl Pts',(-9.78702579600006,11.6,4.76836173399998));
#249840=CARTESIAN_POINT('Ctrl Pts',(-9.78499082900005,15.2,4.76637965599998));
#249841=CARTESIAN_POINT('Ctrl Pts',(-9.78499082900005,11.6,4.76637965599998));
#249842=CARTESIAN_POINT('Ctrl Pts',(-9.78295824900006,15.2,4.76440319899999));
#249843=CARTESIAN_POINT('Ctrl Pts',(-9.78295824900006,11.6,4.76440319899999));
#249844=CARTESIAN_POINT('Ctrl Pts',(-9.78092807100006,15.2,4.76243236299998));
#249845=CARTESIAN_POINT('Ctrl Pts',(-9.78092807100006,11.6,4.76243236299998));
#249846=CARTESIAN_POINT('Ctrl Pts',(-9.77890030600006,15.2,4.76046715199999));
#249847=CARTESIAN_POINT('Ctrl Pts',(-9.77890030600006,11.6,4.76046715199998));
#249848=CARTESIAN_POINT('Ctrl Pts',(-9.77687496800005,15.2,4.75850756499998));
#249849=CARTESIAN_POINT('Ctrl Pts',(-9.77687496800005,11.6,4.75850756499998));
#249850=CARTESIAN_POINT('Ctrl Pts',(-9.77485207000005,15.2,4.75655360399998));
#249851=CARTESIAN_POINT('Ctrl Pts',(-9.77485207000005,11.6,4.75655360399998));
#249852=CARTESIAN_POINT('Ctrl Pts',(-9.77283162500006,15.2,4.75460526999999));
#249853=CARTESIAN_POINT('Ctrl Pts',(-9.77283162500006,11.6,4.75460526999999));
#249854=CARTESIAN_POINT('Ctrl Pts',(-9.77081364700006,15.2,4.75266256599999));
#249855=CARTESIAN_POINT('Ctrl Pts',(-9.77081364700006,11.6,4.75266256599998));
#249856=CARTESIAN_POINT('Ctrl Pts',(-9.76879814800006,15.2,4.75072549099998));
#249857=CARTESIAN_POINT('Ctrl Pts',(-9.76879814800006,11.6,4.75072549099998));
#249858=CARTESIAN_POINT('Ctrl Pts',(-9.76678514200006,15.2,4.74879404799999));
#249859=CARTESIAN_POINT('Ctrl Pts',(-9.76678514200006,11.6,4.74879404799999));
#249860=CARTESIAN_POINT('Ctrl Pts',(-9.76477464200006,15.2,4.74686823699999));
#249861=CARTESIAN_POINT('Ctrl Pts',(-9.76477464200006,11.6,4.74686823699999));
#249862=CARTESIAN_POINT('Ctrl Pts',(-9.76276666200006,15.2,4.74494805999999));
#249863=CARTESIAN_POINT('Ctrl Pts',(-9.76276666200006,11.6,4.74494805999999));
#249864=CARTESIAN_POINT('Ctrl Pts',(-9.76076121400006,15.2,4.74303351799998));
#249865=CARTESIAN_POINT('Ctrl Pts',(-9.76076121400006,11.6,4.74303351799998));
#249866=CARTESIAN_POINT('Ctrl Pts',(-9.75875831300005,15.2,4.74112461299999));
#249867=CARTESIAN_POINT('Ctrl Pts',(-9.75875831300005,11.6,4.74112461299998));
#249868=CARTESIAN_POINT('Ctrl Pts',(-9.75675797100006,15.2,4.73922134599999));
#249869=CARTESIAN_POINT('Ctrl Pts',(-9.75675797100006,11.6,4.73922134599999));
#249870=CARTESIAN_POINT('Ctrl Pts',(-9.75476020300006,15.2,4.73732371799999));
#249871=CARTESIAN_POINT('Ctrl Pts',(-9.75476020300006,11.6,4.73732371799999));
#249872=CARTESIAN_POINT('Ctrl Pts',(-9.75276502000006,15.2,4.73543172899999));
#249873=CARTESIAN_POINT('Ctrl Pts',(-9.75276502000006,11.6,4.73543172899998));
#249874=CARTESIAN_POINT('Ctrl Pts',(-9.75077243800006,15.2,4.73354538299999));
#249875=CARTESIAN_POINT('Ctrl Pts',(-9.75077243800006,11.6,4.73354538299999));
#249876=CARTESIAN_POINT('Ctrl Pts',(-9.74878247000006,15.2,4.73166467999998));
#249877=CARTESIAN_POINT('Ctrl Pts',(-9.74878247000006,11.6,4.73166467999998));
#249878=CARTESIAN_POINT('Ctrl Pts',(-9.74679512900006,15.2,4.72978961999999));
#249879=CARTESIAN_POINT('Ctrl Pts',(-9.74679512900006,11.6,4.72978961999999));
#249880=CARTESIAN_POINT('Ctrl Pts',(-9.74481042800006,15.2,4.72792020599999));
#249881=CARTESIAN_POINT('Ctrl Pts',(-9.74481042800006,11.6,4.72792020599999));
#249882=CARTESIAN_POINT('Ctrl Pts',(-9.74282838300006,15.2,4.72605643799999));
#249883=CARTESIAN_POINT('Ctrl Pts',(-9.74282838300006,11.6,4.72605643799999));
#249884=CARTESIAN_POINT('Ctrl Pts',(-9.74084900600005,15.2,4.72419831799999));
#249885=CARTESIAN_POINT('Ctrl Pts',(-9.74084900600005,11.6,4.72419831799998));
#249886=CARTESIAN_POINT('Ctrl Pts',(-9.73887231000005,15.2,4.72234584699999));
#249887=CARTESIAN_POINT('Ctrl Pts',(-9.73887231000005,11.6,4.72234584699999));
#249888=CARTESIAN_POINT('Ctrl Pts',(-9.73689831000006,15.2,4.72049902699998));
#249889=CARTESIAN_POINT('Ctrl Pts',(-9.73689831000006,11.6,4.72049902699998));
#249890=CARTESIAN_POINT('Ctrl Pts',(-9.73492702000006,15.2,4.71865785699999));
#249891=CARTESIAN_POINT('Ctrl Pts',(-9.73492702000006,11.6,4.71865785699999));
#249892=CARTESIAN_POINT('Ctrl Pts',(-9.73295845400006,15.2,4.71682233999999));
#249893=CARTESIAN_POINT('Ctrl Pts',(-9.73295845400006,11.6,4.71682233999999));
#249894=CARTESIAN_POINT('Ctrl Pts',(-9.73099262500006,15.2,4.71499247599999));
#249895=CARTESIAN_POINT('Ctrl Pts',(-9.73099262500006,11.6,4.71499247599999));
#249896=CARTESIAN_POINT('Ctrl Pts',(-9.72902954700006,15.2,4.71316826799999));
#249897=CARTESIAN_POINT('Ctrl Pts',(-9.72902954700006,11.6,4.71316826799998));
#249898=CARTESIAN_POINT('Ctrl Pts',(-9.72706923400006,15.2,4.71134971599999));
#249899=CARTESIAN_POINT('Ctrl Pts',(-9.72706923400006,11.6,4.71134971599999));
#249900=CARTESIAN_POINT('Ctrl Pts',(-9.72511170000006,15.2,4.70953682099999));
#249901=CARTESIAN_POINT('Ctrl Pts',(-9.72511170000006,11.6,4.70953682099999));
#249902=CARTESIAN_POINT('Ctrl Pts',(-9.72315695900006,15.2,4.70772958399999));
#249903=CARTESIAN_POINT('Ctrl Pts',(-9.72315695900006,11.6,4.70772958399999));
#249904=CARTESIAN_POINT('Ctrl Pts',(-9.72120502600006,15.2,4.70592800699999));
#249905=CARTESIAN_POINT('Ctrl Pts',(-9.72120502600006,11.6,4.70592800699999));
#249906=CARTESIAN_POINT('Ctrl Pts',(-9.71925591500005,15.2,4.70413208999998));
#249907=CARTESIAN_POINT('Ctrl Pts',(-9.71925591500005,11.6,4.70413208999998));
#249908=CARTESIAN_POINT('Ctrl Pts',(-9.71730963800006,15.2,4.70234183599998));
#249909=CARTESIAN_POINT('Ctrl Pts',(-9.71730963800006,11.6,4.70234183599998));
#249910=CARTESIAN_POINT('Ctrl Pts',(-9.71536621200006,15.2,4.70055724399998));
#249911=CARTESIAN_POINT('Ctrl Pts',(-9.71536621200006,11.6,4.70055724399998));
#249912=CARTESIAN_POINT('Ctrl Pts',(-9.71342564900005,15.2,4.69877831599998));
#249913=CARTESIAN_POINT('Ctrl Pts',(-9.71342564900005,11.6,4.69877831599998));
#249914=CARTESIAN_POINT('Ctrl Pts',(-9.71148796400006,15.2,4.69700505399998));
#249915=CARTESIAN_POINT('Ctrl Pts',(-9.71148796400006,11.6,4.69700505399998));
#249916=CARTESIAN_POINT('Ctrl Pts',(-9.70955317200006,15.2,4.69523745799999));
#249917=CARTESIAN_POINT('Ctrl Pts',(-9.70955317200006,11.6,4.69523745799999));
#249918=CARTESIAN_POINT('Ctrl Pts',(-9.70762128700006,15.2,4.69347552899999));
#249919=CARTESIAN_POINT('Ctrl Pts',(-9.70762128700006,11.6,4.69347552899999));
#249920=CARTESIAN_POINT('Ctrl Pts',(-9.70569232300006,15.2,4.69171926799999));
#249921=CARTESIAN_POINT('Ctrl Pts',(-9.70569232300006,11.6,4.69171926799999));
#249922=CARTESIAN_POINT('Ctrl Pts',(-9.70376629500005,15.2,4.68996867699998));
#249923=CARTESIAN_POINT('Ctrl Pts',(-9.70376629500005,11.6,4.68996867699998));
#249924=CARTESIAN_POINT('Ctrl Pts',(-9.70184321600006,15.2,4.68822375699999));
#249925=CARTESIAN_POINT('Ctrl Pts',(-9.70184321600006,11.6,4.68822375699998));
#249926=CARTESIAN_POINT('Ctrl Pts',(-9.69992310200006,15.2,4.68648450799999));
#249927=CARTESIAN_POINT('Ctrl Pts',(-9.69992310200006,11.6,4.68648450799999));
#249928=CARTESIAN_POINT('Ctrl Pts',(-9.69800596700006,15.2,4.68475093299999));
#249929=CARTESIAN_POINT('Ctrl Pts',(-9.69800596700006,11.6,4.68475093299999));
#249930=CARTESIAN_POINT('Ctrl Pts',(-9.69609182600006,15.2,4.68302302999999));
#249931=CARTESIAN_POINT('Ctrl Pts',(-9.69609182600006,11.6,4.68302302999999));
#249932=CARTESIAN_POINT('Ctrl Pts',(-9.69418069300006,15.2,4.68130080299999));
#249933=CARTESIAN_POINT('Ctrl Pts',(-9.69418069300006,11.6,4.68130080299998));
#249934=CARTESIAN_POINT('Ctrl Pts',(-9.69227258300006,15.2,4.67958425199999));
#249935=CARTESIAN_POINT('Ctrl Pts',(-9.69227258300006,11.6,4.67958425199999));
#249936=CARTESIAN_POINT('Ctrl Pts',(-9.69036751000005,15.2,4.67787337699999));
#249937=CARTESIAN_POINT('Ctrl Pts',(-9.69036751000005,11.6,4.67787337699998));
#249938=CARTESIAN_POINT('Ctrl Pts',(-9.68846549000006,15.2,4.67616818099999));
#249939=CARTESIAN_POINT('Ctrl Pts',(-9.68846549000006,11.6,4.67616818099999));
#249940=CARTESIAN_POINT('Ctrl Pts',(-9.68656653600006,15.2,4.67446866399998));
#249941=CARTESIAN_POINT('Ctrl Pts',(-9.68656653600006,11.6,4.67446866399998));
#249942=CARTESIAN_POINT('Ctrl Pts',(-9.68467066400006,15.2,4.67277482499998));
#249943=CARTESIAN_POINT('Ctrl Pts',(-9.68467066400006,11.6,4.67277482499998));
#249944=CARTESIAN_POINT('Ctrl Pts',(-9.68277788900006,15.2,4.67108666899998));
#249945=CARTESIAN_POINT('Ctrl Pts',(-9.68277788900006,11.6,4.67108666899998));
#249946=CARTESIAN_POINT('Ctrl Pts',(-9.68088822600006,15.2,4.66940419399998));
#249947=CARTESIAN_POINT('Ctrl Pts',(-9.68088822600006,11.6,4.66940419399998));
#249948=CARTESIAN_POINT('Ctrl Pts',(-9.67900168900006,15.2,4.66772740199998));
#249949=CARTESIAN_POINT('Ctrl Pts',(-9.67900168900006,11.6,4.66772740199998));
#249950=CARTESIAN_POINT('Ctrl Pts',(-9.67711829400006,15.2,4.66605629399999));
#249951=CARTESIAN_POINT('Ctrl Pts',(-9.67711829400006,11.6,4.66605629399999));
#249952=CARTESIAN_POINT('Ctrl Pts',(-9.67523805500005,15.2,4.66439086999999));
#249953=CARTESIAN_POINT('Ctrl Pts',(-9.67523805500005,11.6,4.66439086999998));
#249954=CARTESIAN_POINT('Ctrl Pts',(-9.67336098800006,15.2,4.66273113399998));
#249955=CARTESIAN_POINT('Ctrl Pts',(-9.67336098800006,11.6,4.66273113399998));
#249956=CARTESIAN_POINT('Ctrl Pts',(-9.67148710700006,15.2,4.66107708199999));
#249957=CARTESIAN_POINT('Ctrl Pts',(-9.67148710700006,11.6,4.66107708199999));
#249958=CARTESIAN_POINT('Ctrl Pts',(-9.66961642800005,15.2,4.65942871899999));
#249959=CARTESIAN_POINT('Ctrl Pts',(-9.66961642800005,11.6,4.65942871899998));
#249960=CARTESIAN_POINT('Ctrl Pts',(-9.66774896600005,15.2,4.65778604499998));
#249961=CARTESIAN_POINT('Ctrl Pts',(-9.66774896600005,11.6,4.65778604499998));
#249962=CARTESIAN_POINT('Ctrl Pts',(-9.66588473600006,15.2,4.65614906099999));
#249963=CARTESIAN_POINT('Ctrl Pts',(-9.66588473600006,11.6,4.65614906099999));
#249964=CARTESIAN_POINT('Ctrl Pts',(-9.66402375400006,15.2,4.65451776599998));
#249965=CARTESIAN_POINT('Ctrl Pts',(-9.66402375400006,11.6,4.65451776599998));
#249966=CARTESIAN_POINT('Ctrl Pts',(-9.66216603400006,15.2,4.65289216299999));
#249967=CARTESIAN_POINT('Ctrl Pts',(-9.66216603400006,11.6,4.65289216299999));
#249968=CARTESIAN_POINT('Ctrl Pts',(-9.66031159300006,15.2,4.65127225199998));
#249969=CARTESIAN_POINT('Ctrl Pts',(-9.66031159300006,11.6,4.65127225199998));
#249970=CARTESIAN_POINT('Ctrl Pts',(-9.65846044500006,15.2,4.64965803399998));
#249971=CARTESIAN_POINT('Ctrl Pts',(-9.65846044500006,11.6,4.64965803399998));
#249972=CARTESIAN_POINT('Ctrl Pts',(-9.65661260600006,15.2,4.64804950999999));
#249973=CARTESIAN_POINT('Ctrl Pts',(-9.65661260600006,11.6,4.64804950999999));
#249974=CARTESIAN_POINT('Ctrl Pts',(-9.65476809200006,15.2,4.64644668199998));
#249975=CARTESIAN_POINT('Ctrl Pts',(-9.65476809200006,11.6,4.64644668199998));
#249976=CARTESIAN_POINT('Ctrl Pts',(-9.65292691700006,15.2,4.64484954899999));
#249977=CARTESIAN_POINT('Ctrl Pts',(-9.65292691700006,11.6,4.64484954899999));
#249978=CARTESIAN_POINT('Ctrl Pts',(-9.65108909700006,15.2,4.64325811299998));
#249979=CARTESIAN_POINT('Ctrl Pts',(-9.65108909700006,11.6,4.64325811299998));
#249980=CARTESIAN_POINT('Ctrl Pts',(-9.64925465000006,15.2,4.64167237399998));
#249981=CARTESIAN_POINT('Ctrl Pts',(-9.64925465000006,11.6,4.64167237399998));
#249982=CARTESIAN_POINT('Ctrl Pts',(-9.64742358900006,15.2,4.64009233399998));
#249983=CARTESIAN_POINT('Ctrl Pts',(-9.64742358900006,11.6,4.64009233399998));
#249984=CARTESIAN_POINT('Ctrl Pts',(-9.64559593000006,15.2,4.63851799299999));
#249985=CARTESIAN_POINT('Ctrl Pts',(-9.64559593000006,11.6,4.63851799299999));
#249986=CARTESIAN_POINT('Ctrl Pts',(-9.64377169000005,15.2,4.63694935199998));
#249987=CARTESIAN_POINT('Ctrl Pts',(-9.64377169000005,11.6,4.63694935199998));
#249988=CARTESIAN_POINT('Ctrl Pts',(-9.64195088400006,15.2,4.63538641099999));
#249989=CARTESIAN_POINT('Ctrl Pts',(-9.64195088400006,11.6,4.63538641099999));
#249990=CARTESIAN_POINT('Ctrl Pts',(-9.64013352800006,15.2,4.63382917199999));
#249991=CARTESIAN_POINT('Ctrl Pts',(-9.64013352800006,11.6,4.63382917199999));
#249992=CARTESIAN_POINT('Ctrl Pts',(-9.63831963700006,15.2,4.63227763599999));
#249993=CARTESIAN_POINT('Ctrl Pts',(-9.63831963700006,11.6,4.63227763599999));
#249994=CARTESIAN_POINT('Ctrl Pts',(-9.63650922900005,15.2,4.63073180299999));
#249995=CARTESIAN_POINT('Ctrl Pts',(-9.63650922900005,11.6,4.63073180299998));
#249996=CARTESIAN_POINT('Ctrl Pts',(-9.63470231800006,15.2,4.62919167299999));
#249997=CARTESIAN_POINT('Ctrl Pts',(-9.63470231800006,11.6,4.62919167299999));
#249998=CARTESIAN_POINT('Ctrl Pts',(-9.63289892100006,15.2,4.62765724899998));
#249999=CARTESIAN_POINT('Ctrl Pts',(-9.63289892100006,11.6,4.62765724899998));
#250000=CARTESIAN_POINT('Ctrl Pts',(-9.63109905400006,15.2,4.62612852999998));
#250001=CARTESIAN_POINT('Ctrl Pts',(-9.63109905400006,11.6,4.62612852999998));
#250002=CARTESIAN_POINT('Ctrl Pts',(-9.62930273200006,15.2,4.62460551699999));
#250003=CARTESIAN_POINT('Ctrl Pts',(-9.62930273200006,11.6,4.62460551699999));
#250004=CARTESIAN_POINT('Ctrl Pts',(-9.62750997400006,15.2,4.62308821099998));
#250005=CARTESIAN_POINT('Ctrl Pts',(-9.62750997400006,11.6,4.62308821099998));
#250006=CARTESIAN_POINT('Ctrl Pts',(-9.62572079300006,15.2,4.62157661399999));
#250007=CARTESIAN_POINT('Ctrl Pts',(-9.62572079300006,11.6,4.62157661399999));
#250008=CARTESIAN_POINT('Ctrl Pts',(-9.62393520600006,15.2,4.62007072399999));
#250009=CARTESIAN_POINT('Ctrl Pts',(-9.62393520600006,11.6,4.62007072399999));
#250010=CARTESIAN_POINT('Ctrl Pts',(-9.62215323100006,15.2,4.61857054399999));
#250011=CARTESIAN_POINT('Ctrl Pts',(-9.62215323100006,11.6,4.61857054399999));
#250012=CARTESIAN_POINT('Ctrl Pts',(-9.62037488400006,15.2,4.61707607299999));
#250013=CARTESIAN_POINT('Ctrl Pts',(-9.62037488400006,11.6,4.61707607299999));
#250014=CARTESIAN_POINT('Ctrl Pts',(-9.61860017900005,15.2,4.61558731399998));
#250015=CARTESIAN_POINT('Ctrl Pts',(-9.61860017900005,11.6,4.61558731399998));
#250016=CARTESIAN_POINT('Ctrl Pts',(-9.61682913600006,15.2,4.61410426599999));
#250017=CARTESIAN_POINT('Ctrl Pts',(-9.61682913600006,11.6,4.61410426599999));
#250018=CARTESIAN_POINT('Ctrl Pts',(-9.61506176900006,15.2,4.61262692999998));
#250019=CARTESIAN_POINT('Ctrl Pts',(-9.61506176900006,11.6,4.61262692999998));
#250020=CARTESIAN_POINT('Ctrl Pts',(-9.61329809500005,15.2,4.61115530599999));
#250021=CARTESIAN_POINT('Ctrl Pts',(-9.61329809500005,11.6,4.61115530599999));
#250022=CARTESIAN_POINT('Ctrl Pts',(-9.61153813200006,15.2,4.60968939499999));
#250023=CARTESIAN_POINT('Ctrl Pts',(-9.61153813200006,11.6,4.60968939499998));
#250024=CARTESIAN_POINT('Ctrl Pts',(-9.60978189400005,15.2,4.60822919899999));
#250025=CARTESIAN_POINT('Ctrl Pts',(-9.60978189400005,11.6,4.60822919899999));
#250026=CARTESIAN_POINT('Ctrl Pts',(-9.60802940000006,15.2,4.60677471699999));
#250027=CARTESIAN_POINT('Ctrl Pts',(-9.60802940000006,11.6,4.60677471699999));
#250028=CARTESIAN_POINT('Ctrl Pts',(-9.60628066600006,15.2,4.60532595099998));
#250029=CARTESIAN_POINT('Ctrl Pts',(-9.60628066600006,11.6,4.60532595099998));
#250030=CARTESIAN_POINT('Ctrl Pts',(-9.60453570800006,15.2,4.60388289999998));
#250031=CARTESIAN_POINT('Ctrl Pts',(-9.60453570800006,11.6,4.60388289999998));
#250032=CARTESIAN_POINT('Ctrl Pts',(-9.60279454500006,15.2,4.60244556599999));
#250033=CARTESIAN_POINT('Ctrl Pts',(-9.60279454500006,11.6,4.60244556599999));
#250034=CARTESIAN_POINT('Ctrl Pts',(-9.60105719300006,15.2,4.60101394899999));
#250035=CARTESIAN_POINT('Ctrl Pts',(-9.60105719300006,11.6,4.60101394899999));
#250036=CARTESIAN_POINT('Ctrl Pts',(-9.59932366800006,15.2,4.59958804999999));
#250037=CARTESIAN_POINT('Ctrl Pts',(-9.59932366800006,11.6,4.59958804999999));
#250038=CARTESIAN_POINT('Ctrl Pts',(-9.59759398800006,15.2,4.59816786899999));
#250039=CARTESIAN_POINT('Ctrl Pts',(-9.59759398800006,11.6,4.59816786899999));
#250040=CARTESIAN_POINT('Ctrl Pts',(-9.59586816900006,15.2,4.59675340699999));
#250041=CARTESIAN_POINT('Ctrl Pts',(-9.59586816900006,11.6,4.59675340699999));
#250042=CARTESIAN_POINT('Ctrl Pts',(-9.59414622900006,15.2,4.59534466299999));
#250043=CARTESIAN_POINT('Ctrl Pts',(-9.59414622900006,11.6,4.59534466299999));
#250044=CARTESIAN_POINT('Ctrl Pts',(-9.59242818600006,15.2,4.59394164099999));
#250045=CARTESIAN_POINT('Ctrl Pts',(-9.59242818600006,11.6,4.59394164099999));
#250046=CARTESIAN_POINT('Ctrl Pts',(-9.59071405500006,15.2,4.59254433899999));
#250047=CARTESIAN_POINT('Ctrl Pts',(-9.59071405500006,11.6,4.59254433899999));
#250048=CARTESIAN_POINT('Ctrl Pts',(-9.58900385500005,15.2,4.59115275799999));
#250049=CARTESIAN_POINT('Ctrl Pts',(-9.58900385500005,11.6,4.59115275799998));
#250050=CARTESIAN_POINT('Ctrl Pts',(-9.58729760300006,15.2,4.58976689899998));
#250051=CARTESIAN_POINT('Ctrl Pts',(-9.58729760300006,11.6,4.58976689899998));
#250052=CARTESIAN_POINT('Ctrl Pts',(-9.58559531500006,15.2,4.58838676099998));
#250053=CARTESIAN_POINT('Ctrl Pts',(-9.58559531500006,11.6,4.58838676099998));
#250054=CARTESIAN_POINT('Ctrl Pts',(-9.58389701200005,15.2,4.58701234699999));
#250055=CARTESIAN_POINT('Ctrl Pts',(-9.58389701200005,11.6,4.58701234699998));
#250056=CARTESIAN_POINT('Ctrl Pts',(-9.58220270800006,15.2,4.58564365599998));
#250057=CARTESIAN_POINT('Ctrl Pts',(-9.58220270800006,11.6,4.58564365599998));
#250058=CARTESIAN_POINT('Ctrl Pts',(-9.58051242300006,15.2,4.58428068699998));
#250059=CARTESIAN_POINT('Ctrl Pts',(-9.58051242300006,11.6,4.58428068699998));
#250060=CARTESIAN_POINT('Ctrl Pts',(-9.57882617200006,15.2,4.58292344399998));
#250061=CARTESIAN_POINT('Ctrl Pts',(-9.57882617200006,11.6,4.58292344399998));
#250062=CARTESIAN_POINT('Ctrl Pts',(-9.57714397400006,15.2,4.58157192499999));
#250063=CARTESIAN_POINT('Ctrl Pts',(-9.57714397400006,11.6,4.58157192499998));
#250064=CARTESIAN_POINT('Ctrl Pts',(-9.57546584800006,15.2,4.58022613099998));
#250065=CARTESIAN_POINT('Ctrl Pts',(-9.57546584800006,11.6,4.58022613099998));
#250066=CARTESIAN_POINT('Ctrl Pts',(-9.57379181000006,15.2,4.57888606299999));
#250067=CARTESIAN_POINT('Ctrl Pts',(-9.57379181000006,11.6,4.57888606299999));
#250068=CARTESIAN_POINT('Ctrl Pts',(-9.57212187800006,15.2,4.57755171999998));
#250069=CARTESIAN_POINT('Ctrl Pts',(-9.57212187800006,11.6,4.57755171999998));
#250070=CARTESIAN_POINT('Ctrl Pts',(-9.57045607000006,15.2,4.57622310399999));
#250071=CARTESIAN_POINT('Ctrl Pts',(-9.57045607000006,11.6,4.57622310399999));
#250072=CARTESIAN_POINT('Ctrl Pts',(-9.56879440600006,15.2,4.57490021399998));
#250073=CARTESIAN_POINT('Ctrl Pts',(-9.56879440600006,11.6,4.57490021399998));
#250074=CARTESIAN_POINT('Ctrl Pts',(-9.56713690100005,15.2,4.57358305199998));
#250075=CARTESIAN_POINT('Ctrl Pts',(-9.56713690100005,11.6,4.57358305199998));
#250076=CARTESIAN_POINT('Ctrl Pts',(-9.56548357500006,15.2,4.57227161699999));
#250077=CARTESIAN_POINT('Ctrl Pts',(-9.56548357500006,11.6,4.57227161699999));
#250078=CARTESIAN_POINT('Ctrl Pts',(-9.56383444500006,15.2,4.57096591099998));
#250079=CARTESIAN_POINT('Ctrl Pts',(-9.56383444500006,11.6,4.57096591099998));
#250080=CARTESIAN_POINT('Ctrl Pts',(-9.56218953100005,15.2,4.56966593299998));
#250081=CARTESIAN_POINT('Ctrl Pts',(-9.56218953100005,11.6,4.56966593299998));
#250082=CARTESIAN_POINT('Ctrl Pts',(-9.56054884800006,15.2,4.56837168399999));
#250083=CARTESIAN_POINT('Ctrl Pts',(-9.56054884800006,11.6,4.56837168399998));
#250084=CARTESIAN_POINT('Ctrl Pts',(-9.55891241700006,15.2,4.56708316299999));
#250085=CARTESIAN_POINT('Ctrl Pts',(-9.55891241700006,11.6,4.56708316299998));
#250086=CARTESIAN_POINT('Ctrl Pts',(-9.55728025600006,15.2,4.56580037199998));
#250087=CARTESIAN_POINT('Ctrl Pts',(-9.55728025600006,11.6,4.56580037199998));
#250088=CARTESIAN_POINT('Ctrl Pts',(-9.55565238300006,15.2,4.56452331099998));
#250089=CARTESIAN_POINT('Ctrl Pts',(-9.55565238300006,11.6,4.56452331099998));
#250090=CARTESIAN_POINT('Ctrl Pts',(-9.55402881600006,15.2,4.56325197999998));
#250091=CARTESIAN_POINT('Ctrl Pts',(-9.55402881600006,11.6,4.56325197999998));
#250092=CARTESIAN_POINT('Ctrl Pts',(-9.55240957500006,15.2,4.56198637899998));
#250093=CARTESIAN_POINT('Ctrl Pts',(-9.55240957500006,11.6,4.56198637899998));
#250094=CARTESIAN_POINT('Ctrl Pts',(-9.55079467700006,15.2,4.56072650899999));
#250095=CARTESIAN_POINT('Ctrl Pts',(-9.55079467700006,11.6,4.56072650899999));
#250096=CARTESIAN_POINT('Ctrl Pts',(-9.54918414200005,15.2,4.55947236999998));
#250097=CARTESIAN_POINT('Ctrl Pts',(-9.54918414200005,11.6,4.55947236999998));
#250098=CARTESIAN_POINT('Ctrl Pts',(-9.54757798700006,15.2,4.55822396199999));
#250099=CARTESIAN_POINT('Ctrl Pts',(-9.54757798700006,11.6,4.55822396199998));
#250100=CARTESIAN_POINT('Ctrl Pts',(-9.54597623200005,15.2,4.55698128599998));
#250101=CARTESIAN_POINT('Ctrl Pts',(-9.54597623200005,11.6,4.55698128599998));
#250102=CARTESIAN_POINT('Ctrl Pts',(-9.54437889600005,15.2,4.55574434099999));
#250103=CARTESIAN_POINT('Ctrl Pts',(-9.54437889600005,11.6,4.55574434099999));
#250104=CARTESIAN_POINT('Ctrl Pts',(-9.54278599800006,15.2,4.55451312899999));
#250105=CARTESIAN_POINT('Ctrl Pts',(-9.54278599800006,11.6,4.55451312899999));
#250106=CARTESIAN_POINT('Ctrl Pts',(-9.54119755600006,15.2,4.55328764899999));
#250107=CARTESIAN_POINT('Ctrl Pts',(-9.54119755600006,11.6,4.55328764899999));
#250108=CARTESIAN_POINT('Ctrl Pts',(-9.53961359000006,15.2,4.55206790099999));
#250109=CARTESIAN_POINT('Ctrl Pts',(-9.53961359000006,11.6,4.55206790099999));
#250110=CARTESIAN_POINT('Ctrl Pts',(-9.53803411900006,15.2,4.55085388699998));
#250111=CARTESIAN_POINT('Ctrl Pts',(-9.53803411900006,11.6,4.55085388699998));
#250112=CARTESIAN_POINT('Ctrl Pts',(-9.53645916300006,15.2,4.54964560499998));
#250113=CARTESIAN_POINT('Ctrl Pts',(-9.53645916300006,11.6,4.54964560499998));
#250114=CARTESIAN_POINT('Ctrl Pts',(-9.53488873900006,15.2,4.54844305599998));
#250115=CARTESIAN_POINT('Ctrl Pts',(-9.53488873900006,11.6,4.54844305599998));
#250116=CARTESIAN_POINT('Ctrl Pts',(-9.53332286700006,15.2,4.54724623999999));
#250117=CARTESIAN_POINT('Ctrl Pts',(-9.53332286700006,11.6,4.54724623999999));
#250118=CARTESIAN_POINT('Ctrl Pts',(-9.53176156700006,15.2,4.54605515799998));
#250119=CARTESIAN_POINT('Ctrl Pts',(-9.53176156700006,11.6,4.54605515799998));
#250120=CARTESIAN_POINT('Ctrl Pts',(-9.53020485900005,15.2,4.54486980999998));
#250121=CARTESIAN_POINT('Ctrl Pts',(-9.53020485900005,11.6,4.54486980999998));
#250122=CARTESIAN_POINT('Ctrl Pts',(-9.52865276200006,15.2,4.54369019499998));
#250123=CARTESIAN_POINT('Ctrl Pts',(-9.52865276200006,11.6,4.54369019499998));
#250124=CARTESIAN_POINT('Ctrl Pts',(-9.52710529500006,15.2,4.54251631399998));
#250125=CARTESIAN_POINT('Ctrl Pts',(-9.52710529500006,11.6,4.54251631399998));
#250126=CARTESIAN_POINT('Ctrl Pts',(-9.52556247800005,15.2,4.54134816799999));
#250127=CARTESIAN_POINT('Ctrl Pts',(-9.52556247800005,11.6,4.54134816799998));
#250128=CARTESIAN_POINT('Ctrl Pts',(-9.52402433000006,15.2,4.54018575399999));
#250129=CARTESIAN_POINT('Ctrl Pts',(-9.52402433000006,11.6,4.54018575399999));
#250130=CARTESIAN_POINT('Ctrl Pts',(-9.52249087200006,15.2,4.53902907599999));
#250131=CARTESIAN_POINT('Ctrl Pts',(-9.52249087200006,11.6,4.53902907599998));
#250132=CARTESIAN_POINT('Ctrl Pts',(-9.52096212300006,15.2,4.53787813199998));
#250133=CARTESIAN_POINT('Ctrl Pts',(-9.52096212300006,11.6,4.53787813199998));
#250134=CARTESIAN_POINT('Ctrl Pts',(-9.51943810400006,15.2,4.53673292199999));
#250135=CARTESIAN_POINT('Ctrl Pts',(-9.51943810400006,11.6,4.53673292199999));
#250136=CARTESIAN_POINT('Ctrl Pts',(-9.51791883400006,15.2,4.53559344699999));
#250137=CARTESIAN_POINT('Ctrl Pts',(-9.51791883400006,11.6,4.53559344699999));
#250138=CARTESIAN_POINT('Ctrl Pts',(-9.51640433300006,15.2,4.53445970499998));
#250139=CARTESIAN_POINT('Ctrl Pts',(-9.51640433300006,11.6,4.53445970499998));
#250140=CARTESIAN_POINT('Ctrl Pts',(-9.51489462200006,15.2,4.53333169899999));
#250141=CARTESIAN_POINT('Ctrl Pts',(-9.51489462200006,11.6,4.53333169899999));
#250142=CARTESIAN_POINT('Ctrl Pts',(-9.51338972000006,15.2,4.53220942699998));
#250143=CARTESIAN_POINT('Ctrl Pts',(-9.51338972000006,11.6,4.53220942699998));
#250144=CARTESIAN_POINT('Ctrl Pts',(-9.51188964800006,15.2,4.53109288999999));
#250145=CARTESIAN_POINT('Ctrl Pts',(-9.51188964800006,11.6,4.53109288999998));
#250146=CARTESIAN_POINT('Ctrl Pts',(-9.51039442600005,15.2,4.52998208699999));
#250147=CARTESIAN_POINT('Ctrl Pts',(-9.51039442600005,11.6,4.52998208699999));
#250148=CARTESIAN_POINT('Ctrl Pts',(-9.50890407400006,15.2,4.52887701899999));
#250149=CARTESIAN_POINT('Ctrl Pts',(-9.50890407400006,11.6,4.52887701899999));
#250150=CARTESIAN_POINT('Ctrl Pts',(-9.50741861400006,15.2,4.52777768499999));
#250151=CARTESIAN_POINT('Ctrl Pts',(-9.50741861400006,11.6,4.52777768499998));
#250152=CARTESIAN_POINT('Ctrl Pts',(-9.50593806600006,15.2,4.52668408599998));
#250153=CARTESIAN_POINT('Ctrl Pts',(-9.50593806600006,11.6,4.52668408599998));
#250154=CARTESIAN_POINT('Ctrl Pts',(-9.50446244800006,15.2,4.52559622099999));
#250155=CARTESIAN_POINT('Ctrl Pts',(-9.50446244800006,11.6,4.52559622099999));
#250156=CARTESIAN_POINT('Ctrl Pts',(-9.50299178500006,15.2,4.52451408999998));
#250157=CARTESIAN_POINT('Ctrl Pts',(-9.50299178500006,11.6,4.52451408999998));
#250158=CARTESIAN_POINT('Ctrl Pts',(-9.50152609500006,15.2,4.52343769399998));
#250159=CARTESIAN_POINT('Ctrl Pts',(-9.50152609500006,11.6,4.52343769399998));
#250160=CARTESIAN_POINT('Ctrl Pts',(-9.50006539900006,15.2,4.52236703199999));
#250161=CARTESIAN_POINT('Ctrl Pts',(-9.50006539900006,11.6,4.52236703199999));
#250162=CARTESIAN_POINT('Ctrl Pts',(-9.49860971900006,15.2,4.52130210399999));
#250163=CARTESIAN_POINT('Ctrl Pts',(-9.49860971900006,11.6,4.52130210399999));
#250164=CARTESIAN_POINT('Ctrl Pts',(-9.49715907600006,15.2,4.52024290899999));
#250165=CARTESIAN_POINT('Ctrl Pts',(-9.49715907600006,11.6,4.52024290899998));
#250166=CARTESIAN_POINT('Ctrl Pts',(-9.49571348900006,15.2,4.51918944999999));
#250167=CARTESIAN_POINT('Ctrl Pts',(-9.49571348900006,11.6,4.51918944999999));
#250168=CARTESIAN_POINT('Ctrl Pts',(-9.49427298200006,15.2,4.51814172299999));
#250169=CARTESIAN_POINT('Ctrl Pts',(-9.49427298200006,11.6,4.51814172299999));
#250170=CARTESIAN_POINT('Ctrl Pts',(-9.49283757400006,15.2,4.51709972999998));
#250171=CARTESIAN_POINT('Ctrl Pts',(-9.49283757400006,11.6,4.51709972999998));
#250172=CARTESIAN_POINT('Ctrl Pts',(-9.49140728700005,15.2,4.51606347099998));
#250173=CARTESIAN_POINT('Ctrl Pts',(-9.49140728700005,11.6,4.51606347099998));
#250174=CARTESIAN_POINT('Ctrl Pts',(-9.48998214300006,15.2,4.51503294499998));
#250175=CARTESIAN_POINT('Ctrl Pts',(-9.48998214300006,11.6,4.51503294499998));
#250176=CARTESIAN_POINT('Ctrl Pts',(-9.48856216300005,15.2,4.51400815099999));
#250177=CARTESIAN_POINT('Ctrl Pts',(-9.48856216300005,11.6,4.51400815099999));
#250178=CARTESIAN_POINT('Ctrl Pts',(-9.48714736900006,15.2,4.51298908999998));
#250179=CARTESIAN_POINT('Ctrl Pts',(-9.48714736900006,11.6,4.51298908999998));
#250180=CARTESIAN_POINT('Ctrl Pts',(-9.48573778000006,15.2,4.51197576299998));
#250181=CARTESIAN_POINT('Ctrl Pts',(-9.48573778000006,11.6,4.51197576299998));
#250182=CARTESIAN_POINT('Ctrl Pts',(-9.48433342200006,15.2,4.51096816699998));
#250183=CARTESIAN_POINT('Ctrl Pts',(-9.48433342200006,11.6,4.51096816699998));
#250184=CARTESIAN_POINT('Ctrl Pts',(-9.48293431400005,15.2,4.50996630299999));
#250185=CARTESIAN_POINT('Ctrl Pts',(-9.48293431400005,11.6,4.50996630299999));
#250186=CARTESIAN_POINT('Ctrl Pts',(-9.48154047900006,15.2,4.50897017199999));
#250187=CARTESIAN_POINT('Ctrl Pts',(-9.48154047900006,11.6,4.50897017199999));
#250188=CARTESIAN_POINT('Ctrl Pts',(-9.48015193800006,15.2,4.50797977199999));
#250189=CARTESIAN_POINT('Ctrl Pts',(-9.48015193800006,11.6,4.50797977199999));
#250190=CARTESIAN_POINT('Ctrl Pts',(-9.47876871400006,15.2,4.50699510299999));
#250191=CARTESIAN_POINT('Ctrl Pts',(-9.47876871400006,11.6,4.50699510299999));
#250192=CARTESIAN_POINT('Ctrl Pts',(-9.47739082700006,15.2,4.50601616499998));
#250193=CARTESIAN_POINT('Ctrl Pts',(-9.47739082700006,11.6,4.50601616499998));
#250194=CARTESIAN_POINT('Ctrl Pts',(-9.47601830200006,15.2,4.50504295799998));
#250195=CARTESIAN_POINT('Ctrl Pts',(-9.47601830200006,11.6,4.50504295799998));
#250196=CARTESIAN_POINT('Ctrl Pts',(-9.47465116000006,15.2,4.50407548099999));
#250197=CARTESIAN_POINT('Ctrl Pts',(-9.47465116000006,11.6,4.50407548099999));
#250198=CARTESIAN_POINT('Ctrl Pts',(-9.47328942300006,15.2,4.50311373399998));
#250199=CARTESIAN_POINT('Ctrl Pts',(-9.47328942300006,11.6,4.50311373399998));
#250200=CARTESIAN_POINT('Ctrl Pts',(-9.47193311400006,15.2,4.50215771699998));
#250201=CARTESIAN_POINT('Ctrl Pts',(-9.47193311400006,11.6,4.50215771699998));
#250202=CARTESIAN_POINT('Ctrl Pts',(-9.47058225500006,15.2,4.50120742799999));
#250203=CARTESIAN_POINT('Ctrl Pts',(-9.47058225500006,11.6,4.50120742799999));
#250204=CARTESIAN_POINT('Ctrl Pts',(-9.46923686900006,15.2,4.50026286999999));
#250205=CARTESIAN_POINT('Ctrl Pts',(-9.46923686900006,11.6,4.50026286999999));
#250206=CARTESIAN_POINT('Ctrl Pts',(-9.46789697900006,15.2,4.49932403899999));
#250207=CARTESIAN_POINT('Ctrl Pts',(-9.46789697900006,11.6,4.49932403899999));
#250208=CARTESIAN_POINT('Ctrl Pts',(-9.46656260800006,15.2,4.49839093599999));
#250209=CARTESIAN_POINT('Ctrl Pts',(-9.46656260800006,11.6,4.49839093599999));
#250210=CARTESIAN_POINT('Ctrl Pts',(-9.46523377700006,15.2,4.49746356099999));
#250211=CARTESIAN_POINT('Ctrl Pts',(-9.46523377700006,11.6,4.49746356099998));
#250212=CARTESIAN_POINT('Ctrl Pts',(-9.46391051100005,15.2,4.49654191199999));
#250213=CARTESIAN_POINT('Ctrl Pts',(-9.46391051100005,11.6,4.49654191199999));
#250214=CARTESIAN_POINT('Ctrl Pts',(-9.46259283200006,15.2,4.49562599099998));
#250215=CARTESIAN_POINT('Ctrl Pts',(-9.46259283200006,11.6,4.49562599099998));
#250216=CARTESIAN_POINT('Ctrl Pts',(-9.46128076500005,15.2,4.49471579599999));
#250217=CARTESIAN_POINT('Ctrl Pts',(-9.46128076500005,11.6,4.49471579599999));
#250218=CARTESIAN_POINT('Ctrl Pts',(-9.45997433000005,15.2,4.49381132699998));
#250219=CARTESIAN_POINT('Ctrl Pts',(-9.45997433000005,11.6,4.49381132699998));
#250220=CARTESIAN_POINT('Ctrl Pts',(-9.45867355200006,15.2,4.49291258199998));
#250221=CARTESIAN_POINT('Ctrl Pts',(-9.45867355200006,11.6,4.49291258199998));
#250222=CARTESIAN_POINT('Ctrl Pts',(-9.45737845600006,15.2,4.49201956299999));
#250223=CARTESIAN_POINT('Ctrl Pts',(-9.45737845600006,11.6,4.49201956299999));
#250224=CARTESIAN_POINT('Ctrl Pts',(-9.45608906200006,15.2,4.49113226799999));
#250225=CARTESIAN_POINT('Ctrl Pts',(-9.45608906200006,11.6,4.49113226799999));
#250226=CARTESIAN_POINT('Ctrl Pts',(-9.45480539700006,15.2,4.49025069599998));
#250227=CARTESIAN_POINT('Ctrl Pts',(-9.45480539700006,11.6,4.49025069599998));
#250228=CARTESIAN_POINT('Ctrl Pts',(-9.45352748300006,15.2,4.48937484699999));
#250229=CARTESIAN_POINT('Ctrl Pts',(-9.45352748300006,11.6,4.48937484699999));
#250230=CARTESIAN_POINT('Ctrl Pts',(-9.45225534400005,15.2,4.48850472099998));
#250231=CARTESIAN_POINT('Ctrl Pts',(-9.45225534400005,11.6,4.48850472099998));
#250232=CARTESIAN_POINT('Ctrl Pts',(-9.45098900300006,15.2,4.48764031599998));
#250233=CARTESIAN_POINT('Ctrl Pts',(-9.45098900300006,11.6,4.48764031599998));
#250234=CARTESIAN_POINT('Ctrl Pts',(-9.44972848600005,15.2,4.48678163399999));
#250235=CARTESIAN_POINT('Ctrl Pts',(-9.44972848600005,11.6,4.48678163399998));
#250236=CARTESIAN_POINT('Ctrl Pts',(-9.44847381600006,15.2,4.48592867099999));
#250237=CARTESIAN_POINT('Ctrl Pts',(-9.44847381600006,11.6,4.48592867099998));
#250238=CARTESIAN_POINT('Ctrl Pts',(-9.44722501700006,15.2,4.48508142899998));
#250239=CARTESIAN_POINT('Ctrl Pts',(-9.44722501700006,11.6,4.48508142899998));
#250240=CARTESIAN_POINT('Ctrl Pts',(-9.44598211300006,15.2,4.48423990499998));
#250241=CARTESIAN_POINT('Ctrl Pts',(-9.44598211300006,11.6,4.48423990499998));
#250242=CARTESIAN_POINT('Ctrl Pts',(-9.44474512900005,15.2,4.48340410099998));
#250243=CARTESIAN_POINT('Ctrl Pts',(-9.44474512900005,11.6,4.48340410099998));
#250244=CARTESIAN_POINT('Ctrl Pts',(-9.44351409000006,15.2,4.48257401399999));
#250245=CARTESIAN_POINT('Ctrl Pts',(-9.44351409000006,11.6,4.48257401399999));
#250246=CARTESIAN_POINT('Ctrl Pts',(-9.44228901900006,15.2,4.48174964399998));
#250247=CARTESIAN_POINT('Ctrl Pts',(-9.44228901900006,11.6,4.48174964399998));
#250248=CARTESIAN_POINT('Ctrl Pts',(-9.44106994200006,15.2,4.48093099099999));
#250249=CARTESIAN_POINT('Ctrl Pts',(-9.44106994200006,11.6,4.48093099099999));
#250250=CARTESIAN_POINT('Ctrl Pts',(-9.43985688300006,15.2,4.48011805499998));
#250251=CARTESIAN_POINT('Ctrl Pts',(-9.43985688300006,11.6,4.48011805499998));
#250252=CARTESIAN_POINT('Ctrl Pts',(-9.43864986800006,15.2,4.47931083199999));
#250253=CARTESIAN_POINT('Ctrl Pts',(-9.43864986800006,11.6,4.47931083199998));
#250254=CARTESIAN_POINT('Ctrl Pts',(-9.43744892000005,15.2,4.47850932399999));
#250255=CARTESIAN_POINT('Ctrl Pts',(-9.43744892000005,11.6,4.47850932399999));
#250256=CARTESIAN_POINT('Ctrl Pts',(-9.43625406500006,15.2,4.47771352899998));
#250257=CARTESIAN_POINT('Ctrl Pts',(-9.43625406500006,11.6,4.47771352899998));
#250258=CARTESIAN_POINT('Ctrl Pts',(-9.43506532900006,15.2,4.47692344699998));
#250259=CARTESIAN_POINT('Ctrl Pts',(-9.43506532900006,11.6,4.47692344699998));
#250260=CARTESIAN_POINT('Ctrl Pts',(-9.43388273800006,15.2,4.47613907699999));
#250261=CARTESIAN_POINT('Ctrl Pts',(-9.43388273800006,11.6,4.47613907699999));
#250262=CARTESIAN_POINT('Ctrl Pts',(-9.43270631400006,15.2,4.47536041899999));
#250263=CARTESIAN_POINT('Ctrl Pts',(-9.43270631400006,11.6,4.47536041899998));
#250264=CARTESIAN_POINT('Ctrl Pts',(-9.43153608500005,15.2,4.47458746899999));
#250265=CARTESIAN_POINT('Ctrl Pts',(-9.43153608500005,11.6,4.47458746899999));
#250266=CARTESIAN_POINT('Ctrl Pts',(-9.43037207700005,15.2,4.47382022999999));
#250267=CARTESIAN_POINT('Ctrl Pts',(-9.43037207700005,11.6,4.47382022999999));
#250268=CARTESIAN_POINT('Ctrl Pts',(-9.42921431500006,15.2,4.47305869799998));
#250269=CARTESIAN_POINT('Ctrl Pts',(-9.42921431500006,11.6,4.47305869799998));
#250270=CARTESIAN_POINT('Ctrl Pts',(-9.42806282300005,15.2,4.47230287499998));
#250271=CARTESIAN_POINT('Ctrl Pts',(-9.42806282300005,11.6,4.47230287499998));
#250272=CARTESIAN_POINT('Ctrl Pts',(-9.42691763000006,15.2,4.47155275699998));
#250273=CARTESIAN_POINT('Ctrl Pts',(-9.42691763000006,11.6,4.47155275699998));
#250274=CARTESIAN_POINT('Ctrl Pts',(-9.42577876100006,15.2,4.47080834499998));
#250275=CARTESIAN_POINT('Ctrl Pts',(-9.42577876100006,11.6,4.47080834499998));
#250276=CARTESIAN_POINT('Ctrl Pts',(-9.42464624100005,15.2,4.47006963699998));
#250277=CARTESIAN_POINT('Ctrl Pts',(-9.42464624100005,11.6,4.47006963699998));
#250278=CARTESIAN_POINT('Ctrl Pts',(-9.42352009700006,15.2,4.46933663299999));
#250279=CARTESIAN_POINT('Ctrl Pts',(-9.42352009700006,11.6,4.46933663299998));
#250280=CARTESIAN_POINT('Ctrl Pts',(-9.42240035600006,15.2,4.46860933299998));
#250281=CARTESIAN_POINT('Ctrl Pts',(-9.42240035600006,11.6,4.46860933299998));
#250282=CARTESIAN_POINT('Ctrl Pts',(-9.42128704400006,15.2,4.46788773299998));
#250283=CARTESIAN_POINT('Ctrl Pts',(-9.42128704400006,11.6,4.46788773299998));
#250284=CARTESIAN_POINT('Ctrl Pts',(-9.42018018800006,15.2,4.46717183299998));
#250285=CARTESIAN_POINT('Ctrl Pts',(-9.42018018800006,11.6,4.46717183299998));
#250286=CARTESIAN_POINT('Ctrl Pts',(-9.41907981300006,15.2,4.46646163399999));
#250287=CARTESIAN_POINT('Ctrl Pts',(-9.41907981300006,11.6,4.46646163399999));
#250288=CARTESIAN_POINT('Ctrl Pts',(-9.41798594800006,15.2,4.46575713399999));
#250289=CARTESIAN_POINT('Ctrl Pts',(-9.41798594800006,11.6,4.46575713399999));
#250290=CARTESIAN_POINT('Ctrl Pts',(-9.41689861900005,15.2,4.46505832999998));
#250291=CARTESIAN_POINT('Ctrl Pts',(-9.41689861900005,11.6,4.46505832999998));
#250292=CARTESIAN_POINT('Ctrl Pts',(-9.41581785300006,15.2,4.46436522199999));
#250293=CARTESIAN_POINT('Ctrl Pts',(-9.41581785300006,11.6,4.46436522199999));
#250294=CARTESIAN_POINT('Ctrl Pts',(-9.41474367800006,15.2,4.46367780999999));
#250295=CARTESIAN_POINT('Ctrl Pts',(-9.41474367800006,11.6,4.46367780999999));
#250296=CARTESIAN_POINT('Ctrl Pts',(-9.41367611900005,15.2,4.46299609199999));
#250297=CARTESIAN_POINT('Ctrl Pts',(-9.41367611900005,11.6,4.46299609199999));
#250298=CARTESIAN_POINT('Ctrl Pts',(-9.41261520700006,15.2,4.46232006599999));
#250299=CARTESIAN_POINT('Ctrl Pts',(-9.41261520700006,11.6,4.46232006599998));
#250300=CARTESIAN_POINT('Ctrl Pts',(-9.41156096700006,15.2,4.46164973199998));
#250301=CARTESIAN_POINT('Ctrl Pts',(-9.41156096700006,11.6,4.46164973199998));
#250302=CARTESIAN_POINT('Ctrl Pts',(-9.41051342700005,15.2,4.46098508799999));
#250303=CARTESIAN_POINT('Ctrl Pts',(-9.41051342700005,11.6,4.46098508799999));
#250304=CARTESIAN_POINT('Ctrl Pts',(-9.40947261500006,15.2,4.46032613399999));
#250305=CARTESIAN_POINT('Ctrl Pts',(-9.40947261500006,11.6,4.46032613399998));
#250306=CARTESIAN_POINT('Ctrl Pts',(-9.40843855900006,15.2,4.45967286799998));
#250307=CARTESIAN_POINT('Ctrl Pts',(-9.40843855900006,11.6,4.45967286799998));
#250308=CARTESIAN_POINT('Ctrl Pts',(-9.40741128800006,15.2,4.45902528699998));
#250309=CARTESIAN_POINT('Ctrl Pts',(-9.40741128800006,11.6,4.45902528699998));
#250310=CARTESIAN_POINT('Ctrl Pts',(-9.40639082900006,15.2,4.45838339299998));
#250311=CARTESIAN_POINT('Ctrl Pts',(-9.40639082900006,11.6,4.45838339299998));
#250312=CARTESIAN_POINT('Ctrl Pts',(-9.40537721000006,15.2,4.45774718299998));
#250313=CARTESIAN_POINT('Ctrl Pts',(-9.40537721000006,11.6,4.45774718299998));
#250314=CARTESIAN_POINT('Ctrl Pts',(-9.40437046000006,15.2,4.45711665599998));
#250315=CARTESIAN_POINT('Ctrl Pts',(-9.40437046000006,11.6,4.45711665599998));
#250316=CARTESIAN_POINT('Ctrl Pts',(-9.40337060800006,15.2,4.45649180999999));
#250317=CARTESIAN_POINT('Ctrl Pts',(-9.40337060800006,11.6,4.45649180999998));
#250318=CARTESIAN_POINT('Ctrl Pts',(-9.40237768200006,15.2,4.45587264399999));
#250319=CARTESIAN_POINT('Ctrl Pts',(-9.40237768200006,11.6,4.45587264399998));
#250320=CARTESIAN_POINT('Ctrl Pts',(-9.40139171200006,15.2,4.45525915699999));
#250321=CARTESIAN_POINT('Ctrl Pts',(-9.40139171200006,11.6,4.45525915699999));
#250322=CARTESIAN_POINT('Ctrl Pts',(-9.40041272400006,15.2,4.45465134699998));
#250323=CARTESIAN_POINT('Ctrl Pts',(-9.40041272400006,11.6,4.45465134699998));
#250324=CARTESIAN_POINT('Ctrl Pts',(-9.39944075100006,15.2,4.45404921299998));
#250325=CARTESIAN_POINT('Ctrl Pts',(-9.39944075100006,11.6,4.45404921299998));
#250326=CARTESIAN_POINT('Ctrl Pts',(-9.39847582000005,15.2,4.45345275499999));
#250327=CARTESIAN_POINT('Ctrl Pts',(-9.39847582000005,11.6,4.45345275499999));
#250328=CARTESIAN_POINT('Ctrl Pts',(-9.39751796100006,15.2,4.45286196799999));
#250329=CARTESIAN_POINT('Ctrl Pts',(-9.39751796100006,11.6,4.45286196799999));
#250330=CARTESIAN_POINT('Ctrl Pts',(-9.39656720200006,15.2,4.45227685299999));
#250331=CARTESIAN_POINT('Ctrl Pts',(-9.39656720200006,11.6,4.45227685299999));
#250332=CARTESIAN_POINT('Ctrl Pts',(-9.39562357500006,15.2,4.45169740899999));
#250333=CARTESIAN_POINT('Ctrl Pts',(-9.39562357500006,11.6,4.45169740899999));
#250334=CARTESIAN_POINT('Ctrl Pts',(-9.39468710800006,15.2,4.45112363199998));
#250335=CARTESIAN_POINT('Ctrl Pts',(-9.39468710800006,11.6,4.45112363199998));
#250336=CARTESIAN_POINT('Ctrl Pts',(-9.39375783100006,15.2,4.45055552199998));
#250337=CARTESIAN_POINT('Ctrl Pts',(-9.39375783100006,11.6,4.45055552199998));
#250338=CARTESIAN_POINT('Ctrl Pts',(-9.39283577600006,15.2,4.44999307799999));
#250339=CARTESIAN_POINT('Ctrl Pts',(-9.39283577600006,11.6,4.44999307799998));
#250340=CARTESIAN_POINT('Ctrl Pts',(-9.39192097100005,15.2,4.44943629799998));
#250341=CARTESIAN_POINT('Ctrl Pts',(-9.39192097100005,11.6,4.44943629799998));
#250342=CARTESIAN_POINT('Ctrl Pts',(-9.39101344700006,15.2,4.44888517999999));
#250343=CARTESIAN_POINT('Ctrl Pts',(-9.39101344700006,11.6,4.44888517999999));
#250344=CARTESIAN_POINT('Ctrl Pts',(-9.39011323600005,15.2,4.44833972299998));
#250345=CARTESIAN_POINT('Ctrl Pts',(-9.39011323600005,11.6,4.44833972299998));
#250346=CARTESIAN_POINT('Ctrl Pts',(-9.38922036600006,15.2,4.44779992399998));
#250347=CARTESIAN_POINT('Ctrl Pts',(-9.38922036600006,11.6,4.44779992399998));
#250348=CARTESIAN_POINT('Ctrl Pts',(-9.38833486900006,15.2,4.44726578299999));
#250349=CARTESIAN_POINT('Ctrl Pts',(-9.38833486900006,11.6,4.44726578299999));
#250350=CARTESIAN_POINT('Ctrl Pts',(-9.38745677700006,15.2,4.44673729799998));
#250351=CARTESIAN_POINT('Ctrl Pts',(-9.38745677700006,11.6,4.44673729799998));
#250352=CARTESIAN_POINT('Ctrl Pts',(-9.38658611800006,15.2,4.44621446599999));
#250353=CARTESIAN_POINT('Ctrl Pts',(-9.38658611800006,11.6,4.44621446599999));
#250354=CARTESIAN_POINT('Ctrl Pts',(-9.38572292800006,15.2,4.44569728599999));
#250355=CARTESIAN_POINT('Ctrl Pts',(-9.38572292800006,11.6,4.44569728599998));
#250356=CARTESIAN_POINT('Ctrl Pts',(-9.38486723400005,15.2,4.44518575599999));
#250357=CARTESIAN_POINT('Ctrl Pts',(-9.38486723400005,11.6,4.44518575599999));
#250358=CARTESIAN_POINT('Ctrl Pts',(-9.38401906900006,15.2,4.44467987499999));
#250359=CARTESIAN_POINT('Ctrl Pts',(-9.38401906900006,11.6,4.44467987499999));
#250360=CARTESIAN_POINT('Ctrl Pts',(-9.38317846500006,15.2,4.44417964099999));
#250361=CARTESIAN_POINT('Ctrl Pts',(-9.38317846500006,11.6,4.44417964099998));
#250362=CARTESIAN_POINT('Ctrl Pts',(-9.38234545400006,15.2,4.44368505099998));
#250363=CARTESIAN_POINT('Ctrl Pts',(-9.38234545400006,11.6,4.44368505099998));
#250364=CARTESIAN_POINT('Ctrl Pts',(-9.38152006800006,15.2,4.44319610499999));
#250365=CARTESIAN_POINT('Ctrl Pts',(-9.38152006800006,11.6,4.44319610499999));
#250366=CARTESIAN_POINT('Ctrl Pts',(-9.38070233900006,15.2,4.44271279999998));
#250367=CARTESIAN_POINT('Ctrl Pts',(-9.38070233900006,11.6,4.44271279999998));
#250368=CARTESIAN_POINT('Ctrl Pts',(-9.37989229900005,15.2,4.44223513399999));
#250369=CARTESIAN_POINT('Ctrl Pts',(-9.37989229900005,11.6,4.44223513399999));
#250370=CARTESIAN_POINT('Ctrl Pts',(-9.37908998000006,15.2,4.44176310499999));
#250371=CARTESIAN_POINT('Ctrl Pts',(-9.37908998000006,11.6,4.44176310499999));
#250372=CARTESIAN_POINT('Ctrl Pts',(-9.37829999300006,15.2,4.44129939799998));
#250373=CARTESIAN_POINT('Ctrl Pts',(-9.37829999300006,11.6,4.44129939799998));
#250374=CARTESIAN_POINT('Ctrl Pts',(-9.37767505800006,15.2,4.44093341099999));
#250375=CARTESIAN_POINT('Ctrl Pts',(-9.37767505800006,11.6,4.44093341099998));
#250376=CARTESIAN_POINT('Ctrl Pts',(-9.37721094100005,15.2,4.44066207099999));
#250377=CARTESIAN_POINT('Ctrl Pts',(-9.37721094100005,11.6,4.44066207099999));
#250378=CARTESIAN_POINT('Ctrl Pts',(-9.37690455300006,15.2,4.44048314699998));
#250379=CARTESIAN_POINT('Ctrl Pts',(-9.37690455300006,11.6,4.44048314699998));
#250380=CARTESIAN_POINT('Ctrl Pts',(-9.37675396800006,15.2,4.44039525799998));
#250381=CARTESIAN_POINT('Ctrl Pts',(-9.37675396800006,11.6,4.44039525799998));
#250382=CARTESIAN_POINT('',(-9.37675396726197,12.2,4.44039525796617));
#250383=CARTESIAN_POINT('',(-9.37675396726197,15.2,4.44039525796617));
#250384=CARTESIAN_POINT('',(-9.37675396700006,12.2,4.44039525799998));
#250385=CARTESIAN_POINT('Ctrl Pts',(-10.2217148780001,12.2,5.26939701899998));
#250386=CARTESIAN_POINT('Ctrl Pts',(-10.2194283575847,12.2,5.26633326844343));
#250387=CARTESIAN_POINT('Ctrl Pts',(-10.2171423378183,12.2,5.26327740164306));
#250388=CARTESIAN_POINT('Ctrl Pts',(-10.2148568145106,12.2,5.26022941979131));
#250389=CARTESIAN_POINT('Ctrl Pts',(-10.212571291203,12.2,5.25718143793957));
#250390=CARTESIAN_POINT('Ctrl Pts',(-10.2102862662399,12.2,5.25414134087888));
#250391=CARTESIAN_POINT('Ctrl Pts',(-10.2080017562504,12.2,5.25110913437833));
#250392=CARTESIAN_POINT('Ctrl Pts',(-10.2057172462609,12.2,5.24807692787778));
#250393=CARTESIAN_POINT('Ctrl Pts',(-10.2034332515483,12.2,5.24505261033232));
#250394=CARTESIAN_POINT('Ctrl Pts',(-10.2011498145062,12.2,5.24203619464918));
#250395=CARTESIAN_POINT('Ctrl Pts',(-10.1988663770492,12.2,5.23901977841805));
#250396=CARTESIAN_POINT('Ctrl Pts',(-10.1965834982841,12.2,5.23601126379749));
#250397=CARTESIAN_POINT('Ctrl Pts',(-10.1943012262858,12.2,5.23301066211247));
#250398=CARTESIAN_POINT('Ctrl Pts',(-10.1920189547022,12.2,5.23001006097256));
#250399=CARTESIAN_POINT('Ctrl Pts',(-10.1897372904352,12.2,5.22701737409891));
#250400=CARTESIAN_POINT('Ctrl Pts',(-10.1874562702264,12.2,5.22403260995806));
#250401=CARTESIAN_POINT('Ctrl Pts',(-10.1851752500177,12.2,5.2210478458172));
#250402=CARTESIAN_POINT('Ctrl Pts',(-10.1828948737922,12.2,5.21807100541948));
#250403=CARTESIAN_POINT('Ctrl Pts',(-10.1806151784896,12.2,5.21510209722224));
#250404=CARTESIAN_POINT('Ctrl Pts',(-10.1783354831871,12.2,5.21213318902499));
#250405=CARTESIAN_POINT('Ctrl Pts',(-10.1760564669297,12.2,5.20917221267545));
#250406=CARTESIAN_POINT('Ctrl Pts',(-10.1737781722521,12.2,5.20621917897761));
#250407=CARTESIAN_POINT('Ctrl Pts',(-10.1714998775745,12.2,5.20326614527977));
#250408=CARTESIAN_POINT('Ctrl Pts',(-10.1692223041823,12.2,5.2003210545142));
#250409=CARTESIAN_POINT('Ctrl Pts',(-10.1669454934732,12.2,5.19738391682855));
#250410=CARTESIAN_POINT('Ctrl Pts',(-10.1646686827642,12.2,5.1944467791429));
#250411=CARTESIAN_POINT('Ctrl Pts',(-10.1623926336802,12.2,5.19151759504837));
#250412=CARTESIAN_POINT('Ctrl Pts',(-10.1601173874711,12.2,5.18859637286176));
#250413=CARTESIAN_POINT('Ctrl Pts',(-10.1578421408486,12.2,5.18567515014445));
#250414=CARTESIAN_POINT('Ctrl Pts',(-10.1555676965681,12.2,5.18276188983774));
#250415=CARTESIAN_POINT('Ctrl Pts',(-10.1532940939877,12.2,5.17985660212492));
#250416=CARTESIAN_POINT('Ctrl Pts',(-10.1510204918205,12.2,5.1769513149399));
#250417=CARTESIAN_POINT('Ctrl Pts',(-10.1487477321747,12.2,5.17405400122943));
#250418=CARTESIAN_POINT('Ctrl Pts',(-10.1464758553522,12.2,5.17116466848266));
#250419=CARTESIAN_POINT('Ctrl Pts',(-10.1434466863931,12.2,5.16731222499526));
#250420=CARTESIAN_POINT('Ctrl Pts',(-10.1404190870807,12.2,5.16347397394543));
#250421=CARTESIAN_POINT('Ctrl Pts',(-10.1373931562724,12.2,5.15964993581268));
#250422=CARTESIAN_POINT('Ctrl Pts',(-10.1351237080631,12.2,5.15678190708286));
#250423=CARTESIAN_POINT('Ctrl Pts',(-10.1328551960955,12.2,5.15392187333583));
#250424=CARTESIAN_POINT('Ctrl Pts',(-10.1305876639694,12.2,5.15106984464668));
#250425=CARTESIAN_POINT('Ctrl Pts',(-10.1283201314313,12.2,5.14821781543941));
#250426=CARTESIAN_POINT('Ctrl Pts',(-10.1260535790853,12.2,5.14537379159276));
#250427=CARTESIAN_POINT('Ctrl Pts',(-10.1237880465062,12.2,5.14253778234836));
#250428=CARTESIAN_POINT('Ctrl Pts',(-10.1215225143386,12.2,5.13970177361917));
#250429=CARTESIAN_POINT('Ctrl Pts',(-10.1192580022095,12.2,5.13687377885858));
#250430=CARTESIAN_POINT('Ctrl Pts',(-10.1169945533455,12.2,5.13405380894608));
#250431=CARTESIAN_POINT('Ctrl Pts',(-10.1147311044814,12.2,5.13123383903358));
#250432=CARTESIAN_POINT('Ctrl Pts',(-10.1124687166213,12.2,5.12842189314187));
#250433=CARTESIAN_POINT('Ctrl Pts',(-10.1102074339953,12.2,5.12561798091111));
#250434=CARTESIAN_POINT('Ctrl Pts',(-10.1079461513692,12.2,5.12281406868035));
#250435=CARTESIAN_POINT('Ctrl Pts',(-10.1056859740846,12.2,5.12001819071531));
#250436=CARTESIAN_POINT('Ctrl Pts',(-10.103426942,12.2,5.11723035506659));
#250437=CARTESIAN_POINT('Ctrl Pts',(-10.1011679099155,12.2,5.11444251941788));
#250438=CARTESIAN_POINT('Ctrl Pts',(-10.0989100241975,12.2,5.11166272795219));
#250439=CARTESIAN_POINT('Ctrl Pts',(-10.0966533284877,12.2,5.10889098830218));
#250440=CARTESIAN_POINT('Ctrl Pts',(-10.0943966327779,12.2,5.10611924865216));
#250441=CARTESIAN_POINT('Ctrl Pts',(-10.0921411251431,12.2,5.10335556185167));
#250442=CARTESIAN_POINT('Ctrl Pts',(-10.0898868499748,12.2,5.10059993711733));
#250443=CARTESIAN_POINT('Ctrl Pts',(-10.087632574397,12.2,5.09784431188239));
#250444=CARTESIAN_POINT('Ctrl Pts',(-10.0853795308196,12.2,5.09509674864976));
#250445=CARTESIAN_POINT('Ctrl Pts',(-10.0831277617842,12.2,5.0923572564194));
#250446=CARTESIAN_POINT('Ctrl Pts',(-10.0808759931578,12.2,5.08961776468671));
#250447=CARTESIAN_POINT('Ctrl Pts',(-10.0786254987287,12.2,5.08688634419262));
#250448=CARTESIAN_POINT('Ctrl Pts',(-10.0763763225316,12.2,5.08416300478145));
#250449=CARTESIAN_POINT('Ctrl Pts',(-10.0741271463344,12.2,5.08143966537029));
#250450=CARTESIAN_POINT('Ctrl Pts',(-10.0718792885568,12.2,5.07872440563927));
#250451=CARTESIAN_POINT('Ctrl Pts',(-10.0696327919719,12.2,5.07601723640499));
#250452=CARTESIAN_POINT('Ctrl Pts',(-10.0673862953869,12.2,5.07331006717071));
#250453=CARTESIAN_POINT('Ctrl Pts',(-10.0651411608352,12.2,5.07061098775214));
#250454=CARTESIAN_POINT('Ctrl Pts',(-10.06289743125,12.2,5.06792000697492));
#250455=CARTESIAN_POINT('Ctrl Pts',(-10.0606537016649,12.2,5.0652290261977));
#250456=CARTESIAN_POINT('Ctrl Pts',(-10.0584113772464,12.2,5.0625461441118));
#250457=CARTESIAN_POINT('Ctrl Pts',(-10.0561705022027,12.2,5.05987137033328));
#250458=CARTESIAN_POINT('Ctrl Pts',(-10.0539296271589,12.2,5.05719659655475));
#250459=CARTESIAN_POINT('Ctrl Pts',(-10.0516902020304,12.2,5.05452993068487));
#250460=CARTESIAN_POINT('Ctrl Pts',(-10.0494522698747,12.2,5.0518713822727));
#250461=CARTESIAN_POINT('Ctrl Pts',(-10.047214337719,12.2,5.04921283386054));
#250462=CARTESIAN_POINT('Ctrl Pts',(-10.0449779002563,12.2,5.04656240179774));
#250463=CARTESIAN_POINT('Ctrl Pts',(-10.0427429997539,12.2,5.04392009605929));
#250464=CARTESIAN_POINT('Ctrl Pts',(-10.0405080988456,12.2,5.04127778984082));
#250465=CARTESIAN_POINT('Ctrl Pts',(-10.0382747369043,12.2,5.03864360962468));
#250466=CARTESIAN_POINT('Ctrl Pts',(-10.0360429574969,12.2,5.0360175644108));
#250467=CARTESIAN_POINT('Ctrl Pts',(-10.0338111784948,12.2,5.03339151967399));
#250468=CARTESIAN_POINT('Ctrl Pts',(-10.0315809835594,12.2,5.03077360997007));
#250469=CARTESIAN_POINT('Ctrl Pts',(-10.0293524160155,12.2,5.02816384419061));
#250470=CARTESIAN_POINT('Ctrl Pts',(-10.0271238484716,12.2,5.02555407841114));
#250471=CARTESIAN_POINT('Ctrl Pts',(-10.0248969088106,12.2,5.02295245608174));
#250472=CARTESIAN_POINT('Ctrl Pts',(-10.0226716432147,12.2,5.02035898674758));
#250473=CARTESIAN_POINT('Ctrl Pts',(-10.0204463776188,12.2,5.01776551741343));
#250474=CARTESIAN_POINT('Ctrl Pts',(-10.0182227858814,12.2,5.01518019958702));
#250475=CARTESIAN_POINT('Ctrl Pts',(-10.0160009132854,12.2,5.01260304425227));
#250476=CARTESIAN_POINT('Ctrl Pts',(-10.0137790406894,12.2,5.01002588891752));
#250477=CARTESIAN_POINT('Ctrl Pts',(-10.0115588869948,12.2,5.0074568946202));
#250478=CARTESIAN_POINT('Ctrl Pts',(-10.0093404984919,12.2,5.00489607079587));
#250479=CARTESIAN_POINT('Ctrl Pts',(-10.007122109989,12.2,5.00233524697152));
#250480=CARTESIAN_POINT('Ctrl Pts',(-10.0049054872027,12.2,4.99978259207998));
#250481=CARTESIAN_POINT('Ctrl Pts',(-10.0026906756995,12.2,4.99723811679629));
#250482=CARTESIAN_POINT('Ctrl Pts',(-9.99973759342713,12.2,4.99384548277655));
#250483=CARTESIAN_POINT('Ctrl Pts',(-9.99678773281922,12.2,4.99046738902674));
#250484=CARTESIAN_POINT('Ctrl Pts',(-9.99384120125637,12.2,4.9871038544393));
#250485=CARTESIAN_POINT('Ctrl Pts',(-9.99163130278496,12.2,4.98458120372787));
#250486=CARTESIAN_POINT('Ctrl Pts',(-9.98942327898192,12.2,4.98206674328923));
#250487=CARTESIAN_POINT('Ctrl Pts',(-9.98721717501038,12.2,4.97956048149388));
#250488=CARTESIAN_POINT('Ctrl Pts',(-9.98427570278115,12.2,4.97621879879653));
#250489=CARTESIAN_POINT('Ctrl Pts',(-9.98133764597426,12.2,4.97289169094571));
#250490=CARTESIAN_POINT('Ctrl Pts',(-9.97840311503692,12.2,4.96957917893334));
#250491=CARTESIAN_POINT('Ctrl Pts',(-9.9754685844994,12.2,4.9662666673723));
#250492=CARTESIAN_POINT('Ctrl Pts',(-9.97253758064199,12.2,4.96296875139826));
#250493=CARTESIAN_POINT('Ctrl Pts',(-9.96961021604772,12.2,4.95968544927681));
#250494=CARTESIAN_POINT('Ctrl Pts',(-9.96668285105459,12.2,4.956402146708));
#250495=CARTESIAN_POINT('Ctrl Pts',(-9.96375912597549,12.2,4.95313345996091));
#250496=CARTESIAN_POINT('Ctrl Pts',(-9.96083915355969,12.2,4.94987940651116));
#250497=CARTESIAN_POINT('Ctrl Pts',(-9.95791918154174,12.2,4.94662535350478));
#250498=CARTESIAN_POINT('Ctrl Pts',(-9.95500296341143,12.2,4.94338593498435));
#250499=CARTESIAN_POINT('Ctrl Pts',(-9.95209061420482,12.2,4.94016117024702));
#250500=CARTESIAN_POINT('Ctrl Pts',(-9.9491782646014,12.2,4.93693640507031));
#250501=CARTESIAN_POINT('Ctrl Pts',(-9.94626978436788,12.2,4.93372629432313));
#250502=CARTESIAN_POINT('Ctrl Pts',(-9.94336528748764,12.2,4.93053085570551));
#250503=CARTESIAN_POINT('Ctrl Pts',(-9.94046079100314,12.2,4.92733541752327));
#250504=CARTESIAN_POINT('Ctrl Pts',(-9.93756027922028,12.2,4.9241546534517));
#250505=CARTESIAN_POINT('Ctrl Pts',(-9.93466386914536,12.2,4.92098857971777));
#250506=CARTESIAN_POINT('Ctrl Pts',(-9.93176745867579,12.2,4.91782250555245));
#250507=CARTESIAN_POINT('Ctrl Pts',(-9.92887515015721,12.2,4.91467112236918));
#250508=CARTESIAN_POINT('Ctrl Pts',(-9.92598706072231,12.2,4.91153445097698));
#250509=CARTESIAN_POINT('Ctrl Pts',(-9.92237694912543,12.2,4.90761361195041));
#250510=CARTESIAN_POINT('Ctrl Pts',(-9.91877343208672,12.2,4.90371575691212));
#250511=CARTESIAN_POINT('Ctrl Pts',(-9.91517674028152,12.2,4.89984092378831));
#250512=CARTESIAN_POINT('Ctrl Pts',(-9.91229938707256,12.2,4.89674105754268));
#250513=CARTESIAN_POINT('Ctrl Pts',(-9.90942640292271,12.2,4.89365592495753));
#250514=CARTESIAN_POINT('Ctrl Pts',(-9.90655790762463,12.2,4.89058554322054));
#250515=CARTESIAN_POINT('Ctrl Pts',(-9.90368941193574,12.2,4.88751516106521));
#250516=CARTESIAN_POINT('Ctrl Pts',(-9.90082540561631,12.2,4.88445953088292));
#250517=CARTESIAN_POINT('Ctrl Pts',(-9.89796601001632,12.2,4.88141866971814));
#250518=CARTESIAN_POINT('Ctrl Pts',(-9.89510661480593,12.2,4.87837780896768));
#250519=CARTESIAN_POINT('Ctrl Pts',(-9.89225183031684,12.2,4.87535171950872));
#250520=CARTESIAN_POINT('Ctrl Pts',(-9.88940177921602,12.2,4.87234041597561));
#250521=CARTESIAN_POINT('Ctrl Pts',(-9.88655172772689,12.2,4.86932911203222));
#250522=CARTESIAN_POINT('Ctrl Pts',(-9.88370640882412,12.2,4.86633259688777));
#250523=CARTESIAN_POINT('Ctrl Pts',(-9.88086594848977,12.2,4.86335088498956));
#250524=CARTESIAN_POINT('Ctrl Pts',(-9.87802548854243,12.2,4.86036917349761));
#250525=CARTESIAN_POINT('Ctrl Pts',(-9.8751898846292,12.2,4.85740226664836));
#250526=CARTESIAN_POINT('Ctrl Pts',(-9.87235926347118,12.2,4.85445018299927));
#250527=CARTESIAN_POINT('Ctrl Pts',(-9.86952864192748,12.2,4.85149809894794));
#250528=CARTESIAN_POINT('Ctrl Pts',(-9.86670300225377,12.2,4.84856083656754));
#250529=CARTESIAN_POINT('Ctrl Pts',(-9.8638824707667,12.2,4.84563841324159));
#250530=CARTESIAN_POINT('Ctrl Pts',(-9.86106193927965,12.2,4.84271598991564));
#250531=CARTESIAN_POINT('Ctrl Pts',(-9.85824651567651,12.2,4.83980840642754));
#250532=CARTESIAN_POINT('Ctrl Pts',(-9.85543632752391,12.2,4.83691567849364));
#250533=CARTESIAN_POINT('Ctrl Pts',(-9.85262613975418,12.2,4.83402295095388));
#250534=CARTESIAN_POINT('Ctrl Pts',(-9.84982118770322,12.2,4.83114507926216));
#250535=CARTESIAN_POINT('Ctrl Pts',(-9.84702159865395,12.2,4.82828207971745));
#250536=CARTESIAN_POINT('Ctrl Pts',(-9.84422200922323,12.2,4.82541907978265));
#250537=CARTESIAN_POINT('Ctrl Pts',(-9.84142778443624,12.2,4.82257095292523));
#250538=CARTESIAN_POINT('Ctrl Pts',(-9.83863905281207,12.2,4.81973771479723));
#250539=CARTESIAN_POINT('Ctrl Pts',(-9.83585032156787,12.2,4.81690447705526));
#250540=CARTESIAN_POINT('Ctrl Pts',(-9.83306708325046,12.2,4.81408612842048));
#250541=CARTESIAN_POINT('Ctrl Pts',(-9.83028946947715,12.2,4.81128268470424));
#250542=CARTESIAN_POINT('Ctrl Pts',(-9.8275118553254,12.2,4.80847924060603));
#250543=CARTESIAN_POINT('Ctrl Pts',(-9.82473986614378,12.2,4.8056907007374));
#250544=CARTESIAN_POINT('Ctrl Pts',(-9.82197363271562,12.2,4.80291708153166));
#250545=CARTESIAN_POINT('Ctrl Pts',(-9.81920739966435,12.2,4.80014346270382));
#250546=CARTESIAN_POINT('Ctrl Pts',(-9.81644692315438,12.2,4.79738476540388));
#250547=CARTESIAN_POINT('Ctrl Pts',(-9.81369233607478,12.2,4.79464100365648));
#250548=CARTESIAN_POINT('Ctrl Pts',(-9.81093774861986,12.2,4.79189724153524));
#250549=CARTESIAN_POINT('Ctrl Pts',(-9.80818905172774,12.2,4.78916841633625));
#250550=CARTESIAN_POINT('Ctrl Pts',(-9.80544637896755,12.2,4.78645454174488));
#250551=CARTESIAN_POINT('Ctrl Pts',(-9.80270370658105,12.2,4.78374066752328));
#250552=CARTESIAN_POINT('Ctrl Pts',(-9.79996705950166,12.2,4.78104174589867));
#250553=CARTESIAN_POINT('Ctrl Pts',(-9.79723657194646,12.2,4.77835778967209));
#250554=CARTESIAN_POINT('Ctrl Pts',(-9.79450608401922,12.2,4.77567383307982));
#250555=CARTESIAN_POINT('Ctrl Pts',(-9.79178175649476,12.2,4.77300484354367));
#250556=CARTESIAN_POINT('Ctrl Pts',(-9.78906372772319,12.2,4.77035083549813));
#250557=CARTESIAN_POINT('Ctrl Pts',(-9.78634569932194,12.2,4.7676968278142));
#250558=CARTESIAN_POINT('Ctrl Pts',(-9.78363396844132,12.2,4.76505780059101));
#250559=CARTESIAN_POINT('Ctrl Pts',(-9.78092867471736,12.2,4.7624337696373));
#250560=CARTESIAN_POINT('Ctrl Pts',(-9.77822338062479,12.2,4.75980973832607));
#250561=CARTESIAN_POINT('Ctrl Pts',(-9.77552452243563,12.2,4.75720070283017));
#250562=CARTESIAN_POINT('Ctrl Pts',(-9.77283224173336,12.2,4.75460667746659));
#250563=CARTESIAN_POINT('Ctrl Pts',(-9.7701399610311,12.2,4.75201265210301));
#250564=CARTESIAN_POINT('Ctrl Pts',(-9.76745425691289,12.2,4.74943363704393));
#250565=CARTESIAN_POINT('Ctrl Pts',(-9.76477527154536,12.2,4.7468696450724));
#250566=CARTESIAN_POINT('Ctrl Pts',(-9.76209628654284,12.2,4.7443056534502));
#250567=CARTESIAN_POINT('Ctrl Pts',(-9.75942401948496,12.2,4.74175668549217));
#250568=CARTESIAN_POINT('Ctrl Pts',(-9.75675861446852,12.2,4.73922275574333));
#250569=CARTESIAN_POINT('Ctrl Pts',(-9.75409320908892,12.2,4.73668882564924));
#250570=CARTESIAN_POINT('Ctrl Pts',(-9.75143466434919,12.2,4.73416993233382));
#250571=CARTESIAN_POINT('Ctrl Pts',(-9.74878312631651,12.2,4.73166609036556));
#250572=CARTESIAN_POINT('Ctrl Pts',(-9.7461315886451,12.2,4.72916224873845));
#250573=CARTESIAN_POINT('Ctrl Pts',(-9.74348705671168,12.2,4.72667345742606));
#250574=CARTESIAN_POINT('Ctrl Pts',(-9.74084967648237,12.2,4.72419973046063));
#250575=CARTESIAN_POINT('Ctrl Pts',(-9.73821229589372,12.2,4.72172600315816));
#250576=CARTESIAN_POINT('Ctrl Pts',(-9.73558206665115,12.2,4.71926734034104));
#250577=CARTESIAN_POINT('Ctrl Pts',(-9.73295913787779,12.2,4.71682375292042));
#250578=CARTESIAN_POINT('Ctrl Pts',(-9.7303362094618,12.2,4.71438016583275));
#250579=CARTESIAN_POINT('Ctrl Pts',(-9.72772057998116,12.2,4.71195165667608));
#250580=CARTESIAN_POINT('Ctrl Pts',(-9.72511239847165,12.2,4.7095382357057));
#250581=CARTESIAN_POINT('Ctrl Pts',(-9.72250421660677,12.2,4.70712481440649));
#250582=CARTESIAN_POINT('Ctrl Pts',(-9.71990348435951,12.2,4.70472648207026));
#250583=CARTESIAN_POINT('Ctrl Pts',(-9.71731035049645,12.2,4.70234325133024));
#250584=CARTESIAN_POINT('Ctrl Pts',(-9.71471721698669,12.2,4.69996002091493));
#250585=CARTESIAN_POINT('Ctrl Pts',(-9.71213168215395,12.2,4.6975918915735));
#250586=CARTESIAN_POINT('Ctrl Pts',(-9.70955389912412,12.2,4.69523887509144));
#250587=CARTESIAN_POINT('Ctrl Pts',(-9.7063316700734,12.2,4.69229760424842));
#250588=CARTESIAN_POINT('Ctrl Pts',(-9.7031215524543,12.2,4.68937994657944));
#250589=CARTESIAN_POINT('Ctrl Pts',(-9.69992384696756,12.2,4.68648592664767));
#250590=CARTESIAN_POINT('Ctrl Pts',(-9.69736568243876,12.2,4.68417071057608));
#250591=CARTESIAN_POINT('Ctrl Pts',(-9.69481546253031,12.2,4.68187062146182));
#250592=CARTESIAN_POINT('Ctrl Pts',(-9.69227334205895,12.2,4.67958567083828));
#250593=CARTESIAN_POINT('Ctrl Pts',(-9.68973122193397,12.2,4.67730072052607));
#250594=CARTESIAN_POINT('Ctrl Pts',(-9.68719720153699,12.2,4.67503090911514));
#250595=CARTESIAN_POINT('Ctrl Pts',(-9.68467143861657,12.2,4.67277624601884));
#250596=CARTESIAN_POINT('Ctrl Pts',(-9.68214567535202,12.2,4.67052158261535));
#250597=CARTESIAN_POINT('Ctrl Pts',(-9.6796281706145,12.2,4.66828206941623));
#250598=CARTESIAN_POINT('Ctrl Pts',(-9.67711908281165,12.2,4.66605771485156));
#250599=CARTESIAN_POINT('Ctrl Pts',(-9.67460999535067,12.2,4.66383336058997));
#250600=CARTESIAN_POINT('Ctrl Pts',(-9.67210932478798,12.2,4.66162416605031));
#250601=CARTESIAN_POINT('Ctrl Pts',(-9.66961723265747,12.2,4.65943014161698));
#250602=CARTESIAN_POINT('Ctrl Pts',(-9.66650211723967,12.2,4.65668761085112));
#250603=CARTESIAN_POINT('Ctrl Pts',(-9.66340040553041,12.2,4.65396878306026));
#250604=CARTESIAN_POINT('Ctrl Pts',(-9.6603124166252,12.2,4.65127367556287));
#250605=CARTESIAN_POINT('Ctrl Pts',(-9.65722442771999,12.2,4.64857856806547));
#250606=CARTESIAN_POINT('Ctrl Pts',(-9.65415016075654,12.2,4.64590718313558));
#250607=CARTESIAN_POINT('Ctrl Pts',(-9.65108994040858,12.2,4.64325953743989));
#250608=CARTESIAN_POINT('Ctrl Pts',(-9.64802972006061,12.2,4.6406118917442));
#250609=CARTESIAN_POINT('Ctrl Pts',(-9.64498354620468,12.2,4.63798798645468));
#250610=CARTESIAN_POINT('Ctrl Pts',(-9.64195174669005,12.2,4.63538783666178));
#250611=CARTESIAN_POINT('Ctrl Pts',(-9.63891994717543,12.2,4.63278768686889));
#250612=CARTESIAN_POINT('Ctrl Pts',(-9.63590252153616,12.2,4.6302112946016));
#250613=CARTESIAN_POINT('Ctrl Pts',(-9.63289980368815,12.2,4.62765867543367));
#250614=CARTESIAN_POINT('Ctrl Pts',(-9.62989708584016,12.2,4.62510605626576));
#250615=CARTESIAN_POINT('Ctrl Pts',(-9.62690907497074,12.2,4.62257720967385));
#250616=CARTESIAN_POINT('Ctrl Pts',(-9.62393610898497,12.2,4.62007215146796));
#250617=CARTESIAN_POINT('Ctrl Pts',(-9.62096314299921,12.2,4.61756709326207));
#250618=CARTESIAN_POINT('Ctrl Pts',(-9.61800522399446,12.2,4.61508582460547));
#250619=CARTESIAN_POINT('Ctrl Pts',(-9.61506269225835,12.2,4.61262835800825));
#250620=CARTESIAN_POINT('Ctrl Pts',(-9.61212016052223,12.2,4.61017089141103));
#250621=CARTESIAN_POINT('Ctrl Pts',(-9.60919301760605,12.2,4.60773722721505));
#250622=CARTESIAN_POINT('Ctrl Pts',(-9.60628161002344,12.2,4.60532737977362));
#250623=CARTESIAN_POINT('Ctrl Pts',(-9.60337020244082,12.2,4.60291753233219));
#250624=CARTESIAN_POINT('Ctrl Pts',(-9.60047453321649,12.2,4.60053150107767));
#250625=CARTESIAN_POINT('Ctrl Pts',(-9.59759495307845,12.2,4.59816929857892));
#250626=CARTESIAN_POINT('Ctrl Pts',(-9.59413945703836,12.2,4.59533465568341));
#250627=CARTESIAN_POINT('Ctrl Pts',(-9.5907071310214,12.2,4.59253432616847));
#250628=CARTESIAN_POINT('Ctrl Pts',(-9.58729859422755,12.2,4.58976832943415));
#250629=CARTESIAN_POINT('Ctrl Pts',(-9.58445814679615,12.2,4.5874633320718));
#250630=CARTESIAN_POINT('Ctrl Pts',(-9.58163422345882,12.2,4.58518217677261));
#250631=CARTESIAN_POINT('Ctrl Pts',(-9.57882718525156,12.2,4.58292487502617));
#250632=CARTESIAN_POINT('Ctrl Pts',(-9.5760201470443,12.2,4.58066757327973));
#250633=CARTESIAN_POINT('Ctrl Pts',(-9.57322999686115,12.2,4.57843412378882));
#250634=CARTESIAN_POINT('Ctrl Pts',(-9.57045710595835,12.2,4.57622453552492));
#250635=CARTESIAN_POINT('Ctrl Pts',(-9.56768421505556,12.2,4.57401494726103));
#250636=CARTESIAN_POINT('Ctrl Pts',(-9.56492858381089,12.2,4.57182922107515));
#250637=CARTESIAN_POINT('Ctrl Pts',(-9.56219058879852,12.2,4.56966736523208));
#250638=CARTESIAN_POINT('Ctrl Pts',(-9.55945259378616,12.2,4.56750550938902));
#250639=CARTESIAN_POINT('Ctrl Pts',(-9.55673223472799,12.2,4.56536752229944));
#250640=CARTESIAN_POINT('Ctrl Pts',(-9.5540298972984,12.2,4.56325341237014));
#250641=CARTESIAN_POINT('Ctrl Pts',(-9.55132755986879,12.2,4.56113930244085));
#250642=CARTESIAN_POINT('Ctrl Pts',(-9.54864324310258,12.2,4.55904906940256));
#250643=CARTESIAN_POINT('Ctrl Pts',(-9.54597733657577,12.2,4.55698271863993));
#250644=CARTESIAN_POINT('Ctrl Pts',(-9.54331143004894,12.2,4.55491636787729));
#250645=CARTESIAN_POINT('Ctrl Pts',(-9.54066393414717,12.2,4.55287389995932));
#250646=CARTESIAN_POINT('Ctrl Pts',(-9.53803524741992,12.2,4.55085531979068));
#250647=CARTESIAN_POINT('Ctrl Pts',(-9.53488082346185,12.2,4.54843302367633));
#250648=CARTESIAN_POINT('Ctrl Pts',(-9.53175348014572,12.2,4.54604512424774));
#250649=CARTESIAN_POINT('Ctrl Pts',(-9.52865391950833,12.2,4.54369162849992));
#250650=CARTESIAN_POINT('Ctrl Pts',(-9.52555435887095,12.2,4.54133813275209));
#250651=CARTESIAN_POINT('Ctrl Pts',(-9.52248257734592,12.2,4.53901904106248));
#250652=CARTESIAN_POINT('Ctrl Pts',(-9.51943929155281,12.2,4.53673435594602));
#250653=CARTESIAN_POINT('Ctrl Pts',(-9.51639600548326,12.2,4.53444967062206));
#250654=CARTESIAN_POINT('Ctrl Pts',(-9.51338121385195,12.2,4.53219939161014));
#250655=CARTESIAN_POINT('Ctrl Pts',(-9.51039564319125,12.2,4.52998352049174));
#250656=CARTESIAN_POINT('Ctrl Pts',(-9.50741007280173,12.2,4.5277676495746));
#250657=CARTESIAN_POINT('Ctrl Pts',(-9.50445372583058,12.2,4.52558618552228));
#250658=CARTESIAN_POINT('Ctrl Pts',(-9.50152734350701,12.2,4.52343912750728));
#250659=CARTESIAN_POINT('Ctrl Pts',(-9.49860096118344,12.2,4.52129206949229));
#250660=CARTESIAN_POINT('Ctrl Pts',(-9.49570454563684,12.2,4.51917941561431));
#250661=CARTESIAN_POINT('Ctrl Pts',(-9.49283885440628,12.2,4.51710116360498));
#250662=CARTESIAN_POINT('Ctrl Pts',(-9.48997316291541,12.2,4.51502291140687));
#250663=CARTESIAN_POINT('Ctrl Pts',(-9.48713819687841,12.2,4.5129790597214));
#250664=CARTESIAN_POINT('Ctrl Pts',(-9.48433473422776,12.2,4.5109695997809));
#250665=CARTESIAN_POINT('Ctrl Pts',(-9.48106402818397,12.2,4.50862523012409));
#250666=CARTESIAN_POINT('Ctrl Pts',(-9.47783619900219,12.2,4.5063276748001));
#250667=CARTESIAN_POINT('Ctrl Pts',(-9.47465251140719,12.2,4.50407691360521));
#250668=CARTESIAN_POINT('Ctrl Pts',(-9.47192363600705,12.2,4.50214768949858));
#250669=CARTESIAN_POINT('Ctrl Pts',(-9.46922719105261,12.2,4.50025284604621));
#250670=CARTESIAN_POINT('Ctrl Pts',(-9.46656399274305,12.2,4.49839236778048));
#250671=CARTESIAN_POINT('Ctrl Pts',(-9.4639007946754,12.2,4.49653188968374));
#250672=CARTESIAN_POINT('Ctrl Pts',(-9.46127084262453,12.2,4.49470577740873));
#250673=CARTESIAN_POINT('Ctrl Pts',(-9.45867497245716,12.2,4.49291401346578));
#250674=CARTESIAN_POINT('Ctrl Pts',(-9.45607910228978,12.2,4.49112224952284));
#250675=CARTESIAN_POINT('Ctrl Pts',(-9.45351731293923,12.2,4.48936483389953));
#250676=CARTESIAN_POINT('Ctrl Pts',(-9.45099045911286,12.2,4.48764174679398));
#250677=CARTESIAN_POINT('Ctrl Pts',(-9.44846360505695,12.2,4.4859186595319));
#250678=CARTESIAN_POINT('Ctrl Pts',(-9.44597168780536,12.2,4.48422990015743));
#250679=CARTESIAN_POINT('Ctrl Pts',(-9.44351558175729,12.2,4.4825754430696));
#250680=CARTESIAN_POINT('Ctrl Pts',(-9.44105947593231,12.2,4.48092098613205));
#250681=CARTESIAN_POINT('Ctrl Pts',(-9.43863918119872,12.2,4.47930083417953));
#250682=CARTESIAN_POINT('Ctrl Pts',(-9.43625559462024,12.2,4.4777149571553));
#250683=CARTESIAN_POINT('Ctrl Pts',(-9.43387200804177,12.2,4.47612908013107));
#250684=CARTESIAN_POINT('Ctrl Pts',(-9.43152513216872,12.2,4.47457748039578));
#250685=CARTESIAN_POINT('Ctrl Pts',(-9.42921588266767,12.2,4.47306012528276));
#250686=CARTESIAN_POINT('Ctrl Pts',(-9.42690663316663,12.2,4.47154277016975));
#250687=CARTESIAN_POINT('Ctrl Pts',(-9.42463501200656,12.2,4.47005965847421));
#250688=CARTESIAN_POINT('Ctrl Pts',(-9.42240196350173,12.2,4.46861075819119));
#250689=CARTESIAN_POINT('Ctrl Pts',(-9.42016891479406,12.2,4.46716185777656));
#250690=CARTESIAN_POINT('Ctrl Pts',(-9.41797443730677,12.2,4.46574716614859));
#250691=CARTESIAN_POINT('Ctrl Pts',(-9.41581950060771,12.2,4.46436664590817));
#250692=CARTESIAN_POINT('Ctrl Pts',(-9.41366456410439,12.2,4.46298612579314));
#250693=CARTESIAN_POINT('Ctrl Pts',(-9.4115491671934,12.2,4.46163977636722));
#250694=CARTESIAN_POINT('Ctrl Pts',(-9.40947430400926,12.2,4.46032755599219));
#250695=CARTESIAN_POINT('Ctrl Pts',(-9.40739944082513,12.2,4.45901533561715));
#250696=CARTESIAN_POINT('Ctrl Pts',(-9.40536511283097,12.2,4.45773724225932));
#250697=CARTESIAN_POINT('Ctrl Pts',(-9.40337233973387,12.2,4.45649323013553));
#250698=CARTESIAN_POINT('Ctrl Pts',(-9.40137956645577,12.2,4.45524921789875));
#250699=CARTESIAN_POINT('Ctrl Pts',(-9.39942834904569,12.2,4.45403928799046));
#250700=CARTESIAN_POINT('Ctrl Pts',(-9.39751973584878,12.2,4.45286338586959));
#250701=CARTESIAN_POINT('Ctrl Pts',(-9.39561112282524,12.2,4.45168748385553));
#250702=CARTESIAN_POINT('Ctrl Pts',(-9.3937451149421,12.2,4.450545611718));
#250703=CARTESIAN_POINT('Ctrl Pts',(-9.3919227912583,12.2,4.44943771350825));
#250704=CARTESIAN_POINT('Ctrl Pts',(-9.3901004675745,12.2,4.4483298152985));
#250705=CARTESIAN_POINT('Ctrl Pts',(-9.38832182911902,12.2,4.44725589135841));
#250706=CARTESIAN_POINT('Ctrl Pts',(-9.38658798534282,12.2,4.44621587909229));
#250707=CARTESIAN_POINT('Ctrl Pts',(-9.38485414140911,12.2,4.4451758667317));
#250708=CARTESIAN_POINT('Ctrl Pts',(-9.38316509182396,12.2,4.44416976661963));
#250709=CARTESIAN_POINT('Ctrl Pts',(-9.38152198207089,12.2,4.44319751515229));
#250710=CARTESIAN_POINT('Ctrl Pts',(-9.37988675819392,12.2,4.44222992987028));
#250711=CARTESIAN_POINT('Ctrl Pts',(-9.37829702764554,12.2,4.44129586542554));
#250712=CARTESIAN_POINT('Ctrl Pts',(-9.37675396800006,12.2,4.44039525799998));
#250713=CARTESIAN_POINT('Ctrl Pts',(-9.37675396800006,15.2,4.44039525799998));
#250714=CARTESIAN_POINT('Ctrl Pts',(-9.37829702764554,15.2,4.44129586542555));
#250715=CARTESIAN_POINT('Ctrl Pts',(-9.3798867581939,15.2,4.44222992987026));
#250716=CARTESIAN_POINT('Ctrl Pts',(-9.38152198207088,15.2,4.44319751515229));
#250717=CARTESIAN_POINT('Ctrl Pts',(-9.38316509182397,15.2,4.44416976661963));
#250718=CARTESIAN_POINT('Ctrl Pts',(-9.3848541414091,15.2,4.44517586673169));
#250719=CARTESIAN_POINT('Ctrl Pts',(-9.38658798534282,15.2,4.44621587909228));
#250720=CARTESIAN_POINT('Ctrl Pts',(-9.38832182911903,15.2,4.44725589135842));
#250721=CARTESIAN_POINT('Ctrl Pts',(-9.39010046757452,15.2,4.44832981529852));
#250722=CARTESIAN_POINT('Ctrl Pts',(-9.39192279125831,15.2,4.44943771350825));
#250723=CARTESIAN_POINT('Ctrl Pts',(-9.39374511494208,15.2,4.45054561171799));
#250724=CARTESIAN_POINT('Ctrl Pts',(-9.39561112282524,15.2,4.45168748385554));
#250725=CARTESIAN_POINT('Ctrl Pts',(-9.39751973584878,15.2,4.45286338586959));
#250726=CARTESIAN_POINT('Ctrl Pts',(-9.39942834904569,15.2,4.45403928799045));
#250727=CARTESIAN_POINT('Ctrl Pts',(-9.40137956645577,15.2,4.45524921789875));
#250728=CARTESIAN_POINT('Ctrl Pts',(-9.40337233973387,15.2,4.45649323013553));
#250729=CARTESIAN_POINT('Ctrl Pts',(-9.40569724162016,15.2,4.45794457757562));
#250730=CARTESIAN_POINT('Ctrl Pts',(-9.40807870360857,15.2,4.45944231251553));
#250731=CARTESIAN_POINT('Ctrl Pts',(-9.41051510879806,15.2,4.4609865103553));
#250732=CARTESIAN_POINT('Ctrl Pts',(-9.41260345634723,15.2,4.46231010865826));
#250733=CARTESIAN_POINT('Ctrl Pts',(-9.41473216945717,15.2,4.46366784207347));
#250734=CARTESIAN_POINT('Ctrl Pts',(-9.41690025999465,15.2,4.46505975415165));
#250735=CARTESIAN_POINT('Ctrl Pts',(-9.41906835033522,15.2,4.4664516661034));
#250736=CARTESIAN_POINT('Ctrl Pts',(-9.42127581723067,15.2,4.46787775468028));
#250737=CARTESIAN_POINT('Ctrl Pts',(-9.42352169774268,15.2,4.46933805896726));
#250738=CARTESIAN_POINT('Ctrl Pts',(-9.42576757825471,15.2,4.47079836325424));
#250739=CARTESIAN_POINT('Ctrl Pts',(-9.42805187253462,15.2,4.47229288560713));
#250740=CARTESIAN_POINT('Ctrl Pts',(-9.43037363836528,15.2,4.47382165671675));
#250741=CARTESIAN_POINT('Ctrl Pts',(-9.43269540440684,15.2,4.47535042796524));
#250742=CARTESIAN_POINT('Ctrl Pts',(-9.43505464471141,15.2,4.47691344918465));
#250743=CARTESIAN_POINT('Ctrl Pts',(-9.43745044351114,15.2,4.47851075244071));
#250744=CARTESIAN_POINT('Ctrl Pts',(-9.43984624209325,15.2,4.48010805555168));
#250745=CARTESIAN_POINT('Ctrl Pts',(-9.4422785964561,15.2,4.4817396391749));
#250746=CARTESIAN_POINT('Ctrl Pts',(-9.44474661536798,15.2,4.48340553036586));
#250747=CARTESIAN_POINT('Ctrl Pts',(-9.44721463427987,15.2,4.48507142155683));
#250748=CARTESIAN_POINT('Ctrl Pts',(-9.44971831756386,15.2,4.48677162025337));
#250749=CARTESIAN_POINT('Ctrl Pts',(-9.45225679338679,15.2,4.48850615118887));
#250750=CARTESIAN_POINT('Ctrl Pts',(-9.45479526920973,15.2,4.49024068212436));
#250751=CARTESIAN_POINT('Ctrl Pts',(-9.45736853522953,15.2,4.49200954390456));
#250752=CARTESIAN_POINT('Ctrl Pts',(-9.45997574396582,15.2,4.49381275783672));
#250753=CARTESIAN_POINT('Ctrl Pts',(-9.46258295293895,15.2,4.49561597193267));
#250754=CARTESIAN_POINT('Ctrl Pts',(-9.46522410139869,15.2,4.49745353707357));
#250755=CARTESIAN_POINT('Ctrl Pts',(-9.46789835887921,15.2,4.49932547109375));
#250756=CARTESIAN_POINT('Ctrl Pts',(-9.47057261611682,15.2,4.5011974049439));
#250757=CARTESIAN_POINT('Ctrl Pts',(-9.47327998429347,15.2,4.50310370639134));
#250758=CARTESIAN_POINT('Ctrl Pts',(-9.47601964760915,15.2,4.50504439040263));
#250759=CARTESIAN_POINT('Ctrl Pts',(-9.47875931092484,15.2,4.50698507441393));
#250760=CARTESIAN_POINT('Ctrl Pts',(-9.48153127183176,15.2,4.50896014002292));
#250761=CARTESIAN_POINT('Ctrl Pts',(-9.48433473422776,15.2,4.5109695997809));
#250762=CARTESIAN_POINT('Ctrl Pts',(-9.48713819687842,15.2,4.5129790597214));
#250763=CARTESIAN_POINT('Ctrl Pts',(-9.48997316291541,15.2,4.51502291140688));
#250764=CARTESIAN_POINT('Ctrl Pts',(-9.49283885440631,15.2,4.517101163605));
#250765=CARTESIAN_POINT('Ctrl Pts',(-9.4957045456369,15.2,4.51917941561435));
#250766=CARTESIAN_POINT('Ctrl Pts',(-9.49860096118346,15.2,4.52129206949231));
#250767=CARTESIAN_POINT('Ctrl Pts',(-9.50152734350701,15.2,4.52343912750729));
#250768=CARTESIAN_POINT('Ctrl Pts',(-9.50445372583056,15.2,4.52558618552227));
#250769=CARTESIAN_POINT('Ctrl Pts',(-9.5074100728017,15.2,4.52776764957458));
#250770=CARTESIAN_POINT('Ctrl Pts',(-9.51039564319125,15.2,4.52998352049174));
#250771=CARTESIAN_POINT('Ctrl Pts',(-9.51338121385199,15.2,4.53219939161017));
#250772=CARTESIAN_POINT('Ctrl Pts',(-9.51639600548326,15.2,4.53444967062205));
#250773=CARTESIAN_POINT('Ctrl Pts',(-9.51943929155281,15.2,4.53673435594603));
#250774=CARTESIAN_POINT('Ctrl Pts',(-9.52248257734592,15.2,4.53901904106248));
#250775=CARTESIAN_POINT('Ctrl Pts',(-9.52555435887099,15.2,4.54133813275212));
#250776=CARTESIAN_POINT('Ctrl Pts',(-9.52865391950834,15.2,4.54369162849992));
#250777=CARTESIAN_POINT('Ctrl Pts',(-9.53175348014569,15.2,4.54604512424771));
#250778=CARTESIAN_POINT('Ctrl Pts',(-9.53488082346189,15.2,4.54843302367636));
#250779=CARTESIAN_POINT('Ctrl Pts',(-9.53803524741992,15.2,4.55085531979068));
#250780=CARTESIAN_POINT('Ctrl Pts',(-9.54066393414713,15.2,4.5528738999593));
#250781=CARTESIAN_POINT('Ctrl Pts',(-9.54331143004896,15.2,4.55491636787731));
#250782=CARTESIAN_POINT('Ctrl Pts',(-9.54597733657577,15.2,4.55698271863993));
#250783=CARTESIAN_POINT('Ctrl Pts',(-9.54864324310257,15.2,4.55904906940256));
#250784=CARTESIAN_POINT('Ctrl Pts',(-9.55132755986875,15.2,4.56113930244082));
#250785=CARTESIAN_POINT('Ctrl Pts',(-9.55402989729839,15.2,4.56325341237013));
#250786=CARTESIAN_POINT('Ctrl Pts',(-9.556732234728,15.2,4.56536752229945));
#250787=CARTESIAN_POINT('Ctrl Pts',(-9.55945259378614,15.2,4.567505509389));
#250788=CARTESIAN_POINT('Ctrl Pts',(-9.56219058879852,15.2,4.56966736523208));
#250789=CARTESIAN_POINT('Ctrl Pts',(-9.5649285838109,15.2,4.57182922107516));
#250790=CARTESIAN_POINT('Ctrl Pts',(-9.56768421505557,15.2,4.57401494726103));
#250791=CARTESIAN_POINT('Ctrl Pts',(-9.57045710595835,15.2,4.57622453552492));
#250792=CARTESIAN_POINT('Ctrl Pts',(-9.57322999686113,15.2,4.57843412378881));
#250793=CARTESIAN_POINT('Ctrl Pts',(-9.57602014704429,15.2,4.58066757327972));
#250794=CARTESIAN_POINT('Ctrl Pts',(-9.57882718525154,15.2,4.58292487502616));
#250795=CARTESIAN_POINT('Ctrl Pts',(-9.58275703880289,15.2,4.58608509752038));
#250796=CARTESIAN_POINT('Ctrl Pts',(-9.58671998870917,15.2,4.58929207286161));
#250797=CARTESIAN_POINT('Ctrl Pts',(-9.5907150381066,15.2,4.59254576955392));
#250798=CARTESIAN_POINT('Ctrl Pts',(-9.59356864477462,15.2,4.59486983858366));
#250799=CARTESIAN_POINT('Ctrl Pts',(-9.59643862780398,15.2,4.59721774655266));
#250800=CARTESIAN_POINT('Ctrl Pts',(-9.59932462961084,15.2,4.59958947981849));
#250801=CARTESIAN_POINT('Ctrl Pts',(-9.60221063110313,15.2,4.6019612128258));
#250802=CARTESIAN_POINT('Ctrl Pts',(-9.60511265215992,15.2,4.60435677266025));
#250803=CARTESIAN_POINT('Ctrl Pts',(-9.6080303396184,15.2,4.60677614565849));
#250804=CARTESIAN_POINT('Ctrl Pts',(-9.6109480273949,15.2,4.60919551892044));
#250805=CARTESIAN_POINT('Ctrl Pts',(-9.61388138179336,15.2,4.61163870707363));
#250806=CARTESIAN_POINT('Ctrl Pts',(-9.61683005463933,15.2,4.61410569366892));
#250807=CARTESIAN_POINT('Ctrl Pts',(-9.6197787274853,15.2,4.61657268026419));
#250808=CARTESIAN_POINT('Ctrl Pts',(-9.62274272011203,15.2,4.61906346794525));
#250809=CARTESIAN_POINT('Ctrl Pts',(-9.62572169116259,15.2,4.62157804049978));
#250810=CARTESIAN_POINT('Ctrl Pts',(-9.62870066221316,15.2,4.62409261305431));
#250811=CARTESIAN_POINT('Ctrl Pts',(-9.63169460858744,15.2,4.62663097110597));
#250812=CARTESIAN_POINT('Ctrl Pts',(-9.63470319629502,15.2,4.62919309929918));
#250813=CARTESIAN_POINT('Ctrl Pts',(-9.63771178400259,15.2,4.63175522749239));
#250814=CARTESIAN_POINT('Ctrl Pts',(-9.64073501212998,15.2,4.63434112531953));
#250815=CARTESIAN_POINT('Ctrl Pts',(-9.64377254830979,15.2,4.63695077684606));
#250816=CARTESIAN_POINT('Ctrl Pts',(-9.64681008448958,15.2,4.63956042837259));
#250817=CARTESIAN_POINT('Ctrl Pts',(-9.64986192876144,15.2,4.64219383236642));
#250818=CARTESIAN_POINT('Ctrl Pts',(-9.65292775556627,15.2,4.64485097305962));
#250819=CARTESIAN_POINT('Ctrl Pts',(-9.6559935823711,15.2,4.64750811375284));
#250820=CARTESIAN_POINT('Ctrl Pts',(-9.65907338836212,15.2,4.65018899106402));
#250821=CARTESIAN_POINT('Ctrl Pts',(-9.66216685372334,15.2,4.65289358600679));
#250822=CARTESIAN_POINT('Ctrl Pts',(-9.66526031908456,15.2,4.65559818094955));
#250823=CARTESIAN_POINT('Ctrl Pts',(-9.6683674429778,15.2,4.65832649205549));
#250824=CARTESIAN_POINT('Ctrl Pts',(-9.67148790749169,15.2,4.66107850420826));
#250825=CARTESIAN_POINT('Ctrl Pts',(-9.67398427923885,15.2,4.66328011405047));
#250826=CARTESIAN_POINT('Ctrl Pts',(-9.67648918842313,15.2,4.66549688995556));
#250827=CARTESIAN_POINT('Ctrl Pts',(-9.67900247489428,15.2,4.66772882335652));
#250828=CARTESIAN_POINT('Ctrl Pts',(-9.681515761023,15.2,4.66996075645338));
#250829=CARTESIAN_POINT('Ctrl Pts',(-9.68403742440756,15.2,4.672207846612));
#250830=CARTESIAN_POINT('Ctrl Pts',(-9.68656730648997,15.2,4.67447008354838));
#250831=CARTESIAN_POINT('Ctrl Pts',(-9.68909718891707,15.2,4.676732320793));
#250832=CARTESIAN_POINT('Ctrl Pts',(-9.69163528862952,15.2,4.67900970358161));
#250833=CARTESIAN_POINT('Ctrl Pts',(-9.694181449158,15.2,4.68130222237477));
#250834=CARTESIAN_POINT('Ctrl Pts',(-9.69672760933955,15.2,4.68359474085557));
#250835=CARTESIAN_POINT('Ctrl Pts',(-9.69928183023395,15.2,4.68590239560939));
#250836=CARTESIAN_POINT('Ctrl Pts',(-9.70184395702398,15.2,4.68822517458518));
#250837=CARTESIAN_POINT('Ctrl Pts',(-9.70568714738355,15.2,4.69170934320709));
#250838=CARTESIAN_POINT('Ctrl Pts',(-9.70954812271937,15.2,4.6952275423941));
#250839=CARTESIAN_POINT('Ctrl Pts',(-9.7134263680773,15.2,4.69877973209607));
#250840=CARTESIAN_POINT('Ctrl Pts',(-9.71601186521744,15.2,4.70114785877916));
#250841=CARTESIAN_POINT('Ctrl Pts',(-9.71860503678607,15.2,4.70353109272755));
#250842=CARTESIAN_POINT('Ctrl Pts',(-9.72120573148336,15.2,4.70592942202492));
#250843=CARTESIAN_POINT('Ctrl Pts',(-9.72380642618065,15.2,4.7083277513223));
#250844=CARTESIAN_POINT('Ctrl Pts',(-9.72641464608994,15.2,4.71074117566034));
#250845=CARTESIAN_POINT('Ctrl Pts',(-9.72903023867769,15.2,4.71316968240533));
#250846=CARTESIAN_POINT('Ctrl Pts',(-9.73295362720292,15.2,4.71681244219195));
#250847=CARTESIAN_POINT('Ctrl Pts',(-9.73689360595874,15.2,4.72048913984397));
#250848=CARTESIAN_POINT('Ctrl Pts',(-9.74084967648236,15.2,4.72419973046063));
#250849=CARTESIAN_POINT('Ctrl Pts',(-9.74348705671167,15.2,4.72667345742605));
#250850=CARTESIAN_POINT('Ctrl Pts',(-9.74613158864511,15.2,4.72916224873846));
#250851=CARTESIAN_POINT('Ctrl Pts',(-9.7487831263165,15.2,4.73166609036555));
#250852=CARTESIAN_POINT('Ctrl Pts',(-9.7520975486767,15.2,4.73479589265528));
#250853=CARTESIAN_POINT('Ctrl Pts',(-9.75542291826356,15.2,4.73794921211305));
#250854=CARTESIAN_POINT('Ctrl Pts',(-9.7587589523878,15.2,4.74112602213122));
#250855=CARTESIAN_POINT('Ctrl Pts',(-9.76142777983264,15.2,4.74366747028427));
#250856=CARTESIAN_POINT('Ctrl Pts',(-9.76410343274775,15.2,4.74622395353028));
#250857=CARTESIAN_POINT('Ctrl Pts',(-9.76678576872771,15.2,4.74879545622696));
#250858=CARTESIAN_POINT('Ctrl Pts',(-9.76946810434219,15.2,4.75136695857326));
#250859=CARTESIAN_POINT('Ctrl Pts',(-9.77215712253867,15.2,4.75395348077768));
#250860=CARTESIAN_POINT('Ctrl Pts',(-9.77485268281764,15.2,4.75655501034124));
#250861=CARTESIAN_POINT('Ctrl Pts',(-9.77754824346387,15.2,4.75915654025926));
#250862=CARTESIAN_POINT('Ctrl Pts',(-9.78025034541972,15.2,4.76177307568519));
#250863=CARTESIAN_POINT('Ctrl Pts',(-9.78295884946855,15.2,4.76440460428506));
#250864=CARTESIAN_POINT('Ctrl Pts',(-9.78566735314835,15.2,4.76703613252638));
#250865=CARTESIAN_POINT('Ctrl Pts',(-9.78838225825046,15.2,4.76968265219224));
#250866=CARTESIAN_POINT('Ctrl Pts',(-9.79110342780512,15.2,4.77234414980644));
#250867=CARTESIAN_POINT('Ctrl Pts',(-9.79382459773054,15.2,4.77500564778328));
#250868=CARTESIAN_POINT('Ctrl Pts',(-9.7965520311705,15.2,4.77768212387824));
#250869=CARTESIAN_POINT('Ctrl Pts',(-9.7992855900417,15.2,4.78037356252493));
#250870=CARTESIAN_POINT('Ctrl Pts',(-9.80270253844448,15.2,4.78373786064993));
#250871=CARTESIAN_POINT('Ctrl Pts',(-9.80612906059742,15.2,4.78712553838071));
#250872=CARTESIAN_POINT('Ctrl Pts',(-9.80956488971024,15.2,4.79053656499345));
#250873=CARTESIAN_POINT('Ctrl Pts',(-9.81300071882306,15.2,4.7939475916062));
#250874=CARTESIAN_POINT('Ctrl Pts',(-9.81644585559219,15.2,4.79738196916389));
#250875=CARTESIAN_POINT('Ctrl Pts',(-9.81990003955099,15.2,4.80083966569287));
#250876=CARTESIAN_POINT('Ctrl Pts',(-9.82266338649212,15.2,4.80360582268993));
#250877=CARTESIAN_POINT('Ctrl Pts',(-9.82543252121545,15.2,4.80638690496179));
#250878=CARTESIAN_POINT('Ctrl Pts',(-9.82820731482136,15.2,4.80918289584279));
#250879=CARTESIAN_POINT('Ctrl Pts',(-9.83306320410427,15.2,4.81407588036073));
#250880=CARTESIAN_POINT('Ctrl Pts',(-9.83793641703867,15.2,4.81901452242558));
#250881=CARTESIAN_POINT('Ctrl Pts',(-9.84282625420647,15.2,4.82399873699799));
#250882=CARTESIAN_POINT('Ctrl Pts',(-9.84701754298989,15.2,4.82827092069546));
#250883=CARTESIAN_POINT('Ctrl Pts',(-9.85122104567787,15.2,4.83257658698693));
#250884=CARTESIAN_POINT('Ctrl Pts',(-9.8554363275239,15.2,4.83691567849363));
#250885=CARTESIAN_POINT('Ctrl Pts',(-9.8589490625232,15.2,4.84053158821392));
#250886=CARTESIAN_POINT('Ctrl Pts',(-9.86246997779467,15.2,4.84417071005058));
#250887=CARTESIAN_POINT('Ctrl Pts',(-9.86599882453013,15.2,4.84783301227091));
#250888=CARTESIAN_POINT('Ctrl Pts',(-9.86882190207234,15.2,4.85076285420684));
#250889=CARTESIAN_POINT('Ctrl Pts',(-9.87165005635413,15.2,4.85370752984939));
#250890=CARTESIAN_POINT('Ctrl Pts',(-9.87448316124364,15.2,4.85666702446861));
#250891=CARTESIAN_POINT('Ctrl Pts',(-9.87731626574712,15.2,4.8596265186846));
#250892=CARTESIAN_POINT('Ctrl Pts',(-9.88015432054869,15.2,4.86260083153209));
#250893=CARTESIAN_POINT('Ctrl Pts',(-9.88299720226023,15.2,4.86558994378622));
#250894=CARTESIAN_POINT('Ctrl Pts',(-9.88726152540856,15.2,4.8700736127783));
#250895=CARTESIAN_POINT('Ctrl Pts',(-9.8915367060163,15.2,4.87459058332362));
#250896=CARTESIAN_POINT('Ctrl Pts',(-9.89582233025032,15.2,4.87914079448973));
#250897=CARTESIAN_POINT('Ctrl Pts',(-9.89867941268372,15.2,4.88217426818715));
#250898=CARTESIAN_POINT('Ctrl Pts',(-9.90154113636733,15.2,4.8852225170903));
#250899=CARTESIAN_POINT('Ctrl Pts',(-9.90440737910916,15.2,4.88828552204722));
#250900=CARTESIAN_POINT('Ctrl Pts',(-9.90799018282933,15.2,4.89211427855635));
#250901=CARTESIAN_POINT('Ctrl Pts',(-9.91158004847632,15.2,4.89596609066453));
#250902=CARTESIAN_POINT('Ctrl Pts',(-9.91517674028152,15.2,4.89984092378832));
#250903=CARTESIAN_POINT('Ctrl Pts',(-9.91805409388249,15.2,4.90294079045629));
#250904=CARTESIAN_POINT('Ctrl Pts',(-9.92093581668955,15.2,4.90605539125659));
#250905=CARTESIAN_POINT('Ctrl Pts',(-9.92382178773601,15.2,4.90918470653923));
#250906=CARTESIAN_POINT('Ctrl Pts',(-9.92670775838926,15.2,4.91231402139548));
#250907=CARTESIAN_POINT('Ctrl Pts',(-9.92959797965857,15.2,4.91545805128225));
#250908=CARTESIAN_POINT('Ctrl Pts',(-9.93249233162174,15.2,4.91861677829165));
#250909=CARTESIAN_POINT('Ctrl Pts',(-9.93538668397927,15.2,4.92177550573144));
#250910=CARTESIAN_POINT('Ctrl Pts',(-9.93828516750391,15.2,4.92494892914987));
#250911=CARTESIAN_POINT('Ctrl Pts',(-9.94118766449569,15.2,4.92813702926903));
#250912=CARTESIAN_POINT('Ctrl Pts',(-9.944090161092,15.2,4.93132512895381));
#250913=CARTESIAN_POINT('Ctrl Pts',(-9.94699667153751,15.2,4.93452790826895));
#250914=CARTESIAN_POINT('Ctrl Pts',(-9.94990707879919,15.2,4.93774534394889));
#250915=CARTESIAN_POINT('Ctrl Pts',(-9.9535450881737,15.2,4.94176713887758));
#250916=CARTESIAN_POINT('Ctrl Pts',(-9.95718918823886,15.2,4.94581183992065));
#250917=CARTESIAN_POINT('Ctrl Pts',(-9.96083915355969,15.2,4.94987940651116));
#250918=CARTESIAN_POINT('Ctrl Pts',(-9.96375912597549,15.2,4.95313345996091));
#250919=CARTESIAN_POINT('Ctrl Pts',(-9.9666828510546,15.2,4.95640214670801));
#250920=CARTESIAN_POINT('Ctrl Pts',(-9.96961021604772,15.2,4.95968544927682));
#250921=CARTESIAN_POINT('Ctrl Pts',(-9.97253758064199,15.2,4.96296875139826));
#250922=CARTESIAN_POINT('Ctrl Pts',(-9.97546858449939,15.2,4.9662666673723));
#250923=CARTESIAN_POINT('Ctrl Pts',(-9.97840311503691,15.2,4.96957917893333));
#250924=CARTESIAN_POINT('Ctrl Pts',(-9.9828049114429,15.2,4.97454794695188));
#250925=CARTESIAN_POINT('Ctrl Pts',(-9.98721464184885,15.2,4.97954955540924));
#250926=CARTESIAN_POINT('Ctrl Pts',(-9.99163192964405,15.2,4.98458393477036));
#250927=CARTESIAN_POINT('Ctrl Pts',(-9.99384057334103,15.2,4.98710112422227));
#250928=CARTESIAN_POINT('Ctrl Pts',(-9.99605110715477,15.2,4.98962650716755));
#250929=CARTESIAN_POINT('Ctrl Pts',(-9.99826348224122,15.2,4.99216007349289));
#250930=CARTESIAN_POINT('Ctrl Pts',(-10.0004758573277,15.2,4.99469363981823));
#250931=CARTESIAN_POINT('Ctrl Pts',(-10.0026900749972,15.2,4.99723539054256));
#250932=CARTESIAN_POINT('Ctrl Pts',(-10.0049060890417,15.2,4.9997853177416));
#250933=CARTESIAN_POINT('Ctrl Pts',(-10.0071221030862,15.2,5.00233524494063));
#250934=CARTESIAN_POINT('Ctrl Pts',(-10.0093399131889,15.2,5.00489334744764));
#250935=CARTESIAN_POINT('Ctrl Pts',(-10.0115594732748,15.2,5.007459617187));
#250936=CARTESIAN_POINT('Ctrl Pts',(-10.0145188869914,15.2,5.01088131048363));
#250937=CARTESIAN_POINT('Ctrl Pts',(-10.0174814111815,15.2,5.0143175234418));
#250938=CARTESIAN_POINT('Ctrl Pts',(-10.0204469377137,15.2,5.01776823552572));
#250939=CARTESIAN_POINT('Ctrl Pts',(-10.0226710824109,15.2,5.02035626935358));
#250940=CARTESIAN_POINT('Ctrl Pts',(-10.0248969161403,15.2,5.02295245807785));
#250941=CARTESIAN_POINT('Ctrl Pts',(-10.0271243932262,15.2,5.02555679381727));
#250942=CARTESIAN_POINT('Ctrl Pts',(-10.0293518703121,15.2,5.0281611295567));
#250943=CARTESIAN_POINT('Ctrl Pts',(-10.0315809903644,15.2,5.03077361197848));
#250944=CARTESIAN_POINT('Ctrl Pts',(-10.0338117084917,15.2,5.03339423225826));
#250945=CARTESIAN_POINT('Ctrl Pts',(-10.036042426619,15.2,5.03601485253804));
#250946=CARTESIAN_POINT('Ctrl Pts',(-10.0382747433379,15.2,5.03864361119251));
#250947=CARTESIAN_POINT('Ctrl Pts',(-10.0405086129649,15.2,5.04128049847098));
#250948=CARTESIAN_POINT('Ctrl Pts',(-10.0427424825919,15.2,5.04391738574945));
#250949=CARTESIAN_POINT('Ctrl Pts',(-10.0449779060203,15.2,5.04656240236814));
#250950=CARTESIAN_POINT('Ctrl Pts',(-10.0472148368423,15.2,5.0492155387367));
#250951=CARTESIAN_POINT('Ctrl Pts',(-10.0494517676643,15.2,5.05186867510526));
#250952=CARTESIAN_POINT('Ctrl Pts',(-10.05169020826,15.2,5.05452993074946));
#250953=CARTESIAN_POINT('Ctrl Pts',(-10.0539301115118,15.2,5.05719929840135));
#250954=CARTESIAN_POINT('Ctrl Pts',(-10.0561700151704,15.2,5.05986866653817));
#250955=CARTESIAN_POINT('Ctrl Pts',(-10.0584113841462,15.2,5.06254614544398));
#250956=CARTESIAN_POINT('Ctrl Pts',(-10.0606541722223,15.2,5.06523172662706));
#250957=CARTESIAN_POINT('Ctrl Pts',(-10.062896959891,15.2,5.06791730732225));
#250958=CARTESIAN_POINT('Ctrl Pts',(-10.065141167843,15.2,5.07061099000869));
#250959=CARTESIAN_POINT('Ctrl Pts',(-10.0673867515115,15.2,5.07331276482789));
#250960=CARTESIAN_POINT('Ctrl Pts',(-10.06963233518,15.2,5.07601453964709));
#250961=CARTESIAN_POINT('Ctrl Pts',(-10.0718792957902,15.2,5.07872440775546));
#250962=CARTESIAN_POINT('Ctrl Pts',(-10.0741275880104,15.2,5.08144235946073));
#250963=CARTESIAN_POINT('Ctrl Pts',(-10.0771253108345,15.2,5.08506629490319));
#250964=CARTESIAN_POINT('Ctrl Pts',(-10.0801254037521,15.2,5.08870460094167));
#250965=CARTESIAN_POINT('Ctrl Pts',(-10.0831277617842,15.2,5.09235725641939));
#250966=CARTESIAN_POINT('Ctrl Pts',(-10.0853795308196,15.2,5.09509674864976));
#250967=CARTESIAN_POINT('Ctrl Pts',(-10.087632574397,15.2,5.09784431188241));
#250968=CARTESIAN_POINT('Ctrl Pts',(-10.0898868499748,15.2,5.10059993711734));
#250969=CARTESIAN_POINT('Ctrl Pts',(-10.0921411251431,15.2,5.10335556185167));
#250970=CARTESIAN_POINT('Ctrl Pts',(-10.0943966327779,15.2,5.10611924865218));
#250971=CARTESIAN_POINT('Ctrl Pts',(-10.0966533284877,15.2,5.10889098830218));
#250972=CARTESIAN_POINT('Ctrl Pts',(-10.0989100241975,15.2,5.1116627279522));
#250973=CARTESIAN_POINT('Ctrl Pts',(-10.1011679099155,15.2,5.11444251941791));
#250974=CARTESIAN_POINT('Ctrl Pts',(-10.103426942,15.2,5.1172303550666));
#250975=CARTESIAN_POINT('Ctrl Pts',(-10.1056859740846,15.2,5.12001819071529));
#250976=CARTESIAN_POINT('Ctrl Pts',(-10.1079461513692,15.2,5.12281406868034));
#250977=CARTESIAN_POINT('Ctrl Pts',(-10.1102074339952,15.2,5.12561798091109));
#250978=CARTESIAN_POINT('Ctrl Pts',(-10.1124687166213,15.2,5.12842189314185));
#250979=CARTESIAN_POINT('Ctrl Pts',(-10.1147311044814,15.2,5.13123383903359));
#250980=CARTESIAN_POINT('Ctrl Pts',(-10.1169945533455,15.2,5.13405380894608));
#250981=CARTESIAN_POINT('Ctrl Pts',(-10.1192580022095,15.2,5.13687377885856));
#250982=CARTESIAN_POINT('Ctrl Pts',(-10.1215225143386,15.2,5.13970177361916));
#250983=CARTESIAN_POINT('Ctrl Pts',(-10.1237880465062,15.2,5.14253778234835));
#250984=CARTESIAN_POINT('Ctrl Pts',(-10.1260535790853,15.2,5.14537379159274));
#250985=CARTESIAN_POINT('Ctrl Pts',(-10.1283201314313,15.2,5.14821781543941));
#250986=CARTESIAN_POINT('Ctrl Pts',(-10.1305876639694,15.2,5.15106984464669));
#250987=CARTESIAN_POINT('Ctrl Pts',(-10.1328551960955,15.2,5.15392187333584));
#250988=CARTESIAN_POINT('Ctrl Pts',(-10.1351237080632,15.2,5.15678190708287));
#250989=CARTESIAN_POINT('Ctrl Pts',(-10.1373931562724,15.2,5.15964993581269));
#250990=CARTESIAN_POINT('Ctrl Pts',(-10.1396626044817,15.2,5.16251796454251));
#250991=CARTESIAN_POINT('Ctrl Pts',(-10.141932990441,15.2,5.16539398774421));
#250992=CARTESIAN_POINT('Ctrl Pts',(-10.1442042744938,15.2,5.16827799744422));
#250993=CARTESIAN_POINT('Ctrl Pts',(-10.1464755585466,15.2,5.17116200714423));
#250994=CARTESIAN_POINT('Ctrl Pts',(-10.1487477383869,15.2,5.17405400273952));
#250995=CARTESIAN_POINT('Ctrl Pts',(-10.151020774523,15.2,5.17695397348064));
#250996=CARTESIAN_POINT('Ctrl Pts',(-10.1548091682208,15.2,5.18178725822477));
#250997=CARTESIAN_POINT('Ctrl Pts',(-10.1585999375556,15.2,5.1866426993944));
#250998=CARTESIAN_POINT('Ctrl Pts',(-10.1623928995001,15.2,5.19152024828326));
#250999=CARTESIAN_POINT('Ctrl Pts',(-10.164668676584,15.2,5.19444677751025));
#251000=CARTESIAN_POINT('Ctrl Pts',(-10.1669452418846,15.2,5.19738126598694));
#251001=CARTESIAN_POINT('Ctrl Pts',(-10.1692225565102,15.2,5.200323704671));
#251002=CARTESIAN_POINT('Ctrl Pts',(-10.1714998711357,15.2,5.20326614335507));
#251003=CARTESIAN_POINT('Ctrl Pts',(-10.1737779343449,15.2,5.20621653165492));
#251004=CARTESIAN_POINT('Ctrl Pts',(-10.1760567055425,15.2,5.20917485944431));
#251005=CARTESIAN_POINT('Ctrl Pts',(-10.1783354767401,15.2,5.21213318723369));
#251006=CARTESIAN_POINT('Ctrl Pts',(-10.1806149537859,15.2,5.21509945337738));
#251007=CARTESIAN_POINT('Ctrl Pts',(-10.1828950989946,15.2,5.21807364864323));
#251008=CARTESIAN_POINT('Ctrl Pts',(-10.1851752446176,15.2,5.2210478444494));
#251009=CARTESIAN_POINT('Ctrl Pts',(-10.1874560588324,15.2,5.22402997029947));
#251010=CARTESIAN_POINT('Ctrl Pts',(-10.1897375045391,15.2,5.22702001565178));
#251011=CARTESIAN_POINT('Ctrl Pts',(-10.1920189498313,15.2,5.23001006046089));
#251012=CARTESIAN_POINT('Ctrl Pts',(-10.1943010283817,15.2,5.23300802638621));
#251013=CARTESIAN_POINT('Ctrl Pts',(-10.1965836989655,15.2,5.23601390156937));
#251014=CARTESIAN_POINT('Ctrl Pts',(-10.1988663695493,15.2,5.23901977675254));
#251015=CARTESIAN_POINT('Ctrl Pts',(-10.2011496313747,15.2,5.24203356109871));
#251016=CARTESIAN_POINT('Ctrl Pts',(-10.2034334355105,15.2,5.24505524325268));
#251017=CARTESIAN_POINT('Ctrl Pts',(-10.2064785075531,15.2,5.24908415260831));
#251018=CARTESIAN_POINT('Ctrl Pts',(-10.2095245385816,15.2,5.25312709922805));
#251019=CARTESIAN_POINT('Ctrl Pts',(-10.2125714572769,15.2,5.25718406539495));
#251020=CARTESIAN_POINT('Ctrl Pts',(-10.2156183763873,15.2,5.2612410321146));
#251021=CARTESIAN_POINT('Ctrl Pts',(-10.2186661838359,15.2,5.26531201788687));
#251022=CARTESIAN_POINT('Ctrl Pts',(-10.2217148780001,15.2,5.26939701899998));
#251023=CARTESIAN_POINT('Ctrl Pts',(-8.88241603300006,15.2,5.36127880599999));
#251024=CARTESIAN_POINT('Ctrl Pts',(-8.88241603300006,11.6,5.36127880599999));
#251025=CARTESIAN_POINT('Ctrl Pts',(-8.88257249800006,15.2,5.36135574399999));
#251026=CARTESIAN_POINT('Ctrl Pts',(-8.88257249800006,11.6,5.36135574399999));
#251027=CARTESIAN_POINT('Ctrl Pts',(-8.88289093000006,15.2,5.36151222999998));
#251028=CARTESIAN_POINT('Ctrl Pts',(-8.88289093000006,11.6,5.36151222999998));
#251029=CARTESIAN_POINT('Ctrl Pts',(-8.88337354800005,15.2,5.36174910399998));
#251030=CARTESIAN_POINT('Ctrl Pts',(-8.88337354800005,11.6,5.36174910399998));
#251031=CARTESIAN_POINT('Ctrl Pts',(-8.88402391700006,15.2,5.36206771099998));
#251032=CARTESIAN_POINT('Ctrl Pts',(-8.88402391700006,11.6,5.36206771099998));
#251033=CARTESIAN_POINT('Ctrl Pts',(-8.88484693900006,15.2,5.36246988099998));
#251034=CARTESIAN_POINT('Ctrl Pts',(-8.88484693900006,11.6,5.36246988099998));
#251035=CARTESIAN_POINT('Ctrl Pts',(-8.88568370900006,15.2,5.36287772799999));
#251036=CARTESIAN_POINT('Ctrl Pts',(-8.88568370900006,11.6,5.36287772799999));
#251037=CARTESIAN_POINT('Ctrl Pts',(-8.88652944600006,15.2,5.36328889699998));
#251038=CARTESIAN_POINT('Ctrl Pts',(-8.88652944600006,11.6,5.36328889699998));
#251039=CARTESIAN_POINT('Ctrl Pts',(-8.88738413200005,15.2,5.36370335799998));
#251040=CARTESIAN_POINT('Ctrl Pts',(-8.88738413200005,11.6,5.36370335799998));
#251041=CARTESIAN_POINT('Ctrl Pts',(-8.88824775000005,15.2,5.36412108299999));
#251042=CARTESIAN_POINT('Ctrl Pts',(-8.88824775000005,11.6,5.36412108299999));
#251043=CARTESIAN_POINT('Ctrl Pts',(-8.88912028500006,15.2,5.36454204499999));
#251044=CARTESIAN_POINT('Ctrl Pts',(-8.88912028500006,11.6,5.36454204499999));
#251045=CARTESIAN_POINT('Ctrl Pts',(-8.89000172000006,15.2,5.36496621499998));
#251046=CARTESIAN_POINT('Ctrl Pts',(-8.89000172000006,11.6,5.36496621499998));
#251047=CARTESIAN_POINT('Ctrl Pts',(-8.89089204000006,15.2,5.36539356699999));
#251048=CARTESIAN_POINT('Ctrl Pts',(-8.89089204000006,11.6,5.36539356699999));
#251049=CARTESIAN_POINT('Ctrl Pts',(-8.89179122800006,15.2,5.36582407199998));
#251050=CARTESIAN_POINT('Ctrl Pts',(-8.89179122800006,11.6,5.36582407199998));
#251051=CARTESIAN_POINT('Ctrl Pts',(-8.89269926800005,15.2,5.36625770499998));
#251052=CARTESIAN_POINT('Ctrl Pts',(-8.89269926800005,11.6,5.36625770499998));
#251053=CARTESIAN_POINT('Ctrl Pts',(-8.89361614600006,15.2,5.36669443599998));
#251054=CARTESIAN_POINT('Ctrl Pts',(-8.89361614600006,11.6,5.36669443599998));
#251055=CARTESIAN_POINT('Ctrl Pts',(-8.89454184300006,15.2,5.36713423999998));
#251056=CARTESIAN_POINT('Ctrl Pts',(-8.89454184300006,11.6,5.36713423999998));
#251057=CARTESIAN_POINT('Ctrl Pts',(-8.89547634600006,15.2,5.36757709099999));
#251058=CARTESIAN_POINT('Ctrl Pts',(-8.89547634600006,11.6,5.36757709099999));
#251059=CARTESIAN_POINT('Ctrl Pts',(-8.89641963900005,15.2,5.36802295899999));
#251060=CARTESIAN_POINT('Ctrl Pts',(-8.89641963900005,11.6,5.36802295899999));
#251061=CARTESIAN_POINT('Ctrl Pts',(-8.89737170500006,15.2,5.36847181999998));
#251062=CARTESIAN_POINT('Ctrl Pts',(-8.89737170500006,11.6,5.36847181999998));
#251063=CARTESIAN_POINT('Ctrl Pts',(-8.89833252800006,15.2,5.36892364599999));
#251064=CARTESIAN_POINT('Ctrl Pts',(-8.89833252800006,11.6,5.36892364599999));
#251065=CARTESIAN_POINT('Ctrl Pts',(-8.89930209500006,15.2,5.36937841199999));
#251066=CARTESIAN_POINT('Ctrl Pts',(-8.89930209500006,11.6,5.36937841199999));
#251067=CARTESIAN_POINT('Ctrl Pts',(-8.90028038900006,15.2,5.36983609199999));
#251068=CARTESIAN_POINT('Ctrl Pts',(-8.90028038900006,11.6,5.36983609199999));
#251069=CARTESIAN_POINT('Ctrl Pts',(-8.90126739500005,15.2,5.37029665799999));
#251070=CARTESIAN_POINT('Ctrl Pts',(-8.90126739500005,11.6,5.37029665799999));
#251071=CARTESIAN_POINT('Ctrl Pts',(-8.90226309800006,15.2,5.37076008699999));
#251072=CARTESIAN_POINT('Ctrl Pts',(-8.90226309800006,11.6,5.37076008699999));
#251073=CARTESIAN_POINT('Ctrl Pts',(-8.90326748200006,15.2,5.37122635099998));
#251074=CARTESIAN_POINT('Ctrl Pts',(-8.90326748200006,11.6,5.37122635099998));
#251075=CARTESIAN_POINT('Ctrl Pts',(-8.90428053200005,15.2,5.37169542499999));
#251076=CARTESIAN_POINT('Ctrl Pts',(-8.90428053200005,11.6,5.37169542499999));
#251077=CARTESIAN_POINT('Ctrl Pts',(-8.90530223300006,15.2,5.37216728299998));
#251078=CARTESIAN_POINT('Ctrl Pts',(-8.90530223300006,11.6,5.37216728299998));
#251079=CARTESIAN_POINT('Ctrl Pts',(-8.90633257000006,15.2,5.37264189999998));
#251080=CARTESIAN_POINT('Ctrl Pts',(-8.90633257000006,11.6,5.37264189999998));
#251081=CARTESIAN_POINT('Ctrl Pts',(-8.90737152800006,15.2,5.37311925099999));
#251082=CARTESIAN_POINT('Ctrl Pts',(-8.90737152800006,11.6,5.37311925099999));
#251083=CARTESIAN_POINT('Ctrl Pts',(-8.90841909200006,15.2,5.37359930999998));
#251084=CARTESIAN_POINT('Ctrl Pts',(-8.90841909200006,11.6,5.37359930999998));
#251085=CARTESIAN_POINT('Ctrl Pts',(-8.90947524800006,15.2,5.37408205399998));
#251086=CARTESIAN_POINT('Ctrl Pts',(-8.90947524800006,11.6,5.37408205399998));
#251087=CARTESIAN_POINT('Ctrl Pts',(-8.91053997900006,15.2,5.37456745499998));
#251088=CARTESIAN_POINT('Ctrl Pts',(-8.91053997900006,11.6,5.37456745499998));
#251089=CARTESIAN_POINT('Ctrl Pts',(-8.91161327100006,15.2,5.37505549099999));
#251090=CARTESIAN_POINT('Ctrl Pts',(-8.91161327100006,11.6,5.37505549099999));
#251091=CARTESIAN_POINT('Ctrl Pts',(-8.91269511200005,15.2,5.37554613499999));
#251092=CARTESIAN_POINT('Ctrl Pts',(-8.91269511200005,11.6,5.37554613499999));
#251093=CARTESIAN_POINT('Ctrl Pts',(-8.91378548400005,15.2,5.37603936499998));
#251094=CARTESIAN_POINT('Ctrl Pts',(-8.91378548400005,11.6,5.37603936499998));
#251095=CARTESIAN_POINT('Ctrl Pts',(-8.91488437300006,15.2,5.37653515499999));
#251096=CARTESIAN_POINT('Ctrl Pts',(-8.91488437300006,11.6,5.37653515499999));
#251097=CARTESIAN_POINT('Ctrl Pts',(-8.91599176500005,15.2,5.37703347999998));
#251098=CARTESIAN_POINT('Ctrl Pts',(-8.91599176500005,11.6,5.37703347999998));
#251099=CARTESIAN_POINT('Ctrl Pts',(-8.91710764600005,15.2,5.37753431799998));
#251100=CARTESIAN_POINT('Ctrl Pts',(-8.91710764600005,11.6,5.37753431799998));
#251101=CARTESIAN_POINT('Ctrl Pts',(-8.91823200100006,15.2,5.37803764299999));
#251102=CARTESIAN_POINT('Ctrl Pts',(-8.91823200100006,11.6,5.37803764299999));
#251103=CARTESIAN_POINT('Ctrl Pts',(-8.91936481600006,15.2,5.37854343099998));
#251104=CARTESIAN_POINT('Ctrl Pts',(-8.91936481600006,11.6,5.37854343099998));
#251105=CARTESIAN_POINT('Ctrl Pts',(-8.92050607600006,15.2,5.37905165999998));
#251106=CARTESIAN_POINT('Ctrl Pts',(-8.92050607600006,11.6,5.37905165999998));
#251107=CARTESIAN_POINT('Ctrl Pts',(-8.92165576600006,15.2,5.37956230499999));
#251108=CARTESIAN_POINT('Ctrl Pts',(-8.92165576600006,11.6,5.37956230499999));
#251109=CARTESIAN_POINT('Ctrl Pts',(-8.92281387300006,15.2,5.38007534099999));
#251110=CARTESIAN_POINT('Ctrl Pts',(-8.92281387300006,11.6,5.38007534099999));
#251111=CARTESIAN_POINT('Ctrl Pts',(-8.92398038300006,15.2,5.38059074799998));
#251112=CARTESIAN_POINT('Ctrl Pts',(-8.92398038300006,11.6,5.38059074799998));
#251113=CARTESIAN_POINT('Ctrl Pts',(-8.92515528200006,15.2,5.38110849999998));
#251114=CARTESIAN_POINT('Ctrl Pts',(-8.92515528200006,11.6,5.38110849999998));
#251115=CARTESIAN_POINT('Ctrl Pts',(-8.92633855400006,15.2,5.38162857399998));
#251116=CARTESIAN_POINT('Ctrl Pts',(-8.92633855400006,11.6,5.38162857399998));
#251117=CARTESIAN_POINT('Ctrl Pts',(-8.92753018700006,15.2,5.38215094799998));
#251118=CARTESIAN_POINT('Ctrl Pts',(-8.92753018700006,11.6,5.38215094799998));
#251119=CARTESIAN_POINT('Ctrl Pts',(-8.92873016600005,15.2,5.38267559699998));
#251120=CARTESIAN_POINT('Ctrl Pts',(-8.92873016600005,11.6,5.38267559699998));
#251121=CARTESIAN_POINT('Ctrl Pts',(-8.92993847700006,15.2,5.38320249899999));
#251122=CARTESIAN_POINT('Ctrl Pts',(-8.92993847700006,11.6,5.38320249899999));
#251123=CARTESIAN_POINT('Ctrl Pts',(-8.93115510700006,15.2,5.38373163199999));
#251124=CARTESIAN_POINT('Ctrl Pts',(-8.93115510700006,11.6,5.38373163199999));
#251125=CARTESIAN_POINT('Ctrl Pts',(-8.93238004200006,15.2,5.38426297199998));
#251126=CARTESIAN_POINT('Ctrl Pts',(-8.93238004200006,11.6,5.38426297199998));
#251127=CARTESIAN_POINT('Ctrl Pts',(-8.93361326800006,15.2,5.38479649699998));
#251128=CARTESIAN_POINT('Ctrl Pts',(-8.93361326800006,11.6,5.38479649699998));
#251129=CARTESIAN_POINT('Ctrl Pts',(-8.93485477100005,15.2,5.38533218399999));
#251130=CARTESIAN_POINT('Ctrl Pts',(-8.93485477100005,11.6,5.38533218399999));
#251131=CARTESIAN_POINT('Ctrl Pts',(-8.93610453600006,15.2,5.38587001099998));
#251132=CARTESIAN_POINT('Ctrl Pts',(-8.93610453600006,11.6,5.38587001099998));
#251133=CARTESIAN_POINT('Ctrl Pts',(-8.93736255200006,15.2,5.38640995599999));
#251134=CARTESIAN_POINT('Ctrl Pts',(-8.93736255200006,11.6,5.38640995599999));
#251135=CARTESIAN_POINT('Ctrl Pts',(-8.93862880300006,15.2,5.38695199699998));
#251136=CARTESIAN_POINT('Ctrl Pts',(-8.93862880300006,11.6,5.38695199699998));
#251137=CARTESIAN_POINT('Ctrl Pts',(-8.93990327800006,15.2,5.38749611099998));
#251138=CARTESIAN_POINT('Ctrl Pts',(-8.93990327800006,11.6,5.38749611099998));
#251139=CARTESIAN_POINT('Ctrl Pts',(-8.94118596100006,15.2,5.38804227499998));
#251140=CARTESIAN_POINT('Ctrl Pts',(-8.94118596100006,11.6,5.38804227499998));
#251141=CARTESIAN_POINT('Ctrl Pts',(-8.94247684000005,15.2,5.38859046999999));
#251142=CARTESIAN_POINT('Ctrl Pts',(-8.94247684000005,11.6,5.38859046999999));
#251143=CARTESIAN_POINT('Ctrl Pts',(-8.94377590200006,15.2,5.38914067099999));
#251144=CARTESIAN_POINT('Ctrl Pts',(-8.94377590200006,11.6,5.38914067099999));
#251145=CARTESIAN_POINT('Ctrl Pts',(-8.94508313100006,15.2,5.38969285799999));
#251146=CARTESIAN_POINT('Ctrl Pts',(-8.94508313100006,11.6,5.38969285799999));
#251147=CARTESIAN_POINT('Ctrl Pts',(-8.94639851700006,15.2,5.39024700899999));
#251148=CARTESIAN_POINT('Ctrl Pts',(-8.94639851700006,11.6,5.39024700899999));
#251149=CARTESIAN_POINT('Ctrl Pts',(-8.94772204500006,15.2,5.39080310299998));
#251150=CARTESIAN_POINT('Ctrl Pts',(-8.94772204500006,11.6,5.39080310299998));
#251151=CARTESIAN_POINT('Ctrl Pts',(-8.94905370100006,15.2,5.39136111899998));
#251152=CARTESIAN_POINT('Ctrl Pts',(-8.94905370100006,11.6,5.39136111899998));
#251153=CARTESIAN_POINT('Ctrl Pts',(-8.95039347300006,15.2,5.39192103299998));
#251154=CARTESIAN_POINT('Ctrl Pts',(-8.95039347300006,11.6,5.39192103299998));
#251155=CARTESIAN_POINT('Ctrl Pts',(-8.95174134800006,15.2,5.39248282599999));
#251156=CARTESIAN_POINT('Ctrl Pts',(-8.95174134800006,11.6,5.39248282599999));
#251157=CARTESIAN_POINT('Ctrl Pts',(-8.95309731300006,15.2,5.39304647699999));
#251158=CARTESIAN_POINT('Ctrl Pts',(-8.95309731300006,11.6,5.39304647699999));
#251159=CARTESIAN_POINT('Ctrl Pts',(-8.95446135400006,15.2,5.39361196399998));
#251160=CARTESIAN_POINT('Ctrl Pts',(-8.95446135400006,11.6,5.39361196399998));
#251161=CARTESIAN_POINT('Ctrl Pts',(-8.95583345800006,15.2,5.39417926699999));
#251162=CARTESIAN_POINT('Ctrl Pts',(-8.95583345800006,11.6,5.39417926699999));
#251163=CARTESIAN_POINT('Ctrl Pts',(-8.95721361300006,15.2,5.39474836399998));
#251164=CARTESIAN_POINT('Ctrl Pts',(-8.95721361300006,11.6,5.39474836399998));
#251165=CARTESIAN_POINT('Ctrl Pts',(-8.95860180400006,15.2,5.39531923399998));
#251166=CARTESIAN_POINT('Ctrl Pts',(-8.95860180400006,11.6,5.39531923399998));
#251167=CARTESIAN_POINT('Ctrl Pts',(-8.95999802100006,15.2,5.39589185899998));
#251168=CARTESIAN_POINT('Ctrl Pts',(-8.95999802100006,11.6,5.39589185899998));
#251169=CARTESIAN_POINT('Ctrl Pts',(-8.96140225000006,15.2,5.39646621499998));
#251170=CARTESIAN_POINT('Ctrl Pts',(-8.96140225000006,11.6,5.39646621499998));
#251171=CARTESIAN_POINT('Ctrl Pts',(-8.96281447700006,15.2,5.39704228299998));
#251172=CARTESIAN_POINT('Ctrl Pts',(-8.96281447700006,11.6,5.39704228299998));
#251173=CARTESIAN_POINT('Ctrl Pts',(-8.96423469000006,15.2,5.39762004299998));
#251174=CARTESIAN_POINT('Ctrl Pts',(-8.96423469000006,11.6,5.39762004299998));
#251175=CARTESIAN_POINT('Ctrl Pts',(-8.96566287700006,15.2,5.39819947399998));
#251176=CARTESIAN_POINT('Ctrl Pts',(-8.96566287700006,11.6,5.39819947399998));
#251177=CARTESIAN_POINT('Ctrl Pts',(-8.96709902400006,15.2,5.39878055599999));
#251178=CARTESIAN_POINT('Ctrl Pts',(-8.96709902400006,11.6,5.39878055599999));
#251179=CARTESIAN_POINT('Ctrl Pts',(-8.96854312000006,15.2,5.39936326899999));
#251180=CARTESIAN_POINT('Ctrl Pts',(-8.96854312000006,11.6,5.39936326899999));
#251181=CARTESIAN_POINT('Ctrl Pts',(-8.96999515100006,15.2,5.39994759299999));
#251182=CARTESIAN_POINT('Ctrl Pts',(-8.96999515100006,11.6,5.39994759299999));
#251183=CARTESIAN_POINT('Ctrl Pts',(-8.97145510400006,15.2,5.40053350699999));
#251184=CARTESIAN_POINT('Ctrl Pts',(-8.97145510400006,11.6,5.40053350699999));
#251185=CARTESIAN_POINT('Ctrl Pts',(-8.97292296700006,15.2,5.40112099299999));
#251186=CARTESIAN_POINT('Ctrl Pts',(-8.97292296700006,11.6,5.40112099299999));
#251187=CARTESIAN_POINT('Ctrl Pts',(-8.97439872900006,15.2,5.40171002899999));
#251188=CARTESIAN_POINT('Ctrl Pts',(-8.97439872900006,11.6,5.40171002899999));
#251189=CARTESIAN_POINT('Ctrl Pts',(-8.97588237600005,15.2,5.40230059799998));
#251190=CARTESIAN_POINT('Ctrl Pts',(-8.97588237600005,11.6,5.40230059799998));
#251191=CARTESIAN_POINT('Ctrl Pts',(-8.97737389600006,15.2,5.40289267699999));
#251192=CARTESIAN_POINT('Ctrl Pts',(-8.97737389600006,11.6,5.40289267699999));
#251193=CARTESIAN_POINT('Ctrl Pts',(-8.97887327600005,15.2,5.40348624899998));
#251194=CARTESIAN_POINT('Ctrl Pts',(-8.97887327600005,11.6,5.40348624899998));
#251195=CARTESIAN_POINT('Ctrl Pts',(-8.98038050400006,15.2,5.40408129299998));
#251196=CARTESIAN_POINT('Ctrl Pts',(-8.98038050400006,11.6,5.40408129299998));
#251197=CARTESIAN_POINT('Ctrl Pts',(-8.98189556800006,15.2,5.40467779099998));
#251198=CARTESIAN_POINT('Ctrl Pts',(-8.98189556800006,11.6,5.40467779099998));
#251199=CARTESIAN_POINT('Ctrl Pts',(-8.98341845500006,15.2,5.40527572299998));
#251200=CARTESIAN_POINT('Ctrl Pts',(-8.98341845500006,11.6,5.40527572299998));
#251201=CARTESIAN_POINT('Ctrl Pts',(-8.98494915400006,15.2,5.40587506999999));
#251202=CARTESIAN_POINT('Ctrl Pts',(-8.98494915400006,11.6,5.40587506999999));
#251203=CARTESIAN_POINT('Ctrl Pts',(-8.98648765200005,15.2,5.40647581199998));
#251204=CARTESIAN_POINT('Ctrl Pts',(-8.98648765200005,11.6,5.40647581199998));
#251205=CARTESIAN_POINT('Ctrl Pts',(-8.98803393600006,15.2,5.40707793199999));
#251206=CARTESIAN_POINT('Ctrl Pts',(-8.98803393600006,11.6,5.40707793199999));
#251207=CARTESIAN_POINT('Ctrl Pts',(-8.98958799600006,15.2,5.40768140799998));
#251208=CARTESIAN_POINT('Ctrl Pts',(-8.98958799600006,11.6,5.40768140799998));
#251209=CARTESIAN_POINT('Ctrl Pts',(-8.99114981800006,15.2,5.40828622299999));
#251210=CARTESIAN_POINT('Ctrl Pts',(-8.99114981800006,11.6,5.40828622299999));
#251211=CARTESIAN_POINT('Ctrl Pts',(-8.99271939000006,15.2,5.40889235799998));
#251212=CARTESIAN_POINT('Ctrl Pts',(-8.99271939000006,11.6,5.40889235799998));
#251213=CARTESIAN_POINT('Ctrl Pts',(-8.99429670100006,15.2,5.40949979499998));
#251214=CARTESIAN_POINT('Ctrl Pts',(-8.99429670100006,11.6,5.40949979499998));
#251215=CARTESIAN_POINT('Ctrl Pts',(-8.99588173900005,15.2,5.41010851499999));
#251216=CARTESIAN_POINT('Ctrl Pts',(-8.99588173900005,11.6,5.41010851499999));
#251217=CARTESIAN_POINT('Ctrl Pts',(-8.99747449100006,15.2,5.41071849699998));
#251218=CARTESIAN_POINT('Ctrl Pts',(-8.99747449100006,11.6,5.41071849699998));
#251219=CARTESIAN_POINT('Ctrl Pts',(-8.99907494600006,15.2,5.41132972599998));
#251220=CARTESIAN_POINT('Ctrl Pts',(-8.99907494600006,11.6,5.41132972599998));
#251221=CARTESIAN_POINT('Ctrl Pts',(-9.00068309100006,15.2,5.41194217999998));
#251222=CARTESIAN_POINT('Ctrl Pts',(-9.00068309100006,11.6,5.41194217999998));
#251223=CARTESIAN_POINT('Ctrl Pts',(-9.00229891600006,15.2,5.41255584399998));
#251224=CARTESIAN_POINT('Ctrl Pts',(-9.00229891600006,11.6,5.41255584399998));
#251225=CARTESIAN_POINT('Ctrl Pts',(-9.00392240700005,15.2,5.41317069799998));
#251226=CARTESIAN_POINT('Ctrl Pts',(-9.00392240700005,11.6,5.41317069799998));
#251227=CARTESIAN_POINT('Ctrl Pts',(-9.00555355400006,15.2,5.41378672399999));
#251228=CARTESIAN_POINT('Ctrl Pts',(-9.00555355400006,11.6,5.41378672399999));
#251229=CARTESIAN_POINT('Ctrl Pts',(-9.00719234500006,15.2,5.41440390399998));
#251230=CARTESIAN_POINT('Ctrl Pts',(-9.00719234500006,11.6,5.41440390399998));
#251231=CARTESIAN_POINT('Ctrl Pts',(-9.00883876700006,15.2,5.41502221999998));
#251232=CARTESIAN_POINT('Ctrl Pts',(-9.00883876700006,11.6,5.41502221999998));
#251233=CARTESIAN_POINT('Ctrl Pts',(-9.01049280800006,15.2,5.41564165399999));
#251234=CARTESIAN_POINT('Ctrl Pts',(-9.01049280800006,11.6,5.41564165399999));
#251235=CARTESIAN_POINT('Ctrl Pts',(-9.01215445900006,15.2,5.41626218699999));
#251236=CARTESIAN_POINT('Ctrl Pts',(-9.01215445900006,11.6,5.41626218699999));
#251237=CARTESIAN_POINT('Ctrl Pts',(-9.01382370600006,15.2,5.41688380299998));
#251238=CARTESIAN_POINT('Ctrl Pts',(-9.01382370600006,11.6,5.41688380299998));
#251239=CARTESIAN_POINT('Ctrl Pts',(-9.01550053900005,15.2,5.41750648399999));
#251240=CARTESIAN_POINT('Ctrl Pts',(-9.01550053900005,11.6,5.41750648399999));
#251241=CARTESIAN_POINT('Ctrl Pts',(-9.01718494500006,15.2,5.41813020999999));
#251242=CARTESIAN_POINT('Ctrl Pts',(-9.01718494500006,11.6,5.41813020999999));
#251243=CARTESIAN_POINT('Ctrl Pts',(-9.01887691300006,15.2,5.41875496599998));
#251244=CARTESIAN_POINT('Ctrl Pts',(-9.01887691300006,11.6,5.41875496599998));
#251245=CARTESIAN_POINT('Ctrl Pts',(-9.02057643200006,15.2,5.41938073299999));
#251246=CARTESIAN_POINT('Ctrl Pts',(-9.02057643200006,11.6,5.41938073299999));
#251247=CARTESIAN_POINT('Ctrl Pts',(-9.02228349000006,15.2,5.42000749399998));
#251248=CARTESIAN_POINT('Ctrl Pts',(-9.02228349000006,11.6,5.42000749399998));
#251249=CARTESIAN_POINT('Ctrl Pts',(-9.02399807600006,15.2,5.42063523199998));
#251250=CARTESIAN_POINT('Ctrl Pts',(-9.02399807600006,11.6,5.42063523199998));
#251251=CARTESIAN_POINT('Ctrl Pts',(-9.02572017800006,15.2,5.42126392899998));
#251252=CARTESIAN_POINT('Ctrl Pts',(-9.02572017800006,11.6,5.42126392899998));
#251253=CARTESIAN_POINT('Ctrl Pts',(-9.02744978400005,15.2,5.42189356799998));
#251254=CARTESIAN_POINT('Ctrl Pts',(-9.02744978400005,11.6,5.42189356799998));
#251255=CARTESIAN_POINT('Ctrl Pts',(-9.02918688400005,15.2,5.42252413099998));
#251256=CARTESIAN_POINT('Ctrl Pts',(-9.02918688400005,11.6,5.42252413099998));
#251257=CARTESIAN_POINT('Ctrl Pts',(-9.03093146700006,15.2,5.42315560199999));
#251258=CARTESIAN_POINT('Ctrl Pts',(-9.03093146700006,11.6,5.42315560199999));
#251259=CARTESIAN_POINT('Ctrl Pts',(-9.03268352000006,15.2,5.42378796399999));
#251260=CARTESIAN_POINT('Ctrl Pts',(-9.03268352000006,11.6,5.42378796399999));
#251261=CARTESIAN_POINT('Ctrl Pts',(-9.03444303300006,15.2,5.42442119899999));
#251262=CARTESIAN_POINT('Ctrl Pts',(-9.03444303300006,11.6,5.42442119899999));
#251263=CARTESIAN_POINT('Ctrl Pts',(-9.03620999400006,15.2,5.42505528999998));
#251264=CARTESIAN_POINT('Ctrl Pts',(-9.03620999400006,11.6,5.42505528999998));
#251265=CARTESIAN_POINT('Ctrl Pts',(-9.03798439200006,15.2,5.42569022099999));
#251266=CARTESIAN_POINT('Ctrl Pts',(-9.03798439200006,11.6,5.42569022099999));
#251267=CARTESIAN_POINT('Ctrl Pts',(-9.03976621700006,15.2,5.42632597599999));
#251268=CARTESIAN_POINT('Ctrl Pts',(-9.03976621700006,11.6,5.42632597599999));
#251269=CARTESIAN_POINT('Ctrl Pts',(-9.04155545700006,15.2,5.42696253499999));
#251270=CARTESIAN_POINT('Ctrl Pts',(-9.04155545700006,11.6,5.42696253499999));
#251271=CARTESIAN_POINT('Ctrl Pts',(-9.04335210000006,15.2,5.42759988499999));
#251272=CARTESIAN_POINT('Ctrl Pts',(-9.04335210000006,11.6,5.42759988499999));
#251273=CARTESIAN_POINT('Ctrl Pts',(-9.04515613500006,15.2,5.42823800699999));
#251274=CARTESIAN_POINT('Ctrl Pts',(-9.04515613500006,11.6,5.42823800699999));
#251275=CARTESIAN_POINT('Ctrl Pts',(-9.04696755200005,15.2,5.42887688499999));
#251276=CARTESIAN_POINT('Ctrl Pts',(-9.04696755200005,11.6,5.42887688499999));
#251277=CARTESIAN_POINT('Ctrl Pts',(-9.04878634100006,15.2,5.42951650299998));
#251278=CARTESIAN_POINT('Ctrl Pts',(-9.04878634100006,11.6,5.42951650299998));
#251279=CARTESIAN_POINT('Ctrl Pts',(-9.05061248800006,15.2,5.43015684399998));
#251280=CARTESIAN_POINT('Ctrl Pts',(-9.05061248800006,11.6,5.43015684399998));
#251281=CARTESIAN_POINT('Ctrl Pts',(-9.05244598400006,15.2,5.43079789199999));
#251282=CARTESIAN_POINT('Ctrl Pts',(-9.05244598400006,11.6,5.43079789199999));
#251283=CARTESIAN_POINT('Ctrl Pts',(-9.05428681800006,15.2,5.43143963099999));
#251284=CARTESIAN_POINT('Ctrl Pts',(-9.05428681800006,11.6,5.43143963099999));
#251285=CARTESIAN_POINT('Ctrl Pts',(-9.05613497800006,15.2,5.43208204499999));
#251286=CARTESIAN_POINT('Ctrl Pts',(-9.05613497800006,11.6,5.43208204499999));
#251287=CARTESIAN_POINT('Ctrl Pts',(-9.05799045400006,15.2,5.43272511599999));
#251288=CARTESIAN_POINT('Ctrl Pts',(-9.05799045400006,11.6,5.43272511599999));
#251289=CARTESIAN_POINT('Ctrl Pts',(-9.05985323600006,15.2,5.43336882999998));
#251290=CARTESIAN_POINT('Ctrl Pts',(-9.05985323600006,11.6,5.43336882999998));
#251291=CARTESIAN_POINT('Ctrl Pts',(-9.06172331100005,15.2,5.43401316999999));
#251292=CARTESIAN_POINT('Ctrl Pts',(-9.06172331100005,11.6,5.43401316999999));
#251293=CARTESIAN_POINT('Ctrl Pts',(-9.06360067000006,15.2,5.43465811899999));
#251294=CARTESIAN_POINT('Ctrl Pts',(-9.06360067000006,11.6,5.43465811899999));
#251295=CARTESIAN_POINT('Ctrl Pts',(-9.06548530100006,15.2,5.43530366299999));
#251296=CARTESIAN_POINT('Ctrl Pts',(-9.06548530100006,11.6,5.43530366299999));
#251297=CARTESIAN_POINT('Ctrl Pts',(-9.06737719300006,15.2,5.43594978599998));
#251298=CARTESIAN_POINT('Ctrl Pts',(-9.06737719300006,11.6,5.43594978599998));
#251299=CARTESIAN_POINT('Ctrl Pts',(-9.06927633700005,15.2,5.43659646999998));
#251300=CARTESIAN_POINT('Ctrl Pts',(-9.06927633700005,11.6,5.43659646999998));
#251301=CARTESIAN_POINT('Ctrl Pts',(-9.07118272000006,15.2,5.43724370099999));
#251302=CARTESIAN_POINT('Ctrl Pts',(-9.07118272000006,11.6,5.43724370099999));
#251303=CARTESIAN_POINT('Ctrl Pts',(-9.07309633400006,15.2,5.43789146299999));
#251304=CARTESIAN_POINT('Ctrl Pts',(-9.07309633400006,11.6,5.43789146299999));
#251305=CARTESIAN_POINT('Ctrl Pts',(-9.07501716700006,15.2,5.43853974199998));
#251306=CARTESIAN_POINT('Ctrl Pts',(-9.07501716700006,11.6,5.43853974199998));
#251307=CARTESIAN_POINT('Ctrl Pts',(-9.07694520800005,15.2,5.43918851899999));
#251308=CARTESIAN_POINT('Ctrl Pts',(-9.07694520800005,11.6,5.43918851899999));
#251309=CARTESIAN_POINT('Ctrl Pts',(-9.07888044600006,15.2,5.43983778099999));
#251310=CARTESIAN_POINT('Ctrl Pts',(-9.07888044600006,11.6,5.43983778099999));
#251311=CARTESIAN_POINT('Ctrl Pts',(-9.08082287200006,15.2,5.44048751199998));
#251312=CARTESIAN_POINT('Ctrl Pts',(-9.08082287200006,11.6,5.44048751199998));
#251313=CARTESIAN_POINT('Ctrl Pts',(-9.08277247500006,15.2,5.44113769599999));
#251314=CARTESIAN_POINT('Ctrl Pts',(-9.08277247500006,11.6,5.44113769599999));
#251315=CARTESIAN_POINT('Ctrl Pts',(-9.08472924200005,15.2,5.44178831899998));
#251316=CARTESIAN_POINT('Ctrl Pts',(-9.08472924200005,11.6,5.44178831899998));
#251317=CARTESIAN_POINT('Ctrl Pts',(-9.08669316600006,15.2,5.44243936399998));
#251318=CARTESIAN_POINT('Ctrl Pts',(-9.08669316600006,11.6,5.44243936399998));
#251319=CARTESIAN_POINT('Ctrl Pts',(-9.08866423500006,15.2,5.44309081699998));
#251320=CARTESIAN_POINT('Ctrl Pts',(-9.08866423500006,11.6,5.44309081699998));
#251321=CARTESIAN_POINT('Ctrl Pts',(-9.09064243800006,15.2,5.44374266199998));
#251322=CARTESIAN_POINT('Ctrl Pts',(-9.09064243800006,11.6,5.44374266199998));
#251323=CARTESIAN_POINT('Ctrl Pts',(-9.09262776600006,15.2,5.44439488499999));
#251324=CARTESIAN_POINT('Ctrl Pts',(-9.09262776600006,11.6,5.44439488499999));
#251325=CARTESIAN_POINT('Ctrl Pts',(-9.09462020800006,15.2,5.44504746899998));
#251326=CARTESIAN_POINT('Ctrl Pts',(-9.09462020800006,11.6,5.44504746899998));
#251327=CARTESIAN_POINT('Ctrl Pts',(-9.09661975200006,15.2,5.44570040099998));
#251328=CARTESIAN_POINT('Ctrl Pts',(-9.09661975200006,11.6,5.44570040099998));
#251329=CARTESIAN_POINT('Ctrl Pts',(-9.09862638900006,15.2,5.44635366599999));
#251330=CARTESIAN_POINT('Ctrl Pts',(-9.09862638900006,11.6,5.44635366599999));
#251331=CARTESIAN_POINT('Ctrl Pts',(-9.10064011000006,15.2,5.44700724699998));
#251332=CARTESIAN_POINT('Ctrl Pts',(-9.10064011000006,11.6,5.44700724699998));
#251333=CARTESIAN_POINT('Ctrl Pts',(-9.10266090200006,15.2,5.44766113199999));
#251334=CARTESIAN_POINT('Ctrl Pts',(-9.10266090200006,11.6,5.44766113199999));
#251335=CARTESIAN_POINT('Ctrl Pts',(-9.10468875600005,15.2,5.44831530299999));
#251336=CARTESIAN_POINT('Ctrl Pts',(-9.10468875600005,11.6,5.44831530299999));
#251337=CARTESIAN_POINT('Ctrl Pts',(-9.10672366200006,15.2,5.44896974899999));
#251338=CARTESIAN_POINT('Ctrl Pts',(-9.10672366200006,11.6,5.44896974899999));
#251339=CARTESIAN_POINT('Ctrl Pts',(-9.10876561000006,15.2,5.44962445199998));
#251340=CARTESIAN_POINT('Ctrl Pts',(-9.10876561000006,11.6,5.44962445199998));
#251341=CARTESIAN_POINT('Ctrl Pts',(-9.11081458900006,15.2,5.45027939999999));
#251342=CARTESIAN_POINT('Ctrl Pts',(-9.11081458900006,11.6,5.45027939999999));
#251343=CARTESIAN_POINT('Ctrl Pts',(-9.11287058900006,15.2,5.45093457599998));
#251344=CARTESIAN_POINT('Ctrl Pts',(-9.11287058900006,11.6,5.45093457599998));
#251345=CARTESIAN_POINT('Ctrl Pts',(-9.11493360000006,15.2,5.45158996699998));
#251346=CARTESIAN_POINT('Ctrl Pts',(-9.11493360000006,11.6,5.45158996699998));
#251347=CARTESIAN_POINT('Ctrl Pts',(-9.11700361100005,15.2,5.45224555799999));
#251348=CARTESIAN_POINT('Ctrl Pts',(-9.11700361100005,11.6,5.45224555799999));
#251349=CARTESIAN_POINT('Ctrl Pts',(-9.11908061400006,15.2,5.45290133499999));
#251350=CARTESIAN_POINT('Ctrl Pts',(-9.11908061400006,11.6,5.45290133499999));
#251351=CARTESIAN_POINT('Ctrl Pts',(-9.12116459600006,15.2,5.45355728299998));
#251352=CARTESIAN_POINT('Ctrl Pts',(-9.12116459600006,11.6,5.45355728299998));
#251353=CARTESIAN_POINT('Ctrl Pts',(-9.12325554900006,15.2,5.45421338899998));
#251354=CARTESIAN_POINT('Ctrl Pts',(-9.12325554900006,11.6,5.45421338899998));
#251355=CARTESIAN_POINT('Ctrl Pts',(-9.12535346300006,15.2,5.45486963699998));
#251356=CARTESIAN_POINT('Ctrl Pts',(-9.12535346300006,11.6,5.45486963699998));
#251357=CARTESIAN_POINT('Ctrl Pts',(-9.12745832700006,15.2,5.45552601299998));
#251358=CARTESIAN_POINT('Ctrl Pts',(-9.12745832700006,11.6,5.45552601299998));
#251359=CARTESIAN_POINT('Ctrl Pts',(-9.12957013000005,15.2,5.45618250499999));
#251360=CARTESIAN_POINT('Ctrl Pts',(-9.12957013000005,11.6,5.45618250499999));
#251361=CARTESIAN_POINT('Ctrl Pts',(-9.13168886400006,15.2,5.45683909699999));
#251362=CARTESIAN_POINT('Ctrl Pts',(-9.13168886400006,11.6,5.45683909699999));
#251363=CARTESIAN_POINT('Ctrl Pts',(-9.13381451900005,15.2,5.45749577499999));
#251364=CARTESIAN_POINT('Ctrl Pts',(-9.13381451900005,11.6,5.45749577499999));
#251365=CARTESIAN_POINT('Ctrl Pts',(-9.13594708400005,15.2,5.45815252399999));
#251366=CARTESIAN_POINT('Ctrl Pts',(-9.13594708400005,11.6,5.45815252399999));
#251367=CARTESIAN_POINT('Ctrl Pts',(-9.13808654800006,15.2,5.45880933299999));
#251368=CARTESIAN_POINT('Ctrl Pts',(-9.13808654800006,11.6,5.45880933299999));
#251369=CARTESIAN_POINT('Ctrl Pts',(-9.14023290400005,15.2,5.45946618599999));
#251370=CARTESIAN_POINT('Ctrl Pts',(-9.14023290400005,11.6,5.45946618599999));
#251371=CARTESIAN_POINT('Ctrl Pts',(-9.14238614100006,15.2,5.46012306899998));
#251372=CARTESIAN_POINT('Ctrl Pts',(-9.14238614100006,11.6,5.46012306899998));
#251373=CARTESIAN_POINT('Ctrl Pts',(-9.14454624700006,15.2,5.46077996999998));
#251374=CARTESIAN_POINT('Ctrl Pts',(-9.14454624700006,11.6,5.46077996999998));
#251375=CARTESIAN_POINT('Ctrl Pts',(-9.14671321500006,15.2,5.46143687199999));
#251376=CARTESIAN_POINT('Ctrl Pts',(-9.14671321500006,11.6,5.46143687199999));
#251377=CARTESIAN_POINT('Ctrl Pts',(-9.14888703300005,15.2,5.46209376499998));
#251378=CARTESIAN_POINT('Ctrl Pts',(-9.14888703300005,11.6,5.46209376499998));
#251379=CARTESIAN_POINT('Ctrl Pts',(-9.15106769300005,15.2,5.46275063199998));
#251380=CARTESIAN_POINT('Ctrl Pts',(-9.15106769300005,11.6,5.46275063199998));
#251381=CARTESIAN_POINT('Ctrl Pts',(-9.15325518500006,15.2,5.46340746199999));
#251382=CARTESIAN_POINT('Ctrl Pts',(-9.15325518500006,11.6,5.46340746199999));
#251383=CARTESIAN_POINT('Ctrl Pts',(-9.15544949700006,15.2,5.46406423999999));
#251384=CARTESIAN_POINT('Ctrl Pts',(-9.15544949700006,11.6,5.46406423999999));
#251385=CARTESIAN_POINT('Ctrl Pts',(-9.15765062100006,15.2,5.46472095299999));
#251386=CARTESIAN_POINT('Ctrl Pts',(-9.15765062100006,11.6,5.46472095299999));
#251387=CARTESIAN_POINT('Ctrl Pts',(-9.15985854800006,15.2,5.46537758799998));
#251388=CARTESIAN_POINT('Ctrl Pts',(-9.15985854800006,11.6,5.46537758799998));
#251389=CARTESIAN_POINT('Ctrl Pts',(-9.16207326800006,15.2,5.46603412999998));
#251390=CARTESIAN_POINT('Ctrl Pts',(-9.16207326800006,11.6,5.46603412999998));
#251391=CARTESIAN_POINT('Ctrl Pts',(-9.16429476900005,15.2,5.46669056699999));
#251392=CARTESIAN_POINT('Ctrl Pts',(-9.16429476900005,11.6,5.46669056699999));
#251393=CARTESIAN_POINT('Ctrl Pts',(-9.16652304500005,15.2,5.46734688499999));
#251394=CARTESIAN_POINT('Ctrl Pts',(-9.16652304500005,11.6,5.46734688499999));
#251395=CARTESIAN_POINT('Ctrl Pts',(-9.16875808300006,15.2,5.46800307099998));
#251396=CARTESIAN_POINT('Ctrl Pts',(-9.16875808300006,11.6,5.46800307099998));
#251397=CARTESIAN_POINT('Ctrl Pts',(-9.17099987400006,15.2,5.46865911099999));
#251398=CARTESIAN_POINT('Ctrl Pts',(-9.17099987400006,11.6,5.46865911099999));
#251399=CARTESIAN_POINT('Ctrl Pts',(-9.17324841100006,15.2,5.46931499399999));
#251400=CARTESIAN_POINT('Ctrl Pts',(-9.17324841100006,11.6,5.46931499399999));
#251401=CARTESIAN_POINT('Ctrl Pts',(-9.17550368100006,15.2,5.46997070399998));
#251402=CARTESIAN_POINT('Ctrl Pts',(-9.17550368100006,11.6,5.46997070399998));
#251403=CARTESIAN_POINT('Ctrl Pts',(-9.17776567700006,15.2,5.47062622899999));
#251404=CARTESIAN_POINT('Ctrl Pts',(-9.17776567700006,11.6,5.47062622899999));
#251405=CARTESIAN_POINT('Ctrl Pts',(-9.18003438700006,15.2,5.47128155699999));
#251406=CARTESIAN_POINT('Ctrl Pts',(-9.18003438700006,11.6,5.47128155699999));
#251407=CARTESIAN_POINT('Ctrl Pts',(-9.18230980500006,15.2,5.47193667299998));
#251408=CARTESIAN_POINT('Ctrl Pts',(-9.18230980500006,11.6,5.47193667299998));
#251409=CARTESIAN_POINT('Ctrl Pts',(-9.18459191800006,15.2,5.47259156599999));
#251410=CARTESIAN_POINT('Ctrl Pts',(-9.18459191800006,11.6,5.47259156599999));
#251411=CARTESIAN_POINT('Ctrl Pts',(-9.18688071800006,15.2,5.47324622199999));
#251412=CARTESIAN_POINT('Ctrl Pts',(-9.18688071800006,11.6,5.47324622199999));
#251413=CARTESIAN_POINT('Ctrl Pts',(-9.18917619500006,15.2,5.47390062799998));
#251414=CARTESIAN_POINT('Ctrl Pts',(-9.18917619500006,11.6,5.47390062799998));
#251415=CARTESIAN_POINT('Ctrl Pts',(-9.19147834000006,15.2,5.47455477199998));
#251416=CARTESIAN_POINT('Ctrl Pts',(-9.19147834000006,11.6,5.47455477199998));
#251417=CARTESIAN_POINT('Ctrl Pts',(-9.19378714400005,15.2,5.47520864099998));
#251418=CARTESIAN_POINT('Ctrl Pts',(-9.19378714400005,11.6,5.47520864099998));
#251419=CARTESIAN_POINT('Ctrl Pts',(-9.19610259600006,15.2,5.47586222099999));
#251420=CARTESIAN_POINT('Ctrl Pts',(-9.19610259600006,11.6,5.47586222099999));
#251421=CARTESIAN_POINT('Ctrl Pts',(-9.19842468800006,15.2,5.47651549999999));
#251422=CARTESIAN_POINT('Ctrl Pts',(-9.19842468800006,11.6,5.47651549999999));
#251423=CARTESIAN_POINT('Ctrl Pts',(-9.20075341100006,15.2,5.47716846599998));
#251424=CARTESIAN_POINT('Ctrl Pts',(-9.20075341100006,11.6,5.47716846599998));
#251425=CARTESIAN_POINT('Ctrl Pts',(-9.20308875400006,15.2,5.47782110499998));
#251426=CARTESIAN_POINT('Ctrl Pts',(-9.20308875400006,11.6,5.47782110499998));
#251427=CARTESIAN_POINT('Ctrl Pts',(-9.20543070800005,15.2,5.47847340599999));
#251428=CARTESIAN_POINT('Ctrl Pts',(-9.20543070800005,11.6,5.47847340599999));
#251429=CARTESIAN_POINT('Ctrl Pts',(-9.20777926500006,15.2,5.47912535599998));
#251430=CARTESIAN_POINT('Ctrl Pts',(-9.20777926500006,11.6,5.47912535599998));
#251431=CARTESIAN_POINT('Ctrl Pts',(-9.21013441500006,15.2,5.47977694199999));
#251432=CARTESIAN_POINT('Ctrl Pts',(-9.21013441500006,11.6,5.47977694199999));
#251433=CARTESIAN_POINT('Ctrl Pts',(-9.21249614800006,15.2,5.48042815199998));
#251434=CARTESIAN_POINT('Ctrl Pts',(-9.21249614800006,11.6,5.48042815199998));
#251435=CARTESIAN_POINT('Ctrl Pts',(-9.21486445500006,15.2,5.48107897299998));
#251436=CARTESIAN_POINT('Ctrl Pts',(-9.21486445500006,11.6,5.48107897299998));
#251437=CARTESIAN_POINT('Ctrl Pts',(-9.21723932700005,15.2,5.48172939299998));
#251438=CARTESIAN_POINT('Ctrl Pts',(-9.21723932700005,11.6,5.48172939299998));
#251439=CARTESIAN_POINT('Ctrl Pts',(-9.21962075500005,15.2,5.48237939999999));
#251440=CARTESIAN_POINT('Ctrl Pts',(-9.21962075500005,11.6,5.48237939999999));
#251441=CARTESIAN_POINT('Ctrl Pts',(-9.22200872900006,15.2,5.48302897999999));
#251442=CARTESIAN_POINT('Ctrl Pts',(-9.22200872900006,11.6,5.48302897999999));
#251443=CARTESIAN_POINT('Ctrl Pts',(-9.22440324100006,15.2,5.48367812299999));
#251444=CARTESIAN_POINT('Ctrl Pts',(-9.22440324100006,11.6,5.48367812299999));
#251445=CARTESIAN_POINT('Ctrl Pts',(-9.22680428000006,15.2,5.48432681599999));
#251446=CARTESIAN_POINT('Ctrl Pts',(-9.22680428000006,11.6,5.48432681599999));
#251447=CARTESIAN_POINT('Ctrl Pts',(-9.22921184000005,15.2,5.48497504599998));
#251448=CARTESIAN_POINT('Ctrl Pts',(-9.22921184000005,11.6,5.48497504599998));
#251449=CARTESIAN_POINT('Ctrl Pts',(-9.23162590700005,15.2,5.48562280199998));
#251450=CARTESIAN_POINT('Ctrl Pts',(-9.23162590700005,11.6,5.48562280199998));
#251451=CARTESIAN_POINT('Ctrl Pts',(-9.23404647600006,15.2,5.48627007099999));
#251452=CARTESIAN_POINT('Ctrl Pts',(-9.23404647600006,11.6,5.48627007099999));
#251453=CARTESIAN_POINT('Ctrl Pts',(-9.23647353600006,15.2,5.48691684199999));
#251454=CARTESIAN_POINT('Ctrl Pts',(-9.23647353600006,11.6,5.48691684199999));
#251455=CARTESIAN_POINT('Ctrl Pts',(-9.23890707800006,15.2,5.48756310099999));
#251456=CARTESIAN_POINT('Ctrl Pts',(-9.23890707800006,11.6,5.48756310099999));
#251457=CARTESIAN_POINT('Ctrl Pts',(-9.24134709500006,15.2,5.48820883899998));
#251458=CARTESIAN_POINT('Ctrl Pts',(-9.24134709500006,11.6,5.48820883899998));
#251459=CARTESIAN_POINT('Ctrl Pts',(-9.24379357400005,15.2,5.48885404199999));
#251460=CARTESIAN_POINT('Ctrl Pts',(-9.24379357400005,11.6,5.48885404199999));
#251461=CARTESIAN_POINT('Ctrl Pts',(-9.24624650800006,15.2,5.48949869799999));
#251462=CARTESIAN_POINT('Ctrl Pts',(-9.24624650800006,11.6,5.48949869799999));
#251463=CARTESIAN_POINT('Ctrl Pts',(-9.24870588900006,15.2,5.49014279599999));
#251464=CARTESIAN_POINT('Ctrl Pts',(-9.24870588900006,11.6,5.49014279599999));
#251465=CARTESIAN_POINT('Ctrl Pts',(-9.25117170700006,15.2,5.49078632299998));
#251466=CARTESIAN_POINT('Ctrl Pts',(-9.25117170700006,11.6,5.49078632299998));
#251467=CARTESIAN_POINT('Ctrl Pts',(-9.25364395300006,15.2,5.49142926899999));
#251468=CARTESIAN_POINT('Ctrl Pts',(-9.25364395300006,11.6,5.49142926899999));
#251469=CARTESIAN_POINT('Ctrl Pts',(-9.25612261700006,15.2,5.49207162099999));
#251470=CARTESIAN_POINT('Ctrl Pts',(-9.25612261700006,11.6,5.49207162099999));
#251471=CARTESIAN_POINT('Ctrl Pts',(-9.25860769100005,15.2,5.49271336799999));
#251472=CARTESIAN_POINT('Ctrl Pts',(-9.25860769100005,11.6,5.49271336799999));
#251473=CARTESIAN_POINT('Ctrl Pts',(-9.26109916600005,15.2,5.49335449699999));
#251474=CARTESIAN_POINT('Ctrl Pts',(-9.26109916600005,11.6,5.49335449699999));
#251475=CARTESIAN_POINT('Ctrl Pts',(-9.26359703400006,15.2,5.49399499799998));
#251476=CARTESIAN_POINT('Ctrl Pts',(-9.26359703400006,11.6,5.49399499799998));
#251477=CARTESIAN_POINT('Ctrl Pts',(-9.26610128400006,15.2,5.49463485799999));
#251478=CARTESIAN_POINT('Ctrl Pts',(-9.26610128400006,11.6,5.49463485799999));
#251479=CARTESIAN_POINT('Ctrl Pts',(-9.26861190800006,15.2,5.49527406699998));
#251480=CARTESIAN_POINT('Ctrl Pts',(-9.26861190800006,11.6,5.49527406699998));
#251481=CARTESIAN_POINT('Ctrl Pts',(-9.27112889900006,15.2,5.49591261299998));
#251482=CARTESIAN_POINT('Ctrl Pts',(-9.27112889900006,11.6,5.49591261299998));
#251483=CARTESIAN_POINT('Ctrl Pts',(-9.27365224500006,15.2,5.49655048299999));
#251484=CARTESIAN_POINT('Ctrl Pts',(-9.27365224500006,11.6,5.49655048299999));
#251485=CARTESIAN_POINT('Ctrl Pts',(-9.27618193800006,15.2,5.49718766699999));
#251486=CARTESIAN_POINT('Ctrl Pts',(-9.27618193800006,11.6,5.49718766699999));
#251487=CARTESIAN_POINT('Ctrl Pts',(-9.27871797000006,15.2,5.49782415299998));
#251488=CARTESIAN_POINT('Ctrl Pts',(-9.27871797000006,11.6,5.49782415299998));
#251489=CARTESIAN_POINT('Ctrl Pts',(-9.28126033200006,15.2,5.49845993099999));
#251490=CARTESIAN_POINT('Ctrl Pts',(-9.28126033200006,11.6,5.49845993099999));
#251491=CARTESIAN_POINT('Ctrl Pts',(-9.28380901600006,15.2,5.49909498699999));
#251492=CARTESIAN_POINT('Ctrl Pts',(-9.28380901600006,11.6,5.49909498699999));
#251493=CARTESIAN_POINT('Ctrl Pts',(-9.28636401000006,15.2,5.49972931199999));
#251494=CARTESIAN_POINT('Ctrl Pts',(-9.28636401000006,11.6,5.49972931199999));
#251495=CARTESIAN_POINT('Ctrl Pts',(-9.28892530800006,15.2,5.50036289399999));
#251496=CARTESIAN_POINT('Ctrl Pts',(-9.28892530800006,11.6,5.50036289399999));
#251497=CARTESIAN_POINT('Ctrl Pts',(-9.29149290100005,15.2,5.50099572199999));
#251498=CARTESIAN_POINT('Ctrl Pts',(-9.29149290100005,11.6,5.50099572199999));
#251499=CARTESIAN_POINT('Ctrl Pts',(-9.29406677900005,15.2,5.50162778399999));
#251500=CARTESIAN_POINT('Ctrl Pts',(-9.29406677900005,11.6,5.50162778399999));
#251501=CARTESIAN_POINT('Ctrl Pts',(-9.29664693500006,15.2,5.50225906999999));
#251502=CARTESIAN_POINT('Ctrl Pts',(-9.29664693500006,11.6,5.50225906999999));
#251503=CARTESIAN_POINT('Ctrl Pts',(-9.29923335800006,15.2,5.50288956699998));
#251504=CARTESIAN_POINT('Ctrl Pts',(-9.29923335800006,11.6,5.50288956699998));
#251505=CARTESIAN_POINT('Ctrl Pts',(-9.30182604200006,15.2,5.50351926599999));
#251506=CARTESIAN_POINT('Ctrl Pts',(-9.30182604200006,11.6,5.50351926599999));
#251507=CARTESIAN_POINT('Ctrl Pts',(-9.30442497600006,15.2,5.50414815599999));
#251508=CARTESIAN_POINT('Ctrl Pts',(-9.30442497600006,11.6,5.50414815599999));
#251509=CARTESIAN_POINT('Ctrl Pts',(-9.30703015100006,15.2,5.50477622499999));
#251510=CARTESIAN_POINT('Ctrl Pts',(-9.30703015100006,11.6,5.50477622499999));
#251511=CARTESIAN_POINT('Ctrl Pts',(-9.30964156100006,15.2,5.50540346099999));
#251512=CARTESIAN_POINT('Ctrl Pts',(-9.30964156100006,11.6,5.50540346099999));
#251513=CARTESIAN_POINT('Ctrl Pts',(-9.31225919500006,15.2,5.50602985399999));
#251514=CARTESIAN_POINT('Ctrl Pts',(-9.31225919500006,11.6,5.50602985399999));
#251515=CARTESIAN_POINT('Ctrl Pts',(-9.31488304500006,15.2,5.50665539299998));
#251516=CARTESIAN_POINT('Ctrl Pts',(-9.31488304500006,11.6,5.50665539299998));
#251517=CARTESIAN_POINT('Ctrl Pts',(-9.31751310300006,15.2,5.50728006899998));
#251518=CARTESIAN_POINT('Ctrl Pts',(-9.31751310300006,11.6,5.50728006899998));
#251519=CARTESIAN_POINT('Ctrl Pts',(-9.32014935900006,15.2,5.50790386899998));
#251520=CARTESIAN_POINT('Ctrl Pts',(-9.32014935900006,11.6,5.50790386899998));
#251521=CARTESIAN_POINT('Ctrl Pts',(-9.32279180500006,15.2,5.50852678299999));
#251522=CARTESIAN_POINT('Ctrl Pts',(-9.32279180500006,11.6,5.50852678299999));
#251523=CARTESIAN_POINT('Ctrl Pts',(-9.32544043300006,15.2,5.50914879899998));
#251524=CARTESIAN_POINT('Ctrl Pts',(-9.32544043300006,11.6,5.50914879899998));
#251525=CARTESIAN_POINT('Ctrl Pts',(-9.32809523400006,15.2,5.50976990799998));
#251526=CARTESIAN_POINT('Ctrl Pts',(-9.32809523400006,11.6,5.50976990799998));
#251527=CARTESIAN_POINT('Ctrl Pts',(-9.33075619900006,15.2,5.51039009699998));
#251528=CARTESIAN_POINT('Ctrl Pts',(-9.33075619900006,11.6,5.51039009699998));
#251529=CARTESIAN_POINT('Ctrl Pts',(-9.33342332100005,15.2,5.51100935799998));
#251530=CARTESIAN_POINT('Ctrl Pts',(-9.33342332100005,11.6,5.51100935799998));
#251531=CARTESIAN_POINT('Ctrl Pts',(-9.33609659000006,15.2,5.51162767899999));
#251532=CARTESIAN_POINT('Ctrl Pts',(-9.33609659000006,11.6,5.51162767899999));
#251533=CARTESIAN_POINT('Ctrl Pts',(-9.33877599800006,15.2,5.51224504999999));
#251534=CARTESIAN_POINT('Ctrl Pts',(-9.33877599800006,11.6,5.51224504999999));
#251535=CARTESIAN_POINT('Ctrl Pts',(-9.34146153500006,15.2,5.51286145899999));
#251536=CARTESIAN_POINT('Ctrl Pts',(-9.34146153500006,11.6,5.51286145899999));
#251537=CARTESIAN_POINT('Ctrl Pts',(-9.34415319400006,15.2,5.51347689699998));
#251538=CARTESIAN_POINT('Ctrl Pts',(-9.34415319400006,11.6,5.51347689699998));
#251539=CARTESIAN_POINT('Ctrl Pts',(-9.34685096600005,15.2,5.51409135199999));
#251540=CARTESIAN_POINT('Ctrl Pts',(-9.34685096600005,11.6,5.51409135199999));
#251541=CARTESIAN_POINT('Ctrl Pts',(-9.34955484400006,15.2,5.51470481499998));
#251542=CARTESIAN_POINT('Ctrl Pts',(-9.34955484400006,11.6,5.51470481499998));
#251543=CARTESIAN_POINT('Ctrl Pts',(-9.35226481800006,15.2,5.51531727499999));
#251544=CARTESIAN_POINT('Ctrl Pts',(-9.35226481800006,11.6,5.51531727499999));
#251545=CARTESIAN_POINT('Ctrl Pts',(-9.35498087900006,15.2,5.51592872299998));
#251546=CARTESIAN_POINT('Ctrl Pts',(-9.35498087900006,11.6,5.51592872299998));
#251547=CARTESIAN_POINT('Ctrl Pts',(-9.35770302000006,15.2,5.51653914499998));
#251548=CARTESIAN_POINT('Ctrl Pts',(-9.35770302000006,11.6,5.51653914499998));
#251549=CARTESIAN_POINT('Ctrl Pts',(-9.36043123200006,15.2,5.51714853399999));
#251550=CARTESIAN_POINT('Ctrl Pts',(-9.36043123200006,11.6,5.51714853399999));
#251551=CARTESIAN_POINT('Ctrl Pts',(-9.36316550600005,15.2,5.51775687799999));
#251552=CARTESIAN_POINT('Ctrl Pts',(-9.36316550600005,11.6,5.51775687799999));
#251553=CARTESIAN_POINT('Ctrl Pts',(-9.36590583500006,15.2,5.51836416599999));
#251554=CARTESIAN_POINT('Ctrl Pts',(-9.36590583500006,11.6,5.51836416599999));
#251555=CARTESIAN_POINT('Ctrl Pts',(-9.36865220900006,15.2,5.51897039099998));
#251556=CARTESIAN_POINT('Ctrl Pts',(-9.36865220900006,11.6,5.51897039099998));
#251557=CARTESIAN_POINT('Ctrl Pts',(-9.37140462000006,15.2,5.51957553899998));
#251558=CARTESIAN_POINT('Ctrl Pts',(-9.37140462000006,11.6,5.51957553899998));
#251559=CARTESIAN_POINT('Ctrl Pts',(-9.37416306100006,15.2,5.52017960199999));
#251560=CARTESIAN_POINT('Ctrl Pts',(-9.37416306100006,11.6,5.52017960199999));
#251561=CARTESIAN_POINT('Ctrl Pts',(-9.37692752300006,15.2,5.52078256899998));
#251562=CARTESIAN_POINT('Ctrl Pts',(-9.37692752300006,11.6,5.52078256899998));
#251563=CARTESIAN_POINT('Ctrl Pts',(-9.37969799600006,15.2,5.52138443099999));
#251564=CARTESIAN_POINT('Ctrl Pts',(-9.37969799600006,11.6,5.52138443099999));
#251565=CARTESIAN_POINT('Ctrl Pts',(-9.38247447400006,15.2,5.52198517699999));
#251566=CARTESIAN_POINT('Ctrl Pts',(-9.38247447400006,11.6,5.52198517699999));
#251567=CARTESIAN_POINT('Ctrl Pts',(-9.38525694800006,15.2,5.52258479699999));
#251568=CARTESIAN_POINT('Ctrl Pts',(-9.38525694800006,11.6,5.52258479699999));
#251569=CARTESIAN_POINT('Ctrl Pts',(-9.38804540900006,15.2,5.52318327999998));
#251570=CARTESIAN_POINT('Ctrl Pts',(-9.38804540900006,11.6,5.52318327999998));
#251571=CARTESIAN_POINT('Ctrl Pts',(-9.39083984900006,15.2,5.52378061799998));
#251572=CARTESIAN_POINT('Ctrl Pts',(-9.39083984900006,11.6,5.52378061799998));
#251573=CARTESIAN_POINT('Ctrl Pts',(-9.39364025900005,15.2,5.52437679899998));
#251574=CARTESIAN_POINT('Ctrl Pts',(-9.39364025900005,11.6,5.52437679899998));
#251575=CARTESIAN_POINT('Ctrl Pts',(-9.39644663200006,15.2,5.52497181399998));
#251576=CARTESIAN_POINT('Ctrl Pts',(-9.39644663200006,11.6,5.52497181399998));
#251577=CARTESIAN_POINT('Ctrl Pts',(-9.39925896000006,15.2,5.52556565399998));
#251578=CARTESIAN_POINT('Ctrl Pts',(-9.39925896000006,11.6,5.52556565399998));
#251579=CARTESIAN_POINT('Ctrl Pts',(-9.40207723400006,15.2,5.52615830699998));
#251580=CARTESIAN_POINT('Ctrl Pts',(-9.40207723400006,11.6,5.52615830699998));
#251581=CARTESIAN_POINT('Ctrl Pts',(-9.40490144600006,15.2,5.52674976499999));
#251582=CARTESIAN_POINT('Ctrl Pts',(-9.40490144600006,11.6,5.52674976499999));
#251583=CARTESIAN_POINT('Ctrl Pts',(-9.40773158700006,15.2,5.52734001699999));
#251584=CARTESIAN_POINT('Ctrl Pts',(-9.40773158700006,11.6,5.52734001699999));
#251585=CARTESIAN_POINT('Ctrl Pts',(-9.41056765000006,15.2,5.52792905499999));
#251586=CARTESIAN_POINT('Ctrl Pts',(-9.41056765000006,11.6,5.52792905499999));
#251587=CARTESIAN_POINT('Ctrl Pts',(-9.41340962600006,15.2,5.52851686599999));
#251588=CARTESIAN_POINT('Ctrl Pts',(-9.41340962600006,11.6,5.52851686599999));
#251589=CARTESIAN_POINT('Ctrl Pts',(-9.41625750700006,15.2,5.52910344399999));
#251590=CARTESIAN_POINT('Ctrl Pts',(-9.41625750700006,11.6,5.52910344399999));
#251591=CARTESIAN_POINT('Ctrl Pts',(-9.41911128500006,15.2,5.52968877599999));
#251592=CARTESIAN_POINT('Ctrl Pts',(-9.41911128500006,11.6,5.52968877599999));
#251593=CARTESIAN_POINT('Ctrl Pts',(-9.42197095100006,15.2,5.53027285299999));
#251594=CARTESIAN_POINT('Ctrl Pts',(-9.42197095100006,11.6,5.53027285299999));
#251595=CARTESIAN_POINT('Ctrl Pts',(-9.42483649800005,15.2,5.53085566799999));
#251596=CARTESIAN_POINT('Ctrl Pts',(-9.42483649800005,11.6,5.53085566799999));
#251597=CARTESIAN_POINT('Ctrl Pts',(-9.42770791800006,15.2,5.53143720799999));
#251598=CARTESIAN_POINT('Ctrl Pts',(-9.42770791800006,11.6,5.53143720799999));
#251599=CARTESIAN_POINT('Ctrl Pts',(-9.43058520300006,15.2,5.53201746599999));
#251600=CARTESIAN_POINT('Ctrl Pts',(-9.43058520300006,11.6,5.53201746599999));
#251601=CARTESIAN_POINT('Ctrl Pts',(-9.43346834300005,15.2,5.53259642999999));
#251602=CARTESIAN_POINT('Ctrl Pts',(-9.43346834300005,11.6,5.53259642999999));
#251603=CARTESIAN_POINT('Ctrl Pts',(-9.43635733100006,15.2,5.53317409299999));
#251604=CARTESIAN_POINT('Ctrl Pts',(-9.43635733100006,11.6,5.53317409299999));
#251605=CARTESIAN_POINT('Ctrl Pts',(-9.43925215900006,15.2,5.53375044299998));
#251606=CARTESIAN_POINT('Ctrl Pts',(-9.43925215900006,11.6,5.53375044299998));
#251607=CARTESIAN_POINT('Ctrl Pts',(-9.44215282000006,15.2,5.53432547199999));
#251608=CARTESIAN_POINT('Ctrl Pts',(-9.44215282000006,11.6,5.53432547199999));
#251609=CARTESIAN_POINT('Ctrl Pts',(-9.44505930500006,15.2,5.53489916999998));
#251610=CARTESIAN_POINT('Ctrl Pts',(-9.44505930500006,11.6,5.53489916999998));
#251611=CARTESIAN_POINT('Ctrl Pts',(-9.44797160500006,15.2,5.53547152899998));
#251612=CARTESIAN_POINT('Ctrl Pts',(-9.44797160500006,11.6,5.53547152899998));
#251613=CARTESIAN_POINT('Ctrl Pts',(-9.45088971300006,15.2,5.53604253699999));
#251614=CARTESIAN_POINT('Ctrl Pts',(-9.45088971300006,11.6,5.53604253699999));
#251615=CARTESIAN_POINT('Ctrl Pts',(-9.45381362100006,15.2,5.53661218699999));
#251616=CARTESIAN_POINT('Ctrl Pts',(-9.45381362100006,11.6,5.53661218699999));
#251617=CARTESIAN_POINT('Ctrl Pts',(-9.45674332000005,15.2,5.53718046699998));
#251618=CARTESIAN_POINT('Ctrl Pts',(-9.45674332000005,11.6,5.53718046699998));
#251619=CARTESIAN_POINT('Ctrl Pts',(-9.45967880400006,15.2,5.53774737099998));
#251620=CARTESIAN_POINT('Ctrl Pts',(-9.45967880400006,11.6,5.53774737099998));
#251621=CARTESIAN_POINT('Ctrl Pts',(-9.46262006300006,15.2,5.53831288699998));
#251622=CARTESIAN_POINT('Ctrl Pts',(-9.46262006300006,11.6,5.53831288699998));
#251623=CARTESIAN_POINT('Ctrl Pts',(-9.46556709000006,15.2,5.53887700699998));
#251624=CARTESIAN_POINT('Ctrl Pts',(-9.46556709000006,11.6,5.53887700699998));
#251625=CARTESIAN_POINT('Ctrl Pts',(-9.46851987800006,15.2,5.53943972199999));
#251626=CARTESIAN_POINT('Ctrl Pts',(-9.46851987800006,11.6,5.53943972199999));
#251627=CARTESIAN_POINT('Ctrl Pts',(-9.47147841600006,15.2,5.54000102199999));
#251628=CARTESIAN_POINT('Ctrl Pts',(-9.47147841600006,11.6,5.54000102199999));
#251629=CARTESIAN_POINT('Ctrl Pts',(-9.47444269900006,15.2,5.54056089699999));
#251630=CARTESIAN_POINT('Ctrl Pts',(-9.47444269900006,11.6,5.54056089699999));
#251631=CARTESIAN_POINT('Ctrl Pts',(-9.47741271700006,15.2,5.54111933999998));
#251632=CARTESIAN_POINT('Ctrl Pts',(-9.47741271700006,11.6,5.54111933999998));
#251633=CARTESIAN_POINT('Ctrl Pts',(-9.48038846400006,15.2,5.54167634099999));
#251634=CARTESIAN_POINT('Ctrl Pts',(-9.48038846400006,11.6,5.54167634099999));
#251635=CARTESIAN_POINT('Ctrl Pts',(-9.48336993000006,15.2,5.54223188999998));
#251636=CARTESIAN_POINT('Ctrl Pts',(-9.48336993000006,11.6,5.54223188999998));
#251637=CARTESIAN_POINT('Ctrl Pts',(-9.48635711000006,15.2,5.54278597899999));
#251638=CARTESIAN_POINT('Ctrl Pts',(-9.48635711000006,11.6,5.54278597899999));
#251639=CARTESIAN_POINT('Ctrl Pts',(-9.48934999300005,15.2,5.54333859899998));
#251640=CARTESIAN_POINT('Ctrl Pts',(-9.48934999300005,11.6,5.54333859899998));
#251641=CARTESIAN_POINT('Ctrl Pts',(-9.49234857200006,15.2,5.54388973899999));
#251642=CARTESIAN_POINT('Ctrl Pts',(-9.49234857200006,11.6,5.54388973899999));
#251643=CARTESIAN_POINT('Ctrl Pts',(-9.49535284000006,15.2,5.54443939299999));
#251644=CARTESIAN_POINT('Ctrl Pts',(-9.49535284000006,11.6,5.54443939299999));
#251645=CARTESIAN_POINT('Ctrl Pts',(-9.49836278900005,15.2,5.54498754999998));
#251646=CARTESIAN_POINT('Ctrl Pts',(-9.49836278900005,11.6,5.54498754999998));
#251647=CARTESIAN_POINT('Ctrl Pts',(-9.50137841100006,15.2,5.54553420099998));
#251648=CARTESIAN_POINT('Ctrl Pts',(-9.50137841100006,11.6,5.54553420099998));
#251649=CARTESIAN_POINT('Ctrl Pts',(-9.50439969700006,15.2,5.54607933899998));
#251650=CARTESIAN_POINT('Ctrl Pts',(-9.50439969700006,11.6,5.54607933899998));
#251651=CARTESIAN_POINT('Ctrl Pts',(-9.50742664100006,15.2,5.54662295199999));
#251652=CARTESIAN_POINT('Ctrl Pts',(-9.50742664100006,11.6,5.54662295199999));
#251653=CARTESIAN_POINT('Ctrl Pts',(-9.51045923400006,15.2,5.54716503299999));
#251654=CARTESIAN_POINT('Ctrl Pts',(-9.51045923400006,11.6,5.54716503299999));
#251655=CARTESIAN_POINT('Ctrl Pts',(-9.51349746800006,15.2,5.54770557499998));
#251656=CARTESIAN_POINT('Ctrl Pts',(-9.51349746800006,11.6,5.54770557499998));
#251657=CARTESIAN_POINT('Ctrl Pts',(-9.51654133700006,15.2,5.54824456499999));
#251658=CARTESIAN_POINT('Ctrl Pts',(-9.51654133700006,11.6,5.54824456499999));
#251659=CARTESIAN_POINT('Ctrl Pts',(-9.51959083100006,15.2,5.54878199699999));
#251660=CARTESIAN_POINT('Ctrl Pts',(-9.51959083100006,11.6,5.54878199699999));
#251661=CARTESIAN_POINT('Ctrl Pts',(-9.52264594400006,15.2,5.54931786199998));
#251662=CARTESIAN_POINT('Ctrl Pts',(-9.52264594400006,11.6,5.54931786199998));
#251663=CARTESIAN_POINT('Ctrl Pts',(-9.52570666500005,15.2,5.54985215099999));
#251664=CARTESIAN_POINT('Ctrl Pts',(-9.52570666500005,11.6,5.54985215099999));
#251665=CARTESIAN_POINT('Ctrl Pts',(-9.52877299100006,15.2,5.55038485499999));
#251666=CARTESIAN_POINT('Ctrl Pts',(-9.52877299100006,11.6,5.55038485499999));
#251667=CARTESIAN_POINT('Ctrl Pts',(-9.53184491100006,15.2,5.55091596499998));
#251668=CARTESIAN_POINT('Ctrl Pts',(-9.53184491100006,11.6,5.55091596499998));
#251669=CARTESIAN_POINT('Ctrl Pts',(-9.53492241700006,15.2,5.55144547299999));
#251670=CARTESIAN_POINT('Ctrl Pts',(-9.53492241700006,11.6,5.55144547299999));
#251671=CARTESIAN_POINT('Ctrl Pts',(-9.53800550500005,15.2,5.55197336999999));
#251672=CARTESIAN_POINT('Ctrl Pts',(-9.53800550500005,11.6,5.55197336999999));
#251673=CARTESIAN_POINT('Ctrl Pts',(-9.54109416200006,15.2,5.55249964699998));
#251674=CARTESIAN_POINT('Ctrl Pts',(-9.54109416200006,11.6,5.55249964699998));
#251675=CARTESIAN_POINT('Ctrl Pts',(-9.54418838400005,15.2,5.55302429599998));
#251676=CARTESIAN_POINT('Ctrl Pts',(-9.54418838400005,11.6,5.55302429599998));
#251677=CARTESIAN_POINT('Ctrl Pts',(-9.54728816200006,15.2,5.55354730899998));
#251678=CARTESIAN_POINT('Ctrl Pts',(-9.54728816200006,11.6,5.55354730899998));
#251679=CARTESIAN_POINT('Ctrl Pts',(-9.55039348900005,15.2,5.55406867699999));
#251680=CARTESIAN_POINT('Ctrl Pts',(-9.55039348900005,11.6,5.55406867699999));
#251681=CARTESIAN_POINT('Ctrl Pts',(-9.55350435500005,15.2,5.55458838999999));
#251682=CARTESIAN_POINT('Ctrl Pts',(-9.55350435500005,11.6,5.55458838999999));
#251683=CARTESIAN_POINT('Ctrl Pts',(-9.55662075600006,15.2,5.55510644099999));
#251684=CARTESIAN_POINT('Ctrl Pts',(-9.55662075600006,11.6,5.55510644099999));
#251685=CARTESIAN_POINT('Ctrl Pts',(-9.55974268200006,15.2,5.55562282199999));
#251686=CARTESIAN_POINT('Ctrl Pts',(-9.55974268200006,11.6,5.55562282199999));
#251687=CARTESIAN_POINT('Ctrl Pts',(-9.56287012600006,15.2,5.55613752299998));
#251688=CARTESIAN_POINT('Ctrl Pts',(-9.56287012600006,11.6,5.55613752299998));
#251689=CARTESIAN_POINT('Ctrl Pts',(-9.56600308000005,15.2,5.55665053699999));
#251690=CARTESIAN_POINT('Ctrl Pts',(-9.56600308000005,11.6,5.55665053699999));
#251691=CARTESIAN_POINT('Ctrl Pts',(-9.56914153600006,15.2,5.55716185399999));
#251692=CARTESIAN_POINT('Ctrl Pts',(-9.56914153600006,11.6,5.55716185399999));
#251693=CARTESIAN_POINT('Ctrl Pts',(-9.57228548800006,15.2,5.55767146699999));
#251694=CARTESIAN_POINT('Ctrl Pts',(-9.57228548800006,11.6,5.55767146699999));
#251695=CARTESIAN_POINT('Ctrl Pts',(-9.57543492600006,15.2,5.55817936699999));
#251696=CARTESIAN_POINT('Ctrl Pts',(-9.57543492600006,11.6,5.55817936699999));
#251697=CARTESIAN_POINT('Ctrl Pts',(-9.57858984400006,15.2,5.55868554599999));
#251698=CARTESIAN_POINT('Ctrl Pts',(-9.57858984400006,11.6,5.55868554599999));
#251699=CARTESIAN_POINT('Ctrl Pts',(-9.58175023400005,15.2,5.55918999599999));
#251700=CARTESIAN_POINT('Ctrl Pts',(-9.58175023400005,11.6,5.55918999599999));
#251701=CARTESIAN_POINT('Ctrl Pts',(-9.58491608900006,15.2,5.55969270699999));
#251702=CARTESIAN_POINT('Ctrl Pts',(-9.58491608900006,11.6,5.55969270699999));
#251703=CARTESIAN_POINT('Ctrl Pts',(-9.58808740100006,15.2,5.56019367399998));
#251704=CARTESIAN_POINT('Ctrl Pts',(-9.58808740100006,11.6,5.56019367399998));
#251705=CARTESIAN_POINT('Ctrl Pts',(-9.59126416200006,15.2,5.56069288399998));
#251706=CARTESIAN_POINT('Ctrl Pts',(-9.59126416200006,11.6,5.56069288399998));
#251707=CARTESIAN_POINT('Ctrl Pts',(-9.59444636500006,15.2,5.56119033399998));
#251708=CARTESIAN_POINT('Ctrl Pts',(-9.59444636500006,11.6,5.56119033399998));
#251709=CARTESIAN_POINT('Ctrl Pts',(-9.59763400200006,15.2,5.56168601199998));
#251710=CARTESIAN_POINT('Ctrl Pts',(-9.59763400200006,11.6,5.56168601199998));
#251711=CARTESIAN_POINT('Ctrl Pts',(-9.60082706500006,15.2,5.56217991099999));
#251712=CARTESIAN_POINT('Ctrl Pts',(-9.60082706500006,11.6,5.56217991099999));
#251713=CARTESIAN_POINT('Ctrl Pts',(-9.60402554800006,15.2,5.56267202299999));
#251714=CARTESIAN_POINT('Ctrl Pts',(-9.60402554800006,11.6,5.56267202299999));
#251715=CARTESIAN_POINT('Ctrl Pts',(-9.60722944200005,15.2,5.56316234099998));
#251716=CARTESIAN_POINT('Ctrl Pts',(-9.60722944200005,11.6,5.56316234099998));
#251717=CARTESIAN_POINT('Ctrl Pts',(-9.61043874100006,15.2,5.56365085399998));
#251718=CARTESIAN_POINT('Ctrl Pts',(-9.61043874100006,11.6,5.56365085399998));
#251719=CARTESIAN_POINT('Ctrl Pts',(-9.61365343600006,15.2,5.56413755599999));
#251720=CARTESIAN_POINT('Ctrl Pts',(-9.61365343600006,11.6,5.56413755599999));
#251721=CARTESIAN_POINT('Ctrl Pts',(-9.61687352100006,15.2,5.56462243899999));
#251722=CARTESIAN_POINT('Ctrl Pts',(-9.61687352100006,11.6,5.56462243899999));
#251723=CARTESIAN_POINT('Ctrl Pts',(-9.62009898600006,15.2,5.56510549499999));
#251724=CARTESIAN_POINT('Ctrl Pts',(-9.62009898600006,11.6,5.56510549499999));
#251725=CARTESIAN_POINT('Ctrl Pts',(-9.62332982600006,15.2,5.56558671499998));
#251726=CARTESIAN_POINT('Ctrl Pts',(-9.62332982600006,11.6,5.56558671499998));
#251727=CARTESIAN_POINT('Ctrl Pts',(-9.62656603200006,15.2,5.56606609099998));
#251728=CARTESIAN_POINT('Ctrl Pts',(-9.62656603200006,11.6,5.56606609099998));
#251729=CARTESIAN_POINT('Ctrl Pts',(-9.62980759800006,15.2,5.56654361499999));
#251730=CARTESIAN_POINT('Ctrl Pts',(-9.62980759800006,11.6,5.56654361499999));
#251731=CARTESIAN_POINT('Ctrl Pts',(-9.63305451500006,15.2,5.56701928099999));
#251732=CARTESIAN_POINT('Ctrl Pts',(-9.63305451500006,11.6,5.56701928099999));
#251733=CARTESIAN_POINT('Ctrl Pts',(-9.63630677600005,15.2,5.56749307899998));
#251734=CARTESIAN_POINT('Ctrl Pts',(-9.63630677600005,11.6,5.56749307899998));
#251735=CARTESIAN_POINT('Ctrl Pts',(-9.63956437500006,15.2,5.56796500199999));
#251736=CARTESIAN_POINT('Ctrl Pts',(-9.63956437500006,11.6,5.56796500199999));
#251737=CARTESIAN_POINT('Ctrl Pts',(-9.64282730300006,15.2,5.56843504199998));
#251738=CARTESIAN_POINT('Ctrl Pts',(-9.64282730300006,11.6,5.56843504199998));
#251739=CARTESIAN_POINT('Ctrl Pts',(-9.64609555300006,15.2,5.56890318999999));
#251740=CARTESIAN_POINT('Ctrl Pts',(-9.64609555300006,11.6,5.56890318999999));
#251741=CARTESIAN_POINT('Ctrl Pts',(-9.64936911700006,15.2,5.56936944099998));
#251742=CARTESIAN_POINT('Ctrl Pts',(-9.64936911700006,11.6,5.56936944099998));
#251743=CARTESIAN_POINT('Ctrl Pts',(-9.65264798900006,15.2,5.56983378399998));
#251744=CARTESIAN_POINT('Ctrl Pts',(-9.65264798900006,11.6,5.56983378399998));
#251745=CARTESIAN_POINT('Ctrl Pts',(-9.65593215900006,15.2,5.57029621199998));
#251746=CARTESIAN_POINT('Ctrl Pts',(-9.65593215900006,11.6,5.57029621199998));
#251747=CARTESIAN_POINT('Ctrl Pts',(-9.65922162400006,15.2,5.57075671799999));
#251748=CARTESIAN_POINT('Ctrl Pts',(-9.65922162400006,11.6,5.57075671799999));
#251749=CARTESIAN_POINT('Ctrl Pts',(-9.66251637200006,15.2,5.57121529599998));
#251750=CARTESIAN_POINT('Ctrl Pts',(-9.66251637200006,11.6,5.57121529599998));
#251751=CARTESIAN_POINT('Ctrl Pts',(-9.66581639800006,15.2,5.57167193399999));
#251752=CARTESIAN_POINT('Ctrl Pts',(-9.66581639800006,11.6,5.57167193399999));
#251753=CARTESIAN_POINT('Ctrl Pts',(-9.66912169500005,15.2,5.57212662699998));
#251754=CARTESIAN_POINT('Ctrl Pts',(-9.66912169500005,11.6,5.57212662699998));
#251755=CARTESIAN_POINT('Ctrl Pts',(-9.67243225500006,15.2,5.57257936599999));
#251756=CARTESIAN_POINT('Ctrl Pts',(-9.67243225500006,11.6,5.57257936599999));
#251757=CARTESIAN_POINT('Ctrl Pts',(-9.67574806900006,15.2,5.57303014499999));
#251758=CARTESIAN_POINT('Ctrl Pts',(-9.67574806900006,11.6,5.57303014499999));
#251759=CARTESIAN_POINT('Ctrl Pts',(-9.67906913300006,15.2,5.57347895599998));
#251760=CARTESIAN_POINT('Ctrl Pts',(-9.67906913300006,11.6,5.57347895599998));
#251761=CARTESIAN_POINT('Ctrl Pts',(-9.68239543700006,15.2,5.57392579099999));
#251762=CARTESIAN_POINT('Ctrl Pts',(-9.68239543700006,11.6,5.57392579099999));
#251763=CARTESIAN_POINT('Ctrl Pts',(-9.68572697500005,15.2,5.57437064099998));
#251764=CARTESIAN_POINT('Ctrl Pts',(-9.68572697500005,11.6,5.57437064099998));
#251765=CARTESIAN_POINT('Ctrl Pts',(-9.68906374000005,15.2,5.57481349999998));
#251766=CARTESIAN_POINT('Ctrl Pts',(-9.68906374000005,11.6,5.57481349999998));
#251767=CARTESIAN_POINT('Ctrl Pts',(-9.69240572300006,15.2,5.57525436099999));
#251768=CARTESIAN_POINT('Ctrl Pts',(-9.69240572300006,11.6,5.57525436099999));
#251769=CARTESIAN_POINT('Ctrl Pts',(-9.69575291800006,15.2,5.57569321499999));
#251770=CARTESIAN_POINT('Ctrl Pts',(-9.69575291800006,11.6,5.57569321499999));
#251771=CARTESIAN_POINT('Ctrl Pts',(-9.69910531700006,15.2,5.57613005499999));
#251772=CARTESIAN_POINT('Ctrl Pts',(-9.69910531700006,11.6,5.57613005499999));
#251773=CARTESIAN_POINT('Ctrl Pts',(-9.70246291400005,15.2,5.57656487399999));
#251774=CARTESIAN_POINT('Ctrl Pts',(-9.70246291400005,11.6,5.57656487399999));
#251775=CARTESIAN_POINT('Ctrl Pts',(-9.70582569900006,15.2,5.57699766299999));
#251776=CARTESIAN_POINT('Ctrl Pts',(-9.70582569900006,11.6,5.57699766299999));
#251777=CARTESIAN_POINT('Ctrl Pts',(-9.70919366900005,15.2,5.57742841599998));
#251778=CARTESIAN_POINT('Ctrl Pts',(-9.70919366900005,11.6,5.57742841599998));
#251779=CARTESIAN_POINT('Ctrl Pts',(-9.71256681200006,15.2,5.57785712499999));
#251780=CARTESIAN_POINT('Ctrl Pts',(-9.71256681200006,11.6,5.57785712499999));
#251781=CARTESIAN_POINT('Ctrl Pts',(-9.71594512500005,15.2,5.57828378299998));
#251782=CARTESIAN_POINT('Ctrl Pts',(-9.71594512500005,11.6,5.57828378299998));
#251783=CARTESIAN_POINT('Ctrl Pts',(-9.71932859800006,15.2,5.57870838199998));
#251784=CARTESIAN_POINT('Ctrl Pts',(-9.71932859800006,11.6,5.57870838199998));
#251785=CARTESIAN_POINT('Ctrl Pts',(-9.72271722500006,15.2,5.57913091399998));
#251786=CARTESIAN_POINT('Ctrl Pts',(-9.72271722500006,11.6,5.57913091399998));
#251787=CARTESIAN_POINT('Ctrl Pts',(-9.72611099800006,15.2,5.57955137399999));
#251788=CARTESIAN_POINT('Ctrl Pts',(-9.72611099800006,11.6,5.57955137399999));
#251789=CARTESIAN_POINT('Ctrl Pts',(-9.72950991000006,15.2,5.57996975199998));
#251790=CARTESIAN_POINT('Ctrl Pts',(-9.72950991000006,11.6,5.57996975199998));
#251791=CARTESIAN_POINT('Ctrl Pts',(-9.73291395500006,15.2,5.58038604299998));
#251792=CARTESIAN_POINT('Ctrl Pts',(-9.73291395500006,11.6,5.58038604299998));
#251793=CARTESIAN_POINT('Ctrl Pts',(-9.73632312400006,15.2,5.58080023799998));
#251794=CARTESIAN_POINT('Ctrl Pts',(-9.73632312400006,11.6,5.58080023799998));
#251795=CARTESIAN_POINT('Ctrl Pts',(-9.73973741000006,15.2,5.58121232999999));
#251796=CARTESIAN_POINT('Ctrl Pts',(-9.73973741000006,11.6,5.58121232999999));
#251797=CARTESIAN_POINT('Ctrl Pts',(-9.74315680900006,15.2,5.58162231199999));
#251798=CARTESIAN_POINT('Ctrl Pts',(-9.74315680900006,11.6,5.58162231199999));
#251799=CARTESIAN_POINT('Ctrl Pts',(-9.74658130800006,15.2,5.58203017699999));
#251800=CARTESIAN_POINT('Ctrl Pts',(-9.74658130800006,11.6,5.58203017699999));
#251801=CARTESIAN_POINT('Ctrl Pts',(-9.75001090500006,15.2,5.58243591699998));
#251802=CARTESIAN_POINT('Ctrl Pts',(-9.75001090500006,11.6,5.58243591699998));
#251803=CARTESIAN_POINT('Ctrl Pts',(-9.75344559100006,15.2,5.58283952599999));
#251804=CARTESIAN_POINT('Ctrl Pts',(-9.75344559100006,11.6,5.58283952599999));
#251805=CARTESIAN_POINT('Ctrl Pts',(-9.75688535800005,15.2,5.58324099599999));
#251806=CARTESIAN_POINT('Ctrl Pts',(-9.75688535800005,11.6,5.58324099599999));
#251807=CARTESIAN_POINT('Ctrl Pts',(-9.76033020000006,15.2,5.58364031899998));
#251808=CARTESIAN_POINT('Ctrl Pts',(-9.76033020000006,11.6,5.58364031899998));
#251809=CARTESIAN_POINT('Ctrl Pts',(-9.76378010900006,15.2,5.58403748999999));
#251810=CARTESIAN_POINT('Ctrl Pts',(-9.76378010900006,11.6,5.58403748999999));
#251811=CARTESIAN_POINT('Ctrl Pts',(-9.76723507900006,15.2,5.58443249899998));
#251812=CARTESIAN_POINT('Ctrl Pts',(-9.76723507900006,11.6,5.58443249899998));
#251813=CARTESIAN_POINT('Ctrl Pts',(-9.77069510200005,15.2,5.58482534199998));
#251814=CARTESIAN_POINT('Ctrl Pts',(-9.77069510200005,11.6,5.58482534199998));
#251815=CARTESIAN_POINT('Ctrl Pts',(-9.77416017100006,15.2,5.58521600999998));
#251816=CARTESIAN_POINT('Ctrl Pts',(-9.77416017100006,11.6,5.58521600999998));
#251817=CARTESIAN_POINT('Ctrl Pts',(-9.77763027800006,15.2,5.58560449599998));
#251818=CARTESIAN_POINT('Ctrl Pts',(-9.77763027800006,11.6,5.58560449599998));
#251819=CARTESIAN_POINT('Ctrl Pts',(-9.78110541800006,15.2,5.58599079299999));
#251820=CARTESIAN_POINT('Ctrl Pts',(-9.78110541800006,11.6,5.58599079299999));
#251821=CARTESIAN_POINT('Ctrl Pts',(-9.78458558400006,15.2,5.58637489499999));
#251822=CARTESIAN_POINT('Ctrl Pts',(-9.78458558400006,11.6,5.58637489499999));
#251823=CARTESIAN_POINT('Ctrl Pts',(-9.78807076600006,15.2,5.58675679399999));
#251824=CARTESIAN_POINT('Ctrl Pts',(-9.78807076600006,11.6,5.58675679399999));
#251825=CARTESIAN_POINT('Ctrl Pts',(-9.79156095900005,15.2,5.58713648399999));
#251826=CARTESIAN_POINT('Ctrl Pts',(-9.79156095900005,11.6,5.58713648399999));
#251827=CARTESIAN_POINT('Ctrl Pts',(-9.79505615600005,15.2,5.58751395499999));
#251828=CARTESIAN_POINT('Ctrl Pts',(-9.79505615600005,11.6,5.58751395499999));
#251829=CARTESIAN_POINT('Ctrl Pts',(-9.79855634900006,15.2,5.58788920399999));
#251830=CARTESIAN_POINT('Ctrl Pts',(-9.79855634900006,11.6,5.58788920399999));
#251831=CARTESIAN_POINT('Ctrl Pts',(-9.80206153200006,15.2,5.58826222199999));
#251832=CARTESIAN_POINT('Ctrl Pts',(-9.80206153200006,11.6,5.58826222199999));
#251833=CARTESIAN_POINT('Ctrl Pts',(-9.80557169700005,15.2,5.58863300199998));
#251834=CARTESIAN_POINT('Ctrl Pts',(-9.80557169700005,11.6,5.58863300199998));
#251835=CARTESIAN_POINT('Ctrl Pts',(-9.80908683800006,15.2,5.58900153799998));
#251836=CARTESIAN_POINT('Ctrl Pts',(-9.80908683800006,11.6,5.58900153799998));
#251837=CARTESIAN_POINT('Ctrl Pts',(-9.81260694600006,15.2,5.58936782199999));
#251838=CARTESIAN_POINT('Ctrl Pts',(-9.81260694600006,11.6,5.58936782199999));
#251839=CARTESIAN_POINT('Ctrl Pts',(-9.81613201600006,15.2,5.58973184899998));
#251840=CARTESIAN_POINT('Ctrl Pts',(-9.81613201600006,11.6,5.58973184899998));
#251841=CARTESIAN_POINT('Ctrl Pts',(-9.81966204100006,15.2,5.59009360999998));
#251842=CARTESIAN_POINT('Ctrl Pts',(-9.81966204100006,11.6,5.59009360999998));
#251843=CARTESIAN_POINT('Ctrl Pts',(-9.82319701200005,15.2,5.59045309799998));
#251844=CARTESIAN_POINT('Ctrl Pts',(-9.82319701200005,11.6,5.59045309799998));
#251845=CARTESIAN_POINT('Ctrl Pts',(-9.82673692500006,15.2,5.59081030799998));
#251846=CARTESIAN_POINT('Ctrl Pts',(-9.82673692500006,11.6,5.59081030799998));
#251847=CARTESIAN_POINT('Ctrl Pts',(-9.83028177000006,15.2,5.59116523399998));
#251848=CARTESIAN_POINT('Ctrl Pts',(-9.83028177000006,11.6,5.59116523399998));
#251849=CARTESIAN_POINT('Ctrl Pts',(-9.83383154200006,15.2,5.59151786499999));
#251850=CARTESIAN_POINT('Ctrl Pts',(-9.83383154200006,11.6,5.59151786499999));
#251851=CARTESIAN_POINT('Ctrl Pts',(-9.83738623300006,15.2,5.59186819799999));
#251852=CARTESIAN_POINT('Ctrl Pts',(-9.83738623300006,11.6,5.59186819799999));
#251853=CARTESIAN_POINT('Ctrl Pts',(-9.84094583600006,15.2,5.59221622599999));
#251854=CARTESIAN_POINT('Ctrl Pts',(-9.84094583600006,11.6,5.59221622599999));
#251855=CARTESIAN_POINT('Ctrl Pts',(-9.84451034500006,15.2,5.59256193999998));
#251856=CARTESIAN_POINT('Ctrl Pts',(-9.84451034500006,11.6,5.59256193999998));
#251857=CARTESIAN_POINT('Ctrl Pts',(-9.84807975200006,15.2,5.59290533499999));
#251858=CARTESIAN_POINT('Ctrl Pts',(-9.84807975200006,11.6,5.59290533499999));
#251859=CARTESIAN_POINT('Ctrl Pts',(-9.85165405100006,15.2,5.59324640399999));
#251860=CARTESIAN_POINT('Ctrl Pts',(-9.85165405100006,11.6,5.59324640399999));
#251861=CARTESIAN_POINT('Ctrl Pts',(-9.85523323300006,15.2,5.59358514099999));
#251862=CARTESIAN_POINT('Ctrl Pts',(-9.85523323300006,11.6,5.59358514099999));
#251863=CARTESIAN_POINT('Ctrl Pts',(-9.85881729400005,15.2,5.59392153799998));
#251864=CARTESIAN_POINT('Ctrl Pts',(-9.85881729400005,11.6,5.59392153799998));
#251865=CARTESIAN_POINT('Ctrl Pts',(-9.86240622600006,15.2,5.59425558899999));
#251866=CARTESIAN_POINT('Ctrl Pts',(-9.86240622600006,11.6,5.59425558899999));
#251867=CARTESIAN_POINT('Ctrl Pts',(-9.86600002100005,15.2,5.59458728699998));
#251868=CARTESIAN_POINT('Ctrl Pts',(-9.86600002100005,11.6,5.59458728699998));
#251869=CARTESIAN_POINT('Ctrl Pts',(-9.86959867100006,15.2,5.59491662699998));
#251870=CARTESIAN_POINT('Ctrl Pts',(-9.86959867100006,11.6,5.59491662699998));
#251871=CARTESIAN_POINT('Ctrl Pts',(-9.87320217400006,15.2,5.59524360099999));
#251872=CARTESIAN_POINT('Ctrl Pts',(-9.87320217400006,11.6,5.59524360099999));
#251873=CARTESIAN_POINT('Ctrl Pts',(-9.87681051700006,15.2,5.59556820099999));
#251874=CARTESIAN_POINT('Ctrl Pts',(-9.87681051700006,11.6,5.59556820099999));
#251875=CARTESIAN_POINT('Ctrl Pts',(-9.88042369800005,15.2,5.59589042299999));
#251876=CARTESIAN_POINT('Ctrl Pts',(-9.88042369800005,11.6,5.59589042299999));
#251877=CARTESIAN_POINT('Ctrl Pts',(-9.88404170800005,15.2,5.59621025999999));
#251878=CARTESIAN_POINT('Ctrl Pts',(-9.88404170800005,11.6,5.59621025999999));
#251879=CARTESIAN_POINT('Ctrl Pts',(-9.88766454000006,15.2,5.59652770399998));
#251880=CARTESIAN_POINT('Ctrl Pts',(-9.88766454000006,11.6,5.59652770399998));
#251881=CARTESIAN_POINT('Ctrl Pts',(-9.89129218700005,15.2,5.59684274999999));
#251882=CARTESIAN_POINT('Ctrl Pts',(-9.89129218700005,11.6,5.59684274999999));
#251883=CARTESIAN_POINT('Ctrl Pts',(-9.89492464300006,15.2,5.59715539099999));
#251884=CARTESIAN_POINT('Ctrl Pts',(-9.89492464300006,11.6,5.59715539099999));
#251885=CARTESIAN_POINT('Ctrl Pts',(-9.89856190100006,15.2,5.59746561999999));
#251886=CARTESIAN_POINT('Ctrl Pts',(-9.89856190100006,11.6,5.59746561999999));
#251887=CARTESIAN_POINT('Ctrl Pts',(-9.90220395200006,15.2,5.59777343199999));
#251888=CARTESIAN_POINT('Ctrl Pts',(-9.90220395200006,11.6,5.59777343199999));
#251889=CARTESIAN_POINT('Ctrl Pts',(-9.90585079300006,15.2,5.59807881899999));
#251890=CARTESIAN_POINT('Ctrl Pts',(-9.90585079300006,11.6,5.59807881899999));
#251891=CARTESIAN_POINT('Ctrl Pts',(-9.90950241400006,15.2,5.59838177499999));
#251892=CARTESIAN_POINT('Ctrl Pts',(-9.90950241400006,11.6,5.59838177499999));
#251893=CARTESIAN_POINT('Ctrl Pts',(-9.91315881000006,15.2,5.59868229499998));
#251894=CARTESIAN_POINT('Ctrl Pts',(-9.91315881000006,11.6,5.59868229499998));
#251895=CARTESIAN_POINT('Ctrl Pts',(-9.91681997300006,15.2,5.59898036999999));
#251896=CARTESIAN_POINT('Ctrl Pts',(-9.91681997300006,11.6,5.59898036999999));
#251897=CARTESIAN_POINT('Ctrl Pts',(-9.92048589700006,15.2,5.59927599599998));
#251898=CARTESIAN_POINT('Ctrl Pts',(-9.92048589700006,11.6,5.59927599599998));
#251899=CARTESIAN_POINT('Ctrl Pts',(-9.92415657500005,15.2,5.59956916599998));
#251900=CARTESIAN_POINT('Ctrl Pts',(-9.92415657500005,11.6,5.59956916599998));
#251901=CARTESIAN_POINT('Ctrl Pts',(-9.92783199800006,15.2,5.59985987199998));
#251902=CARTESIAN_POINT('Ctrl Pts',(-9.92783199800006,11.6,5.59985987199998));
#251903=CARTESIAN_POINT('Ctrl Pts',(-9.93151216200006,15.2,5.60014810999999));
#251904=CARTESIAN_POINT('Ctrl Pts',(-9.93151216200006,11.6,5.60014810999999));
#251905=CARTESIAN_POINT('Ctrl Pts',(-9.93519706000006,15.2,5.60043387199999));
#251906=CARTESIAN_POINT('Ctrl Pts',(-9.93519706000006,11.6,5.60043387199999));
#251907=CARTESIAN_POINT('Ctrl Pts',(-9.93888668400006,15.2,5.60071715299999));
#251908=CARTESIAN_POINT('Ctrl Pts',(-9.93888668400006,11.6,5.60071715299999));
#251909=CARTESIAN_POINT('Ctrl Pts',(-9.94258102800006,15.2,5.60099794499998));
#251910=CARTESIAN_POINT('Ctrl Pts',(-9.94258102800006,11.6,5.60099794499998));
#251911=CARTESIAN_POINT('Ctrl Pts',(-9.94628008500005,15.2,5.60127624499999));
#251912=CARTESIAN_POINT('Ctrl Pts',(-9.94628008500005,11.6,5.60127624499999));
#251913=CARTESIAN_POINT('Ctrl Pts',(-9.94998384800006,15.2,5.60155204399998));
#251914=CARTESIAN_POINT('Ctrl Pts',(-9.94998384800006,11.6,5.60155204399998));
#251915=CARTESIAN_POINT('Ctrl Pts',(-9.95369231100005,15.2,5.60182533599999));
#251916=CARTESIAN_POINT('Ctrl Pts',(-9.95369231100005,11.6,5.60182533599999));
#251917=CARTESIAN_POINT('Ctrl Pts',(-9.95740546800005,15.2,5.60209611699998));
#251918=CARTESIAN_POINT('Ctrl Pts',(-9.95740546800005,11.6,5.60209611699998));
#251919=CARTESIAN_POINT('Ctrl Pts',(-9.96112331000005,15.2,5.60236437799999));
#251920=CARTESIAN_POINT('Ctrl Pts',(-9.96112331000005,11.6,5.60236437799999));
#251921=CARTESIAN_POINT('Ctrl Pts',(-9.96484583100005,15.2,5.60263011399999));
#251922=CARTESIAN_POINT('Ctrl Pts',(-9.96484583100005,11.6,5.60263011399999));
#251923=CARTESIAN_POINT('Ctrl Pts',(-9.96857302300005,15.2,5.60289331699998));
#251924=CARTESIAN_POINT('Ctrl Pts',(-9.96857302300005,11.6,5.60289331699998));
#251925=CARTESIAN_POINT('Ctrl Pts',(-9.97230488000006,15.2,5.60315398299998));
#251926=CARTESIAN_POINT('Ctrl Pts',(-9.97230488000006,11.6,5.60315398299998));
#251927=CARTESIAN_POINT('Ctrl Pts',(-9.97604139600006,15.2,5.60341210499999));
#251928=CARTESIAN_POINT('Ctrl Pts',(-9.97604139600006,11.6,5.60341210499999));
#251929=CARTESIAN_POINT('Ctrl Pts',(-9.97978256300006,15.2,5.60366767599999));
#251930=CARTESIAN_POINT('Ctrl Pts',(-9.97978256300006,11.6,5.60366767599999));
#251931=CARTESIAN_POINT('Ctrl Pts',(-9.98352837700006,15.2,5.60392069199998));
#251932=CARTESIAN_POINT('Ctrl Pts',(-9.98352837700006,11.6,5.60392069199998));
#251933=CARTESIAN_POINT('Ctrl Pts',(-9.98727883000005,15.2,5.60417114799999));
#251934=CARTESIAN_POINT('Ctrl Pts',(-9.98727883000005,11.6,5.60417114799999));
#251935=CARTESIAN_POINT('Ctrl Pts',(-9.99103391600006,15.2,5.60441903699999));
#251936=CARTESIAN_POINT('Ctrl Pts',(-9.99103391600006,11.6,5.60441903699999));
#251937=CARTESIAN_POINT('Ctrl Pts',(-9.99479363100006,15.2,5.60466435399999));
#251938=CARTESIAN_POINT('Ctrl Pts',(-9.99479363100006,11.6,5.60466435399999));
#251939=CARTESIAN_POINT('Ctrl Pts',(-9.99855796500006,15.2,5.60490709199998));
#251940=CARTESIAN_POINT('Ctrl Pts',(-9.99855796500006,11.6,5.60490709199998));
#251941=CARTESIAN_POINT('Ctrl Pts',(-10.0023269120001,15.2,5.60514724399999));
#251942=CARTESIAN_POINT('Ctrl Pts',(-10.0023269120001,11.6,5.60514724399999));
#251943=CARTESIAN_POINT('Ctrl Pts',(-10.0061004630001,15.2,5.60538480399998));
#251944=CARTESIAN_POINT('Ctrl Pts',(-10.0061004630001,11.6,5.60538480399998));
#251945=CARTESIAN_POINT('Ctrl Pts',(-10.0098786100001,15.2,5.60561976299999));
#251946=CARTESIAN_POINT('Ctrl Pts',(-10.0098786100001,11.6,5.60561976299999));
#251947=CARTESIAN_POINT('Ctrl Pts',(-10.0136613450001,15.2,5.60585211399999));
#251948=CARTESIAN_POINT('Ctrl Pts',(-10.0136613450001,11.6,5.60585211399999));
#251949=CARTESIAN_POINT('Ctrl Pts',(-10.0174486610001,15.2,5.60608185199998));
#251950=CARTESIAN_POINT('Ctrl Pts',(-10.0174486610001,11.6,5.60608185199998));
#251951=CARTESIAN_POINT('Ctrl Pts',(-10.0212405510001,15.2,5.60630896999999));
#251952=CARTESIAN_POINT('Ctrl Pts',(-10.0212405510001,11.6,5.60630896999999));
#251953=CARTESIAN_POINT('Ctrl Pts',(-10.0250370120001,15.2,5.60653346399998));
#251954=CARTESIAN_POINT('Ctrl Pts',(-10.0250370120001,11.6,5.60653346399998));
#251955=CARTESIAN_POINT('Ctrl Pts',(-10.0288380390001,15.2,5.60675533199999));
#251956=CARTESIAN_POINT('Ctrl Pts',(-10.0288380390001,11.6,5.60675533199999));
#251957=CARTESIAN_POINT('Ctrl Pts',(-10.0326436310001,15.2,5.60697457399999));
#251958=CARTESIAN_POINT('Ctrl Pts',(-10.0326436310001,11.6,5.60697457399999));
#251959=CARTESIAN_POINT('Ctrl Pts',(-10.0356917560001,15.2,5.60714786299998));
#251960=CARTESIAN_POINT('Ctrl Pts',(-10.0356917560001,11.6,5.60714786299998));
#251961=CARTESIAN_POINT('Ctrl Pts',(-10.0379799050001,15.2,5.60727664799998));
#251962=CARTESIAN_POINT('Ctrl Pts',(-10.0379799050001,11.6,5.60727664799998));
#251963=CARTESIAN_POINT('Ctrl Pts',(-10.0395062490001,15.2,5.60736197799999));
#251964=CARTESIAN_POINT('Ctrl Pts',(-10.0395062490001,11.6,5.60736197799999));
#251965=CARTESIAN_POINT('Ctrl Pts',(-10.0402696490001,15.2,5.60740451199998));
#251966=CARTESIAN_POINT('Ctrl Pts',(-10.0402696490001,11.6,5.60740451199998));
#251967=CARTESIAN_POINT('Ctrl Pts',(-8.88241603300006,15.2,5.36127880599999));
#251968=CARTESIAN_POINT('Ctrl Pts',(-8.8840193341511,15.2,5.36206719179848));
#251969=CARTESIAN_POINT('Ctrl Pts',(-8.88567631015408,15.2,5.36287598639576));
#251970=CARTESIAN_POINT('Ctrl Pts',(-8.88738636482935,15.2,5.36370417391758));
#251971=CARTESIAN_POINT('Ctrl Pts',(-8.88910466625265,15.2,5.36453635537826));
#251972=CARTESIAN_POINT('Ctrl Pts',(-8.89087656219126,15.2,5.3653881201172));
#251973=CARTESIAN_POINT('Ctrl Pts',(-8.89270147763497,15.2,5.36625847962586));
#251974=CARTESIAN_POINT('Ctrl Pts',(-8.89452639291292,15.2,5.36712883905549));
#251975=CARTESIAN_POINT('Ctrl Pts',(-8.89640432653677,15.2,5.36801779327457));
#251976=CARTESIAN_POINT('Ctrl Pts',(-8.89833471396663,15.2,5.36892438099162));
#251977=CARTESIAN_POINT('Ctrl Pts',(-8.90026510139648,15.2,5.36983096870868));
#251978=CARTESIAN_POINT('Ctrl Pts',(-8.90224794602853,15.2,5.37075519315545));
#251979=CARTESIAN_POINT('Ctrl Pts',(-8.90428269455326,15.2,5.37169612091731));
#251980=CARTESIAN_POINT('Ctrl Pts',(-8.9063174432628,15.2,5.37263704876463));
#251981=CARTESIAN_POINT('Ctrl Pts',(-8.90840409854633,15.2,5.3735946808436));
#251982=CARTESIAN_POINT('Ctrl Pts',(-8.91054211949969,15.2,5.3745681138144));
#251983=CARTESIAN_POINT('Ctrl Pts',(-8.91268014025887,15.2,5.37554154669679));
#251984=CARTESIAN_POINT('Ctrl Pts',(-8.9148695309971,15.2,5.37653078096564));
#251985=CARTESIAN_POINT('Ctrl Pts',(-8.91710976450932,15.2,5.37753493976708));
#251986=CARTESIAN_POINT('Ctrl Pts',(-8.91934999802154,15.2,5.37853909856852));
#251987=CARTESIAN_POINT('Ctrl Pts',(-8.9216410736932,15.2,5.37955817934021));
#251988=CARTESIAN_POINT('Ctrl Pts',(-8.92398248010591,15.2,5.38059133421871));
#251989=CARTESIAN_POINT('Ctrl Pts',(-8.9263238867313,15.2,5.38162448919106));
#251990=CARTESIAN_POINT('Ctrl Pts',(-8.92871562071298,15.2,5.38267171465686));
#251991=CARTESIAN_POINT('Ctrl Pts',(-8.93115718351611,15.2,5.38373218388222));
#251992=CARTESIAN_POINT('Ctrl Pts',(-8.93359874609746,15.2,5.38479265301127));
#251993=CARTESIAN_POINT('Ctrl Pts',(-8.93609013543712,15.2,5.38586636418146));
#251994=CARTESIAN_POINT('Ctrl Pts',(-8.93863085909698,15.2,5.38695251530921));
#251995=CARTESIAN_POINT('Ctrl Pts',(-8.94117158275683,15.2,5.38803866643696));
#251996=CARTESIAN_POINT('Ctrl Pts',(-8.94376164087935,15.2,5.38913725323035));
#251997=CARTESIAN_POINT('Ctrl Pts',(-8.94640055236469,15.2,5.39024749468951));
#251998=CARTESIAN_POINT('Ctrl Pts',(-8.94903946385004,15.2,5.39135773614867));
#251999=CARTESIAN_POINT('Ctrl Pts',(-8.95172722664611,15.2,5.39247963140172));
#252000=CARTESIAN_POINT('Ctrl Pts',(-8.95446336946008,15.2,5.39361241785983));
#252001=CARTESIAN_POINT('Ctrl Pts',(-8.95765553624206,15.2,5.39493400212955));
#252002=CARTESIAN_POINT('Ctrl Pts',(-8.96091355247342,15.2,5.39627040849422));
#252003=CARTESIAN_POINT('Ctrl Pts',(-8.96423668332827,15.2,5.39762046069527));
#252004=CARTESIAN_POINT('Ctrl Pts',(-8.967085081056,15.2,5.39877764823612));
#252005=CARTESIAN_POINT('Ctrl Pts',(-8.96998131859761,15.2,5.39994486170677));
#252006=CARTESIAN_POINT('Ctrl Pts',(-8.97292494140413,15.2,5.4011213804134));
#252007=CARTESIAN_POINT('Ctrl Pts',(-8.97586856447803,15.2,5.4022978992269));
#252008=CARTESIAN_POINT('Ctrl Pts',(-8.97885957476477,15.2,5.40348372275796));
#252009=CARTESIAN_POINT('Ctrl Pts',(-8.98189752393241,15.2,5.40467814957344));
#252010=CARTESIAN_POINT('Ctrl Pts',(-8.98493547282408,15.2,5.40587257628041));
#252011=CARTESIAN_POINT('Ctrl Pts',(-8.98802036337031,15.2,5.40707560607001));
#252012=CARTESIAN_POINT('Ctrl Pts',(-8.99115175533785,15.2,5.40828655294234));
#252013=CARTESIAN_POINT('Ctrl Pts',(-8.99428314730538,15.2,5.40949749981467));
#252014=CARTESIAN_POINT('Ctrl Pts',(-8.99746104273554,15.2,5.41071636728638));
#252015=CARTESIAN_POINT('Ctrl Pts',(-9.00068501061524,15.2,5.41194248232466));
#252016=CARTESIAN_POINT('Ctrl Pts',(-9.0039089787878,15.2,5.41316859747432));
#252017=CARTESIAN_POINT('Ctrl Pts',(-9.00717902037317,15.2,5.41440196469138));
#252018=CARTESIAN_POINT('Ctrl Pts',(-9.01049471063921,15.2,5.41564192884258));
#252019=CARTESIAN_POINT('Ctrl Pts',(-9.01381040060406,15.2,5.41688189288116));
#252020=CARTESIAN_POINT('Ctrl Pts',(-9.01717174178186,15.2,5.41812845637257));
#252021=CARTESIAN_POINT('Ctrl Pts',(-9.02057831675677,15.2,5.41938098149941));
#252022=CARTESIAN_POINT('Ctrl Pts',(-9.0239848917317,15.2,5.42063350662624));
#252023=CARTESIAN_POINT('Ctrl Pts',(-9.02743670019061,15.2,5.42189199456684));
#252024=CARTESIAN_POINT('Ctrl Pts',(-9.03093333414386,15.2,5.42315582460389));
#252025=CARTESIAN_POINT('Ctrl Pts',(-9.03501274063439,15.2,5.42463029305699));
#252026=CARTESIAN_POINT('Ctrl Pts',(-9.03915315896396,15.2,5.4261120307306));
#252027=CARTESIAN_POINT('Ctrl Pts',(-9.04335394800668,15.2,5.4276000780244));
#252028=CARTESIAN_POINT('Ctrl Pts',(-9.04695462414212,15.2,5.42887554706717));
#252029=CARTESIAN_POINT('Ctrl Pts',(-9.05059965708492,15.2,5.4301556494736));
#252030=CARTESIAN_POINT('Ctrl Pts',(-9.05428864911456,15.2,5.43143979959334));
#252031=CARTESIAN_POINT('Ctrl Pts',(-9.05797764147928,15.2,5.43272394982973));
#252032=CARTESIAN_POINT('Ctrl Pts',(-9.06171059490176,15.2,5.43401214355649));
#252033=CARTESIAN_POINT('Ctrl Pts',(-9.06548711663208,15.2,5.43530380785827));
#252034=CARTESIAN_POINT('Ctrl Pts',(-9.06863421790251,15.2,5.43638019471775));
#252035=CARTESIAN_POINT('Ctrl Pts',(-9.07181157594484,15.2,5.43745898891341));
#252036=CARTESIAN_POINT('Ctrl Pts',(-9.07501896941952,15.2,5.43853986669136));
#252037=CARTESIAN_POINT('Ctrl Pts',(-9.07822636289421,15.2,5.43962074446931));
#252038=CARTESIAN_POINT('Ctrl Pts',(-9.08146379045268,15.2,5.44070370348617));
#252039=CARTESIAN_POINT('Ctrl Pts',(-9.08473103163568,15.2,5.44178842466686));
#252040=CARTESIAN_POINT('Ctrl Pts',(-9.08799827246255,15.2,5.44287314572932));
#252041=CARTESIAN_POINT('Ctrl Pts',(-9.09129532991322,15.2,5.44395962790417));
#252042=CARTESIAN_POINT('Ctrl Pts',(-9.09462198308987,15.2,5.44504755584101));
#252043=CARTESIAN_POINT('Ctrl Pts',(-9.09794863662913,15.2,5.44613548389646));
#252044=CARTESIAN_POINT('Ctrl Pts',(-9.1013048866151,15.2,5.44722485939632));
#252045=CARTESIAN_POINT('Ctrl Pts',(-9.10469051855715,15.2,5.44831537154901));
#252046=CARTESIAN_POINT('Ctrl Pts',(-9.10807615049921,15.2,5.44940588370169));
#252047=CARTESIAN_POINT('Ctrl Pts',(-9.11149116577466,15.2,5.45049753384086));
#252048=CARTESIAN_POINT('Ctrl Pts',(-9.11493534962527,15.2,5.4515900168815));
#252049=CARTESIAN_POINT('Ctrl Pts',(-9.11837953347588,15.2,5.45268249992214));
#252050=CARTESIAN_POINT('Ctrl Pts',(-9.12185288680039,15.2,5.45377581741736));
#252051=CARTESIAN_POINT('Ctrl Pts',(-9.12535520027111,15.2,5.45486966894511));
#252052=CARTESIAN_POINT('Ctrl Pts',(-9.13025843920647,15.2,5.45640106110782));
#252053=CARTESIAN_POINT('Ctrl Pts',(-9.1352184345454,15.2,5.45793350401421));
#252054=CARTESIAN_POINT('Ctrl Pts',(-9.14023462424361,15.2,5.45946619351725));
#252055=CARTESIAN_POINT('Ctrl Pts',(-9.14381761682939,15.2,5.46056097171666));
#252056=CARTESIAN_POINT('Ctrl Pts',(-9.14742927608118,15.2,5.46165587709381));
#252057=CARTESIAN_POINT('Ctrl Pts',(-9.15106940122156,15.2,5.46275062278825));
#252058=CARTESIAN_POINT('Ctrl Pts',(-9.15470952636195,15.2,5.46384536848269));
#252059=CARTESIAN_POINT('Ctrl Pts',(-9.15837811395712,15.2,5.46493995644377));
#252060=CARTESIAN_POINT('Ctrl Pts',(-9.16207496354193,15.2,5.46603410380488));
#252061=CARTESIAN_POINT('Ctrl Pts',(-9.16577181312675,15.2,5.46712825116596));
#252062=CARTESIAN_POINT('Ctrl Pts',(-9.16949692343519,15.2,5.46822195863343));
#252063=CARTESIAN_POINT('Ctrl Pts',(-9.17325009473577,15.2,5.4693149509102));
#252064=CARTESIAN_POINT('Ctrl Pts',(-9.17700326603634,15.2,5.47040794318698));
#252065=CARTESIAN_POINT('Ctrl Pts',(-9.18078449731264,15.2,5.47150021794281));
#252066=CARTESIAN_POINT('Ctrl Pts',(-9.18459359023155,15.2,5.47259150690106));
#252067=CARTESIAN_POINT('Ctrl Pts',(-9.18840268315046,15.2,5.47368279585931));
#252068=CARTESIAN_POINT('Ctrl Pts',(-9.19223963767545,15.2,5.47477309839254));
#252069=CARTESIAN_POINT('Ctrl Pts',(-9.19610425649715,15.2,5.47586214589244));
#252070=CARTESIAN_POINT('Ctrl Pts',(-9.19996887531887,15.2,5.47695119339233));
#252071=CARTESIAN_POINT('Ctrl Pts',(-9.20386115931602,15.2,5.47803898688665));
#252072=CARTESIAN_POINT('Ctrl Pts',(-9.2077809137627,15.2,5.47912526515041));
#252073=CARTESIAN_POINT('Ctrl Pts',(-9.21170066778212,15.2,5.48021154329576));
#252074=CARTESIAN_POINT('Ctrl Pts',(-9.21564789101556,15.2,5.48129630575956));
#252075=CARTESIAN_POINT('Ctrl Pts',(-9.2196223909968,15.2,5.48237929314167));
#252076=CARTESIAN_POINT('Ctrl Pts',(-9.22359689141125,15.2,5.48346228064183));
#252077=CARTESIAN_POINT('Ctrl Pts',(-9.22759866970303,15.2,5.48454349429199));
#252078=CARTESIAN_POINT('Ctrl Pts',(-9.23162753192301,15.2,5.4856226801255));
#252079=CARTESIAN_POINT('Ctrl Pts',(-9.23485062187466,15.2,5.48648602883934));
#252080=CARTESIAN_POINT('Ctrl Pts',(-9.23809104747093,15.2,5.48734807932755));
#252081=CARTESIAN_POINT('Ctrl Pts',(-9.24134871055221,15.2,5.48820870526724));
#252082=CARTESIAN_POINT('Ctrl Pts',(-9.24460637318962,15.2,5.48906933108967));
#252083=CARTESIAN_POINT('Ctrl Pts',(-9.2478812721132,15.2,5.48992853026584));
#252084=CARTESIAN_POINT('Ctrl Pts',(-9.25117331345341,15.2,5.49078617758477));
#252085=CARTESIAN_POINT('Ctrl Pts',(-9.25528836546509,15.2,5.49185823682106));
#252086=CARTESIAN_POINT('Ctrl Pts',(-9.2594301986347,15.2,5.49292787173243));
#252087=CARTESIAN_POINT('Ctrl Pts',(-9.26359862897977,15.2,5.49399483763543));
#252088=CARTESIAN_POINT('Ctrl Pts',(-9.26693337343756,15.2,5.49484841040436));
#252089=CARTESIAN_POINT('Ctrl Pts',(-9.27028513977554,15.2,5.49570027665594));
#252090=CARTESIAN_POINT('Ctrl Pts',(-9.2736538317523,15.2,5.49655031148391));
#252091=CARTESIAN_POINT('Ctrl Pts',(-9.27786469649376,15.2,5.49761285496097));
#252092=CARTESIAN_POINT('Ctrl Pts',(-9.28210201062762,15.2,5.49867253875812));
#252093=CARTESIAN_POINT('Ctrl Pts',(-9.28636558625399,15.2,5.49972912632741));
#252094=CARTESIAN_POINT('Ctrl Pts',(-9.28977644647625,15.2,5.50057439631374));
#252095=CARTESIAN_POINT('Ctrl Pts',(-9.29320411645626,15.2,5.50141768526991));
#252096=CARTESIAN_POINT('Ctrl Pts',(-9.2966485012285,15.2,5.50225887264579));
#252097=CARTESIAN_POINT('Ctrl Pts',(-9.30009288647004,15.2,5.50310006013629));
#252098=CARTESIAN_POINT('Ctrl Pts',(-9.30355398711643,15.2,5.50393914794005));
#252099=CARTESIAN_POINT('Ctrl Pts',(-9.3070317097107,15.2,5.50477601676723));
#252100=CARTESIAN_POINT('Ctrl Pts',(-9.31137886271662,15.2,5.5058221027442));
#252101=CARTESIAN_POINT('Ctrl Pts',(-9.31575198956426,15.2,5.50686472074589));
#252102=CARTESIAN_POINT('Ctrl Pts',(-9.32015090678784,15.2,5.50790364755125));
#252103=CARTESIAN_POINT('Ctrl Pts',(-9.32367004027901,15.2,5.5087347889276));
#252104=CARTESIAN_POINT('Ctrl Pts',(-9.32720568088073,15.2,5.50956356600996));
#252105=CARTESIAN_POINT('Ctrl Pts',(-9.33075773764424,15.2,5.51038986483156));
#252106=CARTESIAN_POINT('Ctrl Pts',(-9.33608582351545,15.2,5.51162931323283));
#252107=CARTESIAN_POINT('Ctrl Pts',(-9.34145084384792,15.2,5.51286318764083));
#252108=CARTESIAN_POINT('Ctrl Pts',(-9.34685249299762,15.2,5.5140911041021));
#252109=CARTESIAN_POINT('Ctrl Pts',(-9.35045359194011,15.2,5.51490971496473));
#252110=CARTESIAN_POINT('Ctrl Pts',(-9.35407097008452,15.2,5.51572568043034));
#252111=CARTESIAN_POINT('Ctrl Pts',(-9.3577045374531,15.2,5.51653888664182));
#252112=CARTESIAN_POINT('Ctrl Pts',(-9.36224649703511,15.2,5.51755539448927));
#252113=CARTESIAN_POINT('Ctrl Pts',(-9.36681375162889,15.2,5.51856759314494));
#252114=CARTESIAN_POINT('Ctrl Pts',(-9.37140612718314,15.2,5.51957526765906));
#252115=CARTESIAN_POINT('Ctrl Pts',(-9.37599850273737,15.2,5.5205829421732));
#252116=CARTESIAN_POINT('Ctrl Pts',(-9.38061600008199,15.2,5.52158609492269));
#252117=CARTESIAN_POINT('Ctrl Pts',(-9.38525844475581,15.2,5.52258451277446));
#252118=CARTESIAN_POINT('Ctrl Pts',(-9.39082937816199,15.2,5.52378261415306));
#252119=CARTESIAN_POINT('Ctrl Pts',(-9.39643623350076,15.2,5.52497389872179));
#252120=CARTESIAN_POINT('Ctrl Pts',(-9.40207871787664,15.2,5.52615800809593));
#252121=CARTESIAN_POINT('Ctrl Pts',(-9.40584037446891,15.2,5.52694741441706));
#252122=CARTESIAN_POINT('Ctrl Pts',(-9.40961786491746,15.2,5.52773363270154));
#252123=CARTESIAN_POINT('Ctrl Pts',(-9.41341110225258,15.2,5.5285165576922));
#252124=CARTESIAN_POINT('Ctrl Pts',(-9.41720433907087,15.2,5.52929948257618));
#252125=CARTESIAN_POINT('Ctrl Pts',(-9.42101332216117,15.2,5.53007911368064));
#252126=CARTESIAN_POINT('Ctrl Pts',(-9.42483796562467,15.2,5.53085534917308));
#252127=CARTESIAN_POINT('Ctrl Pts',(-9.42866260960928,15.2,5.5316315847713));
#252128=CARTESIAN_POINT('Ctrl Pts',(-9.43250291429818,15.2,5.53240442385252));
#252129=CARTESIAN_POINT('Ctrl Pts',(-9.43635879100832,15.2,5.53317376478333));
#252130=CARTESIAN_POINT('Ctrl Pts',(-9.44021466771848,15.2,5.53394310571416));
#252131=CARTESIAN_POINT('Ctrl Pts',(-9.44408611958045,15.2,5.534708947764));
#252132=CARTESIAN_POINT('Ctrl Pts',(-9.44797305762719,15.2,5.53547119141629));
#252133=CARTESIAN_POINT('Ctrl Pts',(-9.45185999514433,15.2,5.53623343496472));
#252134=CARTESIAN_POINT('Ctrl Pts',(-9.45576242035266,15.2,5.53699207853553));
#252135=CARTESIAN_POINT('Ctrl Pts',(-9.45968024777233,15.2,5.53774702403282));
#252136=CARTESIAN_POINT('Ctrl Pts',(-9.46359807572581,15.2,5.53850196963296));
#252137=CARTESIAN_POINT('Ctrl Pts',(-9.46753130613716,15.2,5.53925321680131));
#252138=CARTESIAN_POINT('Ctrl Pts',(-9.47147985285392,15.2,5.54000066589721));
#252139=CARTESIAN_POINT('Ctrl Pts',(-9.4754283990327,15.2,5.54074811489126));
#252140=CARTESIAN_POINT('Ctrl Pts',(-9.47939226200669,15.2,5.54149176726915));
#252141=CARTESIAN_POINT('Ctrl Pts',(-9.48337135812485,15.2,5.54223152493116));
#252142=CARTESIAN_POINT('Ctrl Pts',(-9.48735045478516,15.2,5.54297128269394));
#252143=CARTESIAN_POINT('Ctrl Pts',(-9.49134478324729,15.2,5.54370714589795));
#252144=CARTESIAN_POINT('Ctrl Pts',(-9.49535426057792,15.2,5.54443901882646));
#252145=CARTESIAN_POINT('Ctrl Pts',(-9.49936373736225,15.2,5.54517089165525));
#252146=CARTESIAN_POINT('Ctrl Pts',(-9.5033883624131,15.2,5.54589877369539));
#252147=CARTESIAN_POINT('Ctrl Pts',(-9.50742805267223,15.2,5.54662256889495));
#252148=CARTESIAN_POINT('Ctrl Pts',(-9.51146774348178,15.2,5.54734636419314));
#252149=CARTESIAN_POINT('Ctrl Pts',(-9.51552249876285,15.2,5.54806607493641));
#252150=CARTESIAN_POINT('Ctrl Pts',(-9.51959223604117,15.2,5.54878160530846));
#252151=CARTESIAN_POINT('Ctrl Pts',(-9.52467940736183,15.2,5.54967601822477));
#252152=CARTESIAN_POINT('Ctrl Pts',(-9.52978998560691,15.2,5.55056390072461));
#252153=CARTESIAN_POINT('Ctrl Pts',(-9.53492381276089,15.2,5.55144507030759));
#252154=CARTESIAN_POINT('Ctrl Pts',(-9.53903087414833,15.2,5.55215000591636));
#252155=CARTESIAN_POINT('Ctrl Pts',(-9.54315281303538,15.2,5.55285064471792));
#252156=CARTESIAN_POINT('Ctrl Pts',(-9.54728954862481,15.2,5.55354689764061));
#252157=CARTESIAN_POINT('Ctrl Pts',(-9.55142628477788,15.2,5.55424315065817));
#252158=CARTESIAN_POINT('Ctrl Pts',(-9.55557781577106,15.2,5.55493501498843));
#252159=CARTESIAN_POINT('Ctrl Pts',(-9.5597440618324,15.2,5.55562240208115));
#252160=CARTESIAN_POINT('Ctrl Pts',(-9.5639103073261,15.2,5.55630978908022));
#252161=CARTESIAN_POINT('Ctrl Pts',(-9.56809126674741,15.2,5.55699269764686));
#252162=CARTESIAN_POINT('Ctrl Pts',(-9.57228685884736,15.2,5.55767103864743));
#252163=CARTESIAN_POINT('Ctrl Pts',(-9.57648245151896,15.2,5.55834937974042));
#252164=CARTESIAN_POINT('Ctrl Pts',(-9.5806926758923,15.2,5.55902315322764));
#252165=CARTESIAN_POINT('Ctrl Pts',(-9.58491745325288,15.2,5.55969227093379));
#252166=CARTESIAN_POINT('Ctrl Pts',(-9.58914223003784,15.2,5.56036138854878));
#252167=CARTESIAN_POINT('Ctrl Pts',(-9.59338155894819,15.2,5.56102585002058));
#252168=CARTESIAN_POINT('Ctrl Pts',(-9.59763535782118,15.2,5.5616855671338));
#252169=CARTESIAN_POINT('Ctrl Pts',(-9.60188915727375,15.2,5.56234528433691));
#252170=CARTESIAN_POINT('Ctrl Pts',(-9.60615742795827,15.2,5.56300025864234));
#252171=CARTESIAN_POINT('Ctrl Pts',(-9.610440090025,15.2,5.56365040123334));
#252172=CARTESIAN_POINT('Ctrl Pts',(-9.61579341731665,15.2,5.56446307942779));
#252173=CARTESIAN_POINT('Ctrl Pts',(-9.6211692296617,15.2,5.56526821231906));
#252174=CARTESIAN_POINT('Ctrl Pts',(-9.62656737197794,15.2,5.5660656280171));
#252175=CARTESIAN_POINT('Ctrl Pts',(-9.63088588547791,15.2,5.56670356052339));
#252176=CARTESIAN_POINT('Ctrl Pts',(-9.63521868980163,15.2,5.56733655680093));
#252177=CARTESIAN_POINT('Ctrl Pts',(-9.63956570655594,15.2,5.567964531139));
#252178=CARTESIAN_POINT('Ctrl Pts',(-9.64499947794302,15.2,5.56874949912575));
#252179=CARTESIAN_POINT('Ctrl Pts',(-9.65045545383529,15.2,5.56952662064318));
#252180=CARTESIAN_POINT('Ctrl Pts',(-9.65593348195848,15.2,5.57029573140773));
#252181=CARTESIAN_POINT('Ctrl Pts',(-9.66141151008166,15.2,5.57106484217227));
#252182=CARTESIAN_POINT('Ctrl Pts',(-9.66691159019583,15.2,5.57182594516328));
#252183=CARTESIAN_POINT('Ctrl Pts',(-9.67243356790073,15.2,5.57257887589591));
#252184=CARTESIAN_POINT('Ctrl Pts',(-9.67574675440329,15.2,5.57303063431907));
#252185=CARTESIAN_POINT('Ctrl Pts',(-9.67906782442966,15.2,5.5734794528186));
#252186=CARTESIAN_POINT('Ctrl Pts',(-9.68239674476597,15.2,5.57392529467781));
#252187=CARTESIAN_POINT('Ctrl Pts',(-9.68572566570703,15.2,5.57437113661801));
#252188=CARTESIAN_POINT('Ctrl Pts',(-9.68906243780864,15.2,5.57481400246571));
#252189=CARTESIAN_POINT('Ctrl Pts',(-9.69240702671247,15.2,5.57525385936256));
#252190=CARTESIAN_POINT('Ctrl Pts',(-9.69798134074204,15.2,5.5759869540841));
#252191=CARTESIAN_POINT('Ctrl Pts',(-9.70357736993304,15.2,5.57671168781106));
#252192=CARTESIAN_POINT('Ctrl Pts',(-9.70919496305979,15.2,5.57742790510202));
#252193=CARTESIAN_POINT('Ctrl Pts',(-9.71256551881337,15.2,5.57785763546099));
#252194=CARTESIAN_POINT('Ctrl Pts',(-9.71594383767483,15.2,5.57828430039318));
#252195=CARTESIAN_POINT('Ctrl Pts',(-9.71932988713853,15.2,5.57870786535692));
#252196=CARTESIAN_POINT('Ctrl Pts',(-9.72384461955176,15.2,5.57927261861627));
#252197=CARTESIAN_POINT('Ctrl Pts',(-9.72837309423991,15.2,5.57983186257181));
#252198=CARTESIAN_POINT('Ctrl Pts',(-9.73291523564548,15.2,5.58038551897136));
#252199=CARTESIAN_POINT('Ctrl Pts',(-9.73632184185437,15.2,5.58080076128988));
#252200=CARTESIAN_POINT('Ctrl Pts',(-9.73973613509606,15.2,5.58121285979195));
#252201=CARTESIAN_POINT('Ctrl Pts',(-9.74315808334569,15.2,5.58162178265253));
#252202=CARTESIAN_POINT('Ctrl Pts',(-9.74658003221697,15.2,5.58203070558739));
#252203=CARTESIAN_POINT('Ctrl Pts',(-9.75000963559875,15.2,5.58243645244636));
#252204=CARTESIAN_POINT('Ctrl Pts',(-9.75344686201599,15.2,5.58283899133776));
#252205=CARTESIAN_POINT('Ctrl Pts',(-9.7580298295316,15.2,5.58337570973774));
#252206=CARTESIAN_POINT('Ctrl Pts',(-9.76262634811119,15.2,5.58390672355407));
#252207=CARTESIAN_POINT('Ctrl Pts',(-9.7672363422552,15.2,5.58443195745798));
#252208=CARTESIAN_POINT('Ctrl Pts',(-9.7729988354063,15.2,5.58508849989153));
#252209=CARTESIAN_POINT('Ctrl Pts',(-9.77878238241668,15.2,5.58573601107224));
#252210=CARTESIAN_POINT('Ctrl Pts',(-9.78458683804167,15.2,5.58637434426668));
#252211=CARTESIAN_POINT('Ctrl Pts',(-9.78806951129013,15.2,5.58675734416943));
#252212=CARTESIAN_POINT('Ctrl Pts',(-9.79155971034661,15.2,5.58713703992232));
#252213=CARTESIAN_POINT('Ctrl Pts',(-9.79505740463555,15.2,5.58751339940893));
#252214=CARTESIAN_POINT('Ctrl Pts',(-9.79855509892447,15.2,5.58788975889555));
#252215=CARTESIAN_POINT('Ctrl Pts',(-9.80206028787347,15.2,5.5882627834897));
#252216=CARTESIAN_POINT('Ctrl Pts',(-9.80557294029547,15.2,5.58863244091179));
#252217=CARTESIAN_POINT('Ctrl Pts',(-9.81142736121148,15.2,5.58924853663765));
#252218=CARTESIAN_POINT('Ctrl Pts',(-9.81730251137116,15.2,5.58985528088261));
#252219=CARTESIAN_POINT('Ctrl Pts',(-9.82319824706455,15.2,5.59045252845256));
#252220=CARTESIAN_POINT('Ctrl Pts',(-9.82673568835205,15.2,5.5908108769815));
#252221=CARTESIAN_POINT('Ctrl Pts',(-9.83028054023903,15.2,5.59116580881902));
#252222=CARTESIAN_POINT('Ctrl Pts',(-9.83383277098396,15.2,5.59151729039005));
#252223=CARTESIAN_POINT('Ctrl Pts',(-9.83738500237421,15.2,5.59186877202494));
#252224=CARTESIAN_POINT('Ctrl Pts',(-9.84094461235821,15.2,5.59221680625885));
#252225=CARTESIAN_POINT('Ctrl Pts',(-9.84451157029427,15.2,5.59256136030845));
#252226=CARTESIAN_POINT('Ctrl Pts',(-9.84807852758235,15.2,5.59290591429546));
#252227=CARTESIAN_POINT('Ctrl Pts',(-9.8516528322367,15.2,5.59324698964932));
#252228=CARTESIAN_POINT('Ctrl Pts',(-9.85523445310719,15.2,5.59358455605341));
#252229=CARTESIAN_POINT('Ctrl Pts',(-9.85881607397769,15.2,5.59392212245751));
#252230=CARTESIAN_POINT('Ctrl Pts',(-9.86240501283424,15.2,5.5942561790275));
#252231=CARTESIAN_POINT('Ctrl Pts',(-9.86600123480328,15.2,5.59458669747531));
#252232=CARTESIAN_POINT('Ctrl Pts',(-9.8707961972109,15.2,5.59502738871904));
#252233=CARTESIAN_POINT('Ctrl Pts',(-9.87560411176278,15.2,5.59546178820603));
#252234=CARTESIAN_POINT('Ctrl Pts',(-9.88042490447848,15.2,5.59588982667169));
#252235=CARTESIAN_POINT('Ctrl Pts',(-9.88404049983629,15.2,5.59621085559384));
#252236=CARTESIAN_POINT('Ctrl Pts',(-9.88766333854615,15.2,5.59652830585663));
#252237=CARTESIAN_POINT('Ctrl Pts',(-9.89129339003303,15.2,5.59684214881843));
#252238=CARTESIAN_POINT('Ctrl Pts',(-9.89492344086046,15.2,5.5971559917232));
#252239=CARTESIAN_POINT('Ctrl Pts',(-9.8985607045125,15.2,5.59746622689483));
#252240=CARTESIAN_POINT('Ctrl Pts',(-9.90220514983904,15.2,5.59777282580004));
#252241=CARTESIAN_POINT('Ctrl Pts',(-9.90584959516559,15.2,5.59807942470525));
#252242=CARTESIAN_POINT('Ctrl Pts',(-9.90950122296962,15.2,5.59838238684315));
#252243=CARTESIAN_POINT('Ctrl Pts',(-9.91316000177,15.2,5.59868168379195));
#252244=CARTESIAN_POINT('Ctrl Pts',(-9.91681878057039,15.2,5.59898098074075));
#252245=CARTESIAN_POINT('Ctrl Pts',(-9.92048471144682,15.2,5.59927661254234));
#252246=CARTESIAN_POINT('Ctrl Pts',(-9.92415776128833,15.2,5.59956855003307));
#252247=CARTESIAN_POINT('Ctrl Pts',(-9.92905516152187,15.2,5.59995780005608));
#252248=CARTESIAN_POINT('Ctrl Pts',(-9.93396521991586,15.2,5.60034048277779));
#252249=CARTESIAN_POINT('Ctrl Pts',(-9.93888786479654,15.2,5.60071653085316));
#252250=CARTESIAN_POINT('Ctrl Pts',(-9.94257984812169,15.2,5.60099856688407));
#252251=CARTESIAN_POINT('Ctrl Pts',(-9.94627891103813,15.2,5.60127687222351));
#252252=CARTESIAN_POINT('Ctrl Pts',(-9.9499850234041,15.2,5.60155141729654));
#252253=CARTESIAN_POINT('Ctrl Pts',(-9.95369113577006,15.2,5.60182596236957));
#252254=CARTESIAN_POINT('Ctrl Pts',(-9.95740429893828,15.2,5.60209674877543));
#252255=CARTESIAN_POINT('Ctrl Pts',(-9.96112447973672,15.2,5.60236374672525));
#252256=CARTESIAN_POINT('Ctrl Pts',(-9.96484466053517,15.2,5.60263074467508));
#252257=CARTESIAN_POINT('Ctrl Pts',(-9.96857185893203,15.2,5.60289395359133));
#252258=CARTESIAN_POINT('Ctrl Pts',(-9.97230604472995,15.2,5.60315334699977));
#252259=CARTESIAN_POINT('Ctrl Pts',(-9.97728495957944,15.2,5.60349920490911));
#252260=CARTESIAN_POINT('Ctrl Pts',(-9.98227629669971,15.2,5.60383827697025));
#252261=CARTESIAN_POINT('Ctrl Pts',(-9.98727998908478,15.2,5.604170506321));
#252262=CARTESIAN_POINT('Ctrl Pts',(-9.99103275803271,15.2,5.60441967831142));
#252263=CARTESIAN_POINT('Ctrl Pts',(-9.99479247889694,15.2,5.60466500108538));
#252264=CARTESIAN_POINT('Ctrl Pts',(-9.99855911863569,15.2,5.6049064455346));
#252265=CARTESIAN_POINT('Ctrl Pts',(-10.0023257583744,15.2,5.60514788998382));
#252266=CARTESIAN_POINT('Ctrl Pts',(-10.0060993167569,15.2,5.60538545652434));
#252267=CARTESIAN_POINT('Ctrl Pts',(-10.0098797570118,15.2,5.60561911101689));
#252268=CARTESIAN_POINT('Ctrl Pts',(-10.0161804909988,15.2,5.6060085351853));
#252269=CARTESIAN_POINT('Ctrl Pts',(-10.0225003316333,15.2,5.60638708414889));
#252270=CARTESIAN_POINT('Ctrl Pts',(-10.028839180665,15.2,5.6067546754843));
#252271=CARTESIAN_POINT('Ctrl Pts',(-10.0326424899459,15.2,5.60697523027754));
#252272=CARTESIAN_POINT('Ctrl Pts',(-10.0364526481964,15.2,5.60719184195524));
#252273=CARTESIAN_POINT('Ctrl Pts',(-10.0402696490001,15.2,5.60740451199998));
#252274=CARTESIAN_POINT('Ctrl Pts',(-8.88241603300006,12.2,5.36127880599999));
#252275=CARTESIAN_POINT('Ctrl Pts',(-8.8840193341511,12.2,5.36206719179848));
#252276=CARTESIAN_POINT('Ctrl Pts',(-8.88567631015408,12.2,5.36287598639576));
#252277=CARTESIAN_POINT('Ctrl Pts',(-8.88738636482935,12.2,5.36370417391758));
#252278=CARTESIAN_POINT('Ctrl Pts',(-8.88910466625265,12.2,5.36453635537826));
#252279=CARTESIAN_POINT('Ctrl Pts',(-8.89087656219126,12.2,5.3653881201172));
#252280=CARTESIAN_POINT('Ctrl Pts',(-8.89270147763497,12.2,5.36625847962586));
#252281=CARTESIAN_POINT('Ctrl Pts',(-8.89452639291292,12.2,5.36712883905548));
#252282=CARTESIAN_POINT('Ctrl Pts',(-8.89640432653677,12.2,5.36801779327457));
#252283=CARTESIAN_POINT('Ctrl Pts',(-8.89833471396663,12.2,5.36892438099162));
#252284=CARTESIAN_POINT('Ctrl Pts',(-8.90026510139648,12.2,5.36983096870868));
#252285=CARTESIAN_POINT('Ctrl Pts',(-8.90224794602853,12.2,5.37075519315545));
#252286=CARTESIAN_POINT('Ctrl Pts',(-8.90428269455326,12.2,5.37169612091731));
#252287=CARTESIAN_POINT('Ctrl Pts',(-8.9063174432628,12.2,5.37263704876463));
#252288=CARTESIAN_POINT('Ctrl Pts',(-8.90840409854632,12.2,5.3735946808436));
#252289=CARTESIAN_POINT('Ctrl Pts',(-8.91054211949969,12.2,5.3745681138144));
#252290=CARTESIAN_POINT('Ctrl Pts',(-8.91268014025887,12.2,5.37554154669679));
#252291=CARTESIAN_POINT('Ctrl Pts',(-8.9148695309971,12.2,5.37653078096564));
#252292=CARTESIAN_POINT('Ctrl Pts',(-8.91710976450932,12.2,5.37753493976708));
#252293=CARTESIAN_POINT('Ctrl Pts',(-8.91934999802154,12.2,5.37853909856852));
#252294=CARTESIAN_POINT('Ctrl Pts',(-8.9216410736932,12.2,5.37955817934021));
#252295=CARTESIAN_POINT('Ctrl Pts',(-8.92398248010591,12.2,5.38059133421871));
#252296=CARTESIAN_POINT('Ctrl Pts',(-8.9263238867313,12.2,5.38162448919106));
#252297=CARTESIAN_POINT('Ctrl Pts',(-8.92871562071298,12.2,5.38267171465686));
#252298=CARTESIAN_POINT('Ctrl Pts',(-8.93115718351611,12.2,5.38373218388222));
#252299=CARTESIAN_POINT('Ctrl Pts',(-8.93359874609746,12.2,5.38479265301126));
#252300=CARTESIAN_POINT('Ctrl Pts',(-8.93609013543712,12.2,5.38586636418146));
#252301=CARTESIAN_POINT('Ctrl Pts',(-8.93863085909698,12.2,5.38695251530921));
#252302=CARTESIAN_POINT('Ctrl Pts',(-8.94117158275683,12.2,5.38803866643696));
#252303=CARTESIAN_POINT('Ctrl Pts',(-8.94376164087935,12.2,5.38913725323035));
#252304=CARTESIAN_POINT('Ctrl Pts',(-8.94640055236469,12.2,5.39024749468951));
#252305=CARTESIAN_POINT('Ctrl Pts',(-8.94903946385004,12.2,5.39135773614867));
#252306=CARTESIAN_POINT('Ctrl Pts',(-8.95172722664611,12.2,5.39247963140172));
#252307=CARTESIAN_POINT('Ctrl Pts',(-8.95446336946008,12.2,5.39361241785983));
#252308=CARTESIAN_POINT('Ctrl Pts',(-8.95765553624206,12.2,5.39493400212955));
#252309=CARTESIAN_POINT('Ctrl Pts',(-8.96091355247342,12.2,5.39627040849422));
#252310=CARTESIAN_POINT('Ctrl Pts',(-8.96423668332826,12.2,5.39762046069527));
#252311=CARTESIAN_POINT('Ctrl Pts',(-8.967085081056,12.2,5.39877764823612));
#252312=CARTESIAN_POINT('Ctrl Pts',(-8.96998131859761,12.2,5.39994486170677));
#252313=CARTESIAN_POINT('Ctrl Pts',(-8.97292494140413,12.2,5.4011213804134));
#252314=CARTESIAN_POINT('Ctrl Pts',(-8.97586856447803,12.2,5.4022978992269));
#252315=CARTESIAN_POINT('Ctrl Pts',(-8.97885957476478,12.2,5.40348372275796));
#252316=CARTESIAN_POINT('Ctrl Pts',(-8.98189752393241,12.2,5.40467814957344));
#252317=CARTESIAN_POINT('Ctrl Pts',(-8.98493547282408,12.2,5.40587257628041));
#252318=CARTESIAN_POINT('Ctrl Pts',(-8.9880203633703,12.2,5.40707560607));
#252319=CARTESIAN_POINT('Ctrl Pts',(-8.99115175533783,12.2,5.40828655294233));
#252320=CARTESIAN_POINT('Ctrl Pts',(-8.99428314730537,12.2,5.40949749981466));
#252321=CARTESIAN_POINT('Ctrl Pts',(-8.99746104273554,12.2,5.41071636728638));
#252322=CARTESIAN_POINT('Ctrl Pts',(-9.00068501061524,12.2,5.41194248232466));
#252323=CARTESIAN_POINT('Ctrl Pts',(-9.0039089787878,12.2,5.41316859747432));
#252324=CARTESIAN_POINT('Ctrl Pts',(-9.00717902037317,12.2,5.41440196469138));
#252325=CARTESIAN_POINT('Ctrl Pts',(-9.01049471063921,12.2,5.41564192884258));
#252326=CARTESIAN_POINT('Ctrl Pts',(-9.01381040060406,12.2,5.41688189288116));
#252327=CARTESIAN_POINT('Ctrl Pts',(-9.01717174178186,12.2,5.41812845637257));
#252328=CARTESIAN_POINT('Ctrl Pts',(-9.02057831675677,12.2,5.41938098149941));
#252329=CARTESIAN_POINT('Ctrl Pts',(-9.0239848917317,12.2,5.42063350662624));
#252330=CARTESIAN_POINT('Ctrl Pts',(-9.02743670019061,12.2,5.42189199456683));
#252331=CARTESIAN_POINT('Ctrl Pts',(-9.03093333414385,12.2,5.42315582460389));
#252332=CARTESIAN_POINT('Ctrl Pts',(-9.03442996841472,12.2,5.42441965475574));
#252333=CARTESIAN_POINT('Ctrl Pts',(-9.03797142664485,12.2,5.42568882635657));
#252334=CARTESIAN_POINT('Ctrl Pts',(-9.04155730810531,12.2,5.42696273282322));
#252335=CARTESIAN_POINT('Ctrl Pts',(-9.04514318924006,12.2,5.42823663917418));
#252336=CARTESIAN_POINT('Ctrl Pts',(-9.0487734905418,12.2,5.42951528046325));
#252337=CARTESIAN_POINT('Ctrl Pts',(-9.05244781849163,12.2,5.43079806474998));
#252338=CARTESIAN_POINT('Ctrl Pts',(-9.05612214644144,12.2,5.43208084903669));
#252339=CARTESIAN_POINT('Ctrl Pts',(-9.05984049951241,12.2,5.43336777709109));
#252340=CARTESIAN_POINT('Ctrl Pts',(-9.0636024876445,12.2,5.43465826760849));
#252341=CARTESIAN_POINT('Ctrl Pts',(-9.06673747786849,12.2,5.43573367641205));
#252342=CARTESIAN_POINT('Ctrl Pts',(-9.06990276764833,12.2,5.4368115602628));
#252343=CARTESIAN_POINT('Ctrl Pts',(-9.07309813854951,12.2,5.43789159213769));
#252344=CARTESIAN_POINT('Ctrl Pts',(-9.0762935094507,12.2,5.43897162401257));
#252345=CARTESIAN_POINT('Ctrl Pts',(-9.0795189588944,12.2,5.44005380197364));
#252346=CARTESIAN_POINT('Ctrl Pts',(-9.08277426583726,12.2,5.4411378056541));
#252347=CARTESIAN_POINT('Ctrl Pts',(-9.08602957278013,12.2,5.44222180933455));
#252348=CARTESIAN_POINT('Ctrl Pts',(-9.08931473773876,12.2,5.44330763819446));
#252349=CARTESIAN_POINT('Ctrl Pts',(-9.09262954448984,12.2,5.44439497528272));
#252350=CARTESIAN_POINT('Ctrl Pts',(-9.09594435124093,12.2,5.44548231237099));
#252351=CARTESIAN_POINT('Ctrl Pts',(-9.09928879714441,12.2,5.44657115890554));
#252352=CARTESIAN_POINT('Ctrl Pts',(-9.10266266749165,12.2,5.44766120355832));
#252353=CARTESIAN_POINT('Ctrl Pts',(-9.10603653783888,12.2,5.4487512482111));
#252354=CARTESIAN_POINT('Ctrl Pts',(-9.10943983401953,12.2,5.44984249250673));
#252355=CARTESIAN_POINT('Ctrl Pts',(-9.11287234174352,12.2,5.45093462973391));
#252356=CARTESIAN_POINT('Ctrl Pts',(-9.11630484946751,12.2,5.45202676696109));
#252357=CARTESIAN_POINT('Ctrl Pts',(-9.11976656842696,12.2,5.45311979833815));
#252358=CARTESIAN_POINT('Ctrl Pts',(-9.12325728947012,12.2,5.45421342458818));
#252359=CARTESIAN_POINT('Ctrl Pts',(-9.12674801051328,12.2,5.4553070508382));
#252360=CARTESIAN_POINT('Ctrl Pts',(-9.13026773159184,12.2,5.45640127216045));
#252361=CARTESIAN_POINT('Ctrl Pts',(-9.13381624673223,12.2,5.4574957928549));
#252362=CARTESIAN_POINT('Ctrl Pts',(-9.13736476187261,12.2,5.45859031354936));
#252363=CARTESIAN_POINT('Ctrl Pts',(-9.14094206901435,12.2,5.45968513642239));
#252364=CARTESIAN_POINT('Ctrl Pts',(-9.14454796287701,12.2,5.46077997043541));
#252365=CARTESIAN_POINT('Ctrl Pts',(-9.14815385673968,12.2,5.46187480444844));
#252366=CARTESIAN_POINT('Ctrl Pts',(-9.15178833831566,12.2,5.4629696498654));
#252367=CARTESIAN_POINT('Ctrl Pts',(-9.15545120047076,12.2,5.46406422389316));
#252368=CARTESIAN_POINT('Ctrl Pts',(-9.15911406262587,12.2,5.46515879792092));
#252369=CARTESIAN_POINT('Ctrl Pts',(-9.16280530921198,12.2,5.46625310067644));
#252370=CARTESIAN_POINT('Ctrl Pts',(-9.16652473601983,12.2,5.46734685213471));
#252371=CARTESIAN_POINT('Ctrl Pts',(-9.17098804802709,12.2,5.46865935383697));
#252372=CARTESIAN_POINT('Ctrl Pts',(-9.17549193793619,12.2,5.46997106231907));
#252373=CARTESIAN_POINT('Ctrl Pts',(-9.18003606418948,12.2,5.47128150410474));
#252374=CARTESIAN_POINT('Ctrl Pts',(-9.18382283620483,12.2,5.4723735389658));
#252375=CARTESIAN_POINT('Ctrl Pts',(-9.18763754887222,12.2,5.47346469435466));
#252376=CARTESIAN_POINT('Ctrl Pts',(-9.1914800049848,12.2,5.47455470331293));
#252377=CARTESIAN_POINT('Ctrl Pts',(-9.19609095215236,12.2,5.47586271401534));
#252378=CARTESIAN_POINT('Ctrl Pts',(-9.20074184915,12.2,5.47716906939287));
#252379=CARTESIAN_POINT('Ctrl Pts',(-9.20543235847785,12.2,5.4784733181789));
#252380=CARTESIAN_POINT('Ctrl Pts',(-9.20934111639308,12.2,5.47956019220676));
#252381=CARTESIAN_POINT('Ctrl Pts',(-9.21327738395769,12.2,5.48064560236669));
#252382=CARTESIAN_POINT('Ctrl Pts',(-9.21724096598949,12.2,5.48172928973273));
#252383=CARTESIAN_POINT('Ctrl Pts',(-9.22120454802129,12.2,5.48281297709876));
#252384=CARTESIAN_POINT('Ctrl Pts',(-9.22519544564443,12.2,5.48389494081666));
#252385=CARTESIAN_POINT('Ctrl Pts',(-9.22921346682499,12.2,5.48497492748332));
#252386=CARTESIAN_POINT('Ctrl Pts',(-9.23242788394462,12.2,5.48583891686375));
#252387=CARTESIAN_POINT('Ctrl Pts',(-9.23565965883015,12.2,5.4867016407468));
#252388=CARTESIAN_POINT('Ctrl Pts',(-9.23890869723122,12.2,5.48756297084915));
#252389=CARTESIAN_POINT('Ctrl Pts',(-9.24296999456853,12.2,5.48863963330106));
#252390=CARTESIAN_POINT('Ctrl Pts',(-9.24705826189028,12.2,5.48971411846532));
#252391=CARTESIAN_POINT('Ctrl Pts',(-9.25117331345342,12.2,5.49078617758477));
#252392=CARTESIAN_POINT('Ctrl Pts',(-9.25446535524217,12.2,5.49164382502054));
#252393=CARTESIAN_POINT('Ctrl Pts',(-9.25777453643259,12.2,5.4924999212062));
#252394=CARTESIAN_POINT('Ctrl Pts',(-9.26110076422498,12.2,5.49335433997499));
#252395=CARTESIAN_POINT('Ctrl Pts',(-9.26442699201738,12.2,5.49420875874378));
#252396=CARTESIAN_POINT('Ctrl Pts',(-9.2677702645923,12.2,5.4950615013957));
#252397=CARTESIAN_POINT('Ctrl Pts',(-9.27113048833273,12.2,5.49591244416412));
#252398=CARTESIAN_POINT('Ctrl Pts',(-9.27449071161533,12.2,5.49676338681659));
#252399=CARTESIAN_POINT('Ctrl Pts',(-9.27786788317086,12.2,5.49761252921759));
#252400=CARTESIAN_POINT('Ctrl Pts',(-9.28126191246435,12.2,5.49845975054108));
#252401=CARTESIAN_POINT('Ctrl Pts',(-9.28465594222028,12.2,5.49930697198001));
#252402=CARTESIAN_POINT('Ctrl Pts',(-9.28806682625804,12.2,5.50015227183102));
#252403=CARTESIAN_POINT('Ctrl Pts',(-9.29149447283542,12.2,5.50099553065453));
#252404=CARTESIAN_POINT('Ctrl Pts',(-9.2949221189458,12.2,5.50183878936316));
#252405=CARTESIAN_POINT('Ctrl Pts',(-9.29836652696233,12.2,5.50268000568594));
#252406=CARTESIAN_POINT('Ctrl Pts',(-9.30182760423387,12.2,5.50351906367305));
#252407=CARTESIAN_POINT('Ctrl Pts',(-9.30528868197698,12.2,5.50435812177448));
#252408=CARTESIAN_POINT('Ctrl Pts',(-9.30876642736289,12.2,5.50519502032855));
#252409=CARTESIAN_POINT('Ctrl Pts',(-9.31226074950713,12.2,5.50602964063776));
#252410=CARTESIAN_POINT('Ctrl Pts',(-9.31575507117526,12.2,5.50686426083325));
#252411=CARTESIAN_POINT('Ctrl Pts',(-9.31926596877066,12.2,5.50769660635815));
#252412=CARTESIAN_POINT('Ctrl Pts',(-9.32279335020345,12.2,5.50852655845712));
#252413=CARTESIAN_POINT('Ctrl Pts',(-9.32632073211684,12.2,5.50935651066919));
#252414=CARTESIAN_POINT('Ctrl Pts',(-9.32986459819609,12.2,5.51018406959484));
#252415=CARTESIAN_POINT('Ctrl Pts',(-9.33342485805786,12.2,5.51100912308408));
#252416=CARTESIAN_POINT('Ctrl Pts',(-9.33698511743456,12.2,5.51183417646092));
#252417=CARTESIAN_POINT('Ctrl Pts',(-9.34056176874994,12.2,5.51265672368185));
#252418=CARTESIAN_POINT('Ctrl Pts',(-9.34415472174539,12.2,5.513476651156));
#252419=CARTESIAN_POINT('Ctrl Pts',(-9.34774767523037,12.2,5.51429657874187));
#252420=CARTESIAN_POINT('Ctrl Pts',(-9.35135693197009,12.2,5.51511388774734));
#252421=CARTESIAN_POINT('Ctrl Pts',(-9.35498239927986,12.2,5.51592846662489));
#252422=CARTESIAN_POINT('Ctrl Pts',(-9.35860786609566,12.2,5.51674304539146));
#252423=CARTESIAN_POINT('Ctrl Pts',(-9.36224954496928,12.2,5.51755489262524));
#252424=CARTESIAN_POINT('Ctrl Pts',(-9.3659073456686,12.2,5.51836390005939));
#252425=CARTESIAN_POINT('Ctrl Pts',(-9.36956514686629,12.2,5.51917290760377));
#252426=CARTESIAN_POINT('Ctrl Pts',(-9.37323906979015,12.2,5.51997907446424));
#252427=CARTESIAN_POINT('Ctrl Pts',(-9.37692902578585,12.2,5.52078229273388));
#252428=CARTESIAN_POINT('Ctrl Pts',(-9.3806189812788,12.2,5.52158551089408));
#252429=CARTESIAN_POINT('Ctrl Pts',(-9.38432497038347,12.2,5.5223857807623));
#252430=CARTESIAN_POINT('Ctrl Pts',(-9.38804690313313,12.2,5.52318299358632));
#252431=CARTESIAN_POINT('Ctrl Pts',(-9.39176883638989,12.2,5.52398020651896));
#252432=CARTESIAN_POINT('Ctrl Pts',(-9.39550671258152,12.2,5.524774363018));
#252433=CARTESIAN_POINT('Ctrl Pts',(-9.39926044650833,12.2,5.52556535728333));
#252434=CARTESIAN_POINT('Ctrl Pts',(-9.40301418043514,12.2,5.52635635154866));
#252435=CARTESIAN_POINT('Ctrl Pts',(-9.40678377028045,12.2,5.52714418344975));
#252436=CARTESIAN_POINT('Ctrl Pts',(-9.41056912887724,12.2,5.52792874843661));
#252437=CARTESIAN_POINT('Ctrl Pts',(-9.4153008263496,12.2,5.52890945450984));
#252438=CARTESIAN_POINT('Ctrl Pts',(-9.42005716142557,12.2,5.52988505483397));
#252439=CARTESIAN_POINT('Ctrl Pts',(-9.42483796562467,12.2,5.53085534917308));
#252440=CARTESIAN_POINT('Ctrl Pts',(-9.42866260960928,12.2,5.5316315847713));
#252441=CARTESIAN_POINT('Ctrl Pts',(-9.43250291429818,12.2,5.53240442385252));
#252442=CARTESIAN_POINT('Ctrl Pts',(-9.43635879100832,12.2,5.53317376478333));
#252443=CARTESIAN_POINT('Ctrl Pts',(-9.44021466771848,12.2,5.53394310571416));
#252444=CARTESIAN_POINT('Ctrl Pts',(-9.44408611958044,12.2,5.534708947764));
#252445=CARTESIAN_POINT('Ctrl Pts',(-9.44797305762718,12.2,5.53547119141629));
#252446=CARTESIAN_POINT('Ctrl Pts',(-9.45185999514432,12.2,5.53623343496471));
#252447=CARTESIAN_POINT('Ctrl Pts',(-9.45576242035266,12.2,5.53699207853553));
#252448=CARTESIAN_POINT('Ctrl Pts',(-9.45968024777233,12.2,5.53774702403282));
#252449=CARTESIAN_POINT('Ctrl Pts',(-9.46359807572581,12.2,5.53850196963296));
#252450=CARTESIAN_POINT('Ctrl Pts',(-9.46753130613716,12.2,5.53925321680131));
#252451=CARTESIAN_POINT('Ctrl Pts',(-9.47147985285392,12.2,5.54000066589721));
#252452=CARTESIAN_POINT('Ctrl Pts',(-9.4754283990327,12.2,5.54074811489126));
#252453=CARTESIAN_POINT('Ctrl Pts',(-9.47939226200669,12.2,5.54149176726915));
#252454=CARTESIAN_POINT('Ctrl Pts',(-9.48337135812485,12.2,5.54223152493116));
#252455=CARTESIAN_POINT('Ctrl Pts',(-9.48735045478516,12.2,5.54297128269394));
#252456=CARTESIAN_POINT('Ctrl Pts',(-9.49134478324729,12.2,5.54370714589795));
#252457=CARTESIAN_POINT('Ctrl Pts',(-9.49535426057792,12.2,5.54443901882646));
#252458=CARTESIAN_POINT('Ctrl Pts',(-9.49936373736225,12.2,5.54517089165525));
#252459=CARTESIAN_POINT('Ctrl Pts',(-9.5033883624131,12.2,5.54589877369539));
#252460=CARTESIAN_POINT('Ctrl Pts',(-9.50742805267223,12.2,5.54662256889495));
#252461=CARTESIAN_POINT('Ctrl Pts',(-9.51146774348177,12.2,5.54734636419314));
#252462=CARTESIAN_POINT('Ctrl Pts',(-9.51552249876285,12.2,5.54806607493641));
#252463=CARTESIAN_POINT('Ctrl Pts',(-9.51959223604117,12.2,5.54878160530846));
#252464=CARTESIAN_POINT('Ctrl Pts',(-9.52467940736183,12.2,5.54967601822477));
#252465=CARTESIAN_POINT('Ctrl Pts',(-9.52978998560691,12.2,5.55056390072461));
#252466=CARTESIAN_POINT('Ctrl Pts',(-9.53492381276089,12.2,5.55144507030759));
#252467=CARTESIAN_POINT('Ctrl Pts',(-9.53903087414833,12.2,5.55215000591636));
#252468=CARTESIAN_POINT('Ctrl Pts',(-9.54315281303538,12.2,5.55285064471792));
#252469=CARTESIAN_POINT('Ctrl Pts',(-9.54728954862481,12.2,5.55354689764061));
#252470=CARTESIAN_POINT('Ctrl Pts',(-9.55142628477788,12.2,5.55424315065817));
#252471=CARTESIAN_POINT('Ctrl Pts',(-9.55557781577105,12.2,5.55493501498843));
#252472=CARTESIAN_POINT('Ctrl Pts',(-9.5597440618324,12.2,5.55562240208115));
#252473=CARTESIAN_POINT('Ctrl Pts',(-9.5639103073261,12.2,5.55630978908022));
#252474=CARTESIAN_POINT('Ctrl Pts',(-9.56809126674741,12.2,5.55699269764686));
#252475=CARTESIAN_POINT('Ctrl Pts',(-9.57228685884736,12.2,5.55767103864743));
#252476=CARTESIAN_POINT('Ctrl Pts',(-9.57648245151896,12.2,5.55834937974042));
#252477=CARTESIAN_POINT('Ctrl Pts',(-9.5806926758923,12.2,5.55902315322764));
#252478=CARTESIAN_POINT('Ctrl Pts',(-9.58491745325288,12.2,5.55969227093379));
#252479=CARTESIAN_POINT('Ctrl Pts',(-9.58914223003784,12.2,5.56036138854878));
#252480=CARTESIAN_POINT('Ctrl Pts',(-9.59338155894819,12.2,5.56102585002058));
#252481=CARTESIAN_POINT('Ctrl Pts',(-9.59763535782118,12.2,5.5616855671338));
#252482=CARTESIAN_POINT('Ctrl Pts',(-9.60188915727375,12.2,5.56234528433691));
#252483=CARTESIAN_POINT('Ctrl Pts',(-9.60615742795827,12.2,5.56300025864234));
#252484=CARTESIAN_POINT('Ctrl Pts',(-9.610440090025,12.2,5.56365040123334));
#252485=CARTESIAN_POINT('Ctrl Pts',(-9.61472275209172,12.2,5.56430054382433));
#252486=CARTESIAN_POINT('Ctrl Pts',(-9.61901980482682,12.2,5.56494585762586));
#252487=CARTESIAN_POINT('Ctrl Pts',(-9.62333116822992,12.2,5.5655862541047));
#252488=CARTESIAN_POINT('Ctrl Pts',(-9.62764253104559,12.2,5.56622665049629));
#252489=CARTESIAN_POINT('Ctrl Pts',(-9.63196820497383,12.2,5.56686213045657));
#252490=CARTESIAN_POINT('Ctrl Pts',(-9.63630811047205,12.2,5.56749261024124));
#252491=CARTESIAN_POINT('Ctrl Pts',(-9.64064801656159,12.2,5.56812309011182));
#252492=CARTESIAN_POINT('Ctrl Pts',(-9.64500215466359,12.2,5.56874856910148));
#252493=CARTESIAN_POINT('Ctrl Pts',(-9.64937044468089,12.2,5.56936896413477));
#252494=CARTESIAN_POINT('Ctrl Pts',(-9.65373873410301,12.2,5.56998935908353));
#252495=CARTESIAN_POINT('Ctrl Pts',(-9.65812117615106,12.2,5.57060466800239));
#252496=CARTESIAN_POINT('Ctrl Pts',(-9.66251769112405,12.2,5.57121481100841));
#252497=CARTESIAN_POINT('Ctrl Pts',(-9.66581507750354,12.2,5.57167241828371));
#252498=CARTESIAN_POINT('Ctrl Pts',(-9.66912038139817,12.2,5.57212711747274));
#252499=CARTESIAN_POINT('Ctrl Pts',(-9.67243356790073,12.2,5.57257887589591));
#252500=CARTESIAN_POINT('Ctrl Pts',(-9.67574675440329,12.2,5.57303063431907));
#252501=CARTESIAN_POINT('Ctrl Pts',(-9.67906782442966,12.2,5.5734794528186));
#252502=CARTESIAN_POINT('Ctrl Pts',(-9.68239674476597,12.2,5.57392529467781));
#252503=CARTESIAN_POINT('Ctrl Pts',(-9.68572566570703,12.2,5.57437113661801));
#252504=CARTESIAN_POINT('Ctrl Pts',(-9.68906243780863,12.2,5.57481400246571));
#252505=CARTESIAN_POINT('Ctrl Pts',(-9.69240702671246,12.2,5.57525385936256));
#252506=CARTESIAN_POINT('Ctrl Pts',(-9.69575161500868,12.2,5.57569371617951));
#252507=CARTESIAN_POINT('Ctrl Pts',(-9.6991040210878,12.2,5.57613056321327));
#252508=CARTESIAN_POINT('Ctrl Pts',(-9.70246421142472,12.2,5.57656436657224));
#252509=CARTESIAN_POINT('Ctrl Pts',(-9.70582440176164,12.2,5.57699816993121));
#252510=CARTESIAN_POINT('Ctrl Pts',(-9.70919237709369,12.2,5.57742892938067));
#252511=CARTESIAN_POINT('Ctrl Pts',(-9.71256810444474,12.2,5.57785661224206));
#252512=CARTESIAN_POINT('Ctrl Pts',(-9.7181943169009,12.2,5.57856941703695));
#252513=CARTESIAN_POINT('Ctrl Pts',(-9.72384206380311,12.2,5.57927367373479));
#252514=CARTESIAN_POINT('Ctrl Pts',(-9.72951119359589,12.2,5.57996923026211));
#252515=CARTESIAN_POINT('Ctrl Pts',(-9.73404649705935,12.2,5.58052567543848));
#252516=CARTESIAN_POINT('Ctrl Pts',(-9.73859548588673,12.2,5.58107655219652));
#252517=CARTESIAN_POINT('Ctrl Pts',(-9.74315808334569,12.2,5.58162178265253));
#252518=CARTESIAN_POINT('Ctrl Pts',(-9.74658003221697,12.2,5.58203070558739));
#252519=CARTESIAN_POINT('Ctrl Pts',(-9.75000963559875,12.2,5.58243645244636));
#252520=CARTESIAN_POINT('Ctrl Pts',(-9.753446862016,12.2,5.58283899133776));
#252521=CARTESIAN_POINT('Ctrl Pts',(-9.75688408780881,12.2,5.58324153015603));
#252522=CARTESIAN_POINT('Ctrl Pts',(-9.7603289359368,12.2,5.58364086020492));
#252523=CARTESIAN_POINT('Ctrl Pts',(-9.76378137490137,12.2,5.58403694962661));
#252524=CARTESIAN_POINT('Ctrl Pts',(-9.76723381386595,12.2,5.5844330390483));
#252525=CARTESIAN_POINT('Ctrl Pts',(-9.7706938435701,12.2,5.58482588814019));
#252526=CARTESIAN_POINT('Ctrl Pts',(-9.7741614309031,12.2,5.58521546454242));
#252527=CARTESIAN_POINT('Ctrl Pts',(-9.77762901823611,12.2,5.58560504094464));
#252528=CARTESIAN_POINT('Ctrl Pts',(-9.78110416479321,12.2,5.58599134436393));
#252529=CARTESIAN_POINT('Ctrl Pts',(-9.78458683804167,12.2,5.58637434426668));
#252530=CARTESIAN_POINT('Ctrl Pts',(-9.78806951129012,12.2,5.58675734416943));
#252531=CARTESIAN_POINT('Ctrl Pts',(-9.79155971034661,12.2,5.58713703992232));
#252532=CARTESIAN_POINT('Ctrl Pts',(-9.79505740463555,12.2,5.58751339940893));
#252533=CARTESIAN_POINT('Ctrl Pts',(-9.79855509892447,12.2,5.58788975889555));
#252534=CARTESIAN_POINT('Ctrl Pts',(-9.80206028787347,12.2,5.5882627834897));
#252535=CARTESIAN_POINT('Ctrl Pts',(-9.80557294029547,12.2,5.58863244091179));
#252536=CARTESIAN_POINT('Ctrl Pts',(-9.80908559271745,12.2,5.58900209833388));
#252537=CARTESIAN_POINT('Ctrl Pts',(-9.81260570726018,12.2,5.58936838911695));
#252538=CARTESIAN_POINT('Ctrl Pts',(-9.81613325396433,12.2,5.58973128243756));
#252539=CARTESIAN_POINT('Ctrl Pts',(-9.81966080130931,12.2,5.5900941758241));
#252540=CARTESIAN_POINT('Ctrl Pts',(-9.82319577992308,12.2,5.59045366969301));
#252541=CARTESIAN_POINT('Ctrl Pts',(-9.82673815881393,12.2,5.59080973703596));
#252542=CARTESIAN_POINT('Ctrl Pts',(-9.83146132959582,12.2,5.59128449338542));
#252543=CARTESIAN_POINT('Ctrl Pts',(-9.8361976552621,12.2,5.591753153644));
#252544=CARTESIAN_POINT('Ctrl Pts',(-9.84094706209519,12.2,5.59221564749548));
#252545=CARTESIAN_POINT('Ctrl Pts',(-9.84450911738179,12.2,5.59256251789984));
#252546=CARTESIAN_POINT('Ctrl Pts',(-9.84807853118457,12.2,5.59290591850444));
#252547=CARTESIAN_POINT('Ctrl Pts',(-9.85165527101195,12.2,5.59324582090924));
#252548=CARTESIAN_POINT('Ctrl Pts',(-9.85523201148911,12.2,5.59358572337579));
#252549=CARTESIAN_POINT('Ctrl Pts',(-9.85881607917667,12.2,5.59392212679134));
#252550=CARTESIAN_POINT('Ctrl Pts',(-9.86240744253293,12.2,5.59425500083924));
#252551=CARTESIAN_POINT('Ctrl Pts',(-9.86599880523677,12.2,5.59458787482666));
#252552=CARTESIAN_POINT('Ctrl Pts',(-9.86959746236442,12.2,5.59491722109231));
#252553=CARTESIAN_POINT('Ctrl Pts',(-9.8732033847894,12.2,5.59524300759634));
#252554=CARTESIAN_POINT('Ctrl Pts',(-9.87801128113769,12.2,5.59567738958199));
#252555=CARTESIAN_POINT('Ctrl Pts',(-9.88283209181486,12.2,5.59610544514953));
#252556=CARTESIAN_POINT('Ctrl Pts',(-9.88766574336331,12.2,5.59652710444881));
#252557=CARTESIAN_POINT('Ctrl Pts',(-9.89129098218929,12.2,5.59684334893764));
#252558=CARTESIAN_POINT('Ctrl Pts',(-9.89492344463978,12.2,5.59715599571005));
#252559=CARTESIAN_POINT('Ctrl Pts',(-9.89856309850657,12.2,5.59746501565764));
#252560=CARTESIAN_POINT('Ctrl Pts',(-9.90220275303456,12.2,5.59777403566139));
#252561=CARTESIAN_POINT('Ctrl Pts',(-9.90584960003122,12.2,5.59807942857243));
#252562=CARTESIAN_POINT('Ctrl Pts',(-9.90950360852158,12.2,5.59838116603245));
#252563=CARTESIAN_POINT('Ctrl Pts',(-9.91315761634814,12.2,5.59868290343766));
#252564=CARTESIAN_POINT('Ctrl Pts',(-9.916818785809,12.2,5.59898098467001));
#252565=CARTESIAN_POINT('Ctrl Pts',(-9.92048708619313,12.2,5.5992753820486));
#252566=CARTESIAN_POINT('Ctrl Pts',(-9.92415538657726,12.2,5.59956977942718));
#252567=CARTESIAN_POINT('Ctrl Pts',(-9.92783081565137,12.2,5.59986049160864));
#252568=CARTESIAN_POINT('Ctrl Pts',(-9.93151334589319,12.2,5.60014749105623));
#252569=CARTESIAN_POINT('Ctrl Pts',(-9.93642338599263,12.2,5.60053015696896));
#252570=CARTESIAN_POINT('Ctrl Pts',(-9.94134604849508,12.2,5.60090622124413));
#252571=CARTESIAN_POINT('Ctrl Pts',(-9.94628126070143,12.2,5.60127561971461));
#252572=CARTESIAN_POINT('Ctrl Pts',(-9.94998267069671,12.2,5.60155266863039));
#252573=CARTESIAN_POINT('Ctrl Pts',(-9.95369114066905,12.2,5.60182596663677));
#252574=CARTESIAN_POINT('Ctrl Pts',(-9.95740664008499,12.2,5.6020954870921));
#252575=CARTESIAN_POINT('Ctrl Pts',(-9.96112213882595,12.2,5.60236500749846));
#252576=CARTESIAN_POINT('Ctrl Pts',(-9.96484466592003,12.2,5.60263074873086));
#252577=CARTESIAN_POINT('Ctrl Pts',(-9.96857418997165,12.2,5.60289268277565));
#252578=CARTESIAN_POINT('Ctrl Pts',(-9.97354688848131,12.2,5.60324192815285));
#252579=CARTESIAN_POINT('Ctrl Pts',(-9.97853202621204,12.2,5.6035844046495));
#252580=CARTESIAN_POINT('Ctrl Pts',(-9.98352953635825,12.2,5.60392005195584));
#252581=CARTESIAN_POINT('Ctrl Pts',(-9.98727766913814,12.2,5.60417178744703));
#252582=CARTESIAN_POINT('Ctrl Pts',(-9.99103276126752,12.2,5.60441968228848));
#252583=CARTESIAN_POINT('Ctrl Pts',(-9.99479478496322,12.2,5.60466370919681));
#252584=CARTESIAN_POINT('Ctrl Pts',(-9.99855680934236,12.2,5.60490773614947));
#252585=CARTESIAN_POINT('Ctrl Pts',(-10.0023257639401,12.2,5.60514789495104));
#252586=CARTESIAN_POINT('Ctrl Pts',(-10.0061016128231,12.2,5.60538415381818));
#252587=CARTESIAN_POINT('Ctrl Pts',(-10.0098774610202,12.2,5.6056204126424));
#252588=CARTESIAN_POINT('Ctrl Pts',(-10.0136602026308,12.2,5.60585276952485));
#252589=CARTESIAN_POINT('Ctrl Pts',(-10.0174498052666,12.2,5.60608119706917));
#252590=CARTESIAN_POINT('Ctrl Pts',(-10.0212394079023,12.2,5.60630962461349));
#252591=CARTESIAN_POINT('Ctrl Pts',(-10.0250358713842,12.2,5.60653412069107));
#252592=CARTESIAN_POINT('Ctrl Pts',(-10.028839180665,12.2,5.6067546754843));
#252593=CARTESIAN_POINT('Ctrl Pts',(-10.0326424899459,12.2,5.60697523027754));
#252594=CARTESIAN_POINT('Ctrl Pts',(-10.0364526481964,12.2,5.60719184195524));
#252595=CARTESIAN_POINT('Ctrl Pts',(-10.0402696490001,12.2,5.60740451199998));
#252596=CARTESIAN_POINT('Origin',(-5.66257110645729E-14,15.2,-1.77635683940025E-14));
#252597=CARTESIAN_POINT('',(-9.55499537100006,15.2,4.04260911599999));
#252598=CARTESIAN_POINT('',(-9.55499537100006,12.2,4.04260911599999));
#252599=CARTESIAN_POINT('',(-9.55499537100006,15.2,4.04260911599999));
#252600=CARTESIAN_POINT('Origin',(-5.66257110645729E-14,12.2,-1.77635683940025E-14));
#252601=CARTESIAN_POINT('Origin',(-5.66257110645729E-14,15.2,-1.77635683940025E-14));
#252602=CARTESIAN_POINT('Origin',(-5.66257110645729E-14,15.2,-1.77635683940025E-14));
#252603=CARTESIAN_POINT('',(-10.7360910480001,15.2,4.12144986899998));
#252604=CARTESIAN_POINT('',(-10.8675859440001,15.2,3.76106045599998));
#252605=CARTESIAN_POINT('Origin',(-5.66257110645729E-14,15.2,-1.77635683940025E-14));
#252606=CARTESIAN_POINT('',(-10.8675859440001,12.2,3.76106045599998));
#252607=CARTESIAN_POINT('',(-10.8675859440001,15.2,3.76106045599998));
#252608=CARTESIAN_POINT('',(-10.7360910480001,12.2,4.12144986899998));
#252609=CARTESIAN_POINT('Origin',(-5.66257110645729E-14,12.2,-1.77635683940025E-14));
#252610=CARTESIAN_POINT('',(-10.7360910480001,15.2,4.12144986899998));
#252611=CARTESIAN_POINT('Ctrl Pts',(-9.55499537100006,15.2,4.04260911699998));
#252612=CARTESIAN_POINT('Ctrl Pts',(-9.55499537100006,11.6,4.04260911699998));
#252613=CARTESIAN_POINT('Ctrl Pts',(-9.55516119300006,15.2,4.04266300499999));
#252614=CARTESIAN_POINT('Ctrl Pts',(-9.55516119300006,11.6,4.04266300499999));
#252615=CARTESIAN_POINT('Ctrl Pts',(-9.55549865500006,15.2,4.04277257899999));
#252616=CARTESIAN_POINT('Ctrl Pts',(-9.55549865500006,11.6,4.04277257899999));
#252617=CARTESIAN_POINT('Ctrl Pts',(-9.55601007100006,15.2,4.04293835899999));
#252618=CARTESIAN_POINT('Ctrl Pts',(-9.55601007100006,11.6,4.04293835899998));
#252619=CARTESIAN_POINT('Ctrl Pts',(-9.55669916300005,15.2,4.04316116599999));
#252620=CARTESIAN_POINT('Ctrl Pts',(-9.55669916300005,11.6,4.04316116599999));
#252621=CARTESIAN_POINT('Ctrl Pts',(-9.55757104200006,15.2,4.04344211399999));
#252622=CARTESIAN_POINT('Ctrl Pts',(-9.55757104200006,11.6,4.04344211399999));
#252623=CARTESIAN_POINT('Ctrl Pts',(-9.55845733900006,15.2,4.04372672599998));
#252624=CARTESIAN_POINT('Ctrl Pts',(-9.55845733900006,11.6,4.04372672599998));
#252625=CARTESIAN_POINT('Ctrl Pts',(-9.55935298100006,15.2,4.04401334799999));
#252626=CARTESIAN_POINT('Ctrl Pts',(-9.55935298100006,11.6,4.04401334799999));
#252627=CARTESIAN_POINT('Ctrl Pts',(-9.56025795200006,15.2,4.04430195599998));
#252628=CARTESIAN_POINT('Ctrl Pts',(-9.56025795200006,11.6,4.04430195599998));
#252629=CARTESIAN_POINT('Ctrl Pts',(-9.56117222800006,15.2,4.04459252399998));
#252630=CARTESIAN_POINT('Ctrl Pts',(-9.56117222800006,11.6,4.04459252399998));
#252631=CARTESIAN_POINT('Ctrl Pts',(-9.56209579100006,15.2,4.04488502599998));
#252632=CARTESIAN_POINT('Ctrl Pts',(-9.56209579100006,11.6,4.04488502599998));
#252633=CARTESIAN_POINT('Ctrl Pts',(-9.56302862000006,15.2,4.04517943699998));
#252634=CARTESIAN_POINT('Ctrl Pts',(-9.56302862000006,11.6,4.04517943699998));
#252635=CARTESIAN_POINT('Ctrl Pts',(-9.56397069600006,15.2,4.04547573399999));
#252636=CARTESIAN_POINT('Ctrl Pts',(-9.56397069600006,11.6,4.04547573399998));
#252637=CARTESIAN_POINT('Ctrl Pts',(-9.56492199900006,15.2,4.04577388999999));
#252638=CARTESIAN_POINT('Ctrl Pts',(-9.56492199900006,11.6,4.04577388999999));
#252639=CARTESIAN_POINT('Ctrl Pts',(-9.56588251000005,15.2,4.04607387999998));
#252640=CARTESIAN_POINT('Ctrl Pts',(-9.56588251000005,11.6,4.04607387999998));
#252641=CARTESIAN_POINT('Ctrl Pts',(-9.56685220800006,15.2,4.04637568199998));
#252642=CARTESIAN_POINT('Ctrl Pts',(-9.56685220800006,11.6,4.04637568199998));
#252643=CARTESIAN_POINT('Ctrl Pts',(-9.56783107300006,15.2,4.04667926899998));
#252644=CARTESIAN_POINT('Ctrl Pts',(-9.56783107300006,11.6,4.04667926899998));
#252645=CARTESIAN_POINT('Ctrl Pts',(-9.56881908800005,15.2,4.04698461699999));
#252646=CARTESIAN_POINT('Ctrl Pts',(-9.56881908800005,11.6,4.04698461699999));
#252647=CARTESIAN_POINT('Ctrl Pts',(-9.56981623300006,15.2,4.04729170299999));
#252648=CARTESIAN_POINT('Ctrl Pts',(-9.56981623300006,11.6,4.04729170299999));
#252649=CARTESIAN_POINT('Ctrl Pts',(-9.57082248800005,15.2,4.04760050199998));
#252650=CARTESIAN_POINT('Ctrl Pts',(-9.57082248800005,11.6,4.04760050199998));
#252651=CARTESIAN_POINT('Ctrl Pts',(-9.57183783400006,15.2,4.04791098999999));
#252652=CARTESIAN_POINT('Ctrl Pts',(-9.57183783400006,11.6,4.04791098999999));
#252653=CARTESIAN_POINT('Ctrl Pts',(-9.57286225200006,15.2,4.04822314299999));
#252654=CARTESIAN_POINT('Ctrl Pts',(-9.57286225200006,11.6,4.04822314299999));
#252655=CARTESIAN_POINT('Ctrl Pts',(-9.57389572300006,15.2,4.04853693899998));
#252656=CARTESIAN_POINT('Ctrl Pts',(-9.57389572300006,11.6,4.04853693899998));
#252657=CARTESIAN_POINT('Ctrl Pts',(-9.57493822900006,15.2,4.04885235199998));
#252658=CARTESIAN_POINT('Ctrl Pts',(-9.57493822900006,11.6,4.04885235199998));
#252659=CARTESIAN_POINT('Ctrl Pts',(-9.57598974800005,15.2,4.04916935999999));
#252660=CARTESIAN_POINT('Ctrl Pts',(-9.57598974800005,11.6,4.04916935999999));
#252661=CARTESIAN_POINT('Ctrl Pts',(-9.57705026600006,15.2,4.04948793999999));
#252662=CARTESIAN_POINT('Ctrl Pts',(-9.57705026600006,11.6,4.04948793999999));
#252663=CARTESIAN_POINT('Ctrl Pts',(-9.57811976000006,15.2,4.04980806699999));
#252664=CARTESIAN_POINT('Ctrl Pts',(-9.57811976000006,11.6,4.04980806699999));
#252665=CARTESIAN_POINT('Ctrl Pts',(-9.57919821400005,15.2,4.05012971899998));
#252666=CARTESIAN_POINT('Ctrl Pts',(-9.57919821400005,11.6,4.05012971899998));
#252667=CARTESIAN_POINT('Ctrl Pts',(-9.58028560900006,15.2,4.05045287299998));
#252668=CARTESIAN_POINT('Ctrl Pts',(-9.58028560900006,11.6,4.05045287299998));
#252669=CARTESIAN_POINT('Ctrl Pts',(-9.58138192600006,15.2,4.05077750599999));
#252670=CARTESIAN_POINT('Ctrl Pts',(-9.58138192600006,11.6,4.05077750599998));
#252671=CARTESIAN_POINT('Ctrl Pts',(-9.58248714800006,15.2,4.05110359599998));
#252672=CARTESIAN_POINT('Ctrl Pts',(-9.58248714800006,11.6,4.05110359599998));
#252673=CARTESIAN_POINT('Ctrl Pts',(-9.58360125400005,15.2,4.05143111799998));
#252674=CARTESIAN_POINT('Ctrl Pts',(-9.58360125400005,11.6,4.05143111799998));
#252675=CARTESIAN_POINT('Ctrl Pts',(-9.58472422800006,15.2,4.05176005199999));
#252676=CARTESIAN_POINT('Ctrl Pts',(-9.58472422800006,11.6,4.05176005199999));
#252677=CARTESIAN_POINT('Ctrl Pts',(-9.58585605100006,15.2,4.05209037499999));
#252678=CARTESIAN_POINT('Ctrl Pts',(-9.58585605100006,11.6,4.05209037499999));
#252679=CARTESIAN_POINT('Ctrl Pts',(-9.58699670500006,15.2,4.05242206399999));
#252680=CARTESIAN_POINT('Ctrl Pts',(-9.58699670500006,11.6,4.05242206399999));
#252681=CARTESIAN_POINT('Ctrl Pts',(-9.58814617200006,15.2,4.05275509699998));
#252682=CARTESIAN_POINT('Ctrl Pts',(-9.58814617200006,11.6,4.05275509699998));
#252683=CARTESIAN_POINT('Ctrl Pts',(-9.58930443500006,15.2,4.05308945199998));
#252684=CARTESIAN_POINT('Ctrl Pts',(-9.58930443500006,11.6,4.05308945199998));
#252685=CARTESIAN_POINT('Ctrl Pts',(-9.59047147500005,15.2,4.05342510699998));
#252686=CARTESIAN_POINT('Ctrl Pts',(-9.59047147500005,11.6,4.05342510699998));
#252687=CARTESIAN_POINT('Ctrl Pts',(-9.59164727400006,15.2,4.05376203999998));
#252688=CARTESIAN_POINT('Ctrl Pts',(-9.59164727400006,11.6,4.05376203999998));
#252689=CARTESIAN_POINT('Ctrl Pts',(-9.59283181500006,15.2,4.05410022899999));
#252690=CARTESIAN_POINT('Ctrl Pts',(-9.59283181500006,11.6,4.05410022899999));
#252691=CARTESIAN_POINT('Ctrl Pts',(-9.59402508100006,15.2,4.05443965299998));
#252692=CARTESIAN_POINT('Ctrl Pts',(-9.59402508100006,11.6,4.05443965299998));
#252693=CARTESIAN_POINT('Ctrl Pts',(-9.59522705300006,15.2,4.05478028999998));
#252694=CARTESIAN_POINT('Ctrl Pts',(-9.59522705300006,11.6,4.05478028999998));
#252695=CARTESIAN_POINT('Ctrl Pts',(-9.59643771400006,15.2,4.05512211999999));
#252696=CARTESIAN_POINT('Ctrl Pts',(-9.59643771400006,11.6,4.05512211999999));
#252697=CARTESIAN_POINT('Ctrl Pts',(-9.59765704500006,15.2,4.05546511899999));
#252698=CARTESIAN_POINT('Ctrl Pts',(-9.59765704500006,11.6,4.05546511899998));
#252699=CARTESIAN_POINT('Ctrl Pts',(-9.59888503300006,15.2,4.05580926699999));
#252700=CARTESIAN_POINT('Ctrl Pts',(-9.59888503300006,11.6,4.05580926699999));
#252701=CARTESIAN_POINT('Ctrl Pts',(-9.60012165600006,15.2,4.05615454399998));
#252702=CARTESIAN_POINT('Ctrl Pts',(-9.60012165600006,11.6,4.05615454399998));
#252703=CARTESIAN_POINT('Ctrl Pts',(-9.60136689800006,15.2,4.05650092799998));
#252704=CARTESIAN_POINT('Ctrl Pts',(-9.60136689800006,11.6,4.05650092799998));
#252705=CARTESIAN_POINT('Ctrl Pts',(-9.60262074400006,15.2,4.05684839599999));
#252706=CARTESIAN_POINT('Ctrl Pts',(-9.60262074400006,11.6,4.05684839599999));
#252707=CARTESIAN_POINT('Ctrl Pts',(-9.60388317400006,15.2,4.05719693099999));
#252708=CARTESIAN_POINT('Ctrl Pts',(-9.60388317400006,11.6,4.05719693099999));
#252709=CARTESIAN_POINT('Ctrl Pts',(-9.60515417300006,15.2,4.05754650999998));
#252710=CARTESIAN_POINT('Ctrl Pts',(-9.60515417300006,11.6,4.05754650999998));
#252711=CARTESIAN_POINT('Ctrl Pts',(-9.60643372200006,15.2,4.05789711199999));
#252712=CARTESIAN_POINT('Ctrl Pts',(-9.60643372200006,11.6,4.05789711199999));
#252713=CARTESIAN_POINT('Ctrl Pts',(-9.60772180600006,15.2,4.05824871799998));
#252714=CARTESIAN_POINT('Ctrl Pts',(-9.60772180600006,11.6,4.05824871799998));
#252715=CARTESIAN_POINT('Ctrl Pts',(-9.60901840800006,15.2,4.05860130499998));
#252716=CARTESIAN_POINT('Ctrl Pts',(-9.60901840800006,11.6,4.05860130499998));
#252717=CARTESIAN_POINT('Ctrl Pts',(-9.61032351000006,15.2,4.05895485699999));
#252718=CARTESIAN_POINT('Ctrl Pts',(-9.61032351000006,11.6,4.05895485699998));
#252719=CARTESIAN_POINT('Ctrl Pts',(-9.61163709700006,15.2,4.05930934899998));
#252720=CARTESIAN_POINT('Ctrl Pts',(-9.61163709700006,11.6,4.05930934899998));
#252721=CARTESIAN_POINT('Ctrl Pts',(-9.61295914900005,15.2,4.05966476399998));
#252722=CARTESIAN_POINT('Ctrl Pts',(-9.61295914900005,11.6,4.05966476399998));
#252723=CARTESIAN_POINT('Ctrl Pts',(-9.61428965300006,15.2,4.06002107999999));
#252724=CARTESIAN_POINT('Ctrl Pts',(-9.61428965300006,11.6,4.06002107999999));
#252725=CARTESIAN_POINT('Ctrl Pts',(-9.61562859000006,15.2,4.06037827999998));
#252726=CARTESIAN_POINT('Ctrl Pts',(-9.61562859000006,11.6,4.06037827999998));
#252727=CARTESIAN_POINT('Ctrl Pts',(-9.61697594500006,15.2,4.06073633999998));
#252728=CARTESIAN_POINT('Ctrl Pts',(-9.61697594500006,11.6,4.06073633999998));
#252729=CARTESIAN_POINT('Ctrl Pts',(-9.61833170200006,15.2,4.06109524299998));
#252730=CARTESIAN_POINT('Ctrl Pts',(-9.61833170200006,11.6,4.06109524299998));
#252731=CARTESIAN_POINT('Ctrl Pts',(-9.61969584100006,15.2,4.06145496799999));
#252732=CARTESIAN_POINT('Ctrl Pts',(-9.61969584100006,11.6,4.06145496799999));
#252733=CARTESIAN_POINT('Ctrl Pts',(-9.62106835000006,15.2,4.06181549699999));
#252734=CARTESIAN_POINT('Ctrl Pts',(-9.62106835000006,11.6,4.06181549699998));
#252735=CARTESIAN_POINT('Ctrl Pts',(-9.62244921100006,15.2,4.06217680799998));
#252736=CARTESIAN_POINT('Ctrl Pts',(-9.62244921100006,11.6,4.06217680799998));
#252737=CARTESIAN_POINT('Ctrl Pts',(-9.62383840700006,15.2,4.06253888499998));
#252738=CARTESIAN_POINT('Ctrl Pts',(-9.62383840700006,11.6,4.06253888499998));
#252739=CARTESIAN_POINT('Ctrl Pts',(-9.62523592300006,15.2,4.06290170499998));
#252740=CARTESIAN_POINT('Ctrl Pts',(-9.62523592300006,11.6,4.06290170499998));
#252741=CARTESIAN_POINT('Ctrl Pts',(-9.62664174300006,15.2,4.06326525199999));
#252742=CARTESIAN_POINT('Ctrl Pts',(-9.62664174300006,11.6,4.06326525199999));
#252743=CARTESIAN_POINT('Ctrl Pts',(-9.62805585000006,15.2,4.06362950399998));
#252744=CARTESIAN_POINT('Ctrl Pts',(-9.62805585000006,11.6,4.06362950399998));
#252745=CARTESIAN_POINT('Ctrl Pts',(-9.62947822800006,15.2,4.06399444399998));
#252746=CARTESIAN_POINT('Ctrl Pts',(-9.62947822800006,11.6,4.06399444399998));
#252747=CARTESIAN_POINT('Ctrl Pts',(-9.63090886200006,15.2,4.06436005199998));
#252748=CARTESIAN_POINT('Ctrl Pts',(-9.63090886200006,11.6,4.06436005199998));
#252749=CARTESIAN_POINT('Ctrl Pts',(-9.63234773700006,15.2,4.06472630899999));
#252750=CARTESIAN_POINT('Ctrl Pts',(-9.63234773700006,11.6,4.06472630899999));
#252751=CARTESIAN_POINT('Ctrl Pts',(-9.63379483400006,15.2,4.06509319699998));
#252752=CARTESIAN_POINT('Ctrl Pts',(-9.63379483400006,11.6,4.06509319699998));
#252753=CARTESIAN_POINT('Ctrl Pts',(-9.63525014000006,15.2,4.06546069799998));
#252754=CARTESIAN_POINT('Ctrl Pts',(-9.63525014000006,11.6,4.06546069799998));
#252755=CARTESIAN_POINT('Ctrl Pts',(-9.63671363700006,15.2,4.06582879099999));
#252756=CARTESIAN_POINT('Ctrl Pts',(-9.63671363700006,11.6,4.06582879099999));
#252757=CARTESIAN_POINT('Ctrl Pts',(-9.63818531300005,15.2,4.06619745799999));
#252758=CARTESIAN_POINT('Ctrl Pts',(-9.63818531300005,11.6,4.06619745799999));
#252759=CARTESIAN_POINT('Ctrl Pts',(-9.63966514800006,15.2,4.06656668199999));
#252760=CARTESIAN_POINT('Ctrl Pts',(-9.63966514800006,11.6,4.06656668199999));
#252761=CARTESIAN_POINT('Ctrl Pts',(-9.64115313000006,15.2,4.06693644299998));
#252762=CARTESIAN_POINT('Ctrl Pts',(-9.64115313000006,11.6,4.06693644299998));
#252763=CARTESIAN_POINT('Ctrl Pts',(-9.64264924100006,15.2,4.06730672499998));
#252764=CARTESIAN_POINT('Ctrl Pts',(-9.64264924100006,11.6,4.06730672499998));
#252765=CARTESIAN_POINT('Ctrl Pts',(-9.64415346700006,15.2,4.06767750699998));
#252766=CARTESIAN_POINT('Ctrl Pts',(-9.64415346700006,11.6,4.06767750699998));
#252767=CARTESIAN_POINT('Ctrl Pts',(-9.64566579300006,15.2,4.06804877199999));
#252768=CARTESIAN_POINT('Ctrl Pts',(-9.64566579300006,11.6,4.06804877199998));
#252769=CARTESIAN_POINT('Ctrl Pts',(-9.64718620100006,15.2,4.06842050299999));
#252770=CARTESIAN_POINT('Ctrl Pts',(-9.64718620100006,11.6,4.06842050299998));
#252771=CARTESIAN_POINT('Ctrl Pts',(-9.64871467900006,15.2,4.06879268099999));
#252772=CARTESIAN_POINT('Ctrl Pts',(-9.64871467900006,11.6,4.06879268099999));
#252773=CARTESIAN_POINT('Ctrl Pts',(-9.65025121000006,15.2,4.06916528799999));
#252774=CARTESIAN_POINT('Ctrl Pts',(-9.65025121000006,11.6,4.06916528799999));
#252775=CARTESIAN_POINT('Ctrl Pts',(-9.65179577900006,15.2,4.06953830699998));
#252776=CARTESIAN_POINT('Ctrl Pts',(-9.65179577900006,11.6,4.06953830699998));
#252777=CARTESIAN_POINT('Ctrl Pts',(-9.65334837100006,15.2,4.06991171799999));
#252778=CARTESIAN_POINT('Ctrl Pts',(-9.65334837100006,11.6,4.06991171799999));
#252779=CARTESIAN_POINT('Ctrl Pts',(-9.65490897100005,15.2,4.07028550599998));
#252780=CARTESIAN_POINT('Ctrl Pts',(-9.65490897100005,11.6,4.07028550599998));
#252781=CARTESIAN_POINT('Ctrl Pts',(-9.65647756400006,15.2,4.07065965099999));
#252782=CARTESIAN_POINT('Ctrl Pts',(-9.65647756400006,11.6,4.07065965099999));
#252783=CARTESIAN_POINT('Ctrl Pts',(-9.65805413400006,15.2,4.07103413899998));
#252784=CARTESIAN_POINT('Ctrl Pts',(-9.65805413400006,11.6,4.07103413899998));
#252785=CARTESIAN_POINT('Ctrl Pts',(-9.65963866800006,15.2,4.07140894899998));
#252786=CARTESIAN_POINT('Ctrl Pts',(-9.65963866800006,11.6,4.07140894899998));
#252787=CARTESIAN_POINT('Ctrl Pts',(-9.66123114800006,15.2,4.07178406499998));
#252788=CARTESIAN_POINT('Ctrl Pts',(-9.66123114800006,11.6,4.07178406499998));
#252789=CARTESIAN_POINT('Ctrl Pts',(-9.66283156300005,15.2,4.07215947099999));
#252790=CARTESIAN_POINT('Ctrl Pts',(-9.66283156300005,11.6,4.07215947099999));
#252791=CARTESIAN_POINT('Ctrl Pts',(-9.66443989600006,15.2,4.07253514799999));
#252792=CARTESIAN_POINT('Ctrl Pts',(-9.66443989600006,11.6,4.07253514799999));
#252793=CARTESIAN_POINT('Ctrl Pts',(-9.66605613200005,15.2,4.07291107899999));
#252794=CARTESIAN_POINT('Ctrl Pts',(-9.66605613200005,11.6,4.07291107899999));
#252795=CARTESIAN_POINT('Ctrl Pts',(-9.66768025600006,15.2,4.07328724699998));
#252796=CARTESIAN_POINT('Ctrl Pts',(-9.66768025600006,11.6,4.07328724699998));
#252797=CARTESIAN_POINT('Ctrl Pts',(-9.66931225600005,15.2,4.07366363599999));
#252798=CARTESIAN_POINT('Ctrl Pts',(-9.66931225600005,11.6,4.07366363599999));
#252799=CARTESIAN_POINT('Ctrl Pts',(-9.67095211400006,15.2,4.07404022799999));
#252800=CARTESIAN_POINT('Ctrl Pts',(-9.67095211400006,11.6,4.07404022799999));
#252801=CARTESIAN_POINT('Ctrl Pts',(-9.67259981800006,15.2,4.07441700699999));
#252802=CARTESIAN_POINT('Ctrl Pts',(-9.67259981800006,11.6,4.07441700699999));
#252803=CARTESIAN_POINT('Ctrl Pts',(-9.67425535200006,15.2,4.07479395599999));
#252804=CARTESIAN_POINT('Ctrl Pts',(-9.67425535200006,11.6,4.07479395599999));
#252805=CARTESIAN_POINT('Ctrl Pts',(-9.67591870200006,15.2,4.07517105799998));
#252806=CARTESIAN_POINT('Ctrl Pts',(-9.67591870200006,11.6,4.07517105799998));
#252807=CARTESIAN_POINT('Ctrl Pts',(-9.67758985300006,15.2,4.07554829499999));
#252808=CARTESIAN_POINT('Ctrl Pts',(-9.67758985300006,11.6,4.07554829499999));
#252809=CARTESIAN_POINT('Ctrl Pts',(-9.67926879200006,15.2,4.07592565399998));
#252810=CARTESIAN_POINT('Ctrl Pts',(-9.67926879200006,11.6,4.07592565399998));
#252811=CARTESIAN_POINT('Ctrl Pts',(-9.68095550300006,15.2,4.07630311599998));
#252812=CARTESIAN_POINT('Ctrl Pts',(-9.68095550300006,11.6,4.07630311599998));
#252813=CARTESIAN_POINT('Ctrl Pts',(-9.68264997200006,15.2,4.07668066399999));
#252814=CARTESIAN_POINT('Ctrl Pts',(-9.68264997200006,11.6,4.07668066399999));
#252815=CARTESIAN_POINT('Ctrl Pts',(-9.68435218600005,15.2,4.07705828399998));
#252816=CARTESIAN_POINT('Ctrl Pts',(-9.68435218600005,11.6,4.07705828399998));
#252817=CARTESIAN_POINT('Ctrl Pts',(-9.68606212900006,15.2,4.07743595699999));
#252818=CARTESIAN_POINT('Ctrl Pts',(-9.68606212900006,11.6,4.07743595699999));
#252819=CARTESIAN_POINT('Ctrl Pts',(-9.68777978900006,15.2,4.07781366999998));
#252820=CARTESIAN_POINT('Ctrl Pts',(-9.68777978900006,11.6,4.07781366999998));
#252821=CARTESIAN_POINT('Ctrl Pts',(-9.68950515000006,15.2,4.07819140399998));
#252822=CARTESIAN_POINT('Ctrl Pts',(-9.68950515000006,11.6,4.07819140399998));
#252823=CARTESIAN_POINT('Ctrl Pts',(-9.69123819800006,15.2,4.07856914399999));
#252824=CARTESIAN_POINT('Ctrl Pts',(-9.69123819800006,11.6,4.07856914399999));
#252825=CARTESIAN_POINT('Ctrl Pts',(-9.69297892100006,15.2,4.07894687399998));
#252826=CARTESIAN_POINT('Ctrl Pts',(-9.69297892100006,11.6,4.07894687399998));
#252827=CARTESIAN_POINT('Ctrl Pts',(-9.69472730100006,15.2,4.07932457799999));
#252828=CARTESIAN_POINT('Ctrl Pts',(-9.69472730100006,11.6,4.07932457799998));
#252829=CARTESIAN_POINT('Ctrl Pts',(-9.69648332900006,15.2,4.07970223999998));
#252830=CARTESIAN_POINT('Ctrl Pts',(-9.69648332900006,11.6,4.07970223999998));
#252831=CARTESIAN_POINT('Ctrl Pts',(-9.69824698700006,15.2,4.08007984399998));
#252832=CARTESIAN_POINT('Ctrl Pts',(-9.69824698700006,11.6,4.08007984399998));
#252833=CARTESIAN_POINT('Ctrl Pts',(-9.70001826300006,15.2,4.08045737499998));
#252834=CARTESIAN_POINT('Ctrl Pts',(-9.70001826300006,11.6,4.08045737499998));
#252835=CARTESIAN_POINT('Ctrl Pts',(-9.70179714400006,15.2,4.08083481799999));
#252836=CARTESIAN_POINT('Ctrl Pts',(-9.70179714400006,11.6,4.08083481799998));
#252837=CARTESIAN_POINT('Ctrl Pts',(-9.70358361300006,15.2,4.08121215499998));
#252838=CARTESIAN_POINT('Ctrl Pts',(-9.70358361300006,11.6,4.08121215499998));
#252839=CARTESIAN_POINT('Ctrl Pts',(-9.70537765900006,15.2,4.08158937199998));
#252840=CARTESIAN_POINT('Ctrl Pts',(-9.70537765900006,11.6,4.08158937199998));
#252841=CARTESIAN_POINT('Ctrl Pts',(-9.70717926800006,15.2,4.08196645299999));
#252842=CARTESIAN_POINT('Ctrl Pts',(-9.70717926800006,11.6,4.08196645299998));
#252843=CARTESIAN_POINT('Ctrl Pts',(-9.70898842600005,15.2,4.08234338299999));
#252844=CARTESIAN_POINT('Ctrl Pts',(-9.70898842600005,11.6,4.08234338299999));
#252845=CARTESIAN_POINT('Ctrl Pts',(-9.71080511900006,15.2,4.08272014699998));
#252846=CARTESIAN_POINT('Ctrl Pts',(-9.71080511900006,11.6,4.08272014699998));
#252847=CARTESIAN_POINT('Ctrl Pts',(-9.71262933300006,15.2,4.08309672899998));
#252848=CARTESIAN_POINT('Ctrl Pts',(-9.71262933300006,11.6,4.08309672899998));
#252849=CARTESIAN_POINT('Ctrl Pts',(-9.71446105500006,15.2,4.08347311399999));
#252850=CARTESIAN_POINT('Ctrl Pts',(-9.71446105500006,11.6,4.08347311399999));
#252851=CARTESIAN_POINT('Ctrl Pts',(-9.71630027200005,15.2,4.08384928499999));
#252852=CARTESIAN_POINT('Ctrl Pts',(-9.71630027200005,11.6,4.08384928499998));
#252853=CARTESIAN_POINT('Ctrl Pts',(-9.71814696900006,15.2,4.08422523099999));
#252854=CARTESIAN_POINT('Ctrl Pts',(-9.71814696900006,11.6,4.08422523099999));
#252855=CARTESIAN_POINT('Ctrl Pts',(-9.72000113500006,15.2,4.08460093399999));
#252856=CARTESIAN_POINT('Ctrl Pts',(-9.72000113500006,11.6,4.08460093399999));
#252857=CARTESIAN_POINT('Ctrl Pts',(-9.72186275500006,15.2,4.08497637899998));
#252858=CARTESIAN_POINT('Ctrl Pts',(-9.72186275500006,11.6,4.08497637899998));
#252859=CARTESIAN_POINT('Ctrl Pts',(-9.72373181400006,15.2,4.08535155199999));
#252860=CARTESIAN_POINT('Ctrl Pts',(-9.72373181400006,11.6,4.08535155199999));
#252861=CARTESIAN_POINT('Ctrl Pts',(-9.72560830200005,15.2,4.08572643799998));
#252862=CARTESIAN_POINT('Ctrl Pts',(-9.72560830200005,11.6,4.08572643799998));
#252863=CARTESIAN_POINT('Ctrl Pts',(-9.72749220300006,15.2,4.08610102199999));
#252864=CARTESIAN_POINT('Ctrl Pts',(-9.72749220300006,11.6,4.08610102199999));
#252865=CARTESIAN_POINT('Ctrl Pts',(-9.72938350600005,15.2,4.08647528899999));
#252866=CARTESIAN_POINT('Ctrl Pts',(-9.72938350600005,11.6,4.08647528899999));
#252867=CARTESIAN_POINT('Ctrl Pts',(-9.73128219600006,15.2,4.08684922499998));
#252868=CARTESIAN_POINT('Ctrl Pts',(-9.73128219600006,11.6,4.08684922499998));
#252869=CARTESIAN_POINT('Ctrl Pts',(-9.73318826000006,15.2,4.08722281399999));
#252870=CARTESIAN_POINT('Ctrl Pts',(-9.73318826000006,11.6,4.08722281399999));
#252871=CARTESIAN_POINT('Ctrl Pts',(-9.73510168600006,15.2,4.08759604299998));
#252872=CARTESIAN_POINT('Ctrl Pts',(-9.73510168600006,11.6,4.08759604299998));
#252873=CARTESIAN_POINT('Ctrl Pts',(-9.73702246000006,15.2,4.08796889699998));
#252874=CARTESIAN_POINT('Ctrl Pts',(-9.73702246000006,11.6,4.08796889699998));
#252875=CARTESIAN_POINT('Ctrl Pts',(-9.73895056800006,15.2,4.08834136099999));
#252876=CARTESIAN_POINT('Ctrl Pts',(-9.73895056800006,11.6,4.08834136099998));
#252877=CARTESIAN_POINT('Ctrl Pts',(-9.74088599900006,15.2,4.08871342199999));
#252878=CARTESIAN_POINT('Ctrl Pts',(-9.74088599900006,11.6,4.08871342199998));
#252879=CARTESIAN_POINT('Ctrl Pts',(-9.74282873900006,15.2,4.08908506299999));
#252880=CARTESIAN_POINT('Ctrl Pts',(-9.74282873900006,11.6,4.08908506299999));
#252881=CARTESIAN_POINT('Ctrl Pts',(-9.74477877400006,15.2,4.08945627299998));
#252882=CARTESIAN_POINT('Ctrl Pts',(-9.74477877400006,11.6,4.08945627299998));
#252883=CARTESIAN_POINT('Ctrl Pts',(-9.74673609300006,15.2,4.08982703499999));
#252884=CARTESIAN_POINT('Ctrl Pts',(-9.74673609300006,11.6,4.08982703499999));
#252885=CARTESIAN_POINT('Ctrl Pts',(-9.74870068200006,15.2,4.09019733599998));
#252886=CARTESIAN_POINT('Ctrl Pts',(-9.74870068200006,11.6,4.09019733599998));
#252887=CARTESIAN_POINT('Ctrl Pts',(-9.75067252800006,15.2,4.09056716199999));
#252888=CARTESIAN_POINT('Ctrl Pts',(-9.75067252800006,11.6,4.09056716199998));
#252889=CARTESIAN_POINT('Ctrl Pts',(-9.75265161800005,15.2,4.09093649899999));
#252890=CARTESIAN_POINT('Ctrl Pts',(-9.75265161800005,11.6,4.09093649899999));
#252891=CARTESIAN_POINT('Ctrl Pts',(-9.75463794100006,15.2,4.09130533199999));
#252892=CARTESIAN_POINT('Ctrl Pts',(-9.75463794100006,11.6,4.09130533199999));
#252893=CARTESIAN_POINT('Ctrl Pts',(-9.75663148100006,15.2,4.09167364799998));
#252894=CARTESIAN_POINT('Ctrl Pts',(-9.75663148100006,11.6,4.09167364799998));
#252895=CARTESIAN_POINT('Ctrl Pts',(-9.75863222800006,15.2,4.09204143399998));
#252896=CARTESIAN_POINT('Ctrl Pts',(-9.75863222800006,11.6,4.09204143399998));
#252897=CARTESIAN_POINT('Ctrl Pts',(-9.76064016800006,15.2,4.09240867399999));
#252898=CARTESIAN_POINT('Ctrl Pts',(-9.76064016800006,11.6,4.09240867399998));
#252899=CARTESIAN_POINT('Ctrl Pts',(-9.76265528900005,15.2,4.09277535599998));
#252900=CARTESIAN_POINT('Ctrl Pts',(-9.76265528900005,11.6,4.09277535599998));
#252901=CARTESIAN_POINT('Ctrl Pts',(-9.76467757800006,15.2,4.09314146399999));
#252902=CARTESIAN_POINT('Ctrl Pts',(-9.76467757800006,11.6,4.09314146399998));
#252903=CARTESIAN_POINT('Ctrl Pts',(-9.76670702300006,15.2,4.09350698699999));
#252904=CARTESIAN_POINT('Ctrl Pts',(-9.76670702300006,11.6,4.09350698699999));
#252905=CARTESIAN_POINT('Ctrl Pts',(-9.76874361000006,15.2,4.09387190999999));
#252906=CARTESIAN_POINT('Ctrl Pts',(-9.76874361000006,11.6,4.09387190999999));
#252907=CARTESIAN_POINT('Ctrl Pts',(-9.77078732700006,15.2,4.09423621999998));
#252908=CARTESIAN_POINT('Ctrl Pts',(-9.77078732700006,11.6,4.09423621999998));
#252909=CARTESIAN_POINT('Ctrl Pts',(-9.77283816300006,15.2,4.09459990199998));
#252910=CARTESIAN_POINT('Ctrl Pts',(-9.77283816300006,11.6,4.09459990199998));
#252911=CARTESIAN_POINT('Ctrl Pts',(-9.77489610300006,15.2,4.09496294399998));
#252912=CARTESIAN_POINT('Ctrl Pts',(-9.77489610300006,11.6,4.09496294399998));
#252913=CARTESIAN_POINT('Ctrl Pts',(-9.77696113600006,15.2,4.09532533299998));
#252914=CARTESIAN_POINT('Ctrl Pts',(-9.77696113600006,11.6,4.09532533299998));
#252915=CARTESIAN_POINT('Ctrl Pts',(-9.77903325100005,15.2,4.09568705499999));
#252916=CARTESIAN_POINT('Ctrl Pts',(-9.77903325100005,11.6,4.09568705499998));
#252917=CARTESIAN_POINT('Ctrl Pts',(-9.78111243200006,15.2,4.09604809499999));
#252918=CARTESIAN_POINT('Ctrl Pts',(-9.78111243200006,11.6,4.09604809499999));
#252919=CARTESIAN_POINT('Ctrl Pts',(-9.78319867100006,15.2,4.09640844199998));
#252920=CARTESIAN_POINT('Ctrl Pts',(-9.78319867100006,11.6,4.09640844199998));
#252921=CARTESIAN_POINT('Ctrl Pts',(-9.78529195100006,15.2,4.09676808199999));
#252922=CARTESIAN_POINT('Ctrl Pts',(-9.78529195100006,11.6,4.09676808199999));
#252923=CARTESIAN_POINT('Ctrl Pts',(-9.78739226300006,15.2,4.09712700199999));
#252924=CARTESIAN_POINT('Ctrl Pts',(-9.78739226300006,11.6,4.09712700199999));
#252925=CARTESIAN_POINT('Ctrl Pts',(-9.78949959500006,15.2,4.09748518799999));
#252926=CARTESIAN_POINT('Ctrl Pts',(-9.78949959500006,11.6,4.09748518799999));
#252927=CARTESIAN_POINT('Ctrl Pts',(-9.79161393300006,15.2,4.09784262799998));
#252928=CARTESIAN_POINT('Ctrl Pts',(-9.79161393300006,11.6,4.09784262799998));
#252929=CARTESIAN_POINT('Ctrl Pts',(-9.79373526500006,15.2,4.09819930899998));
#252930=CARTESIAN_POINT('Ctrl Pts',(-9.79373526500006,11.6,4.09819930899998));
#252931=CARTESIAN_POINT('Ctrl Pts',(-9.79586357800006,15.2,4.09855521699999));
#252932=CARTESIAN_POINT('Ctrl Pts',(-9.79586357800006,11.6,4.09855521699999));
#252933=CARTESIAN_POINT('Ctrl Pts',(-9.79799886300006,15.2,4.09891033999998));
#252934=CARTESIAN_POINT('Ctrl Pts',(-9.79799886300006,11.6,4.09891033999998));
#252935=CARTESIAN_POINT('Ctrl Pts',(-9.80014110600005,15.2,4.09926466599998));
#252936=CARTESIAN_POINT('Ctrl Pts',(-9.80014110600005,11.6,4.09926466599998));
#252937=CARTESIAN_POINT('Ctrl Pts',(-9.80229029300006,15.2,4.09961817999999));
#252938=CARTESIAN_POINT('Ctrl Pts',(-9.80229029300006,11.6,4.09961817999999));
#252939=CARTESIAN_POINT('Ctrl Pts',(-9.80444641500006,15.2,4.09997086899998));
#252940=CARTESIAN_POINT('Ctrl Pts',(-9.80444641500006,11.6,4.09997086899998));
#252941=CARTESIAN_POINT('Ctrl Pts',(-9.80660945900006,15.2,4.10032272299999));
#252942=CARTESIAN_POINT('Ctrl Pts',(-9.80660945900006,11.6,4.10032272299999));
#252943=CARTESIAN_POINT('Ctrl Pts',(-9.80877941300006,15.2,4.10067372699999));
#252944=CARTESIAN_POINT('Ctrl Pts',(-9.80877941300006,11.6,4.10067372699999));
#252945=CARTESIAN_POINT('Ctrl Pts',(-9.81095626400006,15.2,4.10102386999998));
#252946=CARTESIAN_POINT('Ctrl Pts',(-9.81095626400006,11.6,4.10102386999998));
#252947=CARTESIAN_POINT('Ctrl Pts',(-9.81314000100006,15.2,4.10137313799999));
#252948=CARTESIAN_POINT('Ctrl Pts',(-9.81314000100006,11.6,4.10137313799999));
#252949=CARTESIAN_POINT('Ctrl Pts',(-9.81533061200006,15.2,4.10172151899998));
#252950=CARTESIAN_POINT('Ctrl Pts',(-9.81533061200006,11.6,4.10172151899998));
#252951=CARTESIAN_POINT('Ctrl Pts',(-9.81752808600006,15.2,4.10206899999999));
#252952=CARTESIAN_POINT('Ctrl Pts',(-9.81752808600006,11.6,4.10206899999999));
#252953=CARTESIAN_POINT('Ctrl Pts',(-9.81973240800006,15.2,4.10241556999999));
#252954=CARTESIAN_POINT('Ctrl Pts',(-9.81973240800006,11.6,4.10241556999999));
#252955=CARTESIAN_POINT('Ctrl Pts',(-9.82194357100006,15.2,4.10276121599999));
#252956=CARTESIAN_POINT('Ctrl Pts',(-9.82194357100006,11.6,4.10276121599999));
#252957=CARTESIAN_POINT('Ctrl Pts',(-9.82416156000006,15.2,4.10310592499999));
#252958=CARTESIAN_POINT('Ctrl Pts',(-9.82416156000006,11.6,4.10310592499999));
#252959=CARTESIAN_POINT('Ctrl Pts',(-9.82638636300005,15.2,4.10344968399999));
#252960=CARTESIAN_POINT('Ctrl Pts',(-9.82638636300005,11.6,4.10344968399999));
#252961=CARTESIAN_POINT('Ctrl Pts',(-9.82861797000006,15.2,4.10379248299999));
#252962=CARTESIAN_POINT('Ctrl Pts',(-9.82861797000006,11.6,4.10379248299999));
#252963=CARTESIAN_POINT('Ctrl Pts',(-9.83085636800006,15.2,4.10413430699998));
#252964=CARTESIAN_POINT('Ctrl Pts',(-9.83085636800006,11.6,4.10413430699998));
#252965=CARTESIAN_POINT('Ctrl Pts',(-9.83310154600006,15.2,4.10447514799999));
#252966=CARTESIAN_POINT('Ctrl Pts',(-9.83310154600006,11.6,4.10447514799999));
#252967=CARTESIAN_POINT('Ctrl Pts',(-9.83535349200006,15.2,4.10481498899999));
#252968=CARTESIAN_POINT('Ctrl Pts',(-9.83535349200006,11.6,4.10481498899998));
#252969=CARTESIAN_POINT('Ctrl Pts',(-9.83761219400006,15.2,4.10515382099998));
#252970=CARTESIAN_POINT('Ctrl Pts',(-9.83761219400006,11.6,4.10515382099998));
#252971=CARTESIAN_POINT('Ctrl Pts',(-9.83987764100006,15.2,4.10549162999998));
#252972=CARTESIAN_POINT('Ctrl Pts',(-9.83987764100006,11.6,4.10549162999998));
#252973=CARTESIAN_POINT('Ctrl Pts',(-9.84214982200006,15.2,4.10582840699998));
#252974=CARTESIAN_POINT('Ctrl Pts',(-9.84214982200006,11.6,4.10582840699998));
#252975=CARTESIAN_POINT('Ctrl Pts',(-9.84442872400006,15.2,4.10616413599998));
#252976=CARTESIAN_POINT('Ctrl Pts',(-9.84442872400006,11.6,4.10616413599998));
#252977=CARTESIAN_POINT('Ctrl Pts',(-9.84671433600005,15.2,4.10649880899999));
#252978=CARTESIAN_POINT('Ctrl Pts',(-9.84671433600005,11.6,4.10649880899999));
#252979=CARTESIAN_POINT('Ctrl Pts',(-9.84900664700006,15.2,4.10683241099999));
#252980=CARTESIAN_POINT('Ctrl Pts',(-9.84900664700006,11.6,4.10683241099999));
#252981=CARTESIAN_POINT('Ctrl Pts',(-9.85130564400006,15.2,4.10716493199998));
#252982=CARTESIAN_POINT('Ctrl Pts',(-9.85130564400006,11.6,4.10716493199998));
#252983=CARTESIAN_POINT('Ctrl Pts',(-9.85361131800006,15.2,4.10749635999998));
#252984=CARTESIAN_POINT('Ctrl Pts',(-9.85361131800006,11.6,4.10749635999998));
#252985=CARTESIAN_POINT('Ctrl Pts',(-9.85592365600005,15.2,4.10782668199998));
#252986=CARTESIAN_POINT('Ctrl Pts',(-9.85592365600005,11.6,4.10782668199998));
#252987=CARTESIAN_POINT('Ctrl Pts',(-9.85824264700006,15.2,4.10815588899998));
#252988=CARTESIAN_POINT('Ctrl Pts',(-9.85824264700006,11.6,4.10815588899998));
#252989=CARTESIAN_POINT('Ctrl Pts',(-9.86056828000006,15.2,4.10848396699999));
#252990=CARTESIAN_POINT('Ctrl Pts',(-9.86056828000006,11.6,4.10848396699999));
#252991=CARTESIAN_POINT('Ctrl Pts',(-9.86290054200006,15.2,4.10881090399998));
#252992=CARTESIAN_POINT('Ctrl Pts',(-9.86290054200006,11.6,4.10881090399998));
#252993=CARTESIAN_POINT('Ctrl Pts',(-9.86523942400006,15.2,4.10913668999999));
#252994=CARTESIAN_POINT('Ctrl Pts',(-9.86523942400006,11.6,4.10913668999999));
#252995=CARTESIAN_POINT('Ctrl Pts',(-9.86758491300006,15.2,4.10946131299998));
#252996=CARTESIAN_POINT('Ctrl Pts',(-9.86758491300006,11.6,4.10946131299998));
#252997=CARTESIAN_POINT('Ctrl Pts',(-9.86993699900006,15.2,4.10978476199999));
#252998=CARTESIAN_POINT('Ctrl Pts',(-9.86993699900006,11.6,4.10978476199999));
#252999=CARTESIAN_POINT('Ctrl Pts',(-9.87229566900006,15.2,4.11010702399999));
#253000=CARTESIAN_POINT('Ctrl Pts',(-9.87229566900006,11.6,4.11010702399999));
#253001=CARTESIAN_POINT('Ctrl Pts',(-9.87466091400006,15.2,4.11042808899998));
#253002=CARTESIAN_POINT('Ctrl Pts',(-9.87466091400006,11.6,4.11042808899998));
#253003=CARTESIAN_POINT('Ctrl Pts',(-9.87703272000006,15.2,4.11074794499999));
#253004=CARTESIAN_POINT('Ctrl Pts',(-9.87703272000006,11.6,4.11074794499999));
#253005=CARTESIAN_POINT('Ctrl Pts',(-9.87941107900006,15.2,4.11106658099998));
#253006=CARTESIAN_POINT('Ctrl Pts',(-9.87941107900006,11.6,4.11106658099998));
#253007=CARTESIAN_POINT('Ctrl Pts',(-9.88179597700006,15.2,4.11138398499999));
#253008=CARTESIAN_POINT('Ctrl Pts',(-9.88179597700006,11.6,4.11138398499998));
#253009=CARTESIAN_POINT('Ctrl Pts',(-9.88418740600006,15.2,4.11170014699999));
#253010=CARTESIAN_POINT('Ctrl Pts',(-9.88418740600006,11.6,4.11170014699999));
#253011=CARTESIAN_POINT('Ctrl Pts',(-9.88658535100006,15.2,4.11201505499999));
#253012=CARTESIAN_POINT('Ctrl Pts',(-9.88658535100006,11.6,4.11201505499999));
#253013=CARTESIAN_POINT('Ctrl Pts',(-9.88898980500006,15.2,4.11232869699998));
#253014=CARTESIAN_POINT('Ctrl Pts',(-9.88898980500006,11.6,4.11232869699998));
#253015=CARTESIAN_POINT('Ctrl Pts',(-9.89140075400006,15.2,4.11264106399998));
#253016=CARTESIAN_POINT('Ctrl Pts',(-9.89140075400006,11.6,4.11264106399998));
#253017=CARTESIAN_POINT('Ctrl Pts',(-9.89381818800006,15.2,4.11295214299999));
#253018=CARTESIAN_POINT('Ctrl Pts',(-9.89381818800006,11.6,4.11295214299999));
#253019=CARTESIAN_POINT('Ctrl Pts',(-9.89624209600005,15.2,4.11326192399999));
#253020=CARTESIAN_POINT('Ctrl Pts',(-9.89624209600005,11.6,4.11326192399999));
#253021=CARTESIAN_POINT('Ctrl Pts',(-9.89867246700006,15.2,4.11357039599999));
#253022=CARTESIAN_POINT('Ctrl Pts',(-9.89867246700006,11.6,4.11357039599998));
#253023=CARTESIAN_POINT('Ctrl Pts',(-9.90110928900006,15.2,4.11387754799998));
#253024=CARTESIAN_POINT('Ctrl Pts',(-9.90110928900006,11.6,4.11387754799998));
#253025=CARTESIAN_POINT('Ctrl Pts',(-9.90355255300006,15.2,4.11418336699998));
#253026=CARTESIAN_POINT('Ctrl Pts',(-9.90355255300006,11.6,4.11418336699998));
#253027=CARTESIAN_POINT('Ctrl Pts',(-9.90600224700006,15.2,4.11448784599998));
#253028=CARTESIAN_POINT('Ctrl Pts',(-9.90600224700006,11.6,4.11448784599998));
#253029=CARTESIAN_POINT('Ctrl Pts',(-9.90845836000006,15.2,4.11479096999999));
#253030=CARTESIAN_POINT('Ctrl Pts',(-9.90845836000006,11.6,4.11479096999999));
#253031=CARTESIAN_POINT('Ctrl Pts',(-9.91092088200006,15.2,4.11509273099998));
#253032=CARTESIAN_POINT('Ctrl Pts',(-9.91092088200006,11.6,4.11509273099998));
#253033=CARTESIAN_POINT('Ctrl Pts',(-9.91338980100006,15.2,4.11539311699999));
#253034=CARTESIAN_POINT('Ctrl Pts',(-9.91338980100006,11.6,4.11539311699998));
#253035=CARTESIAN_POINT('Ctrl Pts',(-9.91586510700006,15.2,4.11569211899998));
#253036=CARTESIAN_POINT('Ctrl Pts',(-9.91586510700006,11.6,4.11569211899998));
#253037=CARTESIAN_POINT('Ctrl Pts',(-9.91834678800006,15.2,4.11598972399998));
#253038=CARTESIAN_POINT('Ctrl Pts',(-9.91834678800006,11.6,4.11598972399998));
#253039=CARTESIAN_POINT('Ctrl Pts',(-9.92083483500006,15.2,4.11628592099999));
#253040=CARTESIAN_POINT('Ctrl Pts',(-9.92083483500006,11.6,4.11628592099999));
#253041=CARTESIAN_POINT('Ctrl Pts',(-9.92332923600006,15.2,4.11658070199999));
#253042=CARTESIAN_POINT('Ctrl Pts',(-9.92332923600006,11.6,4.11658070199999));
#253043=CARTESIAN_POINT('Ctrl Pts',(-9.92582998100006,15.2,4.11687405499999));
#253044=CARTESIAN_POINT('Ctrl Pts',(-9.92582998100006,11.6,4.11687405499999));
#253045=CARTESIAN_POINT('Ctrl Pts',(-9.92833705900006,15.2,4.11716596899999));
#253046=CARTESIAN_POINT('Ctrl Pts',(-9.92833705900006,11.6,4.11716596899998));
#253047=CARTESIAN_POINT('Ctrl Pts',(-9.93085045900006,15.2,4.11745643499999));
#253048=CARTESIAN_POINT('Ctrl Pts',(-9.93085045900006,11.6,4.11745643499999));
#253049=CARTESIAN_POINT('Ctrl Pts',(-9.93337017000006,15.2,4.11774543999999));
#253050=CARTESIAN_POINT('Ctrl Pts',(-9.93337017000006,11.6,4.11774543999999));
#253051=CARTESIAN_POINT('Ctrl Pts',(-9.93589618200006,15.2,4.11803297499999));
#253052=CARTESIAN_POINT('Ctrl Pts',(-9.93589618200006,11.6,4.11803297499999));
#253053=CARTESIAN_POINT('Ctrl Pts',(-9.93842848600006,15.2,4.11831903099999));
#253054=CARTESIAN_POINT('Ctrl Pts',(-9.93842848600006,11.6,4.11831903099999));
#253055=CARTESIAN_POINT('Ctrl Pts',(-9.94096706800006,15.2,4.11860359499999));
#253056=CARTESIAN_POINT('Ctrl Pts',(-9.94096706800006,11.6,4.11860359499998));
#253057=CARTESIAN_POINT('Ctrl Pts',(-9.94351191900006,15.2,4.11888665699998));
#253058=CARTESIAN_POINT('Ctrl Pts',(-9.94351191900006,11.6,4.11888665699998));
#253059=CARTESIAN_POINT('Ctrl Pts',(-9.94606302900005,15.2,4.11916820899999));
#253060=CARTESIAN_POINT('Ctrl Pts',(-9.94606302900005,11.6,4.11916820899999));
#253061=CARTESIAN_POINT('Ctrl Pts',(-9.94862038700006,15.2,4.11944823899999));
#253062=CARTESIAN_POINT('Ctrl Pts',(-9.94862038700006,11.6,4.11944823899999));
#253063=CARTESIAN_POINT('Ctrl Pts',(-9.95118398200006,15.2,4.11972673699999));
#253064=CARTESIAN_POINT('Ctrl Pts',(-9.95118398200006,11.6,4.11972673699999));
#253065=CARTESIAN_POINT('Ctrl Pts',(-9.95375380500005,15.2,4.12000369299999));
#253066=CARTESIAN_POINT('Ctrl Pts',(-9.95375380500005,11.6,4.12000369299999));
#253067=CARTESIAN_POINT('Ctrl Pts',(-9.95632984400006,15.2,4.12027909599999));
#253068=CARTESIAN_POINT('Ctrl Pts',(-9.95632984400006,11.6,4.12027909599998));
#253069=CARTESIAN_POINT('Ctrl Pts',(-9.95891208900006,15.2,4.12055293699999));
#253070=CARTESIAN_POINT('Ctrl Pts',(-9.95891208900006,11.6,4.12055293699999));
#253071=CARTESIAN_POINT('Ctrl Pts',(-9.96150052900006,15.2,4.12082520499998));
#253072=CARTESIAN_POINT('Ctrl Pts',(-9.96150052900006,11.6,4.12082520499998));
#253073=CARTESIAN_POINT('Ctrl Pts',(-9.96409515500006,15.2,4.12109588999999));
#253074=CARTESIAN_POINT('Ctrl Pts',(-9.96409515500006,11.6,4.12109588999999));
#253075=CARTESIAN_POINT('Ctrl Pts',(-9.96669595600006,15.2,4.12136498299999));
#253076=CARTESIAN_POINT('Ctrl Pts',(-9.96669595600006,11.6,4.12136498299999));
#253077=CARTESIAN_POINT('Ctrl Pts',(-9.96930292000006,15.2,4.12163247299999));
#253078=CARTESIAN_POINT('Ctrl Pts',(-9.96930292000006,11.6,4.12163247299999));
#253079=CARTESIAN_POINT('Ctrl Pts',(-9.97191603900006,15.2,4.12189835099999));
#253080=CARTESIAN_POINT('Ctrl Pts',(-9.97191603900006,11.6,4.12189835099999));
#253081=CARTESIAN_POINT('Ctrl Pts',(-9.97453530200006,15.2,4.12216260499999));
#253082=CARTESIAN_POINT('Ctrl Pts',(-9.97453530200006,11.6,4.12216260499999));
#253083=CARTESIAN_POINT('Ctrl Pts',(-9.97716069800006,15.2,4.12242522699999));
#253084=CARTESIAN_POINT('Ctrl Pts',(-9.97716069800006,11.6,4.12242522699999));
#253085=CARTESIAN_POINT('Ctrl Pts',(-9.97979221700006,15.2,4.12268620699999));
#253086=CARTESIAN_POINT('Ctrl Pts',(-9.97979221700006,11.6,4.12268620699999));
#253087=CARTESIAN_POINT('Ctrl Pts',(-9.98242984800006,15.2,4.12294553499999));
#253088=CARTESIAN_POINT('Ctrl Pts',(-9.98242984800006,11.6,4.12294553499999));
#253089=CARTESIAN_POINT('Ctrl Pts',(-9.98507358300006,15.2,4.12320320099998));
#253090=CARTESIAN_POINT('Ctrl Pts',(-9.98507358300006,11.6,4.12320320099998));
#253091=CARTESIAN_POINT('Ctrl Pts',(-9.98772341000006,15.2,4.12345919499998));
#253092=CARTESIAN_POINT('Ctrl Pts',(-9.98772341000006,11.6,4.12345919499998));
#253093=CARTESIAN_POINT('Ctrl Pts',(-9.99037931900006,15.2,4.12371350699999));
#253094=CARTESIAN_POINT('Ctrl Pts',(-9.99037931900006,11.6,4.12371350699999));
#253095=CARTESIAN_POINT('Ctrl Pts',(-9.99304129900005,15.2,4.12396612799999));
#253096=CARTESIAN_POINT('Ctrl Pts',(-9.99304129900005,11.6,4.12396612799998));
#253097=CARTESIAN_POINT('Ctrl Pts',(-9.99570934200005,15.2,4.12421704799999));
#253098=CARTESIAN_POINT('Ctrl Pts',(-9.99570934200005,11.6,4.12421704799998));
#253099=CARTESIAN_POINT('Ctrl Pts',(-9.99838343600005,15.2,4.12446625799999));
#253100=CARTESIAN_POINT('Ctrl Pts',(-9.99838343600005,11.6,4.12446625799998));
#253101=CARTESIAN_POINT('Ctrl Pts',(-10.0010635710001,15.2,4.12471374699999));
#253102=CARTESIAN_POINT('Ctrl Pts',(-10.0010635710001,11.6,4.12471374699999));
#253103=CARTESIAN_POINT('Ctrl Pts',(-10.0037497380001,15.2,4.12495950799999));
#253104=CARTESIAN_POINT('Ctrl Pts',(-10.0037497380001,11.6,4.12495950799998));
#253105=CARTESIAN_POINT('Ctrl Pts',(-10.0064419260001,15.2,4.12520352799999));
#253106=CARTESIAN_POINT('Ctrl Pts',(-10.0064419260001,11.6,4.12520352799999));
#253107=CARTESIAN_POINT('Ctrl Pts',(-10.0091401250001,15.2,4.12544580099999));
#253108=CARTESIAN_POINT('Ctrl Pts',(-10.0091401250001,11.6,4.12544580099999));
#253109=CARTESIAN_POINT('Ctrl Pts',(-10.0118443250001,15.2,4.12568631499998));
#253110=CARTESIAN_POINT('Ctrl Pts',(-10.0118443250001,11.6,4.12568631499998));
#253111=CARTESIAN_POINT('Ctrl Pts',(-10.0145545170001,15.2,4.12592506099998));
#253112=CARTESIAN_POINT('Ctrl Pts',(-10.0145545170001,11.6,4.12592506099998));
#253113=CARTESIAN_POINT('Ctrl Pts',(-10.0172706880001,15.2,4.12616202899999));
#253114=CARTESIAN_POINT('Ctrl Pts',(-10.0172706880001,11.6,4.12616202899999));
#253115=CARTESIAN_POINT('Ctrl Pts',(-10.0199928310001,15.2,4.12639721199999));
#253116=CARTESIAN_POINT('Ctrl Pts',(-10.0199928310001,11.6,4.12639721199999));
#253117=CARTESIAN_POINT('Ctrl Pts',(-10.0227209350001,15.2,4.12663059799999));
#253118=CARTESIAN_POINT('Ctrl Pts',(-10.0227209350001,11.6,4.12663059799998));
#253119=CARTESIAN_POINT('Ctrl Pts',(-10.0254549900001,15.2,4.12686217999998));
#253120=CARTESIAN_POINT('Ctrl Pts',(-10.0254549900001,11.6,4.12686217999998));
#253121=CARTESIAN_POINT('Ctrl Pts',(-10.0281949850001,15.2,4.12709194699998));
#253122=CARTESIAN_POINT('Ctrl Pts',(-10.0281949850001,11.6,4.12709194699998));
#253123=CARTESIAN_POINT('Ctrl Pts',(-10.0309409120001,15.2,4.12731989099999));
#253124=CARTESIAN_POINT('Ctrl Pts',(-10.0309409120001,11.6,4.12731989099999));
#253125=CARTESIAN_POINT('Ctrl Pts',(-10.0336927600001,15.2,4.12754600099999));
#253126=CARTESIAN_POINT('Ctrl Pts',(-10.0336927600001,11.6,4.12754600099999));
#253127=CARTESIAN_POINT('Ctrl Pts',(-10.0364505200001,15.2,4.12777026899998));
#253128=CARTESIAN_POINT('Ctrl Pts',(-10.0364505200001,11.6,4.12777026899998));
#253129=CARTESIAN_POINT('Ctrl Pts',(-10.0392141810001,15.2,4.12799268699998));
#253130=CARTESIAN_POINT('Ctrl Pts',(-10.0392141810001,11.6,4.12799268699998));
#253131=CARTESIAN_POINT('Ctrl Pts',(-10.0419837320001,15.2,4.12821324399999));
#253132=CARTESIAN_POINT('Ctrl Pts',(-10.0419837320001,11.6,4.12821324399999));
#253133=CARTESIAN_POINT('Ctrl Pts',(-10.0447591670001,15.2,4.12843193099998));
#253134=CARTESIAN_POINT('Ctrl Pts',(-10.0447591670001,11.6,4.12843193099998));
#253135=CARTESIAN_POINT('Ctrl Pts',(-10.0475404720001,15.2,4.12864873899998));
#253136=CARTESIAN_POINT('Ctrl Pts',(-10.0475404720001,11.6,4.12864873899998));
#253137=CARTESIAN_POINT('Ctrl Pts',(-10.0503276400001,15.2,4.12886365899999));
#253138=CARTESIAN_POINT('Ctrl Pts',(-10.0503276400001,11.6,4.12886365899999));
#253139=CARTESIAN_POINT('Ctrl Pts',(-10.0531206590001,15.2,4.12907668399999));
#253140=CARTESIAN_POINT('Ctrl Pts',(-10.0531206590001,11.6,4.12907668399999));
#253141=CARTESIAN_POINT('Ctrl Pts',(-10.0559195220001,15.2,4.12928780199999));
#253142=CARTESIAN_POINT('Ctrl Pts',(-10.0559195220001,11.6,4.12928780199999));
#253143=CARTESIAN_POINT('Ctrl Pts',(-10.0587242160001,15.2,4.12949700499999));
#253144=CARTESIAN_POINT('Ctrl Pts',(-10.0587242160001,11.6,4.12949700499999));
#253145=CARTESIAN_POINT('Ctrl Pts',(-10.0615347350001,15.2,4.12970428599999));
#253146=CARTESIAN_POINT('Ctrl Pts',(-10.0615347350001,11.6,4.12970428599999));
#253147=CARTESIAN_POINT('Ctrl Pts',(-10.0643510650001,15.2,4.12990963299999));
#253148=CARTESIAN_POINT('Ctrl Pts',(-10.0643510650001,11.6,4.12990963299999));
#253149=CARTESIAN_POINT('Ctrl Pts',(-10.0671731990001,15.2,4.13011303899999));
#253150=CARTESIAN_POINT('Ctrl Pts',(-10.0671731990001,11.6,4.13011303899999));
#253151=CARTESIAN_POINT('Ctrl Pts',(-10.0700011270001,15.2,4.13031449499999));
#253152=CARTESIAN_POINT('Ctrl Pts',(-10.0700011270001,11.6,4.13031449499999));
#253153=CARTESIAN_POINT('Ctrl Pts',(-10.0728348400001,15.2,4.13051399199999));
#253154=CARTESIAN_POINT('Ctrl Pts',(-10.0728348400001,11.6,4.13051399199999));
#253155=CARTESIAN_POINT('Ctrl Pts',(-10.0756743260001,15.2,4.13071152099998));
#253156=CARTESIAN_POINT('Ctrl Pts',(-10.0756743260001,11.6,4.13071152099998));
#253157=CARTESIAN_POINT('Ctrl Pts',(-10.0785195780001,15.2,4.13090707399999));
#253158=CARTESIAN_POINT('Ctrl Pts',(-10.0785195780001,11.6,4.13090707399998));
#253159=CARTESIAN_POINT('Ctrl Pts',(-10.0813705840001,15.2,4.13110064099998));
#253160=CARTESIAN_POINT('Ctrl Pts',(-10.0813705840001,11.6,4.13110064099998));
#253161=CARTESIAN_POINT('Ctrl Pts',(-10.0842273370001,15.2,4.13129221499998));
#253162=CARTESIAN_POINT('Ctrl Pts',(-10.0842273370001,11.6,4.13129221499998));
#253163=CARTESIAN_POINT('Ctrl Pts',(-10.0870898240001,15.2,4.13148178499998));
#253164=CARTESIAN_POINT('Ctrl Pts',(-10.0870898240001,11.6,4.13148178499998));
#253165=CARTESIAN_POINT('Ctrl Pts',(-10.0899580390001,15.2,4.13166934399998));
#253166=CARTESIAN_POINT('Ctrl Pts',(-10.0899580390001,11.6,4.13166934399998));
#253167=CARTESIAN_POINT('Ctrl Pts',(-10.0928319700001,15.2,4.13185488299998));
#253168=CARTESIAN_POINT('Ctrl Pts',(-10.0928319700001,11.6,4.13185488299998));
#253169=CARTESIAN_POINT('Ctrl Pts',(-10.0957116090001,15.2,4.13203839299998));
#253170=CARTESIAN_POINT('Ctrl Pts',(-10.0957116090001,11.6,4.13203839299998));
#253171=CARTESIAN_POINT('Ctrl Pts',(-10.0985969450001,15.2,4.13221986699998));
#253172=CARTESIAN_POINT('Ctrl Pts',(-10.0985969450001,11.6,4.13221986699998));
#253173=CARTESIAN_POINT('Ctrl Pts',(-10.1014879690001,15.2,4.13239929399998));
#253174=CARTESIAN_POINT('Ctrl Pts',(-10.1014879690001,11.6,4.13239929399998));
#253175=CARTESIAN_POINT('Ctrl Pts',(-10.1043846720001,15.2,4.13257666799999));
#253176=CARTESIAN_POINT('Ctrl Pts',(-10.1043846720001,11.6,4.13257666799998));
#253177=CARTESIAN_POINT('Ctrl Pts',(-10.1072870450001,15.2,4.13275197899999));
#253178=CARTESIAN_POINT('Ctrl Pts',(-10.1072870450001,11.6,4.13275197899999));
#253179=CARTESIAN_POINT('Ctrl Pts',(-10.1101950770001,15.2,4.13292521799999));
#253180=CARTESIAN_POINT('Ctrl Pts',(-10.1101950770001,11.6,4.13292521799998));
#253181=CARTESIAN_POINT('Ctrl Pts',(-10.1131087590001,15.2,4.13309637799999));
#253182=CARTESIAN_POINT('Ctrl Pts',(-10.1131087590001,11.6,4.13309637799998));
#253183=CARTESIAN_POINT('Ctrl Pts',(-10.1160280820001,15.2,4.13326544999999));
#253184=CARTESIAN_POINT('Ctrl Pts',(-10.1160280820001,11.6,4.13326544999998));
#253185=CARTESIAN_POINT('Ctrl Pts',(-10.1189530370001,15.2,4.13343242499998));
#253186=CARTESIAN_POINT('Ctrl Pts',(-10.1189530370001,11.6,4.13343242499998));
#253187=CARTESIAN_POINT('Ctrl Pts',(-10.1218836130001,15.2,4.13359729699999));
#253188=CARTESIAN_POINT('Ctrl Pts',(-10.1218836130001,11.6,4.13359729699999));
#253189=CARTESIAN_POINT('Ctrl Pts',(-10.1248198030001,15.2,4.13376005499998));
#253190=CARTESIAN_POINT('Ctrl Pts',(-10.1248198030001,11.6,4.13376005499998));
#253191=CARTESIAN_POINT('Ctrl Pts',(-10.1277615950001,15.2,4.13392069099999));
#253192=CARTESIAN_POINT('Ctrl Pts',(-10.1277615950001,11.6,4.13392069099999));
#253193=CARTESIAN_POINT('Ctrl Pts',(-10.1307089820001,15.2,4.13407919799998));
#253194=CARTESIAN_POINT('Ctrl Pts',(-10.1307089820001,11.6,4.13407919799998));
#253195=CARTESIAN_POINT('Ctrl Pts',(-10.1336619530001,15.2,4.13423556699998));
#253196=CARTESIAN_POINT('Ctrl Pts',(-10.1336619530001,11.6,4.13423556699998));
#253197=CARTESIAN_POINT('Ctrl Pts',(-10.1366205000001,15.2,4.13438978999999));
#253198=CARTESIAN_POINT('Ctrl Pts',(-10.1366205000001,11.6,4.13438978999999));
#253199=CARTESIAN_POINT('Ctrl Pts',(-10.1395846120001,15.2,4.13454185899998));
#253200=CARTESIAN_POINT('Ctrl Pts',(-10.1395846120001,11.6,4.13454185899998));
#253201=CARTESIAN_POINT('Ctrl Pts',(-10.1425542810001,15.2,4.13469176499999));
#253202=CARTESIAN_POINT('Ctrl Pts',(-10.1425542810001,11.6,4.13469176499999));
#253203=CARTESIAN_POINT('Ctrl Pts',(-10.1455294970001,15.2,4.13483949999998));
#253204=CARTESIAN_POINT('Ctrl Pts',(-10.1455294970001,11.6,4.13483949999998));
#253205=CARTESIAN_POINT('Ctrl Pts',(-10.1485102510001,15.2,4.13498505799998));
#253206=CARTESIAN_POINT('Ctrl Pts',(-10.1485102510001,11.6,4.13498505799998));
#253207=CARTESIAN_POINT('Ctrl Pts',(-10.1514965350001,15.2,4.13512842799998));
#253208=CARTESIAN_POINT('Ctrl Pts',(-10.1514965350001,11.6,4.13512842799998));
#253209=CARTESIAN_POINT('Ctrl Pts',(-10.1544883380001,15.2,4.13526960399999));
#253210=CARTESIAN_POINT('Ctrl Pts',(-10.1544883380001,11.6,4.13526960399999));
#253211=CARTESIAN_POINT('Ctrl Pts',(-10.1574856510001,15.2,4.13540857599998));
#253212=CARTESIAN_POINT('Ctrl Pts',(-10.1574856510001,11.6,4.13540857599998));
#253213=CARTESIAN_POINT('Ctrl Pts',(-10.1604884650001,15.2,4.13554533699998));
#253214=CARTESIAN_POINT('Ctrl Pts',(-10.1604884650001,11.6,4.13554533699998));
#253215=CARTESIAN_POINT('Ctrl Pts',(-10.1634967710001,15.2,4.13567987999999));
#253216=CARTESIAN_POINT('Ctrl Pts',(-10.1634967710001,11.6,4.13567987999999));
#253217=CARTESIAN_POINT('Ctrl Pts',(-10.1665105610001,15.2,4.13581219599998));
#253218=CARTESIAN_POINT('Ctrl Pts',(-10.1665105610001,11.6,4.13581219599998));
#253219=CARTESIAN_POINT('Ctrl Pts',(-10.1695298240001,15.2,4.13594227699999));
#253220=CARTESIAN_POINT('Ctrl Pts',(-10.1695298240001,11.6,4.13594227699999));
#253221=CARTESIAN_POINT('Ctrl Pts',(-10.1725545500001,15.2,4.13607011499998));
#253222=CARTESIAN_POINT('Ctrl Pts',(-10.1725545500001,11.6,4.13607011499998));
#253223=CARTESIAN_POINT('Ctrl Pts',(-10.1755847340001,15.2,4.13619570299999));
#253224=CARTESIAN_POINT('Ctrl Pts',(-10.1755847340001,11.6,4.13619570299998));
#253225=CARTESIAN_POINT('Ctrl Pts',(-10.1786203620001,15.2,4.13631903199998));
#253226=CARTESIAN_POINT('Ctrl Pts',(-10.1786203620001,11.6,4.13631903199998));
#253227=CARTESIAN_POINT('Ctrl Pts',(-10.1816614280001,15.2,4.13644009499999));
#253228=CARTESIAN_POINT('Ctrl Pts',(-10.1816614280001,11.6,4.13644009499999));
#253229=CARTESIAN_POINT('Ctrl Pts',(-10.1847079220001,15.2,4.13655888299999));
#253230=CARTESIAN_POINT('Ctrl Pts',(-10.1847079220001,11.6,4.13655888299999));
#253231=CARTESIAN_POINT('Ctrl Pts',(-10.1877598350001,15.2,4.13667538999999));
#253232=CARTESIAN_POINT('Ctrl Pts',(-10.1877598350001,11.6,4.13667538999999));
#253233=CARTESIAN_POINT('Ctrl Pts',(-10.1908171570001,15.2,4.13678960699999));
#253234=CARTESIAN_POINT('Ctrl Pts',(-10.1908171570001,11.6,4.13678960699999));
#253235=CARTESIAN_POINT('Ctrl Pts',(-10.1938798810001,15.2,4.13690152799998));
#253236=CARTESIAN_POINT('Ctrl Pts',(-10.1938798810001,11.6,4.13690152799998));
#253237=CARTESIAN_POINT('Ctrl Pts',(-10.1969479960001,15.2,4.13701114199998));
#253238=CARTESIAN_POINT('Ctrl Pts',(-10.1969479960001,11.6,4.13701114199998));
#253239=CARTESIAN_POINT('Ctrl Pts',(-10.2000214950001,15.2,4.13711844399998));
#253240=CARTESIAN_POINT('Ctrl Pts',(-10.2000214950001,11.6,4.13711844399998));
#253241=CARTESIAN_POINT('Ctrl Pts',(-10.2031003670001,15.2,4.13722342499998));
#253242=CARTESIAN_POINT('Ctrl Pts',(-10.2031003670001,11.6,4.13722342499998));
#253243=CARTESIAN_POINT('Ctrl Pts',(-10.2061846030001,15.2,4.13732607699998));
#253244=CARTESIAN_POINT('Ctrl Pts',(-10.2061846030001,11.6,4.13732607699998));
#253245=CARTESIAN_POINT('Ctrl Pts',(-10.2092741960001,15.2,4.13742639399998));
#253246=CARTESIAN_POINT('Ctrl Pts',(-10.2092741960001,11.6,4.13742639399998));
#253247=CARTESIAN_POINT('Ctrl Pts',(-10.2123691360001,15.2,4.13752436799999));
#253248=CARTESIAN_POINT('Ctrl Pts',(-10.2123691360001,11.6,4.13752436799999));
#253249=CARTESIAN_POINT('Ctrl Pts',(-10.2154694120001,15.2,4.13761999099999));
#253250=CARTESIAN_POINT('Ctrl Pts',(-10.2154694120001,11.6,4.13761999099999));
#253251=CARTESIAN_POINT('Ctrl Pts',(-10.2185750180001,15.2,4.13771325499999));
#253252=CARTESIAN_POINT('Ctrl Pts',(-10.2185750180001,11.6,4.13771325499999));
#253253=CARTESIAN_POINT('Ctrl Pts',(-10.2216859440001,15.2,4.13780415299998));
#253254=CARTESIAN_POINT('Ctrl Pts',(-10.2216859440001,11.6,4.13780415299998));
#253255=CARTESIAN_POINT('Ctrl Pts',(-10.2248021810001,15.2,4.13789267699999));
#253256=CARTESIAN_POINT('Ctrl Pts',(-10.2248021810001,11.6,4.13789267699998));
#253257=CARTESIAN_POINT('Ctrl Pts',(-10.2279237210001,15.2,4.13797881999999));
#253258=CARTESIAN_POINT('Ctrl Pts',(-10.2279237210001,11.6,4.13797881999999));
#253259=CARTESIAN_POINT('Ctrl Pts',(-10.2310505530001,15.2,4.13806257599998));
#253260=CARTESIAN_POINT('Ctrl Pts',(-10.2310505530001,11.6,4.13806257599998));
#253261=CARTESIAN_POINT('Ctrl Pts',(-10.2341826700001,15.2,4.13814393399999));
#253262=CARTESIAN_POINT('Ctrl Pts',(-10.2341826700001,11.6,4.13814393399999));
#253263=CARTESIAN_POINT('Ctrl Pts',(-10.2373200620001,15.2,4.13822288999998));
#253264=CARTESIAN_POINT('Ctrl Pts',(-10.2373200620001,11.6,4.13822288999998));
#253265=CARTESIAN_POINT('Ctrl Pts',(-10.2404627220001,15.2,4.13829943499999));
#253266=CARTESIAN_POINT('Ctrl Pts',(-10.2404627220001,11.6,4.13829943499999));
#253267=CARTESIAN_POINT('Ctrl Pts',(-10.2436106390001,15.2,4.13837356099998));
#253268=CARTESIAN_POINT('Ctrl Pts',(-10.2436106390001,11.6,4.13837356099998));
#253269=CARTESIAN_POINT('Ctrl Pts',(-10.2467638050001,15.2,4.13844526199998));
#253270=CARTESIAN_POINT('Ctrl Pts',(-10.2467638050001,11.6,4.13844526199998));
#253271=CARTESIAN_POINT('Ctrl Pts',(-10.2499222120001,15.2,4.13851453099999));
#253272=CARTESIAN_POINT('Ctrl Pts',(-10.2499222120001,11.6,4.13851453099999));
#253273=CARTESIAN_POINT('Ctrl Pts',(-10.2530858490001,15.2,4.13858135799998));
#253274=CARTESIAN_POINT('Ctrl Pts',(-10.2530858490001,11.6,4.13858135799998));
#253275=CARTESIAN_POINT('Ctrl Pts',(-10.2562547100001,15.2,4.13864573899998));
#253276=CARTESIAN_POINT('Ctrl Pts',(-10.2562547100001,11.6,4.13864573899998));
#253277=CARTESIAN_POINT('Ctrl Pts',(-10.2594287840001,15.2,4.13870766499999));
#253278=CARTESIAN_POINT('Ctrl Pts',(-10.2594287840001,11.6,4.13870766499999));
#253279=CARTESIAN_POINT('Ctrl Pts',(-10.2626080630001,15.2,4.13876712999999));
#253280=CARTESIAN_POINT('Ctrl Pts',(-10.2626080630001,11.6,4.13876712999999));
#253281=CARTESIAN_POINT('Ctrl Pts',(-10.2657925390001,15.2,4.13882412399998));
#253282=CARTESIAN_POINT('Ctrl Pts',(-10.2657925390001,11.6,4.13882412399998));
#253283=CARTESIAN_POINT('Ctrl Pts',(-10.2689822020001,15.2,4.13887864299999));
#253284=CARTESIAN_POINT('Ctrl Pts',(-10.2689822020001,11.6,4.13887864299998));
#253285=CARTESIAN_POINT('Ctrl Pts',(-10.2721770450001,15.2,4.13893067799999));
#253286=CARTESIAN_POINT('Ctrl Pts',(-10.2721770450001,11.6,4.13893067799999));
#253287=CARTESIAN_POINT('Ctrl Pts',(-10.2753770580001,15.2,4.13898022199999));
#253288=CARTESIAN_POINT('Ctrl Pts',(-10.2753770580001,11.6,4.13898022199999));
#253289=CARTESIAN_POINT('Ctrl Pts',(-10.2785822320001,15.2,4.13902726899998));
#253290=CARTESIAN_POINT('Ctrl Pts',(-10.2785822320001,11.6,4.13902726899998));
#253291=CARTESIAN_POINT('Ctrl Pts',(-10.2817925600001,15.2,4.13907181099999));
#253292=CARTESIAN_POINT('Ctrl Pts',(-10.2817925600001,11.6,4.13907181099999));
#253293=CARTESIAN_POINT('Ctrl Pts',(-10.2850080310001,15.2,4.13911384099999));
#253294=CARTESIAN_POINT('Ctrl Pts',(-10.2850080310001,11.6,4.13911384099999));
#253295=CARTESIAN_POINT('Ctrl Pts',(-10.2882286380001,15.2,4.13915335199999));
#253296=CARTESIAN_POINT('Ctrl Pts',(-10.2882286380001,11.6,4.13915335199999));
#253297=CARTESIAN_POINT('Ctrl Pts',(-10.2914543720001,15.2,4.13919033599999));
#253298=CARTESIAN_POINT('Ctrl Pts',(-10.2914543720001,11.6,4.13919033599999));
#253299=CARTESIAN_POINT('Ctrl Pts',(-10.2946852240001,15.2,4.13922478899998));
#253300=CARTESIAN_POINT('Ctrl Pts',(-10.2946852240001,11.6,4.13922478899998));
#253301=CARTESIAN_POINT('Ctrl Pts',(-10.2979211850001,15.2,4.13925669999998));
#253302=CARTESIAN_POINT('Ctrl Pts',(-10.2979211850001,11.6,4.13925669999998));
#253303=CARTESIAN_POINT('Ctrl Pts',(-10.3011622480001,15.2,4.13928606399999));
#253304=CARTESIAN_POINT('Ctrl Pts',(-10.3011622480001,11.6,4.13928606399998));
#253305=CARTESIAN_POINT('Ctrl Pts',(-10.3044084030001,15.2,4.13931287499998));
#253306=CARTESIAN_POINT('Ctrl Pts',(-10.3044084030001,11.6,4.13931287499998));
#253307=CARTESIAN_POINT('Ctrl Pts',(-10.3076596430001,15.2,4.13933712499999));
#253308=CARTESIAN_POINT('Ctrl Pts',(-10.3076596430001,11.6,4.13933712499999));
#253309=CARTESIAN_POINT('Ctrl Pts',(-10.3109159570001,15.2,4.13935880599999));
#253310=CARTESIAN_POINT('Ctrl Pts',(-10.3109159570001,11.6,4.13935880599999));
#253311=CARTESIAN_POINT('Ctrl Pts',(-10.3141773370001,15.2,4.13937791399999));
#253312=CARTESIAN_POINT('Ctrl Pts',(-10.3141773370001,11.6,4.13937791399999));
#253313=CARTESIAN_POINT('Ctrl Pts',(-10.3174437770001,15.2,4.13939443899999));
#253314=CARTESIAN_POINT('Ctrl Pts',(-10.3174437770001,11.6,4.13939443899999));
#253315=CARTESIAN_POINT('Ctrl Pts',(-10.3207152650001,15.2,4.13940837599998));
#253316=CARTESIAN_POINT('Ctrl Pts',(-10.3207152650001,11.6,4.13940837599998));
#253317=CARTESIAN_POINT('Ctrl Pts',(-10.3239917950001,15.2,4.13941971799999));
#253318=CARTESIAN_POINT('Ctrl Pts',(-10.3239917950001,11.6,4.13941971799998));
#253319=CARTESIAN_POINT('Ctrl Pts',(-10.3272733590001,15.2,4.13942845699999));
#253320=CARTESIAN_POINT('Ctrl Pts',(-10.3272733590001,11.6,4.13942845699999));
#253321=CARTESIAN_POINT('Ctrl Pts',(-10.3305599450001,15.2,4.13943458699999));
#253322=CARTESIAN_POINT('Ctrl Pts',(-10.3305599450001,11.6,4.13943458699999));
#253323=CARTESIAN_POINT('Ctrl Pts',(-10.3338515480001,15.2,4.13943810199999));
#253324=CARTESIAN_POINT('Ctrl Pts',(-10.3338515480001,11.6,4.13943810199999));
#253325=CARTESIAN_POINT('Ctrl Pts',(-10.3371481570001,15.2,4.13943899399998));
#253326=CARTESIAN_POINT('Ctrl Pts',(-10.3371481570001,11.6,4.13943899399998));
#253327=CARTESIAN_POINT('Ctrl Pts',(-10.3404497650001,15.2,4.13943725699998));
#253328=CARTESIAN_POINT('Ctrl Pts',(-10.3404497650001,11.6,4.13943725699998));
#253329=CARTESIAN_POINT('Ctrl Pts',(-10.3437563640001,15.2,4.13943288499999));
#253330=CARTESIAN_POINT('Ctrl Pts',(-10.3437563640001,11.6,4.13943288499999));
#253331=CARTESIAN_POINT('Ctrl Pts',(-10.3470679440001,15.2,4.13942586999998));
#253332=CARTESIAN_POINT('Ctrl Pts',(-10.3470679440001,11.6,4.13942586999998));
#253333=CARTESIAN_POINT('Ctrl Pts',(-10.3503844980001,15.2,4.13941620499998));
#253334=CARTESIAN_POINT('Ctrl Pts',(-10.3503844980001,11.6,4.13941620499998));
#253335=CARTESIAN_POINT('Ctrl Pts',(-10.3537060160001,15.2,4.13940388499999));
#253336=CARTESIAN_POINT('Ctrl Pts',(-10.3537060160001,11.6,4.13940388499999));
#253337=CARTESIAN_POINT('Ctrl Pts',(-10.3570324910001,15.2,4.13938890199999));
#253338=CARTESIAN_POINT('Ctrl Pts',(-10.3570324910001,11.6,4.13938890199999));
#253339=CARTESIAN_POINT('Ctrl Pts',(-10.3603639140001,15.2,4.13937124899999));
#253340=CARTESIAN_POINT('Ctrl Pts',(-10.3603639140001,11.6,4.13937124899998));
#253341=CARTESIAN_POINT('Ctrl Pts',(-10.3637002770001,15.2,4.13935092199999));
#253342=CARTESIAN_POINT('Ctrl Pts',(-10.3637002770001,11.6,4.13935092199999));
#253343=CARTESIAN_POINT('Ctrl Pts',(-10.3670415720001,15.2,4.13932791199999));
#253344=CARTESIAN_POINT('Ctrl Pts',(-10.3670415720001,11.6,4.13932791199999));
#253345=CARTESIAN_POINT('Ctrl Pts',(-10.3703877890001,15.2,4.13930221299999));
#253346=CARTESIAN_POINT('Ctrl Pts',(-10.3703877890001,11.6,4.13930221299999));
#253347=CARTESIAN_POINT('Ctrl Pts',(-10.3737389220001,15.2,4.13927381799999));
#253348=CARTESIAN_POINT('Ctrl Pts',(-10.3737389220001,11.6,4.13927381799999));
#253349=CARTESIAN_POINT('Ctrl Pts',(-10.3770949600001,15.2,4.13924272199999));
#253350=CARTESIAN_POINT('Ctrl Pts',(-10.3770949600001,11.6,4.13924272199999));
#253351=CARTESIAN_POINT('Ctrl Pts',(-10.3804558970001,15.2,4.13920891799999));
#253352=CARTESIAN_POINT('Ctrl Pts',(-10.3804558970001,11.6,4.13920891799999));
#253353=CARTESIAN_POINT('Ctrl Pts',(-10.3838217220001,15.2,4.13917239799999));
#253354=CARTESIAN_POINT('Ctrl Pts',(-10.3838217220001,11.6,4.13917239799999));
#253355=CARTESIAN_POINT('Ctrl Pts',(-10.3871924310001,15.2,4.13913315699999));
#253356=CARTESIAN_POINT('Ctrl Pts',(-10.3871924310001,11.6,4.13913315699998));
#253357=CARTESIAN_POINT('Ctrl Pts',(-10.3905680110001,15.2,4.13909118899999));
#253358=CARTESIAN_POINT('Ctrl Pts',(-10.3905680110001,11.6,4.13909118899999));
#253359=CARTESIAN_POINT('Ctrl Pts',(-10.3939484570001,15.2,4.13904648699998));
#253360=CARTESIAN_POINT('Ctrl Pts',(-10.3939484570001,11.6,4.13904648699998));
#253361=CARTESIAN_POINT('Ctrl Pts',(-10.3973337590001,15.2,4.13899904299999));
#253362=CARTESIAN_POINT('Ctrl Pts',(-10.3973337590001,11.6,4.13899904299999));
#253363=CARTESIAN_POINT('Ctrl Pts',(-10.4007239090001,15.2,4.13894885299998));
#253364=CARTESIAN_POINT('Ctrl Pts',(-10.4007239090001,11.6,4.13894885299998));
#253365=CARTESIAN_POINT('Ctrl Pts',(-10.4041188990001,15.2,4.13889590999998));
#253366=CARTESIAN_POINT('Ctrl Pts',(-10.4041188990001,11.6,4.13889590999998));
#253367=CARTESIAN_POINT('Ctrl Pts',(-10.4075187210001,15.2,4.13884020699999));
#253368=CARTESIAN_POINT('Ctrl Pts',(-10.4075187210001,11.6,4.13884020699999));
#253369=CARTESIAN_POINT('Ctrl Pts',(-10.4109233670001,15.2,4.13878173799999));
#253370=CARTESIAN_POINT('Ctrl Pts',(-10.4109233670001,11.6,4.13878173799999));
#253371=CARTESIAN_POINT('Ctrl Pts',(-10.4143328290001,15.2,4.13872049599998));
#253372=CARTESIAN_POINT('Ctrl Pts',(-10.4143328290001,11.6,4.13872049599998));
#253373=CARTESIAN_POINT('Ctrl Pts',(-10.4177470960001,15.2,4.13865647699998));
#253374=CARTESIAN_POINT('Ctrl Pts',(-10.4177470960001,11.6,4.13865647699998));
#253375=CARTESIAN_POINT('Ctrl Pts',(-10.4211661640001,15.2,4.13858967199998));
#253376=CARTESIAN_POINT('Ctrl Pts',(-10.4211661640001,11.6,4.13858967199998));
#253377=CARTESIAN_POINT('Ctrl Pts',(-10.4245900210001,15.2,4.13852007699998));
#253378=CARTESIAN_POINT('Ctrl Pts',(-10.4245900210001,11.6,4.13852007699998));
#253379=CARTESIAN_POINT('Ctrl Pts',(-10.4280186620001,15.2,4.13844768399999));
#253380=CARTESIAN_POINT('Ctrl Pts',(-10.4280186620001,11.6,4.13844768399999));
#253381=CARTESIAN_POINT('Ctrl Pts',(-10.4314520770001,15.2,4.13837248799998));
#253382=CARTESIAN_POINT('Ctrl Pts',(-10.4314520770001,11.6,4.13837248799998));
#253383=CARTESIAN_POINT('Ctrl Pts',(-10.4348902580001,15.2,4.13829448199999));
#253384=CARTESIAN_POINT('Ctrl Pts',(-10.4348902580001,11.6,4.13829448199999));
#253385=CARTESIAN_POINT('Ctrl Pts',(-10.4383331970001,15.2,4.13821365999999));
#253386=CARTESIAN_POINT('Ctrl Pts',(-10.4383331970001,11.6,4.13821365999999));
#253387=CARTESIAN_POINT('Ctrl Pts',(-10.4417808860001,15.2,4.13813001599999));
#253388=CARTESIAN_POINT('Ctrl Pts',(-10.4417808860001,11.6,4.13813001599998));
#253389=CARTESIAN_POINT('Ctrl Pts',(-10.4452333170001,15.2,4.13804354299998));
#253390=CARTESIAN_POINT('Ctrl Pts',(-10.4452333170001,11.6,4.13804354299998));
#253391=CARTESIAN_POINT('Ctrl Pts',(-10.4486904820001,15.2,4.13795423799999));
#253392=CARTESIAN_POINT('Ctrl Pts',(-10.4486904820001,11.6,4.13795423799998));
#253393=CARTESIAN_POINT('Ctrl Pts',(-10.4521523720001,15.2,4.13786209099998));
#253394=CARTESIAN_POINT('Ctrl Pts',(-10.4521523720001,11.6,4.13786209099998));
#253395=CARTESIAN_POINT('Ctrl Pts',(-10.4556189810001,15.2,4.13776709799999));
#253396=CARTESIAN_POINT('Ctrl Pts',(-10.4556189810001,11.6,4.13776709799999));
#253397=CARTESIAN_POINT('Ctrl Pts',(-10.4590902980001,15.2,4.13766925199998));
#253398=CARTESIAN_POINT('Ctrl Pts',(-10.4590902980001,11.6,4.13766925199998));
#253399=CARTESIAN_POINT('Ctrl Pts',(-10.4625663170001,15.2,4.13756854899999));
#253400=CARTESIAN_POINT('Ctrl Pts',(-10.4625663170001,11.6,4.13756854899999));
#253401=CARTESIAN_POINT('Ctrl Pts',(-10.4660470290001,15.2,4.13746497899999));
#253402=CARTESIAN_POINT('Ctrl Pts',(-10.4660470290001,11.6,4.13746497899999));
#253403=CARTESIAN_POINT('Ctrl Pts',(-10.4695324260001,15.2,4.13735853999999));
#253404=CARTESIAN_POINT('Ctrl Pts',(-10.4695324260001,11.6,4.13735853999999));
#253405=CARTESIAN_POINT('Ctrl Pts',(-10.4730225010001,15.2,4.13724922399999));
#253406=CARTESIAN_POINT('Ctrl Pts',(-10.4730225010001,11.6,4.13724922399999));
#253407=CARTESIAN_POINT('Ctrl Pts',(-10.4765172450001,15.2,4.13713702599999));
#253408=CARTESIAN_POINT('Ctrl Pts',(-10.4765172450001,11.6,4.13713702599999));
#253409=CARTESIAN_POINT('Ctrl Pts',(-10.4800166500001,15.2,4.13702193899999));
#253410=CARTESIAN_POINT('Ctrl Pts',(-10.4800166500001,11.6,4.13702193899999));
#253411=CARTESIAN_POINT('Ctrl Pts',(-10.4835207080001,15.2,4.13690395699999));
#253412=CARTESIAN_POINT('Ctrl Pts',(-10.4835207080001,11.6,4.13690395699999));
#253413=CARTESIAN_POINT('Ctrl Pts',(-10.4870294120001,15.2,4.13678307599999));
#253414=CARTESIAN_POINT('Ctrl Pts',(-10.4870294120001,11.6,4.13678307599999));
#253415=CARTESIAN_POINT('Ctrl Pts',(-10.4905427520001,15.2,4.13665928699999));
#253416=CARTESIAN_POINT('Ctrl Pts',(-10.4905427520001,11.6,4.13665928699999));
#253417=CARTESIAN_POINT('Ctrl Pts',(-10.4940607220001,15.2,4.13653258699998));
#253418=CARTESIAN_POINT('Ctrl Pts',(-10.4940607220001,11.6,4.13653258699998));
#253419=CARTESIAN_POINT('Ctrl Pts',(-10.4975833130001,15.2,4.13640296899998));
#253420=CARTESIAN_POINT('Ctrl Pts',(-10.4975833130001,11.6,4.13640296899998));
#253421=CARTESIAN_POINT('Ctrl Pts',(-10.5011105170001,15.2,4.13627042599998));
#253422=CARTESIAN_POINT('Ctrl Pts',(-10.5011105170001,11.6,4.13627042599998));
#253423=CARTESIAN_POINT('Ctrl Pts',(-10.5046423270001,15.2,4.13613495399999));
#253424=CARTESIAN_POINT('Ctrl Pts',(-10.5046423270001,11.6,4.13613495399998));
#253425=CARTESIAN_POINT('Ctrl Pts',(-10.5081787340001,15.2,4.13599654699999));
#253426=CARTESIAN_POINT('Ctrl Pts',(-10.5081787340001,11.6,4.13599654699999));
#253427=CARTESIAN_POINT('Ctrl Pts',(-10.5117197300001,15.2,4.13585519699998));
#253428=CARTESIAN_POINT('Ctrl Pts',(-10.5117197300001,11.6,4.13585519699998));
#253429=CARTESIAN_POINT('Ctrl Pts',(-10.5152653080001,15.2,4.13571090099998));
#253430=CARTESIAN_POINT('Ctrl Pts',(-10.5152653080001,11.6,4.13571090099998));
#253431=CARTESIAN_POINT('Ctrl Pts',(-10.5188154600001,15.2,4.13556365299999));
#253432=CARTESIAN_POINT('Ctrl Pts',(-10.5188154600001,11.6,4.13556365299998));
#253433=CARTESIAN_POINT('Ctrl Pts',(-10.5223701770001,15.2,4.13541344499999));
#253434=CARTESIAN_POINT('Ctrl Pts',(-10.5223701770001,11.6,4.13541344499999));
#253435=CARTESIAN_POINT('Ctrl Pts',(-10.5259294520001,15.2,4.13526027299999));
#253436=CARTESIAN_POINT('Ctrl Pts',(-10.5259294520001,11.6,4.13526027299999));
#253437=CARTESIAN_POINT('Ctrl Pts',(-10.5294932760001,15.2,4.13510413099999));
#253438=CARTESIAN_POINT('Ctrl Pts',(-10.5294932760001,11.6,4.13510413099999));
#253439=CARTESIAN_POINT('Ctrl Pts',(-10.5330616440001,15.2,4.13494501199998));
#253440=CARTESIAN_POINT('Ctrl Pts',(-10.5330616440001,11.6,4.13494501199998));
#253441=CARTESIAN_POINT('Ctrl Pts',(-10.5366345450001,15.2,4.13478291199999));
#253442=CARTESIAN_POINT('Ctrl Pts',(-10.5366345450001,11.6,4.13478291199999));
#253443=CARTESIAN_POINT('Ctrl Pts',(-10.5402119720001,15.2,4.13461782599998));
#253444=CARTESIAN_POINT('Ctrl Pts',(-10.5402119720001,11.6,4.13461782599998));
#253445=CARTESIAN_POINT('Ctrl Pts',(-10.5437939180001,15.2,4.13444974599999));
#253446=CARTESIAN_POINT('Ctrl Pts',(-10.5437939180001,11.6,4.13444974599999));
#253447=CARTESIAN_POINT('Ctrl Pts',(-10.5473803750001,15.2,4.13427866799999));
#253448=CARTESIAN_POINT('Ctrl Pts',(-10.5473803750001,11.6,4.13427866799999));
#253449=CARTESIAN_POINT('Ctrl Pts',(-10.5509713340001,15.2,4.13410458499998));
#253450=CARTESIAN_POINT('Ctrl Pts',(-10.5509713340001,11.6,4.13410458499998));
#253451=CARTESIAN_POINT('Ctrl Pts',(-10.5545667880001,15.2,4.13392749399998));
#253452=CARTESIAN_POINT('Ctrl Pts',(-10.5545667880001,11.6,4.13392749399998));
#253453=CARTESIAN_POINT('Ctrl Pts',(-10.5581667290001,15.2,4.13374738699999));
#253454=CARTESIAN_POINT('Ctrl Pts',(-10.5581667290001,11.6,4.13374738699999));
#253455=CARTESIAN_POINT('Ctrl Pts',(-10.5617711500001,15.2,4.13356425799999));
#253456=CARTESIAN_POINT('Ctrl Pts',(-10.5617711500001,11.6,4.13356425799999));
#253457=CARTESIAN_POINT('Ctrl Pts',(-10.5653800430001,15.2,4.13337810299998));
#253458=CARTESIAN_POINT('Ctrl Pts',(-10.5653800430001,11.6,4.13337810299998));
#253459=CARTESIAN_POINT('Ctrl Pts',(-10.5689933990001,15.2,4.13318891799998));
#253460=CARTESIAN_POINT('Ctrl Pts',(-10.5689933990001,11.6,4.13318891799998));
#253461=CARTESIAN_POINT('Ctrl Pts',(-10.5726112110001,15.2,4.13299669399999));
#253462=CARTESIAN_POINT('Ctrl Pts',(-10.5726112110001,11.6,4.13299669399999));
#253463=CARTESIAN_POINT('Ctrl Pts',(-10.5762334720001,15.2,4.13280142599999));
#253464=CARTESIAN_POINT('Ctrl Pts',(-10.5762334720001,11.6,4.13280142599999));
#253465=CARTESIAN_POINT('Ctrl Pts',(-10.5798601730001,15.2,4.13260311199998));
#253466=CARTESIAN_POINT('Ctrl Pts',(-10.5798601730001,11.6,4.13260311199998));
#253467=CARTESIAN_POINT('Ctrl Pts',(-10.5834913070001,15.2,4.13240174199998));
#253468=CARTESIAN_POINT('Ctrl Pts',(-10.5834913070001,11.6,4.13240174199998));
#253469=CARTESIAN_POINT('Ctrl Pts',(-10.5871268660001,15.2,4.13219731299999));
#253470=CARTESIAN_POINT('Ctrl Pts',(-10.5871268660001,11.6,4.13219731299998));
#253471=CARTESIAN_POINT('Ctrl Pts',(-10.5907668410001,15.2,4.13198981899999));
#253472=CARTESIAN_POINT('Ctrl Pts',(-10.5907668410001,11.6,4.13198981899999));
#253473=CARTESIAN_POINT('Ctrl Pts',(-10.5944112280001,15.2,4.13177925499999));
#253474=CARTESIAN_POINT('Ctrl Pts',(-10.5944112280001,11.6,4.13177925499998));
#253475=CARTESIAN_POINT('Ctrl Pts',(-10.5980600150001,15.2,4.13156561499999));
#253476=CARTESIAN_POINT('Ctrl Pts',(-10.5980600150001,11.6,4.13156561499999));
#253477=CARTESIAN_POINT('Ctrl Pts',(-10.6017131970001,15.2,4.13134889499998));
#253478=CARTESIAN_POINT('Ctrl Pts',(-10.6017131970001,11.6,4.13134889499998));
#253479=CARTESIAN_POINT('Ctrl Pts',(-10.6053707650001,15.2,4.13112908799998));
#253480=CARTESIAN_POINT('Ctrl Pts',(-10.6053707650001,11.6,4.13112908799998));
#253481=CARTESIAN_POINT('Ctrl Pts',(-10.6090327130001,15.2,4.13090618899999));
#253482=CARTESIAN_POINT('Ctrl Pts',(-10.6090327130001,11.6,4.13090618899999));
#253483=CARTESIAN_POINT('Ctrl Pts',(-10.6126990310001,15.2,4.13068019299998));
#253484=CARTESIAN_POINT('Ctrl Pts',(-10.6126990310001,11.6,4.13068019299998));
#253485=CARTESIAN_POINT('Ctrl Pts',(-10.6163697120001,15.2,4.13045109399999));
#253486=CARTESIAN_POINT('Ctrl Pts',(-10.6163697120001,11.6,4.13045109399999));
#253487=CARTESIAN_POINT('Ctrl Pts',(-10.6200447500001,15.2,4.13021888799998));
#253488=CARTESIAN_POINT('Ctrl Pts',(-10.6200447500001,11.6,4.13021888799998));
#253489=CARTESIAN_POINT('Ctrl Pts',(-10.6237241360001,15.2,4.12998356799999));
#253490=CARTESIAN_POINT('Ctrl Pts',(-10.6237241360001,11.6,4.12998356799999));
#253491=CARTESIAN_POINT('Ctrl Pts',(-10.6274078610001,15.2,4.12974512999998));
#253492=CARTESIAN_POINT('Ctrl Pts',(-10.6274078610001,11.6,4.12974512999998));
#253493=CARTESIAN_POINT('Ctrl Pts',(-10.6310959200001,15.2,4.12950356799998));
#253494=CARTESIAN_POINT('Ctrl Pts',(-10.6310959200001,11.6,4.12950356799998));
#253495=CARTESIAN_POINT('Ctrl Pts',(-10.6347883040001,15.2,4.12925887599998));
#253496=CARTESIAN_POINT('Ctrl Pts',(-10.6347883040001,11.6,4.12925887599998));
#253497=CARTESIAN_POINT('Ctrl Pts',(-10.6384850050001,15.2,4.12901105099999));
#253498=CARTESIAN_POINT('Ctrl Pts',(-10.6384850050001,11.6,4.12901105099999));
#253499=CARTESIAN_POINT('Ctrl Pts',(-10.6421860180001,15.2,4.12876008799999));
#253500=CARTESIAN_POINT('Ctrl Pts',(-10.6421860180001,11.6,4.12876008799999));
#253501=CARTESIAN_POINT('Ctrl Pts',(-10.6458913320001,15.2,4.12850597899999));
#253502=CARTESIAN_POINT('Ctrl Pts',(-10.6458913320001,11.6,4.12850597899998));
#253503=CARTESIAN_POINT('Ctrl Pts',(-10.6496009430001,15.2,4.12824872099999));
#253504=CARTESIAN_POINT('Ctrl Pts',(-10.6496009430001,11.6,4.12824872099998));
#253505=CARTESIAN_POINT('Ctrl Pts',(-10.6533148400001,15.2,4.12798830699998));
#253506=CARTESIAN_POINT('Ctrl Pts',(-10.6533148400001,11.6,4.12798830699998));
#253507=CARTESIAN_POINT('Ctrl Pts',(-10.6570330180001,15.2,4.12772473399999));
#253508=CARTESIAN_POINT('Ctrl Pts',(-10.6570330180001,11.6,4.12772473399999));
#253509=CARTESIAN_POINT('Ctrl Pts',(-10.6607554670001,15.2,4.12745799499999));
#253510=CARTESIAN_POINT('Ctrl Pts',(-10.6607554670001,11.6,4.12745799499999));
#253511=CARTESIAN_POINT('Ctrl Pts',(-10.6644821790001,15.2,4.12718808499999));
#253512=CARTESIAN_POINT('Ctrl Pts',(-10.6644821790001,11.6,4.12718808499999));
#253513=CARTESIAN_POINT('Ctrl Pts',(-10.6682131480001,15.2,4.12691499899999));
#253514=CARTESIAN_POINT('Ctrl Pts',(-10.6682131480001,11.6,4.12691499899999));
#253515=CARTESIAN_POINT('Ctrl Pts',(-10.6719483670001,15.2,4.12663873099999));
#253516=CARTESIAN_POINT('Ctrl Pts',(-10.6719483670001,11.6,4.12663873099999));
#253517=CARTESIAN_POINT('Ctrl Pts',(-10.6756878260001,15.2,4.12635927799998));
#253518=CARTESIAN_POINT('Ctrl Pts',(-10.6756878260001,11.6,4.12635927799998));
#253519=CARTESIAN_POINT('Ctrl Pts',(-10.6794315200001,15.2,4.12607663399999));
#253520=CARTESIAN_POINT('Ctrl Pts',(-10.6794315200001,11.6,4.12607663399999));
#253521=CARTESIAN_POINT('Ctrl Pts',(-10.6831794430001,15.2,4.12579079399999));
#253522=CARTESIAN_POINT('Ctrl Pts',(-10.6831794430001,11.6,4.12579079399999));
#253523=CARTESIAN_POINT('Ctrl Pts',(-10.6869315860001,15.2,4.12550175599999));
#253524=CARTESIAN_POINT('Ctrl Pts',(-10.6869315860001,11.6,4.12550175599998));
#253525=CARTESIAN_POINT('Ctrl Pts',(-10.6906879440001,15.2,4.12520951199999));
#253526=CARTESIAN_POINT('Ctrl Pts',(-10.6906879440001,11.6,4.12520951199998));
#253527=CARTESIAN_POINT('Ctrl Pts',(-10.6944485080001,15.2,4.12491405999998));
#253528=CARTESIAN_POINT('Ctrl Pts',(-10.6944485080001,11.6,4.12491405999998));
#253529=CARTESIAN_POINT('Ctrl Pts',(-10.6982132700001,15.2,4.12461538999998));
#253530=CARTESIAN_POINT('Ctrl Pts',(-10.6982132700001,11.6,4.12461538999998));
#253531=CARTESIAN_POINT('Ctrl Pts',(-10.7019822200001,15.2,4.12431349999999));
#253532=CARTESIAN_POINT('Ctrl Pts',(-10.7019822200001,11.6,4.12431349999998));
#253533=CARTESIAN_POINT('Ctrl Pts',(-10.7057553490001,15.2,4.12400838099998));
#253534=CARTESIAN_POINT('Ctrl Pts',(-10.7057553490001,11.6,4.12400838099998));
#253535=CARTESIAN_POINT('Ctrl Pts',(-10.7095326480001,15.2,4.12370002799998));
#253536=CARTESIAN_POINT('Ctrl Pts',(-10.7095326480001,11.6,4.12370002799998));
#253537=CARTESIAN_POINT('Ctrl Pts',(-10.7133141100001,15.2,4.12338843599999));
#253538=CARTESIAN_POINT('Ctrl Pts',(-10.7133141100001,11.6,4.12338843599999));
#253539=CARTESIAN_POINT('Ctrl Pts',(-10.7170997260001,15.2,4.12307359999998));
#253540=CARTESIAN_POINT('Ctrl Pts',(-10.7170997260001,11.6,4.12307359999998));
#253541=CARTESIAN_POINT('Ctrl Pts',(-10.7208894930001,15.2,4.12275551699998));
#253542=CARTESIAN_POINT('Ctrl Pts',(-10.7208894930001,11.6,4.12275551699998));
#253543=CARTESIAN_POINT('Ctrl Pts',(-10.7246834070001,15.2,4.12243418399999));
#253544=CARTESIAN_POINT('Ctrl Pts',(-10.7246834070001,11.6,4.12243418399999));
#253545=CARTESIAN_POINT('Ctrl Pts',(-10.7284814650001,15.2,4.12210960099999));
#253546=CARTESIAN_POINT('Ctrl Pts',(-10.7284814650001,11.6,4.12210960099998));
#253547=CARTESIAN_POINT('Ctrl Pts',(-10.7315232270001,15.2,4.12184733399998));
#253548=CARTESIAN_POINT('Ctrl Pts',(-10.7315232270001,11.6,4.12184733399998));
#253549=CARTESIAN_POINT('Ctrl Pts',(-10.7338064110001,15.2,4.12164916999998));
#253550=CARTESIAN_POINT('Ctrl Pts',(-10.7338064110001,11.6,4.12164916999998));
#253551=CARTESIAN_POINT('Ctrl Pts',(-10.7353293650001,15.2,4.12151641099998));
#253552=CARTESIAN_POINT('Ctrl Pts',(-10.7353293650001,11.6,4.12151641099998));
#253553=CARTESIAN_POINT('Ctrl Pts',(-10.7360910480001,15.2,4.12144986899998));
#253554=CARTESIAN_POINT('Ctrl Pts',(-10.7360910480001,11.6,4.12144986899998));
#253555=CARTESIAN_POINT('Ctrl Pts',(-9.55499537100006,15.2,4.04260911699998));
#253556=CARTESIAN_POINT('Ctrl Pts',(-9.55669455126496,15.2,4.04316130806102));
#253557=CARTESIAN_POINT('Ctrl Pts',(-9.55844976571224,15.2,4.0437260538932));
#253558=CARTESIAN_POINT('Ctrl Pts',(-9.56026027810168,15.2,4.04430244593684));
#253559=CARTESIAN_POINT('Ctrl Pts',(-9.56207952169703,15.2,4.04488161763427));
#253560=CARTESIAN_POINT('Ctrl Pts',(-9.563954601157,15.2,4.04547254503639));
#253561=CARTESIAN_POINT('Ctrl Pts',(-9.56588480694515,15.2,4.04607433301654));
#253562=CARTESIAN_POINT('Ctrl Pts',(-9.56781501255799,15.2,4.04667612094203));
#253563=CARTESIAN_POINT('Ctrl Pts',(-9.56980034124075,15.2,4.0472887691226));
#253564=CARTESIAN_POINT('Ctrl Pts',(-9.57184010199996,15.2,4.04791140626664));
#253565=CARTESIAN_POINT('Ctrl Pts',(-9.57387986275917,15.2,4.04853404341067));
#253566=CARTESIAN_POINT('Ctrl Pts',(-9.57597405465781,15.2,4.04916667292137));
#253567=CARTESIAN_POINT('Ctrl Pts',(-9.57812199976731,15.2,4.04980844817958));
#253568=CARTESIAN_POINT('Ctrl Pts',(-9.5802699450719,15.2,4.05045022349609));
#253569=CARTESIAN_POINT('Ctrl Pts',(-9.58247164646091,15.2,4.05110114611867));
#253570=CARTESIAN_POINT('Ctrl Pts',(-9.58472644050408,15.2,4.05176039932183));
#253571=CARTESIAN_POINT('Ctrl Pts',(-9.58698123434243,15.2,4.05241965246511));
#253572=CARTESIAN_POINT('Ctrl Pts',(-9.58928912240927,15.2,4.05308723561338));
#253573=CARTESIAN_POINT('Ctrl Pts',(-9.59164945950104,15.2,4.05376235400861));
#253574=CARTESIAN_POINT('Ctrl Pts',(-9.59400979659281,15.2,4.05443747240384));
#253575=CARTESIAN_POINT('Ctrl Pts',(-9.59642258392434,15.2,4.05512012772112));
#253576=CARTESIAN_POINT('Ctrl Pts',(-9.59888719166586,15.2,4.05580954919576));
#253577=CARTESIAN_POINT('Ctrl Pts',(-9.60135179963124,15.2,4.05649897073303));
#253578=CARTESIAN_POINT('Ctrl Pts',(-9.60386822553645,15.2,4.05719515850451));
#253579=CARTESIAN_POINT('Ctrl Pts',(-9.60643585601319,15.2,4.05789736304319));
#253580=CARTESIAN_POINT('Ctrl Pts',(-9.60900348625671,15.2,4.05859956751807));
#253581=CARTESIAN_POINT('Ctrl Pts',(-9.61162232335711,15.2,4.05930778842291));
#253582=CARTESIAN_POINT('Ctrl Pts',(-9.614291761429,15.2,4.06002130098055));
#253583=CARTESIAN_POINT('Ctrl Pts',(-9.61696119950089,15.2,4.06073481353819));
#253584=CARTESIAN_POINT('Ctrl Pts',(-9.61968124038537,15.2,4.06145361467872));
#253585=CARTESIAN_POINT('Ctrl Pts',(-9.62245129461588,15.2,4.06217699940224));
#253586=CARTESIAN_POINT('Ctrl Pts',(-9.62522134884639,15.2,4.06290038412575));
#253587=CARTESIAN_POINT('Ctrl Pts',(-9.62804141584483,15.2,4.06362835228872));
#253588=CARTESIAN_POINT('Ctrl Pts',(-9.63091092190387,15.2,4.06436021417854));
#253589=CARTESIAN_POINT('Ctrl Pts',(-9.63378042822357,15.2,4.06509207613484));
#253590=CARTESIAN_POINT('Ctrl Pts',(-9.63669937019805,15.2,4.06582783428319));
#253591=CARTESIAN_POINT('Ctrl Pts',(-9.63966718486192,15.2,4.0665668163236));
#253592=CARTESIAN_POINT('Ctrl Pts',(-9.64263499925622,15.2,4.06730579829689));
#253593=CARTESIAN_POINT('Ctrl Pts',(-9.64565168602948,15.2,4.06804800619833));
#253594=CARTESIAN_POINT('Ctrl Pts',(-9.64871669226525,15.2,4.06879278825798));
#253595=CARTESIAN_POINT('Ctrl Pts',(-9.65178169850103,15.2,4.06953757031763));
#253596=CARTESIAN_POINT('Ctrl Pts',(-9.65489502331519,15.2,4.07028492457067));
#253597=CARTESIAN_POINT('Ctrl Pts',(-9.65805612461376,15.2,4.07103421945998));
#253598=CARTESIAN_POINT('Ctrl Pts',(-9.66121722619947,15.2,4.07178351441735));
#253599=CARTESIAN_POINT('Ctrl Pts',(-9.6644261034481,15.2,4.0725347480666));
#253600=CARTESIAN_POINT('Ctrl Pts',(-9.66768222512764,15.2,4.07328730227434));
#253601=CARTESIAN_POINT('Ctrl Pts',(-9.6709383465114,15.2,4.07403985641372));
#253602=CARTESIAN_POINT('Ctrl Pts',(-9.67424171249674,15.2,4.0747937321403));
#253603=CARTESIAN_POINT('Ctrl Pts',(-9.67759179997346,15.2,4.07554832544964));
#253604=CARTESIAN_POINT('Ctrl Pts',(-9.68094188745019,15.2,4.07630291875899));
#253605=CARTESIAN_POINT('Ctrl Pts',(-9.6843386955196,15.2,4.07705823106177));
#253606=CARTESIAN_POINT('Ctrl Pts',(-9.68778171389136,15.2,4.07781367520097));
#253607=CARTESIAN_POINT('Ctrl Pts',(-9.69122473257588,15.2,4.0785691194088));
#253608=CARTESIAN_POINT('Ctrl Pts',(-9.69471395954516,15.2,4.07932469324418));
#253609=CARTESIAN_POINT('Ctrl Pts',(-9.69824889183372,15.2,4.08007982582303));
#253610=CARTESIAN_POINT('Ctrl Pts',(-9.70178382380118,15.2,4.08083495833329));
#253611=CARTESIAN_POINT('Ctrl Pts',(-9.70536446121434,15.2,4.08158965010223));
#253612=CARTESIAN_POINT('Ctrl Pts',(-9.70899030975022,15.2,4.08234334149171));
#253613=CARTESIAN_POINT('Ctrl Pts',(-9.7126161582861,15.2,4.08309703288118));
#253614=CARTESIAN_POINT('Ctrl Pts',(-9.71628721459259,15.2,4.083849723842));
#253615=CARTESIAN_POINT('Ctrl Pts',(-9.72000299814063,15.2,4.08460086943565));
#253616=CARTESIAN_POINT('Ctrl Pts',(-9.72433807917169,15.2,4.08547720600707));
#253617=CARTESIAN_POINT('Ctrl Pts',(-9.72873403127503,15.2,4.08635143902531));
#253618=CARTESIAN_POINT('Ctrl Pts',(-9.73319010048331,15.2,4.08722272398332));
#253619=CARTESIAN_POINT('Ctrl Pts',(-9.73764616969159,15.2,4.08809400894134));
#253620=CARTESIAN_POINT('Ctrl Pts',(-9.74216235387668,15.2,4.08896234888187));
#253621=CARTESIAN_POINT('Ctrl Pts',(-9.74673791088781,15.2,4.08982691981334));
#253622=CARTESIAN_POINT('Ctrl Pts',(-9.75000616584487,15.2,4.09044447046906));
#253623=CARTESIAN_POINT('Ctrl Pts',(-9.75330471231626,15.2,4.09106009923596));
#253624=CARTESIAN_POINT('Ctrl Pts',(-9.75663328315204,15.2,4.09167351555522));
#253625=CARTESIAN_POINT('Ctrl Pts',(-9.75996185398783,15.2,4.09228693187448));
#253626=CARTESIAN_POINT('Ctrl Pts',(-9.76332045076296,15.2,4.09289813404092));
#253627=CARTESIAN_POINT('Ctrl Pts',(-9.76670880895986,15.2,4.09350683709628));
#253628=CARTESIAN_POINT('Ctrl Pts',(-9.77009716678742,15.2,4.09411554008528));
#253629=CARTESIAN_POINT('Ctrl Pts',(-9.77351528492723,15.2,4.09472174240883));
#253630=CARTESIAN_POINT('Ctrl Pts',(-9.77696290600738,15.2,4.09532516616273));
#253631=CARTESIAN_POINT('Ctrl Pts',(-9.78041052746331,15.2,4.09592858998241));
#253632=CARTESIAN_POINT('Ctrl Pts',(-9.78388764933264,15.2,4.09652923191047));
#253633=CARTESIAN_POINT('Ctrl Pts',(-9.78739401752469,15.2,4.0971268184385));
#253634=CARTESIAN_POINT('Ctrl Pts',(-9.79090038571675,15.2,4.09772440496652));
#253635=CARTESIAN_POINT('Ctrl Pts',(-9.79443599718798,15.2,4.09831893500158));
#253636=CARTESIAN_POINT('Ctrl Pts',(-9.79800060208629,15.2,4.09891014065635));
#253637=CARTESIAN_POINT('Ctrl Pts',(-9.80156520698459,15.2,4.09950134631112));
#253638=CARTESIAN_POINT('Ctrl Pts',(-9.80515880119807,15.2,4.10008922425601));
#253639=CARTESIAN_POINT('Ctrl Pts',(-9.80878113702993,15.2,4.10067351168676));
#253640=CARTESIAN_POINT('Ctrl Pts',(-9.81240347286178,15.2,4.10125779911751));
#253641=CARTESIAN_POINT('Ctrl Pts',(-9.81605454863878,15.2,4.10183849410094));
#253642=CARTESIAN_POINT('Ctrl Pts',(-9.81973411794285,15.2,4.10241533896225));
#253643=CARTESIAN_POINT('Ctrl Pts',(-9.82341368724693,15.2,4.10299218382356));
#253644=CARTESIAN_POINT('Ctrl Pts',(-9.8271217512366,15.2,4.10356517540819));
#253645=CARTESIAN_POINT('Ctrl Pts',(-9.83085806298962,15.2,4.10413406117469));
#253646=CARTESIAN_POINT('Ctrl Pts',(-9.8360888995253,15.2,4.10493050126017));
#253647=CARTESIAN_POINT('Ctrl Pts',(-9.84137510306443,15.2,4.10571888958012));
#253648=CARTESIAN_POINT('Ctrl Pts',(-9.84671601098299,15.2,4.10649854132806));
#253649=CARTESIAN_POINT('Ctrl Pts',(-9.85053094515112,15.2,4.10705543542506));
#253650=CARTESIAN_POINT('Ctrl Pts',(-9.85437378940413,15.2,4.10760787110875));
#253651=CARTESIAN_POINT('Ctrl Pts',(-9.85824430793272,15.2,4.10815560683023));
#253652=CARTESIAN_POINT('Ctrl Pts',(-9.86288892999829,15.2,4.10881288967213));
#253653=CARTESIAN_POINT('Ctrl Pts',(-9.8675733997966,15.2,4.10946339959004));
#253654=CARTESIAN_POINT('Ctrl Pts',(-9.87229731270832,15.2,4.11010672473333));
#253655=CARTESIAN_POINT('Ctrl Pts',(-9.87702122562003,15.2,4.11075004987663));
#253656=CARTESIAN_POINT('Ctrl Pts',(-9.88178458059536,15.2,4.11138619022881));
#253657=CARTESIAN_POINT('Ctrl Pts',(-9.88658697766821,15.2,4.11201473845649));
#253658=CARTESIAN_POINT('Ctrl Pts',(-9.89058897537431,15.2,4.11253852866525));
#253659=CARTESIAN_POINT('Ctrl Pts',(-9.89461808639513,15.2,4.11305704756442));
#253660=CARTESIAN_POINT('Ctrl Pts',(-9.89867407930424,15.2,4.11357006592376));
#253661=CARTESIAN_POINT('Ctrl Pts',(-9.90273007221334,15.2,4.1140830842831));
#253662=CARTESIAN_POINT('Ctrl Pts',(-9.90681294836055,15.2,4.11459059953352));
#253663=CARTESIAN_POINT('Ctrl Pts',(-9.91092248099806,15.2,4.11509238724215));
#253664=CARTESIAN_POINT('Ctrl Pts',(-9.91503201363557,15.2,4.11559417495078));
#253665=CARTESIAN_POINT('Ctrl Pts',(-9.91916820151262,15.2,4.11609023490649));
#253666=CARTESIAN_POINT('Ctrl Pts',(-9.92333082171958,15.2,4.11658034497625));
#253667=CARTESIAN_POINT('Ctrl Pts',(-9.92666091806663,15.2,4.11697243305342));
#253668=CARTESIAN_POINT('Ctrl Pts',(-9.93000793111592,15.2,4.11736071351595));
#253669=CARTESIAN_POINT('Ctrl Pts',(-9.93337174574653,15.2,4.11774507255575));
#253670=CARTESIAN_POINT('Ctrl Pts',(-9.93673555991882,15.2,4.11812943154319));
#253671=CARTESIAN_POINT('Ctrl Pts',(-9.94011617757625,15.2,4.11850987124414));
#253672=CARTESIAN_POINT('Ctrl Pts',(-9.94351348346409,15.2,4.11888627943586));
#253673=CARTESIAN_POINT('Ctrl Pts',(-9.9469107898148,15.2,4.11926268767886));
#253674=CARTESIAN_POINT('Ctrl Pts',(-9.95032478566477,15.2,4.11963506655472));
#253675=CARTESIAN_POINT('Ctrl Pts',(-9.95375535929726,15.2,4.12000330479674));
#253676=CARTESIAN_POINT('Ctrl Pts',(-9.95718593246236,15.2,4.12037154298859));
#253677=CARTESIAN_POINT('Ctrl Pts',(-9.96063308162847,15.2,4.12073564105328));
#253678=CARTESIAN_POINT('Ctrl Pts',(-9.96409669823916,15.2,4.1210954919311));
#253679=CARTESIAN_POINT('Ctrl Pts',(-9.96756031532177,15.2,4.12145534285795));
#253680=CARTESIAN_POINT('Ctrl Pts',(-9.97104039718604,15.2,4.12181094732649));
#253681=CARTESIAN_POINT('Ctrl Pts',(-9.97453683554432,15.2,4.12216219701201));
#253682=CARTESIAN_POINT('Ctrl Pts',(-9.9780332734262,15.2,4.12251344664968));
#253683=CARTESIAN_POINT('Ctrl Pts',(-9.98154606561872,15.2,4.12286034408266));
#253684=CARTESIAN_POINT('Ctrl Pts',(-9.98507510543966,15.2,4.12320278294401));
#253685=CARTESIAN_POINT('Ctrl Pts',(-9.99125092572734,15.2,4.12380205100968));
#253686=CARTESIAN_POINT('Ctrl Pts',(-9.99747649767144,15.2,4.12438766347715));
#253687=CARTESIAN_POINT('Ctrl Pts',(-10.0037512432559,15.2,4.12495907280812));
#253688=CARTESIAN_POINT('Ctrl Pts',(-10.0073368123009,15.2,4.12528559243852));
#253689=CARTESIAN_POINT('Ctrl Pts',(-10.0109384379705,15.2,4.12560747483783));
#253690=CARTESIAN_POINT('Ctrl Pts',(-10.0145560123915,15.2,4.12592461657685));
#253691=CARTESIAN_POINT('Ctrl Pts',(-10.0181735863196,15.2,4.12624175827267));
#253692=CARTESIAN_POINT('Ctrl Pts',(-10.0218071094151,15.2,4.12655416133019));
#253693=CARTESIAN_POINT('Ctrl Pts',(-10.0254564747268,15.2,4.12686172624981));
#253694=CARTESIAN_POINT('Ctrl Pts',(-10.0318428646439,15.2,4.12739996491152));
#253695=CARTESIAN_POINT('Ctrl Pts',(-10.0382777734669,15.2,4.12792338551636));
#253696=CARTESIAN_POINT('Ctrl Pts',(-10.0447606348613,15.2,4.12843146127369));
#253697=CARTESIAN_POINT('Ctrl Pts',(-10.0484651267262,15.2,4.12872179024963));
#253698=CARTESIAN_POINT('Ctrl Pts',(-10.0521852758934,15.2,4.12900711006824));
#253699=CARTESIAN_POINT('Ctrl Pts',(-10.0559209791976,15.2,4.12928732321252));
#253700=CARTESIAN_POINT('Ctrl Pts',(-10.0605906087095,15.2,4.12963758967151));
#253701=CARTESIAN_POINT('Ctrl Pts',(-10.0652845397351,15.2,4.12997987894394));
#253702=CARTESIAN_POINT('Ctrl Pts',(-10.0700025726774,15.2,4.13031400521119));
#253703=CARTESIAN_POINT('Ctrl Pts',(-10.073776999237,15.2,4.13058130623956));
#253704=CARTESIAN_POINT('Ctrl Pts',(-10.0775668492473,15.2,4.1308433830573));
#253705=CARTESIAN_POINT('Ctrl Pts',(-10.0813720210112,15.2,4.13110014273761));
#253706=CARTESIAN_POINT('Ctrl Pts',(-10.0861284854569,15.2,4.13142109232051));
#253707=CARTESIAN_POINT('Ctrl Pts',(-10.0909088891353,15.2,4.13173373190362));
#253708=CARTESIAN_POINT('Ctrl Pts',(-10.095713033581,15.2,4.13203788398651));
#253709=CARTESIAN_POINT('Ctrl Pts',(-10.1024388353861,15.2,4.13246369687604));
#253710=CARTESIAN_POINT('Ctrl Pts',(-10.1092111673848,15.2,4.1328728723868));
#253711=CARTESIAN_POINT('Ctrl Pts',(-10.1160294893463,15.2,4.13326492573837));
#253712=CARTESIAN_POINT('Ctrl Pts',(-10.1218737659958,15.2,4.13360097150754));
#253713=CARTESIAN_POINT('Ctrl Pts',(-10.127751830557,15.2,4.13392443983384));
#253714=CARTESIAN_POINT('Ctrl Pts',(-10.1336633472973,15.2,4.13423503051688));
#253715=CARTESIAN_POINT('Ctrl Pts',(-10.1376043579206,15.2,4.13444209094403));
#253716=CARTESIAN_POINT('Ctrl Pts',(-10.1415602353375,15.2,4.13464342796343));
#253717=CARTESIAN_POINT('Ctrl Pts',(-10.1455308809322,15.2,4.13483895567994));
#253718=CARTESIAN_POINT('Ctrl Pts',(-10.1504941883314,15.2,4.13508336534555));
#253719=CARTESIAN_POINT('Ctrl Pts',(-10.1554805721959,15.2,4.13531869691245));
#253720=CARTESIAN_POINT('Ctrl Pts',(-10.1604898376809,15.2,4.1355447824685));
#253721=CARTESIAN_POINT('Ctrl Pts',(-10.1644972502872,15.2,4.13572565092319));
#253722=CARTESIAN_POINT('Ctrl Pts',(-10.1685193089231,15.2,4.1359006027105));
#253723=CARTESIAN_POINT('Ctrl Pts',(-10.1725559147551,15.2,4.13606955249709));
#253724=CARTESIAN_POINT('Ctrl Pts',(-10.1765925200372,15.2,4.13623850226067));
#253725=CARTESIAN_POINT('Ctrl Pts',(-10.1806436727997,15.2,4.13640145021156));
#253726=CARTESIAN_POINT('Ctrl Pts',(-10.1847092760769,15.2,4.13655831269936));
#253727=CARTESIAN_POINT('Ctrl Pts',(-10.1908076818238,15.2,4.13679360646312));
#253728=CARTESIAN_POINT('Ctrl Pts',(-10.1969386013006,15.2,4.13701521093252));
#253729=CARTESIAN_POINT('Ctrl Pts',(-10.203101708613,15.2,4.13722284278672));
#253730=CARTESIAN_POINT('Ctrl Pts',(-10.2072104462614,15.2,4.13736126400401));
#253731=CARTESIAN_POINT('Ctrl Pts',(-10.21133349069,15.2,4.13749347742454));
#253732=CARTESIAN_POINT('Ctrl Pts',(-10.2154707441286,15.2,4.13761940124799));
#253733=CARTESIAN_POINT('Ctrl Pts',(-10.2216766251321,15.2,4.1378082870089));
#253734=CARTESIAN_POINT('Ctrl Pts',(-10.2279144815312,15.2,4.1379830205514));
#253735=CARTESIAN_POINT('Ctrl Pts',(-10.2341839894584,15.2,4.13814333347581));
#253736=CARTESIAN_POINT('Ctrl Pts',(-10.2383636608404,15.2,4.1382502087442));
#253737=CARTESIAN_POINT('Ctrl Pts',(-10.2425574012693,15.2,4.13835067492662));
#253738=CARTESIAN_POINT('Ctrl Pts',(-10.2467651152221,15.2,4.13844465397495));
#253739=CARTESIAN_POINT('Ctrl Pts',(-10.2520247580932,15.2,4.13856212779495));
#253740=CARTESIAN_POINT('Ctrl Pts',(-10.2573062343166,15.2,4.13866946410557));
#253741=CARTESIAN_POINT('Ctrl Pts',(-10.2626093622333,15.2,4.13876651230001));
#253742=CARTESIAN_POINT('Ctrl Pts',(-10.2668518647979,15.2,4.1388441508598));
#253743=CARTESIAN_POINT('Ctrl Pts',(-10.2711082249529,15.2,4.13891520451883));
#253744=CARTESIAN_POINT('Ctrl Pts',(-10.2753783489648,15.2,4.13897959774387));
#253745=CARTESIAN_POINT('Ctrl Pts',(-10.280716003107,15.2,4.13906008926202));
#253746=CARTESIAN_POINT('Ctrl Pts',(-10.2860751643011,15.2,4.13913017339785));
#253747=CARTESIAN_POINT('Ctrl Pts',(-10.2914556507962,15.2,4.13918970318389));
#253748=CARTESIAN_POINT('Ctrl Pts',(-10.2989883328277,15.2,4.13927304489473));
#253749=CARTESIAN_POINT('Ctrl Pts',(-10.3065628132273,15.2,4.13933569791323));
#253750=CARTESIAN_POINT('Ctrl Pts',(-10.3141786015944,15.2,4.13937726828967));
#253751=CARTESIAN_POINT('Ctrl Pts',(-10.3185304808307,15.2,4.13940102279142));
#253752=CARTESIAN_POINT('Ctrl Pts',(-10.322895849013,15.2,4.13941789275098));
#253753=CARTESIAN_POINT('Ctrl Pts',(-10.3272746151938,15.2,4.13942780475142));
#253754=CARTESIAN_POINT('Ctrl Pts',(-10.331653380778,15.2,4.13943771675049));
#253755=CARTESIAN_POINT('Ctrl Pts',(-10.336045542401,15.2,4.13944067167726));
#253756=CARTESIAN_POINT('Ctrl Pts',(-10.3404510123733,15.2,4.13943659823361));
#253757=CARTESIAN_POINT('Ctrl Pts',(-10.3470592182321,15.2,4.13943048806731));
#253758=CARTESIAN_POINT('Ctrl Pts',(-10.3536973646947,15.2,4.1394085615407));
#253759=CARTESIAN_POINT('Ctrl Pts',(-10.3603651497268,15.2,4.13937058045421));
#253760=CARTESIAN_POINT('Ctrl Pts',(-10.36369904194,15.2,4.13935158991268));
#253761=CARTESIAN_POINT('Ctrl Pts',(-10.3670403442681,15.2,4.13932858651225));
#253762=CARTESIAN_POINT('Ctrl Pts',(-10.3703890186063,15.2,4.13930153901141));
#253763=CARTESIAN_POINT('Ctrl Pts',(-10.3737376929445,15.2,4.13927449151058));
#253764=CARTESIAN_POINT('Ctrl Pts',(-10.3770937391716,15.2,4.13924340156186));
#253765=CARTESIAN_POINT('Ctrl Pts',(-10.3804571194251,15.2,4.13920823902111));
#253766=CARTESIAN_POINT('Ctrl Pts',(-10.3838204996785,15.2,4.13917307648037));
#253767=CARTESIAN_POINT('Ctrl Pts',(-10.3871912152061,15.2,4.13913384111511));
#253768=CARTESIAN_POINT('Ctrl Pts',(-10.3905692274583,15.2,4.13909050549168));
#253769=CARTESIAN_POINT('Ctrl Pts',(-10.3939472397106,15.2,4.13904716986826));
#253770=CARTESIAN_POINT('Ctrl Pts',(-10.3973325494209,15.2,4.13899973183666));
#253771=CARTESIAN_POINT('Ctrl Pts',(-10.4007251186303,15.2,4.13894816475556));
#253772=CARTESIAN_POINT('Ctrl Pts',(-10.4063794008515,15.2,4.13886221961728));
#253773=CARTESIAN_POINT('Ctrl Pts',(-10.4120538514322,15.2,4.13876480144498));
#253774=CARTESIAN_POINT('Ctrl Pts',(-10.4177482961802,15.2,4.13865578054174));
#253775=CARTESIAN_POINT('Ctrl Pts',(-10.4223038522269,15.2,4.13856856381439));
#253776=CARTESIAN_POINT('Ctrl Pts',(-10.4268722058869,15.2,4.13847392088687));
#253777=CARTESIAN_POINT('Ctrl Pts',(-10.431453269249,15.2,4.13837178549165));
#253778=CARTESIAN_POINT('Ctrl Pts',(-10.4348890664585,15.2,4.13829518395218));
#253779=CARTESIAN_POINT('Ctrl Pts',(-10.4383320126671,15.2,4.13821436768797));
#253780=CARTESIAN_POINT('Ctrl Pts',(-10.4417820718757,15.2,4.13812930877402));
#253781=CARTESIAN_POINT('Ctrl Pts',(-10.4475321707656,15.2,4.13798754391229));
#253782=CARTESIAN_POINT('Ctrl Pts',(-10.4533020282315,15.2,4.13783399616208));
#253783=CARTESIAN_POINT('Ctrl Pts',(-10.4590914741471,15.2,4.13766853768077));
#253784=CARTESIAN_POINT('Ctrl Pts',(-10.463723030501,15.2,4.13753617090654));
#253785=CARTESIAN_POINT('Ctrl Pts',(-10.4683671232037,15.2,4.13739618014944));
#253786=CARTESIAN_POINT('Ctrl Pts',(-10.4730236678778,15.2,4.13724850349535));
#253787=CARTESIAN_POINT('Ctrl Pts',(-10.4788443491962,15.2,4.13706390766265));
#253788=CARTESIAN_POINT('Ctrl Pts',(-10.4846844851346,15.2,4.1368673007574));
#253789=CARTESIAN_POINT('Ctrl Pts',(-10.4905439090919,15.2,4.13665855923026));
#253790=CARTESIAN_POINT('Ctrl Pts',(-10.4940595633386,15.2,4.13653331431852));
#253791=CARTESIAN_POINT('Ctrl Pts',(-10.4975821614199,15.2,4.13640370167721));
#253792=CARTESIAN_POINT('Ctrl Pts',(-10.5011116678005,15.2,4.13626969375923));
#253793=CARTESIAN_POINT('Ctrl Pts',(-10.5058176767355,15.2,4.13609101651903));
#253794=CARTESIAN_POINT('Ctrl Pts',(-10.5105359658977,15.2,4.13590452642293));
#253795=CARTESIAN_POINT('Ctrl Pts',(-10.5152664518785,15.2,4.13571016296738));
#253796=CARTESIAN_POINT('Ctrl Pts',(-10.5188143160419,15.2,4.13556439038896));
#253797=CARTESIAN_POINT('Ctrl Pts',(-10.5223690404961,15.2,4.13541418802773));
#253798=CARTESIAN_POINT('Ctrl Pts',(-10.5259305892833,15.2,4.13525953049169));
#253799=CARTESIAN_POINT('Ctrl Pts',(-10.5294921380706,15.2,4.13510487295564));
#253800=CARTESIAN_POINT('Ctrl Pts',(-10.5330605128242,15.2,4.1349457590281));
#253801=CARTESIAN_POINT('Ctrl Pts',(-10.5366356761104,15.2,4.13478216549277));
#253802=CARTESIAN_POINT('Ctrl Pts',(-10.5425942818039,15.2,4.13450950959064));
#253803=CARTESIAN_POINT('Ctrl Pts',(-10.5485717479089,15.2,4.13422440600763));
#253804=CARTESIAN_POINT('Ctrl Pts',(-10.5545679093663,15.2,4.13392674003607));
#253805=CARTESIAN_POINT('Ctrl Pts',(-10.5605640708236,15.2,4.13362907406451));
#253806=CARTESIAN_POINT('Ctrl Pts',(-10.5665789301472,15.2,4.13331884351273));
#253807=CARTESIAN_POINT('Ctrl Pts',(-10.5726123232301,15.2,4.13299593302519));
#253808=CARTESIAN_POINT('Ctrl Pts',(-10.5774390379594,15.2,4.13273760462109));
#253809=CARTESIAN_POINT('Ctrl Pts',(-10.5822776152914,15.2,4.1324711626737));
#253810=CARTESIAN_POINT('Ctrl Pts',(-10.5871279708347,15.2,4.13219654671345));
#253811=CARTESIAN_POINT('Ctrl Pts',(-10.5919783257172,15.2,4.13192193079062));
#253812=CARTESIAN_POINT('Ctrl Pts',(-10.5968404610259,15.2,4.13163914193274));
#253813=CARTESIAN_POINT('Ctrl Pts',(-10.6017142931267,15.2,4.1313481232904));
#253814=CARTESIAN_POINT('Ctrl Pts',(-10.6053696673683,15.2,4.13112985929873));
#253815=CARTESIAN_POINT('Ctrl Pts',(-10.6090316220411,15.2,4.13090696522989));
#253816=CARTESIAN_POINT('Ctrl Pts',(-10.6127001210486,15.2,4.13067941731066));
#253817=CARTESIAN_POINT('Ctrl Pts',(-10.6163686200562,15.2,4.13045186939144));
#253818=CARTESIAN_POINT('Ctrl Pts',(-10.6200436651988,15.2,4.13021966794241));
#253819=CARTESIAN_POINT('Ctrl Pts',(-10.6237252199808,15.2,4.12998278853499));
#253820=CARTESIAN_POINT('Ctrl Pts',(-10.6274067754316,15.2,4.12974590908453));
#253821=CARTESIAN_POINT('Ctrl Pts',(-10.6310948415843,15.2,4.12950435154942));
#253822=CARTESIAN_POINT('Ctrl Pts',(-10.6347893840804,15.2,4.12925809267966));
#253823=CARTESIAN_POINT('Ctrl Pts',(-10.6384839259054,15.2,4.12901183385464));
#253824=CARTESIAN_POINT('Ctrl Pts',(-10.6421849448551,15.2,4.12876087559652));
#253825=CARTESIAN_POINT('Ctrl Pts',(-10.6458924065959,15.2,4.12850519168874));
#253826=CARTESIAN_POINT('Ctrl Pts',(-10.6508356886925,15.2,4.12816427982717));
#253827=CARTESIAN_POINT('Ctrl Pts',(-10.6557904256494,15.2,4.12781496884533));
#253828=CARTESIAN_POINT('Ctrl Pts',(-10.6607565320461,15.2,4.12745720230189));
#253829=CARTESIAN_POINT('Ctrl Pts',(-10.6644811120128,15.2,4.12718887738212));
#253830=CARTESIAN_POINT('Ctrl Pts',(-10.6682120879886,15.2,4.12691579564985));
#253831=CARTESIAN_POINT('Ctrl Pts',(-10.6719494262269,15.2,4.12663793478559));
#253832=CARTESIAN_POINT('Ctrl Pts',(-10.6756867651442,15.2,4.12636007387086));
#253833=CARTESIAN_POINT('Ctrl Pts',(-10.6794304658883,15.2,4.12607743384645));
#253834=CARTESIAN_POINT('Ctrl Pts',(-10.6831804988509,15.2,4.12578999438735));
#253835=CARTESIAN_POINT('Ctrl Pts',(-10.6881805416655,15.2,4.12540674186226));
#253836=CARTESIAN_POINT('Ctrl Pts',(-10.6931918433981,15.2,4.12501495888548));
#253837=CARTESIAN_POINT('Ctrl Pts',(-10.6982143165979,15.2,4.12461458497433));
#253838=CARTESIAN_POINT('Ctrl Pts',(-10.7019811716688,15.2,4.12431430452734));
#253839=CARTESIAN_POINT('Ctrl Pts',(-10.7057543081181,15.2,4.12400919123026));
#253840=CARTESIAN_POINT('Ctrl Pts',(-10.7095336880022,15.2,4.12369921830994));
#253841=CARTESIAN_POINT('Ctrl Pts',(-10.7145728616387,15.2,4.1232859210453));
#253842=CARTESIAN_POINT('Ctrl Pts',(-10.7196231286485,15.2,4.12286398219));
#253843=CARTESIAN_POINT('Ctrl Pts',(-10.7246844434413,15.2,4.12243337145863));
#253844=CARTESIAN_POINT('Ctrl Pts',(-10.7284804291911,15.2,4.12211041343944));
#253845=CARTESIAN_POINT('Ctrl Pts',(-10.7322826323082,15.2,4.12178257906042));
#253846=CARTESIAN_POINT('Ctrl Pts',(-10.7360910480001,15.2,4.12144986899998));
#253847=CARTESIAN_POINT('Ctrl Pts',(-9.55499537100006,12.2,4.04260911699998));
#253848=CARTESIAN_POINT('Ctrl Pts',(-9.55669455126496,12.2,4.04316130806102));
#253849=CARTESIAN_POINT('Ctrl Pts',(-9.55844976571224,12.2,4.0437260538932));
#253850=CARTESIAN_POINT('Ctrl Pts',(-9.56026027810168,12.2,4.04430244593684));
#253851=CARTESIAN_POINT('Ctrl Pts',(-9.56207952169703,12.2,4.04488161763427));
#253852=CARTESIAN_POINT('Ctrl Pts',(-9.563954601157,12.2,4.04547254503639));
#253853=CARTESIAN_POINT('Ctrl Pts',(-9.56588480694515,12.2,4.04607433301654));
#253854=CARTESIAN_POINT('Ctrl Pts',(-9.56781501255799,12.2,4.04667612094203));
#253855=CARTESIAN_POINT('Ctrl Pts',(-9.56980034124075,12.2,4.04728876912259));
#253856=CARTESIAN_POINT('Ctrl Pts',(-9.57184010199996,12.2,4.04791140626663));
#253857=CARTESIAN_POINT('Ctrl Pts',(-9.57387986275916,12.2,4.04853404341067));
#253858=CARTESIAN_POINT('Ctrl Pts',(-9.57597405465781,12.2,4.04916667292137));
#253859=CARTESIAN_POINT('Ctrl Pts',(-9.57812199976731,12.2,4.04980844817958));
#253860=CARTESIAN_POINT('Ctrl Pts',(-9.5802699450719,12.2,4.05045022349609));
#253861=CARTESIAN_POINT('Ctrl Pts',(-9.58247164646092,12.2,4.05110114611867));
#253862=CARTESIAN_POINT('Ctrl Pts',(-9.58472644050408,12.2,4.05176039932183));
#253863=CARTESIAN_POINT('Ctrl Pts',(-9.58698123434243,12.2,4.05241965246511));
#253864=CARTESIAN_POINT('Ctrl Pts',(-9.58928912240927,12.2,4.05308723561338));
#253865=CARTESIAN_POINT('Ctrl Pts',(-9.59164945950104,12.2,4.05376235400861));
#253866=CARTESIAN_POINT('Ctrl Pts',(-9.59400979659281,12.2,4.05443747240384));
#253867=CARTESIAN_POINT('Ctrl Pts',(-9.59642258392434,12.2,4.05512012772111));
#253868=CARTESIAN_POINT('Ctrl Pts',(-9.59888719166586,12.2,4.05580954919576));
#253869=CARTESIAN_POINT('Ctrl Pts',(-9.60135179963124,12.2,4.05649897073303));
#253870=CARTESIAN_POINT('Ctrl Pts',(-9.60386822553645,12.2,4.05719515850451));
#253871=CARTESIAN_POINT('Ctrl Pts',(-9.60643585601319,12.2,4.05789736304318));
#253872=CARTESIAN_POINT('Ctrl Pts',(-9.60900348625671,12.2,4.05859956751808));
#253873=CARTESIAN_POINT('Ctrl Pts',(-9.61162232335711,12.2,4.05930778842291));
#253874=CARTESIAN_POINT('Ctrl Pts',(-9.614291761429,12.2,4.06002130098055));
#253875=CARTESIAN_POINT('Ctrl Pts',(-9.61696119950089,12.2,4.06073481353819));
#253876=CARTESIAN_POINT('Ctrl Pts',(-9.61968124038537,12.2,4.06145361467873));
#253877=CARTESIAN_POINT('Ctrl Pts',(-9.62245129461588,12.2,4.06217699940224));
#253878=CARTESIAN_POINT('Ctrl Pts',(-9.62568302471922,12.2,4.06302094829014));
#253879=CARTESIAN_POINT('Ctrl Pts',(-9.6289828284303,12.2,4.06387113444311));
#253880=CARTESIAN_POINT('Ctrl Pts',(-9.63234979270746,12.2,4.06472646678995));
#253881=CARTESIAN_POINT('Ctrl Pts',(-9.63523576193808,12.2,4.06545960876348));
#253882=CARTESIAN_POINT('Ctrl Pts',(-9.63817107189807,12.2,4.06619653327835));
#253883=CARTESIAN_POINT('Ctrl Pts',(-9.64115516212088,12.2,4.06693657316799));
#253884=CARTESIAN_POINT('Ctrl Pts',(-9.64413925234367,12.2,4.06767661305763));
#253885=CARTESIAN_POINT('Ctrl Pts',(-9.64717212177936,12.2,4.0684197680043));
#253886=CARTESIAN_POINT('Ctrl Pts',(-9.65025321916415,12.2,4.06916539089371));
#253887=CARTESIAN_POINT('Ctrl Pts',(-9.65384783296631,12.2,4.07003528430984));
#253888=CARTESIAN_POINT('Ctrl Pts',(-9.65750809002614,12.2,4.07090853182331));
#253889=CARTESIAN_POINT('Ctrl Pts',(-9.66123313152617,12.2,4.07178413743409));
#253890=CARTESIAN_POINT('Ctrl Pts',(-9.66442602436478,12.2,4.07253465655826));
#253891=CARTESIAN_POINT('Ctrl Pts',(-9.66766651597591,12.2,4.07328690653263));
#253892=CARTESIAN_POINT('Ctrl Pts',(-9.67095407582499,12.2,4.07404027482377));
#253893=CARTESIAN_POINT('Ctrl Pts',(-9.67424163537545,12.2,4.07479364304648));
#253894=CARTESIAN_POINT('Ctrl Pts',(-9.67757626506359,12.2,4.07554813017687));
#253895=CARTESIAN_POINT('Ctrl Pts',(-9.68095744269278,12.2,4.07630313756613));
#253896=CARTESIAN_POINT('Ctrl Pts',(-9.68433862032196,12.2,4.07705814495539));
#253897=CARTESIAN_POINT('Ctrl Pts',(-9.68776634813906,12.2,4.07781367415292));
#253898=CARTESIAN_POINT('Ctrl Pts',(-9.69124011651085,12.2,4.07856914145881));
#253899=CARTESIAN_POINT('Ctrl Pts',(-9.69471388488263,12.2,4.0793246087647));
#253900=CARTESIAN_POINT('Ctrl Pts',(-9.69823369312732,12.2,4.08008001414509));
#253901=CARTESIAN_POINT('Ctrl Pts',(-9.70179904066136,12.2,4.08083479145105));
#253902=CARTESIAN_POINT('Ctrl Pts',(-9.70536438851924,12.2,4.08158956882556));
#253903=CARTESIAN_POINT('Ctrl Pts',(-9.70897527616608,12.2,4.08234371540028));
#253904=CARTESIAN_POINT('Ctrl Pts',(-9.71263121019966,12.2,4.0830966797744));
#253905=CARTESIAN_POINT('Ctrl Pts',(-9.71628714390117,12.2,4.08384964408013));
#253906=CARTESIAN_POINT('Ctrl Pts',(-9.7199881264841,12.2,4.08460142377348));
#253907=CARTESIAN_POINT('Ctrl Pts',(-9.72373367119828,12.2,4.08535148024965));
#253908=CARTESIAN_POINT('Ctrl Pts',(-9.72747921591246,12.2,4.08610153672581));
#253909=CARTESIAN_POINT('Ctrl Pts',(-9.7312693250577,12.2,4.08684986869563));
#253910=CARTESIAN_POINT('Ctrl Pts',(-9.73510352258207,12.2,4.08759594916867));
#253911=CARTESIAN_POINT('Ctrl Pts',(-9.73957675325933,12.2,4.08846637643239));
#253912=CARTESIAN_POINT('Ctrl Pts',(-9.74410999118372,12.2,4.0893337384545));
#253913=CARTESIAN_POINT('Ctrl Pts',(-9.7487024962482,12.2,4.09019721724965));
#253914=CARTESIAN_POINT('Ctrl Pts',(-9.75198285695747,12.2,4.09081398780802));
#253915=CARTESIAN_POINT('Ctrl Pts',(-9.7552934555722,12.2,4.0914287778111));
#253916=CARTESIAN_POINT('Ctrl Pts',(-9.75863402626664,12.2,4.09204129753332));
#253917=CARTESIAN_POINT('Ctrl Pts',(-9.76197459696108,12.2,4.09265381725555));
#253918=CARTESIAN_POINT('Ctrl Pts',(-9.76534514075853,12.2,4.09326406450868));
#253919=CARTESIAN_POINT('Ctrl Pts',(-9.76874539251017,12.2,4.09387175673366));
#253920=CARTESIAN_POINT('Ctrl Pts',(-9.77214564426181,12.2,4.09447944895863));
#253921=CARTESIAN_POINT('Ctrl Pts',(-9.77557560612487,12.2,4.09508458471173));
#253922=CARTESIAN_POINT('Ctrl Pts',(-9.77903501779307,12.2,4.0956868845727));
#253923=CARTESIAN_POINT('Ctrl Pts',(-9.78318631164409,12.2,4.0964096443796));
#253924=CARTESIAN_POINT('Ctrl Pts',(-9.78738001350006,12.2,4.09712831947848));
#253925=CARTESIAN_POINT('Ctrl Pts',(-9.791615681261,12.2,4.09784243820272));
#253926=CARTESIAN_POINT('Ctrl Pts',(-9.79514540452336,12.2,4.09843753716122));
#253927=CARTESIAN_POINT('Ctrl Pts',(-9.79870427072626,12.2,4.09902947286921));
#253928=CARTESIAN_POINT('Ctrl Pts',(-9.80229202671468,12.2,4.09961797377467));
#253929=CARTESIAN_POINT('Ctrl Pts',(-9.80587978270311,12.2,4.10020647468013));
#253930=CARTESIAN_POINT('Ctrl Pts',(-9.80949643110553,12.2,4.10079154381111));
#253931=CARTESIAN_POINT('Ctrl Pts',(-9.81314171950832,12.2,4.10137291624166));
#253932=CARTESIAN_POINT('Ctrl Pts',(-9.81678700791111,12.2,4.10195428867222));
#253933=CARTESIAN_POINT('Ctrl Pts',(-9.82046093836287,12.2,4.1025319657866));
#253934=CARTESIAN_POINT('Ctrl Pts',(-9.82416326351867,12.2,4.10310568752531));
#253935=CARTESIAN_POINT('Ctrl Pts',(-9.82786558867447,12.2,4.10367940926402));
#253936=CARTESIAN_POINT('Ctrl Pts',(-9.83159630951673,12.2,4.1042491775094));
#253937=CARTESIAN_POINT('Ctrl Pts',(-9.83535518125433,12.2,4.10481473674529));
#253938=CARTESIAN_POINT('Ctrl Pts',(-9.83911405299192,12.2,4.10538029598118));
#253939=CARTESIAN_POINT('Ctrl Pts',(-9.84290107681485,12.2,4.10594164723106));
#253940=CARTESIAN_POINT('Ctrl Pts',(-9.84671601098299,12.2,4.10649854132806));
#253941=CARTESIAN_POINT('Ctrl Pts',(-9.85053094515113,12.2,4.10705543542506));
#253942=CARTESIAN_POINT('Ctrl Pts',(-9.85437378940413,12.2,4.10760787110875));
#253943=CARTESIAN_POINT('Ctrl Pts',(-9.85824430793272,12.2,4.10815560683023));
#253944=CARTESIAN_POINT('Ctrl Pts',(-9.86211482646132,12.2,4.10870334255171));
#253945=CARTESIAN_POINT('Ctrl Pts',(-9.86601301707236,12.2,4.10924637444301));
#253946=CARTESIAN_POINT('Ctrl Pts',(-9.86993864554681,12.2,4.10978446534538));
#253947=CARTESIAN_POINT('Ctrl Pts',(-9.87386427402126,12.2,4.11032255624775));
#253948=CARTESIAN_POINT('Ctrl Pts',(-9.87781733930727,12.2,4.11085570441391));
#253949=CARTESIAN_POINT('Ctrl Pts',(-9.88179761021228,12.2,4.11138367455239));
#253950=CARTESIAN_POINT('Ctrl Pts',(-9.8857778811173,12.2,4.11191164469086));
#253951=CARTESIAN_POINT('Ctrl Pts',(-9.88978535688662,12.2,4.11243443668478));
#253952=CARTESIAN_POINT('Ctrl Pts',(-9.8938198070277,12.2,4.11295181855934));
#253953=CARTESIAN_POINT('Ctrl Pts',(-9.89785425672904,12.2,4.11346920037751));
#253954=CARTESIAN_POINT('Ctrl Pts',(-9.90191568062972,12.2,4.11398117306071));
#253955=CARTESIAN_POINT('Ctrl Pts',(-9.90600385122359,12.2,4.1144875072421));
#253956=CARTESIAN_POINT('Ctrl Pts',(-9.91009202226308,12.2,4.11499384147868));
#253957=CARTESIAN_POINT('Ctrl Pts',(-9.91420694039377,12.2,4.11549453827923));
#253958=CARTESIAN_POINT('Ctrl Pts',(-9.9183483789333,12.2,4.11598937196027));
#253959=CARTESIAN_POINT('Ctrl Pts',(-9.92166152994549,12.2,4.11638523892668));
#253960=CARTESIAN_POINT('Ctrl Pts',(-9.92499165519351,12.2,4.11677735483291));
#253961=CARTESIAN_POINT('Ctrl Pts',(-9.92833863950227,12.2,4.11716560696693));
#253962=CARTESIAN_POINT('Ctrl Pts',(-9.93168562335501,12.2,4.11755385904805));
#253963=CARTESIAN_POINT('Ctrl Pts',(-9.93504946587814,12.2,4.11793824593794));
#253964=CARTESIAN_POINT('Ctrl Pts',(-9.93843005498894,12.2,4.1183186579628));
#253965=CARTESIAN_POINT('Ctrl Pts',(-9.94181064456033,12.2,4.11869907003949));
#253966=CARTESIAN_POINT('Ctrl Pts',(-9.94520797852505,12.2,4.11907550509082));
#253967=CARTESIAN_POINT('Ctrl Pts',(-9.94862194626665,12.2,4.11944785600001));
#253968=CARTESIAN_POINT('Ctrl Pts',(-9.95203591400825,12.2,4.11982020690919));
#253969=CARTESIAN_POINT('Ctrl Pts',(-9.95546651591849,12.2,4.12018847229845));
#253970=CARTESIAN_POINT('Ctrl Pts',(-9.95891363833028,12.2,4.12055254381786));
#253971=CARTESIAN_POINT('Ctrl Pts',(-9.96236076027238,12.2,4.12091661528767));
#253972=CARTESIAN_POINT('Ctrl Pts',(-9.96582440471358,12.2,4.1212764925022));
#253973=CARTESIAN_POINT('Ctrl Pts',(-9.96930445872263,12.2,4.12163206997476));
#253974=CARTESIAN_POINT('Ctrl Pts',(-9.97278451320583,12.2,4.12198764749577));
#253975=CARTESIAN_POINT('Ctrl Pts',(-9.97628097979512,12.2,4.12233892314937));
#253976=CARTESIAN_POINT('Ctrl Pts',(-9.97979374559934,12.2,4.12268579405672));
#253977=CARTESIAN_POINT('Ctrl Pts',(-9.98330651092493,12.2,4.1230326649168));
#253978=CARTESIAN_POINT('Ctrl Pts',(-9.98683557849843,12.2,4.12337512996355));
#253979=CARTESIAN_POINT('Ctrl Pts',(-9.99038083648532,12.2,4.123713084214));
#253980=CARTESIAN_POINT('Ctrl Pts',(-9.99392609495527,12.2,4.12405103851049));
#253981=CARTESIAN_POINT('Ctrl Pts',(-9.99748754557189,12.2,4.12438448274153));
#253982=CARTESIAN_POINT('Ctrl Pts',(-10.0010650795025,12.2,4.1247133149977));
#253983=CARTESIAN_POINT('Ctrl Pts',(-10.0046426129457,12.2,4.12504214720907));
#253984=CARTESIAN_POINT('Ctrl Pts',(-10.0082362295234,12.2,4.12536636738021));
#253985=CARTESIAN_POINT('Ctrl Pts',(-10.0118458226717,12.2,4.1256858729655));
#253986=CARTESIAN_POINT('Ctrl Pts',(-10.0154554163118,12.2,4.12600537859433));
#253987=CARTESIAN_POINT('Ctrl Pts',(-10.0190809846733,12.2,4.12632016930872));
#253988=CARTESIAN_POINT('Ctrl Pts',(-10.0227224230395,12.2,4.12663014699197));
#253989=CARTESIAN_POINT('Ctrl Pts',(-10.0263638609095,12.2,4.12694012463298));
#253990=CARTESIAN_POINT('Ctrl Pts',(-10.0300211666797,12.2,4.12724528935442));
#253991=CARTESIAN_POINT('Ctrl Pts',(-10.0336942374504,12.2,4.12754554045641));
#253992=CARTESIAN_POINT('Ctrl Pts',(-10.0373673087216,12.2,4.12784579159931));
#253993=CARTESIAN_POINT('Ctrl Pts',(-10.0410561424917,12.2,4.1281411322582));
#253994=CARTESIAN_POINT('Ctrl Pts',(-10.0447606348613,12.2,4.12843146127369));
#253995=CARTESIAN_POINT('Ctrl Pts',(-10.0484651267262,12.2,4.12872179024963));
#253996=CARTESIAN_POINT('Ctrl Pts',(-10.0521852758934,12.2,4.12900711006824));
#253997=CARTESIAN_POINT('Ctrl Pts',(-10.0559209791976,12.2,4.12928732321252));
#253998=CARTESIAN_POINT('Ctrl Pts',(-10.0596566830107,12.2,4.12956753639498));
#253999=CARTESIAN_POINT('Ctrl Pts',(-10.063407940344,12.2,4.12984264448427));
#254000=CARTESIAN_POINT('Ctrl Pts',(-10.0671746475109,12.2,4.13011255150019));
#254001=CARTESIAN_POINT('Ctrl Pts',(-10.0709413541646,12.2,4.13038245847933));
#254002=CARTESIAN_POINT('Ctrl Pts',(-10.074723511955,12.2,4.13064716511437));
#254003=CARTESIAN_POINT('Ctrl Pts',(-10.0785210159208,12.2,4.13090657748259));
#254004=CARTESIAN_POINT('Ctrl Pts',(-10.082318520404,12.2,4.13116598988616));
#254005=CARTESIAN_POINT('Ctrl Pts',(-10.0861313716025,12.2,4.13142010798645));
#254006=CARTESIAN_POINT('Ctrl Pts',(-10.0899594680333,12.2,4.131668839));
#254007=CARTESIAN_POINT('Ctrl Pts',(-10.0937875644642,12.2,4.13191757001356));
#254008=CARTESIAN_POINT('Ctrl Pts',(-10.0976309055024,12.2,4.13216091429871));
#254009=CARTESIAN_POINT('Ctrl Pts',(-10.1014893893809,12.2,4.13239878075556));
#254010=CARTESIAN_POINT('Ctrl Pts',(-10.1053478727336,12.2,4.13263664718));
#254011=CARTESIAN_POINT('Ctrl Pts',(-10.1092215005477,12.2,4.13286903568402));
#254012=CARTESIAN_POINT('Ctrl Pts',(-10.1131101692473,12.2,4.13309585599985));
#254013=CARTESIAN_POINT('Ctrl Pts',(-10.1179710055193,12.2,4.13337938141782));
#254014=CARTESIAN_POINT('Ctrl Pts',(-10.1228553458,12.2,4.13365420734445));
#254015=CARTESIAN_POINT('Ctrl Pts',(-10.1277629937167,12.2,4.13392015873334));
#254016=CARTESIAN_POINT('Ctrl Pts',(-10.131689112264,12.2,4.13413291985605));
#254017=CARTESIAN_POINT('Ctrl Pts',(-10.135630148663,12.2,4.13434000255865));
#254018=CARTESIAN_POINT('Ctrl Pts',(-10.1395860018801,12.2,4.13454131829125));
#254019=CARTESIAN_POINT('Ctrl Pts',(-10.1435418545583,12.2,4.13474263399643));
#254020=CARTESIAN_POINT('Ctrl Pts',(-10.1475125248495,12.2,4.13493818303673));
#254021=CARTESIAN_POINT('Ctrl Pts',(-10.151497914764,12.2,4.13512787946654));
#254022=CARTESIAN_POINT('Ctrl Pts',(-10.1554833052214,12.2,4.13531757592221));
#254023=CARTESIAN_POINT('Ctrl Pts',(-10.1594834128,12.2,4.13550141822278));
#254024=CARTESIAN_POINT('Ctrl Pts',(-10.1634981426314,12.2,4.13567932328743));
#254025=CARTESIAN_POINT('Ctrl Pts',(-10.1675128719158,12.2,4.13585722832783));
#254026=CARTESIAN_POINT('Ctrl Pts',(-10.1715422215122,12.2,4.13602919448845));
#254027=CARTESIAN_POINT('Ctrl Pts',(-10.1755860947362,12.2,4.13619513825305));
#254028=CARTESIAN_POINT('Ctrl Pts',(-10.1796299685112,12.2,4.13636108204027));
#254029=CARTESIAN_POINT('Ctrl Pts',(-10.1836883649963,12.2,4.13652100236288));
#254030=CARTESIAN_POINT('Ctrl Pts',(-10.1877611876081,12.2,4.13667481753753));
#254031=CARTESIAN_POINT('Ctrl Pts',(-10.191834009665,12.2,4.13682863269122));
#254032=CARTESIAN_POINT('Ctrl Pts',(-10.1959212582477,12.2,4.13697634268618));
#254033=CARTESIAN_POINT('Ctrl Pts',(-10.2000228376716,12.2,4.13711786373777));
#254034=CARTESIAN_POINT('Ctrl Pts',(-10.2041244176543,12.2,4.13725938480864));
#254035=CARTESIAN_POINT('Ctrl Pts',(-10.2082403270979,12.2,4.1373947164761));
#254036=CARTESIAN_POINT('Ctrl Pts',(-10.2123704703794,12.2,4.1375237802605));
#254037=CARTESIAN_POINT('Ctrl Pts',(-10.2165006130983,12.2,4.13765284402732));
#254038=CARTESIAN_POINT('Ctrl Pts',(-10.2206449894421,12.2,4.13777563780373));
#254039=CARTESIAN_POINT('Ctrl Pts',(-10.2248035060451,12.2,4.1378920817393));
#254040=CARTESIAN_POINT('Ctrl Pts',(-10.2289620232147,12.2,4.13800852569074));
#254041=CARTESIAN_POINT('Ctrl Pts',(-10.2331346783889,12.2,4.13811862086342));
#254042=CARTESIAN_POINT('Ctrl Pts',(-10.2373213789695,12.2,4.13822228725841));
#254043=CARTESIAN_POINT('Ctrl Pts',(-10.2415080789797,12.2,4.13832595363928));
#254044=CARTESIAN_POINT('Ctrl Pts',(-10.245708824143,12.2,4.13842319065304));
#254045=CARTESIAN_POINT('Ctrl Pts',(-10.2499235188526,12.2,4.13851392053517));
#254046=CARTESIAN_POINT('Ctrl Pts',(-10.2541382141364,12.2,4.13860465042967));
#254047=CARTESIAN_POINT('Ctrl Pts',(-10.2583668596688,12.2,4.13868887374023));
#254048=CARTESIAN_POINT('Ctrl Pts',(-10.2626093622333,12.2,4.13876651230001));
#254049=CARTESIAN_POINT('Ctrl Pts',(-10.2668518647979,12.2,4.1388441508598));
#254050=CARTESIAN_POINT('Ctrl Pts',(-10.2711082249529,12.2,4.13891520451882));
#254051=CARTESIAN_POINT('Ctrl Pts',(-10.2753783489648,12.2,4.13897959774387));
#254052=CARTESIAN_POINT('Ctrl Pts',(-10.2796484723949,12.2,4.13904399096014));
#254053=CARTESIAN_POINT('Ctrl Pts',(-10.2839323604123,12.2,4.13910172428722));
#254054=CARTESIAN_POINT('Ctrl Pts',(-10.2882299197471,12.2,4.13915272028331));
#254055=CARTESIAN_POINT('Ctrl Pts',(-10.2925274796674,12.2,4.13920371628634));
#254056=CARTESIAN_POINT('Ctrl Pts',(-10.2968387104395,12.2,4.1392479765159));
#254057=CARTESIAN_POINT('Ctrl Pts',(-10.3011635217321,12.2,4.13928542573946));
#254058=CARTESIAN_POINT('Ctrl Pts',(-10.3054883324355,12.2,4.13932287495793));
#254059=CARTESIAN_POINT('Ctrl Pts',(-10.309826722951,12.2,4.13935351379117));
#254060=CARTESIAN_POINT('Ctrl Pts',(-10.3141786015944,12.2,4.13937726828967));
#254061=CARTESIAN_POINT('Ctrl Pts',(-10.3185304808307,12.2,4.13940102279141));
#254062=CARTESIAN_POINT('Ctrl Pts',(-10.322895849013,12.2,4.13941789275098));
#254063=CARTESIAN_POINT('Ctrl Pts',(-10.3272746151938,12.2,4.13942780475142));
#254064=CARTESIAN_POINT('Ctrl Pts',(-10.331653380778,12.2,4.13943771675049));
#254065=CARTESIAN_POINT('Ctrl Pts',(-10.336045542401,12.2,4.13944067167726));
#254066=CARTESIAN_POINT('Ctrl Pts',(-10.3404510123733,12.2,4.13943659823361));
#254067=CARTESIAN_POINT('Ctrl Pts',(-10.3459578502889,12.2,4.13943150642863));
#254068=CARTESIAN_POINT('Ctrl Pts',(-10.3514854804939,12.2,4.1394154319567));
#254069=CARTESIAN_POINT('Ctrl Pts',(-10.3570337276456,12.2,4.13938823452673));
#254070=CARTESIAN_POINT('Ctrl Pts',(-10.3603626758157,12.2,4.13937191606934));
#254071=CARTESIAN_POINT('Ctrl Pts',(-10.3636990465084,12.2,4.13935159478789));
#254072=CARTESIAN_POINT('Ctrl Pts',(-10.3670428018865,12.2,4.13932723974635));
#254073=CARTESIAN_POINT('Ctrl Pts',(-10.3703865572645,12.2,4.13930288470483));
#254074=CARTESIAN_POINT('Ctrl Pts',(-10.3737376973076,12.2,4.13927449562202));
#254075=CARTESIAN_POINT('Ctrl Pts',(-10.3770961839762,12.2,4.13924204499875));
#254076=CARTESIAN_POINT('Ctrl Pts',(-10.3804546712549,12.2,4.13920959436959));
#254077=CARTESIAN_POINT('Ctrl Pts',(-10.3838205053108,12.2,4.13917308028095));
#254078=CARTESIAN_POINT('Ctrl Pts',(-10.387193649552,12.2,4.13913247523283));
#254079=CARTESIAN_POINT('Ctrl Pts',(-10.3905667931805,12.2,4.13909187019208));
#254080=CARTESIAN_POINT('Ctrl Pts',(-10.3939472461585,12.2,4.13904717392654));
#254081=CARTESIAN_POINT('Ctrl Pts',(-10.3973349713694,12.2,4.13899835646962));
#254082=CARTESIAN_POINT('Ctrl Pts',(-10.4018519381121,12.2,4.13893326653002));
#254083=CARTESIAN_POINT('Ctrl Pts',(-10.4063818328503,12.2,4.13886085272782));
#254084=CARTESIAN_POINT('Ctrl Pts',(-10.4109245703159,12.2,4.13878104478656));
#254085=CARTESIAN_POINT('Ctrl Pts',(-10.4143316235698,12.2,4.13872118882789));
#254086=CARTESIAN_POINT('Ctrl Pts',(-10.4177458988961,12.2,4.13865717497849));
#254087=CARTESIAN_POINT('Ctrl Pts',(-10.4211673605625,12.2,4.13858897448154));
#254088=CARTESIAN_POINT('Ctrl Pts',(-10.4245888228504,12.2,4.1385207739722));
#254089=CARTESIAN_POINT('Ctrl Pts',(-10.4280174714154,12.2,4.13844838704502));
#254090=CARTESIAN_POINT('Ctrl Pts',(-10.431453269249,12.2,4.13837178549164));
#254091=CARTESIAN_POINT('Ctrl Pts',(-10.4360343319869,12.2,4.13826965011034));
#254092=CARTESIAN_POINT('Ctrl Pts',(-10.440628104103,12.2,4.13816002099669));
#254093=CARTESIAN_POINT('Ctrl Pts',(-10.445234500115,12.2,4.13804283495119));
#254094=CARTESIAN_POINT('Ctrl Pts',(-10.4486892972809,12.2,4.13795494541308));
#254095=CARTESIAN_POINT('Ctrl Pts',(-10.4521511950325,12.2,4.13786280475278));
#254096=CARTESIAN_POINT('Ctrl Pts',(-10.4556201573706,12.2,4.13776638479363));
#254097=CARTESIAN_POINT('Ctrl Pts',(-10.4590891197087,12.2,4.13766996483448));
#254098=CARTESIAN_POINT('Ctrl Pts',(-10.4625651457516,12.2,4.13756926663517));
#254099=CARTESIAN_POINT('Ctrl Pts',(-10.466048199499,12.2,4.1374642617229));
#254100=CARTESIAN_POINT('Ctrl Pts',(-10.4695312538793,12.2,4.13735925679156));
#254101=CARTESIAN_POINT('Ctrl Pts',(-10.4730213366699,12.2,4.13724994679234));
#254102=CARTESIAN_POINT('Ctrl Pts',(-10.4765184110124,12.2,4.13713630373357));
#254103=CARTESIAN_POINT('Ctrl Pts',(-10.4800154847196,12.2,4.13702266069544));
#254104=CARTESIAN_POINT('Ctrl Pts',(-10.4835195502098,12.2,4.13690468453255));
#254105=CARTESIAN_POINT('Ctrl Pts',(-10.4870305714162,12.2,4.13678234903661));
#254106=CARTESIAN_POINT('Ctrl Pts',(-10.491711932812,12.2,4.13661923504944));
#254107=CARTESIAN_POINT('Ctrl Pts',(-10.4964056595068,12.2,4.13644837097509));
#254108=CARTESIAN_POINT('Ctrl Pts',(-10.5011116678005,12.2,4.13626969375923));
#254109=CARTESIAN_POINT('Ctrl Pts',(-10.5046411741811,12.2,4.13613568584125));
#254110=CARTESIAN_POINT('Ctrl Pts',(-10.5081775884739,12.2,4.13599728387535));
#254111=CARTESIAN_POINT('Ctrl Pts',(-10.5117208747192,12.2,4.13585446050615));
#254112=CARTESIAN_POINT('Ctrl Pts',(-10.5152641616082,12.2,4.13571163711099));
#254113=CARTESIAN_POINT('Ctrl Pts',(-10.5188143214076,12.2,4.1355643943896));
#254114=CARTESIAN_POINT('Ctrl Pts',(-10.5223713172588,12.2,4.13541270395028));
#254115=CARTESIAN_POINT('Ctrl Pts',(-10.5271139773168,12.2,4.13521045007712));
#254116=CARTESIAN_POINT('Ctrl Pts',(-10.5318687919454,12.2,4.13500029019664));
#254117=CARTESIAN_POINT('Ctrl Pts',(-10.5366356761104,12.2,4.13478216549277));
#254118=CARTESIAN_POINT('Ctrl Pts',(-10.5402108393966,12.2,4.13461857195744));
#254119=CARTESIAN_POINT('Ctrl Pts',(-10.5437927925323,12.2,4.13445049773075));
#254120=CARTESIAN_POINT('Ctrl Pts',(-10.5473814997343,12.2,4.13427791682097));
#254121=CARTESIAN_POINT('Ctrl Pts',(-10.5509702075883,12.2,4.13410533587983));
#254122=CARTESIAN_POINT('Ctrl Pts',(-10.5545656688775,12.2,4.13392824992077));
#254123=CARTESIAN_POINT('Ctrl Pts',(-10.558167849777,12.2,4.13374663147709));
#254124=CARTESIAN_POINT('Ctrl Pts',(-10.561770030022,12.2,4.1335650130664));
#254125=CARTESIAN_POINT('Ctrl Pts',(-10.5653789302329,12.2,4.13337886333287));
#254126=CARTESIAN_POINT('Ctrl Pts',(-10.5689945136996,12.2,4.13318815824641));
#254127=CARTESIAN_POINT('Ctrl Pts',(-10.5738152914363,12.2,4.13293388480935));
#254128=CARTESIAN_POINT('Ctrl Pts',(-10.578647952187,12.2,4.13267151039107));
#254129=CARTESIAN_POINT('Ctrl Pts',(-10.5834924128458,12.2,4.13240097724706));
#254130=CARTESIAN_POINT('Ctrl Pts',(-10.5871257585048,12.2,4.13219807737983));
#254131=CARTESIAN_POINT('Ctrl Pts',(-10.5907657411051,12.2,4.13199058847125));
#254132=CARTESIAN_POINT('Ctrl Pts',(-10.5944123272634,12.2,4.13177848606292));
#254133=CARTESIAN_POINT('Ctrl Pts',(-10.5980589140841,12.2,4.13156638361606));
#254134=CARTESIAN_POINT('Ctrl Pts',(-10.6017121028984,12.2,4.13134966840122));
#254135=CARTESIAN_POINT('Ctrl Pts',(-10.6053718607645,12.2,4.13112831495176));
#254136=CARTESIAN_POINT('Ctrl Pts',(-10.6090316179658,12.2,4.1309069615425));
#254137=CARTESIAN_POINT('Ctrl Pts',(-10.6126979430099,12.2,4.13068097014236));
#254138=CARTESIAN_POINT('Ctrl Pts',(-10.6163708019357,12.2,4.13045031718034));
#254139=CARTESIAN_POINT('Ctrl Pts',(-10.6200436608615,12.2,4.13021966421833));
#254140=CARTESIAN_POINT('Ctrl Pts',(-10.6237230535852,12.2,4.12998434946547));
#254141=CARTESIAN_POINT('Ctrl Pts',(-10.6274089448685,12.2,4.12974434897378));
#254142=CARTESIAN_POINT('Ctrl Pts',(-10.6323234663564,12.2,4.12942434833273));
#254143=CARTESIAN_POINT('Ctrl Pts',(-10.6372495424059,12.2,4.12909601684613));
#254144=CARTESIAN_POINT('Ctrl Pts',(-10.6421870925011,12.2,4.12875930159673));
#254145=CARTESIAN_POINT('Ctrl Pts',(-10.6458902559134,12.2,4.12850676510234));
#254146=CARTESIAN_POINT('Ctrl Pts',(-10.6495998736025,12.2,4.12824951111496));
#254147=CARTESIAN_POINT('Ctrl Pts',(-10.6533159110185,12.2,4.12798751715956));
#254148=CARTESIAN_POINT('Ctrl Pts',(-10.6595093051365,12.2,4.1275508606783));
#254149=CARTESIAN_POINT('Ctrl Pts',(-10.6657205296157,12.2,4.12710103619236));
#254150=CARTESIAN_POINT('Ctrl Pts',(-10.6719494262269,12.2,4.12663793478559));
#254151=CARTESIAN_POINT('Ctrl Pts',(-10.6769325443307,12.2,4.1262674535996));
#254152=CARTESIAN_POINT('Ctrl Pts',(-10.6819269728883,12.2,4.12588847646003));
#254153=CARTESIAN_POINT('Ctrl Pts',(-10.6869326397167,12.2,4.12550095455002));
#254154=CARTESIAN_POINT('Ctrl Pts',(-10.690686889497,12.2,4.12521031314391));
#254155=CARTESIAN_POINT('Ctrl Pts',(-10.6944474615269,12.2,4.12491486542134));
#254156=CARTESIAN_POINT('Ctrl Pts',(-10.6982143165979,12.2,4.12461458497433));
#254157=CARTESIAN_POINT('Ctrl Pts',(-10.7019811716688,12.2,4.12431430452733));
#254158=CARTESIAN_POINT('Ctrl Pts',(-10.7057543081181,12.2,4.12400919123026));
#254159=CARTESIAN_POINT('Ctrl Pts',(-10.7095336880022,12.2,4.12369921830994));
#254160=CARTESIAN_POINT('Ctrl Pts',(-10.7133130678863,12.2,4.12338924538962));
#254161=CARTESIAN_POINT('Ctrl Pts',(-10.717098688862,12.2,4.12307441270743));
#254162=CARTESIAN_POINT('Ctrl Pts',(-10.7208905289317,12.2,4.12275470459471));
#254163=CARTESIAN_POINT('Ctrl Pts',(-10.7259463161506,12.2,4.12232842707236));
#254164=CARTESIAN_POINT('Ctrl Pts',(-10.7310131599497,12.2,4.12189348245419));
#254165=CARTESIAN_POINT('Ctrl Pts',(-10.7360910480001,12.2,4.12144986899998));
#254166=CARTESIAN_POINT('Ctrl Pts',(-10.8675859440001,15.2,3.76106045599998));
#254167=CARTESIAN_POINT('Ctrl Pts',(-10.8675859440001,11.6,3.76106045599998));
#254168=CARTESIAN_POINT('Ctrl Pts',(-10.8670460920001,15.2,3.76051902299999));
#254169=CARTESIAN_POINT('Ctrl Pts',(-10.8670460920001,11.6,3.76051902299999));
#254170=CARTESIAN_POINT('Ctrl Pts',(-10.8659664940001,15.2,3.75943667499998));
#254171=CARTESIAN_POINT('Ctrl Pts',(-10.8659664940001,11.6,3.75943667499998));
#254172=CARTESIAN_POINT('Ctrl Pts',(-10.8643474220001,15.2,3.75781469799998));
#254173=CARTESIAN_POINT('Ctrl Pts',(-10.8643474220001,11.6,3.75781469799998));
#254174=CARTESIAN_POINT('Ctrl Pts',(-10.8621893020001,15.2,3.75565515599998));
#254175=CARTESIAN_POINT('Ctrl Pts',(-10.8621893020001,11.6,3.75565515599998));
#254176=CARTESIAN_POINT('Ctrl Pts',(-10.8594927310001,15.2,3.75296088399999));
#254177=CARTESIAN_POINT('Ctrl Pts',(-10.8594927310001,11.6,3.75296088399998));
#254178=CARTESIAN_POINT('Ctrl Pts',(-10.8567972360001,15.2,3.75027176899999));
#254179=CARTESIAN_POINT('Ctrl Pts',(-10.8567972360001,11.6,3.75027176899999));
#254180=CARTESIAN_POINT('Ctrl Pts',(-10.8541028210001,15.2,3.74758780899998));
#254181=CARTESIAN_POINT('Ctrl Pts',(-10.8541028210001,11.6,3.74758780899998));
#254182=CARTESIAN_POINT('Ctrl Pts',(-10.8514094910001,15.2,3.74490900599999));
#254183=CARTESIAN_POINT('Ctrl Pts',(-10.8514094910001,11.6,3.74490900599999));
#254184=CARTESIAN_POINT('Ctrl Pts',(-10.8487172500001,15.2,3.74223536099999));
#254185=CARTESIAN_POINT('Ctrl Pts',(-10.8487172500001,11.6,3.74223536099999));
#254186=CARTESIAN_POINT('Ctrl Pts',(-10.8460261070001,15.2,3.73956687399998));
#254187=CARTESIAN_POINT('Ctrl Pts',(-10.8460261070001,11.6,3.73956687399998));
#254188=CARTESIAN_POINT('Ctrl Pts',(-10.8433360710001,15.2,3.73690354799999));
#254189=CARTESIAN_POINT('Ctrl Pts',(-10.8433360710001,11.6,3.73690354799999));
#254190=CARTESIAN_POINT('Ctrl Pts',(-10.8406471530001,15.2,3.73424538199998));
#254191=CARTESIAN_POINT('Ctrl Pts',(-10.8406471530001,11.6,3.73424538199998));
#254192=CARTESIAN_POINT('Ctrl Pts',(-10.8379593660001,15.2,3.73159237899999));
#254193=CARTESIAN_POINT('Ctrl Pts',(-10.8379593660001,11.6,3.73159237899999));
#254194=CARTESIAN_POINT('Ctrl Pts',(-10.8352727180001,15.2,3.72894453799999));
#254195=CARTESIAN_POINT('Ctrl Pts',(-10.8352727180001,11.6,3.72894453799999));
#254196=CARTESIAN_POINT('Ctrl Pts',(-10.8325872200001,15.2,3.72630186199999));
#254197=CARTESIAN_POINT('Ctrl Pts',(-10.8325872200001,11.6,3.72630186199999));
#254198=CARTESIAN_POINT('Ctrl Pts',(-10.8299028840001,15.2,3.72366435199999));
#254199=CARTESIAN_POINT('Ctrl Pts',(-10.8299028840001,11.6,3.72366435199999));
#254200=CARTESIAN_POINT('Ctrl Pts',(-10.8272197160001,15.2,3.72103200799998));
#254201=CARTESIAN_POINT('Ctrl Pts',(-10.8272197160001,11.6,3.72103200799998));
#254202=CARTESIAN_POINT('Ctrl Pts',(-10.8245377250001,15.2,3.71840482999998));
#254203=CARTESIAN_POINT('Ctrl Pts',(-10.8245377250001,11.6,3.71840482999998));
#254204=CARTESIAN_POINT('Ctrl Pts',(-10.8218569190001,15.2,3.71578282199999));
#254205=CARTESIAN_POINT('Ctrl Pts',(-10.8218569190001,11.6,3.71578282199999));
#254206=CARTESIAN_POINT('Ctrl Pts',(-10.8191773060001,15.2,3.71316598199999));
#254207=CARTESIAN_POINT('Ctrl Pts',(-10.8191773060001,11.6,3.71316598199999));
#254208=CARTESIAN_POINT('Ctrl Pts',(-10.8164988950001,15.2,3.71055431199999));
#254209=CARTESIAN_POINT('Ctrl Pts',(-10.8164988950001,11.6,3.71055431199998));
#254210=CARTESIAN_POINT('Ctrl Pts',(-10.8138216940001,15.2,3.70794781399999));
#254211=CARTESIAN_POINT('Ctrl Pts',(-10.8138216940001,11.6,3.70794781399999));
#254212=CARTESIAN_POINT('Ctrl Pts',(-10.8111457130001,15.2,3.70534648599998));
#254213=CARTESIAN_POINT('Ctrl Pts',(-10.8111457130001,11.6,3.70534648599998));
#254214=CARTESIAN_POINT('Ctrl Pts',(-10.8084709620001,15.2,3.70275033099999));
#254215=CARTESIAN_POINT('Ctrl Pts',(-10.8084709620001,11.6,3.70275033099999));
#254216=CARTESIAN_POINT('Ctrl Pts',(-10.8057974490001,15.2,3.70015935099998));
#254217=CARTESIAN_POINT('Ctrl Pts',(-10.8057974490001,11.6,3.70015935099998));
#254218=CARTESIAN_POINT('Ctrl Pts',(-10.8031251850001,15.2,3.69757354499999));
#254219=CARTESIAN_POINT('Ctrl Pts',(-10.8031251850001,11.6,3.69757354499999));
#254220=CARTESIAN_POINT('Ctrl Pts',(-10.8004541780001,15.2,3.69499291399999));
#254221=CARTESIAN_POINT('Ctrl Pts',(-10.8004541780001,11.6,3.69499291399999));
#254222=CARTESIAN_POINT('Ctrl Pts',(-10.7977844380001,15.2,3.69241746099998));
#254223=CARTESIAN_POINT('Ctrl Pts',(-10.7977844380001,11.6,3.69241746099998));
#254224=CARTESIAN_POINT('Ctrl Pts',(-10.7951159740001,15.2,3.68984718499998));
#254225=CARTESIAN_POINT('Ctrl Pts',(-10.7951159740001,11.6,3.68984718499998));
#254226=CARTESIAN_POINT('Ctrl Pts',(-10.7924487950001,15.2,3.68728208699999));
#254227=CARTESIAN_POINT('Ctrl Pts',(-10.7924487950001,11.6,3.68728208699999));
#254228=CARTESIAN_POINT('Ctrl Pts',(-10.7897829100001,15.2,3.68472216799999));
#254229=CARTESIAN_POINT('Ctrl Pts',(-10.7897829100001,11.6,3.68472216799999));
#254230=CARTESIAN_POINT('Ctrl Pts',(-10.7871183270001,15.2,3.68216742999999));
#254231=CARTESIAN_POINT('Ctrl Pts',(-10.7871183270001,11.6,3.68216742999999));
#254232=CARTESIAN_POINT('Ctrl Pts',(-10.7844550570001,15.2,3.67961787199999));
#254233=CARTESIAN_POINT('Ctrl Pts',(-10.7844550570001,11.6,3.67961787199999));
#254234=CARTESIAN_POINT('Ctrl Pts',(-10.7817931080001,15.2,3.67707349599999));
#254235=CARTESIAN_POINT('Ctrl Pts',(-10.7817931080001,11.6,3.67707349599998));
#254236=CARTESIAN_POINT('Ctrl Pts',(-10.7791324900001,15.2,3.67453430299998));
#254237=CARTESIAN_POINT('Ctrl Pts',(-10.7791324900001,11.6,3.67453430299998));
#254238=CARTESIAN_POINT('Ctrl Pts',(-10.7764732120001,15.2,3.67200029299998));
#254239=CARTESIAN_POINT('Ctrl Pts',(-10.7764732120001,11.6,3.67200029299998));
#254240=CARTESIAN_POINT('Ctrl Pts',(-10.7738152830001,15.2,3.66947146699999));
#254241=CARTESIAN_POINT('Ctrl Pts',(-10.7738152830001,11.6,3.66947146699999));
#254242=CARTESIAN_POINT('Ctrl Pts',(-10.7711587130001,15.2,3.66694782799998));
#254243=CARTESIAN_POINT('Ctrl Pts',(-10.7711587130001,11.6,3.66694782799998));
#254244=CARTESIAN_POINT('Ctrl Pts',(-10.7685035120001,15.2,3.66442937399999));
#254245=CARTESIAN_POINT('Ctrl Pts',(-10.7685035120001,11.6,3.66442937399999));
#254246=CARTESIAN_POINT('Ctrl Pts',(-10.7658496880001,15.2,3.66191610799999));
#254247=CARTESIAN_POINT('Ctrl Pts',(-10.7658496880001,11.6,3.66191610799999));
#254248=CARTESIAN_POINT('Ctrl Pts',(-10.7631972500001,15.2,3.65940802799999));
#254249=CARTESIAN_POINT('Ctrl Pts',(-10.7631972500001,11.6,3.65940802799999));
#254250=CARTESIAN_POINT('Ctrl Pts',(-10.7605462090001,15.2,3.65690513799999));
#254251=CARTESIAN_POINT('Ctrl Pts',(-10.7605462090001,11.6,3.65690513799999));
#254252=CARTESIAN_POINT('Ctrl Pts',(-10.7578965730001,15.2,3.65440743699998));
#254253=CARTESIAN_POINT('Ctrl Pts',(-10.7578965730001,11.6,3.65440743699998));
#254254=CARTESIAN_POINT('Ctrl Pts',(-10.7552483530001,15.2,3.65191492699999));
#254255=CARTESIAN_POINT('Ctrl Pts',(-10.7552483530001,11.6,3.65191492699999));
#254256=CARTESIAN_POINT('Ctrl Pts',(-10.7526015570001,15.2,3.64942760599998));
#254257=CARTESIAN_POINT('Ctrl Pts',(-10.7526015570001,11.6,3.64942760599998));
#254258=CARTESIAN_POINT('Ctrl Pts',(-10.7499561940001,15.2,3.64694547899998));
#254259=CARTESIAN_POINT('Ctrl Pts',(-10.7499561940001,11.6,3.64694547899998));
#254260=CARTESIAN_POINT('Ctrl Pts',(-10.7473122750001,15.2,3.64446854399999));
#254261=CARTESIAN_POINT('Ctrl Pts',(-10.7473122750001,11.6,3.64446854399999));
#254262=CARTESIAN_POINT('Ctrl Pts',(-10.7446698090001,15.2,3.64199680199999));
#254263=CARTESIAN_POINT('Ctrl Pts',(-10.7446698090001,11.6,3.64199680199999));
#254264=CARTESIAN_POINT('Ctrl Pts',(-10.7420288050001,15.2,3.63953025399999));
#254265=CARTESIAN_POINT('Ctrl Pts',(-10.7420288050001,11.6,3.63953025399999));
#254266=CARTESIAN_POINT('Ctrl Pts',(-10.7393892730001,15.2,3.63706890199998));
#254267=CARTESIAN_POINT('Ctrl Pts',(-10.7393892730001,11.6,3.63706890199998));
#254268=CARTESIAN_POINT('Ctrl Pts',(-10.7367512220001,15.2,3.63461274599998));
#254269=CARTESIAN_POINT('Ctrl Pts',(-10.7367512220001,11.6,3.63461274599998));
#254270=CARTESIAN_POINT('Ctrl Pts',(-10.7341146620001,15.2,3.63216178499999));
#254271=CARTESIAN_POINT('Ctrl Pts',(-10.7341146620001,11.6,3.63216178499999));
#254272=CARTESIAN_POINT('Ctrl Pts',(-10.7314796030001,15.2,3.62971602199998));
#254273=CARTESIAN_POINT('Ctrl Pts',(-10.7314796030001,11.6,3.62971602199998));
#254274=CARTESIAN_POINT('Ctrl Pts',(-10.7288460530001,15.2,3.62727545699999));
#254275=CARTESIAN_POINT('Ctrl Pts',(-10.7288460530001,11.6,3.62727545699998));
#254276=CARTESIAN_POINT('Ctrl Pts',(-10.7262140240001,15.2,3.62484009099998));
#254277=CARTESIAN_POINT('Ctrl Pts',(-10.7262140240001,11.6,3.62484009099998));
#254278=CARTESIAN_POINT('Ctrl Pts',(-10.7235835250001,15.2,3.62240992399999));
#254279=CARTESIAN_POINT('Ctrl Pts',(-10.7235835250001,11.6,3.62240992399998));
#254280=CARTESIAN_POINT('Ctrl Pts',(-10.7209545640001,15.2,3.61998495799998));
#254281=CARTESIAN_POINT('Ctrl Pts',(-10.7209545640001,11.6,3.61998495799998));
#254282=CARTESIAN_POINT('Ctrl Pts',(-10.7183271510001,15.2,3.61756519299998));
#254283=CARTESIAN_POINT('Ctrl Pts',(-10.7183271510001,11.6,3.61756519299998));
#254284=CARTESIAN_POINT('Ctrl Pts',(-10.7157012970001,15.2,3.61515062899999));
#254285=CARTESIAN_POINT('Ctrl Pts',(-10.7157012970001,11.6,3.61515062899999));
#254286=CARTESIAN_POINT('Ctrl Pts',(-10.7130770100001,15.2,3.61274126799999));
#254287=CARTESIAN_POINT('Ctrl Pts',(-10.7130770100001,11.6,3.61274126799999));
#254288=CARTESIAN_POINT('Ctrl Pts',(-10.7104543020001,15.2,3.61033710899999));
#254289=CARTESIAN_POINT('Ctrl Pts',(-10.7104543020001,11.6,3.61033710899999));
#254290=CARTESIAN_POINT('Ctrl Pts',(-10.7078331810001,15.2,3.60793815499999));
#254291=CARTESIAN_POINT('Ctrl Pts',(-10.7078331810001,11.6,3.60793815499999));
#254292=CARTESIAN_POINT('Ctrl Pts',(-10.7052136580001,15.2,3.60554440499998));
#254293=CARTESIAN_POINT('Ctrl Pts',(-10.7052136580001,11.6,3.60554440499998));
#254294=CARTESIAN_POINT('Ctrl Pts',(-10.7025957410001,15.2,3.60315585999999));
#254295=CARTESIAN_POINT('Ctrl Pts',(-10.7025957410001,11.6,3.60315585999999));
#254296=CARTESIAN_POINT('Ctrl Pts',(-10.6999794400001,15.2,3.60077252099998));
#254297=CARTESIAN_POINT('Ctrl Pts',(-10.6999794400001,11.6,3.60077252099998));
#254298=CARTESIAN_POINT('Ctrl Pts',(-10.6973647670001,15.2,3.59839438899999));
#254299=CARTESIAN_POINT('Ctrl Pts',(-10.6973647670001,11.6,3.59839438899999));
#254300=CARTESIAN_POINT('Ctrl Pts',(-10.6947517300001,15.2,3.59602146299999));
#254301=CARTESIAN_POINT('Ctrl Pts',(-10.6947517300001,11.6,3.59602146299998));
#254302=CARTESIAN_POINT('Ctrl Pts',(-10.6921403400001,15.2,3.59365374499999));
#254303=CARTESIAN_POINT('Ctrl Pts',(-10.6921403400001,11.6,3.59365374499998));
#254304=CARTESIAN_POINT('Ctrl Pts',(-10.6895306050001,15.2,3.59129123499999));
#254305=CARTESIAN_POINT('Ctrl Pts',(-10.6895306050001,11.6,3.59129123499999));
#254306=CARTESIAN_POINT('Ctrl Pts',(-10.6869225370001,15.2,3.58893393499999));
#254307=CARTESIAN_POINT('Ctrl Pts',(-10.6869225370001,11.6,3.58893393499999));
#254308=CARTESIAN_POINT('Ctrl Pts',(-10.6843161440001,15.2,3.58658184499999));
#254309=CARTESIAN_POINT('Ctrl Pts',(-10.6843161440001,11.6,3.58658184499998));
#254310=CARTESIAN_POINT('Ctrl Pts',(-10.6817114370001,15.2,3.58423496499999));
#254311=CARTESIAN_POINT('Ctrl Pts',(-10.6817114370001,11.6,3.58423496499999));
#254312=CARTESIAN_POINT('Ctrl Pts',(-10.6791084260001,15.2,3.58189329599998));
#254313=CARTESIAN_POINT('Ctrl Pts',(-10.6791084260001,11.6,3.58189329599998));
#254314=CARTESIAN_POINT('Ctrl Pts',(-10.6765071210001,15.2,3.57955683899998));
#254315=CARTESIAN_POINT('Ctrl Pts',(-10.6765071210001,11.6,3.57955683899998));
#254316=CARTESIAN_POINT('Ctrl Pts',(-10.6739075300001,15.2,3.57722559299999));
#254317=CARTESIAN_POINT('Ctrl Pts',(-10.6739075300001,11.6,3.57722559299999));
#254318=CARTESIAN_POINT('Ctrl Pts',(-10.6713096660001,15.2,3.57489956099998));
#254319=CARTESIAN_POINT('Ctrl Pts',(-10.6713096660001,11.6,3.57489956099998));
#254320=CARTESIAN_POINT('Ctrl Pts',(-10.6687135380001,15.2,3.57257874199998));
#254321=CARTESIAN_POINT('Ctrl Pts',(-10.6687135380001,11.6,3.57257874199998));
#254322=CARTESIAN_POINT('Ctrl Pts',(-10.6661191560001,15.2,3.57026313699999));
#254323=CARTESIAN_POINT('Ctrl Pts',(-10.6661191560001,11.6,3.57026313699999));
#254324=CARTESIAN_POINT('Ctrl Pts',(-10.6635265280001,15.2,3.56795274599998));
#254325=CARTESIAN_POINT('Ctrl Pts',(-10.6635265280001,11.6,3.56795274599998));
#254326=CARTESIAN_POINT('Ctrl Pts',(-10.6609356680001,15.2,3.56564757199998));
#254327=CARTESIAN_POINT('Ctrl Pts',(-10.6609356680001,11.6,3.56564757199998));
#254328=CARTESIAN_POINT('Ctrl Pts',(-10.6583465820001,15.2,3.56334761199999));
#254329=CARTESIAN_POINT('Ctrl Pts',(-10.6583465820001,11.6,3.56334761199999));
#254330=CARTESIAN_POINT('Ctrl Pts',(-10.6557592820001,15.2,3.56105286799998));
#254331=CARTESIAN_POINT('Ctrl Pts',(-10.6557592820001,11.6,3.56105286799998));
#254332=CARTESIAN_POINT('Ctrl Pts',(-10.6531737790001,15.2,3.55876334199999));
#254333=CARTESIAN_POINT('Ctrl Pts',(-10.6531737790001,11.6,3.55876334199999));
#254334=CARTESIAN_POINT('Ctrl Pts',(-10.6505900820001,15.2,3.55647903299998));
#254335=CARTESIAN_POINT('Ctrl Pts',(-10.6505900820001,11.6,3.55647903299998));
#254336=CARTESIAN_POINT('Ctrl Pts',(-10.6480082030001,15.2,3.55419994099999));
#254337=CARTESIAN_POINT('Ctrl Pts',(-10.6480082030001,11.6,3.55419994099999));
#254338=CARTESIAN_POINT('Ctrl Pts',(-10.6454281490001,15.2,3.55192606799999));
#254339=CARTESIAN_POINT('Ctrl Pts',(-10.6454281490001,11.6,3.55192606799999));
#254340=CARTESIAN_POINT('Ctrl Pts',(-10.6428499330001,15.2,3.54965741499999));
#254341=CARTESIAN_POINT('Ctrl Pts',(-10.6428499330001,11.6,3.54965741499999));
#254342=CARTESIAN_POINT('Ctrl Pts',(-10.6402735620001,15.2,3.54739398099999));
#254343=CARTESIAN_POINT('Ctrl Pts',(-10.6402735620001,11.6,3.54739398099999));
#254344=CARTESIAN_POINT('Ctrl Pts',(-10.6376990500001,15.2,3.54513576599999));
#254345=CARTESIAN_POINT('Ctrl Pts',(-10.6376990500001,11.6,3.54513576599999));
#254346=CARTESIAN_POINT('Ctrl Pts',(-10.6351264060001,15.2,3.54288277199998));
#254347=CARTESIAN_POINT('Ctrl Pts',(-10.6351264060001,11.6,3.54288277199998));
#254348=CARTESIAN_POINT('Ctrl Pts',(-10.6325556390001,15.2,3.54063499899999));
#254349=CARTESIAN_POINT('Ctrl Pts',(-10.6325556390001,11.6,3.54063499899999));
#254350=CARTESIAN_POINT('Ctrl Pts',(-10.6299867610001,15.2,3.53839244699999));
#254351=CARTESIAN_POINT('Ctrl Pts',(-10.6299867610001,11.6,3.53839244699999));
#254352=CARTESIAN_POINT('Ctrl Pts',(-10.6274197800001,15.2,3.53615511799998));
#254353=CARTESIAN_POINT('Ctrl Pts',(-10.6274197800001,11.6,3.53615511799998));
#254354=CARTESIAN_POINT('Ctrl Pts',(-10.6248547090001,15.2,3.53392300999998));
#254355=CARTESIAN_POINT('Ctrl Pts',(-10.6248547090001,11.6,3.53392300999998));
#254356=CARTESIAN_POINT('Ctrl Pts',(-10.6222915560001,15.2,3.53169612599999));
#254357=CARTESIAN_POINT('Ctrl Pts',(-10.6222915560001,11.6,3.53169612599999));
#254358=CARTESIAN_POINT('Ctrl Pts',(-10.6197303340001,15.2,3.52947446499999));
#254359=CARTESIAN_POINT('Ctrl Pts',(-10.6197303340001,11.6,3.52947446499999));
#254360=CARTESIAN_POINT('Ctrl Pts',(-10.6171710520001,15.2,3.52725802799998));
#254361=CARTESIAN_POINT('Ctrl Pts',(-10.6171710520001,11.6,3.52725802799998));
#254362=CARTESIAN_POINT('Ctrl Pts',(-10.6146137200001,15.2,3.52504681499998));
#254363=CARTESIAN_POINT('Ctrl Pts',(-10.6146137200001,11.6,3.52504681499998));
#254364=CARTESIAN_POINT('Ctrl Pts',(-10.6120583480001,15.2,3.52284082599999));
#254365=CARTESIAN_POINT('Ctrl Pts',(-10.6120583480001,11.6,3.52284082599999));
#254366=CARTESIAN_POINT('Ctrl Pts',(-10.6095049490001,15.2,3.52064006199999));
#254367=CARTESIAN_POINT('Ctrl Pts',(-10.6095049490001,11.6,3.52064006199999));
#254368=CARTESIAN_POINT('Ctrl Pts',(-10.6069535310001,15.2,3.51844452499999));
#254369=CARTESIAN_POINT('Ctrl Pts',(-10.6069535310001,11.6,3.51844452499999));
#254370=CARTESIAN_POINT('Ctrl Pts',(-10.6044041060001,15.2,3.51625421299998));
#254371=CARTESIAN_POINT('Ctrl Pts',(-10.6044041060001,11.6,3.51625421299998));
#254372=CARTESIAN_POINT('Ctrl Pts',(-10.6018566830001,15.2,3.51406912799998));
#254373=CARTESIAN_POINT('Ctrl Pts',(-10.6018566830001,11.6,3.51406912799998));
#254374=CARTESIAN_POINT('Ctrl Pts',(-10.5993112740001,15.2,3.51188926799999));
#254375=CARTESIAN_POINT('Ctrl Pts',(-10.5993112740001,11.6,3.51188926799999));
#254376=CARTESIAN_POINT('Ctrl Pts',(-10.5967678890001,15.2,3.50971463699998));
#254377=CARTESIAN_POINT('Ctrl Pts',(-10.5967678890001,11.6,3.50971463699998));
#254378=CARTESIAN_POINT('Ctrl Pts',(-10.5942265380001,15.2,3.50754523199999));
#254379=CARTESIAN_POINT('Ctrl Pts',(-10.5942265380001,11.6,3.50754523199999));
#254380=CARTESIAN_POINT('Ctrl Pts',(-10.5916872330001,15.2,3.50538105599998));
#254381=CARTESIAN_POINT('Ctrl Pts',(-10.5916872330001,11.6,3.50538105599998));
#254382=CARTESIAN_POINT('Ctrl Pts',(-10.5891499840001,15.2,3.50322210699999));
#254383=CARTESIAN_POINT('Ctrl Pts',(-10.5891499840001,11.6,3.50322210699999));
#254384=CARTESIAN_POINT('Ctrl Pts',(-10.5866148010001,15.2,3.50106838699999));
#254385=CARTESIAN_POINT('Ctrl Pts',(-10.5866148010001,11.6,3.50106838699999));
#254386=CARTESIAN_POINT('Ctrl Pts',(-10.5840816950001,15.2,3.49891989599998));
#254387=CARTESIAN_POINT('Ctrl Pts',(-10.5840816950001,11.6,3.49891989599998));
#254388=CARTESIAN_POINT('Ctrl Pts',(-10.5815506770001,15.2,3.49677663499998));
#254389=CARTESIAN_POINT('Ctrl Pts',(-10.5815506770001,11.6,3.49677663499998));
#254390=CARTESIAN_POINT('Ctrl Pts',(-10.5790217580001,15.2,3.49463860299998));
#254391=CARTESIAN_POINT('Ctrl Pts',(-10.5790217580001,11.6,3.49463860299998));
#254392=CARTESIAN_POINT('Ctrl Pts',(-10.5764949480001,15.2,3.49250580099999));
#254393=CARTESIAN_POINT('Ctrl Pts',(-10.5764949480001,11.6,3.49250580099999));
#254394=CARTESIAN_POINT('Ctrl Pts',(-10.5739702580001,15.2,3.49037822899999));
#254395=CARTESIAN_POINT('Ctrl Pts',(-10.5739702580001,11.6,3.49037822899999));
#254396=CARTESIAN_POINT('Ctrl Pts',(-10.5714477000001,15.2,3.48825588799999));
#254397=CARTESIAN_POINT('Ctrl Pts',(-10.5714477000001,11.6,3.48825588799999));
#254398=CARTESIAN_POINT('Ctrl Pts',(-10.5689272830001,15.2,3.48613877799998));
#254399=CARTESIAN_POINT('Ctrl Pts',(-10.5689272830001,11.6,3.48613877799998));
#254400=CARTESIAN_POINT('Ctrl Pts',(-10.5664090190001,15.2,3.48402689799999));
#254401=CARTESIAN_POINT('Ctrl Pts',(-10.5664090190001,11.6,3.48402689799999));
#254402=CARTESIAN_POINT('Ctrl Pts',(-10.5638929170001,15.2,3.48192024999998));
#254403=CARTESIAN_POINT('Ctrl Pts',(-10.5638929170001,11.6,3.48192024999998));
#254404=CARTESIAN_POINT('Ctrl Pts',(-10.5613789900001,15.2,3.47981883399999));
#254405=CARTESIAN_POINT('Ctrl Pts',(-10.5613789900001,11.6,3.47981883399999));
#254406=CARTESIAN_POINT('Ctrl Pts',(-10.5588672490001,15.2,3.47772264899999));
#254407=CARTESIAN_POINT('Ctrl Pts',(-10.5588672490001,11.6,3.47772264899999));
#254408=CARTESIAN_POINT('Ctrl Pts',(-10.5563577040001,15.2,3.47563169699999));
#254409=CARTESIAN_POINT('Ctrl Pts',(-10.5563577040001,11.6,3.47563169699999));
#254410=CARTESIAN_POINT('Ctrl Pts',(-10.5538503660001,15.2,3.47354597799999));
#254411=CARTESIAN_POINT('Ctrl Pts',(-10.5538503660001,11.6,3.47354597799999));
#254412=CARTESIAN_POINT('Ctrl Pts',(-10.5513452450001,15.2,3.47146549099998));
#254413=CARTESIAN_POINT('Ctrl Pts',(-10.5513452450001,11.6,3.47146549099998));
#254414=CARTESIAN_POINT('Ctrl Pts',(-10.5488423530001,15.2,3.46939023799998));
#254415=CARTESIAN_POINT('Ctrl Pts',(-10.5488423530001,11.6,3.46939023799998));
#254416=CARTESIAN_POINT('Ctrl Pts',(-10.5463417020001,15.2,3.46732021699999));
#254417=CARTESIAN_POINT('Ctrl Pts',(-10.5463417020001,11.6,3.46732021699999));
#254418=CARTESIAN_POINT('Ctrl Pts',(-10.5438433010001,15.2,3.46525543099999));
#254419=CARTESIAN_POINT('Ctrl Pts',(-10.5438433010001,11.6,3.46525543099998));
#254420=CARTESIAN_POINT('Ctrl Pts',(-10.5413471640001,15.2,3.46319587699998));
#254421=CARTESIAN_POINT('Ctrl Pts',(-10.5413471640001,11.6,3.46319587699998));
#254422=CARTESIAN_POINT('Ctrl Pts',(-10.5388532990001,15.2,3.46114155699999));
#254423=CARTESIAN_POINT('Ctrl Pts',(-10.5388532990001,11.6,3.46114155699999));
#254424=CARTESIAN_POINT('Ctrl Pts',(-10.5363617170001,15.2,3.45909247099998));
#254425=CARTESIAN_POINT('Ctrl Pts',(-10.5363617170001,11.6,3.45909247099998));
#254426=CARTESIAN_POINT('Ctrl Pts',(-10.5338724320001,15.2,3.45704862099999));
#254427=CARTESIAN_POINT('Ctrl Pts',(-10.5338724320001,11.6,3.45704862099998));
#254428=CARTESIAN_POINT('Ctrl Pts',(-10.5313854540001,15.2,3.45501000399998));
#254429=CARTESIAN_POINT('Ctrl Pts',(-10.5313854540001,11.6,3.45501000399998));
#254430=CARTESIAN_POINT('Ctrl Pts',(-10.5289007930001,15.2,3.45297662099998));
#254431=CARTESIAN_POINT('Ctrl Pts',(-10.5289007930001,11.6,3.45297662099998));
#254432=CARTESIAN_POINT('Ctrl Pts',(-10.5264184600001,15.2,3.45094847299999));
#254433=CARTESIAN_POINT('Ctrl Pts',(-10.5264184600001,11.6,3.45094847299999));
#254434=CARTESIAN_POINT('Ctrl Pts',(-10.5239384690001,15.2,3.44892556099998));
#254435=CARTESIAN_POINT('Ctrl Pts',(-10.5239384690001,11.6,3.44892556099998));
#254436=CARTESIAN_POINT('Ctrl Pts',(-10.5214608280001,15.2,3.44690788299998));
#254437=CARTESIAN_POINT('Ctrl Pts',(-10.5214608280001,11.6,3.44690788299998));
#254438=CARTESIAN_POINT('Ctrl Pts',(-10.5189855500001,15.2,3.44489544099999));
#254439=CARTESIAN_POINT('Ctrl Pts',(-10.5189855500001,11.6,3.44489544099999));
#254440=CARTESIAN_POINT('Ctrl Pts',(-10.5165126460001,15.2,3.44288823299999));
#254441=CARTESIAN_POINT('Ctrl Pts',(-10.5165126460001,11.6,3.44288823299999));
#254442=CARTESIAN_POINT('Ctrl Pts',(-10.5140421270001,15.2,3.44088626199999));
#254443=CARTESIAN_POINT('Ctrl Pts',(-10.5140421270001,11.6,3.44088626199999));
#254444=CARTESIAN_POINT('Ctrl Pts',(-10.5115740050001,15.2,3.43888952499999));
#254445=CARTESIAN_POINT('Ctrl Pts',(-10.5115740050001,11.6,3.43888952499999));
#254446=CARTESIAN_POINT('Ctrl Pts',(-10.5091082900001,15.2,3.43689802399999));
#254447=CARTESIAN_POINT('Ctrl Pts',(-10.5091082900001,11.6,3.43689802399999));
#254448=CARTESIAN_POINT('Ctrl Pts',(-10.5066449960001,15.2,3.43491175999999));
#254449=CARTESIAN_POINT('Ctrl Pts',(-10.5066449960001,11.6,3.43491175999999));
#254450=CARTESIAN_POINT('Ctrl Pts',(-10.5041841310001,15.2,3.43293073099999));
#254451=CARTESIAN_POINT('Ctrl Pts',(-10.5041841310001,11.6,3.43293073099999));
#254452=CARTESIAN_POINT('Ctrl Pts',(-10.5017257090001,15.2,3.43095493799999));
#254453=CARTESIAN_POINT('Ctrl Pts',(-10.5017257090001,11.6,3.43095493799999));
#254454=CARTESIAN_POINT('Ctrl Pts',(-10.4992697400001,15.2,3.42898438099999));
#254455=CARTESIAN_POINT('Ctrl Pts',(-10.4992697400001,11.6,3.42898438099999));
#254456=CARTESIAN_POINT('Ctrl Pts',(-10.4968162370001,15.2,3.42701905899998));
#254457=CARTESIAN_POINT('Ctrl Pts',(-10.4968162370001,11.6,3.42701905899998));
#254458=CARTESIAN_POINT('Ctrl Pts',(-10.4943652100001,15.2,3.42505897499999));
#254459=CARTESIAN_POINT('Ctrl Pts',(-10.4943652100001,11.6,3.42505897499999));
#254460=CARTESIAN_POINT('Ctrl Pts',(-10.4919166710001,15.2,3.42310412499998));
#254461=CARTESIAN_POINT('Ctrl Pts',(-10.4919166710001,11.6,3.42310412499998));
#254462=CARTESIAN_POINT('Ctrl Pts',(-10.4894706320001,15.2,3.42115451299998));
#254463=CARTESIAN_POINT('Ctrl Pts',(-10.4894706320001,11.6,3.42115451299998));
#254464=CARTESIAN_POINT('Ctrl Pts',(-10.4870271040001,15.2,3.41921013599999));
#254465=CARTESIAN_POINT('Ctrl Pts',(-10.4870271040001,11.6,3.41921013599999));
#254466=CARTESIAN_POINT('Ctrl Pts',(-10.4845861000001,15.2,3.41727099599999));
#254467=CARTESIAN_POINT('Ctrl Pts',(-10.4845861000001,11.6,3.41727099599999));
#254468=CARTESIAN_POINT('Ctrl Pts',(-10.4821476300001,15.2,3.41533709199999));
#254469=CARTESIAN_POINT('Ctrl Pts',(-10.4821476300001,11.6,3.41533709199999));
#254470=CARTESIAN_POINT('Ctrl Pts',(-10.4797117050001,15.2,3.41340842399998));
#254471=CARTESIAN_POINT('Ctrl Pts',(-10.4797117050001,11.6,3.41340842399998));
#254472=CARTESIAN_POINT('Ctrl Pts',(-10.4772783390001,15.2,3.41148499199999));
#254473=CARTESIAN_POINT('Ctrl Pts',(-10.4772783390001,11.6,3.41148499199999));
#254474=CARTESIAN_POINT('Ctrl Pts',(-10.4748475420001,15.2,3.40956679599999));
#254475=CARTESIAN_POINT('Ctrl Pts',(-10.4748475420001,11.6,3.40956679599999));
#254476=CARTESIAN_POINT('Ctrl Pts',(-10.4724193270001,15.2,3.40765383599998));
#254477=CARTESIAN_POINT('Ctrl Pts',(-10.4724193270001,11.6,3.40765383599998));
#254478=CARTESIAN_POINT('Ctrl Pts',(-10.4699937050001,15.2,3.40574611299999));
#254479=CARTESIAN_POINT('Ctrl Pts',(-10.4699937050001,11.6,3.40574611299999));
#254480=CARTESIAN_POINT('Ctrl Pts',(-10.4675706860001,15.2,3.40384362499999));
#254481=CARTESIAN_POINT('Ctrl Pts',(-10.4675706860001,11.6,3.40384362499999));
#254482=CARTESIAN_POINT('Ctrl Pts',(-10.4651502850001,15.2,3.40194637399998));
#254483=CARTESIAN_POINT('Ctrl Pts',(-10.4651502850001,11.6,3.40194637399998));
#254484=CARTESIAN_POINT('Ctrl Pts',(-10.4627325130001,15.2,3.40005435799998));
#254485=CARTESIAN_POINT('Ctrl Pts',(-10.4627325130001,11.6,3.40005435799998));
#254486=CARTESIAN_POINT('Ctrl Pts',(-10.4603173810001,15.2,3.39816757999999));
#254487=CARTESIAN_POINT('Ctrl Pts',(-10.4603173810001,11.6,3.39816757999999));
#254488=CARTESIAN_POINT('Ctrl Pts',(-10.4579049000001,15.2,3.39628603499998));
#254489=CARTESIAN_POINT('Ctrl Pts',(-10.4579049000001,11.6,3.39628603499998));
#254490=CARTESIAN_POINT('Ctrl Pts',(-10.4554950840001,15.2,3.39440972699999));
#254491=CARTESIAN_POINT('Ctrl Pts',(-10.4554950840001,11.6,3.39440972699998));
#254492=CARTESIAN_POINT('Ctrl Pts',(-10.4530879440001,15.2,3.39253865399999));
#254493=CARTESIAN_POINT('Ctrl Pts',(-10.4530879440001,11.6,3.39253865399999));
#254494=CARTESIAN_POINT('Ctrl Pts',(-10.4506834930001,15.2,3.39067281699998));
#254495=CARTESIAN_POINT('Ctrl Pts',(-10.4506834930001,11.6,3.39067281699998));
#254496=CARTESIAN_POINT('Ctrl Pts',(-10.4482817400001,15.2,3.38881221399999));
#254497=CARTESIAN_POINT('Ctrl Pts',(-10.4482817400001,11.6,3.38881221399999));
#254498=CARTESIAN_POINT('Ctrl Pts',(-10.4458827010001,15.2,3.38695684799998));
#254499=CARTESIAN_POINT('Ctrl Pts',(-10.4458827010001,11.6,3.38695684799998));
#254500=CARTESIAN_POINT('Ctrl Pts',(-10.4434863850001,15.2,3.38510671599998));
#254501=CARTESIAN_POINT('Ctrl Pts',(-10.4434863850001,11.6,3.38510671599998));
#254502=CARTESIAN_POINT('Ctrl Pts',(-10.4410928060001,15.2,3.38326181899999));
#254503=CARTESIAN_POINT('Ctrl Pts',(-10.4410928060001,11.6,3.38326181899998));
#254504=CARTESIAN_POINT('Ctrl Pts',(-10.4387019740001,15.2,3.38142215599999));
#254505=CARTESIAN_POINT('Ctrl Pts',(-10.4387019740001,11.6,3.38142215599999));
#254506=CARTESIAN_POINT('Ctrl Pts',(-10.4363139020001,15.2,3.37958772799999));
#254507=CARTESIAN_POINT('Ctrl Pts',(-10.4363139020001,11.6,3.37958772799999));
#254508=CARTESIAN_POINT('Ctrl Pts',(-10.4339286050001,15.2,3.37775853599998));
#254509=CARTESIAN_POINT('Ctrl Pts',(-10.4339286050001,11.6,3.37775853599998));
#254510=CARTESIAN_POINT('Ctrl Pts',(-10.4315460910001,15.2,3.37593457599999));
#254511=CARTESIAN_POINT('Ctrl Pts',(-10.4315460910001,11.6,3.37593457599999));
#254512=CARTESIAN_POINT('Ctrl Pts',(-10.4291663730001,15.2,3.37411585099999));
#254513=CARTESIAN_POINT('Ctrl Pts',(-10.4291663730001,11.6,3.37411585099999));
#254514=CARTESIAN_POINT('Ctrl Pts',(-10.4267894660001,15.2,3.37230235899998));
#254515=CARTESIAN_POINT('Ctrl Pts',(-10.4267894660001,11.6,3.37230235899998));
#254516=CARTESIAN_POINT('Ctrl Pts',(-10.4244153790001,15.2,3.37049410099999));
#254517=CARTESIAN_POINT('Ctrl Pts',(-10.4244153790001,11.6,3.37049410099999));
#254518=CARTESIAN_POINT('Ctrl Pts',(-10.4220441260001,15.2,3.36869107699999));
#254519=CARTESIAN_POINT('Ctrl Pts',(-10.4220441260001,11.6,3.36869107699999));
#254520=CARTESIAN_POINT('Ctrl Pts',(-10.4196757190001,15.2,3.36689328499999));
#254521=CARTESIAN_POINT('Ctrl Pts',(-10.4196757190001,11.6,3.36689328499999));
#254522=CARTESIAN_POINT('Ctrl Pts',(-10.4173101710001,15.2,3.36510072599999));
#254523=CARTESIAN_POINT('Ctrl Pts',(-10.4173101710001,11.6,3.36510072599999));
#254524=CARTESIAN_POINT('Ctrl Pts',(-10.4149474930001,15.2,3.36331339999998));
#254525=CARTESIAN_POINT('Ctrl Pts',(-10.4149474930001,11.6,3.36331339999998));
#254526=CARTESIAN_POINT('Ctrl Pts',(-10.4125876980001,15.2,3.36153130599998));
#254527=CARTESIAN_POINT('Ctrl Pts',(-10.4125876980001,11.6,3.36153130599998));
#254528=CARTESIAN_POINT('Ctrl Pts',(-10.4102307990001,15.2,3.35975444399998));
#254529=CARTESIAN_POINT('Ctrl Pts',(-10.4102307990001,11.6,3.35975444399998));
#254530=CARTESIAN_POINT('Ctrl Pts',(-10.4078768090001,15.2,3.35798281399998));
#254531=CARTESIAN_POINT('Ctrl Pts',(-10.4078768090001,11.6,3.35798281399998));
#254532=CARTESIAN_POINT('Ctrl Pts',(-10.4055257380001,15.2,3.35621641399998));
#254533=CARTESIAN_POINT('Ctrl Pts',(-10.4055257380001,11.6,3.35621641399998));
#254534=CARTESIAN_POINT('Ctrl Pts',(-10.4031776000001,15.2,3.35445524599999));
#254535=CARTESIAN_POINT('Ctrl Pts',(-10.4031776000001,11.6,3.35445524599999));
#254536=CARTESIAN_POINT('Ctrl Pts',(-10.4008324080001,15.2,3.35269930899998));
#254537=CARTESIAN_POINT('Ctrl Pts',(-10.4008324080001,11.6,3.35269930899998));
#254538=CARTESIAN_POINT('Ctrl Pts',(-10.3984901750001,15.2,3.35094860299999));
#254539=CARTESIAN_POINT('Ctrl Pts',(-10.3984901750001,11.6,3.35094860299999));
#254540=CARTESIAN_POINT('Ctrl Pts',(-10.3961509110001,15.2,3.34920312599999));
#254541=CARTESIAN_POINT('Ctrl Pts',(-10.3961509110001,11.6,3.34920312599999));
#254542=CARTESIAN_POINT('Ctrl Pts',(-10.3938146310001,15.2,3.34746287999998));
#254543=CARTESIAN_POINT('Ctrl Pts',(-10.3938146310001,11.6,3.34746287999998));
#254544=CARTESIAN_POINT('Ctrl Pts',(-10.3914813470001,15.2,3.34572786199999));
#254545=CARTESIAN_POINT('Ctrl Pts',(-10.3914813470001,11.6,3.34572786199998));
#254546=CARTESIAN_POINT('Ctrl Pts',(-10.3891510720001,15.2,3.34399807399999));
#254547=CARTESIAN_POINT('Ctrl Pts',(-10.3891510720001,11.6,3.34399807399999));
#254548=CARTESIAN_POINT('Ctrl Pts',(-10.3868238190001,15.2,3.34227351299998));
#254549=CARTESIAN_POINT('Ctrl Pts',(-10.3868238190001,11.6,3.34227351299998));
#254550=CARTESIAN_POINT('Ctrl Pts',(-10.3844995990001,15.2,3.34055418199998));
#254551=CARTESIAN_POINT('Ctrl Pts',(-10.3844995990001,11.6,3.34055418199998));
#254552=CARTESIAN_POINT('Ctrl Pts',(-10.3821784260001,15.2,3.33884007799998));
#254553=CARTESIAN_POINT('Ctrl Pts',(-10.3821784260001,11.6,3.33884007799998));
#254554=CARTESIAN_POINT('Ctrl Pts',(-10.3798603140001,15.2,3.33713120199998));
#254555=CARTESIAN_POINT('Ctrl Pts',(-10.3798603140001,11.6,3.33713120199998));
#254556=CARTESIAN_POINT('Ctrl Pts',(-10.3775452740001,15.2,3.33542755199999));
#254557=CARTESIAN_POINT('Ctrl Pts',(-10.3775452740001,11.6,3.33542755199998));
#254558=CARTESIAN_POINT('Ctrl Pts',(-10.3752333190001,15.2,3.33372912899998));
#254559=CARTESIAN_POINT('Ctrl Pts',(-10.3752333190001,11.6,3.33372912899998));
#254560=CARTESIAN_POINT('Ctrl Pts',(-10.3729244630001,15.2,3.33203593199999));
#254561=CARTESIAN_POINT('Ctrl Pts',(-10.3729244630001,11.6,3.33203593199999));
#254562=CARTESIAN_POINT('Ctrl Pts',(-10.3706187180001,15.2,3.33034796199998));
#254563=CARTESIAN_POINT('Ctrl Pts',(-10.3706187180001,11.6,3.33034796199998));
#254564=CARTESIAN_POINT('Ctrl Pts',(-10.3683160970001,15.2,3.32866521499999));
#254565=CARTESIAN_POINT('Ctrl Pts',(-10.3683160970001,11.6,3.32866521499999));
#254566=CARTESIAN_POINT('Ctrl Pts',(-10.3660166140001,15.2,3.32698769399999));
#254567=CARTESIAN_POINT('Ctrl Pts',(-10.3660166140001,11.6,3.32698769399998));
#254568=CARTESIAN_POINT('Ctrl Pts',(-10.3637202810001,15.2,3.32531539599999));
#254569=CARTESIAN_POINT('Ctrl Pts',(-10.3637202810001,11.6,3.32531539599999));
#254570=CARTESIAN_POINT('Ctrl Pts',(-10.3614271110001,15.2,3.32364832299999));
#254571=CARTESIAN_POINT('Ctrl Pts',(-10.3614271110001,11.6,3.32364832299999));
#254572=CARTESIAN_POINT('Ctrl Pts',(-10.3591371170001,15.2,3.32198647299998));
#254573=CARTESIAN_POINT('Ctrl Pts',(-10.3591371170001,11.6,3.32198647299998));
#254574=CARTESIAN_POINT('Ctrl Pts',(-10.3568503140001,15.2,3.32032984499998));
#254575=CARTESIAN_POINT('Ctrl Pts',(-10.3568503140001,11.6,3.32032984499998));
#254576=CARTESIAN_POINT('Ctrl Pts',(-10.3545667120001,15.2,3.31867843999999));
#254577=CARTESIAN_POINT('Ctrl Pts',(-10.3545667120001,11.6,3.31867843999999));
#254578=CARTESIAN_POINT('Ctrl Pts',(-10.3522863270001,15.2,3.31703225499999));
#254579=CARTESIAN_POINT('Ctrl Pts',(-10.3522863270001,11.6,3.31703225499999));
#254580=CARTESIAN_POINT('Ctrl Pts',(-10.3500091710001,15.2,3.31539129199999));
#254581=CARTESIAN_POINT('Ctrl Pts',(-10.3500091710001,11.6,3.31539129199999));
#254582=CARTESIAN_POINT('Ctrl Pts',(-10.3477352560001,15.2,3.31375554999998));
#254583=CARTESIAN_POINT('Ctrl Pts',(-10.3477352560001,11.6,3.31375554999998));
#254584=CARTESIAN_POINT('Ctrl Pts',(-10.3454645980001,15.2,3.31212502699999));
#254585=CARTESIAN_POINT('Ctrl Pts',(-10.3454645980001,11.6,3.31212502699999));
#254586=CARTESIAN_POINT('Ctrl Pts',(-10.3431972080001,15.2,3.31049972399998));
#254587=CARTESIAN_POINT('Ctrl Pts',(-10.3431972080001,11.6,3.31049972399998));
#254588=CARTESIAN_POINT('Ctrl Pts',(-10.3409331010001,15.2,3.30887963799999));
#254589=CARTESIAN_POINT('Ctrl Pts',(-10.3409331010001,11.6,3.30887963799999));
#254590=CARTESIAN_POINT('Ctrl Pts',(-10.3386722900001,15.2,3.30726477199998));
#254591=CARTESIAN_POINT('Ctrl Pts',(-10.3386722900001,11.6,3.30726477199998));
#254592=CARTESIAN_POINT('Ctrl Pts',(-10.3364147870001,15.2,3.30565512299999));
#254593=CARTESIAN_POINT('Ctrl Pts',(-10.3364147870001,11.6,3.30565512299999));
#254594=CARTESIAN_POINT('Ctrl Pts',(-10.3341606070001,15.2,3.30405068899999));
#254595=CARTESIAN_POINT('Ctrl Pts',(-10.3341606070001,11.6,3.30405068899999));
#254596=CARTESIAN_POINT('Ctrl Pts',(-10.3319097620001,15.2,3.30245147299999));
#254597=CARTESIAN_POINT('Ctrl Pts',(-10.3319097620001,11.6,3.30245147299998));
#254598=CARTESIAN_POINT('Ctrl Pts',(-10.3296622670001,15.2,3.30085747299999));
#254599=CARTESIAN_POINT('Ctrl Pts',(-10.3296622670001,11.6,3.30085747299999));
#254600=CARTESIAN_POINT('Ctrl Pts',(-10.3274181360001,15.2,3.29926868599999));
#254601=CARTESIAN_POINT('Ctrl Pts',(-10.3274181360001,11.6,3.29926868599998));
#254602=CARTESIAN_POINT('Ctrl Pts',(-10.3251773800001,15.2,3.29768511399998));
#254603=CARTESIAN_POINT('Ctrl Pts',(-10.3251773800001,11.6,3.29768511399998));
#254604=CARTESIAN_POINT('Ctrl Pts',(-10.3229400150001,15.2,3.29610675499998));
#254605=CARTESIAN_POINT('Ctrl Pts',(-10.3229400150001,11.6,3.29610675499998));
#254606=CARTESIAN_POINT('Ctrl Pts',(-10.3207060530001,15.2,3.29453360999998));
#254607=CARTESIAN_POINT('Ctrl Pts',(-10.3207060530001,11.6,3.29453360999998));
#254608=CARTESIAN_POINT('Ctrl Pts',(-10.3184755090001,15.2,3.29296567599999));
#254609=CARTESIAN_POINT('Ctrl Pts',(-10.3184755090001,11.6,3.29296567599999));
#254610=CARTESIAN_POINT('Ctrl Pts',(-10.3162483960001,15.2,3.29140295299998));
#254611=CARTESIAN_POINT('Ctrl Pts',(-10.3162483960001,11.6,3.29140295299998));
#254612=CARTESIAN_POINT('Ctrl Pts',(-10.3140247280001,15.2,3.28984543999999));
#254613=CARTESIAN_POINT('Ctrl Pts',(-10.3140247280001,11.6,3.28984543999999));
#254614=CARTESIAN_POINT('Ctrl Pts',(-10.3118045180001,15.2,3.28829313799999));
#254615=CARTESIAN_POINT('Ctrl Pts',(-10.3118045180001,11.6,3.28829313799999));
#254616=CARTESIAN_POINT('Ctrl Pts',(-10.3095877810001,15.2,3.28674604399998));
#254617=CARTESIAN_POINT('Ctrl Pts',(-10.3095877810001,11.6,3.28674604399998));
#254618=CARTESIAN_POINT('Ctrl Pts',(-10.3073745300001,15.2,3.28520415899998));
#254619=CARTESIAN_POINT('Ctrl Pts',(-10.3073745300001,11.6,3.28520415899998));
#254620=CARTESIAN_POINT('Ctrl Pts',(-10.3051647790001,15.2,3.28366748199999));
#254621=CARTESIAN_POINT('Ctrl Pts',(-10.3051647790001,11.6,3.28366748199999));
#254622=CARTESIAN_POINT('Ctrl Pts',(-10.3029585420001,15.2,3.28213600999998));
#254623=CARTESIAN_POINT('Ctrl Pts',(-10.3029585420001,11.6,3.28213600999998));
#254624=CARTESIAN_POINT('Ctrl Pts',(-10.3007558330001,15.2,3.28060974499999));
#254625=CARTESIAN_POINT('Ctrl Pts',(-10.3007558330001,11.6,3.28060974499999));
#254626=CARTESIAN_POINT('Ctrl Pts',(-10.2985566670001,15.2,3.27908868399999));
#254627=CARTESIAN_POINT('Ctrl Pts',(-10.2985566670001,11.6,3.27908868399999));
#254628=CARTESIAN_POINT('Ctrl Pts',(-10.2963610560001,15.2,3.27757282799999));
#254629=CARTESIAN_POINT('Ctrl Pts',(-10.2963610560001,11.6,3.27757282799999));
#254630=CARTESIAN_POINT('Ctrl Pts',(-10.2941690160001,15.2,3.27606217499999));
#254631=CARTESIAN_POINT('Ctrl Pts',(-10.2941690160001,11.6,3.27606217499999));
#254632=CARTESIAN_POINT('Ctrl Pts',(-10.2919805600001,15.2,3.27455672399999));
#254633=CARTESIAN_POINT('Ctrl Pts',(-10.2919805600001,11.6,3.27455672399999));
#254634=CARTESIAN_POINT('Ctrl Pts',(-10.2897957010001,15.2,3.27305647499998));
#254635=CARTESIAN_POINT('Ctrl Pts',(-10.2897957010001,11.6,3.27305647499998));
#254636=CARTESIAN_POINT('Ctrl Pts',(-10.2876144550001,15.2,3.27156142699998));
#254637=CARTESIAN_POINT('Ctrl Pts',(-10.2876144550001,11.6,3.27156142699998));
#254638=CARTESIAN_POINT('Ctrl Pts',(-10.2854368370001,15.2,3.27007157799999));
#254639=CARTESIAN_POINT('Ctrl Pts',(-10.2854368370001,11.6,3.27007157799999));
#254640=CARTESIAN_POINT('Ctrl Pts',(-10.2832628580001,15.2,3.26858692799998));
#254641=CARTESIAN_POINT('Ctrl Pts',(-10.2832628580001,11.6,3.26858692799998));
#254642=CARTESIAN_POINT('Ctrl Pts',(-10.2810925340001,15.2,3.26710747599999));
#254643=CARTESIAN_POINT('Ctrl Pts',(-10.2810925340001,11.6,3.26710747599999));
#254644=CARTESIAN_POINT('Ctrl Pts',(-10.2789258800001,15.2,3.26563322099998));
#254645=CARTESIAN_POINT('Ctrl Pts',(-10.2789258800001,11.6,3.26563322099998));
#254646=CARTESIAN_POINT('Ctrl Pts',(-10.2767629100001,15.2,3.26416416199999));
#254647=CARTESIAN_POINT('Ctrl Pts',(-10.2767629100001,11.6,3.26416416199999));
#254648=CARTESIAN_POINT('Ctrl Pts',(-10.2746036380001,15.2,3.26270029799999));
#254649=CARTESIAN_POINT('Ctrl Pts',(-10.2746036380001,11.6,3.26270029799998));
#254650=CARTESIAN_POINT('Ctrl Pts',(-10.2724480790001,15.2,3.26124162799999));
#254651=CARTESIAN_POINT('Ctrl Pts',(-10.2724480790001,11.6,3.26124162799999));
#254652=CARTESIAN_POINT('Ctrl Pts',(-10.2702962470001,15.2,3.25978815099998));
#254653=CARTESIAN_POINT('Ctrl Pts',(-10.2702962470001,11.6,3.25978815099998));
#254654=CARTESIAN_POINT('Ctrl Pts',(-10.2681481560001,15.2,3.25833986599999));
#254655=CARTESIAN_POINT('Ctrl Pts',(-10.2681481560001,11.6,3.25833986599999));
#254656=CARTESIAN_POINT('Ctrl Pts',(-10.2660038210001,15.2,3.25689677199998));
#254657=CARTESIAN_POINT('Ctrl Pts',(-10.2660038210001,11.6,3.25689677199998));
#254658=CARTESIAN_POINT('Ctrl Pts',(-10.2638632570001,15.2,3.25545886899998));
#254659=CARTESIAN_POINT('Ctrl Pts',(-10.2638632570001,11.6,3.25545886899998));
#254660=CARTESIAN_POINT('Ctrl Pts',(-10.2617264780001,15.2,3.25402615399998));
#254661=CARTESIAN_POINT('Ctrl Pts',(-10.2617264780001,11.6,3.25402615399998));
#254662=CARTESIAN_POINT('Ctrl Pts',(-10.2595934990001,15.2,3.25259862599999));
#254663=CARTESIAN_POINT('Ctrl Pts',(-10.2595934990001,11.6,3.25259862599999));
#254664=CARTESIAN_POINT('Ctrl Pts',(-10.2574643340001,15.2,3.25117628699999));
#254665=CARTESIAN_POINT('Ctrl Pts',(-10.2574643340001,11.6,3.25117628699999));
#254666=CARTESIAN_POINT('Ctrl Pts',(-10.2553389990001,15.2,3.24975913199999));
#254667=CARTESIAN_POINT('Ctrl Pts',(-10.2553389990001,11.6,3.24975913199999));
#254668=CARTESIAN_POINT('Ctrl Pts',(-10.2532175070001,15.2,3.24834716199998));
#254669=CARTESIAN_POINT('Ctrl Pts',(-10.2532175070001,11.6,3.24834716199998));
#254670=CARTESIAN_POINT('Ctrl Pts',(-10.2510998750001,15.2,3.24694037699999));
#254671=CARTESIAN_POINT('Ctrl Pts',(-10.2510998750001,11.6,3.24694037699999));
#254672=CARTESIAN_POINT('Ctrl Pts',(-10.2489861160001,15.2,3.24553877299999));
#254673=CARTESIAN_POINT('Ctrl Pts',(-10.2489861160001,11.6,3.24553877299999));
#254674=CARTESIAN_POINT('Ctrl Pts',(-10.2468762450001,15.2,3.24414234899999));
#254675=CARTESIAN_POINT('Ctrl Pts',(-10.2468762450001,11.6,3.24414234899999));
#254676=CARTESIAN_POINT('Ctrl Pts',(-10.2447702790001,15.2,3.24275110699999));
#254677=CARTESIAN_POINT('Ctrl Pts',(-10.2447702790001,11.6,3.24275110699999));
#254678=CARTESIAN_POINT('Ctrl Pts',(-10.2426682300001,15.2,3.24136504299998));
#254679=CARTESIAN_POINT('Ctrl Pts',(-10.2426682300001,11.6,3.24136504299998));
#254680=CARTESIAN_POINT('Ctrl Pts',(-10.2405701150001,15.2,3.23998415799998));
#254681=CARTESIAN_POINT('Ctrl Pts',(-10.2405701150001,11.6,3.23998415799998));
#254682=CARTESIAN_POINT('Ctrl Pts',(-10.2384759480001,15.2,3.23860844899999));
#254683=CARTESIAN_POINT('Ctrl Pts',(-10.2384759480001,11.6,3.23860844899999));
#254684=CARTESIAN_POINT('Ctrl Pts',(-10.2363857440001,15.2,3.23723791499999));
#254685=CARTESIAN_POINT('Ctrl Pts',(-10.2363857440001,11.6,3.23723791499999));
#254686=CARTESIAN_POINT('Ctrl Pts',(-10.2342995200001,15.2,3.23587255499999));
#254687=CARTESIAN_POINT('Ctrl Pts',(-10.2342995200001,11.6,3.23587255499999));
#254688=CARTESIAN_POINT('Ctrl Pts',(-10.2322172890001,15.2,3.23451236899999));
#254689=CARTESIAN_POINT('Ctrl Pts',(-10.2322172890001,11.6,3.23451236899999));
#254690=CARTESIAN_POINT('Ctrl Pts',(-10.2301390670001,15.2,3.23315735299998));
#254691=CARTESIAN_POINT('Ctrl Pts',(-10.2301390670001,11.6,3.23315735299998));
#254692=CARTESIAN_POINT('Ctrl Pts',(-10.2280648700001,15.2,3.23180750899999));
#254693=CARTESIAN_POINT('Ctrl Pts',(-10.2280648700001,11.6,3.23180750899999));
#254694=CARTESIAN_POINT('Ctrl Pts',(-10.2259947110001,15.2,3.23046283299998));
#254695=CARTESIAN_POINT('Ctrl Pts',(-10.2259947110001,11.6,3.23046283299998));
#254696=CARTESIAN_POINT('Ctrl Pts',(-10.2239286080001,15.2,3.22912332499998));
#254697=CARTESIAN_POINT('Ctrl Pts',(-10.2239286080001,11.6,3.22912332499998));
#254698=CARTESIAN_POINT('Ctrl Pts',(-10.2218665760001,15.2,3.22778898299998));
#254699=CARTESIAN_POINT('Ctrl Pts',(-10.2218665760001,11.6,3.22778898299998));
#254700=CARTESIAN_POINT('Ctrl Pts',(-10.2198086280001,15.2,3.22645980699999));
#254701=CARTESIAN_POINT('Ctrl Pts',(-10.2198086280001,11.6,3.22645980699999));
#254702=CARTESIAN_POINT('Ctrl Pts',(-10.2177547810001,15.2,3.22513579499999));
#254703=CARTESIAN_POINT('Ctrl Pts',(-10.2177547810001,11.6,3.22513579499999));
#254704=CARTESIAN_POINT('Ctrl Pts',(-10.2157050510001,15.2,3.22381694599999));
#254705=CARTESIAN_POINT('Ctrl Pts',(-10.2157050510001,11.6,3.22381694599999));
#254706=CARTESIAN_POINT('Ctrl Pts',(-10.2136594530001,15.2,3.22250325599998));
#254707=CARTESIAN_POINT('Ctrl Pts',(-10.2136594530001,11.6,3.22250325599998));
#254708=CARTESIAN_POINT('Ctrl Pts',(-10.2116180040001,15.2,3.22119472699999));
#254709=CARTESIAN_POINT('Ctrl Pts',(-10.2116180040001,11.6,3.22119472699998));
#254710=CARTESIAN_POINT('Ctrl Pts',(-10.2095807170001,15.2,3.21989135599999));
#254711=CARTESIAN_POINT('Ctrl Pts',(-10.2095807170001,11.6,3.21989135599999));
#254712=CARTESIAN_POINT('Ctrl Pts',(-10.2075476090001,15.2,3.21859314199998));
#254713=CARTESIAN_POINT('Ctrl Pts',(-10.2075476090001,11.6,3.21859314199998));
#254714=CARTESIAN_POINT('Ctrl Pts',(-10.2055186960001,15.2,3.21730008499999));
#254715=CARTESIAN_POINT('Ctrl Pts',(-10.2055186960001,11.6,3.21730008499999));
#254716=CARTESIAN_POINT('Ctrl Pts',(-10.2034939940001,15.2,3.21601217999999));
#254717=CARTESIAN_POINT('Ctrl Pts',(-10.2034939940001,11.6,3.21601217999999));
#254718=CARTESIAN_POINT('Ctrl Pts',(-10.2014735180001,15.2,3.21472942799998));
#254719=CARTESIAN_POINT('Ctrl Pts',(-10.2014735180001,11.6,3.21472942799998));
#254720=CARTESIAN_POINT('Ctrl Pts',(-10.1994572830001,15.2,3.21345182899999));
#254721=CARTESIAN_POINT('Ctrl Pts',(-10.1994572830001,11.6,3.21345182899999));
#254722=CARTESIAN_POINT('Ctrl Pts',(-10.1974453070001,15.2,3.21217937799998));
#254723=CARTESIAN_POINT('Ctrl Pts',(-10.1974453070001,11.6,3.21217937799998));
#254724=CARTESIAN_POINT('Ctrl Pts',(-10.1954376050001,15.2,3.21091207499999));
#254725=CARTESIAN_POINT('Ctrl Pts',(-10.1954376050001,11.6,3.21091207499998));
#254726=CARTESIAN_POINT('Ctrl Pts',(-10.1934341930001,15.2,3.20964991899999));
#254727=CARTESIAN_POINT('Ctrl Pts',(-10.1934341930001,11.6,3.20964991899999));
#254728=CARTESIAN_POINT('Ctrl Pts',(-10.1914350860001,15.2,3.20839290799999));
#254729=CARTESIAN_POINT('Ctrl Pts',(-10.1914350860001,11.6,3.20839290799999));
#254730=CARTESIAN_POINT('Ctrl Pts',(-10.1894403010001,15.2,3.20714103999999));
#254731=CARTESIAN_POINT('Ctrl Pts',(-10.1894403010001,11.6,3.20714103999999));
#254732=CARTESIAN_POINT('Ctrl Pts',(-10.1874498540001,15.2,3.20589431399998));
#254733=CARTESIAN_POINT('Ctrl Pts',(-10.1874498540001,11.6,3.20589431399998));
#254734=CARTESIAN_POINT('Ctrl Pts',(-10.1854637630001,15.2,3.20465272999999));
#254735=CARTESIAN_POINT('Ctrl Pts',(-10.1854637630001,11.6,3.20465272999999));
#254736=CARTESIAN_POINT('Ctrl Pts',(-10.1834820400001,15.2,3.20341628299998));
#254737=CARTESIAN_POINT('Ctrl Pts',(-10.1834820400001,11.6,3.20341628299998));
#254738=CARTESIAN_POINT('Ctrl Pts',(-10.1815047050001,15.2,3.20218497399999));
#254739=CARTESIAN_POINT('Ctrl Pts',(-10.1815047050001,11.6,3.20218497399999));
#254740=CARTESIAN_POINT('Ctrl Pts',(-10.1795317740001,15.2,3.20095879999998));
#254741=CARTESIAN_POINT('Ctrl Pts',(-10.1795317740001,11.6,3.20095879999998));
#254742=CARTESIAN_POINT('Ctrl Pts',(-10.1775632610001,15.2,3.19973776199999));
#254743=CARTESIAN_POINT('Ctrl Pts',(-10.1775632610001,11.6,3.19973776199999));
#254744=CARTESIAN_POINT('Ctrl Pts',(-10.1755991840001,15.2,3.19852185499998));
#254745=CARTESIAN_POINT('Ctrl Pts',(-10.1755991840001,11.6,3.19852185499998));
#254746=CARTESIAN_POINT('Ctrl Pts',(-10.1736395590001,15.2,3.19731107799999));
#254747=CARTESIAN_POINT('Ctrl Pts',(-10.1736395590001,11.6,3.19731107799999));
#254748=CARTESIAN_POINT('Ctrl Pts',(-10.1716844030001,15.2,3.19610542999998));
#254749=CARTESIAN_POINT('Ctrl Pts',(-10.1716844030001,11.6,3.19610542999998));
#254750=CARTESIAN_POINT('Ctrl Pts',(-10.1697337330001,15.2,3.19490490899998));
#254751=CARTESIAN_POINT('Ctrl Pts',(-10.1697337330001,11.6,3.19490490899998));
#254752=CARTESIAN_POINT('Ctrl Pts',(-10.1677875630001,15.2,3.19370951499998));
#254753=CARTESIAN_POINT('Ctrl Pts',(-10.1677875630001,11.6,3.19370951499998));
#254754=CARTESIAN_POINT('Ctrl Pts',(-10.1658459140001,15.2,3.19251924299999));
#254755=CARTESIAN_POINT('Ctrl Pts',(-10.1658459140001,11.6,3.19251924299999));
#254756=CARTESIAN_POINT('Ctrl Pts',(-10.1639087980001,15.2,3.19133409299998));
#254757=CARTESIAN_POINT('Ctrl Pts',(-10.1639087980001,11.6,3.19133409299998));
#254758=CARTESIAN_POINT('Ctrl Pts',(-10.1619762350001,15.2,3.19015406399998));
#254759=CARTESIAN_POINT('Ctrl Pts',(-10.1619762350001,11.6,3.19015406399998));
#254760=CARTESIAN_POINT('Ctrl Pts',(-10.1600482390001,15.2,3.18897915399998));
#254761=CARTESIAN_POINT('Ctrl Pts',(-10.1600482390001,11.6,3.18897915399998));
#254762=CARTESIAN_POINT('Ctrl Pts',(-10.1581248300001,15.2,3.18780935899999));
#254763=CARTESIAN_POINT('Ctrl Pts',(-10.1581248300001,11.6,3.18780935899999));
#254764=CARTESIAN_POINT('Ctrl Pts',(-10.1562060230001,15.2,3.18664467999999));
#254765=CARTESIAN_POINT('Ctrl Pts',(-10.1562060230001,11.6,3.18664467999999));
#254766=CARTESIAN_POINT('Ctrl Pts',(-10.1542918360001,15.2,3.18548511399998));
#254767=CARTESIAN_POINT('Ctrl Pts',(-10.1542918360001,11.6,3.18548511399998));
#254768=CARTESIAN_POINT('Ctrl Pts',(-10.1523822840001,15.2,3.18433065799999));
#254769=CARTESIAN_POINT('Ctrl Pts',(-10.1523822840001,11.6,3.18433065799999));
#254770=CARTESIAN_POINT('Ctrl Pts',(-10.1504773870001,15.2,3.18318131199998));
#254771=CARTESIAN_POINT('Ctrl Pts',(-10.1504773870001,11.6,3.18318131199998));
#254772=CARTESIAN_POINT('Ctrl Pts',(-10.1485771590001,15.2,3.18203707299999));
#254773=CARTESIAN_POINT('Ctrl Pts',(-10.1485771590001,11.6,3.18203707299999));
#254774=CARTESIAN_POINT('Ctrl Pts',(-10.1466816200001,15.2,3.18089793999999));
#254775=CARTESIAN_POINT('Ctrl Pts',(-10.1466816200001,11.6,3.18089793999999));
#254776=CARTESIAN_POINT('Ctrl Pts',(-10.1447907840001,15.2,3.17976390999998));
#254777=CARTESIAN_POINT('Ctrl Pts',(-10.1447907840001,11.6,3.17976390999998));
#254778=CARTESIAN_POINT('Ctrl Pts',(-10.1429046700001,15.2,3.17863498199999));
#254779=CARTESIAN_POINT('Ctrl Pts',(-10.1429046700001,11.6,3.17863498199999));
#254780=CARTESIAN_POINT('Ctrl Pts',(-10.1410232970001,15.2,3.17751115299998));
#254781=CARTESIAN_POINT('Ctrl Pts',(-10.1410232970001,11.6,3.17751115299998));
#254782=CARTESIAN_POINT('Ctrl Pts',(-10.1391466790001,15.2,3.17639242199999));
#254783=CARTESIAN_POINT('Ctrl Pts',(-10.1391466790001,11.6,3.17639242199998));
#254784=CARTESIAN_POINT('Ctrl Pts',(-10.1372748360001,15.2,3.17527878599999));
#254785=CARTESIAN_POINT('Ctrl Pts',(-10.1372748360001,11.6,3.17527878599999));
#254786=CARTESIAN_POINT('Ctrl Pts',(-10.1354077850001,15.2,3.17417024399998));
#254787=CARTESIAN_POINT('Ctrl Pts',(-10.1354077850001,11.6,3.17417024399998));
#254788=CARTESIAN_POINT('Ctrl Pts',(-10.1335455420001,15.2,3.17306679399999));
#254789=CARTESIAN_POINT('Ctrl Pts',(-10.1335455420001,11.6,3.17306679399999));
#254790=CARTESIAN_POINT('Ctrl Pts',(-10.1316881250001,15.2,3.17196843299998));
#254791=CARTESIAN_POINT('Ctrl Pts',(-10.1316881250001,11.6,3.17196843299998));
#254792=CARTESIAN_POINT('Ctrl Pts',(-10.1298355530001,15.2,3.17087515999999));
#254793=CARTESIAN_POINT('Ctrl Pts',(-10.1298355530001,11.6,3.17087515999999));
#254794=CARTESIAN_POINT('Ctrl Pts',(-10.1279878430001,15.2,3.16978697199998));
#254795=CARTESIAN_POINT('Ctrl Pts',(-10.1279878430001,11.6,3.16978697199998));
#254796=CARTESIAN_POINT('Ctrl Pts',(-10.1261450120001,15.2,3.16870386699998));
#254797=CARTESIAN_POINT('Ctrl Pts',(-10.1261450120001,11.6,3.16870386699998));
#254798=CARTESIAN_POINT('Ctrl Pts',(-10.1243070780001,15.2,3.16762584299998));
#254799=CARTESIAN_POINT('Ctrl Pts',(-10.1243070780001,11.6,3.16762584299998));
#254800=CARTESIAN_POINT('Ctrl Pts',(-10.1224740600001,15.2,3.16655289799999));
#254801=CARTESIAN_POINT('Ctrl Pts',(-10.1224740600001,11.6,3.16655289799999));
#254802=CARTESIAN_POINT('Ctrl Pts',(-10.1206459750001,15.2,3.16548503099998));
#254803=CARTESIAN_POINT('Ctrl Pts',(-10.1206459750001,11.6,3.16548503099998));
#254804=CARTESIAN_POINT('Ctrl Pts',(-10.1188228400001,15.2,3.16442223699998));
#254805=CARTESIAN_POINT('Ctrl Pts',(-10.1188228400001,11.6,3.16442223699998));
#254806=CARTESIAN_POINT('Ctrl Pts',(-10.1170046750001,15.2,3.16336451599999));
#254807=CARTESIAN_POINT('Ctrl Pts',(-10.1170046750001,11.6,3.16336451599999));
#254808=CARTESIAN_POINT('Ctrl Pts',(-10.1151914960001,15.2,3.16231186599998));
#254809=CARTESIAN_POINT('Ctrl Pts',(-10.1151914960001,11.6,3.16231186599998));
#254810=CARTESIAN_POINT('Ctrl Pts',(-10.1133833240001,15.2,3.16126428399999));
#254811=CARTESIAN_POINT('Ctrl Pts',(-10.1133833240001,11.6,3.16126428399999));
#254812=CARTESIAN_POINT('Ctrl Pts',(-10.1115801740001,15.2,3.16022176699998));
#254813=CARTESIAN_POINT('Ctrl Pts',(-10.1115801740001,11.6,3.16022176699998));
#254814=CARTESIAN_POINT('Ctrl Pts',(-10.1097820650001,15.2,3.15918431399999));
#254815=CARTESIAN_POINT('Ctrl Pts',(-10.1097820650001,11.6,3.15918431399999));
#254816=CARTESIAN_POINT('Ctrl Pts',(-10.1079890170001,15.2,3.15815192199998));
#254817=CARTESIAN_POINT('Ctrl Pts',(-10.1079890170001,11.6,3.15815192199998));
#254818=CARTESIAN_POINT('Ctrl Pts',(-10.1062010460001,15.2,3.15712458799998));
#254819=CARTESIAN_POINT('Ctrl Pts',(-10.1062010460001,11.6,3.15712458799998));
#254820=CARTESIAN_POINT('Ctrl Pts',(-10.1044181730001,15.2,3.15610231199998));
#254821=CARTESIAN_POINT('Ctrl Pts',(-10.1044181730001,11.6,3.15610231199998));
#254822=CARTESIAN_POINT('Ctrl Pts',(-10.1026404140001,15.2,3.15508508899998));
#254823=CARTESIAN_POINT('Ctrl Pts',(-10.1026404140001,11.6,3.15508508899998));
#254824=CARTESIAN_POINT('Ctrl Pts',(-10.1008677890001,15.2,3.15407291799998));
#254825=CARTESIAN_POINT('Ctrl Pts',(-10.1008677890001,11.6,3.15407291799998));
#254826=CARTESIAN_POINT('Ctrl Pts',(-10.0991003160001,15.2,3.15306579799999));
#254827=CARTESIAN_POINT('Ctrl Pts',(-10.0991003160001,11.6,3.15306579799999));
#254828=CARTESIAN_POINT('Ctrl Pts',(-10.0973380130001,15.2,3.15206372299999));
#254829=CARTESIAN_POINT('Ctrl Pts',(-10.0973380130001,11.6,3.15206372299999));
#254830=CARTESIAN_POINT('Ctrl Pts',(-10.0955809000001,15.2,3.15106669399999));
#254831=CARTESIAN_POINT('Ctrl Pts',(-10.0955809000001,11.6,3.15106669399999));
#254832=CARTESIAN_POINT('Ctrl Pts',(-10.0938289960001,15.2,3.15007470699998));
#254833=CARTESIAN_POINT('Ctrl Pts',(-10.0938289960001,11.6,3.15007470699998));
#254834=CARTESIAN_POINT('Ctrl Pts',(-10.0920823180001,15.2,3.14908775899998));
#254835=CARTESIAN_POINT('Ctrl Pts',(-10.0920823180001,11.6,3.14908775899998));
#254836=CARTESIAN_POINT('Ctrl Pts',(-10.0903408870001,15.2,3.14810584799999));
#254837=CARTESIAN_POINT('Ctrl Pts',(-10.0903408870001,11.6,3.14810584799999));
#254838=CARTESIAN_POINT('Ctrl Pts',(-10.0886047200001,15.2,3.14712897299999));
#254839=CARTESIAN_POINT('Ctrl Pts',(-10.0886047200001,11.6,3.14712897299999));
#254840=CARTESIAN_POINT('Ctrl Pts',(-10.0868738370001,15.2,3.14615712899998));
#254841=CARTESIAN_POINT('Ctrl Pts',(-10.0868738370001,11.6,3.14615712899998));
#254842=CARTESIAN_POINT('Ctrl Pts',(-10.0851482570001,15.2,3.14519031499999));
#254843=CARTESIAN_POINT('Ctrl Pts',(-10.0851482570001,11.6,3.14519031499999));
#254844=CARTESIAN_POINT('Ctrl Pts',(-10.0834279990001,15.2,3.14422852799999));
#254845=CARTESIAN_POINT('Ctrl Pts',(-10.0834279990001,11.6,3.14422852799999));
#254846=CARTESIAN_POINT('Ctrl Pts',(-10.0817130830001,15.2,3.14327176499998));
#254847=CARTESIAN_POINT('Ctrl Pts',(-10.0817130830001,11.6,3.14327176499998));
#254848=CARTESIAN_POINT('Ctrl Pts',(-10.0800035270001,15.2,3.14232002499998));
#254849=CARTESIAN_POINT('Ctrl Pts',(-10.0800035270001,11.6,3.14232002499998));
#254850=CARTESIAN_POINT('Ctrl Pts',(-10.0782993510001,15.2,3.14137330299998));
#254851=CARTESIAN_POINT('Ctrl Pts',(-10.0782993510001,11.6,3.14137330299998));
#254852=CARTESIAN_POINT('Ctrl Pts',(-10.0766005740001,15.2,3.14043159799999));
#254853=CARTESIAN_POINT('Ctrl Pts',(-10.0766005740001,11.6,3.14043159799999));
#254854=CARTESIAN_POINT('Ctrl Pts',(-10.0749072160001,15.2,3.13949490699999));
#254855=CARTESIAN_POINT('Ctrl Pts',(-10.0749072160001,11.6,3.13949490699999));
#254856=CARTESIAN_POINT('Ctrl Pts',(-10.0732192960001,15.2,3.13856322799998));
#254857=CARTESIAN_POINT('Ctrl Pts',(-10.0732192960001,11.6,3.13856322799998));
#254858=CARTESIAN_POINT('Ctrl Pts',(-10.0715368340001,15.2,3.13763655699999));
#254859=CARTESIAN_POINT('Ctrl Pts',(-10.0715368340001,11.6,3.13763655699999));
#254860=CARTESIAN_POINT('Ctrl Pts',(-10.0698598500001,15.2,3.13671489099999));
#254861=CARTESIAN_POINT('Ctrl Pts',(-10.0698598500001,11.6,3.13671489099998));
#254862=CARTESIAN_POINT('Ctrl Pts',(-10.0681883620001,15.2,3.13579822799999));
#254863=CARTESIAN_POINT('Ctrl Pts',(-10.0681883620001,11.6,3.13579822799999));
#254864=CARTESIAN_POINT('Ctrl Pts',(-10.0665223920001,15.2,3.13488656499998));
#254865=CARTESIAN_POINT('Ctrl Pts',(-10.0665223920001,11.6,3.13488656499998));
#254866=CARTESIAN_POINT('Ctrl Pts',(-10.0648619590001,15.2,3.13397989999999));
#254867=CARTESIAN_POINT('Ctrl Pts',(-10.0648619590001,11.6,3.13397989999999));
#254868=CARTESIAN_POINT('Ctrl Pts',(-10.0632070820001,15.2,3.13307822999998));
#254869=CARTESIAN_POINT('Ctrl Pts',(-10.0632070820001,11.6,3.13307822999998));
#254870=CARTESIAN_POINT('Ctrl Pts',(-10.0615577810001,15.2,3.13218154999999));
#254871=CARTESIAN_POINT('Ctrl Pts',(-10.0615577810001,11.6,3.13218154999999));
#254872=CARTESIAN_POINT('Ctrl Pts',(-10.0599140780001,15.2,3.13128986099999));
#254873=CARTESIAN_POINT('Ctrl Pts',(-10.0599140780001,11.6,3.13128986099999));
#254874=CARTESIAN_POINT('Ctrl Pts',(-10.0582759920001,15.2,3.13040315599999));
#254875=CARTESIAN_POINT('Ctrl Pts',(-10.0582759920001,11.6,3.13040315599999));
#254876=CARTESIAN_POINT('Ctrl Pts',(-10.0566435420001,15.2,3.12952143599999));
#254877=CARTESIAN_POINT('Ctrl Pts',(-10.0566435420001,11.6,3.12952143599999));
#254878=CARTESIAN_POINT('Ctrl Pts',(-10.0550167500001,15.2,3.12864469399998));
#254879=CARTESIAN_POINT('Ctrl Pts',(-10.0550167500001,11.6,3.12864469399998));
#254880=CARTESIAN_POINT('Ctrl Pts',(-10.0533956360001,15.2,3.12777292999999));
#254881=CARTESIAN_POINT('Ctrl Pts',(-10.0533956360001,11.6,3.12777292999999));
#254882=CARTESIAN_POINT('Ctrl Pts',(-10.0517802200001,15.2,3.12690613999998));
#254883=CARTESIAN_POINT('Ctrl Pts',(-10.0517802200001,11.6,3.12690613999998));
#254884=CARTESIAN_POINT('Ctrl Pts',(-10.0501705220001,15.2,3.12604432099998));
#254885=CARTESIAN_POINT('Ctrl Pts',(-10.0501705220001,11.6,3.12604432099998));
#254886=CARTESIAN_POINT('Ctrl Pts',(-10.0485665630001,15.2,3.12518747099999));
#254887=CARTESIAN_POINT('Ctrl Pts',(-10.0485665630001,11.6,3.12518747099999));
#254888=CARTESIAN_POINT('Ctrl Pts',(-10.0469683640001,15.2,3.12433558599999));
#254889=CARTESIAN_POINT('Ctrl Pts',(-10.0469683640001,11.6,3.12433558599999));
#254890=CARTESIAN_POINT('Ctrl Pts',(-10.0453759450001,15.2,3.12348866199999));
#254891=CARTESIAN_POINT('Ctrl Pts',(-10.0453759450001,11.6,3.12348866199999));
#254892=CARTESIAN_POINT('Ctrl Pts',(-10.0437893290001,15.2,3.12264669699999));
#254893=CARTESIAN_POINT('Ctrl Pts',(-10.0437893290001,11.6,3.12264669699999));
#254894=CARTESIAN_POINT('Ctrl Pts',(-10.0422085330001,15.2,3.12180968699998));
#254895=CARTESIAN_POINT('Ctrl Pts',(-10.0422085330001,11.6,3.12180968699998));
#254896=CARTESIAN_POINT('Ctrl Pts',(-10.0406335810001,15.2,3.12097763199999));
#254897=CARTESIAN_POINT('Ctrl Pts',(-10.0406335810001,11.6,3.12097763199999));
#254898=CARTESIAN_POINT('Ctrl Pts',(-10.0390644920001,15.2,3.12015052399998));
#254899=CARTESIAN_POINT('Ctrl Pts',(-10.0390644920001,11.6,3.12015052399998));
#254900=CARTESIAN_POINT('Ctrl Pts',(-10.0375012890001,15.2,3.11932836399999));
#254901=CARTESIAN_POINT('Ctrl Pts',(-10.0375012890001,11.6,3.11932836399999));
#254902=CARTESIAN_POINT('Ctrl Pts',(-10.0359439910001,15.2,3.11851114499999));
#254903=CARTESIAN_POINT('Ctrl Pts',(-10.0359439910001,11.6,3.11851114499999));
#254904=CARTESIAN_POINT('Ctrl Pts',(-10.0343926210001,15.2,3.11769886699999));
#254905=CARTESIAN_POINT('Ctrl Pts',(-10.0343926210001,11.6,3.11769886699999));
#254906=CARTESIAN_POINT('Ctrl Pts',(-10.0328472000001,15.2,3.11689152499999));
#254907=CARTESIAN_POINT('Ctrl Pts',(-10.0328472000001,11.6,3.11689152499999));
#254908=CARTESIAN_POINT('Ctrl Pts',(-10.0313077490001,15.2,3.11608911699999));
#254909=CARTESIAN_POINT('Ctrl Pts',(-10.0313077490001,11.6,3.11608911699999));
#254910=CARTESIAN_POINT('Ctrl Pts',(-10.0297742890001,15.2,3.11529163799998));
#254911=CARTESIAN_POINT('Ctrl Pts',(-10.0297742890001,11.6,3.11529163799998));
#254912=CARTESIAN_POINT('Ctrl Pts',(-10.0282468420001,15.2,3.11449908599998));
#254913=CARTESIAN_POINT('Ctrl Pts',(-10.0282468420001,11.6,3.11449908599998));
#254914=CARTESIAN_POINT('Ctrl Pts',(-10.0267254290001,15.2,3.11371145699999));
#254915=CARTESIAN_POINT('Ctrl Pts',(-10.0267254290001,11.6,3.11371145699999));
#254916=CARTESIAN_POINT('Ctrl Pts',(-10.0252100730001,15.2,3.11292874799998));
#254917=CARTESIAN_POINT('Ctrl Pts',(-10.0252100730001,11.6,3.11292874799998));
#254918=CARTESIAN_POINT('Ctrl Pts',(-10.0237007950001,15.2,3.11215095499998));
#254919=CARTESIAN_POINT('Ctrl Pts',(-10.0237007950001,11.6,3.11215095499998));
#254920=CARTESIAN_POINT('Ctrl Pts',(-10.0221976160001,15.2,3.11137807499998));
#254921=CARTESIAN_POINT('Ctrl Pts',(-10.0221976160001,11.6,3.11137807499998));
#254922=CARTESIAN_POINT('Ctrl Pts',(-10.0207005590001,15.2,3.11061010399998));
#254923=CARTESIAN_POINT('Ctrl Pts',(-10.0207005590001,11.6,3.11061010399998));
#254924=CARTESIAN_POINT('Ctrl Pts',(-10.0192096460001,15.2,3.10984703899998));
#254925=CARTESIAN_POINT('Ctrl Pts',(-10.0192096460001,11.6,3.10984703899998));
#254926=CARTESIAN_POINT('Ctrl Pts',(-10.0177248990001,15.2,3.10908887699998));
#254927=CARTESIAN_POINT('Ctrl Pts',(-10.0177248990001,11.6,3.10908887699998));
#254928=CARTESIAN_POINT('Ctrl Pts',(-10.0162463390001,15.2,3.10833561299999));
#254929=CARTESIAN_POINT('Ctrl Pts',(-10.0162463390001,11.6,3.10833561299999));
#254930=CARTESIAN_POINT('Ctrl Pts',(-10.0147739910001,15.2,3.10758724499999));
#254931=CARTESIAN_POINT('Ctrl Pts',(-10.0147739910001,11.6,3.10758724499998));
#254932=CARTESIAN_POINT('Ctrl Pts',(-10.0133078740001,15.2,3.10684376799998));
#254933=CARTESIAN_POINT('Ctrl Pts',(-10.0133078740001,11.6,3.10684376799998));
#254934=CARTESIAN_POINT('Ctrl Pts',(-10.0118480130001,15.2,3.10610517999999));
#254935=CARTESIAN_POINT('Ctrl Pts',(-10.0118480130001,11.6,3.10610517999999));
#254936=CARTESIAN_POINT('Ctrl Pts',(-10.0103944280001,15.2,3.10537147599998));
#254937=CARTESIAN_POINT('Ctrl Pts',(-10.0103944280001,11.6,3.10537147599998));
#254938=CARTESIAN_POINT('Ctrl Pts',(-10.0089471450001,15.2,3.10464265199998));
#254939=CARTESIAN_POINT('Ctrl Pts',(-10.0089471450001,11.6,3.10464265199998));
#254940=CARTESIAN_POINT('Ctrl Pts',(-10.0075061830001,15.2,3.10391870599998));
#254941=CARTESIAN_POINT('Ctrl Pts',(-10.0075061830001,11.6,3.10391870599998));
#254942=CARTESIAN_POINT('Ctrl Pts',(-10.0060715670001,15.2,3.10319963199999));
#254943=CARTESIAN_POINT('Ctrl Pts',(-10.0060715670001,11.6,3.10319963199999));
#254944=CARTESIAN_POINT('Ctrl Pts',(-10.0046433200001,15.2,3.10248542899998));
#254945=CARTESIAN_POINT('Ctrl Pts',(-10.0046433200001,11.6,3.10248542899998));
#254946=CARTESIAN_POINT('Ctrl Pts',(-10.0032214630001,15.2,3.10177608999999));
#254947=CARTESIAN_POINT('Ctrl Pts',(-10.0032214630001,11.6,3.10177608999999));
#254948=CARTESIAN_POINT('Ctrl Pts',(-10.0018060210001,15.2,3.10107161299998));
#254949=CARTESIAN_POINT('Ctrl Pts',(-10.0018060210001,11.6,3.10107161299998));
#254950=CARTESIAN_POINT('Ctrl Pts',(-10.0003970160001,15.2,3.10037199499998));
#254951=CARTESIAN_POINT('Ctrl Pts',(-10.0003970160001,11.6,3.10037199499998));
#254952=CARTESIAN_POINT('Ctrl Pts',(-9.99899447200006,15.2,3.09967723099999));
#254953=CARTESIAN_POINT('Ctrl Pts',(-9.99899447200006,11.6,3.09967723099999));
#254954=CARTESIAN_POINT('Ctrl Pts',(-9.99759841200006,15.2,3.09898731699998));
#254955=CARTESIAN_POINT('Ctrl Pts',(-9.99759841200006,11.6,3.09898731699998));
#254956=CARTESIAN_POINT('Ctrl Pts',(-9.99620885900006,15.2,3.09830224999998));
#254957=CARTESIAN_POINT('Ctrl Pts',(-9.99620885900006,11.6,3.09830224999998));
#254958=CARTESIAN_POINT('Ctrl Pts',(-9.99482583700006,15.2,3.09762202399998));
#254959=CARTESIAN_POINT('Ctrl Pts',(-9.99482583700006,11.6,3.09762202399998));
#254960=CARTESIAN_POINT('Ctrl Pts',(-9.99344936900006,15.2,3.09694663699998));
#254961=CARTESIAN_POINT('Ctrl Pts',(-9.99344936900006,11.6,3.09694663699998));
#254962=CARTESIAN_POINT('Ctrl Pts',(-9.99207947800006,15.2,3.09627608399998));
#254963=CARTESIAN_POINT('Ctrl Pts',(-9.99207947800006,11.6,3.09627608399998));
#254964=CARTESIAN_POINT('Ctrl Pts',(-9.99071619000006,15.2,3.09561036199998));
#254965=CARTESIAN_POINT('Ctrl Pts',(-9.99071619000006,11.6,3.09561036199998));
#254966=CARTESIAN_POINT('Ctrl Pts',(-9.98935952600006,15.2,3.09494946599998));
#254967=CARTESIAN_POINT('Ctrl Pts',(-9.98935952600006,11.6,3.09494946599998));
#254968=CARTESIAN_POINT('Ctrl Pts',(-9.98800951200005,15.2,3.09429339199998));
#254969=CARTESIAN_POINT('Ctrl Pts',(-9.98800951200005,11.6,3.09429339199998));
#254970=CARTESIAN_POINT('Ctrl Pts',(-9.98666617200006,15.2,3.09364213599999));
#254971=CARTESIAN_POINT('Ctrl Pts',(-9.98666617200006,11.6,3.09364213599999));
#254972=CARTESIAN_POINT('Ctrl Pts',(-9.98532952900005,15.2,3.09299569299998));
#254973=CARTESIAN_POINT('Ctrl Pts',(-9.98532952900005,11.6,3.09299569299998));
#254974=CARTESIAN_POINT('Ctrl Pts',(-9.98399960800005,15.2,3.09235406099998));
#254975=CARTESIAN_POINT('Ctrl Pts',(-9.98399960800005,11.6,3.09235406099998));
#254976=CARTESIAN_POINT('Ctrl Pts',(-9.98267643200006,15.2,3.09171723299999));
#254977=CARTESIAN_POINT('Ctrl Pts',(-9.98267643200006,11.6,3.09171723299999));
#254978=CARTESIAN_POINT('Ctrl Pts',(-9.98136002800005,15.2,3.09108520699999));
#254979=CARTESIAN_POINT('Ctrl Pts',(-9.98136002800005,11.6,3.09108520699999));
#254980=CARTESIAN_POINT('Ctrl Pts',(-9.98005041800005,15.2,3.09045797699999));
#254981=CARTESIAN_POINT('Ctrl Pts',(-9.98005041800005,11.6,3.09045797699999));
#254982=CARTESIAN_POINT('Ctrl Pts',(-9.97874762800006,15.2,3.08983553999998));
#254983=CARTESIAN_POINT('Ctrl Pts',(-9.97874762800006,11.6,3.08983553999998));
#254984=CARTESIAN_POINT('Ctrl Pts',(-9.97745168200005,15.2,3.08921789099998));
#254985=CARTESIAN_POINT('Ctrl Pts',(-9.97745168200005,11.6,3.08921789099998));
#254986=CARTESIAN_POINT('Ctrl Pts',(-9.97616260500006,15.2,3.08860502599998));
#254987=CARTESIAN_POINT('Ctrl Pts',(-9.97616260500006,11.6,3.08860502599998));
#254988=CARTESIAN_POINT('Ctrl Pts',(-9.97488042200006,15.2,3.08799693999998));
#254989=CARTESIAN_POINT('Ctrl Pts',(-9.97488042200006,11.6,3.08799693999998));
#254990=CARTESIAN_POINT('Ctrl Pts',(-9.97360515900005,15.2,3.08739362899999));
#254991=CARTESIAN_POINT('Ctrl Pts',(-9.97360515900005,11.6,3.08739362899999));
#254992=CARTESIAN_POINT('Ctrl Pts',(-9.97233683900006,15.2,3.08679508799998));
#254993=CARTESIAN_POINT('Ctrl Pts',(-9.97233683900006,11.6,3.08679508799998));
#254994=CARTESIAN_POINT('Ctrl Pts',(-9.97107548900006,15.2,3.08620131299998));
#254995=CARTESIAN_POINT('Ctrl Pts',(-9.97107548900006,11.6,3.08620131299998));
#254996=CARTESIAN_POINT('Ctrl Pts',(-9.96982113400006,15.2,3.08561229999999));
#254997=CARTESIAN_POINT('Ctrl Pts',(-9.96982113400006,11.6,3.08561229999999));
#254998=CARTESIAN_POINT('Ctrl Pts',(-9.96857379800005,15.2,3.08502804299999));
#254999=CARTESIAN_POINT('Ctrl Pts',(-9.96857379800005,11.6,3.08502804299999));
#255000=CARTESIAN_POINT('Ctrl Pts',(-9.96733350800006,15.2,3.08444853899999));
#255001=CARTESIAN_POINT('Ctrl Pts',(-9.96733350800006,11.6,3.08444853899999));
#255002=CARTESIAN_POINT('Ctrl Pts',(-9.96610029100006,15.2,3.08387378199999));
#255003=CARTESIAN_POINT('Ctrl Pts',(-9.96610029100006,11.6,3.08387378199999));
#255004=CARTESIAN_POINT('Ctrl Pts',(-9.96487416900005,15.2,3.08330376799999));
#255005=CARTESIAN_POINT('Ctrl Pts',(-9.96487416900005,11.6,3.08330376799999));
#255006=CARTESIAN_POINT('Ctrl Pts',(-9.96365517100006,15.2,3.08273849199999));
#255007=CARTESIAN_POINT('Ctrl Pts',(-9.96365517100006,11.6,3.08273849199999));
#255008=CARTESIAN_POINT('Ctrl Pts',(-9.96244332100006,15.2,3.08217794899999));
#255009=CARTESIAN_POINT('Ctrl Pts',(-9.96244332100006,11.6,3.08217794899999));
#255010=CARTESIAN_POINT('Ctrl Pts',(-9.96123864600006,15.2,3.08162213599999));
#255011=CARTESIAN_POINT('Ctrl Pts',(-9.96123864600006,11.6,3.08162213599999));
#255012=CARTESIAN_POINT('Ctrl Pts',(-9.96004117300006,15.2,3.08107104599999));
#255013=CARTESIAN_POINT('Ctrl Pts',(-9.96004117300006,11.6,3.08107104599999));
#255014=CARTESIAN_POINT('Ctrl Pts',(-9.95885092700006,15.2,3.08052467499999));
#255015=CARTESIAN_POINT('Ctrl Pts',(-9.95885092700006,11.6,3.08052467499999));
#255016=CARTESIAN_POINT('Ctrl Pts',(-9.95766793500006,15.2,3.07998301799999));
#255017=CARTESIAN_POINT('Ctrl Pts',(-9.95766793500006,11.6,3.07998301799999));
#255018=CARTESIAN_POINT('Ctrl Pts',(-9.95649222300005,15.2,3.07944606999998));
#255019=CARTESIAN_POINT('Ctrl Pts',(-9.95649222300005,11.6,3.07944606999998));
#255020=CARTESIAN_POINT('Ctrl Pts',(-9.95532381800006,15.2,3.07891382599998));
#255021=CARTESIAN_POINT('Ctrl Pts',(-9.95532381800006,11.6,3.07891382599998));
#255022=CARTESIAN_POINT('Ctrl Pts',(-9.95416274700006,15.2,3.07838628199999));
#255023=CARTESIAN_POINT('Ctrl Pts',(-9.95416274700006,11.6,3.07838628199998));
#255024=CARTESIAN_POINT('Ctrl Pts',(-9.95300903700005,15.2,3.07786343099998));
#255025=CARTESIAN_POINT('Ctrl Pts',(-9.95300903700005,11.6,3.07786343099998));
#255026=CARTESIAN_POINT('Ctrl Pts',(-9.95186271400006,15.2,3.07734527099999));
#255027=CARTESIAN_POINT('Ctrl Pts',(-9.95186271400006,11.6,3.07734527099999));
#255028=CARTESIAN_POINT('Ctrl Pts',(-9.95072380600006,15.2,3.07683179399999));
#255029=CARTESIAN_POINT('Ctrl Pts',(-9.95072380600006,11.6,3.07683179399999));
#255030=CARTESIAN_POINT('Ctrl Pts',(-9.94959234000006,15.2,3.07632299599998));
#255031=CARTESIAN_POINT('Ctrl Pts',(-9.94959234000006,11.6,3.07632299599998));
#255032=CARTESIAN_POINT('Ctrl Pts',(-9.94846834300006,15.2,3.07581887199999));
#255033=CARTESIAN_POINT('Ctrl Pts',(-9.94846834300006,11.6,3.07581887199999));
#255034=CARTESIAN_POINT('Ctrl Pts',(-9.94735184300006,15.2,3.07531941599999));
#255035=CARTESIAN_POINT('Ctrl Pts',(-9.94735184300006,11.6,3.07531941599999));
#255036=CARTESIAN_POINT('Ctrl Pts',(-9.94624286800006,15.2,3.07482462399999));
#255037=CARTESIAN_POINT('Ctrl Pts',(-9.94624286800006,11.6,3.07482462399999));
#255038=CARTESIAN_POINT('Ctrl Pts',(-9.94514144400006,15.2,3.07433448899998));
#255039=CARTESIAN_POINT('Ctrl Pts',(-9.94514144400006,11.6,3.07433448899998));
#255040=CARTESIAN_POINT('Ctrl Pts',(-9.94404760100006,15.2,3.07384900799998));
#255041=CARTESIAN_POINT('Ctrl Pts',(-9.94404760100006,11.6,3.07384900799998));
#255042=CARTESIAN_POINT('Ctrl Pts',(-9.94296136500006,15.2,3.07336817399998));
#255043=CARTESIAN_POINT('Ctrl Pts',(-9.94296136500006,11.6,3.07336817399998));
#255044=CARTESIAN_POINT('Ctrl Pts',(-9.94188276500006,15.2,3.07289198099999));
#255045=CARTESIAN_POINT('Ctrl Pts',(-9.94188276500006,11.6,3.07289198099999));
#255046=CARTESIAN_POINT('Ctrl Pts',(-9.94081182900005,15.2,3.07242042699999));
#255047=CARTESIAN_POINT('Ctrl Pts',(-9.94081182900005,11.6,3.07242042699999));
#255048=CARTESIAN_POINT('Ctrl Pts',(-9.93974858600006,15.2,3.07195350199999));
#255049=CARTESIAN_POINT('Ctrl Pts',(-9.93974858600006,11.6,3.07195350199999));
#255050=CARTESIAN_POINT('Ctrl Pts',(-9.93869306400006,15.2,3.07149120299999));
#255051=CARTESIAN_POINT('Ctrl Pts',(-9.93869306400006,11.6,3.07149120299999));
#255052=CARTESIAN_POINT('Ctrl Pts',(-9.93764529000006,15.2,3.07103352399999));
#255053=CARTESIAN_POINT('Ctrl Pts',(-9.93764529000006,11.6,3.07103352399999));
#255054=CARTESIAN_POINT('Ctrl Pts',(-9.93660529600006,15.2,3.07058045999998));
#255055=CARTESIAN_POINT('Ctrl Pts',(-9.93660529600006,11.6,3.07058045999998));
#255056=CARTESIAN_POINT('Ctrl Pts',(-9.93557310900006,15.2,3.07013200499998));
#255057=CARTESIAN_POINT('Ctrl Pts',(-9.93557310900006,11.6,3.07013200499998));
#255058=CARTESIAN_POINT('Ctrl Pts',(-9.93454875700006,15.2,3.06968815199999));
#255059=CARTESIAN_POINT('Ctrl Pts',(-9.93454875700006,11.6,3.06968815199998));
#255060=CARTESIAN_POINT('Ctrl Pts',(-9.93353227100006,15.2,3.06924889799999));
#255061=CARTESIAN_POINT('Ctrl Pts',(-9.93353227100006,11.6,3.06924889799999));
#255062=CARTESIAN_POINT('Ctrl Pts',(-9.93252368000006,15.2,3.06881423499998));
#255063=CARTESIAN_POINT('Ctrl Pts',(-9.93252368000006,11.6,3.06881423499998));
#255064=CARTESIAN_POINT('Ctrl Pts',(-9.93152301100006,15.2,3.06838415799999));
#255065=CARTESIAN_POINT('Ctrl Pts',(-9.93152301100006,11.6,3.06838415799999));
#255066=CARTESIAN_POINT('Ctrl Pts',(-9.93053029600006,15.2,3.06795866099999));
#255067=CARTESIAN_POINT('Ctrl Pts',(-9.93053029600006,11.6,3.06795866099998));
#255068=CARTESIAN_POINT('Ctrl Pts',(-9.92954556500005,15.2,3.06753773799999));
#255069=CARTESIAN_POINT('Ctrl Pts',(-9.92954556500005,11.6,3.06753773799999));
#255070=CARTESIAN_POINT('Ctrl Pts',(-9.92856884700006,15.2,3.06712138399998));
#255071=CARTESIAN_POINT('Ctrl Pts',(-9.92856884700006,11.6,3.06712138399998));
#255072=CARTESIAN_POINT('Ctrl Pts',(-9.92760017000006,15.2,3.06670959199998));
#255073=CARTESIAN_POINT('Ctrl Pts',(-9.92760017000006,11.6,3.06670959199998));
#255074=CARTESIAN_POINT('Ctrl Pts',(-9.92663956700006,15.2,3.06630235699998));
#255075=CARTESIAN_POINT('Ctrl Pts',(-9.92663956700006,11.6,3.06630235699998));
#255076=CARTESIAN_POINT('Ctrl Pts',(-9.92568706800006,15.2,3.06589967099999));
#255077=CARTESIAN_POINT('Ctrl Pts',(-9.92568706800006,11.6,3.06589967099998));
#255078=CARTESIAN_POINT('Ctrl Pts',(-9.92474270200006,15.2,3.06550152999999));
#255079=CARTESIAN_POINT('Ctrl Pts',(-9.92474270200006,11.6,3.06550152999999));
#255080=CARTESIAN_POINT('Ctrl Pts',(-9.92380649900005,15.2,3.06510792799998));
#255081=CARTESIAN_POINT('Ctrl Pts',(-9.92380649900005,11.6,3.06510792799998));
#255082=CARTESIAN_POINT('Ctrl Pts',(-9.92287849100006,15.2,3.06471885699998));
#255083=CARTESIAN_POINT('Ctrl Pts',(-9.92287849100006,11.6,3.06471885699998));
#255084=CARTESIAN_POINT('Ctrl Pts',(-9.92195870900006,15.2,3.06433431199999));
#255085=CARTESIAN_POINT('Ctrl Pts',(-9.92195870900006,11.6,3.06433431199999));
#255086=CARTESIAN_POINT('Ctrl Pts',(-9.92104718300006,15.2,3.06395428599998));
#255087=CARTESIAN_POINT('Ctrl Pts',(-9.92104718300006,11.6,3.06395428599998));
#255088=CARTESIAN_POINT('Ctrl Pts',(-9.92014394400006,15.2,3.06357877499998));
#255089=CARTESIAN_POINT('Ctrl Pts',(-9.92014394400006,11.6,3.06357877499998));
#255090=CARTESIAN_POINT('Ctrl Pts',(-9.91924902500006,15.2,3.06320776899998));
#255091=CARTESIAN_POINT('Ctrl Pts',(-9.91924902500006,11.6,3.06320776899998));
#255092=CARTESIAN_POINT('Ctrl Pts',(-9.91836245600006,15.2,3.06284126399999));
#255093=CARTESIAN_POINT('Ctrl Pts',(-9.91836245600006,11.6,3.06284126399999));
#255094=CARTESIAN_POINT('Ctrl Pts',(-9.91748426900006,15.2,3.06247925299999));
#255095=CARTESIAN_POINT('Ctrl Pts',(-9.91748426900006,11.6,3.06247925299999));
#255096=CARTESIAN_POINT('Ctrl Pts',(-9.91661449500005,15.2,3.06212172999999));
#255097=CARTESIAN_POINT('Ctrl Pts',(-9.91661449500005,11.6,3.06212172999999));
#255098=CARTESIAN_POINT('Ctrl Pts',(-9.91575316600006,15.2,3.06176868799999));
#255099=CARTESIAN_POINT('Ctrl Pts',(-9.91575316600006,11.6,3.06176868799999));
#255100=CARTESIAN_POINT('Ctrl Pts',(-9.91490522600006,15.2,3.06142212699999));
#255101=CARTESIAN_POINT('Ctrl Pts',(-9.91490522600006,11.6,3.06142212699999));
#255102=CARTESIAN_POINT('Ctrl Pts',(-9.91423456700005,15.2,3.06114880399999));
#255103=CARTESIAN_POINT('Ctrl Pts',(-9.91423456700005,11.6,3.06114880399999));
#255104=CARTESIAN_POINT('Ctrl Pts',(-9.91373655900006,15.2,3.06094627499998));
#255105=CARTESIAN_POINT('Ctrl Pts',(-9.91373655900006,11.6,3.06094627499998));
#255106=CARTESIAN_POINT('Ctrl Pts',(-9.91340782700006,15.2,3.06081277699998));
#255107=CARTESIAN_POINT('Ctrl Pts',(-9.91340782700006,11.6,3.06081277699998));
#255108=CARTESIAN_POINT('Ctrl Pts',(-9.91324626500005,15.2,3.06074721299999));
#255109=CARTESIAN_POINT('Ctrl Pts',(-9.91324626500005,11.6,3.06074721299999));
#255110=CARTESIAN_POINT('',(-9.91324626490332,12.2,3.06074721230345));
#255111=CARTESIAN_POINT('',(-9.91324626490332,15.2,3.06074721230345));
#255112=CARTESIAN_POINT('',(-9.91324626500005,12.2,3.06074721199998));
#255113=CARTESIAN_POINT('Ctrl Pts',(-10.8675859440001,12.2,3.76106045599998));
#255114=CARTESIAN_POINT('Ctrl Pts',(-10.8648866835097,12.2,3.75835329050819));
#255115=CARTESIAN_POINT('Ctrl Pts',(-10.8621890332054,12.2,3.75565386693063));
#255116=CARTESIAN_POINT('Ctrl Pts',(-10.859493000351,12.2,3.75296217351306));
#255117=CARTESIAN_POINT('Ctrl Pts',(-10.8567969674967,12.2,3.75027048009549));
#255118=CARTESIAN_POINT('Ctrl Pts',(-10.8541025488079,12.2,3.74758652000514));
#255119=CARTESIAN_POINT('Ctrl Pts',(-10.8514097638127,12.2,3.74491029600946));
#255120=CARTESIAN_POINT('Ctrl Pts',(-10.8487169788175,12.2,3.74223407201377));
#255121=CARTESIAN_POINT('Ctrl Pts',(-10.8460258270055,12.2,3.73956558443436));
#255122=CARTESIAN_POINT('Ctrl Pts',(-10.843336351103,12.2,3.73690483861331));
#255123=CARTESIAN_POINT('Ctrl Pts',(-10.8406468747119,12.2,3.7342440923089));
#255124=CARTESIAN_POINT('Ctrl Pts',(-10.8379590773546,12.2,3.73159108737333));
#255125=CARTESIAN_POINT('Ctrl Pts',(-10.8352730049228,12.2,3.72894582865661));
#255126=CARTESIAN_POINT('Ctrl Pts',(-10.832586932979,12.2,3.72630057042045));
#255127=CARTESIAN_POINT('Ctrl Pts',(-10.8299025886434,12.2,3.72366305998386));
#255128=CARTESIAN_POINT('Ctrl Pts',(-10.8272200099493,12.2,3.72103329924675));
#255129=CARTESIAN_POINT('Ctrl Pts',(-10.8245374312553,12.2,3.71840353850965));
#255130=CARTESIAN_POINT('Ctrl Pts',(-10.8218566176958,12.2,3.71578152924774));
#255131=CARTESIAN_POINT('Ctrl Pts',(-10.8191776064893,12.2,3.71316727449756));
#255132=CARTESIAN_POINT('Ctrl Pts',(-10.8156055917095,12.2,3.70968160165563));
#255133=CARTESIAN_POINT('Ctrl Pts',(-10.8120367800946,12.2,3.7062097149535));
#255134=CARTESIAN_POINT('Ctrl Pts',(-10.808471272108,12.2,3.70275162529033));
#255135=CARTESIAN_POINT('Ctrl Pts',(-10.8057971405108,12.2,3.700158057454));
#255136=CARTESIAN_POINT('Ctrl Pts',(-10.8031248672557,12.2,3.69757225019487));
#255137=CARTESIAN_POINT('Ctrl Pts',(-10.8004544941596,12.2,3.6949942079046));
#255138=CARTESIAN_POINT('Ctrl Pts',(-10.7977841215485,12.2,3.69241616608267));
#255139=CARTESIAN_POINT('Ctrl Pts',(-10.7951156493957,12.2,3.68984588976031));
#255140=CARTESIAN_POINT('Ctrl Pts',(-10.7924491182011,12.2,3.68728338147908));
#255141=CARTESIAN_POINT('Ctrl Pts',(-10.7897825870065,12.2,3.68472087319785));
#255142=CARTESIAN_POINT('Ctrl Pts',(-10.7871179959296,12.2,3.68216613428329));
#255143=CARTESIAN_POINT('Ctrl Pts',(-10.7844553872643,12.2,3.67961916748928));
#255144=CARTESIAN_POINT('Ctrl Pts',(-10.7817927785989,12.2,3.67707220069528));
#255145=CARTESIAN_POINT('Ctrl Pts',(-10.7791321518846,12.2,3.67453300677179));
#255146=CARTESIAN_POINT('Ctrl Pts',(-10.7764735492608,12.2,3.6720015890189));
#255147=CARTESIAN_POINT('Ctrl Pts',(-10.773814946637,12.2,3.66947017126601));
#255148=CARTESIAN_POINT('Ctrl Pts',(-10.7711583682432,12.2,3.66694653110023));
#255149=CARTESIAN_POINT('Ctrl Pts',(-10.7685038565478,12.2,3.66443067123262));
#255150=CARTESIAN_POINT('Ctrl Pts',(-10.7658493448523,12.2,3.66191481136502));
#255151=CARTESIAN_POINT('Ctrl Pts',(-10.7631968984651,12.2,3.65940673118856));
#255152=CARTESIAN_POINT('Ctrl Pts',(-10.7605465608528,12.2,3.65690643582));
#255153=CARTESIAN_POINT('Ctrl Pts',(-10.7570127770487,12.2,3.6535727083591));
#255154=CARTESIAN_POINT('Ctrl Pts',(-10.753482742078,12.2,3.6502528186067));
#255155=CARTESIAN_POINT('Ctrl Pts',(-10.749956554981,12.2,3.64694677702268));
#255156=CARTESIAN_POINT('Ctrl Pts',(-10.7473119148984,12.2,3.6444672460599));
#255157=CARTESIAN_POINT('Ctrl Pts',(-10.7446694401185,12.2,3.64199550282386));
#255158=CARTESIAN_POINT('Ctrl Pts',(-10.7420291729941,12.2,3.63953155298551));
#255159=CARTESIAN_POINT('Ctrl Pts',(-10.7393889058697,12.2,3.63706760314717));
#255160=CARTESIAN_POINT('Ctrl Pts',(-10.7367508461752,12.2,3.63461144652866));
#255161=CARTESIAN_POINT('Ctrl Pts',(-10.7341150375207,12.2,3.63216308474193));
#255162=CARTESIAN_POINT('Ctrl Pts',(-10.7314792288663,12.2,3.6297147229552));
#255163=CARTESIAN_POINT('Ctrl Pts',(-10.7288456702617,12.2,3.62727415762628));
#255164=CARTESIAN_POINT('Ctrl Pts',(-10.7262144070653,12.2,3.62484139129694));
#255165=CARTESIAN_POINT('Ctrl Pts',(-10.7235831433909,12.2,3.62240862452564));
#255166=CARTESIAN_POINT('Ctrl Pts',(-10.7209541732422,12.2,3.61998365750656));
#255167=CARTESIAN_POINT('Ctrl Pts',(-10.7183275401524,12.2,3.61756649273966));
#255168=CARTESIAN_POINT('Ctrl Pts',(-10.7157009075398,12.2,3.61514932841188));
#255169=CARTESIAN_POINT('Ctrl Pts',(-10.7130766121022,12.2,3.61273996628369));
#255170=CARTESIAN_POINT('Ctrl Pts',(-10.7104546984893,12.2,3.61033840995496));
#255171=CARTESIAN_POINT('Ctrl Pts',(-10.7078327848764,12.2,3.60793685362623));
#255172=CARTESIAN_POINT('Ctrl Pts',(-10.7052132530144,12.2,3.60554310333854));
#255173=CARTESIAN_POINT('Ctrl Pts',(-10.7025961450143,12.2,3.60315716149777));
#255174=CARTESIAN_POINT('Ctrl Pts',(-10.6999790370142,12.2,3.600771219657));
#255175=CARTESIAN_POINT('Ctrl Pts',(-10.6973643543527,12.2,3.59839308682676));
#255176=CARTESIAN_POINT('Ctrl Pts',(-10.6947521417274,12.2,3.59602276498542));
#255177=CARTESIAN_POINT('Ctrl Pts',(-10.6921399291021,12.2,3.59365244314408));
#255178=CARTESIAN_POINT('Ctrl Pts',(-10.6895301856731,12.2,3.59128993267185));
#255179=CARTESIAN_POINT('Ctrl Pts',(-10.6869229560593,12.2,3.58893523775673));
#255180=CARTESIAN_POINT('Ctrl Pts',(-10.6834466495917,12.2,3.58579564425137));
#255181=CARTESIAN_POINT('Ctrl Pts',(-10.6799748122803,12.2,3.58266994358657));
#255182=CARTESIAN_POINT('Ctrl Pts',(-10.6765075492583,12.2,3.579558141529));
#255183=CARTESIAN_POINT('Ctrl Pts',(-10.6730402867087,12.2,3.57644633989542));
#255184=CARTESIAN_POINT('Ctrl Pts',(-10.6695776003868,12.2,3.57334843804238));
#255185=CARTESIAN_POINT('Ctrl Pts',(-10.6661195950518,12.2,3.57026444097251));
#255186=CARTESIAN_POINT('Ctrl Pts',(-10.6635260909328,12.2,3.56795144306506));
#255187=CARTESIAN_POINT('Ctrl Pts',(-10.6609352210039,12.2,3.56564626825169));
#255188=CARTESIAN_POINT('Ctrl Pts',(-10.6583470290559,12.2,3.56334891650076));
#255189=CARTESIAN_POINT('Ctrl Pts',(-10.6557588366377,12.2,3.56105156433247));
#255190=CARTESIAN_POINT('Ctrl Pts',(-10.6531733234787,12.2,3.5587620375164));
#255191=CARTESIAN_POINT('Ctrl Pts',(-10.6505905358953,12.2,3.55648033676919));
#255192=CARTESIAN_POINT('Ctrl Pts',(-10.6480077487812,12.2,3.55419863643649));
#255193=CARTESIAN_POINT('Ctrl Pts',(-10.6454276865586,12.2,3.55192476297005));
#255194=CARTESIAN_POINT('Ctrl Pts',(-10.6428503940275,12.2,3.5496587195114));
#255195=CARTESIAN_POINT('Ctrl Pts',(-10.6402731014964,12.2,3.54739267605275));
#255196=CARTESIAN_POINT('Ctrl Pts',(-10.6376985798159,12.2,3.5451344606763));
#255197=CARTESIAN_POINT('Ctrl Pts',(-10.6351268752727,12.2,3.5428840772479));
#255198=CARTESIAN_POINT('Ctrl Pts',(-10.6325551707295,12.2,3.5406336938195));
#255199=CARTESIAN_POINT('Ctrl Pts',(-10.6299862825041,12.2,3.53839114168094));
#255200=CARTESIAN_POINT('Ctrl Pts',(-10.6274202574607,12.2,3.53615642329363));
#255201=CARTESIAN_POINT('Ctrl Pts',(-10.6248542324173,12.2,3.53392170490632));
#255202=CARTESIAN_POINT('Ctrl Pts',(-10.622291070403,12.2,3.531694820112));
#255203=CARTESIAN_POINT('Ctrl Pts',(-10.6197308192875,12.2,3.5294757712336));
#255204=CARTESIAN_POINT('Ctrl Pts',(-10.6171705681719,12.2,3.5272567223552));
#255205=CARTESIAN_POINT('Ctrl Pts',(-10.6146132262978,12.2,3.52504550903462));
#255206=CARTESIAN_POINT('Ctrl Pts',(-10.6120588417652,12.2,3.52284213273861));
#255207=CARTESIAN_POINT('Ctrl Pts',(-10.6086529954124,12.2,3.5199042974104));
#255208=CARTESIAN_POINT('Ctrl Pts',(-10.6052524067926,12.2,3.51698039769193));
#255209=CARTESIAN_POINT('Ctrl Pts',(-10.6018571864811,12.2,3.51407043429795));
#255210=CARTESIAN_POINT('Ctrl Pts',(-10.5993107714787,12.2,3.5118879619507));
#255211=CARTESIAN_POINT('Ctrl Pts',(-10.5967673764883,12.2,3.50971332959972));
#255212=CARTESIAN_POINT('Ctrl Pts',(-10.5942270494857,12.2,3.50754653921024));
#255213=CARTESIAN_POINT('Ctrl Pts',(-10.5908399465079,12.2,3.50465748509517));
#255214=CARTESIAN_POINT('Ctrl Pts',(-10.5874582980759,12.2,3.50178237116998));
#255215=CARTESIAN_POINT('Ctrl Pts',(-10.584082216448,12.2,3.49892120301547));
#255216=CARTESIAN_POINT('Ctrl Pts',(-10.5807061352801,12.2,3.49606003525078));
#255217=CARTESIAN_POINT('Ctrl Pts',(-10.5773356218088,12.2,3.49321281202043));
#255218=CARTESIAN_POINT('Ctrl Pts',(-10.5739707912502,12.2,3.49037953697335));
#255219=CARTESIAN_POINT('Ctrl Pts',(-10.5706059602331,12.2,3.48754626154024));
#255220=CARTESIAN_POINT('Ctrl Pts',(-10.5672468119299,12.2,3.48472693393198));
#255221=CARTESIAN_POINT('Ctrl Pts',(-10.5638934602468,12.2,3.4819215575846));
#255222=CARTESIAN_POINT('Ctrl Pts',(-10.5605401090206,12.2,3.47911618161945));
#255223=CARTESIAN_POINT('Ctrl Pts',(-10.5571925583782,12.2,3.47632475663708));
#255224=CARTESIAN_POINT('Ctrl Pts',(-10.5538509205399,12.2,3.47354728625212));
#255225=CARTESIAN_POINT('Ctrl Pts',(-10.5505092822463,12.2,3.47076981548872));
#255226=CARTESIAN_POINT('Ctrl Pts',(-10.5471735576367,12.2,3.46800629902145));
#255227=CARTESIAN_POINT('Ctrl Pts',(-10.5438438666779,12.2,3.46525673881695));
#255228=CARTESIAN_POINT('Ctrl Pts',(-10.5405141761727,12.2,3.46250717898708));
#255229=CARTESIAN_POINT('Ctrl Pts',(-10.5371905166821,12.2,3.45977157437072));
#255230=CARTESIAN_POINT('Ctrl Pts',(-10.5338730092315,12.2,3.45704992967827));
#255231=CARTESIAN_POINT('Ctrl Pts',(-10.5305555013288,12.2,3.45432828461499));
#255232=CARTESIAN_POINT('Ctrl Pts',(-10.5272441432846,12.2,3.45162059612574));
#255233=CARTESIAN_POINT('Ctrl Pts',(-10.5239390562716,12.2,3.44892686931318));
#255234=CARTESIAN_POINT('Ctrl Pts',(-10.5206339697088,12.2,3.44623314286764));
#255235=CARTESIAN_POINT('Ctrl Pts',(-10.5173351526143,12.2,3.44355337614984));
#255236=CARTESIAN_POINT('Ctrl Pts',(-10.5140427267717,12.2,3.44088757097746));
#255237=CARTESIAN_POINT('Ctrl Pts',(-10.5107503004805,12.2,3.43822176544185));
#255238=CARTESIAN_POINT('Ctrl Pts',(-10.5074642652414,12.2,3.43556992142328));
#255239=CARTESIAN_POINT('Ctrl Pts',(-10.5041847417145,12.2,3.4329320399898));
#255240=CARTESIAN_POINT('Ctrl Pts',(-10.5009052186344,12.2,3.43029415891573));
#255241=CARTESIAN_POINT('Ctrl Pts',(-10.4976322082677,12.2,3.42767023978141));
#255242=CARTESIAN_POINT('Ctrl Pts',(-10.4943658325341,12.2,3.42506028399333));
#255243=CARTESIAN_POINT('Ctrl Pts',(-10.4910994563553,12.2,3.42245032784964));
#255244=CARTESIAN_POINT('Ctrl Pts',(-10.4878397151856,12.2,3.41985433453786));
#255245=CARTESIAN_POINT('Ctrl Pts',(-10.4845867335084,12.2,3.41727230500826));
#255246=CARTESIAN_POINT('Ctrl Pts',(-10.4813337518311,12.2,3.41469027547866));
#255247=CARTESIAN_POINT('Ctrl Pts',(-10.4780875271296,12.2,3.4121222086729));
#255248=CARTESIAN_POINT('Ctrl Pts',(-10.4748481869537,12.2,3.40956810459068));
#255249=CARTESIAN_POINT('Ctrl Pts',(-10.470799012396,12.2,3.4063754750099));
#255250=CARTESIAN_POINT('Ctrl Pts',(-10.466760591561,12.2,3.40320466264262));
#255251=CARTESIAN_POINT('Ctrl Pts',(-10.4627331735268,12.2,3.40005566784516));
#255252=CARTESIAN_POINT('Ctrl Pts',(-10.4595112385727,12.2,3.3975364715953));
#255253=CARTESIAN_POINT('Ctrl Pts',(-10.4562963425026,12.2,3.39503123649959));
#255254=CARTESIAN_POINT('Ctrl Pts',(-10.4530886162167,12.2,3.39253996297493));
#255255=CARTESIAN_POINT('Ctrl Pts',(-10.4498808899308,12.2,3.39004868945026));
#255256=CARTESIAN_POINT('Ctrl Pts',(-10.4466803308679,12.2,3.38757137713001));
#255257=CARTESIAN_POINT('Ctrl Pts',(-10.4434870686946,12.2,3.38510802433052));
#255258=CARTESIAN_POINT('Ctrl Pts',(-10.4402938069564,12.2,3.38264467186666));
#255259=CARTESIAN_POINT('Ctrl Pts',(-10.4371078402922,12.2,3.38019527878154));
#255260=CARTESIAN_POINT('Ctrl Pts',(-10.4339293010516,12.2,3.37775984425749));
#255261=CARTESIAN_POINT('Ctrl Pts',(-10.4307507613779,12.2,3.37532440940161));
#255262=CARTESIAN_POINT('Ctrl Pts',(-10.4275796459097,12.2,3.37290293082871));
#255263=CARTESIAN_POINT('Ctrl Pts',(-10.4244160870244,12.2,3.370495409134));
#255264=CARTESIAN_POINT('Ctrl Pts',(-10.42125252857,12.2,3.36808788776732));
#255265=CARTESIAN_POINT('Ctrl Pts',(-10.4180965276395,12.2,3.36569432139819));
#255266=CARTESIAN_POINT('Ctrl Pts',(-10.4149482140075,12.2,3.36331470820292));
#255267=CARTESIAN_POINT('Ctrl Pts',(-10.4117998999465,12.2,3.36093509468343));
#255268=CARTESIAN_POINT('Ctrl Pts',(-10.4086592756559,12.2,3.35856943385453));
#255269=CARTESIAN_POINT('Ctrl Pts',(-10.4055264709857,12.2,3.35621772178281));
#255270=CARTESIAN_POINT('Ctrl Pts',(-10.4023936667422,12.2,3.35386601003151));
#255271=CARTESIAN_POINT('Ctrl Pts',(-10.3992686851623,12.2,3.35152824936178));
#255272=CARTESIAN_POINT('Ctrl Pts',(-10.3961516574274,12.2,3.34920443404554));
#255273=CARTESIAN_POINT('Ctrl Pts',(-10.3930346292677,12.2,3.34688061841268));
#255274=CARTESIAN_POINT('Ctrl Pts',(-10.3899255578012,12.2,3.34457074838659));
#255275=CARTESIAN_POINT('Ctrl Pts',(-10.3868245770216,12.2,3.34227482026237));
#255276=CARTESIAN_POINT('Ctrl Pts',(-10.3829483512584,12.2,3.3394049102635));
#255277=CARTESIAN_POINT('Ctrl Pts',(-10.3790847675087,12.2,3.33655678533073));
#255278=CARTESIAN_POINT('Ctrl Pts',(-10.3752340934816,12.2,3.33373043533189));
#255279=CARTESIAN_POINT('Ctrl Pts',(-10.3721535545118,12.2,3.33146935551765));
#255280=CARTESIAN_POINT('Ctrl Pts',(-10.3690812778008,12.2,3.32922221276817));
#255281=CARTESIAN_POINT('Ctrl Pts',(-10.366017401953,12.2,3.32698900011572));
#255282=CARTESIAN_POINT('Ctrl Pts',(-10.3629535256877,12.2,3.32475578715899));
#255283=CARTESIAN_POINT('Ctrl Pts',(-10.3598980494387,12.2,3.32253650610016));
#255284=CARTESIAN_POINT('Ctrl Pts',(-10.356851114051,12.2,3.32033115053644));
#255285=CARTESIAN_POINT('Ctrl Pts',(-10.3538041790785,12.2,3.3181257952732));
#255286=CARTESIAN_POINT('Ctrl Pts',(-10.3507657842903,12.2,3.31593436500993));
#255287=CARTESIAN_POINT('Ctrl Pts',(-10.3477360707037,12.2,3.31375685513096));
#255288=CARTESIAN_POINT('Ctrl Pts',(-10.3447063567044,12.2,3.3115793449553));
#255289=CARTESIAN_POINT('Ctrl Pts',(-10.3416853250341,12.2,3.30941575332812));
#255290=CARTESIAN_POINT('Ctrl Pts',(-10.338673117023,12.2,3.3072660762568));
#255291=CARTESIAN_POINT('Ctrl Pts',(-10.3356609094222,12.2,3.30511639947838));
#255292=CARTESIAN_POINT('Ctrl Pts',(-10.3326575241652,12.2,3.30298063452204));
#255293=CARTESIAN_POINT('Ctrl Pts',(-10.3296631084646,12.2,3.30085877663853));
#255294=CARTESIAN_POINT('Ctrl Pts',(-10.3266686923561,12.2,3.29873691846591));
#255295=CARTESIAN_POINT('Ctrl Pts',(-10.3236832434233,12.2,3.29662896572238));
#255296=CARTESIAN_POINT('Ctrl Pts',(-10.3207069074834,12.2,3.29453491277493));
#255297=CARTESIAN_POINT('Ctrl Pts',(-10.3177305715434,12.2,3.29244085982747));
#255298=CARTESIAN_POINT('Ctrl Pts',(-10.3147633490211,12.2,3.29036070391775));
#255299=CARTESIAN_POINT('Ctrl Pts',(-10.3118053857497,12.2,3.28829443969544));
#255300=CARTESIAN_POINT('Ctrl Pts',(-10.3088474228814,12.2,3.28622817575465));
#255301=CARTESIAN_POINT('Ctrl Pts',(-10.3058987195057,12.2,3.2841758029412));
#255302=CARTESIAN_POINT('Ctrl Pts',(-10.3029594240104,12.2,3.28213731170965));
#255303=CARTESIAN_POINT('Ctrl Pts',(-10.3000201281146,12.2,3.28009882020036));
#255304=CARTESIAN_POINT('Ctrl Pts',(-10.2970902409029,12.2,3.27807421134324));
#255305=CARTESIAN_POINT('Ctrl Pts',(-10.2941699115226,12.2,3.27606347517953));
#255306=CARTESIAN_POINT('Ctrl Pts',(-10.2912495825401,12.2,3.27405273928978));
#255307=CARTESIAN_POINT('Ctrl Pts',(-10.2883388099591,12.2,3.27205587713153));
#255308=CARTESIAN_POINT('Ctrl Pts',(-10.2854377470289,12.2,3.27007287790384));
#255309=CARTESIAN_POINT('Ctrl Pts',(-10.2825366837035,12.2,3.26808987840595));
#255310=CARTESIAN_POINT('Ctrl Pts',(-10.279645327446,12.2,3.26612074278043));
#255311=CARTESIAN_POINT('Ctrl Pts',(-10.2767638340903,12.2,3.26416546046629));
#255312=CARTESIAN_POINT('Ctrl Pts',(-10.2738823411272,12.2,3.26221017841855));
#255313=CARTESIAN_POINT('Ctrl Pts',(-10.2710107106674,12.2,3.26026874981486));
#255314=CARTESIAN_POINT('Ctrl Pts',(-10.268149095234,12.2,3.25834116391597));
#255315=CARTESIAN_POINT('Ctrl Pts',(-10.2652874794108,12.2,3.25641357775446));
#255316=CARTESIAN_POINT('Ctrl Pts',(-10.2624358801054,12.2,3.25449983463905));
#255317=CARTESIAN_POINT('Ctrl Pts',(-10.2595944522845,12.2,3.25259992303641));
#255318=CARTESIAN_POINT('Ctrl Pts',(-10.2567530248508,12.2,3.25070001169263));
#255319=CARTESIAN_POINT('Ctrl Pts',(-10.2539217693651,12.2,3.24881393209946));
#255320=CARTESIAN_POINT('Ctrl Pts',(-10.2511008436761,12.2,3.24694167254669));
#255321=CARTESIAN_POINT('Ctrl Pts',(-10.2482799176027,12.2,3.24506941273881));
#255322=CARTESIAN_POINT('Ctrl Pts',(-10.2454693210092,12.2,3.24321097044334));
#255323=CARTESIAN_POINT('Ctrl Pts',(-10.2426692132462,12.2,3.24136633756593));
#255324=CARTESIAN_POINT('Ctrl Pts',(-10.2391690787332,12.2,3.23906054659484));
#255325=CARTESIAN_POINT('Ctrl Pts',(-10.2356853329669,12.2,3.23677632987318));
#255326=CARTESIAN_POINT('Ctrl Pts',(-10.2322182910234,12.2,3.23451366140209));
#255327=CARTESIAN_POINT('Ctrl Pts',(-10.2280578408423,12.2,3.23179845933543));
#255328=CARTESIAN_POINT('Ctrl Pts',(-10.2239214453629,12.2,3.22911428617519));
#255329=CARTESIAN_POINT('Ctrl Pts',(-10.2198096532435,12.2,3.22646109800947));
#255330=CARTESIAN_POINT('Ctrl Pts',(-10.2163831596863,12.2,3.22425010779104));
#255331=CARTESIAN_POINT('Ctrl Pts',(-10.2129737552833,12.2,3.22206063282769));
#255332=CARTESIAN_POINT('Ctrl Pts',(-10.2095817617417,12.2,3.21989264525826));
#255333=CARTESIAN_POINT('Ctrl Pts',(-10.2061897682,12.2,3.21772465768884));
#255334=CARTESIAN_POINT('Ctrl Pts',(-10.2028151879334,12.2,3.21557815805548));
#255335=CARTESIAN_POINT('Ctrl Pts',(-10.199458347725,12.2,3.2134531160416));
#255336=CARTESIAN_POINT('Ctrl Pts',(-10.1961015075167,12.2,3.2113280740277));
#255337=CARTESIAN_POINT('Ctrl Pts',(-10.1927624098355,12.2,3.20922448725264));
#255338=CARTESIAN_POINT('Ctrl Pts',(-10.1894413855149,12.2,3.20714232550713));
#255339=CARTESIAN_POINT('Ctrl Pts',(-10.1861203611943,12.2,3.20506016376162));
#255340=CARTESIAN_POINT('Ctrl Pts',(-10.1828174127621,12.2,3.20299942742668));
#255341=CARTESIAN_POINT('Ctrl Pts',(-10.1795328783186,12.2,3.20096008381668));
#255342=CARTESIAN_POINT('Ctrl Pts',(-10.1762483438752,12.2,3.19892074020669));
#255343=CARTESIAN_POINT('Ctrl Pts',(-10.1729822220812,12.2,3.19690278675725));
#255344=CARTESIAN_POINT('Ctrl Pts',(-10.1697348578461,12.2,3.19490619057781));
#255345=CARTESIAN_POINT('Ctrl Pts',(-10.1664874936109,12.2,3.19290959439837));
#255346=CARTESIAN_POINT('Ctrl Pts',(-10.1632588872309,12.2,3.19093435370264));
#255347=CARTESIAN_POINT('Ctrl Pts',(-10.1600493853358,12.2,3.18898043256485));
#255348=CARTESIAN_POINT('Ctrl Pts',(-10.1568398834407,12.2,3.18702651142707));
#255349=CARTESIAN_POINT('Ctrl Pts',(-10.1536494890226,12.2,3.18509390962597));
#255350=CARTESIAN_POINT('Ctrl Pts',(-10.1504785538853,12.2,3.1831825885166));
#255351=CARTESIAN_POINT('Ctrl Pts',(-10.147307618748,12.2,3.18127126740723));
#255352=CARTESIAN_POINT('Ctrl Pts',(-10.1441561421943,12.2,3.17938122751488));
#255353=CARTESIAN_POINT('Ctrl Pts',(-10.1410244853904,12.2,3.17751242723883));
#255354=CARTESIAN_POINT('Ctrl Pts',(-10.1378928289278,12.2,3.17564362716648));
#255355=CARTESIAN_POINT('Ctrl Pts',(-10.1347809913024,12.2,3.17379606696927));
#255356=CARTESIAN_POINT('Ctrl Pts',(-10.1316893366377,12.2,3.17196970522216));
#255357=CARTESIAN_POINT('Ctrl Pts',(-10.1285976816361,12.2,3.17014334327599));
#255358=CARTESIAN_POINT('Ctrl Pts',(-10.1255262104563,12.2,3.16833817811835));
#255359=CARTESIAN_POINT('Ctrl Pts',(-10.1224752936491,12.2,3.16655416769995));
#255360=CARTESIAN_POINT('Ctrl Pts',(-10.1194243768418,12.2,3.16477015728156));
#255361=CARTESIAN_POINT('Ctrl Pts',(-10.1163940126735,12.2,3.1630073000018));
#255362=CARTESIAN_POINT('Ctrl Pts',(-10.1133845798828,12.2,3.16126555046886));
#255363=CARTESIAN_POINT('Ctrl Pts',(-10.1103751470921,12.2,3.15952380093593));
#255364=CARTESIAN_POINT('Ctrl Pts',(-10.1073866425619,12.2,3.1578031583123));
#255365=CARTESIAN_POINT('Ctrl Pts',(-10.1044194517275,12.2,3.15610357539454));
#255366=CARTESIAN_POINT('Ctrl Pts',(-10.1008588225322,12.2,3.15406407578209));
#255367=CARTESIAN_POINT('Ctrl Pts',(-10.0973288811739,12.2,3.15205490206503));
#255368=CARTESIAN_POINT('Ctrl Pts',(-10.093830302152,12.2,3.15007596654256));
#255369=CARTESIAN_POINT('Ctrl Pts',(-10.0903317234479,12.2,3.14809703119985));
#255370=CARTESIAN_POINT('Ctrl Pts',(-10.0868645050034,12.2,3.14614833417447));
#255371=CARTESIAN_POINT('Ctrl Pts',(-10.0834293342962,12.2,3.14422978391216));
#255372=CARTESIAN_POINT('Ctrl Pts',(-10.0799941635892,12.2,3.14231123364986));
#255373=CARTESIAN_POINT('Ctrl Pts',(-10.0765910392295,12.2,3.1404228306268));
#255374=CARTESIAN_POINT('Ctrl Pts',(-10.0732206606838,12.2,3.13856448010967));
#255375=CARTESIAN_POINT('Ctrl Pts',(-10.0698502821382,12.2,3.13670612959254));
#255376=CARTESIAN_POINT('Ctrl Pts',(-10.0665126507591,12.2,3.134877828016));
#255377=CARTESIAN_POINT('Ctrl Pts',(-10.0632084763768,12.2,3.13307947774596));
#255378=CARTESIAN_POINT('Ctrl Pts',(-10.0599043016944,12.2,3.13128112731257));
#255379=CARTESIAN_POINT('Ctrl Pts',(-10.0566335871653,12.2,3.12951272809042));
#255380=CARTESIAN_POINT('Ctrl Pts',(-10.0533970603237,12.2,3.12777417341364));
#255381=CARTESIAN_POINT('Ctrl Pts',(-10.0501605337762,12.2,3.12603561889478));
#255382=CARTESIAN_POINT('Ctrl Pts',(-10.0469581925425,12.2,3.12432691106407));
#255383=CARTESIAN_POINT('Ctrl Pts',(-10.0437907840598,12.2,3.12264793578403));
#255384=CARTESIAN_POINT('Ctrl Pts',(-10.040623375577,12.2,3.12096896050399));
#255385=CARTESIAN_POINT('Ctrl Pts',(-10.0374908959775,12.2,3.11931972172799));
#255386=CARTESIAN_POINT('Ctrl Pts',(-10.0343941085876,12.2,3.11770010120148));
#255387=CARTESIAN_POINT('Ctrl Pts',(-10.0312973209163,12.2,3.11608048052785));
#255388=CARTESIAN_POINT('Ctrl Pts',(-10.0282362230213,12.2,3.11449047960202));
#255389=CARTESIAN_POINT('Ctrl Pts',(-10.0252115922075,12.2,3.11292997685738));
#255390=CARTESIAN_POINT('Ctrl Pts',(-10.0221869616684,12.2,3.11136947425449));
#255391=CARTESIAN_POINT('Ctrl Pts',(-10.0191987961761,12.2,3.1098384695037));
#255392=CARTESIAN_POINT('Ctrl Pts',(-10.01624789195,12.2,3.10833683697493));
#255393=CARTESIAN_POINT('Ctrl Pts',(-10.0128051701741,12.2,3.1065849322671));
#255394=CARTESIAN_POINT('Ctrl Pts',(-10.0094131616831,12.2,3.10487300692428));
#255395=CARTESIAN_POINT('Ctrl Pts',(-10.0060731590775,12.2,3.10320084962194));
#255396=CARTESIAN_POINT('Ctrl Pts',(-10.0027331567319,12.2,3.10152869244979));
#255397=CARTESIAN_POINT('Ctrl Pts',(-9.99944515810944,12.2,3.09989630294632));
#255398=CARTESIAN_POINT('Ctrl Pts',(-9.99621049204389,12.2,3.0983034604321));
#255399=CARTESIAN_POINT('Ctrl Pts',(-9.99343792080676,12.2,3.09693816668903));
#255400=CARTESIAN_POINT('Ctrl Pts',(-9.99070453057342,12.2,3.09560192724046));
#255401=CARTESIAN_POINT('Ctrl Pts',(-9.98801118034504,12.2,3.09429459642047));
#255402=CARTESIAN_POINT('Ctrl Pts',(-9.98531783036131,12.2,3.09298726571924));
#255403=CARTESIAN_POINT('Ctrl Pts',(-9.98266451873488,12.2,3.09170884286084));
#255404=CARTESIAN_POINT('Ctrl Pts',(-9.9800521229845,12.2,3.09045917523384));
#255405=CARTESIAN_POINT('Ctrl Pts',(-9.97743972723414,12.2,3.08920950760683));
#255406=CARTESIAN_POINT('Ctrl Pts',(-9.97486824733664,12.2,3.08798859625519));
#255407=CARTESIAN_POINT('Ctrl Pts',(-9.97233858175906,12.2,3.0867962796299));
#255408=CARTESIAN_POINT('Ctrl Pts',(-9.9698089159517,12.2,3.08560396289631));
#255409=CARTESIAN_POINT('Ctrl Pts',(-9.96732106555814,12.2,3.08444024334045));
#255410=CARTESIAN_POINT('Ctrl Pts',(-9.96487594972188,12.2,3.08330495239018));
#255411=CARTESIAN_POINT('Ctrl Pts',(-9.96243083410772,12.2,3.08216966154304));
#255412=CARTESIAN_POINT('Ctrl Pts',(-9.96002845450592,12.2,3.08106280104407));
#255413=CARTESIAN_POINT('Ctrl Pts',(-9.95766975500831,12.2,3.07998419524993));
#255414=CARTESIAN_POINT('Ctrl Pts',(-9.9553110555107,12.2,3.0789055894558));
#255415=CARTESIAN_POINT('Ctrl Pts',(-9.95299603625324,12.2,3.07785523960613));
#255416=CARTESIAN_POINT('Ctrl Pts',(-9.95072566671972,12.2,3.07683296384056));
#255417=CARTESIAN_POINT('Ctrl Pts',(-9.94845529697996,12.2,3.07581068798214));
#255418=CARTESIAN_POINT('Ctrl Pts',(-9.94622957706972,12.2,3.07481648578705));
#255419=CARTESIAN_POINT('Ctrl Pts',(-9.94404950253736,12.2,3.07385016965295));
#255420=CARTESIAN_POINT('Ctrl Pts',(-9.94186942820301,12.2,3.07288385360662));
#255421=CARTESIAN_POINT('Ctrl Pts',(-9.93973499797421,12.2,3.07194542162885));
#255422=CARTESIAN_POINT('Ctrl Pts',(-9.93764723495736,12.2,3.07103467774119));
#255423=CARTESIAN_POINT('Ctrl Pts',(-9.9355594719405,12.2,3.07012393385354));
#255424=CARTESIAN_POINT('Ctrl Pts',(-9.93351837835514,12.2,3.0692408780168));
#255425=CARTESIAN_POINT('Ctrl Pts',(-9.93152499959215,12.2,3.06838530304668));
#255426=CARTESIAN_POINT('Ctrl Pts',(-9.92953162064808,12.2,3.06752972799885));
#255427=CARTESIAN_POINT('Ctrl Pts',(-9.92758596123495,12.2,3.0667016350211));
#255428=CARTESIAN_POINT('Ctrl Pts',(-9.92568910105156,12.2,3.06590080714599));
#255429=CARTESIAN_POINT('Ctrl Pts',(-9.92379224104047,12.2,3.06509997934361));
#255430=CARTESIAN_POINT('Ctrl Pts',(-9.92194417655968,12.2,3.06432641939773));
#255431=CARTESIAN_POINT('Ctrl Pts',(-9.92014602387718,12.2,3.06357990125936));
#255432=CARTESIAN_POINT('Ctrl Pts',(-9.91775711673322,12.2,3.06258812646115));
#255433=CARTESIAN_POINT('Ctrl Pts',(-9.91545630147826,12.2,3.06164407508172));
#255434=CARTESIAN_POINT('Ctrl Pts',(-9.91324626500005,12.2,3.06074721299999));
#255435=CARTESIAN_POINT('Ctrl Pts',(-9.91324626500005,15.2,3.06074721299999));
#255436=CARTESIAN_POINT('Ctrl Pts',(-9.91490179640639,15.2,3.0614190495774));
#255437=CARTESIAN_POINT('Ctrl Pts',(-9.91660827013208,15.2,3.06211736672399));
#255438=CARTESIAN_POINT('Ctrl Pts',(-9.91836455129929,15.2,3.06284238742887));
#255439=CARTESIAN_POINT('Ctrl Pts',(-9.92012930214203,15.2,3.06357090455005));
#255440=CARTESIAN_POINT('Ctrl Pts',(-9.92194434197449,15.2,3.06432638668404));
#255441=CARTESIAN_POINT('Ctrl Pts',(-9.92380854792209,15.2,3.06510906085072));
#255442=CARTESIAN_POINT('Ctrl Pts',(-9.92567275370037,15.2,3.0658917349463));
#255443=CARTESIAN_POINT('Ctrl Pts',(-9.92758612406289,15.2,3.06670160226368));
#255444=CARTESIAN_POINT('Ctrl Pts',(-9.92954756824164,15.2,3.06753888023327));
#255445=CARTESIAN_POINT('Ctrl Pts',(-9.93150901242039,15.2,3.06837615820286));
#255446=CARTESIAN_POINT('Ctrl Pts',(-9.93351853346753,15.2,3.06924084660314));
#255447=CARTESIAN_POINT('Ctrl Pts',(-9.93557506757615,15.2,3.07013315544702));
#255448=CARTESIAN_POINT('Ctrl Pts',(-9.93763160187157,15.2,3.07102546437195));
#255449=CARTESIAN_POINT('Ctrl Pts',(-9.93973514987236,15.2,3.07194539273305));
#255450=CARTESIAN_POINT('Ctrl Pts',(-9.94188468124262,15.2,3.07289314078658));
#255451=CARTESIAN_POINT('Ctrl Pts',(-9.94439246754838,15.2,3.07399884671991));
#255452=CARTESIAN_POINT('Ctrl Pts',(-9.94696283892296,15.2,3.07514242100738));
#255453=CARTESIAN_POINT('Ctrl Pts',(-9.94959420704024,15.2,3.07632416439369));
#255454=CARTESIAN_POINT('Ctrl Pts',(-9.9518496656899,15.2,3.07733708741453));
#255455=CARTESIAN_POINT('Ctrl Pts',(-9.95414993737473,15.2,3.07837805331461));
#255456=CARTESIAN_POINT('Ctrl Pts',(-9.9564940500055,15.2,3.07944724612482));
#255457=CARTESIAN_POINT('Ctrl Pts',(-9.95883816242334,15.2,3.0805164388379));
#255458=CARTESIAN_POINT('Ctrl Pts',(-9.96122611435326,15.2,3.08161385563617));
#255459=CARTESIAN_POINT('Ctrl Pts',(-9.96365695802609,15.2,3.08273967526712));
#255460=CARTESIAN_POINT('Ctrl Pts',(-9.96608780169892,15.2,3.08386549489807));
#255461=CARTESIAN_POINT('Ctrl Pts',(-9.9685615367813,15.2,3.08501971462982));
#255462=CARTESIAN_POINT('Ctrl Pts',(-9.97107723760472,15.2,3.08620250341892));
#255463=CARTESIAN_POINT('Ctrl Pts',(-9.97359293865666,15.2,3.08738529231547));
#255464=CARTESIAN_POINT('Ctrl Pts',(-9.97615060723048,15.2,3.0885966503239));
#255465=CARTESIAN_POINT('Ctrl Pts',(-9.97874933929158,15.2,3.08983673714344));
#255466=CARTESIAN_POINT('Ctrl Pts',(-9.98134807111662,15.2,3.09107682385034));
#255467=CARTESIAN_POINT('Ctrl Pts',(-9.98398786750849,15.2,3.09234563980833));
#255468=CARTESIAN_POINT('Ctrl Pts',(-9.98666784641287,15.2,3.09364333934578));
#255469=CARTESIAN_POINT('Ctrl Pts',(-9.98934782531727,15.2,3.09494103888323));
#255470=CARTESIAN_POINT('Ctrl Pts',(-9.99206798928508,15.2,3.09626762011837));
#255471=CARTESIAN_POINT('Ctrl Pts',(-9.99482747534976,15.2,3.09762323365117));
#255472=CARTESIAN_POINT('Ctrl Pts',(-9.99758696141443,15.2,3.09897884718398));
#255473=CARTESIAN_POINT('Ctrl Pts',(-10.0003857714381,15.2,3.10036348897419));
#255474=CARTESIAN_POINT('Ctrl Pts',(-10.0032230664157,15.2,3.1017773053375));
#255475=CARTESIAN_POINT('Ctrl Pts',(-10.0060603616511,15.2,3.10319112182923));
#255476=CARTESIAN_POINT('Ctrl Pts',(-10.0089361398819,15.2,3.10463410825712));
#255477=CARTESIAN_POINT('Ctrl Pts',(-10.0118495822089,15.2,3.10610640108863));
#255478=CARTESIAN_POINT('Ctrl Pts',(-10.0147630242714,15.2,3.10757869378641));
#255479=CARTESIAN_POINT('Ctrl Pts',(-10.0177141286141,15.2,3.10908029397352));
#255480=CARTESIAN_POINT('Ctrl Pts',(-10.0207020948373,15.2,3.11061133041661));
#255481=CARTESIAN_POINT('Ctrl Pts',(-10.0236900610605,15.2,3.1121423668597));
#255482=CARTESIAN_POINT('Ctrl Pts',(-10.026714888605,15.2,3.11370283811974));
#255483=CARTESIAN_POINT('Ctrl Pts',(-10.029775791908,15.2,3.11529286955996));
#255484=CARTESIAN_POINT('Ctrl Pts',(-10.0328366954891,15.2,3.11688290114462));
#255485=CARTESIAN_POINT('Ctrl Pts',(-10.0359336749653,15.2,3.11850249243209));
#255486=CARTESIAN_POINT('Ctrl Pts',(-10.0390659636375,15.2,3.12015176102328));
#255487=CARTESIAN_POINT('Ctrl Pts',(-10.0421982520253,15.2,3.12180102946465));
#255488=CARTESIAN_POINT('Ctrl Pts',(-10.0453658485088,15.2,3.12347997663689));
#255489=CARTESIAN_POINT('Ctrl Pts',(-10.0485680029902,15.2,3.12518871224916));
#255490=CARTESIAN_POINT('Ctrl Pts',(-10.0517701574717,15.2,3.12689744786143));
#255491=CARTESIAN_POINT('Ctrl Pts',(-10.0550068682063,15.2,3.12863597655681));
#255492=CARTESIAN_POINT('Ctrl Pts',(-10.0582774006685,15.2,3.13040440199052));
#255493=CARTESIAN_POINT('Ctrl Pts',(-10.0615479334278,15.2,3.13217282758486));
#255494=CARTESIAN_POINT('Ctrl Pts',(-10.0648522868641,15.2,3.13397115157582));
#255495=CARTESIAN_POINT('Ctrl Pts',(-10.0681897417979,15.2,3.13579947818521));
#255496=CARTESIAN_POINT('Ctrl Pts',(-10.0715271964287,15.2,3.13762780462852));
#255497=CARTESIAN_POINT('Ctrl Pts',(-10.074897751132,15.2,3.13948612996855));
#255498=CARTESIAN_POINT('Ctrl Pts',(-10.0783007007583,15.2,3.14137455723326));
#255499=CARTESIAN_POINT('Ctrl Pts',(-10.0817036503847,15.2,3.14326298449798));
#255500=CARTESIAN_POINT('Ctrl Pts',(-10.0851389938609,15.2,3.14518151107001));
#255501=CARTESIAN_POINT('Ctrl Pts',(-10.0886060406564,15.2,3.14713023059483));
#255502=CARTESIAN_POINT('Ctrl Pts',(-10.0914952464242,15.2,3.14875416359118));
#255503=CARTESIAN_POINT('Ctrl Pts',(-10.0944064663428,15.2,3.15039906414221));
#255504=CARTESIAN_POINT('Ctrl Pts',(-10.0973393103,15.2,3.15206498434944));
#255505=CARTESIAN_POINT('Ctrl Pts',(-10.1002721542572,15.2,3.15373090455667));
#255506=CARTESIAN_POINT('Ctrl Pts',(-10.1032266195011,15.2,3.15541784366724));
#255507=CARTESIAN_POINT('Ctrl Pts',(-10.1062023202639,15.2,3.15712585234669));
#255508=CARTESIAN_POINT('Ctrl Pts',(-10.1091780210266,15.2,3.15883386102613));
#255509=CARTESIAN_POINT('Ctrl Pts',(-10.1121749576847,15.2,3.16056293924108));
#255510=CARTESIAN_POINT('Ctrl Pts',(-10.1151927476984,15.2,3.16231313299898));
#255511=CARTESIAN_POINT('Ctrl Pts',(-10.118210537712,15.2,3.16406332675688));
#255512=CARTESIAN_POINT('Ctrl Pts',(-10.1212491828166,15.2,3.16583463838325));
#255513=CARTESIAN_POINT('Ctrl Pts',(-10.1243083069833,15.2,3.16762711275826));
#255514=CARTESIAN_POINT('Ctrl Pts',(-10.12736743115,15.2,3.16941958713328));
#255515=CARTESIAN_POINT('Ctrl Pts',(-10.1304470343987,15.2,3.17123322348144));
#255516=CARTESIAN_POINT('Ctrl Pts',(-10.13354674851,15.2,3.1730680662676));
#255517=CARTESIAN_POINT('Ctrl Pts',(-10.1366464626214,15.2,3.17490290905376));
#255518=CARTESIAN_POINT('Ctrl Pts',(-10.1397662852044,15.2,3.1767589591106));
#255519=CARTESIAN_POINT('Ctrl Pts',(-10.1429058554138,15.2,3.1786362568895));
#255520=CARTESIAN_POINT('Ctrl Pts',(-10.1460454256232,15.2,3.1805135546684));
#255521=CARTESIAN_POINT('Ctrl Pts',(-10.1492047427681,15.2,3.18241210039117));
#255522=CARTESIAN_POINT('Ctrl Pts',(-10.152383447908,15.2,3.18433193560062));
#255523=CARTESIAN_POINT('Ctrl Pts',(-10.1555621530479,15.2,3.18625177081007));
#255524=CARTESIAN_POINT('Ctrl Pts',(-10.1587602468726,15.2,3.18819289427828));
#255525=CARTESIAN_POINT('Ctrl Pts',(-10.1619773771735,15.2,3.19015534396115));
#255526=CARTESIAN_POINT('Ctrl Pts',(-10.1651945074745,15.2,3.19211779364402));
#255527=CARTESIAN_POINT('Ctrl Pts',(-10.168430672052,15.2,3.19410157105491));
#255528=CARTESIAN_POINT('Ctrl Pts',(-10.1716855249007,15.2,3.19610671202887));
#255529=CARTESIAN_POINT('Ctrl Pts',(-10.1749403777495,15.2,3.19811185300284));
#255530=CARTESIAN_POINT('Ctrl Pts',(-10.1782139201625,15.2,3.20013835541051));
#255531=CARTESIAN_POINT('Ctrl Pts',(-10.1815058064139,15.2,3.20218625805114));
#255532=CARTESIAN_POINT('Ctrl Pts',(-10.1847976923066,15.2,3.20423416046855));
#255533=CARTESIAN_POINT('Ctrl Pts',(-10.1881079253789,15.2,3.2063034610061));
#255534=CARTESIAN_POINT('Ctrl Pts',(-10.1914361660564,15.2,3.20839419348481));
#255535=CARTESIAN_POINT('Ctrl Pts',(-10.1947644070966,15.2,3.21048492619141));
#255536=CARTESIAN_POINT('Ctrl Pts',(-10.1981106542948,15.2,3.21259708975038));
#255537=CARTESIAN_POINT('Ctrl Pts',(-10.201474577835,15.2,3.21473071592919));
#255538=CARTESIAN_POINT('Ctrl Pts',(-10.2048385013752,15.2,3.216864342108));
#255539=CARTESIAN_POINT('Ctrl Pts',(-10.2082200995068,15.2,3.21901943262257));
#255540=CARTESIAN_POINT('Ctrl Pts',(-10.2116190440888,15.2,3.2211960162319));
#255541=CARTESIAN_POINT('Ctrl Pts',(-10.2163775665775,15.2,3.22424323333242));
#255542=CARTESIAN_POINT('Ctrl Pts',(-10.2211700890845,15.2,3.2273325767247));
#255543=CARTESIAN_POINT('Ctrl Pts',(-10.2259957249731,15.2,3.23046412498205));
#255544=CARTESIAN_POINT('Ctrl Pts',(-10.2294426076971,15.2,3.23270094513103));
#255545=CARTESIAN_POINT('Ctrl Pts',(-10.2329063843833,15.2,3.23495929677216));
#255546=CARTESIAN_POINT('Ctrl Pts',(-10.2363867389667,15.2,3.23723920850826));
#255547=CARTESIAN_POINT('Ctrl Pts',(-10.23986709355,15.2,3.23951912024437));
#255548=CARTESIAN_POINT('Ctrl Pts',(-10.2433640257081,15.2,3.2418205893017));
#255549=CARTESIAN_POINT('Ctrl Pts',(-10.2468772212103,15.2,3.2441436444512));
#255550=CARTESIAN_POINT('Ctrl Pts',(-10.2496877773822,15.2,3.24600208841888));
#255551=CARTESIAN_POINT('Ctrl Pts',(-10.2525087432196,15.2,3.24787434481106));
#255552=CARTESIAN_POINT('Ctrl Pts',(-10.2553399593204,15.2,3.24976042793323));
#255553=CARTESIAN_POINT('Ctrl Pts',(-10.2588789797358,15.2,3.25211803202867));
#255554=CARTESIAN_POINT('Ctrl Pts',(-10.2624340161231,15.2,3.25449723837101));
#255555=CARTESIAN_POINT('Ctrl Pts',(-10.2660047632746,15.2,3.2568980694109));
#255556=CARTESIAN_POINT('Ctrl Pts',(-10.2688613611515,15.2,3.25881873434749));
#255557=CARTESIAN_POINT('Ctrl Pts',(-10.2717280136849,15.2,3.26075324027506));
#255558=CARTESIAN_POINT('Ctrl Pts',(-10.2746045662436,15.2,3.26270159650126));
#255559=CARTESIAN_POINT('Ctrl Pts',(-10.2774811184105,15.2,3.26464995246201));
#255560=CARTESIAN_POINT('Ctrl Pts',(-10.2803675712281,15.2,3.2666121592287));
#255561=CARTESIAN_POINT('Ctrl Pts',(-10.2832637712682,15.2,3.26858822717685));
#255562=CARTESIAN_POINT('Ctrl Pts',(-10.2861599717028,15.2,3.27056429539425));
#255563=CARTESIAN_POINT('Ctrl Pts',(-10.2890659173939,15.2,3.27255422432683));
#255564=CARTESIAN_POINT('Ctrl Pts',(-10.291981459275,15.2,3.27455802449159));
#255565=CARTESIAN_POINT('Ctrl Pts',(-10.2948970011561,15.2,3.27656182465636));
#255566=CARTESIAN_POINT('Ctrl Pts',(-10.2978221372106,15.2,3.27857949547553));
#255567=CARTESIAN_POINT('Ctrl Pts',(-10.3007567192048,15.2,3.28061104636543));
#255568=CARTESIAN_POINT('Ctrl Pts',(-10.3036913007992,15.2,3.28264259697854));
#255569=CARTESIAN_POINT('Ctrl Pts',(-10.3066353289011,15.2,3.28468802705759));
#255570=CARTESIAN_POINT('Ctrl Pts',(-10.3095886525063,15.2,3.28674734623186));
#255571=CARTESIAN_POINT('Ctrl Pts',(-10.312541976514,15.2,3.28880666568672));
#255572=CARTESIAN_POINT('Ctrl Pts',(-10.315504597248,15.2,3.29087987424546));
#255573=CARTESIAN_POINT('Ctrl Pts',(-10.3184763672442,15.2,3.29296697908285));
#255574=CARTESIAN_POINT('Ctrl Pts',(-10.3214481368356,15.2,3.29505408363586));
#255575=CARTESIAN_POINT('Ctrl Pts',(-10.3244290566257,15.2,3.29715508371764));
#255576=CARTESIAN_POINT('Ctrl Pts',(-10.3274189795473,15.2,3.29926998954384));
#255577=CARTESIAN_POINT('Ctrl Pts',(-10.3304089028764,15.2,3.30138489565818));
#255578=CARTESIAN_POINT('Ctrl Pts',(-10.3334078306799,15.2,3.30351370493313));
#255579=CARTESIAN_POINT('Ctrl Pts',(-10.3364156181615,15.2,3.3056564271026));
#255580=CARTESIAN_POINT('Ctrl Pts',(-10.3394234052333,15.2,3.30779914898013));
#255581=CARTESIAN_POINT('Ctrl Pts',(-10.3424400511451,15.2,3.30995578118986));
#255582=CARTESIAN_POINT('Ctrl Pts',(-10.3454654147861,15.2,3.31212633178928));
#255583=CARTESIAN_POINT('Ctrl Pts',(-10.3484907788393,15.2,3.31429688268444));
#255584=CARTESIAN_POINT('Ctrl Pts',(-10.3515248598547,15.2,3.31648135171185));
#255585=CARTESIAN_POINT('Ctrl Pts',(-10.3545675164655,15.2,3.31867974522145));
#255586=CARTESIAN_POINT('Ctrl Pts',(-10.3591315009672,15.2,3.32197733518632));
#255587=CARTESIAN_POINT('Ctrl Pts',(-10.3637147797943,15.2,3.32530625355529));
#255588=CARTESIAN_POINT('Ctrl Pts',(-10.3683168814813,15.2,3.32866652144842));
#255589=CARTESIAN_POINT('Ctrl Pts',(-10.3721519663598,15.2,3.33146674479442));
#255590=CARTESIAN_POINT('Ctrl Pts',(-10.3760001236834,15.2,3.33428873678882));
#255591=CARTESIAN_POINT('Ctrl Pts',(-10.3798610820167,15.2,3.33713250852493));
#255592=CARTESIAN_POINT('Ctrl Pts',(-10.3829498488517,15.2,3.3394075260378));
#255593=CARTESIAN_POINT('Ctrl Pts',(-10.3860468104877,15.2,3.3416964817162));
#255594=CARTESIAN_POINT('Ctrl Pts',(-10.389151827991,15.2,3.34399938117647));
#255595=CARTESIAN_POINT('Ctrl Pts',(-10.3938093538231,15.2,3.34745373005311));
#255596=CARTESIAN_POINT('Ctrl Pts',(-10.3984850090923,15.2,3.35093944899316));
#255597=CARTESIAN_POINT('Ctrl Pts',(-10.4031783367559,15.2,3.35445655395008));
#255598=CARTESIAN_POINT('Ctrl Pts',(-10.4063072217228,15.2,3.35680129048154));
#255599=CARTESIAN_POINT('Ctrl Pts',(-10.4094439605215,15.2,3.35915997647408));
#255600=CARTESIAN_POINT('Ctrl Pts',(-10.4125884214859,15.2,3.36153261361201));
#255601=CARTESIAN_POINT('Ctrl Pts',(-10.4157328828787,15.2,3.36390525107321));
#255602=CARTESIAN_POINT('Ctrl Pts',(-10.4188850653795,15.2,3.36629184082924));
#255603=CARTESIAN_POINT('Ctrl Pts',(-10.4220448375105,15.2,3.36869238502657));
#255604=CARTESIAN_POINT('Ctrl Pts',(-10.425204609211,15.2,3.37109292889682));
#255605=CARTESIAN_POINT('Ctrl Pts',(-10.4283719699801,15.2,3.37350742790006));
#255606=CARTESIAN_POINT('Ctrl Pts',(-10.4315467894976,15.2,3.37593588431122));
#255607=CARTESIAN_POINT('Ctrl Pts',(-10.4347216094477,15.2,3.37836434105326));
#255608=CARTESIAN_POINT('Ctrl Pts',(-10.4379038865457,15.2,3.3808067540494));
#255609=CARTESIAN_POINT('Ctrl Pts',(-10.441093492775,15.2,3.38326312751659));
#255610=CARTESIAN_POINT('Ctrl Pts',(-10.4442830990044,15.2,3.38571950098379));
#255611=CARTESIAN_POINT('Ctrl Pts',(-10.4474800332957,15.2,3.38818983253317));
#255612=CARTESIAN_POINT('Ctrl Pts',(-10.4506841680822,15.2,3.39067412594779));
#255613=CARTESIAN_POINT('Ctrl Pts',(-10.4538883024322,15.2,3.39315841902392));
#255614=CARTESIAN_POINT('Ctrl Pts',(-10.4570996364978,15.2,3.39565667293709));
#255615=CARTESIAN_POINT('Ctrl Pts',(-10.460318043512,15.2,3.39816888811968));
#255616=CARTESIAN_POINT('Ctrl Pts',(-10.4643410526086,15.2,3.40130915735464));
#255617=CARTESIAN_POINT('Ctrl Pts',(-10.4683751125128,15.2,3.40447124263936));
#255618=CARTESIAN_POINT('Ctrl Pts',(-10.4724199752395,15.2,3.4076551452232));
#255619=CARTESIAN_POINT('Ctrl Pts',(-10.4756558655972,15.2,3.41020226742909));
#255620=CARTESIAN_POINT('Ctrl Pts',(-10.4788986713508,15.2,3.41276335327921));
#255621=CARTESIAN_POINT('Ctrl Pts',(-10.4821482668063,15.2,3.41533840142096));
#255622=CARTESIAN_POINT('Ctrl Pts',(-10.4853978618192,15.2,3.41791344921187));
#255623=CARTESIAN_POINT('Ctrl Pts',(-10.48865424527,15.2,3.42050245983154));
#255624=CARTESIAN_POINT('Ctrl Pts',(-10.491917295725,15.2,3.42310543422893));
#255625=CARTESIAN_POINT('Ctrl Pts',(-10.4951803466246,15.2,3.42570840898098));
#255626=CARTESIAN_POINT('Ctrl Pts',(-10.4984500630188,15.2,3.42832534704185));
#255627=CARTESIAN_POINT('Ctrl Pts',(-10.5017263227505,15.2,3.43095624737344));
#255628=CARTESIAN_POINT('Ctrl Pts',(-10.5050025820358,15.2,3.43358714734657));
#255629=CARTESIAN_POINT('Ctrl Pts',(-10.5082853834505,15.2,3.43623200882598));
#255630=CARTESIAN_POINT('Ctrl Pts',(-10.5115746065145,15.2,3.43889083377437));
#255631=CARTESIAN_POINT('Ctrl Pts',(-10.5148638300267,15.2,3.44154965908503));
#255632=CARTESIAN_POINT('Ctrl Pts',(-10.5181594741563,15.2,3.44422244537237));
#255633=CARTESIAN_POINT('Ctrl Pts',(-10.5214614190034,15.2,3.44690919218637));
#255634=CARTESIAN_POINT('Ctrl Pts',(-10.5247633634005,15.2,3.4495959386343));
#255635=CARTESIAN_POINT('Ctrl Pts',(-10.52807160805,15.2,3.45229664563806));
#255636=CARTESIAN_POINT('Ctrl Pts',(-10.5313860327774,15.2,3.45501131210608));
#255637=CARTESIAN_POINT('Ctrl Pts',(-10.5347004579565,15.2,3.45772597894398));
#255638=CARTESIAN_POINT('Ctrl Pts',(-10.5380210651709,15.2,3.46045460300166));
#255639=CARTESIAN_POINT('Ctrl Pts',(-10.541347732297,15.2,3.4631971857076));
#255640=CARTESIAN_POINT('Ctrl Pts',(-10.54467439897,15.2,3.46593976803986));
#255641=CARTESIAN_POINT('Ctrl Pts',(-10.5480071279777,15.2,3.46869630590821));
#255642=CARTESIAN_POINT('Ctrl Pts',(-10.5513458017042,15.2,3.47146679901363));
#255643=CARTESIAN_POINT('Ctrl Pts',(-10.5555191442034,15.2,3.4749299156785));
#255644=CARTESIAN_POINT('Ctrl Pts',(-10.5597017708714,15.2,3.47841483734146));
#255645=CARTESIAN_POINT('Ctrl Pts',(-10.5638934602468,15.2,3.48192155758459));
#255646=CARTESIAN_POINT('Ctrl Pts',(-10.5672468119299,15.2,3.48472693393199));
#255647=CARTESIAN_POINT('Ctrl Pts',(-10.5706059602331,15.2,3.48754626154025));
#255648=CARTESIAN_POINT('Ctrl Pts',(-10.5739707912502,15.2,3.49037953697335));
#255649=CARTESIAN_POINT('Ctrl Pts',(-10.5773356218088,15.2,3.49321281202042));
#255650=CARTESIAN_POINT('Ctrl Pts',(-10.5807061352802,15.2,3.4960600352508));
#255651=CARTESIAN_POINT('Ctrl Pts',(-10.584082216448,15.2,3.49892120301546));
#255652=CARTESIAN_POINT('Ctrl Pts',(-10.5874582980759,15.2,3.50178237116996));
#255653=CARTESIAN_POINT('Ctrl Pts',(-10.5908399465079,15.2,3.50465748509516));
#255654=CARTESIAN_POINT('Ctrl Pts',(-10.5942270494857,15.2,3.50754653921024));
#255655=CARTESIAN_POINT('Ctrl Pts',(-10.5984609279772,15.2,3.51115785665726));
#255656=CARTESIAN_POINT('Ctrl Pts',(-10.602703328461,15.2,3.51479095735461));
#255657=CARTESIAN_POINT('Ctrl Pts',(-10.6069540295031,15.2,3.51844583152242));
#255658=CARTESIAN_POINT('Ctrl Pts',(-10.6095044500357,15.2,3.52063875594344));
#255659=CARTESIAN_POINT('Ctrl Pts',(-10.6120578590762,15.2,3.52283952013017));
#255660=CARTESIAN_POINT('Ctrl Pts',(-10.614614210025,15.2,3.52504812100826));
#255661=CARTESIAN_POINT('Ctrl Pts',(-10.6171705609738,15.2,3.52725672188634));
#255662=CARTESIAN_POINT('Ctrl Pts',(-10.6197298519475,15.2,3.52947315910579));
#255663=CARTESIAN_POINT('Ctrl Pts',(-10.6222920384375,15.2,3.53169743152428));
#255664=CARTESIAN_POINT('Ctrl Pts',(-10.6248542249275,15.2,3.53392170394277));
#255665=CARTESIAN_POINT('Ctrl Pts',(-10.6274193061352,15.2,3.53615381175369));
#255666=CARTESIAN_POINT('Ctrl Pts',(-10.6299872347949,15.2,3.5383937522833));
#255667=CARTESIAN_POINT('Ctrl Pts',(-10.6325551634546,15.2,3.54063369281291));
#255668=CARTESIAN_POINT('Ctrl Pts',(-10.6351259392829,15.2,3.54288146640791));
#255669=CARTESIAN_POINT('Ctrl Pts',(-10.637699516439,15.2,3.54513707074155));
#255670=CARTESIAN_POINT('Ctrl Pts',(-10.6411309529588,15.2,3.54814454345958));
#255671=CARTESIAN_POINT('Ctrl Pts',(-10.6445673715569,15.2,3.55116593574284));
#255672=CARTESIAN_POINT('Ctrl Pts',(-10.6480086593,15.2,3.55420124574159));
#255673=CARTESIAN_POINT('Ctrl Pts',(-10.6505896248729,15.2,3.55647772803387));
#255674=CARTESIAN_POINT('Ctrl Pts',(-10.653173330379,15.2,3.55876203735084));
#255675=CARTESIAN_POINT('Ctrl Pts',(-10.6557597309515,15.2,3.56105417222522));
#255676=CARTESIAN_POINT('Ctrl Pts',(-10.658346131524,15.2,3.5633463070996));
#255677=CARTESIAN_POINT('Ctrl Pts',(-10.6609352262303,15.2,3.56564626722296));
#255678=CARTESIAN_POINT('Ctrl Pts',(-10.663526969432,15.2,3.56795404975351));
#255679=CARTESIAN_POINT('Ctrl Pts',(-10.6661187126336,15.2,3.57026183228405));
#255680=CARTESIAN_POINT('Ctrl Pts',(-10.6687131043286,15.2,3.57257743834558));
#255681=CARTESIAN_POINT('Ctrl Pts',(-10.6713100994422,15.2,3.57490086376009));
#255682=CARTESIAN_POINT('Ctrl Pts',(-10.6756384247888,15.2,3.57877323959165));
#255683=CARTESIAN_POINT('Ctrl Pts',(-10.6799739830493,15.2,3.58266733873398));
#255684=CARTESIAN_POINT('Ctrl Pts',(-10.6843165649237,15.2,3.58658314699608));
#255685=CARTESIAN_POINT('Ctrl Pts',(-10.686922114427,15.2,3.5889326322948));
#255686=CARTESIAN_POINT('Ctrl Pts',(-10.6895301923061,15.2,3.59128993327075));
#255687=CARTESIAN_POINT('Ctrl Pts',(-10.6921407543525,15.2,3.59365504753221));
#255688=CARTESIAN_POINT('Ctrl Pts',(-10.6964916899899,15.2,3.59759690363209));
#255689=CARTESIAN_POINT('Ctrl Pts',(-10.7008495273388,15.2,3.60156046047041));
#255690=CARTESIAN_POINT('Ctrl Pts',(-10.7052140589458,15.2,3.60554570572867));
#255691=CARTESIAN_POINT('Ctrl Pts',(-10.7078327785761,15.2,3.60793685349177));
#255692=CARTESIAN_POINT('Ctrl Pts',(-10.7104539082404,15.2,3.61033580879043));
#255693=CARTESIAN_POINT('Ctrl Pts',(-10.7130774052886,15.2,3.61274256905795));
#255694=CARTESIAN_POINT('Ctrl Pts',(-10.7157009018603,15.2,3.61514932888825));
#255695=CARTESIAN_POINT('Ctrl Pts',(-10.7183267652652,15.2,3.61756389310142));
#255696=CARTESIAN_POINT('Ctrl Pts',(-10.7209549512949,15.2,3.6199862585141));
#255697=CARTESIAN_POINT('Ctrl Pts',(-10.7244591991754,15.2,3.62321607891765));
#255698=CARTESIAN_POINT('Ctrl Pts',(-10.7279675751078,15.2,3.62645976929894));
#255699=CARTESIAN_POINT('Ctrl Pts',(-10.7314799797091,15.2,3.62971732097566));
#255700=CARTESIAN_POINT('Ctrl Pts',(-10.7341142837583,15.2,3.63216048528799));
#255701=CARTESIAN_POINT('Ctrl Pts',(-10.7367508527415,15.2,3.63461144712754));
#255702=CARTESIAN_POINT('Ctrl Pts',(-10.7393896438336,15.2,3.63707020152762));
#255703=CARTESIAN_POINT('Ctrl Pts',(-10.7420284344464,15.2,3.63952895548101));
#255704=CARTESIAN_POINT('Ctrl Pts',(-10.7446694469752,15.2,3.64199550427745));
#255705=CARTESIAN_POINT('Ctrl Pts',(-10.7473126387614,15.2,3.64446984272873));
#255706=CARTESIAN_POINT('Ctrl Pts',(-10.7499558305477,15.2,3.64694418118));
#255707=CARTESIAN_POINT('Ctrl Pts',(-10.7526012021013,15.2,3.64942630929459));
#255708=CARTESIAN_POINT('Ctrl Pts',(-10.755248709297,15.2,3.6519162245798));
#255709=CARTESIAN_POINT('Ctrl Pts',(-10.7578962164926,15.2,3.654406139865));
#255710=CARTESIAN_POINT('Ctrl Pts',(-10.7605458606131,15.2,3.6569038406743));
#255711=CARTESIAN_POINT('Ctrl Pts',(-10.763197599225,15.2,3.65940932545826));
#255712=CARTESIAN_POINT('Ctrl Pts',(-10.7676171637389,15.2,3.66358513358326));
#255713=CARTESIAN_POINT('Ctrl Pts',(-10.7720425447268,15.2,3.66778255927747));
#255714=CARTESIAN_POINT('Ctrl Pts',(-10.7764735492608,15.2,3.6720015890189));
#255715=CARTESIAN_POINT('Ctrl Pts',(-10.7791321518846,15.2,3.67453300677179));
#255716=CARTESIAN_POINT('Ctrl Pts',(-10.781792778599,15.2,3.6770722006953));
#255717=CARTESIAN_POINT('Ctrl Pts',(-10.7844553872643,15.2,3.67961916748929));
#255718=CARTESIAN_POINT('Ctrl Pts',(-10.7871179959296,15.2,3.68216613428328));
#255719=CARTESIAN_POINT('Ctrl Pts',(-10.7897825870065,15.2,3.68472087319786));
#255720=CARTESIAN_POINT('Ctrl Pts',(-10.7924491182011,15.2,3.68728338147908));
#255721=CARTESIAN_POINT('Ctrl Pts',(-10.7951156493957,15.2,3.68984588976029));
#255722=CARTESIAN_POINT('Ctrl Pts',(-10.7977841215485,15.2,3.69241616608266));
#255723=CARTESIAN_POINT('Ctrl Pts',(-10.8004544941596,15.2,3.69499420790458));
#255724=CARTESIAN_POINT('Ctrl Pts',(-10.8031248672557,15.2,3.69757225019485));
#255725=CARTESIAN_POINT('Ctrl Pts',(-10.8057971405108,15.2,3.70015805745401));
#255726=CARTESIAN_POINT('Ctrl Pts',(-10.808471272108,15.2,3.70275162529034));
#255727=CARTESIAN_POINT('Ctrl Pts',(-10.8120367800946,15.2,3.70620971495349));
#255728=CARTESIAN_POINT('Ctrl Pts',(-10.8156055917095,15.2,3.70968160165562));
#255729=CARTESIAN_POINT('Ctrl Pts',(-10.8191776064893,15.2,3.71316727449756));
#255730=CARTESIAN_POINT('Ctrl Pts',(-10.8218566176958,15.2,3.71578152924775));
#255731=CARTESIAN_POINT('Ctrl Pts',(-10.8245374312553,15.2,3.71840353850963));
#255732=CARTESIAN_POINT('Ctrl Pts',(-10.8272200099493,15.2,3.72103329924674));
#255733=CARTESIAN_POINT('Ctrl Pts',(-10.8299025886434,15.2,3.72366305998386));
#255734=CARTESIAN_POINT('Ctrl Pts',(-10.832586932979,15.2,3.72630057042044));
#255735=CARTESIAN_POINT('Ctrl Pts',(-10.8352730049228,15.2,3.7289458286566));
#255736=CARTESIAN_POINT('Ctrl Pts',(-10.8379590773546,15.2,3.73159108737332));
#255737=CARTESIAN_POINT('Ctrl Pts',(-10.8406468747119,15.2,3.7342440923089));
#255738=CARTESIAN_POINT('Ctrl Pts',(-10.843336351103,15.2,3.73690483861332));
#255739=CARTESIAN_POINT('Ctrl Pts',(-10.8460258270055,15.2,3.73956558443437));
#255740=CARTESIAN_POINT('Ctrl Pts',(-10.8487169788175,15.2,3.74223407201378));
#255741=CARTESIAN_POINT('Ctrl Pts',(-10.8514097638127,15.2,3.74491029600946));
#255742=CARTESIAN_POINT('Ctrl Pts',(-10.8541025488079,15.2,3.74758652000514));
#255743=CARTESIAN_POINT('Ctrl Pts',(-10.8567969674967,15.2,3.75027048009548));
#255744=CARTESIAN_POINT('Ctrl Pts',(-10.859493000351,15.2,3.75296217351306));
#255745=CARTESIAN_POINT('Ctrl Pts',(-10.8621890332054,15.2,3.75565386693064));
#255746=CARTESIAN_POINT('Ctrl Pts',(-10.8648866835097,15.2,3.75835329050819));
#255747=CARTESIAN_POINT('Ctrl Pts',(-10.8675859440001,15.2,3.76106045599998));
#255748=CARTESIAN_POINT('Origin',(-5.66257110645729E-14,15.2,-1.77635683940025E-14));
#255749=CARTESIAN_POINT('',(-10.0330625580001,15.2,2.64164356399998));
#255750=CARTESIAN_POINT('',(-10.0330625580001,12.2,2.64164356399998));
#255751=CARTESIAN_POINT('',(-10.0330625580001,15.2,2.64164356399998));
#255752=CARTESIAN_POINT('Origin',(-5.66257110645729E-14,12.2,-1.77635683940025E-14));
#255753=CARTESIAN_POINT('Origin',(-5.66257110645729E-14,15.2,-1.77635683940025E-14));
#255754=CARTESIAN_POINT('Origin',(-5.66257110645729E-14,15.2,-1.77635683940025E-14));
#255755=CARTESIAN_POINT('',(-11.213356592485,15.2,2.55159438995864));
#255756=CARTESIAN_POINT('',(-11.292224299446,15.2,2.17615954695745));
#255757=CARTESIAN_POINT('Origin',(-5.66257110645729E-14,15.2,-1.77635683940025E-14));
#255758=CARTESIAN_POINT('',(-11.292224299446,12.2,2.17615954695745));
#255759=CARTESIAN_POINT('',(-11.2922243000001,15.2,2.17615954699999));
#255760=CARTESIAN_POINT('',(-11.213356592485,12.2,2.55159438995864));
#255761=CARTESIAN_POINT('Origin',(-5.66257110645729E-14,12.2,-1.77635683940025E-14));
#255762=CARTESIAN_POINT('',(-11.2133565930001,15.2,2.55159438999998));
#255763=CARTESIAN_POINT('Ctrl Pts',(-11.2922242990001,15.2,2.17615954699999));
#255764=CARTESIAN_POINT('Ctrl Pts',(-11.2922242990001,11.6,2.17615954699998));
#255765=CARTESIAN_POINT('Ctrl Pts',(-11.2916128880001,15.2,2.17570045599999));
#255766=CARTESIAN_POINT('Ctrl Pts',(-11.2916128880001,11.6,2.17570045599999));
#255767=CARTESIAN_POINT('Ctrl Pts',(-11.2903902450001,15.2,2.17478276599998));
#255768=CARTESIAN_POINT('Ctrl Pts',(-11.2903902450001,11.6,2.17478276599998));
#255769=CARTESIAN_POINT('Ctrl Pts',(-11.2885568210001,15.2,2.17340771699998));
#255770=CARTESIAN_POINT('Ctrl Pts',(-11.2885568210001,11.6,2.17340771699998));
#255771=CARTESIAN_POINT('Ctrl Pts',(-11.2861133340001,15.2,2.17157728699998));
#255772=CARTESIAN_POINT('Ctrl Pts',(-11.2861133340001,11.6,2.17157728699998));
#255773=CARTESIAN_POINT('Ctrl Pts',(-11.2830607740001,15.2,2.16929420299998));
#255774=CARTESIAN_POINT('Ctrl Pts',(-11.2830607740001,11.6,2.16929420299998));
#255775=CARTESIAN_POINT('Ctrl Pts',(-11.2800100150001,15.2,2.16701606599999));
#255776=CARTESIAN_POINT('Ctrl Pts',(-11.2800100150001,11.6,2.16701606599999));
#255777=CARTESIAN_POINT('Ctrl Pts',(-11.2769610580001,15.2,2.16474288099999));
#255778=CARTESIAN_POINT('Ctrl Pts',(-11.2769610580001,11.6,2.16474288099999));
#255779=CARTESIAN_POINT('Ctrl Pts',(-11.2739139080001,15.2,2.16247464499999));
#255780=CARTESIAN_POINT('Ctrl Pts',(-11.2739139080001,11.6,2.16247464499998));
#255781=CARTESIAN_POINT('Ctrl Pts',(-11.2708685710001,15.2,2.16021135999998));
#255782=CARTESIAN_POINT('Ctrl Pts',(-11.2708685710001,11.6,2.16021135999998));
#255783=CARTESIAN_POINT('Ctrl Pts',(-11.2678250540001,15.2,2.15795302499998));
#255784=CARTESIAN_POINT('Ctrl Pts',(-11.2678250540001,11.6,2.15795302499998));
#255785=CARTESIAN_POINT('Ctrl Pts',(-11.2647833690001,15.2,2.15569963899998));
#255786=CARTESIAN_POINT('Ctrl Pts',(-11.2647833690001,11.6,2.15569963899998));
#255787=CARTESIAN_POINT('Ctrl Pts',(-11.2617435240001,15.2,2.15345120199999));
#255788=CARTESIAN_POINT('Ctrl Pts',(-11.2617435240001,11.6,2.15345120199998));
#255789=CARTESIAN_POINT('Ctrl Pts',(-11.2587055320001,15.2,2.15120771399999));
#255790=CARTESIAN_POINT('Ctrl Pts',(-11.2587055320001,11.6,2.15120771399999));
#255791=CARTESIAN_POINT('Ctrl Pts',(-11.2556694030001,15.2,2.14896917499999));
#255792=CARTESIAN_POINT('Ctrl Pts',(-11.2556694030001,11.6,2.14896917499999));
#255793=CARTESIAN_POINT('Ctrl Pts',(-11.2526351490001,15.2,2.14673558399999));
#255794=CARTESIAN_POINT('Ctrl Pts',(-11.2526351490001,11.6,2.14673558399999));
#255795=CARTESIAN_POINT('Ctrl Pts',(-11.2496027780001,15.2,2.14450693999999));
#255796=CARTESIAN_POINT('Ctrl Pts',(-11.2496027780001,11.6,2.14450693999999));
#255797=CARTESIAN_POINT('Ctrl Pts',(-11.2465723000001,15.2,2.14228324399999));
#255798=CARTESIAN_POINT('Ctrl Pts',(-11.2465723000001,11.6,2.14228324399999));
#255799=CARTESIAN_POINT('Ctrl Pts',(-11.2435437210001,15.2,2.14006449399998));
#255800=CARTESIAN_POINT('Ctrl Pts',(-11.2435437210001,11.6,2.14006449399998));
#255801=CARTESIAN_POINT('Ctrl Pts',(-11.2405170510001,15.2,2.13785069299998));
#255802=CARTESIAN_POINT('Ctrl Pts',(-11.2405170510001,11.6,2.13785069299998));
#255803=CARTESIAN_POINT('Ctrl Pts',(-11.2374922970001,15.2,2.13564183799999));
#255804=CARTESIAN_POINT('Ctrl Pts',(-11.2374922970001,11.6,2.13564183799999));
#255805=CARTESIAN_POINT('Ctrl Pts',(-11.2344694690001,15.2,2.13343792899999));
#255806=CARTESIAN_POINT('Ctrl Pts',(-11.2344694690001,11.6,2.13343792899999));
#255807=CARTESIAN_POINT('Ctrl Pts',(-11.2314485750001,15.2,2.13123896599999));
#255808=CARTESIAN_POINT('Ctrl Pts',(-11.2314485750001,11.6,2.13123896599999));
#255809=CARTESIAN_POINT('Ctrl Pts',(-11.2284296250001,15.2,2.12904494799998));
#255810=CARTESIAN_POINT('Ctrl Pts',(-11.2284296250001,11.6,2.12904494799998));
#255811=CARTESIAN_POINT('Ctrl Pts',(-11.2254126260001,15.2,2.12685587499998));
#255812=CARTESIAN_POINT('Ctrl Pts',(-11.2254126260001,11.6,2.12685587499998));
#255813=CARTESIAN_POINT('Ctrl Pts',(-11.2223975920001,15.2,2.12467174699999));
#255814=CARTESIAN_POINT('Ctrl Pts',(-11.2223975920001,11.6,2.12467174699999));
#255815=CARTESIAN_POINT('Ctrl Pts',(-11.2193845280001,15.2,2.12249256399998));
#255816=CARTESIAN_POINT('Ctrl Pts',(-11.2193845280001,11.6,2.12249256399998));
#255817=CARTESIAN_POINT('Ctrl Pts',(-11.2163734460001,15.2,2.12031832499999));
#255818=CARTESIAN_POINT('Ctrl Pts',(-11.2163734460001,11.6,2.12031832499999));
#255819=CARTESIAN_POINT('Ctrl Pts',(-11.2133643550001,15.2,2.11814902899999));
#255820=CARTESIAN_POINT('Ctrl Pts',(-11.2133643550001,11.6,2.11814902899999));
#255821=CARTESIAN_POINT('Ctrl Pts',(-11.2103572640001,15.2,2.11598467699998));
#255822=CARTESIAN_POINT('Ctrl Pts',(-11.2103572640001,11.6,2.11598467699998));
#255823=CARTESIAN_POINT('Ctrl Pts',(-11.2073521820001,15.2,2.11382526699999));
#255824=CARTESIAN_POINT('Ctrl Pts',(-11.2073521820001,11.6,2.11382526699999));
#255825=CARTESIAN_POINT('Ctrl Pts',(-11.2043491170001,15.2,2.11167079899999));
#255826=CARTESIAN_POINT('Ctrl Pts',(-11.2043491170001,11.6,2.11167079899999));
#255827=CARTESIAN_POINT('Ctrl Pts',(-11.2013480790001,15.2,2.10952127399999));
#255828=CARTESIAN_POINT('Ctrl Pts',(-11.2013480790001,11.6,2.10952127399999));
#255829=CARTESIAN_POINT('Ctrl Pts',(-11.1983490770001,15.2,2.10737668999998));
#255830=CARTESIAN_POINT('Ctrl Pts',(-11.1983490770001,11.6,2.10737668999998));
#255831=CARTESIAN_POINT('Ctrl Pts',(-11.1953521200001,15.2,2.10523704699999));
#255832=CARTESIAN_POINT('Ctrl Pts',(-11.1953521200001,11.6,2.10523704699999));
#255833=CARTESIAN_POINT('Ctrl Pts',(-11.1923572190001,15.2,2.10310234499998));
#255834=CARTESIAN_POINT('Ctrl Pts',(-11.1923572190001,11.6,2.10310234499998));
#255835=CARTESIAN_POINT('Ctrl Pts',(-11.1893643810001,15.2,2.10097258199998));
#255836=CARTESIAN_POINT('Ctrl Pts',(-11.1893643810001,11.6,2.10097258199998));
#255837=CARTESIAN_POINT('Ctrl Pts',(-11.1863736160001,15.2,2.09884775999999));
#255838=CARTESIAN_POINT('Ctrl Pts',(-11.1863736160001,11.6,2.09884775999999));
#255839=CARTESIAN_POINT('Ctrl Pts',(-11.1833849350001,15.2,2.09672787599999));
#255840=CARTESIAN_POINT('Ctrl Pts',(-11.1833849350001,11.6,2.09672787599999));
#255841=CARTESIAN_POINT('Ctrl Pts',(-11.1803983470001,15.2,2.09461293099999));
#255842=CARTESIAN_POINT('Ctrl Pts',(-11.1803983470001,11.6,2.09461293099999));
#255843=CARTESIAN_POINT('Ctrl Pts',(-11.1774138590001,15.2,2.09250292499998));
#255844=CARTESIAN_POINT('Ctrl Pts',(-11.1774138590001,11.6,2.09250292499998));
#255845=CARTESIAN_POINT('Ctrl Pts',(-11.1744314830001,15.2,2.09039785499999));
#255846=CARTESIAN_POINT('Ctrl Pts',(-11.1744314830001,11.6,2.09039785499999));
#255847=CARTESIAN_POINT('Ctrl Pts',(-11.1714512270001,15.2,2.08829772299998));
#255848=CARTESIAN_POINT('Ctrl Pts',(-11.1714512270001,11.6,2.08829772299998));
#255849=CARTESIAN_POINT('Ctrl Pts',(-11.1684731010001,15.2,2.08620252799999));
#255850=CARTESIAN_POINT('Ctrl Pts',(-11.1684731010001,11.6,2.08620252799998));
#255851=CARTESIAN_POINT('Ctrl Pts',(-11.1654971140001,15.2,2.08411226799999));
#255852=CARTESIAN_POINT('Ctrl Pts',(-11.1654971140001,11.6,2.08411226799999));
#255853=CARTESIAN_POINT('Ctrl Pts',(-11.1625232760001,15.2,2.08202694399999));
#255854=CARTESIAN_POINT('Ctrl Pts',(-11.1625232760001,11.6,2.08202694399999));
#255855=CARTESIAN_POINT('Ctrl Pts',(-11.1595515960001,15.2,2.07994655599999));
#255856=CARTESIAN_POINT('Ctrl Pts',(-11.1595515960001,11.6,2.07994655599998));
#255857=CARTESIAN_POINT('Ctrl Pts',(-11.1565820830001,15.2,2.07787110099999));
#255858=CARTESIAN_POINT('Ctrl Pts',(-11.1565820830001,11.6,2.07787110099999));
#255859=CARTESIAN_POINT('Ctrl Pts',(-11.1536147480001,15.2,2.07580057999999));
#255860=CARTESIAN_POINT('Ctrl Pts',(-11.1536147480001,11.6,2.07580057999999));
#255861=CARTESIAN_POINT('Ctrl Pts',(-11.1506495990001,15.2,2.07373499299999));
#255862=CARTESIAN_POINT('Ctrl Pts',(-11.1506495990001,11.6,2.07373499299999));
#255863=CARTESIAN_POINT('Ctrl Pts',(-11.1476866470001,15.2,2.07167433799999));
#255864=CARTESIAN_POINT('Ctrl Pts',(-11.1476866470001,11.6,2.07167433799999));
#255865=CARTESIAN_POINT('Ctrl Pts',(-11.1447259000001,15.2,2.06961861399999));
#255866=CARTESIAN_POINT('Ctrl Pts',(-11.1447259000001,11.6,2.06961861399999));
#255867=CARTESIAN_POINT('Ctrl Pts',(-11.1417673690001,15.2,2.06756782399999));
#255868=CARTESIAN_POINT('Ctrl Pts',(-11.1417673690001,11.6,2.06756782399998));
#255869=CARTESIAN_POINT('Ctrl Pts',(-11.1388110630001,15.2,2.06552196299999));
#255870=CARTESIAN_POINT('Ctrl Pts',(-11.1388110630001,11.6,2.06552196299999));
#255871=CARTESIAN_POINT('Ctrl Pts',(-11.1358569910001,15.2,2.06348103199999));
#255872=CARTESIAN_POINT('Ctrl Pts',(-11.1358569910001,11.6,2.06348103199998));
#255873=CARTESIAN_POINT('Ctrl Pts',(-11.1329051630001,15.2,2.06144503099999));
#255874=CARTESIAN_POINT('Ctrl Pts',(-11.1329051630001,11.6,2.06144503099999));
#255875=CARTESIAN_POINT('Ctrl Pts',(-11.1299555890001,15.2,2.05941395899998));
#255876=CARTESIAN_POINT('Ctrl Pts',(-11.1299555890001,11.6,2.05941395899998));
#255877=CARTESIAN_POINT('Ctrl Pts',(-11.1270082780001,15.2,2.05738781699999));
#255878=CARTESIAN_POINT('Ctrl Pts',(-11.1270082780001,11.6,2.05738781699999));
#255879=CARTESIAN_POINT('Ctrl Pts',(-11.1240632410001,15.2,2.05536660099999));
#255880=CARTESIAN_POINT('Ctrl Pts',(-11.1240632410001,11.6,2.05536660099999));
#255881=CARTESIAN_POINT('Ctrl Pts',(-11.1211204850001,15.2,2.05335031099999));
#255882=CARTESIAN_POINT('Ctrl Pts',(-11.1211204850001,11.6,2.05335031099999));
#255883=CARTESIAN_POINT('Ctrl Pts',(-11.1181800230001,15.2,2.05133894799999));
#255884=CARTESIAN_POINT('Ctrl Pts',(-11.1181800230001,11.6,2.05133894799999));
#255885=CARTESIAN_POINT('Ctrl Pts',(-11.1152418620001,15.2,2.04933251099999));
#255886=CARTESIAN_POINT('Ctrl Pts',(-11.1152418620001,11.6,2.04933251099999));
#255887=CARTESIAN_POINT('Ctrl Pts',(-11.1123060130001,15.2,2.04733099899999));
#255888=CARTESIAN_POINT('Ctrl Pts',(-11.1123060130001,11.6,2.04733099899999));
#255889=CARTESIAN_POINT('Ctrl Pts',(-11.1093724870001,15.2,2.04533441099999));
#255890=CARTESIAN_POINT('Ctrl Pts',(-11.1093724870001,11.6,2.04533441099999));
#255891=CARTESIAN_POINT('Ctrl Pts',(-11.1064412920001,15.2,2.04334274599999));
#255892=CARTESIAN_POINT('Ctrl Pts',(-11.1064412920001,11.6,2.04334274599998));
#255893=CARTESIAN_POINT('Ctrl Pts',(-11.1035124380001,15.2,2.04135600499999));
#255894=CARTESIAN_POINT('Ctrl Pts',(-11.1035124380001,11.6,2.04135600499999));
#255895=CARTESIAN_POINT('Ctrl Pts',(-11.1005859330001,15.2,2.03937418499998));
#255896=CARTESIAN_POINT('Ctrl Pts',(-11.1005859330001,11.6,2.03937418499998));
#255897=CARTESIAN_POINT('Ctrl Pts',(-11.0976617910001,15.2,2.03739728599999));
#255898=CARTESIAN_POINT('Ctrl Pts',(-11.0976617910001,11.6,2.03739728599999));
#255899=CARTESIAN_POINT('Ctrl Pts',(-11.0947400190001,15.2,2.03542530799998));
#255900=CARTESIAN_POINT('Ctrl Pts',(-11.0947400190001,11.6,2.03542530799998));
#255901=CARTESIAN_POINT('Ctrl Pts',(-11.0918206280001,15.2,2.03345824899999));
#255902=CARTESIAN_POINT('Ctrl Pts',(-11.0918206280001,11.6,2.03345824899999));
#255903=CARTESIAN_POINT('Ctrl Pts',(-11.0889036270001,15.2,2.03149611099999));
#255904=CARTESIAN_POINT('Ctrl Pts',(-11.0889036270001,11.6,2.03149611099999));
#255905=CARTESIAN_POINT('Ctrl Pts',(-11.0859890260001,15.2,2.02953888899998));
#255906=CARTESIAN_POINT('Ctrl Pts',(-11.0859890260001,11.6,2.02953888899998));
#255907=CARTESIAN_POINT('Ctrl Pts',(-11.0830768350001,15.2,2.02758658599999));
#255908=CARTESIAN_POINT('Ctrl Pts',(-11.0830768350001,11.6,2.02758658599999));
#255909=CARTESIAN_POINT('Ctrl Pts',(-11.0801670650001,15.2,2.02563919799998));
#255910=CARTESIAN_POINT('Ctrl Pts',(-11.0801670650001,11.6,2.02563919799998));
#255911=CARTESIAN_POINT('Ctrl Pts',(-11.0772597250001,15.2,2.02369672799998));
#255912=CARTESIAN_POINT('Ctrl Pts',(-11.0772597250001,11.6,2.02369672799998));
#255913=CARTESIAN_POINT('Ctrl Pts',(-11.0743548250001,15.2,2.02175917099999));
#255914=CARTESIAN_POINT('Ctrl Pts',(-11.0743548250001,11.6,2.02175917099999));
#255915=CARTESIAN_POINT('Ctrl Pts',(-11.0714523740001,15.2,2.01982652899999));
#255916=CARTESIAN_POINT('Ctrl Pts',(-11.0714523740001,11.6,2.01982652899999));
#255917=CARTESIAN_POINT('Ctrl Pts',(-11.0685523830001,15.2,2.01789879999998));
#255918=CARTESIAN_POINT('Ctrl Pts',(-11.0685523830001,11.6,2.01789879999998));
#255919=CARTESIAN_POINT('Ctrl Pts',(-11.0656548630001,15.2,2.01597598299998));
#255920=CARTESIAN_POINT('Ctrl Pts',(-11.0656548630001,11.6,2.01597598299998));
#255921=CARTESIAN_POINT('Ctrl Pts',(-11.0627598220001,15.2,2.01405807899999));
#255922=CARTESIAN_POINT('Ctrl Pts',(-11.0627598220001,11.6,2.01405807899999));
#255923=CARTESIAN_POINT('Ctrl Pts',(-11.0598672710001,15.2,2.01214508499998));
#255924=CARTESIAN_POINT('Ctrl Pts',(-11.0598672710001,11.6,2.01214508499998));
#255925=CARTESIAN_POINT('Ctrl Pts',(-11.0569772200001,15.2,2.01023700099999));
#255926=CARTESIAN_POINT('Ctrl Pts',(-11.0569772200001,11.6,2.01023700099999));
#255927=CARTESIAN_POINT('Ctrl Pts',(-11.0540896800001,15.2,2.00833382599999));
#255928=CARTESIAN_POINT('Ctrl Pts',(-11.0540896800001,11.6,2.00833382599999));
#255929=CARTESIAN_POINT('Ctrl Pts',(-11.0512046610001,15.2,2.00643555899998));
#255930=CARTESIAN_POINT('Ctrl Pts',(-11.0512046610001,11.6,2.00643555899998));
#255931=CARTESIAN_POINT('Ctrl Pts',(-11.0483221710001,15.2,2.00454219899999));
#255932=CARTESIAN_POINT('Ctrl Pts',(-11.0483221710001,11.6,2.00454219899999));
#255933=CARTESIAN_POINT('Ctrl Pts',(-11.0454422220001,15.2,2.00265374599998));
#255934=CARTESIAN_POINT('Ctrl Pts',(-11.0454422220001,11.6,2.00265374599998));
#255935=CARTESIAN_POINT('Ctrl Pts',(-11.0425648240001,15.2,2.00077019799998));
#255936=CARTESIAN_POINT('Ctrl Pts',(-11.0425648240001,11.6,2.00077019799998));
#255937=CARTESIAN_POINT('Ctrl Pts',(-11.0396899870001,15.2,1.99889155399998));
#255938=CARTESIAN_POINT('Ctrl Pts',(-11.0396899870001,11.6,1.99889155399998));
#255939=CARTESIAN_POINT('Ctrl Pts',(-11.0368177200001,15.2,1.99701781299999));
#255940=CARTESIAN_POINT('Ctrl Pts',(-11.0368177200001,11.6,1.99701781299999));
#255941=CARTESIAN_POINT('Ctrl Pts',(-11.0339480350001,15.2,1.99514897599999));
#255942=CARTESIAN_POINT('Ctrl Pts',(-11.0339480350001,11.6,1.99514897599998));
#255943=CARTESIAN_POINT('Ctrl Pts',(-11.0310809420001,15.2,1.99328503899999));
#255944=CARTESIAN_POINT('Ctrl Pts',(-11.0310809420001,11.6,1.99328503899999));
#255945=CARTESIAN_POINT('Ctrl Pts',(-11.0282164510001,15.2,1.99142600399998));
#255946=CARTESIAN_POINT('Ctrl Pts',(-11.0282164510001,11.6,1.99142600399998));
#255947=CARTESIAN_POINT('Ctrl Pts',(-11.0253545710001,15.2,1.98957186699999));
#255948=CARTESIAN_POINT('Ctrl Pts',(-11.0253545710001,11.6,1.98957186699999));
#255949=CARTESIAN_POINT('Ctrl Pts',(-11.0224953140001,15.2,1.98772262999999));
#255950=CARTESIAN_POINT('Ctrl Pts',(-11.0224953140001,11.6,1.98772262999999));
#255951=CARTESIAN_POINT('Ctrl Pts',(-11.0196386900001,15.2,1.98587828999999));
#255952=CARTESIAN_POINT('Ctrl Pts',(-11.0196386900001,11.6,1.98587828999999));
#255953=CARTESIAN_POINT('Ctrl Pts',(-11.0167847080001,15.2,1.98403884699998));
#255954=CARTESIAN_POINT('Ctrl Pts',(-11.0167847080001,11.6,1.98403884699998));
#255955=CARTESIAN_POINT('Ctrl Pts',(-11.0139333790001,15.2,1.98220429899999));
#255956=CARTESIAN_POINT('Ctrl Pts',(-11.0139333790001,11.6,1.98220429899999));
#255957=CARTESIAN_POINT('Ctrl Pts',(-11.0110847150001,15.2,1.98037464599999));
#255958=CARTESIAN_POINT('Ctrl Pts',(-11.0110847150001,11.6,1.98037464599999));
#255959=CARTESIAN_POINT('Ctrl Pts',(-11.0082387250001,15.2,1.97854988499999));
#255960=CARTESIAN_POINT('Ctrl Pts',(-11.0082387250001,11.6,1.97854988499999));
#255961=CARTESIAN_POINT('Ctrl Pts',(-11.0053954180001,15.2,1.97673001799998));
#255962=CARTESIAN_POINT('Ctrl Pts',(-11.0053954180001,11.6,1.97673001799998));
#255963=CARTESIAN_POINT('Ctrl Pts',(-11.0025548070001,15.2,1.97491504299999));
#255964=CARTESIAN_POINT('Ctrl Pts',(-11.0025548070001,11.6,1.97491504299998));
#255965=CARTESIAN_POINT('Ctrl Pts',(-10.9997169010001,15.2,1.97310495599998));
#255966=CARTESIAN_POINT('Ctrl Pts',(-10.9997169010001,11.6,1.97310495599998));
#255967=CARTESIAN_POINT('Ctrl Pts',(-10.9968817120001,15.2,1.97129975899998));
#255968=CARTESIAN_POINT('Ctrl Pts',(-10.9968817120001,11.6,1.97129975899998));
#255969=CARTESIAN_POINT('Ctrl Pts',(-10.9940492480001,15.2,1.96949945099998));
#255970=CARTESIAN_POINT('Ctrl Pts',(-10.9940492480001,11.6,1.96949945099998));
#255971=CARTESIAN_POINT('Ctrl Pts',(-10.9912195210001,15.2,1.96770402999999));
#255972=CARTESIAN_POINT('Ctrl Pts',(-10.9912195210001,11.6,1.96770402999999));
#255973=CARTESIAN_POINT('Ctrl Pts',(-10.9883925420001,15.2,1.96591349399998));
#255974=CARTESIAN_POINT('Ctrl Pts',(-10.9883925420001,11.6,1.96591349399998));
#255975=CARTESIAN_POINT('Ctrl Pts',(-10.9855683200001,15.2,1.96412784299998));
#255976=CARTESIAN_POINT('Ctrl Pts',(-10.9855683200001,11.6,1.96412784299998));
#255977=CARTESIAN_POINT('Ctrl Pts',(-10.9827468670001,15.2,1.96234707499999));
#255978=CARTESIAN_POINT('Ctrl Pts',(-10.9827468670001,11.6,1.96234707499999));
#255979=CARTESIAN_POINT('Ctrl Pts',(-10.9799281930001,15.2,1.96057118999999));
#255980=CARTESIAN_POINT('Ctrl Pts',(-10.9799281930001,11.6,1.96057118999999));
#255981=CARTESIAN_POINT('Ctrl Pts',(-10.9771123080001,15.2,1.95880018599999));
#255982=CARTESIAN_POINT('Ctrl Pts',(-10.9771123080001,11.6,1.95880018599999));
#255983=CARTESIAN_POINT('Ctrl Pts',(-10.9742992230001,15.2,1.95703406199998));
#255984=CARTESIAN_POINT('Ctrl Pts',(-10.9742992230001,11.6,1.95703406199998));
#255985=CARTESIAN_POINT('Ctrl Pts',(-10.9714889500001,15.2,1.95527281799999));
#255986=CARTESIAN_POINT('Ctrl Pts',(-10.9714889500001,11.6,1.95527281799999));
#255987=CARTESIAN_POINT('Ctrl Pts',(-10.9686814980001,15.2,1.95351644999999));
#255988=CARTESIAN_POINT('Ctrl Pts',(-10.9686814980001,11.6,1.95351644999999));
#255989=CARTESIAN_POINT('Ctrl Pts',(-10.9658768780001,15.2,1.95176495999998));
#255990=CARTESIAN_POINT('Ctrl Pts',(-10.9658768780001,11.6,1.95176495999998));
#255991=CARTESIAN_POINT('Ctrl Pts',(-10.9630751010001,15.2,1.95001834399998));
#255992=CARTESIAN_POINT('Ctrl Pts',(-10.9630751010001,11.6,1.95001834399998));
#255993=CARTESIAN_POINT('Ctrl Pts',(-10.9602761780001,15.2,1.94827660199998));
#255994=CARTESIAN_POINT('Ctrl Pts',(-10.9602761780001,11.6,1.94827660199998));
#255995=CARTESIAN_POINT('Ctrl Pts',(-10.9574801190001,15.2,1.94653973399999));
#255996=CARTESIAN_POINT('Ctrl Pts',(-10.9574801190001,11.6,1.94653973399999));
#255997=CARTESIAN_POINT('Ctrl Pts',(-10.9546869340001,15.2,1.94480773699999));
#255998=CARTESIAN_POINT('Ctrl Pts',(-10.9546869340001,11.6,1.94480773699999));
#255999=CARTESIAN_POINT('Ctrl Pts',(-10.9518966360001,15.2,1.94308060999999));
#256000=CARTESIAN_POINT('Ctrl Pts',(-10.9518966360001,11.6,1.94308060999999));
#256001=CARTESIAN_POINT('Ctrl Pts',(-10.9491092350001,15.2,1.94135835299999));
#256002=CARTESIAN_POINT('Ctrl Pts',(-10.9491092350001,11.6,1.94135835299999));
#256003=CARTESIAN_POINT('Ctrl Pts',(-10.9463247410001,15.2,1.93964096299998));
#256004=CARTESIAN_POINT('Ctrl Pts',(-10.9463247410001,11.6,1.93964096299998));
#256005=CARTESIAN_POINT('Ctrl Pts',(-10.9435431660001,15.2,1.93792843899999));
#256006=CARTESIAN_POINT('Ctrl Pts',(-10.9435431660001,11.6,1.93792843899998));
#256007=CARTESIAN_POINT('Ctrl Pts',(-10.9407645200001,15.2,1.93622078099999));
#256008=CARTESIAN_POINT('Ctrl Pts',(-10.9407645200001,11.6,1.93622078099999));
#256009=CARTESIAN_POINT('Ctrl Pts',(-10.9379888140001,15.2,1.93451798599999));
#256010=CARTESIAN_POINT('Ctrl Pts',(-10.9379888140001,11.6,1.93451798599999));
#256011=CARTESIAN_POINT('Ctrl Pts',(-10.9352160590001,15.2,1.93282005499999));
#256012=CARTESIAN_POINT('Ctrl Pts',(-10.9352160590001,11.6,1.93282005499999));
#256013=CARTESIAN_POINT('Ctrl Pts',(-10.9324462660001,15.2,1.93112698299998));
#256014=CARTESIAN_POINT('Ctrl Pts',(-10.9324462660001,11.6,1.93112698299998));
#256015=CARTESIAN_POINT('Ctrl Pts',(-10.9296794470001,15.2,1.92943877199999));
#256016=CARTESIAN_POINT('Ctrl Pts',(-10.9296794470001,11.6,1.92943877199998));
#256017=CARTESIAN_POINT('Ctrl Pts',(-10.9269156100001,15.2,1.92775541899998));
#256018=CARTESIAN_POINT('Ctrl Pts',(-10.9269156100001,11.6,1.92775541899998));
#256019=CARTESIAN_POINT('Ctrl Pts',(-10.9241547690001,15.2,1.92607692399998));
#256020=CARTESIAN_POINT('Ctrl Pts',(-10.9241547690001,11.6,1.92607692399998));
#256021=CARTESIAN_POINT('Ctrl Pts',(-10.9213969330001,15.2,1.92440328399998));
#256022=CARTESIAN_POINT('Ctrl Pts',(-10.9213969330001,11.6,1.92440328399998));
#256023=CARTESIAN_POINT('Ctrl Pts',(-10.9186421150001,15.2,1.92273449799998));
#256024=CARTESIAN_POINT('Ctrl Pts',(-10.9186421150001,11.6,1.92273449799998));
#256025=CARTESIAN_POINT('Ctrl Pts',(-10.9158903240001,15.2,1.92107056499998));
#256026=CARTESIAN_POINT('Ctrl Pts',(-10.9158903240001,11.6,1.92107056499998));
#256027=CARTESIAN_POINT('Ctrl Pts',(-10.9131415730001,15.2,1.91941148499998));
#256028=CARTESIAN_POINT('Ctrl Pts',(-10.9131415730001,11.6,1.91941148499998));
#256029=CARTESIAN_POINT('Ctrl Pts',(-10.9103958720001,15.2,1.91775725399999));
#256030=CARTESIAN_POINT('Ctrl Pts',(-10.9103958720001,11.6,1.91775725399998));
#256031=CARTESIAN_POINT('Ctrl Pts',(-10.9076532320001,15.2,1.91610787099998));
#256032=CARTESIAN_POINT('Ctrl Pts',(-10.9076532320001,11.6,1.91610787099998));
#256033=CARTESIAN_POINT('Ctrl Pts',(-10.9049136650001,15.2,1.91446333499998));
#256034=CARTESIAN_POINT('Ctrl Pts',(-10.9049136650001,11.6,1.91446333499998));
#256035=CARTESIAN_POINT('Ctrl Pts',(-10.9021771820001,15.2,1.91282364399999));
#256036=CARTESIAN_POINT('Ctrl Pts',(-10.9021771820001,11.6,1.91282364399999));
#256037=CARTESIAN_POINT('Ctrl Pts',(-10.8994437930001,15.2,1.91118879899999));
#256038=CARTESIAN_POINT('Ctrl Pts',(-10.8994437930001,11.6,1.91118879899998));
#256039=CARTESIAN_POINT('Ctrl Pts',(-10.8967135100001,15.2,1.90955879499999));
#256040=CARTESIAN_POINT('Ctrl Pts',(-10.8967135100001,11.6,1.90955879499999));
#256041=CARTESIAN_POINT('Ctrl Pts',(-10.8939863450001,15.2,1.90793363399999));
#256042=CARTESIAN_POINT('Ctrl Pts',(-10.8939863450001,11.6,1.90793363399999));
#256043=CARTESIAN_POINT('Ctrl Pts',(-10.8912623070001,15.2,1.90631331199999));
#256044=CARTESIAN_POINT('Ctrl Pts',(-10.8912623070001,11.6,1.90631331199999));
#256045=CARTESIAN_POINT('Ctrl Pts',(-10.8885414100001,15.2,1.90469782799998));
#256046=CARTESIAN_POINT('Ctrl Pts',(-10.8885414100001,11.6,1.90469782799998));
#256047=CARTESIAN_POINT('Ctrl Pts',(-10.8858236640001,15.2,1.90308717999998));
#256048=CARTESIAN_POINT('Ctrl Pts',(-10.8858236640001,11.6,1.90308717999998));
#256049=CARTESIAN_POINT('Ctrl Pts',(-10.8831090800001,15.2,1.90148136799999));
#256050=CARTESIAN_POINT('Ctrl Pts',(-10.8831090800001,11.6,1.90148136799999));
#256051=CARTESIAN_POINT('Ctrl Pts',(-10.8803976700001,15.2,1.89988038899998));
#256052=CARTESIAN_POINT('Ctrl Pts',(-10.8803976700001,11.6,1.89988038899998));
#256053=CARTESIAN_POINT('Ctrl Pts',(-10.8776894460001,15.2,1.89828424199999));
#256054=CARTESIAN_POINT('Ctrl Pts',(-10.8776894460001,11.6,1.89828424199999));
#256055=CARTESIAN_POINT('Ctrl Pts',(-10.8749844180001,15.2,1.89669292499998));
#256056=CARTESIAN_POINT('Ctrl Pts',(-10.8749844180001,11.6,1.89669292499998));
#256057=CARTESIAN_POINT('Ctrl Pts',(-10.8722825980001,15.2,1.89510643799998));
#256058=CARTESIAN_POINT('Ctrl Pts',(-10.8722825980001,11.6,1.89510643799998));
#256059=CARTESIAN_POINT('Ctrl Pts',(-10.8695839980001,15.2,1.89352477599999));
#256060=CARTESIAN_POINT('Ctrl Pts',(-10.8695839980001,11.6,1.89352477599999));
#256061=CARTESIAN_POINT('Ctrl Pts',(-10.8668886270001,15.2,1.89194794099999));
#256062=CARTESIAN_POINT('Ctrl Pts',(-10.8668886270001,11.6,1.89194794099999));
#256063=CARTESIAN_POINT('Ctrl Pts',(-10.8641965010001,15.2,1.89037592899998));
#256064=CARTESIAN_POINT('Ctrl Pts',(-10.8641965010001,11.6,1.89037592899998));
#256065=CARTESIAN_POINT('Ctrl Pts',(-10.8615076260001,15.2,1.88880873999999));
#256066=CARTESIAN_POINT('Ctrl Pts',(-10.8615076260001,11.6,1.88880873999999));
#256067=CARTESIAN_POINT('Ctrl Pts',(-10.8588220190001,15.2,1.88724637099998));
#256068=CARTESIAN_POINT('Ctrl Pts',(-10.8588220190001,11.6,1.88724637099998));
#256069=CARTESIAN_POINT('Ctrl Pts',(-10.8561396880001,15.2,1.88568882099998));
#256070=CARTESIAN_POINT('Ctrl Pts',(-10.8561396880001,11.6,1.88568882099998));
#256071=CARTESIAN_POINT('Ctrl Pts',(-10.8534606450001,15.2,1.88413608899999));
#256072=CARTESIAN_POINT('Ctrl Pts',(-10.8534606450001,11.6,1.88413608899999));
#256073=CARTESIAN_POINT('Ctrl Pts',(-10.8507849030001,15.2,1.88258817099999));
#256074=CARTESIAN_POINT('Ctrl Pts',(-10.8507849030001,11.6,1.88258817099999));
#256075=CARTESIAN_POINT('Ctrl Pts',(-10.8481124720001,15.2,1.88104506799998));
#256076=CARTESIAN_POINT('Ctrl Pts',(-10.8481124720001,11.6,1.88104506799998));
#256077=CARTESIAN_POINT('Ctrl Pts',(-10.8454433650001,15.2,1.87950677599999));
#256078=CARTESIAN_POINT('Ctrl Pts',(-10.8454433650001,11.6,1.87950677599999));
#256079=CARTESIAN_POINT('Ctrl Pts',(-10.8427775930001,15.2,1.87797329499999));
#256080=CARTESIAN_POINT('Ctrl Pts',(-10.8427775930001,11.6,1.87797329499999));
#256081=CARTESIAN_POINT('Ctrl Pts',(-10.8401151680001,15.2,1.87644462199998));
#256082=CARTESIAN_POINT('Ctrl Pts',(-10.8401151680001,11.6,1.87644462199998));
#256083=CARTESIAN_POINT('Ctrl Pts',(-10.8374561020001,15.2,1.87492075599998));
#256084=CARTESIAN_POINT('Ctrl Pts',(-10.8374561020001,11.6,1.87492075599998));
#256085=CARTESIAN_POINT('Ctrl Pts',(-10.8348004050001,15.2,1.87340169499999));
#256086=CARTESIAN_POINT('Ctrl Pts',(-10.8348004050001,11.6,1.87340169499999));
#256087=CARTESIAN_POINT('Ctrl Pts',(-10.8321480920001,15.2,1.87188743799998));
#256088=CARTESIAN_POINT('Ctrl Pts',(-10.8321480920001,11.6,1.87188743799998));
#256089=CARTESIAN_POINT('Ctrl Pts',(-10.8294991720001,15.2,1.87037798199999));
#256090=CARTESIAN_POINT('Ctrl Pts',(-10.8294991720001,11.6,1.87037798199999));
#256091=CARTESIAN_POINT('Ctrl Pts',(-10.8268536570001,15.2,1.86887332499999));
#256092=CARTESIAN_POINT('Ctrl Pts',(-10.8268536570001,11.6,1.86887332499999));
#256093=CARTESIAN_POINT('Ctrl Pts',(-10.8242115600001,15.2,1.86737346599998));
#256094=CARTESIAN_POINT('Ctrl Pts',(-10.8242115600001,11.6,1.86737346599998));
#256095=CARTESIAN_POINT('Ctrl Pts',(-10.8215728930001,15.2,1.86587840299998));
#256096=CARTESIAN_POINT('Ctrl Pts',(-10.8215728930001,11.6,1.86587840299998));
#256097=CARTESIAN_POINT('Ctrl Pts',(-10.8189376670001,15.2,1.86438813399999));
#256098=CARTESIAN_POINT('Ctrl Pts',(-10.8189376670001,11.6,1.86438813399999));
#256099=CARTESIAN_POINT('Ctrl Pts',(-10.8163058940001,15.2,1.86290265699999));
#256100=CARTESIAN_POINT('Ctrl Pts',(-10.8163058940001,11.6,1.86290265699998));
#256101=CARTESIAN_POINT('Ctrl Pts',(-10.8136775860001,15.2,1.86142197099999));
#256102=CARTESIAN_POINT('Ctrl Pts',(-10.8136775860001,11.6,1.86142197099999));
#256103=CARTESIAN_POINT('Ctrl Pts',(-10.8110527560001,15.2,1.85994607399998));
#256104=CARTESIAN_POINT('Ctrl Pts',(-10.8110527560001,11.6,1.85994607399998));
#256105=CARTESIAN_POINT('Ctrl Pts',(-10.8084314150001,15.2,1.85847496199999));
#256106=CARTESIAN_POINT('Ctrl Pts',(-10.8084314150001,11.6,1.85847496199999));
#256107=CARTESIAN_POINT('Ctrl Pts',(-10.8058135750001,15.2,1.85700863499999));
#256108=CARTESIAN_POINT('Ctrl Pts',(-10.8058135750001,11.6,1.85700863499999));
#256109=CARTESIAN_POINT('Ctrl Pts',(-10.8031992490001,15.2,1.85554709099998));
#256110=CARTESIAN_POINT('Ctrl Pts',(-10.8031992490001,11.6,1.85554709099998));
#256111=CARTESIAN_POINT('Ctrl Pts',(-10.8005884480001,15.2,1.85409032699999));
#256112=CARTESIAN_POINT('Ctrl Pts',(-10.8005884480001,11.6,1.85409032699999));
#256113=CARTESIAN_POINT('Ctrl Pts',(-10.7979811840001,15.2,1.85263834199999));
#256114=CARTESIAN_POINT('Ctrl Pts',(-10.7979811840001,11.6,1.85263834199999));
#256115=CARTESIAN_POINT('Ctrl Pts',(-10.7953774700001,15.2,1.85119113499999));
#256116=CARTESIAN_POINT('Ctrl Pts',(-10.7953774700001,11.6,1.85119113499998));
#256117=CARTESIAN_POINT('Ctrl Pts',(-10.7927773170001,15.2,1.84974870099999));
#256118=CARTESIAN_POINT('Ctrl Pts',(-10.7927773170001,11.6,1.84974870099999));
#256119=CARTESIAN_POINT('Ctrl Pts',(-10.7901807400001,15.2,1.84831103999999));
#256120=CARTESIAN_POINT('Ctrl Pts',(-10.7901807400001,11.6,1.84831103999999));
#256121=CARTESIAN_POINT('Ctrl Pts',(-10.7875877470001,15.2,1.84687815099998));
#256122=CARTESIAN_POINT('Ctrl Pts',(-10.7875877470001,11.6,1.84687815099998));
#256123=CARTESIAN_POINT('Ctrl Pts',(-10.7849983530001,15.2,1.84545002999998));
#256124=CARTESIAN_POINT('Ctrl Pts',(-10.7849983530001,11.6,1.84545002999998));
#256125=CARTESIAN_POINT('Ctrl Pts',(-10.7824125710001,15.2,1.84402667599999));
#256126=CARTESIAN_POINT('Ctrl Pts',(-10.7824125710001,11.6,1.84402667599999));
#256127=CARTESIAN_POINT('Ctrl Pts',(-10.7798304100001,15.2,1.84260808499999));
#256128=CARTESIAN_POINT('Ctrl Pts',(-10.7798304100001,11.6,1.84260808499999));
#256129=CARTESIAN_POINT('Ctrl Pts',(-10.7772518860001,15.2,1.84119425799999));
#256130=CARTESIAN_POINT('Ctrl Pts',(-10.7772518860001,11.6,1.84119425799999));
#256131=CARTESIAN_POINT('Ctrl Pts',(-10.7746770080001,15.2,1.83978519099998));
#256132=CARTESIAN_POINT('Ctrl Pts',(-10.7746770080001,11.6,1.83978519099998));
#256133=CARTESIAN_POINT('Ctrl Pts',(-10.7721057910001,15.2,1.83838088299999));
#256134=CARTESIAN_POINT('Ctrl Pts',(-10.7721057910001,11.6,1.83838088299999));
#256135=CARTESIAN_POINT('Ctrl Pts',(-10.7695382460001,15.2,1.83698133099998));
#256136=CARTESIAN_POINT('Ctrl Pts',(-10.7695382460001,11.6,1.83698133099998));
#256137=CARTESIAN_POINT('Ctrl Pts',(-10.7669743860001,15.2,1.83558653199999));
#256138=CARTESIAN_POINT('Ctrl Pts',(-10.7669743860001,11.6,1.83558653199999));
#256139=CARTESIAN_POINT('Ctrl Pts',(-10.7644142240001,15.2,1.83419648599998));
#256140=CARTESIAN_POINT('Ctrl Pts',(-10.7644142240001,11.6,1.83419648599998));
#256141=CARTESIAN_POINT('Ctrl Pts',(-10.7618577700001,15.2,1.83281118899998));
#256142=CARTESIAN_POINT('Ctrl Pts',(-10.7618577700001,11.6,1.83281118899998));
#256143=CARTESIAN_POINT('Ctrl Pts',(-10.7593050390001,15.2,1.83143063999998));
#256144=CARTESIAN_POINT('Ctrl Pts',(-10.7593050390001,11.6,1.83143063999998));
#256145=CARTESIAN_POINT('Ctrl Pts',(-10.7567560430001,15.2,1.83005483699999));
#256146=CARTESIAN_POINT('Ctrl Pts',(-10.7567560430001,11.6,1.83005483699999));
#256147=CARTESIAN_POINT('Ctrl Pts',(-10.7542107950001,15.2,1.82868377599998));
#256148=CARTESIAN_POINT('Ctrl Pts',(-10.7542107950001,11.6,1.82868377599998));
#256149=CARTESIAN_POINT('Ctrl Pts',(-10.7516693050001,15.2,1.82731745599999));
#256150=CARTESIAN_POINT('Ctrl Pts',(-10.7516693050001,11.6,1.82731745599999));
#256151=CARTESIAN_POINT('Ctrl Pts',(-10.7491315890001,15.2,1.82595587599998));
#256152=CARTESIAN_POINT('Ctrl Pts',(-10.7491315890001,11.6,1.82595587599998));
#256153=CARTESIAN_POINT('Ctrl Pts',(-10.7465976590001,15.2,1.82459903199998));
#256154=CARTESIAN_POINT('Ctrl Pts',(-10.7465976590001,11.6,1.82459903199998));
#256155=CARTESIAN_POINT('Ctrl Pts',(-10.7440675260001,15.2,1.82324692199999));
#256156=CARTESIAN_POINT('Ctrl Pts',(-10.7440675260001,11.6,1.82324692199999));
#256157=CARTESIAN_POINT('Ctrl Pts',(-10.7415412030001,15.2,1.82189954399998));
#256158=CARTESIAN_POINT('Ctrl Pts',(-10.7415412030001,11.6,1.82189954399998));
#256159=CARTESIAN_POINT('Ctrl Pts',(-10.7390187040001,15.2,1.82055689499999));
#256160=CARTESIAN_POINT('Ctrl Pts',(-10.7390187040001,11.6,1.82055689499998));
#256161=CARTESIAN_POINT('Ctrl Pts',(-10.7365000410001,15.2,1.81921897399999));
#256162=CARTESIAN_POINT('Ctrl Pts',(-10.7365000410001,11.6,1.81921897399999));
#256163=CARTESIAN_POINT('Ctrl Pts',(-10.7339852270001,15.2,1.81788577899999));
#256164=CARTESIAN_POINT('Ctrl Pts',(-10.7339852270001,11.6,1.81788577899999));
#256165=CARTESIAN_POINT('Ctrl Pts',(-10.7314742750001,15.2,1.81655730499998));
#256166=CARTESIAN_POINT('Ctrl Pts',(-10.7314742750001,11.6,1.81655730499998));
#256167=CARTESIAN_POINT('Ctrl Pts',(-10.7289671960001,15.2,1.81523355299999));
#256168=CARTESIAN_POINT('Ctrl Pts',(-10.7289671960001,11.6,1.81523355299999));
#256169=CARTESIAN_POINT('Ctrl Pts',(-10.7264640050001,15.2,1.81391451699998));
#256170=CARTESIAN_POINT('Ctrl Pts',(-10.7264640050001,11.6,1.81391451699998));
#256171=CARTESIAN_POINT('Ctrl Pts',(-10.7239647150001,15.2,1.81260019699998));
#256172=CARTESIAN_POINT('Ctrl Pts',(-10.7239647150001,11.6,1.81260019699998));
#256173=CARTESIAN_POINT('Ctrl Pts',(-10.7214693390001,15.2,1.81129059099999));
#256174=CARTESIAN_POINT('Ctrl Pts',(-10.7214693390001,11.6,1.81129059099999));
#256175=CARTESIAN_POINT('Ctrl Pts',(-10.7189778870001,15.2,1.80998569599998));
#256176=CARTESIAN_POINT('Ctrl Pts',(-10.7189778870001,11.6,1.80998569599998));
#256177=CARTESIAN_POINT('Ctrl Pts',(-10.7164903760001,15.2,1.80868550799998));
#256178=CARTESIAN_POINT('Ctrl Pts',(-10.7164903760001,11.6,1.80868550799998));
#256179=CARTESIAN_POINT('Ctrl Pts',(-10.7140068170001,15.2,1.80739002699998));
#256180=CARTESIAN_POINT('Ctrl Pts',(-10.7140068170001,11.6,1.80739002699998));
#256181=CARTESIAN_POINT('Ctrl Pts',(-10.7115272230001,15.2,1.80609924899999));
#256182=CARTESIAN_POINT('Ctrl Pts',(-10.7115272230001,11.6,1.80609924899999));
#256183=CARTESIAN_POINT('Ctrl Pts',(-10.7090516070001,15.2,1.80481317199999));
#256184=CARTESIAN_POINT('Ctrl Pts',(-10.7090516070001,11.6,1.80481317199999));
#256185=CARTESIAN_POINT('Ctrl Pts',(-10.7065799830001,15.2,1.80353179299999));
#256186=CARTESIAN_POINT('Ctrl Pts',(-10.7065799830001,11.6,1.80353179299999));
#256187=CARTESIAN_POINT('Ctrl Pts',(-10.7041123640001,15.2,1.80225510999998));
#256188=CARTESIAN_POINT('Ctrl Pts',(-10.7041123640001,11.6,1.80225510999998));
#256189=CARTESIAN_POINT('Ctrl Pts',(-10.7016487620001,15.2,1.80098312099998));
#256190=CARTESIAN_POINT('Ctrl Pts',(-10.7016487620001,11.6,1.80098312099998));
#256191=CARTESIAN_POINT('Ctrl Pts',(-10.6991891910001,15.2,1.79971582199999));
#256192=CARTESIAN_POINT('Ctrl Pts',(-10.6991891910001,11.6,1.79971582199998));
#256193=CARTESIAN_POINT('Ctrl Pts',(-10.6967336660001,15.2,1.79845321199998));
#256194=CARTESIAN_POINT('Ctrl Pts',(-10.6967336660001,11.6,1.79845321199998));
#256195=CARTESIAN_POINT('Ctrl Pts',(-10.6942821970001,15.2,1.79719528699998));
#256196=CARTESIAN_POINT('Ctrl Pts',(-10.6942821970001,11.6,1.79719528699998));
#256197=CARTESIAN_POINT('Ctrl Pts',(-10.6918347990001,15.2,1.79594204599999));
#256198=CARTESIAN_POINT('Ctrl Pts',(-10.6918347990001,11.6,1.79594204599998));
#256199=CARTESIAN_POINT('Ctrl Pts',(-10.6893914850001,15.2,1.79469348499998));
#256200=CARTESIAN_POINT('Ctrl Pts',(-10.6893914850001,11.6,1.79469348499998));
#256201=CARTESIAN_POINT('Ctrl Pts',(-10.6869522690001,15.2,1.79344960299999));
#256202=CARTESIAN_POINT('Ctrl Pts',(-10.6869522690001,11.6,1.79344960299999));
#256203=CARTESIAN_POINT('Ctrl Pts',(-10.6845171640001,15.2,1.79221039399998));
#256204=CARTESIAN_POINT('Ctrl Pts',(-10.6845171640001,11.6,1.79221039399998));
#256205=CARTESIAN_POINT('Ctrl Pts',(-10.6820861830001,15.2,1.79097585899999));
#256206=CARTESIAN_POINT('Ctrl Pts',(-10.6820861830001,11.6,1.79097585899999));
#256207=CARTESIAN_POINT('Ctrl Pts',(-10.6796593400001,15.2,1.78974599499998));
#256208=CARTESIAN_POINT('Ctrl Pts',(-10.6796593400001,11.6,1.78974599499998));
#256209=CARTESIAN_POINT('Ctrl Pts',(-10.6772366490001,15.2,1.78852079599999));
#256210=CARTESIAN_POINT('Ctrl Pts',(-10.6772366490001,11.6,1.78852079599999));
#256211=CARTESIAN_POINT('Ctrl Pts',(-10.6748181230001,15.2,1.78730026299998));
#256212=CARTESIAN_POINT('Ctrl Pts',(-10.6748181230001,11.6,1.78730026299998));
#256213=CARTESIAN_POINT('Ctrl Pts',(-10.6724037740001,15.2,1.78608439099999));
#256214=CARTESIAN_POINT('Ctrl Pts',(-10.6724037740001,11.6,1.78608439099999));
#256215=CARTESIAN_POINT('Ctrl Pts',(-10.6699936180001,15.2,1.78487317899998));
#256216=CARTESIAN_POINT('Ctrl Pts',(-10.6699936180001,11.6,1.78487317899998));
#256217=CARTESIAN_POINT('Ctrl Pts',(-10.6675876670001,15.2,1.78366662199998));
#256218=CARTESIAN_POINT('Ctrl Pts',(-10.6675876670001,11.6,1.78366662199998));
#256219=CARTESIAN_POINT('Ctrl Pts',(-10.6651859350001,15.2,1.78246471899998));
#256220=CARTESIAN_POINT('Ctrl Pts',(-10.6651859350001,11.6,1.78246471899998));
#256221=CARTESIAN_POINT('Ctrl Pts',(-10.6627884370001,15.2,1.78126746699999));
#256222=CARTESIAN_POINT('Ctrl Pts',(-10.6627884370001,11.6,1.78126746699998));
#256223=CARTESIAN_POINT('Ctrl Pts',(-10.6603951850001,15.2,1.78007486299999));
#256224=CARTESIAN_POINT('Ctrl Pts',(-10.6603951850001,11.6,1.78007486299998));
#256225=CARTESIAN_POINT('Ctrl Pts',(-10.6580061940001,15.2,1.77888690299998));
#256226=CARTESIAN_POINT('Ctrl Pts',(-10.6580061940001,11.6,1.77888690299998));
#256227=CARTESIAN_POINT('Ctrl Pts',(-10.6556214770001,15.2,1.77770358699998));
#256228=CARTESIAN_POINT('Ctrl Pts',(-10.6556214770001,11.6,1.77770358699998));
#256229=CARTESIAN_POINT('Ctrl Pts',(-10.6532410480001,15.2,1.77652490999999));
#256230=CARTESIAN_POINT('Ctrl Pts',(-10.6532410480001,11.6,1.77652490999999));
#256231=CARTESIAN_POINT('Ctrl Pts',(-10.6508649200001,15.2,1.77535086899999));
#256232=CARTESIAN_POINT('Ctrl Pts',(-10.6508649200001,11.6,1.77535086899998));
#256233=CARTESIAN_POINT('Ctrl Pts',(-10.6484931090001,15.2,1.77418146099999));
#256234=CARTESIAN_POINT('Ctrl Pts',(-10.6484931090001,11.6,1.77418146099999));
#256235=CARTESIAN_POINT('Ctrl Pts',(-10.6461256270001,15.2,1.77301668399998));
#256236=CARTESIAN_POINT('Ctrl Pts',(-10.6461256270001,11.6,1.77301668399998));
#256237=CARTESIAN_POINT('Ctrl Pts',(-10.6437624890001,15.2,1.77185653499999));
#256238=CARTESIAN_POINT('Ctrl Pts',(-10.6437624890001,11.6,1.77185653499999));
#256239=CARTESIAN_POINT('Ctrl Pts',(-10.6414037090001,15.2,1.77070101099998));
#256240=CARTESIAN_POINT('Ctrl Pts',(-10.6414037090001,11.6,1.77070101099998));
#256241=CARTESIAN_POINT('Ctrl Pts',(-10.6390493000001,15.2,1.76955010999999));
#256242=CARTESIAN_POINT('Ctrl Pts',(-10.6390493000001,11.6,1.76955010999999));
#256243=CARTESIAN_POINT('Ctrl Pts',(-10.6366992770001,15.2,1.76840382499998));
#256244=CARTESIAN_POINT('Ctrl Pts',(-10.6366992770001,11.6,1.76840382499998));
#256245=CARTESIAN_POINT('Ctrl Pts',(-10.6343536530001,15.2,1.76726215799999));
#256246=CARTESIAN_POINT('Ctrl Pts',(-10.6343536530001,11.6,1.76726215799999));
#256247=CARTESIAN_POINT('Ctrl Pts',(-10.6320124440001,15.2,1.76612510399998));
#256248=CARTESIAN_POINT('Ctrl Pts',(-10.6320124440001,11.6,1.76612510399998));
#256249=CARTESIAN_POINT('Ctrl Pts',(-10.6296756630001,15.2,1.76499265799999));
#256250=CARTESIAN_POINT('Ctrl Pts',(-10.6296756630001,11.6,1.76499265799999));
#256251=CARTESIAN_POINT('Ctrl Pts',(-10.6273433250001,15.2,1.76386481999999));
#256252=CARTESIAN_POINT('Ctrl Pts',(-10.6273433250001,11.6,1.76386481999998));
#256253=CARTESIAN_POINT('Ctrl Pts',(-10.6250154420001,15.2,1.76274158499998));
#256254=CARTESIAN_POINT('Ctrl Pts',(-10.6250154420001,11.6,1.76274158499998));
#256255=CARTESIAN_POINT('Ctrl Pts',(-10.6226920310001,15.2,1.76162295199998));
#256256=CARTESIAN_POINT('Ctrl Pts',(-10.6226920310001,11.6,1.76162295199998));
#256257=CARTESIAN_POINT('Ctrl Pts',(-10.6203731050001,15.2,1.76050891499999));
#256258=CARTESIAN_POINT('Ctrl Pts',(-10.6203731050001,11.6,1.76050891499999));
#256259=CARTESIAN_POINT('Ctrl Pts',(-10.6180586770001,15.2,1.75939947299999));
#256260=CARTESIAN_POINT('Ctrl Pts',(-10.6180586770001,11.6,1.75939947299998));
#256261=CARTESIAN_POINT('Ctrl Pts',(-10.6157487650001,15.2,1.75829462199999));
#256262=CARTESIAN_POINT('Ctrl Pts',(-10.6157487650001,11.6,1.75829462199998));
#256263=CARTESIAN_POINT('Ctrl Pts',(-10.6134433800001,15.2,1.75719435899999));
#256264=CARTESIAN_POINT('Ctrl Pts',(-10.6134433800001,11.6,1.75719435899999));
#256265=CARTESIAN_POINT('Ctrl Pts',(-10.6111425380001,15.2,1.75609868099999));
#256266=CARTESIAN_POINT('Ctrl Pts',(-10.6111425380001,11.6,1.75609868099999));
#256267=CARTESIAN_POINT('Ctrl Pts',(-10.6088462540001,15.2,1.75500758399998));
#256268=CARTESIAN_POINT('Ctrl Pts',(-10.6088462540001,11.6,1.75500758399998));
#256269=CARTESIAN_POINT('Ctrl Pts',(-10.6065545400001,15.2,1.75392106599999));
#256270=CARTESIAN_POINT('Ctrl Pts',(-10.6065545400001,11.6,1.75392106599999));
#256271=CARTESIAN_POINT('Ctrl Pts',(-10.6042674140001,15.2,1.75283912199999));
#256272=CARTESIAN_POINT('Ctrl Pts',(-10.6042674140001,11.6,1.75283912199998));
#256273=CARTESIAN_POINT('Ctrl Pts',(-10.6019848890001,15.2,1.75176175199999));
#256274=CARTESIAN_POINT('Ctrl Pts',(-10.6019848890001,11.6,1.75176175199998));
#256275=CARTESIAN_POINT('Ctrl Pts',(-10.5997069780001,15.2,1.75068894899999));
#256276=CARTESIAN_POINT('Ctrl Pts',(-10.5997069780001,11.6,1.75068894899999));
#256277=CARTESIAN_POINT('Ctrl Pts',(-10.5974336980001,15.2,1.74962071099999));
#256278=CARTESIAN_POINT('Ctrl Pts',(-10.5974336980001,11.6,1.74962071099999));
#256279=CARTESIAN_POINT('Ctrl Pts',(-10.5951650630001,15.2,1.74855703599999));
#256280=CARTESIAN_POINT('Ctrl Pts',(-10.5951650630001,11.6,1.74855703599999));
#256281=CARTESIAN_POINT('Ctrl Pts',(-10.5929010880001,15.2,1.74749791899998));
#256282=CARTESIAN_POINT('Ctrl Pts',(-10.5929010880001,11.6,1.74749791899998));
#256283=CARTESIAN_POINT('Ctrl Pts',(-10.5906417870001,15.2,1.74644335699998));
#256284=CARTESIAN_POINT('Ctrl Pts',(-10.5906417870001,11.6,1.74644335699998));
#256285=CARTESIAN_POINT('Ctrl Pts',(-10.5883871760001,15.2,1.74539334799999));
#256286=CARTESIAN_POINT('Ctrl Pts',(-10.5883871760001,11.6,1.74539334799999));
#256287=CARTESIAN_POINT('Ctrl Pts',(-10.5861372680001,15.2,1.74434788599998));
#256288=CARTESIAN_POINT('Ctrl Pts',(-10.5861372680001,11.6,1.74434788599998));
#256289=CARTESIAN_POINT('Ctrl Pts',(-10.5838920800001,15.2,1.74330696999998));
#256290=CARTESIAN_POINT('Ctrl Pts',(-10.5838920800001,11.6,1.74330696999998));
#256291=CARTESIAN_POINT('Ctrl Pts',(-10.5816516250001,15.2,1.74227059599998));
#256292=CARTESIAN_POINT('Ctrl Pts',(-10.5816516250001,11.6,1.74227059599998));
#256293=CARTESIAN_POINT('Ctrl Pts',(-10.5794159210001,15.2,1.74123875899999));
#256294=CARTESIAN_POINT('Ctrl Pts',(-10.5794159210001,11.6,1.74123875899999));
#256295=CARTESIAN_POINT('Ctrl Pts',(-10.5771849800001,15.2,1.74021145699998));
#256296=CARTESIAN_POINT('Ctrl Pts',(-10.5771849800001,11.6,1.74021145699998));
#256297=CARTESIAN_POINT('Ctrl Pts',(-10.5749588180001,15.2,1.73918868699999));
#256298=CARTESIAN_POINT('Ctrl Pts',(-10.5749588180001,11.6,1.73918868699999));
#256299=CARTESIAN_POINT('Ctrl Pts',(-10.5727374500001,15.2,1.73817044399998));
#256300=CARTESIAN_POINT('Ctrl Pts',(-10.5727374500001,11.6,1.73817044399998));
#256301=CARTESIAN_POINT('Ctrl Pts',(-10.5705208910001,15.2,1.73715672499998));
#256302=CARTESIAN_POINT('Ctrl Pts',(-10.5705208910001,11.6,1.73715672499998));
#256303=CARTESIAN_POINT('Ctrl Pts',(-10.5683091580001,15.2,1.73614752599998));
#256304=CARTESIAN_POINT('Ctrl Pts',(-10.5683091580001,11.6,1.73614752599998));
#256305=CARTESIAN_POINT('Ctrl Pts',(-10.5661022630001,15.2,1.73514284399999));
#256306=CARTESIAN_POINT('Ctrl Pts',(-10.5661022630001,11.6,1.73514284399999));
#256307=CARTESIAN_POINT('Ctrl Pts',(-10.5639002250001,15.2,1.73414267699998));
#256308=CARTESIAN_POINT('Ctrl Pts',(-10.5639002250001,11.6,1.73414267699998));
#256309=CARTESIAN_POINT('Ctrl Pts',(-10.5617030560001,15.2,1.73314701799999));
#256310=CARTESIAN_POINT('Ctrl Pts',(-10.5617030560001,11.6,1.73314701799998));
#256311=CARTESIAN_POINT('Ctrl Pts',(-10.5595107720001,15.2,1.73215586599999));
#256312=CARTESIAN_POINT('Ctrl Pts',(-10.5595107720001,11.6,1.73215586599999));
#256313=CARTESIAN_POINT('Ctrl Pts',(-10.5573233910001,15.2,1.73116921599998));
#256314=CARTESIAN_POINT('Ctrl Pts',(-10.5573233910001,11.6,1.73116921599998));
#256315=CARTESIAN_POINT('Ctrl Pts',(-10.5551409250001,15.2,1.73018706499999));
#256316=CARTESIAN_POINT('Ctrl Pts',(-10.5551409250001,11.6,1.73018706499999));
#256317=CARTESIAN_POINT('Ctrl Pts',(-10.5529633920001,15.2,1.72920940799999));
#256318=CARTESIAN_POINT('Ctrl Pts',(-10.5529633920001,11.6,1.72920940799999));
#256319=CARTESIAN_POINT('Ctrl Pts',(-10.5507908060001,15.2,1.72823624299999));
#256320=CARTESIAN_POINT('Ctrl Pts',(-10.5507908060001,11.6,1.72823624299998));
#256321=CARTESIAN_POINT('Ctrl Pts',(-10.5486231830001,15.2,1.72726756599999));
#256322=CARTESIAN_POINT('Ctrl Pts',(-10.5486231830001,11.6,1.72726756599999));
#256323=CARTESIAN_POINT('Ctrl Pts',(-10.5464605390001,15.2,1.72630337199998));
#256324=CARTESIAN_POINT('Ctrl Pts',(-10.5464605390001,11.6,1.72630337199998));
#256325=CARTESIAN_POINT('Ctrl Pts',(-10.5443028890001,15.2,1.72534365799998));
#256326=CARTESIAN_POINT('Ctrl Pts',(-10.5443028890001,11.6,1.72534365799998));
#256327=CARTESIAN_POINT('Ctrl Pts',(-10.5421502500001,15.2,1.72438842099998));
#256328=CARTESIAN_POINT('Ctrl Pts',(-10.5421502500001,11.6,1.72438842099998));
#256329=CARTESIAN_POINT('Ctrl Pts',(-10.5400026350001,15.2,1.72343765499999));
#256330=CARTESIAN_POINT('Ctrl Pts',(-10.5400026350001,11.6,1.72343765499999));
#256331=CARTESIAN_POINT('Ctrl Pts',(-10.5378600620001,15.2,1.72249135799999));
#256332=CARTESIAN_POINT('Ctrl Pts',(-10.5378600620001,11.6,1.72249135799999));
#256333=CARTESIAN_POINT('Ctrl Pts',(-10.5357225470001,15.2,1.72154952499998));
#256334=CARTESIAN_POINT('Ctrl Pts',(-10.5357225470001,11.6,1.72154952499998));
#256335=CARTESIAN_POINT('Ctrl Pts',(-10.5335901050001,15.2,1.72061215299999));
#256336=CARTESIAN_POINT('Ctrl Pts',(-10.5335901050001,11.6,1.72061215299998));
#256337=CARTESIAN_POINT('Ctrl Pts',(-10.5314627510001,15.2,1.71967923799999));
#256338=CARTESIAN_POINT('Ctrl Pts',(-10.5314627510001,11.6,1.71967923799999));
#256339=CARTESIAN_POINT('Ctrl Pts',(-10.5293405040001,15.2,1.71875077499998));
#256340=CARTESIAN_POINT('Ctrl Pts',(-10.5293405040001,11.6,1.71875077499998));
#256341=CARTESIAN_POINT('Ctrl Pts',(-10.5272233760001,15.2,1.71782676099999));
#256342=CARTESIAN_POINT('Ctrl Pts',(-10.5272233760001,11.6,1.71782676099998));
#256343=CARTESIAN_POINT('Ctrl Pts',(-10.5251113870001,15.2,1.71690719299999));
#256344=CARTESIAN_POINT('Ctrl Pts',(-10.5251113870001,11.6,1.71690719299999));
#256345=CARTESIAN_POINT('Ctrl Pts',(-10.5230045500001,15.2,1.71599206399998));
#256346=CARTESIAN_POINT('Ctrl Pts',(-10.5230045500001,11.6,1.71599206399998));
#256347=CARTESIAN_POINT('Ctrl Pts',(-10.5209028820001,15.2,1.71508137299998));
#256348=CARTESIAN_POINT('Ctrl Pts',(-10.5209028820001,11.6,1.71508137299998));
#256349=CARTESIAN_POINT('Ctrl Pts',(-10.5188064000001,15.2,1.71417511399999));
#256350=CARTESIAN_POINT('Ctrl Pts',(-10.5188064000001,11.6,1.71417511399999));
#256351=CARTESIAN_POINT('Ctrl Pts',(-10.5167151200001,15.2,1.71327328299999));
#256352=CARTESIAN_POINT('Ctrl Pts',(-10.5167151200001,11.6,1.71327328299998));
#256353=CARTESIAN_POINT('Ctrl Pts',(-10.5146290570001,15.2,1.71237587699999));
#256354=CARTESIAN_POINT('Ctrl Pts',(-10.5146290570001,11.6,1.71237587699998));
#256355=CARTESIAN_POINT('Ctrl Pts',(-10.5125482280001,15.2,1.71148289099999));
#256356=CARTESIAN_POINT('Ctrl Pts',(-10.5125482280001,11.6,1.71148289099999));
#256357=CARTESIAN_POINT('Ctrl Pts',(-10.5104726510001,15.2,1.71059432099999));
#256358=CARTESIAN_POINT('Ctrl Pts',(-10.5104726510001,11.6,1.71059432099998));
#256359=CARTESIAN_POINT('Ctrl Pts',(-10.5084023400001,15.2,1.70971016399998));
#256360=CARTESIAN_POINT('Ctrl Pts',(-10.5084023400001,11.6,1.70971016399998));
#256361=CARTESIAN_POINT('Ctrl Pts',(-10.5063373130001,15.2,1.70883041399998));
#256362=CARTESIAN_POINT('Ctrl Pts',(-10.5063373130001,11.6,1.70883041399998));
#256363=CARTESIAN_POINT('Ctrl Pts',(-10.5042775850001,15.2,1.70795506799998));
#256364=CARTESIAN_POINT('Ctrl Pts',(-10.5042775850001,11.6,1.70795506799998));
#256365=CARTESIAN_POINT('Ctrl Pts',(-10.5022231740001,15.2,1.70708412099998));
#256366=CARTESIAN_POINT('Ctrl Pts',(-10.5022231740001,11.6,1.70708412099998));
#256367=CARTESIAN_POINT('Ctrl Pts',(-10.5001740970001,15.2,1.70621756899999));
#256368=CARTESIAN_POINT('Ctrl Pts',(-10.5001740970001,11.6,1.70621756899999));
#256369=CARTESIAN_POINT('Ctrl Pts',(-10.4981303680001,15.2,1.70535540799999));
#256370=CARTESIAN_POINT('Ctrl Pts',(-10.4981303680001,11.6,1.70535540799999));
#256371=CARTESIAN_POINT('Ctrl Pts',(-10.4960920060001,15.2,1.70449763199999));
#256372=CARTESIAN_POINT('Ctrl Pts',(-10.4960920060001,11.6,1.70449763199999));
#256373=CARTESIAN_POINT('Ctrl Pts',(-10.4940590280001,15.2,1.70364423899999));
#256374=CARTESIAN_POINT('Ctrl Pts',(-10.4940590280001,11.6,1.70364423899999));
#256375=CARTESIAN_POINT('Ctrl Pts',(-10.4920314490001,15.2,1.70279522299999));
#256376=CARTESIAN_POINT('Ctrl Pts',(-10.4920314490001,11.6,1.70279522299999));
#256377=CARTESIAN_POINT('Ctrl Pts',(-10.4900092880001,15.2,1.70195057999999));
#256378=CARTESIAN_POINT('Ctrl Pts',(-10.4900092880001,11.6,1.70195057999999));
#256379=CARTESIAN_POINT('Ctrl Pts',(-10.4879925600001,15.2,1.70111030699998));
#256380=CARTESIAN_POINT('Ctrl Pts',(-10.4879925600001,11.6,1.70111030699998));
#256381=CARTESIAN_POINT('Ctrl Pts',(-10.4859812820001,15.2,1.70027439699998));
#256382=CARTESIAN_POINT('Ctrl Pts',(-10.4859812820001,11.6,1.70027439699998));
#256383=CARTESIAN_POINT('Ctrl Pts',(-10.4839754720001,15.2,1.69944284799998));
#256384=CARTESIAN_POINT('Ctrl Pts',(-10.4839754720001,11.6,1.69944284799998));
#256385=CARTESIAN_POINT('Ctrl Pts',(-10.4819751470001,15.2,1.69861565499998));
#256386=CARTESIAN_POINT('Ctrl Pts',(-10.4819751470001,11.6,1.69861565499998));
#256387=CARTESIAN_POINT('Ctrl Pts',(-10.4799803230001,15.2,1.69779281099999));
#256388=CARTESIAN_POINT('Ctrl Pts',(-10.4799803230001,11.6,1.69779281099998));
#256389=CARTESIAN_POINT('Ctrl Pts',(-10.4779910190001,15.2,1.69697431399999));
#256390=CARTESIAN_POINT('Ctrl Pts',(-10.4779910190001,11.6,1.69697431399999));
#256391=CARTESIAN_POINT('Ctrl Pts',(-10.4760072500001,15.2,1.69616015899999));
#256392=CARTESIAN_POINT('Ctrl Pts',(-10.4760072500001,11.6,1.69616015899999));
#256393=CARTESIAN_POINT('Ctrl Pts',(-10.4740290340001,15.2,1.69535034099999));
#256394=CARTESIAN_POINT('Ctrl Pts',(-10.4740290340001,11.6,1.69535034099999));
#256395=CARTESIAN_POINT('Ctrl Pts',(-10.4720563900001,15.2,1.69454485499998));
#256396=CARTESIAN_POINT('Ctrl Pts',(-10.4720563900001,11.6,1.69454485499998));
#256397=CARTESIAN_POINT('Ctrl Pts',(-10.4700893330001,15.2,1.69374369699999));
#256398=CARTESIAN_POINT('Ctrl Pts',(-10.4700893330001,11.6,1.69374369699998));
#256399=CARTESIAN_POINT('Ctrl Pts',(-10.4681278810001,15.2,1.69294686299999));
#256400=CARTESIAN_POINT('Ctrl Pts',(-10.4681278810001,11.6,1.69294686299999));
#256401=CARTESIAN_POINT('Ctrl Pts',(-10.4661720530001,15.2,1.69215434599999));
#256402=CARTESIAN_POINT('Ctrl Pts',(-10.4661720530001,11.6,1.69215434599999));
#256403=CARTESIAN_POINT('Ctrl Pts',(-10.4642218640001,15.2,1.69136614299998));
#256404=CARTESIAN_POINT('Ctrl Pts',(-10.4642218640001,11.6,1.69136614299998));
#256405=CARTESIAN_POINT('Ctrl Pts',(-10.4622773340001,15.2,1.69058224899999));
#256406=CARTESIAN_POINT('Ctrl Pts',(-10.4622773340001,11.6,1.69058224899999));
#256407=CARTESIAN_POINT('Ctrl Pts',(-10.4603384780001,15.2,1.68980265999998));
#256408=CARTESIAN_POINT('Ctrl Pts',(-10.4603384780001,11.6,1.68980265999998));
#256409=CARTESIAN_POINT('Ctrl Pts',(-10.4584053160001,15.2,1.68902736899998));
#256410=CARTESIAN_POINT('Ctrl Pts',(-10.4584053160001,11.6,1.68902736899998));
#256411=CARTESIAN_POINT('Ctrl Pts',(-10.4564778650001,15.2,1.68825637299999));
#256412=CARTESIAN_POINT('Ctrl Pts',(-10.4564778650001,11.6,1.68825637299999));
#256413=CARTESIAN_POINT('Ctrl Pts',(-10.4545561420001,15.2,1.68748966599999));
#256414=CARTESIAN_POINT('Ctrl Pts',(-10.4545561420001,11.6,1.68748966599999));
#256415=CARTESIAN_POINT('Ctrl Pts',(-10.4526401670001,15.2,1.68672724499999));
#256416=CARTESIAN_POINT('Ctrl Pts',(-10.4526401670001,11.6,1.68672724499999));
#256417=CARTESIAN_POINT('Ctrl Pts',(-10.4507299550001,15.2,1.68596910299998));
#256418=CARTESIAN_POINT('Ctrl Pts',(-10.4507299550001,11.6,1.68596910299998));
#256419=CARTESIAN_POINT('Ctrl Pts',(-10.4488255250001,15.2,1.68521523599999));
#256420=CARTESIAN_POINT('Ctrl Pts',(-10.4488255250001,11.6,1.68521523599999));
#256421=CARTESIAN_POINT('Ctrl Pts',(-10.4469268960001,15.2,1.68446563799999));
#256422=CARTESIAN_POINT('Ctrl Pts',(-10.4469268960001,11.6,1.68446563799999));
#256423=CARTESIAN_POINT('Ctrl Pts',(-10.4450340850001,15.2,1.68372030599999));
#256424=CARTESIAN_POINT('Ctrl Pts',(-10.4450340850001,11.6,1.68372030599999));
#256425=CARTESIAN_POINT('Ctrl Pts',(-10.4431471100001,15.2,1.68297923299999));
#256426=CARTESIAN_POINT('Ctrl Pts',(-10.4431471100001,11.6,1.68297923299999));
#256427=CARTESIAN_POINT('Ctrl Pts',(-10.4412659910001,15.2,1.68224241499999));
#256428=CARTESIAN_POINT('Ctrl Pts',(-10.4412659910001,11.6,1.68224241499999));
#256429=CARTESIAN_POINT('Ctrl Pts',(-10.4393907430001,15.2,1.68150984699999));
#256430=CARTESIAN_POINT('Ctrl Pts',(-10.4393907430001,11.6,1.68150984699999));
#256431=CARTESIAN_POINT('Ctrl Pts',(-10.4375213870001,15.2,1.68078152299998));
#256432=CARTESIAN_POINT('Ctrl Pts',(-10.4375213870001,11.6,1.68078152299998));
#256433=CARTESIAN_POINT('Ctrl Pts',(-10.4356579400001,15.2,1.68005743899998));
#256434=CARTESIAN_POINT('Ctrl Pts',(-10.4356579400001,11.6,1.68005743899998));
#256435=CARTESIAN_POINT('Ctrl Pts',(-10.4338004210001,15.2,1.67933758899999));
#256436=CARTESIAN_POINT('Ctrl Pts',(-10.4338004210001,11.6,1.67933758899998));
#256437=CARTESIAN_POINT('Ctrl Pts',(-10.4319488490001,15.2,1.67862196699998));
#256438=CARTESIAN_POINT('Ctrl Pts',(-10.4319488490001,11.6,1.67862196699998));
#256439=CARTESIAN_POINT('Ctrl Pts',(-10.4301032410001,15.2,1.67791056899999));
#256440=CARTESIAN_POINT('Ctrl Pts',(-10.4301032410001,11.6,1.67791056899999));
#256441=CARTESIAN_POINT('Ctrl Pts',(-10.4282636170001,15.2,1.67720339099999));
#256442=CARTESIAN_POINT('Ctrl Pts',(-10.4282636170001,11.6,1.67720339099999));
#256443=CARTESIAN_POINT('Ctrl Pts',(-10.4264299930001,15.2,1.67650042499998));
#256444=CARTESIAN_POINT('Ctrl Pts',(-10.4264299930001,11.6,1.67650042499998));
#256445=CARTESIAN_POINT('Ctrl Pts',(-10.4246023920001,15.2,1.67580166599999));
#256446=CARTESIAN_POINT('Ctrl Pts',(-10.4246023920001,11.6,1.67580166599999));
#256447=CARTESIAN_POINT('Ctrl Pts',(-10.4227808290001,15.2,1.67510710999998));
#256448=CARTESIAN_POINT('Ctrl Pts',(-10.4227808290001,11.6,1.67510710999998));
#256449=CARTESIAN_POINT('Ctrl Pts',(-10.4209653250001,15.2,1.67441675099999));
#256450=CARTESIAN_POINT('Ctrl Pts',(-10.4209653250001,11.6,1.67441675099999));
#256451=CARTESIAN_POINT('Ctrl Pts',(-10.4191558970001,15.2,1.67373058499999));
#256452=CARTESIAN_POINT('Ctrl Pts',(-10.4191558970001,11.6,1.67373058499999));
#256453=CARTESIAN_POINT('Ctrl Pts',(-10.4173525660001,15.2,1.67304860399998));
#256454=CARTESIAN_POINT('Ctrl Pts',(-10.4173525660001,11.6,1.67304860399998));
#256455=CARTESIAN_POINT('Ctrl Pts',(-10.4155553510001,15.2,1.67237080499998));
#256456=CARTESIAN_POINT('Ctrl Pts',(-10.4155553510001,11.6,1.67237080499998));
#256457=CARTESIAN_POINT('Ctrl Pts',(-10.4137642690001,15.2,1.67169717899998));
#256458=CARTESIAN_POINT('Ctrl Pts',(-10.4137642690001,11.6,1.67169717899998));
#256459=CARTESIAN_POINT('Ctrl Pts',(-10.4119793400001,15.2,1.67102772499998));
#256460=CARTESIAN_POINT('Ctrl Pts',(-10.4119793400001,11.6,1.67102772499998));
#256461=CARTESIAN_POINT('Ctrl Pts',(-10.4102005840001,15.2,1.67036243499998));
#256462=CARTESIAN_POINT('Ctrl Pts',(-10.4102005840001,11.6,1.67036243499998));
#256463=CARTESIAN_POINT('Ctrl Pts',(-10.4084280180001,15.2,1.66970130199998));
#256464=CARTESIAN_POINT('Ctrl Pts',(-10.4084280180001,11.6,1.66970130199998));
#256465=CARTESIAN_POINT('Ctrl Pts',(-10.4066616650001,15.2,1.66904432199999));
#256466=CARTESIAN_POINT('Ctrl Pts',(-10.4066616650001,11.6,1.66904432199999));
#256467=CARTESIAN_POINT('Ctrl Pts',(-10.4049015420001,15.2,1.66839148999999));
#256468=CARTESIAN_POINT('Ctrl Pts',(-10.4049015420001,11.6,1.66839148999998));
#256469=CARTESIAN_POINT('Ctrl Pts',(-10.4031476680001,15.2,1.66774279999998));
#256470=CARTESIAN_POINT('Ctrl Pts',(-10.4031476680001,11.6,1.66774279999998));
#256471=CARTESIAN_POINT('Ctrl Pts',(-10.4014000640001,15.2,1.66709824499998));
#256472=CARTESIAN_POINT('Ctrl Pts',(-10.4014000640001,11.6,1.66709824499998));
#256473=CARTESIAN_POINT('Ctrl Pts',(-10.3996587490001,15.2,1.66645781999998));
#256474=CARTESIAN_POINT('Ctrl Pts',(-10.3996587490001,11.6,1.66645781999998));
#256475=CARTESIAN_POINT('Ctrl Pts',(-10.3979237410001,15.2,1.66582151999998));
#256476=CARTESIAN_POINT('Ctrl Pts',(-10.3979237410001,11.6,1.66582151999998));
#256477=CARTESIAN_POINT('Ctrl Pts',(-10.3961950630001,15.2,1.66518933799999));
#256478=CARTESIAN_POINT('Ctrl Pts',(-10.3961950630001,11.6,1.66518933799999));
#256479=CARTESIAN_POINT('Ctrl Pts',(-10.3944727320001,15.2,1.66456126899998));
#256480=CARTESIAN_POINT('Ctrl Pts',(-10.3944727320001,11.6,1.66456126899998));
#256481=CARTESIAN_POINT('Ctrl Pts',(-10.3927567690001,15.2,1.66393730599999));
#256482=CARTESIAN_POINT('Ctrl Pts',(-10.3927567690001,11.6,1.66393730599998));
#256483=CARTESIAN_POINT('Ctrl Pts',(-10.3910471940001,15.2,1.66331744399999));
#256484=CARTESIAN_POINT('Ctrl Pts',(-10.3910471940001,11.6,1.66331744399998));
#256485=CARTESIAN_POINT('Ctrl Pts',(-10.3893440270001,15.2,1.66270167599999));
#256486=CARTESIAN_POINT('Ctrl Pts',(-10.3893440270001,11.6,1.66270167599999));
#256487=CARTESIAN_POINT('Ctrl Pts',(-10.3876472860001,15.2,1.66208999799998));
#256488=CARTESIAN_POINT('Ctrl Pts',(-10.3876472860001,11.6,1.66208999799998));
#256489=CARTESIAN_POINT('Ctrl Pts',(-10.3859569940001,15.2,1.66148240199998));
#256490=CARTESIAN_POINT('Ctrl Pts',(-10.3859569940001,11.6,1.66148240199998));
#256491=CARTESIAN_POINT('Ctrl Pts',(-10.3842731710001,15.2,1.66087888299999));
#256492=CARTESIAN_POINT('Ctrl Pts',(-10.3842731710001,11.6,1.66087888299998));
#256493=CARTESIAN_POINT('Ctrl Pts',(-10.3825958360001,15.2,1.66027943499999));
#256494=CARTESIAN_POINT('Ctrl Pts',(-10.3825958360001,11.6,1.66027943499999));
#256495=CARTESIAN_POINT('Ctrl Pts',(-10.3809250080001,15.2,1.65968405099999));
#256496=CARTESIAN_POINT('Ctrl Pts',(-10.3809250080001,11.6,1.65968405099999));
#256497=CARTESIAN_POINT('Ctrl Pts',(-10.3792607110001,15.2,1.65909272599999));
#256498=CARTESIAN_POINT('Ctrl Pts',(-10.3792607110001,11.6,1.65909272599999));
#256499=CARTESIAN_POINT('Ctrl Pts',(-10.3776029620001,15.2,1.65850545199998));
#256500=CARTESIAN_POINT('Ctrl Pts',(-10.3776029620001,11.6,1.65850545199998));
#256501=CARTESIAN_POINT('Ctrl Pts',(-10.3759517830001,15.2,1.65792222499999));
#256502=CARTESIAN_POINT('Ctrl Pts',(-10.3759517830001,11.6,1.65792222499999));
#256503=CARTESIAN_POINT('Ctrl Pts',(-10.3743071950001,15.2,1.65734303799999));
#256504=CARTESIAN_POINT('Ctrl Pts',(-10.3743071950001,11.6,1.65734303799998));
#256505=CARTESIAN_POINT('Ctrl Pts',(-10.3726692190001,15.2,1.65676788299999));
#256506=CARTESIAN_POINT('Ctrl Pts',(-10.3726692190001,11.6,1.65676788299999));
#256507=CARTESIAN_POINT('Ctrl Pts',(-10.3710378740001,15.2,1.65619675499999));
#256508=CARTESIAN_POINT('Ctrl Pts',(-10.3710378740001,11.6,1.65619675499999));
#256509=CARTESIAN_POINT('Ctrl Pts',(-10.3694131820001,15.2,1.65562964899999));
#256510=CARTESIAN_POINT('Ctrl Pts',(-10.3694131820001,11.6,1.65562964899999));
#256511=CARTESIAN_POINT('Ctrl Pts',(-10.3677951640001,15.2,1.65506655599998));
#256512=CARTESIAN_POINT('Ctrl Pts',(-10.3677951640001,11.6,1.65506655599998));
#256513=CARTESIAN_POINT('Ctrl Pts',(-10.3661838400001,15.2,1.65450747099999));
#256514=CARTESIAN_POINT('Ctrl Pts',(-10.3661838400001,11.6,1.65450747099999));
#256515=CARTESIAN_POINT('Ctrl Pts',(-10.3645792330001,15.2,1.65395238799999));
#256516=CARTESIAN_POINT('Ctrl Pts',(-10.3645792330001,11.6,1.65395238799999));
#256517=CARTESIAN_POINT('Ctrl Pts',(-10.3629813620001,15.2,1.65340129999999));
#256518=CARTESIAN_POINT('Ctrl Pts',(-10.3629813620001,11.6,1.65340129999999));
#256519=CARTESIAN_POINT('Ctrl Pts',(-10.3613902500001,15.2,1.65285419899998));
#256520=CARTESIAN_POINT('Ctrl Pts',(-10.3613902500001,11.6,1.65285419899998));
#256521=CARTESIAN_POINT('Ctrl Pts',(-10.3598059160001,15.2,1.65231107999999));
#256522=CARTESIAN_POINT('Ctrl Pts',(-10.3598059160001,11.6,1.65231107999999));
#256523=CARTESIAN_POINT('Ctrl Pts',(-10.3582283850001,15.2,1.65177193599999));
#256524=CARTESIAN_POINT('Ctrl Pts',(-10.3582283850001,11.6,1.65177193599999));
#256525=CARTESIAN_POINT('Ctrl Pts',(-10.3566576740001,15.2,1.65123676099999));
#256526=CARTESIAN_POINT('Ctrl Pts',(-10.3566576740001,11.6,1.65123676099999));
#256527=CARTESIAN_POINT('Ctrl Pts',(-10.3550938080001,15.2,1.65070554699998));
#256528=CARTESIAN_POINT('Ctrl Pts',(-10.3550938080001,11.6,1.65070554699998));
#256529=CARTESIAN_POINT('Ctrl Pts',(-10.3535368060001,15.2,1.65017828799999));
#256530=CARTESIAN_POINT('Ctrl Pts',(-10.3535368060001,11.6,1.65017828799999));
#256531=CARTESIAN_POINT('Ctrl Pts',(-10.3519866920001,15.2,1.64965497699999));
#256532=CARTESIAN_POINT('Ctrl Pts',(-10.3519866920001,11.6,1.64965497699999));
#256533=CARTESIAN_POINT('Ctrl Pts',(-10.3504434860001,15.2,1.64913560699999));
#256534=CARTESIAN_POINT('Ctrl Pts',(-10.3504434860001,11.6,1.64913560699999));
#256535=CARTESIAN_POINT('Ctrl Pts',(-10.3489072110001,15.2,1.64862017299999));
#256536=CARTESIAN_POINT('Ctrl Pts',(-10.3489072110001,11.6,1.64862017299999));
#256537=CARTESIAN_POINT('Ctrl Pts',(-10.3473778890001,15.2,1.64810866399999));
#256538=CARTESIAN_POINT('Ctrl Pts',(-10.3473778890001,11.6,1.64810866399998));
#256539=CARTESIAN_POINT('Ctrl Pts',(-10.3458555400001,15.2,1.64760107799999));
#256540=CARTESIAN_POINT('Ctrl Pts',(-10.3458555400001,11.6,1.64760107799998));
#256541=CARTESIAN_POINT('Ctrl Pts',(-10.3443401890001,15.2,1.64709740399998));
#256542=CARTESIAN_POINT('Ctrl Pts',(-10.3443401890001,11.6,1.64709740399998));
#256543=CARTESIAN_POINT('Ctrl Pts',(-10.3428318550001,15.2,1.64659763699999));
#256544=CARTESIAN_POINT('Ctrl Pts',(-10.3428318550001,11.6,1.64659763699999));
#256545=CARTESIAN_POINT('Ctrl Pts',(-10.3413305630001,15.2,1.64610176999998));
#256546=CARTESIAN_POINT('Ctrl Pts',(-10.3413305630001,11.6,1.64610176999998));
#256547=CARTESIAN_POINT('Ctrl Pts',(-10.3398363340001,15.2,1.64560979499999));
#256548=CARTESIAN_POINT('Ctrl Pts',(-10.3398363340001,11.6,1.64560979499999));
#256549=CARTESIAN_POINT('Ctrl Pts',(-10.3383491910001,15.2,1.64512170499998));
#256550=CARTESIAN_POINT('Ctrl Pts',(-10.3383491910001,11.6,1.64512170499998));
#256551=CARTESIAN_POINT('Ctrl Pts',(-10.3368691540001,15.2,1.64463749399999));
#256552=CARTESIAN_POINT('Ctrl Pts',(-10.3368691540001,11.6,1.64463749399998));
#256553=CARTESIAN_POINT('Ctrl Pts',(-10.3353962500001,15.2,1.64415715299999));
#256554=CARTESIAN_POINT('Ctrl Pts',(-10.3353962500001,11.6,1.64415715299999));
#256555=CARTESIAN_POINT('Ctrl Pts',(-10.3339304990001,15.2,1.64368067599999));
#256556=CARTESIAN_POINT('Ctrl Pts',(-10.3339304990001,11.6,1.64368067599999));
#256557=CARTESIAN_POINT('Ctrl Pts',(-10.3324719230001,15.2,1.64320805599999));
#256558=CARTESIAN_POINT('Ctrl Pts',(-10.3324719230001,11.6,1.64320805599999));
#256559=CARTESIAN_POINT('Ctrl Pts',(-10.3310205470001,15.2,1.64273928299998));
#256560=CARTESIAN_POINT('Ctrl Pts',(-10.3310205470001,11.6,1.64273928299998));
#256561=CARTESIAN_POINT('Ctrl Pts',(-10.3295763920001,15.2,1.64227435299999));
#256562=CARTESIAN_POINT('Ctrl Pts',(-10.3295763920001,11.6,1.64227435299999));
#256563=CARTESIAN_POINT('Ctrl Pts',(-10.3281394820001,15.2,1.64181325699999));
#256564=CARTESIAN_POINT('Ctrl Pts',(-10.3281394820001,11.6,1.64181325699999));
#256565=CARTESIAN_POINT('Ctrl Pts',(-10.3267098410001,15.2,1.64135598899998));
#256566=CARTESIAN_POINT('Ctrl Pts',(-10.3267098410001,11.6,1.64135598899998));
#256567=CARTESIAN_POINT('Ctrl Pts',(-10.3252874890001,15.2,1.64090253799999));
#256568=CARTESIAN_POINT('Ctrl Pts',(-10.3252874890001,11.6,1.64090253799999));
#256569=CARTESIAN_POINT('Ctrl Pts',(-10.3238724540001,15.2,1.64045289999999));
#256570=CARTESIAN_POINT('Ctrl Pts',(-10.3238724540001,11.6,1.64045289999999));
#256571=CARTESIAN_POINT('Ctrl Pts',(-10.3224647550001,15.2,1.64000706499999));
#256572=CARTESIAN_POINT('Ctrl Pts',(-10.3224647550001,11.6,1.64000706499999));
#256573=CARTESIAN_POINT('Ctrl Pts',(-10.3210644180001,15.2,1.63956502799998));
#256574=CARTESIAN_POINT('Ctrl Pts',(-10.3210644180001,11.6,1.63956502799998));
#256575=CARTESIAN_POINT('Ctrl Pts',(-10.3196714660001,15.2,1.63912677799999));
#256576=CARTESIAN_POINT('Ctrl Pts',(-10.3196714660001,11.6,1.63912677799999));
#256577=CARTESIAN_POINT('Ctrl Pts',(-10.3182859220001,15.2,1.63869230999998));
#256578=CARTESIAN_POINT('Ctrl Pts',(-10.3182859220001,11.6,1.63869230999998));
#256579=CARTESIAN_POINT('Ctrl Pts',(-10.3169078100001,15.2,1.63826161499999));
#256580=CARTESIAN_POINT('Ctrl Pts',(-10.3169078100001,11.6,1.63826161499998));
#256581=CARTESIAN_POINT('Ctrl Pts',(-10.3155371550001,15.2,1.63783468499998));
#256582=CARTESIAN_POINT('Ctrl Pts',(-10.3155371550001,11.6,1.63783468499998));
#256583=CARTESIAN_POINT('Ctrl Pts',(-10.3141739780001,15.2,1.63741151199998));
#256584=CARTESIAN_POINT('Ctrl Pts',(-10.3141739780001,11.6,1.63741151199998));
#256585=CARTESIAN_POINT('Ctrl Pts',(-10.3128183080001,15.2,1.63699208999999));
#256586=CARTESIAN_POINT('Ctrl Pts',(-10.3128183080001,11.6,1.63699208999999));
#256587=CARTESIAN_POINT('Ctrl Pts',(-10.3114701640001,15.2,1.63657640799999));
#256588=CARTESIAN_POINT('Ctrl Pts',(-10.3114701640001,11.6,1.63657640799999));
#256589=CARTESIAN_POINT('Ctrl Pts',(-10.3101295730001,15.2,1.63616446099998));
#256590=CARTESIAN_POINT('Ctrl Pts',(-10.3101295730001,11.6,1.63616446099998));
#256591=CARTESIAN_POINT('Ctrl Pts',(-10.3087965590001,15.2,1.63575623899999));
#256592=CARTESIAN_POINT('Ctrl Pts',(-10.3087965590001,11.6,1.63575623899999));
#256593=CARTESIAN_POINT('Ctrl Pts',(-10.3074711460001,15.2,1.63535173399998));
#256594=CARTESIAN_POINT('Ctrl Pts',(-10.3074711460001,11.6,1.63535173399998));
#256595=CARTESIAN_POINT('Ctrl Pts',(-10.3061533570001,15.2,1.63495093799999));
#256596=CARTESIAN_POINT('Ctrl Pts',(-10.3061533570001,11.6,1.63495093799999));
#256597=CARTESIAN_POINT('Ctrl Pts',(-10.3048432200001,15.2,1.63455384399999));
#256598=CARTESIAN_POINT('Ctrl Pts',(-10.3048432200001,11.6,1.63455384399999));
#256599=CARTESIAN_POINT('Ctrl Pts',(-10.3035407580001,15.2,1.63416044299999));
#256600=CARTESIAN_POINT('Ctrl Pts',(-10.3035407580001,11.6,1.63416044299999));
#256601=CARTESIAN_POINT('Ctrl Pts',(-10.3022459950001,15.2,1.63377072599999));
#256602=CARTESIAN_POINT('Ctrl Pts',(-10.3022459950001,11.6,1.63377072599999));
#256603=CARTESIAN_POINT('Ctrl Pts',(-10.3009589570001,15.2,1.63338468499999));
#256604=CARTESIAN_POINT('Ctrl Pts',(-10.3009589570001,11.6,1.63338468499999));
#256605=CARTESIAN_POINT('Ctrl Pts',(-10.2996796700001,15.2,1.63300231199999));
#256606=CARTESIAN_POINT('Ctrl Pts',(-10.2996796700001,11.6,1.63300231199999));
#256607=CARTESIAN_POINT('Ctrl Pts',(-10.2984081560001,15.2,1.63262359999999));
#256608=CARTESIAN_POINT('Ctrl Pts',(-10.2984081560001,11.6,1.63262359999999));
#256609=CARTESIAN_POINT('Ctrl Pts',(-10.2971444420001,15.2,1.63224853699999));
#256610=CARTESIAN_POINT('Ctrl Pts',(-10.2971444420001,11.6,1.63224853699999));
#256611=CARTESIAN_POINT('Ctrl Pts',(-10.2958885550001,15.2,1.63187711599999));
#256612=CARTESIAN_POINT('Ctrl Pts',(-10.2958885550001,11.6,1.63187711599999));
#256613=CARTESIAN_POINT('Ctrl Pts',(-10.2946405180001,15.2,1.63150932999998));
#256614=CARTESIAN_POINT('Ctrl Pts',(-10.2946405180001,11.6,1.63150932999998));
#256615=CARTESIAN_POINT('Ctrl Pts',(-10.2934003580001,15.2,1.63114516899999));
#256616=CARTESIAN_POINT('Ctrl Pts',(-10.2934003580001,11.6,1.63114516899999));
#256617=CARTESIAN_POINT('Ctrl Pts',(-10.2921680990001,15.2,1.63078462399998));
#256618=CARTESIAN_POINT('Ctrl Pts',(-10.2921680990001,11.6,1.63078462399998));
#256619=CARTESIAN_POINT('Ctrl Pts',(-10.2909437690001,15.2,1.63042768599999));
#256620=CARTESIAN_POINT('Ctrl Pts',(-10.2909437690001,11.6,1.63042768599999));
#256621=CARTESIAN_POINT('Ctrl Pts',(-10.2897273920001,15.2,1.63007434899999));
#256622=CARTESIAN_POINT('Ctrl Pts',(-10.2897273920001,11.6,1.63007434899999));
#256623=CARTESIAN_POINT('Ctrl Pts',(-10.2885189960001,15.2,1.62972459999999));
#256624=CARTESIAN_POINT('Ctrl Pts',(-10.2885189960001,11.6,1.62972459999999));
#256625=CARTESIAN_POINT('Ctrl Pts',(-10.2873186040001,15.2,1.62937843299999));
#256626=CARTESIAN_POINT('Ctrl Pts',(-10.2873186040001,11.6,1.62937843299999));
#256627=CARTESIAN_POINT('Ctrl Pts',(-10.2861262460001,15.2,1.62903583899999));
#256628=CARTESIAN_POINT('Ctrl Pts',(-10.2861262460001,11.6,1.62903583899999));
#256629=CARTESIAN_POINT('Ctrl Pts',(-10.2849419460001,15.2,1.62869680699998));
#256630=CARTESIAN_POINT('Ctrl Pts',(-10.2849419460001,11.6,1.62869680699998));
#256631=CARTESIAN_POINT('Ctrl Pts',(-10.2837657300001,15.2,1.62836132999999));
#256632=CARTESIAN_POINT('Ctrl Pts',(-10.2837657300001,11.6,1.62836132999999));
#256633=CARTESIAN_POINT('Ctrl Pts',(-10.2825976260001,15.2,1.62802939699999));
#256634=CARTESIAN_POINT('Ctrl Pts',(-10.2825976260001,11.6,1.62802939699999));
#256635=CARTESIAN_POINT('Ctrl Pts',(-10.2814376600001,15.2,1.62770100099999));
#256636=CARTESIAN_POINT('Ctrl Pts',(-10.2814376600001,11.6,1.62770100099999));
#256637=CARTESIAN_POINT('Ctrl Pts',(-10.2802858580001,15.2,1.62737613099999));
#256638=CARTESIAN_POINT('Ctrl Pts',(-10.2802858580001,11.6,1.62737613099999));
#256639=CARTESIAN_POINT('Ctrl Pts',(-10.2791422490001,15.2,1.62705477899999));
#256640=CARTESIAN_POINT('Ctrl Pts',(-10.2791422490001,11.6,1.62705477899999));
#256641=CARTESIAN_POINT('Ctrl Pts',(-10.2780068590001,15.2,1.62673693499999));
#256642=CARTESIAN_POINT('Ctrl Pts',(-10.2780068590001,11.6,1.62673693499999));
#256643=CARTESIAN_POINT('Ctrl Pts',(-10.2768797140001,15.2,1.62642258899998));
#256644=CARTESIAN_POINT('Ctrl Pts',(-10.2768797140001,11.6,1.62642258899998));
#256645=CARTESIAN_POINT('Ctrl Pts',(-10.2757608430001,15.2,1.62611173199998));
#256646=CARTESIAN_POINT('Ctrl Pts',(-10.2757608430001,11.6,1.62611173199998));
#256647=CARTESIAN_POINT('Ctrl Pts',(-10.2746502720001,15.2,1.62580435599998));
#256648=CARTESIAN_POINT('Ctrl Pts',(-10.2746502720001,11.6,1.62580435599998));
#256649=CARTESIAN_POINT('Ctrl Pts',(-10.2735480290001,15.2,1.62550044899998));
#256650=CARTESIAN_POINT('Ctrl Pts',(-10.2735480290001,11.6,1.62550044899998));
#256651=CARTESIAN_POINT('Ctrl Pts',(-10.2724541430001,15.2,1.62520000299998));
#256652=CARTESIAN_POINT('Ctrl Pts',(-10.2724541430001,11.6,1.62520000299998));
#256653=CARTESIAN_POINT('Ctrl Pts',(-10.2713686400001,15.2,1.62490300799998));
#256654=CARTESIAN_POINT('Ctrl Pts',(-10.2713686400001,11.6,1.62490300799998));
#256655=CARTESIAN_POINT('Ctrl Pts',(-10.2702915480001,15.2,1.62460945399999));
#256656=CARTESIAN_POINT('Ctrl Pts',(-10.2702915480001,11.6,1.62460945399999));
#256657=CARTESIAN_POINT('Ctrl Pts',(-10.2692228960001,15.2,1.62431933099999));
#256658=CARTESIAN_POINT('Ctrl Pts',(-10.2692228960001,11.6,1.62431933099999));
#256659=CARTESIAN_POINT('Ctrl Pts',(-10.2681627110001,15.2,1.62403262999999));
#256660=CARTESIAN_POINT('Ctrl Pts',(-10.2681627110001,11.6,1.62403262999998));
#256661=CARTESIAN_POINT('Ctrl Pts',(-10.2671110220001,15.2,1.62374933999998));
#256662=CARTESIAN_POINT('Ctrl Pts',(-10.2671110220001,11.6,1.62374933999998));
#256663=CARTESIAN_POINT('Ctrl Pts',(-10.2660678570001,15.2,1.62346945199999));
#256664=CARTESIAN_POINT('Ctrl Pts',(-10.2660678570001,11.6,1.62346945199999));
#256665=CARTESIAN_POINT('Ctrl Pts',(-10.2650332450001,15.2,1.62319295599998));
#256666=CARTESIAN_POINT('Ctrl Pts',(-10.2650332450001,11.6,1.62319295599998));
#256667=CARTESIAN_POINT('Ctrl Pts',(-10.2640072150001,15.2,1.62291984099999));
#256668=CARTESIAN_POINT('Ctrl Pts',(-10.2640072150001,11.6,1.62291984099999));
#256669=CARTESIAN_POINT('Ctrl Pts',(-10.2629897940001,15.2,1.62265009799999));
#256670=CARTESIAN_POINT('Ctrl Pts',(-10.2629897940001,11.6,1.62265009799999));
#256671=CARTESIAN_POINT('Ctrl Pts',(-10.2619810130001,15.2,1.62238371499999));
#256672=CARTESIAN_POINT('Ctrl Pts',(-10.2619810130001,11.6,1.62238371499999));
#256673=CARTESIAN_POINT('Ctrl Pts',(-10.2609809010001,15.2,1.62212068299999));
#256674=CARTESIAN_POINT('Ctrl Pts',(-10.2609809010001,11.6,1.62212068299999));
#256675=CARTESIAN_POINT('Ctrl Pts',(-10.2599894860001,15.2,1.62186099199999));
#256676=CARTESIAN_POINT('Ctrl Pts',(-10.2599894860001,11.6,1.62186099199999));
#256677=CARTESIAN_POINT('Ctrl Pts',(-10.2590067970001,15.2,1.62160463199998));
#256678=CARTESIAN_POINT('Ctrl Pts',(-10.2590067970001,11.6,1.62160463199998));
#256679=CARTESIAN_POINT('Ctrl Pts',(-10.2580328640001,15.2,1.62135158999998));
#256680=CARTESIAN_POINT('Ctrl Pts',(-10.2580328640001,11.6,1.62135158999998));
#256681=CARTESIAN_POINT('Ctrl Pts',(-10.2570677170001,15.2,1.62110185799999));
#256682=CARTESIAN_POINT('Ctrl Pts',(-10.2570677170001,11.6,1.62110185799999));
#256683=CARTESIAN_POINT('Ctrl Pts',(-10.2561113860001,15.2,1.62085542499999));
#256684=CARTESIAN_POINT('Ctrl Pts',(-10.2561113860001,11.6,1.62085542499998));
#256685=CARTESIAN_POINT('Ctrl Pts',(-10.2551639010001,15.2,1.62061227799999));
#256686=CARTESIAN_POINT('Ctrl Pts',(-10.2551639010001,11.6,1.62061227799999));
#256687=CARTESIAN_POINT('Ctrl Pts',(-10.2542252910001,15.2,1.62037240999998));
#256688=CARTESIAN_POINT('Ctrl Pts',(-10.2542252910001,11.6,1.62037240999998));
#256689=CARTESIAN_POINT('Ctrl Pts',(-10.2532955860001,15.2,1.62013580699998));
#256690=CARTESIAN_POINT('Ctrl Pts',(-10.2532955860001,11.6,1.62013580699998));
#256691=CARTESIAN_POINT('Ctrl Pts',(-10.2523748180001,15.2,1.61990246099998));
#256692=CARTESIAN_POINT('Ctrl Pts',(-10.2523748180001,11.6,1.61990246099998));
#256693=CARTESIAN_POINT('Ctrl Pts',(-10.2514630160001,15.2,1.61967235699999));
#256694=CARTESIAN_POINT('Ctrl Pts',(-10.2514630160001,11.6,1.61967235699999));
#256695=CARTESIAN_POINT('Ctrl Pts',(-10.2505602120001,15.2,1.61944548899998));
#256696=CARTESIAN_POINT('Ctrl Pts',(-10.2505602120001,11.6,1.61944548899998));
#256697=CARTESIAN_POINT('Ctrl Pts',(-10.2496715820001,15.2,1.61922312999998));
#256698=CARTESIAN_POINT('Ctrl Pts',(-10.2496715820001,11.6,1.61922312999998));
#256699=CARTESIAN_POINT('Ctrl Pts',(-10.2489688520001,15.2,1.61904803399999));
#256700=CARTESIAN_POINT('Ctrl Pts',(-10.2489688520001,11.6,1.61904803399999));
#256701=CARTESIAN_POINT('Ctrl Pts',(-10.2484470900001,15.2,1.61891843999999));
#256702=CARTESIAN_POINT('Ctrl Pts',(-10.2484470900001,11.6,1.61891843999999));
#256703=CARTESIAN_POINT('Ctrl Pts',(-10.2481027040001,15.2,1.61883308499998));
#256704=CARTESIAN_POINT('Ctrl Pts',(-10.2481027040001,11.6,1.61883308499998));
#256705=CARTESIAN_POINT('Ctrl Pts',(-10.2479334570001,15.2,1.61879117999999));
#256706=CARTESIAN_POINT('Ctrl Pts',(-10.2479334570001,11.6,1.61879117999999));
#256707=CARTESIAN_POINT('',(-10.2479334563364,12.2,1.61879117933379));
#256708=CARTESIAN_POINT('',(-10.2479334563364,15.2,1.61879117933379));
#256709=CARTESIAN_POINT('',(-10.2479334560001,12.2,1.61879117899999));
#256710=CARTESIAN_POINT('Ctrl Pts',(-11.2922242990001,12.2,2.17615954699998));
#256711=CARTESIAN_POINT('Ctrl Pts',(-11.288148224556,12.2,2.17309893949932));
#256712=CARTESIAN_POINT('Ctrl Pts',(-11.2840769420896,12.2,2.17005151815676));
#256713=CARTESIAN_POINT('Ctrl Pts',(-11.2800104648685,12.2,2.16701730343719));
#256714=CARTESIAN_POINT('Ctrl Pts',(-11.2769606072297,12.2,2.16474164260421));
#256715=CARTESIAN_POINT('Ctrl Pts',(-11.2739134517022,12.2,2.16247340717588));
#256716=CARTESIAN_POINT('Ctrl Pts',(-11.2708690254527,12.2,2.16021259706259));
#256717=CARTESIAN_POINT('Ctrl Pts',(-11.2678245992032,12.2,2.1579517869493));
#256718=CARTESIAN_POINT('Ctrl Pts',(-11.2647829043248,12.2,2.15569840142299));
#256719=CARTESIAN_POINT('Ctrl Pts',(-11.2617439868938,12.2,2.15345243900525));
#256720=CARTESIAN_POINT('Ctrl Pts',(-11.2587050694628,12.2,2.15120647658751));
#256721=CARTESIAN_POINT('Ctrl Pts',(-11.2556689314065,12.2,2.14896793818554));
#256722=CARTESIAN_POINT('Ctrl Pts',(-11.2526356197667,12.2,2.14673682076659));
#256723=CARTESIAN_POINT('Ctrl Pts',(-11.2496023081269,12.2,2.14450570334765));
#256724=CARTESIAN_POINT('Ctrl Pts',(-11.246571822237,12.2,2.14228200686175));
#256725=CARTESIAN_POINT('Ctrl Pts',(-11.2435441985551,12.2,2.14006573144163));
#256726=CARTESIAN_POINT('Ctrl Pts',(-11.2405165748732,12.2,2.1378494560215));
#256727=CARTESIAN_POINT('Ctrl Pts',(-11.2374918133929,12.2,2.13564060199011));
#256728=CARTESIAN_POINT('Ctrl Pts',(-11.2344699531014,12.2,2.1334391659176));
#256729=CARTESIAN_POINT('Ctrl Pts',(-11.2314480928099,12.2,2.13123772984508));
#256730=CARTESIAN_POINT('Ctrl Pts',(-11.2284291334317,12.2,2.12904371214819));
#256731=CARTESIAN_POINT('Ctrl Pts',(-11.2254131178325,12.2,2.12685711172662));
#256732=CARTESIAN_POINT('Ctrl Pts',(-11.2223971016855,12.2,2.12467051090782));
#256733=CARTESIAN_POINT('Ctrl Pts',(-11.2193840292809,12.2,2.12249132810778));
#256734=CARTESIAN_POINT('Ctrl Pts',(-11.2163739430938,12.2,2.12031956029316));
#256735=CARTESIAN_POINT('Ctrl Pts',(-11.2133638574536,12.2,2.11814779287309));
#256736=CARTESIAN_POINT('Ctrl Pts',(-11.2103567585799,12.2,2.1159834411526));
#256737=CARTESIAN_POINT('Ctrl Pts',(-11.2073526859393,12.2,2.11382650227328));
#256738=CARTESIAN_POINT('Ctrl Pts',(-11.2033472559338,12.2,2.11095058389815));
#256739=CARTESIAN_POINT('Ctrl Pts',(-11.1993472054199,12.2,2.10808784600184));
#256740=CARTESIAN_POINT('Ctrl Pts',(-11.1953526345464,12.2,2.10523828264682));
#256741=CARTESIAN_POINT('Ctrl Pts',(-11.1923567062552,12.2,2.1031011100335));
#256742=CARTESIAN_POINT('Ctrl Pts',(-11.1893638596936,12.2,2.10097134800317));
#256743=CARTESIAN_POINT('Ctrl Pts',(-11.1863741376351,12.2,2.09884899499594));
#256744=CARTESIAN_POINT('Ctrl Pts',(-11.1833844150335,12.2,2.09672664160315));
#256745=CARTESIAN_POINT('Ctrl Pts',(-11.1803978179162,12.2,2.09461169692912));
#256746=CARTESIAN_POINT('Ctrl Pts',(-11.1774143863163,12.2,2.09250415858217));
#256747=CARTESIAN_POINT('Ctrl Pts',(-11.1744309552585,12.2,2.09039662061809));
#256748=CARTESIAN_POINT('Ctrl Pts',(-11.1714506910338,12.2,2.08829648901194));
#256749=CARTESIAN_POINT('Ctrl Pts',(-11.1684736354339,12.2,2.08620376154695));
#256750=CARTESIAN_POINT('Ctrl Pts',(-11.165496579834,12.2,2.08411103408196));
#256751=CARTESIAN_POINT('Ctrl Pts',(-11.1625227333362,12.2,2.08202571079862));
#256752=CARTESIAN_POINT('Ctrl Pts',(-11.159552137764,12.2,2.07994778928138));
#256753=CARTESIAN_POINT('Ctrl Pts',(-11.1565815421918,12.2,2.07786986776415));
#256754=CARTESIAN_POINT('Ctrl Pts',(-11.1536141978418,12.2,2.07579934706958));
#256755=CARTESIAN_POINT('Ctrl Pts',(-11.1506501482277,12.2,2.07373622601015));
#256756=CARTESIAN_POINT('Ctrl Pts',(-11.1476860986136,12.2,2.07167310495071));
#256757=CARTESIAN_POINT('Ctrl Pts',(-11.1447253432153,12.2,2.06961738211622));
#256758=CARTESIAN_POINT('Ctrl Pts',(-11.1417679255724,12.2,2.06756905652332));
#256759=CARTESIAN_POINT('Ctrl Pts',(-11.1388105079296,12.2,2.06552073093042));
#256760=CARTESIAN_POINT('Ctrl Pts',(-11.1358564272366,12.2,2.06347980013705));
#256761=CARTESIAN_POINT('Ctrl Pts',(-11.132905727135,12.2,2.06144626370992));
#256762=CARTESIAN_POINT('Ctrl Pts',(-11.1299550264973,12.2,2.05941272691336));
#256763=CARTESIAN_POINT('Ctrl Pts',(-11.1270077067523,12.2,2.05738658531891));
#256764=CARTESIAN_POINT('Ctrl Pts',(-11.1240638106583,12.2,2.05536783206819));
#256765=CARTESIAN_POINT('Ctrl Pts',(-11.1201386167575,12.2,2.05267616167846));
#256766=CARTESIAN_POINT('Ctrl Pts',(-11.1162195093366,12.2,2.04999763011203));
#256767=CARTESIAN_POINT('Ctrl Pts',(-11.112306594045,12.2,2.04733223021796));
#256768=CARTESIAN_POINT('Ctrl Pts',(-11.109371907443,12.2,2.04533318020661));
#256769=CARTESIAN_POINT('Ctrl Pts',(-11.1064407044901,12.2,2.0433415163118));
#256770=CARTESIAN_POINT('Ctrl Pts',(-11.1035130258665,12.2,2.04135723565891));
#256771=CARTESIAN_POINT('Ctrl Pts',(-11.1005853472429,12.2,2.03937295500603));
#256772=CARTESIAN_POINT('Ctrl Pts',(-11.0976611954311,12.2,2.03739605664207));
#256773=CARTESIAN_POINT('Ctrl Pts',(-11.0947406148701,12.2,2.03542653821263));
#256774=CARTESIAN_POINT('Ctrl Pts',(-11.0918200337784,12.2,2.03345701942538));
#256775=CARTESIAN_POINT('Ctrl Pts',(-11.0889030234212,12.2,2.03149488109023));
#256776=CARTESIAN_POINT('Ctrl Pts',(-11.0859896278733,12.2,2.02954011826547));
#256777=CARTESIAN_POINT('Ctrl Pts',(-11.0830762328546,12.2,2.02758535579584));
#256778=CARTESIAN_POINT('Ctrl Pts',(-11.0801664537774,12.2,2.02563796965079));
#256779=CARTESIAN_POINT('Ctrl Pts',(-11.077260334675,12.2,2.02369795609693));
#256780=CARTESIAN_POINT('Ctrl Pts',(-11.0743542155726,12.2,2.02175794254307));
#256781=CARTESIAN_POINT('Ctrl Pts',(-11.0714517553386,12.2,2.01982530095362));
#256782=CARTESIAN_POINT('Ctrl Pts',(-11.0685530007224,12.2,2.01790002801485));
#256783=CARTESIAN_POINT('Ctrl Pts',(-11.064687994743,12.2,2.01533299754641));
#256784=CARTESIAN_POINT('Ctrl Pts',(-11.0608295742239,12.2,2.01277906790344));
#256785=CARTESIAN_POINT('Ctrl Pts',(-11.0569778483715,12.2,2.01023822866536));
#256786=CARTESIAN_POINT('Ctrl Pts',(-11.0540890533261,12.2,2.00833259880407));
#256787=CARTESIAN_POINT('Ctrl Pts',(-11.0512040246068,12.2,2.00643433217819));
#256788=CARTESIAN_POINT('Ctrl Pts',(-11.0483228056053,12.2,2.00454342532106));
#256789=CARTESIAN_POINT('Ctrl Pts',(-11.0454415871271,12.2,2.00265251880743));
#256790=CARTESIAN_POINT('Ctrl Pts',(-11.0425641802321,12.2,2.0007689719934));
#256791=CARTESIAN_POINT('Ctrl Pts',(-11.0396906292119,12.2,1.99889277956221));
#256792=CARTESIAN_POINT('Ctrl Pts',(-11.0368170781916,12.2,1.99701658713102));
#256793=CARTESIAN_POINT('Ctrl Pts',(-11.0339473836063,12.2,1.99514775047236));
#256794=CARTESIAN_POINT('Ctrl Pts',(-11.0310815924891,12.2,1.99328626444825));
#256795=CARTESIAN_POINT('Ctrl Pts',(-11.0282158013719,12.2,1.99142477842413));
#256796=CARTESIAN_POINT('Ctrl Pts',(-11.0253539118618,12.2,1.98957064284293));
#256797=CARTESIAN_POINT('Ctrl Pts',(-11.0224959722443,12.2,1.98772385427662));
#256798=CARTESIAN_POINT('Ctrl Pts',(-11.0196380326268,12.2,1.98587706571031));
#256799=CARTESIAN_POINT('Ctrl Pts',(-11.0167840410575,12.2,1.98403762348383));
#256800=CARTESIAN_POINT('Ctrl Pts',(-11.0139340455357,12.2,1.98220552292476));
#256801=CARTESIAN_POINT('Ctrl Pts',(-11.0110840500139,12.2,1.98037342236568));
#256802=CARTESIAN_POINT('Ctrl Pts',(-11.0082380505669,12.2,1.97854866256446));
#256803=CARTESIAN_POINT('Ctrl Pts',(-11.0053960925862,12.2,1.97673124137947));
#256804=CARTESIAN_POINT('Ctrl Pts',(-11.0016068149345,12.2,1.97430801291271));
#256805=CARTESIAN_POINT('Ctrl Pts',(-10.9978247251842,12.2,1.97189782577868));
#256806=CARTESIAN_POINT('Ctrl Pts',(-10.9940499322391,12.2,1.96950067274831));
#256807=CARTESIAN_POINT('Ctrl Pts',(-10.9912188377875,12.2,1.96770280813883));
#256808=CARTESIAN_POINT('Ctrl Pts',(-10.9883918487295,12.2,1.9659122732949));
#256809=CARTESIAN_POINT('Ctrl Pts',(-10.9855690122359,12.2,1.96412906376822));
#256810=CARTESIAN_POINT('Ctrl Pts',(-10.9808642845756,12.2,1.96115704778245));
#256811=CARTESIAN_POINT('Ctrl Pts',(-10.9761710913778,12.2,1.95820538052215));
#256812=CARTESIAN_POINT('Ctrl Pts',(-10.9714896552667,12.2,1.95527403704994));
#256813=CARTESIAN_POINT('Ctrl Pts',(-10.9677445061737,12.2,1.95292896214436));
#256814=CARTESIAN_POINT('Ctrl Pts',(-10.9640068804816,12.2,1.95059689372084));
#256815=CARTESIAN_POINT('Ctrl Pts',(-10.9602768933902,12.2,1.94827782009577));
#256816=CARTESIAN_POINT('Ctrl Pts',(-10.956546906807,12.2,1.94595874678669));
#256817=CARTESIAN_POINT('Ctrl Pts',(-10.9528245569269,12.2,1.9436526678134));
#256818=CARTESIAN_POINT('Ctrl Pts',(-10.9491099617692,12.2,1.94135956976817));
#256819=CARTESIAN_POINT('Ctrl Pts',(-10.9453953661054,12.2,1.9390664714105));
#256820=CARTESIAN_POINT('Ctrl Pts',(-10.9416885241238,12.2,1.9367863525904));
#256821=CARTESIAN_POINT('Ctrl Pts',(-10.9379895511452,12.2,1.93451920157926));
#256822=CARTESIAN_POINT('Ctrl Pts',(-10.9342905786707,12.2,1.93225205087702));
#256823=CARTESIAN_POINT('Ctrl Pts',(-10.9305994763479,12.2,1.92999786564257));
#256824=CARTESIAN_POINT('Ctrl Pts',(-10.9269163592595,12.2,1.92775663365828));
#256825=CARTESIAN_POINT('Ctrl Pts',(-10.9232332416694,12.2,1.92551540136861));
#256826=CARTESIAN_POINT('Ctrl Pts',(-10.9195581105475,12.2,1.92328712034772));
#256827=CARTESIAN_POINT('Ctrl Pts',(-10.915891083443,12.2,1.92107177789522));
#256828=CARTESIAN_POINT('Ctrl Pts',(-10.912224056838,12.2,1.91885643574456));
#256829=CARTESIAN_POINT('Ctrl Pts',(-10.9085651348257,12.2,1.91665403099813));
#256830=CARTESIAN_POINT('Ctrl Pts',(-10.9049144362902,12.2,1.91446454645404));
#256831=CARTESIAN_POINT('Ctrl Pts',(-10.9012637372574,12.2,1.91227506161164));
#256832=CARTESIAN_POINT('Ctrl Pts',(-10.8976212607477,12.2,1.91009849932637));
#256833=CARTESIAN_POINT('Ctrl Pts',(-10.8939871264947,12.2,1.90793484359818));
#256834=CARTESIAN_POINT('Ctrl Pts',(-10.8903529927368,12.2,1.90577118816479));
#256835=CARTESIAN_POINT('Ctrl Pts',(-10.8867272019107,12.2,1.90362043739894));
#256836=CARTESIAN_POINT('Ctrl Pts',(-10.883109874025,12.2,1.90148257657689));
#256837=CARTESIAN_POINT('Ctrl Pts',(-10.8794925456464,12.2,1.89934471546356));
#256838=CARTESIAN_POINT('Ctrl Pts',(-10.8758836817098,12.2,1.89721974375));
#256839=CARTESIAN_POINT('Ctrl Pts',(-10.8722834026808,12.2,1.89510764413572));
#256840=CARTESIAN_POINT('Ctrl Pts',(-10.8686831241423,12.2,1.89299554480923));
#256841=CARTESIAN_POINT('Ctrl Pts',(-10.86509142983,12.2,1.89089631741071));
#256842=CARTESIAN_POINT('Ctrl Pts',(-10.8615084435108,12.2,1.88880994535773));
#256843=CARTESIAN_POINT('Ctrl Pts',(-10.8579254567035,12.2,1.88672357302047));
#256844=CARTESIAN_POINT('Ctrl Pts',(-10.854351178372,12.2,1.88465005566183));
#256845=CARTESIAN_POINT('Ctrl Pts',(-10.8507857307726,12.2,1.88258937470686));
#256846=CARTESIAN_POINT('Ctrl Pts',(-10.8463289215163,12.2,1.88001352365354));
#256847=CARTESIAN_POINT('Ctrl Pts',(-10.8418859114319,12.2,1.87745772979982));
#256848=CARTESIAN_POINT('Ctrl Pts',(-10.8374569440021,12.2,1.87492195709255));
#256849=CARTESIAN_POINT('Ctrl Pts',(-10.8339137703479,12.2,1.87289333909257));
#256850=CARTESIAN_POINT('Ctrl Pts',(-10.8303795850586,12.2,1.87087753549001));
#256851=CARTESIAN_POINT('Ctrl Pts',(-10.826854512068,12.2,1.8688745248191));
#256852=CARTESIAN_POINT('Ctrl Pts',(-10.8233294385972,12.2,1.86687151387529));
#256853=CARTESIAN_POINT('Ctrl Pts',(-10.8198134797272,12.2,1.86488129701604));
#256854=CARTESIAN_POINT('Ctrl Pts',(-10.8163067602584,12.2,1.8629038547416));
#256855=CARTESIAN_POINT('Ctrl Pts',(-10.8128000407895,12.2,1.86092641246716));
#256856=CARTESIAN_POINT('Ctrl Pts',(-10.8093025624355,12.2,1.85896174480533));
#256857=CARTESIAN_POINT('Ctrl Pts',(-10.8058144529131,12.2,1.85700983042247));
#256858=CARTESIAN_POINT('Ctrl Pts',(-10.8023263438658,12.2,1.85505791630556));
#256859=CARTESIAN_POINT('Ctrl Pts',(-10.7988476032401,12.2,1.85311875575534));
#256860=CARTESIAN_POINT('Ctrl Pts',(-10.7953783602857,12.2,1.85119232829292));
#256861=CARTESIAN_POINT('Ctrl Pts',(-10.7910418062382,12.2,1.84878429376803));
#256862=CARTESIAN_POINT('Ctrl Pts',(-10.7867200937389,12.2,1.84639615449994));
#256863=CARTESIAN_POINT('Ctrl Pts',(-10.7824134763083,12.2,1.8440278667916));
#256864=CARTESIAN_POINT('Ctrl Pts',(-10.7789681821761,12.2,1.84213323652166));
#256865=CARTESIAN_POINT('Ctrl Pts',(-10.7755325486423,12.2,1.84025131212824));
#256866=CARTESIAN_POINT('Ctrl Pts',(-10.7721067084566,12.2,1.83838207169433));
#256867=CARTESIAN_POINT('Ctrl Pts',(-10.7686808687376,12.2,1.8365128315151));
#256868=CARTESIAN_POINT('Ctrl Pts',(-10.7652648222977,12.2,1.83465627335054));
#256869=CARTESIAN_POINT('Ctrl Pts',(-10.7618587007273,12.2,1.83281237599286));
#256870=CARTESIAN_POINT('Ctrl Pts',(-10.7584525786929,12.2,1.83096847838395));
#256871=CARTESIAN_POINT('Ctrl Pts',(-10.7550563838744,12.2,1.8291372410532));
#256872=CARTESIAN_POINT('Ctrl Pts',(-10.7516702479131,12.2,1.8273186406776));
#256873=CARTESIAN_POINT('Ctrl Pts',(-10.7482841124131,12.2,1.82550004054978));
#256874=CARTESIAN_POINT('Ctrl Pts',(-10.744908038873,12.2,1.82369407782311));
#256875=CARTESIAN_POINT('Ctrl Pts',(-10.7415421592586,12.2,1.82190072641333));
#256876=CARTESIAN_POINT('Ctrl Pts',(-10.7381762791856,12.2,1.82010737475919));
#256877=CARTESIAN_POINT('Ctrl Pts',(-10.7348205957021,12.2,1.81832663631315));
#256878=CARTESIAN_POINT('Ctrl Pts',(-10.731475242798,12.2,1.8165584851851));
#256879=CARTESIAN_POINT('Ctrl Pts',(-10.7281298903497,12.2,1.81479033429797));
#256880=CARTESIAN_POINT('Ctrl Pts',(-10.7247948705591,12.2,1.8130347697981));
#256881=CARTESIAN_POINT('Ctrl Pts',(-10.7214703203302,12.2,1.81129176888421));
#256882=CARTESIAN_POINT('Ctrl Pts',(-10.7181457696483,12.2,1.80954876773283));
#256883=CARTESIAN_POINT('Ctrl Pts',(-10.7148316892511,12.2,1.8078183278052));
#256884=CARTESIAN_POINT('Ctrl Pts',(-10.7115282172384,12.2,1.80610042410129));
#256885=CARTESIAN_POINT('Ctrl Pts',(-10.7082247456758,12.2,1.80438252063144));
#256886=CARTESIAN_POINT('Ctrl Pts',(-10.7049318838535,12.2,1.80267715266237));
#256887=CARTESIAN_POINT('Ctrl Pts',(-10.7016497702347,12.2,1.80098429377065));
#256888=CARTESIAN_POINT('Ctrl Pts',(-10.6983676561686,12.2,1.79929143464827));
#256889=CARTESIAN_POINT('Ctrl Pts',(-10.6950962930856,12.2,1.79761108425657));
#256890=CARTESIAN_POINT('Ctrl Pts',(-10.6918358197419,12.2,1.79594321588871));
#256891=CARTESIAN_POINT('Ctrl Pts',(-10.6885753468425,12.2,1.79427534774809));
#256892=CARTESIAN_POINT('Ctrl Pts',(-10.6853257655437,12.2,1.79261996002721));
#256893=CARTESIAN_POINT('Ctrl Pts',(-10.6820872180295,12.2,1.79097702699356));
#256894=CARTESIAN_POINT('Ctrl Pts',(-10.6788486700741,12.2,1.78933409373607));
#256895=CARTESIAN_POINT('Ctrl Pts',(-10.6756211575154,12.2,1.78770361239432));
#256896=CARTESIAN_POINT('Ctrl Pts',(-10.6724048222145,12.2,1.78608555596551));
#256897=CARTESIAN_POINT('Ctrl Pts',(-10.6691884873518,12.2,1.78446749975716));
#256898=CARTESIAN_POINT('Ctrl Pts',(-10.6659833306206,12.2,1.78286186684534));
#256899=CARTESIAN_POINT('Ctrl Pts',(-10.6627894990472,12.2,1.7812686292521));
#256900=CARTESIAN_POINT('Ctrl Pts',(-10.6595956670386,12.2,1.77967539144178));
#256901=CARTESIAN_POINT('Ctrl Pts',(-10.6564131598367,12.2,1.77809454808542));
#256902=CARTESIAN_POINT('Ctrl Pts',(-10.653242123275,12.2,1.77652606899993));
#256903=CARTESIAN_POINT('Ctrl Pts',(-10.6500710867133,12.2,1.77495758991445));
#256904=CARTESIAN_POINT('Ctrl Pts',(-10.6469115219807,12.2,1.77340147336653));
#256905=CARTESIAN_POINT('Ctrl Pts',(-10.643763577977,12.2,1.77185769100587));
#256906=CARTESIAN_POINT('Ctrl Pts',(-10.6406156344022,12.2,1.77031390885555));
#256907=CARTESIAN_POINT('Ctrl Pts',(-10.6374793102082,12.2,1.76878245902262));
#256908=CARTESIAN_POINT('Ctrl Pts',(-10.6343547567271,12.2,1.76726331125097));
#256909=CARTESIAN_POINT('Ctrl Pts',(-10.6312302028204,12.2,1.76574416327235));
#256910=CARTESIAN_POINT('Ctrl Pts',(-10.6281174206275,12.2,1.76423731434967));
#256911=CARTESIAN_POINT('Ctrl Pts',(-10.6250165594597,12.2,1.76274273521391));
#256912=CARTESIAN_POINT('Ctrl Pts',(-10.6219156987144,12.2,1.76124815628179));
#256913=CARTESIAN_POINT('Ctrl Pts',(-10.6188267599592,12.2,1.75976584533418));
#256914=CARTESIAN_POINT('Ctrl Pts',(-10.6157498970433,12.2,1.75829576912023));
#256915=CARTESIAN_POINT('Ctrl Pts',(-10.6126730337082,12.2,1.75682569270598));
#256916=CARTESIAN_POINT('Ctrl Pts',(-10.609608245111,12.2,1.75536785109296));
#256917=CARTESIAN_POINT('Ctrl Pts',(-10.6065556865155,12.2,1.7539222093319));
#256918=CARTESIAN_POINT('Ctrl Pts',(-10.6035031283358,12.2,1.75247656776782));
#256919=CARTESIAN_POINT('Ctrl Pts',(-10.6004628009815,12.2,1.75104312744808));
#256920=CARTESIAN_POINT('Ctrl Pts',(-10.597434859506,12.2,1.74962185184124));
#256921=CARTESIAN_POINT('Ctrl Pts',(-10.5928929466739,12.2,1.74748993814051));
#256922=CARTESIAN_POINT('Ctrl Pts',(-10.588378903462,12.2,1.74538539612655));
#256923=CARTESIAN_POINT('Ctrl Pts',(-10.5838932628027,12.2,1.74330810526518));
#256924=CARTESIAN_POINT('Ctrl Pts',(-10.5801552295312,12.2,1.74157702983041));
#256925=CARTESIAN_POINT('Ctrl Pts',(-10.5764369226267,12.2,1.73986487718285));
#256926=CARTESIAN_POINT('Ctrl Pts',(-10.5727386527504,12.2,1.73817157521309));
#256927=CARTESIAN_POINT('Ctrl Pts',(-10.569040382471,12.2,1.73647827305876));
#256928=CARTESIAN_POINT('Ctrl Pts',(-10.5653621528857,12.2,1.7348038211847));
#256929=CARTESIAN_POINT('Ctrl Pts',(-10.5617042777451,12.2,1.73314814493317));
#256930=CARTESIAN_POINT('Ctrl Pts',(-10.5580464026046,12.2,1.73149246868164));
#256931=CARTESIAN_POINT('Ctrl Pts',(-10.5544088858359,12.2,1.72985556749646));
#256932=CARTESIAN_POINT('Ctrl Pts',(-10.5507920472231,12.2,1.72823736520327));
#256933=CARTESIAN_POINT('Ctrl Pts',(-10.5471752086103,12.2,1.72661916291008));
#256934=CARTESIAN_POINT('Ctrl Pts',(-10.543579050384,12.2,1.72501965880824));
#256935=CARTESIAN_POINT('Ctrl Pts',(-10.5400038958984,12.2,1.72343877240852));
#256936=CARTESIAN_POINT('Ctrl Pts',(-10.5364287414128,12.2,1.72185788600881));
#256937=CARTESIAN_POINT('Ctrl Pts',(-10.5328745943267,12.2,1.72029561860198));
#256938=CARTESIAN_POINT('Ctrl Pts',(-10.5293417840478,12.2,1.71875188735101));
#256939=CARTESIAN_POINT('Ctrl Pts',(-10.525808973769,12.2,1.71720815610005));
#256940=CARTESIAN_POINT('Ctrl Pts',(-10.5222975002351,12.2,1.71568296326067));
#256941=CARTESIAN_POINT('Ctrl Pts',(-10.51880770072,12.2,1.71417622110692));
#256942=CARTESIAN_POINT('Ctrl Pts',(-10.515317901205,12.2,1.71266947895318));
#256943=CARTESIAN_POINT('Ctrl Pts',(-10.5118497737009,12.2,1.71118118890747));
#256944=CARTESIAN_POINT('Ctrl Pts',(-10.5084036609769,12.2,1.70971126577574));
#256945=CARTESIAN_POINT('Ctrl Pts',(-10.5049575482528,12.2,1.70824134264402));
#256946=CARTESIAN_POINT('Ctrl Pts',(-10.5015334497333,12.2,1.70678978567216));
#256947=CARTESIAN_POINT('Ctrl Pts',(-10.4981317097333,12.2,1.70535650428327));
#256948=CARTESIAN_POINT('Ctrl Pts',(-10.4947299697333,12.2,1.70392322289439));
#256949=CARTESIAN_POINT('Ctrl Pts',(-10.4913505917578,12.2,1.70250821758881));
#256950=CARTESIAN_POINT('Ctrl Pts',(-10.4879939225065,12.2,1.70111139779085));
#256951=CARTESIAN_POINT('Ctrl Pts',(-10.4846372532552,12.2,1.69971457799288));
#256952=CARTESIAN_POINT('Ctrl Pts',(-10.4813032944324,12.2,1.6983359434379));
#256953=CARTESIAN_POINT('Ctrl Pts',(-10.4779924025586,12.2,1.69697539941107));
#256954=CARTESIAN_POINT('Ctrl Pts',(-10.4746815106848,12.2,1.69561485538424));
#256955=CARTESIAN_POINT('Ctrl Pts',(-10.471393684391,12.2,1.69427240205694));
#256956=CARTESIAN_POINT('Ctrl Pts',(-10.4681292867533,12.2,1.69294794219676));
#256957=CARTESIAN_POINT('Ctrl Pts',(-10.4648648891156,12.2,1.69162348233659));
#256958=CARTESIAN_POINT('Ctrl Pts',(-10.4616239186746,12.2,1.69031701576354));
#256959=CARTESIAN_POINT('Ctrl Pts',(-10.4584067433766,12.2,1.68902844257542));
#256960=CARTESIAN_POINT('Ctrl Pts',(-10.4551895680787,12.2,1.68773986938729));
#256961=CARTESIAN_POINT('Ctrl Pts',(-10.4519961881502,12.2,1.68646919123461));
#256962=CARTESIAN_POINT('Ctrl Pts',(-10.4488269748188,12.2,1.68521630311107));
#256963=CARTESIAN_POINT('Ctrl Pts',(-10.4456577614874,12.2,1.68396341498752));
#256964=CARTESIAN_POINT('Ctrl Pts',(-10.4425127162509,12.2,1.68272831855038));
#256965=CARTESIAN_POINT('Ctrl Pts',(-10.4393922155585,12.2,1.68151090785737));
#256966=CARTESIAN_POINT('Ctrl Pts',(-10.4356476148636,12.2,1.68005001507885));
#256967=CARTESIAN_POINT('Ctrl Pts',(-10.4319383614733,12.2,1.6786145889792));
#256968=CARTESIAN_POINT('Ctrl Pts',(-10.4282651168583,12.2,1.6772044439482));
#256969=CARTESIAN_POINT('Ctrl Pts',(-10.4245918722433,12.2,1.67579429891719));
#256970=CARTESIAN_POINT('Ctrl Pts',(-10.4209546380505,12.2,1.67440943047585));
#256971=CARTESIAN_POINT('Ctrl Pts',(-10.4173540951797,12.2,1.67304964952415));
#256972=CARTESIAN_POINT('Ctrl Pts',(-10.4137535523089,12.2,1.67168986857245));
#256973=CARTESIAN_POINT('Ctrl Pts',(-10.4101896957755,12.2,1.67035517200516));
#256974=CARTESIAN_POINT('Ctrl Pts',(-10.4066632229011,12.2,1.66904535913438));
#256975=CARTESIAN_POINT('Ctrl Pts',(-10.4031367497063,12.2,1.66773554614464));
#256976=CARTESIAN_POINT('Ctrl Pts',(-10.3996476556151,12.2,1.6664506182323));
#256977=CARTESIAN_POINT('Ctrl Pts',(-10.3961966495954,12.2,1.66519036616469));
#256978=CARTESIAN_POINT('Ctrl Pts',(-10.3927456438891,12.2,1.66393011421156));
#256979=CARTESIAN_POINT('Ctrl Pts',(-10.389332722886,12.2,1.66269453712038));
#256980=CARTESIAN_POINT('Ctrl Pts',(-10.3859586112432,12.2,1.66148342124216));
#256981=CARTESIAN_POINT('Ctrl Pts',(-10.3825844996004,12.2,1.66027230536394));
#256982=CARTESIAN_POINT('Ctrl Pts',(-10.3792491944922,12.2,1.65908565032773));
#256983=CARTESIAN_POINT('Ctrl Pts',(-10.3759534311092,12.2,1.65792323511832));
#256984=CARTESIAN_POINT('Ctrl Pts',(-10.3726576674269,12.2,1.65676081980332));
#256985=CARTESIAN_POINT('Ctrl Pts',(-10.3694014467392,12.2,1.65562264058221));
#256986=CARTESIAN_POINT('Ctrl Pts',(-10.3661855189056,12.2,1.65450847138389));
#256987=CARTESIAN_POINT('Ctrl Pts',(-10.3629695913642,12.2,1.65339430228676));
#256988=CARTESIAN_POINT('Ctrl Pts',(-10.3597939584194,12.2,1.65230414139452));
#256989=CARTESIAN_POINT('Ctrl Pts',(-10.3566593852,12.2,1.6512377512666));
#256990=CARTESIAN_POINT('Ctrl Pts',(-10.3535248119805,12.2,1.65017136113868));
#256991=CARTESIAN_POINT('Ctrl Pts',(-10.3504312997662,12.2,1.64912874083394));
#256992=CARTESIAN_POINT('Ctrl Pts',(-10.3473796326243,12.2,1.64810964478603));
#256993=CARTESIAN_POINT('Ctrl Pts',(-10.3443279652051,12.2,1.64709054864556));
#256994=CARTESIAN_POINT('Ctrl Pts',(-10.3413181436622,12.2,1.64609497698116));
#256995=CARTESIAN_POINT('Ctrl Pts',(-10.3383509672714,12.2,1.64512267463094));
#256996=CARTESIAN_POINT('Ctrl Pts',(-10.3353837911501,12.2,1.64415037236905));
#256997=CARTESIAN_POINT('Ctrl Pts',(-10.3324592641453,12.2,1.6432013387413));
#256998=CARTESIAN_POINT('Ctrl Pts',(-10.32957820325,12.2,1.64227531152494));
#256999=CARTESIAN_POINT('Ctrl Pts',(-10.3266971423546,12.2,1.64134928430858));
#257000=CARTESIAN_POINT('Ctrl Pts',(-10.3238595497276,12.2,1.6404462632318));
#257001=CARTESIAN_POINT('Ctrl Pts',(-10.3210662645203,12.2,1.63956597488516));
#257002=CARTESIAN_POINT('Ctrl Pts',(-10.3182729790593,12.2,1.63868568645855));
#257003=CARTESIAN_POINT('Ctrl Pts',(-10.3155239995829,12.2,1.63782813033625));
#257004=CARTESIAN_POINT('Ctrl Pts',(-10.3128201892719,12.2,1.63699302495893));
#257005=CARTESIAN_POINT('Ctrl Pts',(-10.3101163792066,12.2,1.63615791965746));
#257006=CARTESIAN_POINT('Ctrl Pts',(-10.3074577337573,12.2,1.63534526372441));
#257007=CARTESIAN_POINT('Ctrl Pts',(-10.3048451387571,12.2,1.63455476724959));
#257008=CARTESIAN_POINT('Ctrl Pts',(-10.302232543757,12.2,1.63376427077477));
#257009=CARTESIAN_POINT('Ctrl Pts',(-10.299665995598,12.2,1.63299593268122));
#257010=CARTESIAN_POINT('Ctrl Pts',(-10.2971463988542,12.2,1.63224944754072));
#257011=CARTESIAN_POINT('Ctrl Pts',(-10.2946268018815,12.2,1.63150296233242));
#257012=CARTESIAN_POINT('Ctrl Pts',(-10.2921541558229,12.2,1.63077833360183));
#257013=CARTESIAN_POINT('Ctrl Pts',(-10.289729386944,12.2,1.63007524598165));
#257014=CARTESIAN_POINT('Ctrl Pts',(-10.2873046182854,12.2,1.62937215842533));
#257015=CARTESIAN_POINT('Ctrl Pts',(-10.2849277259532,12.2,1.6286906116558));
#257016=CARTESIAN_POINT('Ctrl Pts',(-10.2825996603733,12.2,1.62803028118072));
#257017=CARTESIAN_POINT('Ctrl Pts',(-10.2802715947934,12.2,1.62736995070563));
#257018=CARTESIAN_POINT('Ctrl Pts',(-10.2779923555595,12.2,1.62673083689551));
#257019=CARTESIAN_POINT('Ctrl Pts',(-10.2757629181383,12.2,1.62611260225039));
#257020=CARTESIAN_POINT('Ctrl Pts',(-10.2735334807172,12.2,1.62549436760528));
#257021=CARTESIAN_POINT('Ctrl Pts',(-10.2713538452582,12.2,1.62489701219327));
#257022=CARTESIAN_POINT('Ctrl Pts',(-10.2692250129987,12.2,1.62432018654616));
#257023=CARTESIAN_POINT('Ctrl Pts',(-10.2670961805458,12.2,1.62374336084665));
#257024=CARTESIAN_POINT('Ctrl Pts',(-10.2650181509812,12.2,1.62318706577415));
#257025=CARTESIAN_POINT('Ctrl Pts',(-10.2629919538731,12.2,1.62265093799582));
#257026=CARTESIAN_POINT('Ctrl Pts',(-10.260965756949,12.2,1.62211481026618));
#257027=CARTESIAN_POINT('Ctrl Pts',(-10.2589913939399,12.2,1.62159884971778));
#257028=CARTESIAN_POINT('Ctrl Pts',(-10.2570699210009,12.2,1.62110268273351));
#257029=CARTESIAN_POINT('Ctrl Pts',(-10.2538766876538,12.2,1.62027811896908));
#257030=CARTESIAN_POINT('Ctrl Pts',(-10.2508295201298,12.2,1.61950823569637));
#257031=CARTESIAN_POINT('Ctrl Pts',(-10.2479334570001,12.2,1.61879117999999));
#257032=CARTESIAN_POINT('Ctrl Pts',(-10.2479334570001,15.2,1.61879117999999));
#257033=CARTESIAN_POINT('Ctrl Pts',(-10.249667749424,15.2,1.61922058509445));
#257034=CARTESIAN_POINT('Ctrl Pts',(-10.2514562330726,15.2,1.61966892566345));
#257035=CARTESIAN_POINT('Ctrl Pts',(-10.2532978200233,15.2,1.6201366211404));
#257036=CARTESIAN_POINT('Ctrl Pts',(-10.2551482880371,15.2,1.62060657208134));
#257037=CARTESIAN_POINT('Ctrl Pts',(-10.257052368982,15.2,1.62109605778657));
#257038=CARTESIAN_POINT('Ctrl Pts',(-10.2590089861894,15.2,1.62160546159094));
#257039=CARTESIAN_POINT('Ctrl Pts',(-10.2609656032191,15.2,1.62211486534904));
#257040=CARTESIAN_POINT('Ctrl Pts',(-10.2629747532248,15.2,1.62264418861991));
#257041=CARTESIAN_POINT('Ctrl Pts',(-10.2650353904833,15.2,1.62319380126661));
#257042=CARTESIAN_POINT('Ctrl Pts',(-10.2670960277418,15.2,1.62374341391331));
#257043=CARTESIAN_POINT('Ctrl Pts',(-10.2692081522727,15.2,1.62431331751935));
#257044=CARTESIAN_POINT('Ctrl Pts',(-10.2713707425492,15.2,1.62490386819287));
#257045=CARTESIAN_POINT('Ctrl Pts',(-10.2735333330222,15.2,1.62549441892003));
#257046=CARTESIAN_POINT('Ctrl Pts',(-10.2757463899782,15.2,1.62610561795797));
#257047=CARTESIAN_POINT('Ctrl Pts',(-10.2780089205216,15.2,1.62673780957719));
#257048=CARTESIAN_POINT('Ctrl Pts',(-10.2806485391806,15.2,1.62747536638016));
#257049=CARTESIAN_POINT('Ctrl Pts',(-10.2833554975187,15.2,1.6282414973953));
#257050=CARTESIAN_POINT('Ctrl Pts',(-10.2861282602868,15.2,1.6290367294674));
#257051=CARTESIAN_POINT('Ctrl Pts',(-10.2885049143657,15.2,1.62971835703736));
#257052=CARTESIAN_POINT('Ctrl Pts',(-10.2909299187482,15.2,1.63042136553797));
#257053=CARTESIAN_POINT('Ctrl Pts',(-10.2934023335528,15.2,1.63114607307894));
#257054=CARTESIAN_POINT('Ctrl Pts',(-10.2958747481328,15.2,1.63187078055409));
#257055=CARTESIAN_POINT('Ctrl Pts',(-10.2983945737993,15.2,1.63261718678302));
#257056=CARTESIAN_POINT('Ctrl Pts',(-10.3009608947178,15.2,1.63338560200863));
#257057=CARTESIAN_POINT('Ctrl Pts',(-10.3035272156363,15.2,1.63415401723425));
#257058=CARTESIAN_POINT('Ctrl Pts',(-10.3061400361122,15.2,1.63494443990291));
#257059=CARTESIAN_POINT('Ctrl Pts',(-10.308798459097,15.2,1.63575716820575));
#257060=CARTESIAN_POINT('Ctrl Pts',(-10.3114568823232,15.2,1.6365698965824));
#257061=CARTESIAN_POINT('Ctrl Pts',(-10.3141609111968,15.2,1.63740492996182));
#257062=CARTESIAN_POINT('Ctrl Pts',(-10.3169096745163,15.2,1.63826255634343));
#257063=CARTESIAN_POINT('Ctrl Pts',(-10.3196584375861,15.2,1.63912018264714));
#257064=CARTESIAN_POINT('Ctrl Pts',(-10.3224519353476,15.2,1.64000040111441));
#257065=CARTESIAN_POINT('Ctrl Pts',(-10.3252893183298,15.2,1.64090349124926));
#257066=CARTESIAN_POINT('Ctrl Pts',(-10.3281267013119,15.2,1.64180658138411));
#257067=CARTESIAN_POINT('Ctrl Pts',(-10.3310079696406,15.2,1.64273254179215));
#257068=CARTESIAN_POINT('Ctrl Pts',(-10.3339322926158,15.2,1.64368164017332));
#257069=CARTESIAN_POINT('Ctrl Pts',(-10.3368566155909,15.2,1.64463073855448));
#257070=CARTESIAN_POINT('Ctrl Pts',(-10.3398239930841,15.2,1.64560297667086));
#257071=CARTESIAN_POINT('Ctrl Pts',(-10.3428336151386,15.2,1.64659861188309));
#257072=CARTESIAN_POINT('Ctrl Pts',(-10.3458432374665,15.2,1.64759424718577));
#257073=CARTESIAN_POINT('Ctrl Pts',(-10.3488951026067,15.2,1.64861328026567));
#257074=CARTESIAN_POINT('Ctrl Pts',(-10.3519884191937,15.2,1.64965596232354));
#257075=CARTESIAN_POINT('Ctrl Pts',(-10.3550817354998,15.2,1.65069864428669));
#257076=CARTESIAN_POINT('Ctrl Pts',(-10.3582165021609,15.2,1.6517649734646));
#257077=CARTESIAN_POINT('Ctrl Pts',(-10.3613919443771,15.2,1.65285519442396));
#257078=CARTESIAN_POINT('Ctrl Pts',(-10.3645673865933,15.2,1.65394541538332));
#257079=CARTESIAN_POINT('Ctrl Pts',(-10.3677835035911,15.2,1.65505952521889));
#257080=CARTESIAN_POINT('Ctrl Pts',(-10.3710395368868,15.2,1.65619776034255));
#257081=CARTESIAN_POINT('Ctrl Pts',(-10.3742955704781,15.2,1.6573359955696));
#257082=CARTESIAN_POINT('Ctrl Pts',(-10.3775915191068,15.2,1.65849835564065));
#257083=CARTESIAN_POINT('Ctrl Pts',(-10.3809266408736,15.2,1.65968506578972));
#257084=CARTESIAN_POINT('Ctrl Pts',(-10.3848176158138,15.2,1.66106956080195));
#257085=CARTESIAN_POINT('Ctrl Pts',(-10.3887619087675,15.2,1.66248720085672));
#257086=CARTESIAN_POINT('Ctrl Pts',(-10.3927583656266,15.2,1.6639383310977));
#257087=CARTESIAN_POINT('Ctrl Pts',(-10.3961839004773,15.2,1.6651821571638));
#257088=CARTESIAN_POINT('Ctrl Pts',(-10.3996477608152,15.2,1.66645058776564));
#257089=CARTESIAN_POINT('Ctrl Pts',(-10.4031492356743,15.2,1.66774383383719));
#257090=CARTESIAN_POINT('Ctrl Pts',(-10.4066507102154,15.2,1.66903707979128));
#257091=CARTESIAN_POINT('Ctrl Pts',(-10.4101897996955,15.2,1.67035514123376));
#257092=CARTESIAN_POINT('Ctrl Pts',(-10.4137658072484,15.2,1.671698221941));
#257093=CARTESIAN_POINT('Ctrl Pts',(-10.4173418148013,15.2,1.67304130264824));
#257094=CARTESIAN_POINT('Ctrl Pts',(-10.4209547402873,15.2,1.67440940080042));
#257095=CARTESIAN_POINT('Ctrl Pts',(-10.4246039011522,15.2,1.67580271658141));
#257096=CARTESIAN_POINT('Ctrl Pts',(-10.4282530623487,15.2,1.67719603248896));
#257097=CARTESIAN_POINT('Ctrl Pts',(-10.4319384591359,15.2,1.67861456248737));
#257098=CARTESIAN_POINT('Ctrl Pts',(-10.43565942236,15.2,1.68005849763969));
#257099=CARTESIAN_POINT('Ctrl Pts',(-10.4387602248778,15.2,1.6812617768677));
#257100=CARTESIAN_POINT('Ctrl Pts',(-10.4418857253989,15.2,1.6824826993383));
#257101=CARTESIAN_POINT('Ctrl Pts',(-10.4450355444287,15.2,1.68372137093697));
#257102=CARTESIAN_POINT('Ctrl Pts',(-10.4481853634584,15.2,1.68496004253563));
#257103=CARTESIAN_POINT('Ctrl Pts',(-10.4513595001386,15.2,1.68621646360405));
#257104=CARTESIAN_POINT('Ctrl Pts',(-10.4545575793766,15.2,1.68749073763329));
#257105=CARTESIAN_POINT('Ctrl Pts',(-10.4577556582661,15.2,1.68876501152363));
#257106=CARTESIAN_POINT('Ctrl Pts',(-10.4609776819034,15.2,1.69005713877285));
#257107=CARTESIAN_POINT('Ctrl Pts',(-10.4642232782838,15.2,1.69136722008692));
#257108=CARTESIAN_POINT('Ctrl Pts',(-10.4681179945771,15.2,1.69293931792085));
#257109=CARTESIAN_POINT('Ctrl Pts',(-10.4720466563404,15.2,1.69453726941559));
#257110=CARTESIAN_POINT('Ctrl Pts',(-10.4760086384744,15.2,1.69616124333856));
#257111=CARTESIAN_POINT('Ctrl Pts',(-10.4793102900728,15.2,1.69751455486727));
#257112=CARTESIAN_POINT('Ctrl Pts',(-10.4826350783087,15.2,1.69888593766284));
#257113=CARTESIAN_POINT('Ctrl Pts',(-10.4859826493804,15.2,1.70027548738631));
#257114=CARTESIAN_POINT('Ctrl Pts',(-10.489330220452,15.2,1.70166503710978));
#257115=CARTESIAN_POINT('Ctrl Pts',(-10.4927005713142,15.2,1.70307275317942));
#257116=CARTESIAN_POINT('Ctrl Pts',(-10.4960933524271,15.2,1.70449872790313));
#257117=CARTESIAN_POINT('Ctrl Pts',(-10.5001646896147,15.2,1.70620989750942));
#257118=CARTESIAN_POINT('Ctrl Pts',(-10.5042683258583,15.2,1.70794735808176));
#257119=CARTESIAN_POINT('Ctrl Pts',(-10.5084036609769,15.2,1.70971126577574));
#257120=CARTESIAN_POINT('Ctrl Pts',(-10.5125389960955,15.2,1.71147517346972));
#257121=CARTESIAN_POINT('Ctrl Pts',(-10.5167060311669,15.2,1.71326553015153));
#257122=CARTESIAN_POINT('Ctrl Pts',(-10.520904178263,15.2,1.71508248091769));
#257123=CARTESIAN_POINT('Ctrl Pts',(-10.5244026343035,15.2,1.71659660661117));
#257124=CARTESIAN_POINT('Ctrl Pts',(-10.5279226954474,15.2,1.71812920202735));
#257125=CARTESIAN_POINT('Ctrl Pts',(-10.5314640274602,15.2,1.71968035091527));
#257126=CARTESIAN_POINT('Ctrl Pts',(-10.5357136257212,15.2,1.72154172951316));
#257127=CARTESIAN_POINT('Ctrl Pts',(-10.5399938549055,15.2,1.72342982533764));
#257128=CARTESIAN_POINT('Ctrl Pts',(-10.5443041412469,15.2,1.72534477701621));
#257129=CARTESIAN_POINT('Ctrl Pts',(-10.5478960466618,15.2,1.72694057013968));
#257130=CARTESIAN_POINT('Ctrl Pts',(-10.5515088274653,15.2,1.72855501449341));
#257131=CARTESIAN_POINT('Ctrl Pts',(-10.5551421577414,15.2,1.73018818831133));
#257132=CARTESIAN_POINT('Ctrl Pts',(-10.5587754880175,15.2,1.73182136212924));
#257133=CARTESIAN_POINT('Ctrl Pts',(-10.5624293680322,15.2,1.73347326436629));
#257134=CARTESIAN_POINT('Ctrl Pts',(-10.5661034767111,15.2,1.73514397248975));
#257135=CARTESIAN_POINT('Ctrl Pts',(-10.5712472289416,15.2,1.737482963899));
#257136=CARTESIAN_POINT('Ctrl Pts',(-10.5764306300097,15.2,1.73985881671164));
#257137=CARTESIAN_POINT('Ctrl Pts',(-10.581652812698,15.2,1.742271730274));
#257138=CARTESIAN_POINT('Ctrl Pts',(-10.5853829431315,15.2,1.74399523993456));
#257139=CARTESIAN_POINT('Ctrl Pts',(-10.5891328619333,15.2,1.74573765824437));
#257140=CARTESIAN_POINT('Ctrl Pts',(-10.5929022565167,15.2,1.74749905775826));
#257141=CARTESIAN_POINT('Ctrl Pts',(-10.5966716511,15.2,1.74926045727215));
#257142=CARTESIAN_POINT('Ctrl Pts',(-10.6004605235403,15.2,1.75104083661492));
#257143=CARTESIAN_POINT('Ctrl Pts',(-10.6042685642521,15.2,1.75284026544259));
#257144=CARTESIAN_POINT('Ctrl Pts',(-10.6073149965725,15.2,1.75427980838704));
#257145=CARTESIAN_POINT('Ctrl Pts',(-10.6103736992141,15.2,1.75573154406763));
#257146=CARTESIAN_POINT('Ctrl Pts',(-10.6134445152396,15.2,1.75719550500225));
#257147=CARTESIAN_POINT('Ctrl Pts',(-10.6172830355853,15.2,1.75902545632013));
#257148=CARTESIAN_POINT('Ctrl Pts',(-10.6211404832112,15.2,1.76087451139604));
#257149=CARTESIAN_POINT('Ctrl Pts',(-10.6250165594597,15.2,1.76274273521391));
#257150=CARTESIAN_POINT('Ctrl Pts',(-10.6281174206274,15.2,1.76423731434966));
#257151=CARTESIAN_POINT('Ctrl Pts',(-10.6312302028204,15.2,1.76574416327235));
#257152=CARTESIAN_POINT('Ctrl Pts',(-10.6343547567271,15.2,1.76726331125097));
#257153=CARTESIAN_POINT('Ctrl Pts',(-10.6374793102082,15.2,1.76878245902261));
#257154=CARTESIAN_POINT('Ctrl Pts',(-10.6406156344022,15.2,1.77031390885556));
#257155=CARTESIAN_POINT('Ctrl Pts',(-10.643763577977,15.2,1.77185769100587));
#257156=CARTESIAN_POINT('Ctrl Pts',(-10.6469115219807,15.2,1.77340147336651));
#257157=CARTESIAN_POINT('Ctrl Pts',(-10.6500710867133,15.2,1.77495758991445));
#257158=CARTESIAN_POINT('Ctrl Pts',(-10.653242123275,15.2,1.77652606899993));
#257159=CARTESIAN_POINT('Ctrl Pts',(-10.6579986776855,15.2,1.77887878741445));
#257160=CARTESIAN_POINT('Ctrl Pts',(-10.662781040646,15.2,1.78125932488582));
#257161=CARTESIAN_POINT('Ctrl Pts',(-10.6675887212933,15.2,1.78366778525035));
#257162=CARTESIAN_POINT('Ctrl Pts',(-10.6723964023774,15.2,1.78607624583364));
#257163=CARTESIAN_POINT('Ctrl Pts',(-10.6772293960964,15.2,1.78851262710733));
#257164=CARTESIAN_POINT('Ctrl Pts',(-10.6820872180295,15.2,1.79097702699357));
#257165=CARTESIAN_POINT('Ctrl Pts',(-10.6861354027532,15.2,1.7930306934535));
#257166=CARTESIAN_POINT('Ctrl Pts',(-10.6902008280438,15.2,1.79510381956652));
#257167=CARTESIAN_POINT('Ctrl Pts',(-10.6942832152673,15.2,1.79719645824866));
#257168=CARTESIAN_POINT('Ctrl Pts',(-10.6983656020459,15.2,1.7992890967027));
#257169=CARTESIAN_POINT('Ctrl Pts',(-10.7024649500561,15.2,1.80140124834397));
#257170=CARTESIAN_POINT('Ctrl Pts',(-10.7065809837033,15.2,1.80353296672111));
#257171=CARTESIAN_POINT('Ctrl Pts',(-10.7098738111594,15.2,1.80523834170165));
#257172=CARTESIAN_POINT('Ctrl Pts',(-10.7131773185027,15.2,1.80695623840007));
#257173=CARTESIAN_POINT('Ctrl Pts',(-10.7164913640167,15.2,1.8086866847166));
#257174=CARTESIAN_POINT('Ctrl Pts',(-10.7198054095306,15.2,1.81041713103312));
#257175=CARTESIAN_POINT('Ctrl Pts',(-10.7231299947236,15.2,1.81216012539557));
#257176=CARTESIAN_POINT('Ctrl Pts',(-10.7264649807953,15.2,1.81391569627031));
#257177=CARTESIAN_POINT('Ctrl Pts',(-10.7306337127033,15.2,1.81611015950494));
#257178=CARTESIAN_POINT('Ctrl Pts',(-10.7348186963209,15.2,1.81832426840286));
#257179=CARTESIAN_POINT('Ctrl Pts',(-10.7390196624589,15.2,1.82055807669943));
#257180=CARTESIAN_POINT('Ctrl Pts',(-10.7432206290548,15.2,1.82279188523947));
#257181=CARTESIAN_POINT('Ctrl Pts',(-10.7474375781921,15.2,1.825045390332));
#257182=CARTESIAN_POINT('Ctrl Pts',(-10.7516702479131,15.2,1.8273186406776));
#257183=CARTESIAN_POINT('Ctrl Pts',(-10.7550563838744,15.2,1.8291372410532));
#257184=CARTESIAN_POINT('Ctrl Pts',(-10.7584525786929,15.2,1.83096847838395));
#257185=CARTESIAN_POINT('Ctrl Pts',(-10.7618587007273,15.2,1.83281237599286));
#257186=CARTESIAN_POINT('Ctrl Pts',(-10.766967883315,15.2,1.83557822215499));
#257187=CARTESIAN_POINT('Ctrl Pts',(-10.7720993974574,15.2,1.83837255355835));
#257188=CARTESIAN_POINT('Ctrl Pts',(-10.7772527972692,15.2,1.84119544787121));
#257189=CARTESIAN_POINT('Ctrl Pts',(-10.7806883974559,15.2,1.84307737758405));
#257190=CARTESIAN_POINT('Ctrl Pts',(-10.7841337237158,15.2,1.84497200279841));
#257191=CARTESIAN_POINT('Ctrl Pts',(-10.7875886470159,15.2,1.84687934318098));
#257192=CARTESIAN_POINT('Ctrl Pts',(-10.7910435698452,15.2,1.84878668330368));
#257193=CARTESIAN_POINT('Ctrl Pts',(-10.7945080870906,15.2,1.85070674124876));
#257194=CARTESIAN_POINT('Ctrl Pts',(-10.7979820709793,15.2,1.85263953618621));
#257195=CARTESIAN_POINT('Ctrl Pts',(-10.8014560553414,15.2,1.85457233138701));
#257196=CARTESIAN_POINT('Ctrl Pts',(-10.8049395044086,15.2,1.85651786550815));
#257197=CARTESIAN_POINT('Ctrl Pts',(-10.808432290544,15.2,1.85847615839348));
#257198=CARTESIAN_POINT('Ctrl Pts',(-10.8119250762035,15.2,1.86043445101199));
#257199=CARTESIAN_POINT('Ctrl Pts',(-10.8154271986306,15.2,1.86240550101407));
#257200=CARTESIAN_POINT('Ctrl Pts',(-10.8189385296759,15.2,1.86438933168391));
#257201=CARTESIAN_POINT('Ctrl Pts',(-10.8224498611997,15.2,1.86637316262406));
#257202=CARTESIAN_POINT('Ctrl Pts',(-10.8259704011216,15.2,1.86836977281543));
#257203=CARTESIAN_POINT('Ctrl Pts',(-10.8295000232584,15.2,1.87037918175827));
#257204=CARTESIAN_POINT('Ctrl Pts',(-10.8339120506889,15.2,1.87289094279992));
#257205=CARTESIAN_POINT('Ctrl Pts',(-10.8383382672322,15.2,1.87542270172858));
#257206=CARTESIAN_POINT('Ctrl Pts',(-10.8427784297524,15.2,1.877974497018));
#257207=CARTESIAN_POINT('Ctrl Pts',(-10.8463305594782,15.2,1.88001593308265));
#257208=CARTESIAN_POINT('Ctrl Pts',(-10.8498916145452,15.2,1.88207019220727));
#257209=CARTESIAN_POINT('Ctrl Pts',(-10.8534614696414,15.2,1.88413729220364));
#257210=CARTESIAN_POINT('Ctrl Pts',(-10.8579237888763,15.2,1.88672116741033));
#257211=CARTESIAN_POINT('Ctrl Pts',(-10.862399858275,15.2,1.88932510699725));
#257212=CARTESIAN_POINT('Ctrl Pts',(-10.8668894375794,15.2,1.89194914644005));
#257213=CARTESIAN_POINT('Ctrl Pts',(-10.8722769330384,15.2,1.89509799394301));
#257214=CARTESIAN_POINT('Ctrl Pts',(-10.8776838814571,15.2,1.89827578490691));
#257215=CARTESIAN_POINT('Ctrl Pts',(-10.883109874025,15.2,1.90148257657689));
#257216=CARTESIAN_POINT('Ctrl Pts',(-10.8867272019107,15.2,1.90362043739893));
#257217=CARTESIAN_POINT('Ctrl Pts',(-10.8903529927368,15.2,1.90577118816479));
#257218=CARTESIAN_POINT('Ctrl Pts',(-10.8939871264947,15.2,1.90793484359818));
#257219=CARTESIAN_POINT('Ctrl Pts',(-10.8976212607477,15.2,1.91009849932637));
#257220=CARTESIAN_POINT('Ctrl Pts',(-10.9012637372574,15.2,1.91227506161165));
#257221=CARTESIAN_POINT('Ctrl Pts',(-10.9049144362902,15.2,1.91446454645405));
#257222=CARTESIAN_POINT('Ctrl Pts',(-10.9085651348257,15.2,1.91665403099813));
#257223=CARTESIAN_POINT('Ctrl Pts',(-10.912224056838,15.2,1.91885643574456));
#257224=CARTESIAN_POINT('Ctrl Pts',(-10.915891083443,15.2,1.92107177789521));
#257225=CARTESIAN_POINT('Ctrl Pts',(-10.9195581105475,15.2,1.9232871203477));
#257226=CARTESIAN_POINT('Ctrl Pts',(-10.9232332416694,15.2,1.92551540136861));
#257227=CARTESIAN_POINT('Ctrl Pts',(-10.9269163592595,15.2,1.92775663365828));
#257228=CARTESIAN_POINT('Ctrl Pts',(-10.9305994763479,15.2,1.92999786564257));
#257229=CARTESIAN_POINT('Ctrl Pts',(-10.9342905786707,15.2,1.93225205087703));
#257230=CARTESIAN_POINT('Ctrl Pts',(-10.9379895511452,15.2,1.93451920157926));
#257231=CARTESIAN_POINT('Ctrl Pts',(-10.9416885241238,15.2,1.93678635259038));
#257232=CARTESIAN_POINT('Ctrl Pts',(-10.9453953661055,15.2,1.93906647141052));
#257233=CARTESIAN_POINT('Ctrl Pts',(-10.9491099617692,15.2,1.94135956976817));
#257234=CARTESIAN_POINT('Ctrl Pts',(-10.9528245569269,15.2,1.94365266781338));
#257235=CARTESIAN_POINT('Ctrl Pts',(-10.956546906807,15.2,1.94595874678667));
#257236=CARTESIAN_POINT('Ctrl Pts',(-10.9602768933902,15.2,1.94827782009577));
#257237=CARTESIAN_POINT('Ctrl Pts',(-10.9658718740273,15.2,1.95175643053337));
#257238=CARTESIAN_POINT('Ctrl Pts',(-10.9714840399244,15.2,1.95526427792379));
#257239=CARTESIAN_POINT('Ctrl Pts',(-10.9771130083152,15.2,1.95880140620116));
#257240=CARTESIAN_POINT('Ctrl Pts',(-10.9808656533978,15.2,1.96115949139812));
#257241=CARTESIAN_POINT('Ctrl Pts',(-10.9846257646821,15.2,1.96353059018655));
#257242=CARTESIAN_POINT('Ctrl Pts',(-10.9883932307284,15.2,1.96591471488739));
#257243=CARTESIAN_POINT('Ctrl Pts',(-10.9921606972879,15.2,1.96829883991306));
#257244=CARTESIAN_POINT('Ctrl Pts',(-10.9959355180971,15.2,1.9706959892621));
#257245=CARTESIAN_POINT('Ctrl Pts',(-10.999717580526,15.2,1.97310617867209));
#257246=CARTESIAN_POINT('Ctrl Pts',(-11.0025541270899,15.2,1.97491382056539));
#257247=CARTESIAN_POINT('Ctrl Pts',(-11.0053947483034,15.2,1.97672879453281));
#257248=CARTESIAN_POINT('Ctrl Pts',(-11.0082393957834,15.2,1.9785511084666));
#257249=CARTESIAN_POINT('Ctrl Pts',(-11.0110840432633,15.2,1.98037342240038));
#257250=CARTESIAN_POINT('Ctrl Pts',(-11.0139327165098,15.2,1.98220307505055));
#257251=CARTESIAN_POINT('Ctrl Pts',(-11.0167853709475,15.2,1.98404007056649));
#257252=CARTESIAN_POINT('Ctrl Pts',(-11.0196380253851,15.2,1.98587706608243));
#257253=CARTESIAN_POINT('Ctrl Pts',(-11.0224946585581,15.2,1.98772140453404));
#257254=CARTESIAN_POINT('Ctrl Pts',(-11.0253552261799,15.2,1.98957309160008));
#257255=CARTESIAN_POINT('Ctrl Pts',(-11.0282157938018,15.2,1.99142477866612));
#257256=CARTESIAN_POINT('Ctrl Pts',(-11.0310802943128,15.2,1.99328381362856));
#257257=CARTESIAN_POINT('Ctrl Pts',(-11.0339486823747,15.2,1.99515020064307));
#257258=CARTESIAN_POINT('Ctrl Pts',(-11.0368170709577,15.2,1.99701658799663));
#257259=CARTESIAN_POINT('Ctrl Pts',(-11.0396893477418,15.2,1.9988903280523));
#257260=CARTESIAN_POINT('Ctrl Pts',(-11.0425654648687,15.2,2.00077142441002));
#257261=CARTESIAN_POINT('Ctrl Pts',(-11.045441581473,15.2,2.002652520426));
#257262=CARTESIAN_POINT('Ctrl Pts',(-11.0483215400355,15.2,2.0045409724916));
#257263=CARTESIAN_POINT('Ctrl Pts',(-11.0512052935978,15.2,2.00643678596503));
#257264=CARTESIAN_POINT('Ctrl Pts',(-11.05408904716,15.2,2.00833259943846));
#257265=CARTESIAN_POINT('Ctrl Pts',(-11.0569765959779,15.2,2.01023577351237));
#257266=CARTESIAN_POINT('Ctrl Pts',(-11.059867896011,15.2,2.01214631249334));
#257267=CARTESIAN_POINT('Ctrl Pts',(-11.0627591960441,15.2,2.01405685147431));
#257268=CARTESIAN_POINT('Ctrl Pts',(-11.0656542461062,15.2,2.01597475507609));
#257269=CARTESIAN_POINT('Ctrl Pts',(-11.0685530007224,15.2,2.01790002801486));
#257270=CARTESIAN_POINT('Ctrl Pts',(-11.0714517553386,15.2,2.01982530095362));
#257271=CARTESIAN_POINT('Ctrl Pts',(-11.0743542155726,15.2,2.02175794254306));
#257272=CARTESIAN_POINT('Ctrl Pts',(-11.077260334675,15.2,2.02369795609693));
#257273=CARTESIAN_POINT('Ctrl Pts',(-11.0801664537774,15.2,2.02563796965079));
#257274=CARTESIAN_POINT('Ctrl Pts',(-11.0830762328546,15.2,2.02758535579583));
#257275=CARTESIAN_POINT('Ctrl Pts',(-11.0859896278732,15.2,2.02954011826547));
#257276=CARTESIAN_POINT('Ctrl Pts',(-11.0889030234212,15.2,2.03149488109022));
#257277=CARTESIAN_POINT('Ctrl Pts',(-11.0918200337784,15.2,2.03345701942539));
#257278=CARTESIAN_POINT('Ctrl Pts',(-11.0947406148701,15.2,2.03542653821263));
#257279=CARTESIAN_POINT('Ctrl Pts',(-11.0976611954311,15.2,2.03739605664208));
#257280=CARTESIAN_POINT('Ctrl Pts',(-11.1005853472429,15.2,2.03937295500602));
#257281=CARTESIAN_POINT('Ctrl Pts',(-11.1035130258665,15.2,2.04135723565892));
#257282=CARTESIAN_POINT('Ctrl Pts',(-11.1083924904165,15.2,2.04466437020056));
#257283=CARTESIAN_POINT('Ctrl Pts',(-11.1132817476734,15.2,2.04799201313066));
#257284=CARTESIAN_POINT('Ctrl Pts',(-11.1181805989241,15.2,2.05134017993789));
#257285=CARTESIAN_POINT('Ctrl Pts',(-11.1211199095678,15.2,2.05334907994923));
#257286=CARTESIAN_POINT('Ctrl Pts',(-11.1240626736446,15.2,2.05536536966019));
#257287=CARTESIAN_POINT('Ctrl Pts',(-11.1270088467879,15.2,2.05738904875397));
#257288=CARTESIAN_POINT('Ctrl Pts',(-11.1299550199311,15.2,2.05941272784775));
#257289=CARTESIAN_POINT('Ctrl Pts',(-11.1329046029407,15.2,2.061443798524));
#257290=CARTESIAN_POINT('Ctrl Pts',(-11.135857552,15.2,2.0634822644916));
#257291=CARTESIAN_POINT('Ctrl Pts',(-11.1388105010594,15.2,2.06552073045919));
#257292=CARTESIAN_POINT('Ctrl Pts',(-11.141766815602,15.2,2.0675665902015));
#257293=CARTESIAN_POINT('Ctrl Pts',(-11.1447264536608,15.2,2.06961984720959));
#257294=CARTESIAN_POINT('Ctrl Pts',(-11.1476860917197,15.2,2.07167310421767));
#257295=CARTESIAN_POINT('Ctrl Pts',(-11.1506490527028,15.2,2.07373375897259));
#257296=CARTESIAN_POINT('Ctrl Pts',(-11.1536152939512,15.2,2.07580181308322));
#257297=CARTESIAN_POINT('Ctrl Pts',(-11.1565815351995,15.2,2.07786986719385));
#257298=CARTESIAN_POINT('Ctrl Pts',(-11.1595510567104,15.2,2.07994532147257));
#257299=CARTESIAN_POINT('Ctrl Pts',(-11.162523814852,15.2,2.08202817752088));
#257300=CARTESIAN_POINT('Ctrl Pts',(-11.1664874927341,15.2,2.08480531917088));
#257301=CARTESIAN_POINT('Ctrl Pts',(-11.1704569258,15.2,2.0875956213777));
#257302=CARTESIAN_POINT('Ctrl Pts',(-11.1744320130167,15.2,2.09039908947493));
#257303=CARTESIAN_POINT('Ctrl Pts',(-11.1784071002334,15.2,2.09320255757216));
#257304=CARTESIAN_POINT('Ctrl Pts',(-11.1823878411951,15.2,2.0960191907293));
#257305=CARTESIAN_POINT('Ctrl Pts',(-11.1863741376351,15.2,2.09884899499595));
#257306=CARTESIAN_POINT('Ctrl Pts',(-11.1893638596936,15.2,2.10097134800316));
#257307=CARTESIAN_POINT('Ctrl Pts',(-11.1923567062552,15.2,2.10310111003352));
#257308=CARTESIAN_POINT('Ctrl Pts',(-11.1953526345464,15.2,2.10523828264683));
#257309=CARTESIAN_POINT('Ctrl Pts',(-11.1983485628375,15.2,2.10737545526014));
#257310=CARTESIAN_POINT('Ctrl Pts',(-11.2013475734695,15.2,2.1095200384955));
#257311=CARTESIAN_POINT('Ctrl Pts',(-11.204349624069,15.2,2.11167203495962));
#257312=CARTESIAN_POINT('Ctrl Pts',(-11.2073516746685,15.2,2.11382403142374));
#257313=CARTESIAN_POINT('Ctrl Pts',(-11.2103567648593,15.2,2.11598344101199));
#257314=CARTESIAN_POINT('Ctrl Pts',(-11.213364855,15.2,2.11815026497493));
#257315=CARTESIAN_POINT('Ctrl Pts',(-11.2163729451407,15.2,2.12031708893787));
#257316=CARTESIAN_POINT('Ctrl Pts',(-11.219384036048,15.2,2.12249132754217));
#257317=CARTESIAN_POINT('Ctrl Pts',(-11.2223980842299,15.2,2.12467298300392));
#257318=CARTESIAN_POINT('Ctrl Pts',(-11.2254121324118,15.2,2.12685463846567));
#257319=CARTESIAN_POINT('Ctrl Pts',(-11.2284291390583,15.2,2.12904371126263));
#257320=CARTESIAN_POINT('Ctrl Pts',(-11.2314490603908,15.2,2.13124020183337));
#257321=CARTESIAN_POINT('Ctrl Pts',(-11.2344689817233,15.2,2.13343669240411));
#257322=CARTESIAN_POINT('Ctrl Pts',(-11.2374918181841,15.2,2.13564060099922));
#257323=CARTESIAN_POINT('Ctrl Pts',(-11.2405175293654,15.2,2.13785192904286));
#257324=CARTESIAN_POINT('Ctrl Pts',(-11.2435432410964,15.2,2.14006325748823));
#257325=CARTESIAN_POINT('Ctrl Pts',(-11.2465718276033,15.2,2.14228200709404));
#257326=CARTESIAN_POINT('Ctrl Pts',(-11.2496032518776,15.2,2.14450817746025));
#257327=CARTESIAN_POINT('Ctrl Pts',(-11.2526346756011,15.2,2.14673434742203));
#257328=CARTESIAN_POINT('Ctrl Pts',(-11.2556689386246,15.2,2.14896793802511));
#257329=CARTESIAN_POINT('Ctrl Pts',(-11.2587059980978,15.2,2.151208951486));
#257330=CARTESIAN_POINT('Ctrl Pts',(-11.261743057571,15.2,2.1534499649469));
#257331=CARTESIAN_POINT('Ctrl Pts',(-11.2647829118995,15.2,2.15569840179033));
#257332=CARTESIAN_POINT('Ctrl Pts',(-11.2678255119695,15.2,2.15795426226032));
#257333=CARTESIAN_POINT('Ctrl Pts',(-11.2718823118785,15.2,2.1609620760837));
#257334=CARTESIAN_POINT('Ctrl Pts',(-11.2759439882014,15.2,2.16398308913101));
#257335=CARTESIAN_POINT('Ctrl Pts',(-11.2800104648685,15.2,2.16701730343717));
#257336=CARTESIAN_POINT('Ctrl Pts',(-11.2840769420896,15.2,2.17005151815675));
#257337=CARTESIAN_POINT('Ctrl Pts',(-11.288148224556,15.2,2.17309893949932));
#257338=CARTESIAN_POINT('Ctrl Pts',(-11.2922242990001,15.2,2.17615954699999));
#257339=CARTESIAN_POINT('Ctrl Pts',(-10.0330625580001,15.2,2.64164356399998));
#257340=CARTESIAN_POINT('Ctrl Pts',(-10.0330625580001,11.6,2.64164356399998));
#257341=CARTESIAN_POINT('Ctrl Pts',(-10.0332343610001,15.2,2.64167330399999));
#257342=CARTESIAN_POINT('Ctrl Pts',(-10.0332343610001,11.6,2.64167330399999));
#257343=CARTESIAN_POINT('Ctrl Pts',(-10.0335839820001,15.2,2.64173373799999));
#257344=CARTESIAN_POINT('Ctrl Pts',(-10.0335839820001,11.6,2.64173373799998));
#257345=CARTESIAN_POINT('Ctrl Pts',(-10.0341137860001,15.2,2.64182504799999));
#257346=CARTESIAN_POINT('Ctrl Pts',(-10.0341137860001,11.6,2.64182504799999));
#257347=CARTESIAN_POINT('Ctrl Pts',(-10.0348275720001,15.2,2.64194751899999));
#257348=CARTESIAN_POINT('Ctrl Pts',(-10.0348275720001,11.6,2.64194751899998));
#257349=CARTESIAN_POINT('Ctrl Pts',(-10.0357305600001,15.2,2.64210152599999));
#257350=CARTESIAN_POINT('Ctrl Pts',(-10.0357305600001,11.6,2.64210152599999));
#257351=CARTESIAN_POINT('Ctrl Pts',(-10.0366483400001,15.2,2.64225710799998));
#257352=CARTESIAN_POINT('Ctrl Pts',(-10.0366483400001,11.6,2.64225710799998));
#257353=CARTESIAN_POINT('Ctrl Pts',(-10.0375756570001,15.2,2.64241334899998));
#257354=CARTESIAN_POINT('Ctrl Pts',(-10.0375756570001,11.6,2.64241334899998));
#257355=CARTESIAN_POINT('Ctrl Pts',(-10.0385124890001,15.2,2.64257022899999));
#257356=CARTESIAN_POINT('Ctrl Pts',(-10.0385124890001,11.6,2.64257022899999));
#257357=CARTESIAN_POINT('Ctrl Pts',(-10.0394588120001,15.2,2.64272772499999));
#257358=CARTESIAN_POINT('Ctrl Pts',(-10.0394588120001,11.6,2.64272772499999));
#257359=CARTESIAN_POINT('Ctrl Pts',(-10.0404146010001,15.2,2.64288581199998));
#257360=CARTESIAN_POINT('Ctrl Pts',(-10.0404146010001,11.6,2.64288581199998));
#257361=CARTESIAN_POINT('Ctrl Pts',(-10.0413798350001,15.2,2.64304447199999));
#257362=CARTESIAN_POINT('Ctrl Pts',(-10.0413798350001,11.6,2.64304447199999));
#257363=CARTESIAN_POINT('Ctrl Pts',(-10.0423544890001,15.2,2.64320368099998));
#257364=CARTESIAN_POINT('Ctrl Pts',(-10.0423544890001,11.6,2.64320368099998));
#257365=CARTESIAN_POINT('Ctrl Pts',(-10.0433385410001,15.2,2.64336341799999));
#257366=CARTESIAN_POINT('Ctrl Pts',(-10.0433385410001,11.6,2.64336341799999));
#257367=CARTESIAN_POINT('Ctrl Pts',(-10.0443319680001,15.2,2.64352366099998));
#257368=CARTESIAN_POINT('Ctrl Pts',(-10.0443319680001,11.6,2.64352366099998));
#257369=CARTESIAN_POINT('Ctrl Pts',(-10.0453347470001,15.2,2.64368438699999));
#257370=CARTESIAN_POINT('Ctrl Pts',(-10.0453347470001,11.6,2.64368438699999));
#257371=CARTESIAN_POINT('Ctrl Pts',(-10.0463468550001,15.2,2.64384557699999));
#257372=CARTESIAN_POINT('Ctrl Pts',(-10.0463468550001,11.6,2.64384557699999));
#257373=CARTESIAN_POINT('Ctrl Pts',(-10.0473682690001,15.2,2.64400720799999));
#257374=CARTESIAN_POINT('Ctrl Pts',(-10.0473682690001,11.6,2.64400720799999));
#257375=CARTESIAN_POINT('Ctrl Pts',(-10.0483989660001,15.2,2.64416925999999));
#257376=CARTESIAN_POINT('Ctrl Pts',(-10.0483989660001,11.6,2.64416925999999));
#257377=CARTESIAN_POINT('Ctrl Pts',(-10.0494389260001,15.2,2.64433171099999));
#257378=CARTESIAN_POINT('Ctrl Pts',(-10.0494389260001,11.6,2.64433171099998));
#257379=CARTESIAN_POINT('Ctrl Pts',(-10.0504881240001,15.2,2.64449453999998));
#257380=CARTESIAN_POINT('Ctrl Pts',(-10.0504881240001,11.6,2.64449453999998));
#257381=CARTESIAN_POINT('Ctrl Pts',(-10.0515465390001,15.2,2.64465772599999));
#257382=CARTESIAN_POINT('Ctrl Pts',(-10.0515465390001,11.6,2.64465772599999));
#257383=CARTESIAN_POINT('Ctrl Pts',(-10.0526141480001,15.2,2.64482124899998));
#257384=CARTESIAN_POINT('Ctrl Pts',(-10.0526141480001,11.6,2.64482124899998));
#257385=CARTESIAN_POINT('Ctrl Pts',(-10.0536909300001,15.2,2.64498508799999));
#257386=CARTESIAN_POINT('Ctrl Pts',(-10.0536909300001,11.6,2.64498508799999));
#257387=CARTESIAN_POINT('Ctrl Pts',(-10.0547768630001,15.2,2.64514922199999));
#257388=CARTESIAN_POINT('Ctrl Pts',(-10.0547768630001,11.6,2.64514922199999));
#257389=CARTESIAN_POINT('Ctrl Pts',(-10.0558719240001,15.2,2.64531363099999));
#257390=CARTESIAN_POINT('Ctrl Pts',(-10.0558719240001,11.6,2.64531363099999));
#257391=CARTESIAN_POINT('Ctrl Pts',(-10.0569760920001,15.2,2.64547829499998));
#257392=CARTESIAN_POINT('Ctrl Pts',(-10.0569760920001,11.6,2.64547829499998));
#257393=CARTESIAN_POINT('Ctrl Pts',(-10.0580893450001,15.2,2.64564319399998));
#257394=CARTESIAN_POINT('Ctrl Pts',(-10.0580893450001,11.6,2.64564319399998));
#257395=CARTESIAN_POINT('Ctrl Pts',(-10.0592116610001,15.2,2.64580830499998));
#257396=CARTESIAN_POINT('Ctrl Pts',(-10.0592116610001,11.6,2.64580830499998));
#257397=CARTESIAN_POINT('Ctrl Pts',(-10.0603430200001,15.2,2.64597361199999));
#257398=CARTESIAN_POINT('Ctrl Pts',(-10.0603430200001,11.6,2.64597361199999));
#257399=CARTESIAN_POINT('Ctrl Pts',(-10.0614833980001,15.2,2.64613909299998));
#257400=CARTESIAN_POINT('Ctrl Pts',(-10.0614833980001,11.6,2.64613909299998));
#257401=CARTESIAN_POINT('Ctrl Pts',(-10.0626327760001,15.2,2.64630472799999));
#257402=CARTESIAN_POINT('Ctrl Pts',(-10.0626327760001,11.6,2.64630472799999));
#257403=CARTESIAN_POINT('Ctrl Pts',(-10.0637911310001,15.2,2.64647049799999));
#257404=CARTESIAN_POINT('Ctrl Pts',(-10.0637911310001,11.6,2.64647049799999));
#257405=CARTESIAN_POINT('Ctrl Pts',(-10.0649584440001,15.2,2.64663638399998));
#257406=CARTESIAN_POINT('Ctrl Pts',(-10.0649584440001,11.6,2.64663638399998));
#257407=CARTESIAN_POINT('Ctrl Pts',(-10.0661346930001,15.2,2.64680236399998));
#257408=CARTESIAN_POINT('Ctrl Pts',(-10.0661346930001,11.6,2.64680236399998));
#257409=CARTESIAN_POINT('Ctrl Pts',(-10.0673198560001,15.2,2.64696842199999));
#257410=CARTESIAN_POINT('Ctrl Pts',(-10.0673198560001,11.6,2.64696842199999));
#257411=CARTESIAN_POINT('Ctrl Pts',(-10.0685139130001,15.2,2.64713453499999));
#257412=CARTESIAN_POINT('Ctrl Pts',(-10.0685139130001,11.6,2.64713453499999));
#257413=CARTESIAN_POINT('Ctrl Pts',(-10.0697168420001,15.2,2.64730068599999));
#257414=CARTESIAN_POINT('Ctrl Pts',(-10.0697168420001,11.6,2.64730068599999));
#257415=CARTESIAN_POINT('Ctrl Pts',(-10.0709286240001,15.2,2.64746685699999));
#257416=CARTESIAN_POINT('Ctrl Pts',(-10.0709286240001,11.6,2.64746685699999));
#257417=CARTESIAN_POINT('Ctrl Pts',(-10.0721492380001,15.2,2.64763302599999));
#257418=CARTESIAN_POINT('Ctrl Pts',(-10.0721492380001,11.6,2.64763302599999));
#257419=CARTESIAN_POINT('Ctrl Pts',(-10.0733786630001,15.2,2.64779917599999));
#257420=CARTESIAN_POINT('Ctrl Pts',(-10.0733786630001,11.6,2.64779917599998));
#257421=CARTESIAN_POINT('Ctrl Pts',(-10.0746168780001,15.2,2.64796528799998));
#257422=CARTESIAN_POINT('Ctrl Pts',(-10.0746168780001,11.6,2.64796528799998));
#257423=CARTESIAN_POINT('Ctrl Pts',(-10.0758638630001,15.2,2.64813134199999));
#257424=CARTESIAN_POINT('Ctrl Pts',(-10.0758638630001,11.6,2.64813134199999));
#257425=CARTESIAN_POINT('Ctrl Pts',(-10.0771195980001,15.2,2.64829732099999));
#257426=CARTESIAN_POINT('Ctrl Pts',(-10.0771195980001,11.6,2.64829732099999));
#257427=CARTESIAN_POINT('Ctrl Pts',(-10.0783840630001,15.2,2.64846320699998));
#257428=CARTESIAN_POINT('Ctrl Pts',(-10.0783840630001,11.6,2.64846320699998));
#257429=CARTESIAN_POINT('Ctrl Pts',(-10.0796572370001,15.2,2.64862897899998));
#257430=CARTESIAN_POINT('Ctrl Pts',(-10.0796572370001,11.6,2.64862897899998));
#257431=CARTESIAN_POINT('Ctrl Pts',(-10.0809391000001,15.2,2.64879461899999));
#257432=CARTESIAN_POINT('Ctrl Pts',(-10.0809391000001,11.6,2.64879461899999));
#257433=CARTESIAN_POINT('Ctrl Pts',(-10.0822296340001,15.2,2.64896011099999));
#257434=CARTESIAN_POINT('Ctrl Pts',(-10.0822296340001,11.6,2.64896011099999));
#257435=CARTESIAN_POINT('Ctrl Pts',(-10.0835288160001,15.2,2.64912543499998));
#257436=CARTESIAN_POINT('Ctrl Pts',(-10.0835288160001,11.6,2.64912543499998));
#257437=CARTESIAN_POINT('Ctrl Pts',(-10.0848366280001,15.2,2.64929057399999));
#257438=CARTESIAN_POINT('Ctrl Pts',(-10.0848366280001,11.6,2.64929057399998));
#257439=CARTESIAN_POINT('Ctrl Pts',(-10.0861530500001,15.2,2.64945550899998));
#257440=CARTESIAN_POINT('Ctrl Pts',(-10.0861530500001,11.6,2.64945550899998));
#257441=CARTESIAN_POINT('Ctrl Pts',(-10.0874780620001,15.2,2.64962022099999));
#257442=CARTESIAN_POINT('Ctrl Pts',(-10.0874780620001,11.6,2.64962022099999));
#257443=CARTESIAN_POINT('Ctrl Pts',(-10.0888116440001,15.2,2.64978469499999));
#257444=CARTESIAN_POINT('Ctrl Pts',(-10.0888116440001,11.6,2.64978469499999));
#257445=CARTESIAN_POINT('Ctrl Pts',(-10.0901537780001,15.2,2.64994891199999));
#257446=CARTESIAN_POINT('Ctrl Pts',(-10.0901537780001,11.6,2.64994891199999));
#257447=CARTESIAN_POINT('Ctrl Pts',(-10.0915044430001,15.2,2.65011285399999));
#257448=CARTESIAN_POINT('Ctrl Pts',(-10.0915044430001,11.6,2.65011285399999));
#257449=CARTESIAN_POINT('Ctrl Pts',(-10.0928636200001,15.2,2.65027650399999));
#257450=CARTESIAN_POINT('Ctrl Pts',(-10.0928636200001,11.6,2.65027650399999));
#257451=CARTESIAN_POINT('Ctrl Pts',(-10.0942312910001,15.2,2.65043984299999));
#257452=CARTESIAN_POINT('Ctrl Pts',(-10.0942312910001,11.6,2.65043984299999));
#257453=CARTESIAN_POINT('Ctrl Pts',(-10.0956074340001,15.2,2.65060285499998));
#257454=CARTESIAN_POINT('Ctrl Pts',(-10.0956074340001,11.6,2.65060285499998));
#257455=CARTESIAN_POINT('Ctrl Pts',(-10.0969920330001,15.2,2.65076552299998));
#257456=CARTESIAN_POINT('Ctrl Pts',(-10.0969920330001,11.6,2.65076552299998));
#257457=CARTESIAN_POINT('Ctrl Pts',(-10.0983850660001,15.2,2.65092782899998));
#257458=CARTESIAN_POINT('Ctrl Pts',(-10.0983850660001,11.6,2.65092782899998));
#257459=CARTESIAN_POINT('Ctrl Pts',(-10.0997865150001,15.2,2.65108975499999));
#257460=CARTESIAN_POINT('Ctrl Pts',(-10.0997865150001,11.6,2.65108975499999));
#257461=CARTESIAN_POINT('Ctrl Pts',(-10.1011963620001,15.2,2.65125128599998));
#257462=CARTESIAN_POINT('Ctrl Pts',(-10.1011963620001,11.6,2.65125128599998));
#257463=CARTESIAN_POINT('Ctrl Pts',(-10.1026145880001,15.2,2.65141240299998));
#257464=CARTESIAN_POINT('Ctrl Pts',(-10.1026145880001,11.6,2.65141240299998));
#257465=CARTESIAN_POINT('Ctrl Pts',(-10.1040411730001,15.2,2.65157308999999));
#257466=CARTESIAN_POINT('Ctrl Pts',(-10.1040411730001,11.6,2.65157308999999));
#257467=CARTESIAN_POINT('Ctrl Pts',(-10.1054760990001,15.2,2.65173333099998));
#257468=CARTESIAN_POINT('Ctrl Pts',(-10.1054760990001,11.6,2.65173333099998));
#257469=CARTESIAN_POINT('Ctrl Pts',(-10.1069193480001,15.2,2.65189310799999));
#257470=CARTESIAN_POINT('Ctrl Pts',(-10.1069193480001,11.6,2.65189310799998));
#257471=CARTESIAN_POINT('Ctrl Pts',(-10.1083709000001,15.2,2.65205240499998));
#257472=CARTESIAN_POINT('Ctrl Pts',(-10.1083709000001,11.6,2.65205240499998));
#257473=CARTESIAN_POINT('Ctrl Pts',(-10.1098307370001,15.2,2.65221120399998));
#257474=CARTESIAN_POINT('Ctrl Pts',(-10.1098307370001,11.6,2.65221120399998));
#257475=CARTESIAN_POINT('Ctrl Pts',(-10.1112988410001,15.2,2.65236948899998));
#257476=CARTESIAN_POINT('Ctrl Pts',(-10.1112988410001,11.6,2.65236948899998));
#257477=CARTESIAN_POINT('Ctrl Pts',(-10.1127751920001,15.2,2.65252724599998));
#257478=CARTESIAN_POINT('Ctrl Pts',(-10.1127751920001,11.6,2.65252724599998));
#257479=CARTESIAN_POINT('Ctrl Pts',(-10.1142597750001,15.2,2.65268445599999));
#257480=CARTESIAN_POINT('Ctrl Pts',(-10.1142597750001,11.6,2.65268445599998));
#257481=CARTESIAN_POINT('Ctrl Pts',(-10.1157525680001,15.2,2.65284110399998));
#257482=CARTESIAN_POINT('Ctrl Pts',(-10.1157525680001,11.6,2.65284110399998));
#257483=CARTESIAN_POINT('Ctrl Pts',(-10.1172535550001,15.2,2.65299717299998));
#257484=CARTESIAN_POINT('Ctrl Pts',(-10.1172535550001,11.6,2.65299717299998));
#257485=CARTESIAN_POINT('Ctrl Pts',(-10.1187627170001,15.2,2.65315264699999));
#257486=CARTESIAN_POINT('Ctrl Pts',(-10.1187627170001,11.6,2.65315264699999));
#257487=CARTESIAN_POINT('Ctrl Pts',(-10.1202800360001,15.2,2.65330750999999));
#257488=CARTESIAN_POINT('Ctrl Pts',(-10.1202800360001,11.6,2.65330750999999));
#257489=CARTESIAN_POINT('Ctrl Pts',(-10.1218054950001,15.2,2.65346174599999));
#257490=CARTESIAN_POINT('Ctrl Pts',(-10.1218054950001,11.6,2.65346174599998));
#257491=CARTESIAN_POINT('Ctrl Pts',(-10.1233390740001,15.2,2.65361533999998));
#257492=CARTESIAN_POINT('Ctrl Pts',(-10.1233390740001,11.6,2.65361533999998));
#257493=CARTESIAN_POINT('Ctrl Pts',(-10.1248807580001,15.2,2.65376827399999));
#257494=CARTESIAN_POINT('Ctrl Pts',(-10.1248807580001,11.6,2.65376827399999));
#257495=CARTESIAN_POINT('Ctrl Pts',(-10.1264305260001,15.2,2.65392053499999));
#257496=CARTESIAN_POINT('Ctrl Pts',(-10.1264305260001,11.6,2.65392053499998));
#257497=CARTESIAN_POINT('Ctrl Pts',(-10.1279883630001,15.2,2.65407210499998));
#257498=CARTESIAN_POINT('Ctrl Pts',(-10.1279883630001,11.6,2.65407210499998));
#257499=CARTESIAN_POINT('Ctrl Pts',(-10.1295542490001,15.2,2.65422296899998));
#257500=CARTESIAN_POINT('Ctrl Pts',(-10.1295542490001,11.6,2.65422296899998));
#257501=CARTESIAN_POINT('Ctrl Pts',(-10.1311281680001,15.2,2.65437311199998));
#257502=CARTESIAN_POINT('Ctrl Pts',(-10.1311281680001,11.6,2.65437311199998));
#257503=CARTESIAN_POINT('Ctrl Pts',(-10.1327101010001,15.2,2.65452251899998));
#257504=CARTESIAN_POINT('Ctrl Pts',(-10.1327101010001,11.6,2.65452251899998));
#257505=CARTESIAN_POINT('Ctrl Pts',(-10.1343000320001,15.2,2.65467117299998));
#257506=CARTESIAN_POINT('Ctrl Pts',(-10.1343000320001,11.6,2.65467117299998));
#257507=CARTESIAN_POINT('Ctrl Pts',(-10.1358979420001,15.2,2.65481905899998));
#257508=CARTESIAN_POINT('Ctrl Pts',(-10.1358979420001,11.6,2.65481905899998));
#257509=CARTESIAN_POINT('Ctrl Pts',(-10.1375038160001,15.2,2.65496616399999));
#257510=CARTESIAN_POINT('Ctrl Pts',(-10.1375038160001,11.6,2.65496616399999));
#257511=CARTESIAN_POINT('Ctrl Pts',(-10.1391176340001,15.2,2.65511246899998));
#257512=CARTESIAN_POINT('Ctrl Pts',(-10.1391176340001,11.6,2.65511246899998));
#257513=CARTESIAN_POINT('Ctrl Pts',(-10.1407393800001,15.2,2.65525796199999));
#257514=CARTESIAN_POINT('Ctrl Pts',(-10.1407393800001,11.6,2.65525796199999));
#257515=CARTESIAN_POINT('Ctrl Pts',(-10.1423690360001,15.2,2.65540262599998));
#257516=CARTESIAN_POINT('Ctrl Pts',(-10.1423690360001,11.6,2.65540262599998));
#257517=CARTESIAN_POINT('Ctrl Pts',(-10.1440065870001,15.2,2.65554644699999));
#257518=CARTESIAN_POINT('Ctrl Pts',(-10.1440065870001,11.6,2.65554644699999));
#257519=CARTESIAN_POINT('Ctrl Pts',(-10.1456520130001,15.2,2.65568941099998));
#257520=CARTESIAN_POINT('Ctrl Pts',(-10.1456520130001,11.6,2.65568941099998));
#257521=CARTESIAN_POINT('Ctrl Pts',(-10.1473052990001,15.2,2.65583150099998));
#257522=CARTESIAN_POINT('Ctrl Pts',(-10.1473052990001,11.6,2.65583150099998));
#257523=CARTESIAN_POINT('Ctrl Pts',(-10.1489664270001,15.2,2.65597270399999));
#257524=CARTESIAN_POINT('Ctrl Pts',(-10.1489664270001,11.6,2.65597270399999));
#257525=CARTESIAN_POINT('Ctrl Pts',(-10.1506353810001,15.2,2.65611300399998));
#257526=CARTESIAN_POINT('Ctrl Pts',(-10.1506353810001,11.6,2.65611300399998));
#257527=CARTESIAN_POINT('Ctrl Pts',(-10.1523121420001,15.2,2.65625238599998));
#257528=CARTESIAN_POINT('Ctrl Pts',(-10.1523121420001,11.6,2.65625238599998));
#257529=CARTESIAN_POINT('Ctrl Pts',(-10.1539966950001,15.2,2.65639083799999));
#257530=CARTESIAN_POINT('Ctrl Pts',(-10.1539966950001,11.6,2.65639083799999));
#257531=CARTESIAN_POINT('Ctrl Pts',(-10.1556890250001,15.2,2.65652834299999));
#257532=CARTESIAN_POINT('Ctrl Pts',(-10.1556890250001,11.6,2.65652834299999));
#257533=CARTESIAN_POINT('Ctrl Pts',(-10.1573891100001,15.2,2.65666488699999));
#257534=CARTESIAN_POINT('Ctrl Pts',(-10.1573891100001,11.6,2.65666488699999));
#257535=CARTESIAN_POINT('Ctrl Pts',(-10.1590969390001,15.2,2.65680045599999));
#257536=CARTESIAN_POINT('Ctrl Pts',(-10.1590969390001,11.6,2.65680045599999));
#257537=CARTESIAN_POINT('Ctrl Pts',(-10.1608124920001,15.2,2.65693503499998));
#257538=CARTESIAN_POINT('Ctrl Pts',(-10.1608124920001,11.6,2.65693503499998));
#257539=CARTESIAN_POINT('Ctrl Pts',(-10.1625357530001,15.2,2.65706861099999));
#257540=CARTESIAN_POINT('Ctrl Pts',(-10.1625357530001,11.6,2.65706861099999));
#257541=CARTESIAN_POINT('Ctrl Pts',(-10.1642667060001,15.2,2.65720116799999));
#257542=CARTESIAN_POINT('Ctrl Pts',(-10.1642667060001,11.6,2.65720116799999));
#257543=CARTESIAN_POINT('Ctrl Pts',(-10.1660053350001,15.2,2.65733269399998));
#257544=CARTESIAN_POINT('Ctrl Pts',(-10.1660053350001,11.6,2.65733269399998));
#257545=CARTESIAN_POINT('Ctrl Pts',(-10.1677516220001,15.2,2.65746317399999));
#257546=CARTESIAN_POINT('Ctrl Pts',(-10.1677516220001,11.6,2.65746317399999));
#257547=CARTESIAN_POINT('Ctrl Pts',(-10.1695055520001,15.2,2.65759259199999));
#257548=CARTESIAN_POINT('Ctrl Pts',(-10.1695055520001,11.6,2.65759259199999));
#257549=CARTESIAN_POINT('Ctrl Pts',(-10.1712671090001,15.2,2.65772093799999));
#257550=CARTESIAN_POINT('Ctrl Pts',(-10.1712671090001,11.6,2.65772093799999));
#257551=CARTESIAN_POINT('Ctrl Pts',(-10.1730362760001,15.2,2.65784819299999));
#257552=CARTESIAN_POINT('Ctrl Pts',(-10.1730362760001,11.6,2.65784819299998));
#257553=CARTESIAN_POINT('Ctrl Pts',(-10.1748130360001,15.2,2.65797434899999));
#257554=CARTESIAN_POINT('Ctrl Pts',(-10.1748130360001,11.6,2.65797434899999));
#257555=CARTESIAN_POINT('Ctrl Pts',(-10.1765973750001,15.2,2.65809938799999));
#257556=CARTESIAN_POINT('Ctrl Pts',(-10.1765973750001,11.6,2.65809938799999));
#257557=CARTESIAN_POINT('Ctrl Pts',(-10.1783892740001,15.2,2.65822329699999));
#257558=CARTESIAN_POINT('Ctrl Pts',(-10.1783892740001,11.6,2.65822329699999));
#257559=CARTESIAN_POINT('Ctrl Pts',(-10.1801887200001,15.2,2.65834606199999));
#257560=CARTESIAN_POINT('Ctrl Pts',(-10.1801887200001,11.6,2.65834606199999));
#257561=CARTESIAN_POINT('Ctrl Pts',(-10.1819956950001,15.2,2.65846767299998));
#257562=CARTESIAN_POINT('Ctrl Pts',(-10.1819956950001,11.6,2.65846767299998));
#257563=CARTESIAN_POINT('Ctrl Pts',(-10.1838101840001,15.2,2.65858811199998));
#257564=CARTESIAN_POINT('Ctrl Pts',(-10.1838101840001,11.6,2.65858811199998));
#257565=CARTESIAN_POINT('Ctrl Pts',(-10.1856321710001,15.2,2.65870736699998));
#257566=CARTESIAN_POINT('Ctrl Pts',(-10.1856321710001,11.6,2.65870736699998));
#257567=CARTESIAN_POINT('Ctrl Pts',(-10.1874616400001,15.2,2.65882542499998));
#257568=CARTESIAN_POINT('Ctrl Pts',(-10.1874616400001,11.6,2.65882542499998));
#257569=CARTESIAN_POINT('Ctrl Pts',(-10.1892985750001,15.2,2.65894227199999));
#257570=CARTESIAN_POINT('Ctrl Pts',(-10.1892985750001,11.6,2.65894227199999));
#257571=CARTESIAN_POINT('Ctrl Pts',(-10.1911429610001,15.2,2.65905789599999));
#257572=CARTESIAN_POINT('Ctrl Pts',(-10.1911429610001,11.6,2.65905789599999));
#257573=CARTESIAN_POINT('Ctrl Pts',(-10.1929947820001,15.2,2.65917228199999));
#257574=CARTESIAN_POINT('Ctrl Pts',(-10.1929947820001,11.6,2.65917228199999));
#257575=CARTESIAN_POINT('Ctrl Pts',(-10.1948540200001,15.2,2.65928541799998));
#257576=CARTESIAN_POINT('Ctrl Pts',(-10.1948540200001,11.6,2.65928541799998));
#257577=CARTESIAN_POINT('Ctrl Pts',(-10.1967206650001,15.2,2.65939729099999));
#257578=CARTESIAN_POINT('Ctrl Pts',(-10.1967206650001,11.6,2.65939729099998));
#257579=CARTESIAN_POINT('Ctrl Pts',(-10.1985946950001,15.2,2.65950788699998));
#257580=CARTESIAN_POINT('Ctrl Pts',(-10.1985946950001,11.6,2.65950788699998));
#257581=CARTESIAN_POINT('Ctrl Pts',(-10.2004760990001,15.2,2.65961719299998));
#257582=CARTESIAN_POINT('Ctrl Pts',(-10.2004760990001,11.6,2.65961719299998));
#257583=CARTESIAN_POINT('Ctrl Pts',(-10.2023648590001,15.2,2.65972519599998));
#257584=CARTESIAN_POINT('Ctrl Pts',(-10.2023648590001,11.6,2.65972519599998));
#257585=CARTESIAN_POINT('Ctrl Pts',(-10.2042609620001,15.2,2.65983188399999));
#257586=CARTESIAN_POINT('Ctrl Pts',(-10.2042609620001,11.6,2.65983188399999));
#257587=CARTESIAN_POINT('Ctrl Pts',(-10.2061643900001,15.2,2.65993724299998));
#257588=CARTESIAN_POINT('Ctrl Pts',(-10.2061643900001,11.6,2.65993724299998));
#257589=CARTESIAN_POINT('Ctrl Pts',(-10.2080751300001,15.2,2.66004126199999));
#257590=CARTESIAN_POINT('Ctrl Pts',(-10.2080751300001,11.6,2.66004126199999));
#257591=CARTESIAN_POINT('Ctrl Pts',(-10.2099931640001,15.2,2.66014392599998));
#257592=CARTESIAN_POINT('Ctrl Pts',(-10.2099931640001,11.6,2.66014392599998));
#257593=CARTESIAN_POINT('Ctrl Pts',(-10.2119184800001,15.2,2.66024522299999));
#257594=CARTESIAN_POINT('Ctrl Pts',(-10.2119184800001,11.6,2.66024522299999));
#257595=CARTESIAN_POINT('Ctrl Pts',(-10.2138510600001,15.2,2.66034513999998));
#257596=CARTESIAN_POINT('Ctrl Pts',(-10.2138510600001,11.6,2.66034513999998));
#257597=CARTESIAN_POINT('Ctrl Pts',(-10.2157908920001,15.2,2.66044366699998));
#257598=CARTESIAN_POINT('Ctrl Pts',(-10.2157908920001,11.6,2.66044366699998));
#257599=CARTESIAN_POINT('Ctrl Pts',(-10.2177379570001,15.2,2.66054078699998));
#257600=CARTESIAN_POINT('Ctrl Pts',(-10.2177379570001,11.6,2.66054078699998));
#257601=CARTESIAN_POINT('Ctrl Pts',(-10.2196922430001,15.2,2.66063649199998));
#257602=CARTESIAN_POINT('Ctrl Pts',(-10.2196922430001,11.6,2.66063649199998));
#257603=CARTESIAN_POINT('Ctrl Pts',(-10.2216537340001,15.2,2.66073076599999));
#257604=CARTESIAN_POINT('Ctrl Pts',(-10.2216537340001,11.6,2.66073076599999));
#257605=CARTESIAN_POINT('Ctrl Pts',(-10.2236224150001,15.2,2.66082359899999));
#257606=CARTESIAN_POINT('Ctrl Pts',(-10.2236224150001,11.6,2.66082359899999));
#257607=CARTESIAN_POINT('Ctrl Pts',(-10.2255982700001,15.2,2.66091497699998));
#257608=CARTESIAN_POINT('Ctrl Pts',(-10.2255982700001,11.6,2.66091497699998));
#257609=CARTESIAN_POINT('Ctrl Pts',(-10.2275812850001,15.2,2.66100488799999));
#257610=CARTESIAN_POINT('Ctrl Pts',(-10.2275812850001,11.6,2.66100488799999));
#257611=CARTESIAN_POINT('Ctrl Pts',(-10.2295714460001,15.2,2.66109332199999));
#257612=CARTESIAN_POINT('Ctrl Pts',(-10.2295714460001,11.6,2.66109332199999));
#257613=CARTESIAN_POINT('Ctrl Pts',(-10.2315687380001,15.2,2.66118026399998));
#257614=CARTESIAN_POINT('Ctrl Pts',(-10.2315687380001,11.6,2.66118026399998));
#257615=CARTESIAN_POINT('Ctrl Pts',(-10.2335731450001,15.2,2.66126570199999));
#257616=CARTESIAN_POINT('Ctrl Pts',(-10.2335731450001,11.6,2.66126570199999));
#257617=CARTESIAN_POINT('Ctrl Pts',(-10.2355846530001,15.2,2.66134962599998));
#257618=CARTESIAN_POINT('Ctrl Pts',(-10.2355846530001,11.6,2.66134962599998));
#257619=CARTESIAN_POINT('Ctrl Pts',(-10.2376032480001,15.2,2.66143202199999));
#257620=CARTESIAN_POINT('Ctrl Pts',(-10.2376032480001,11.6,2.66143202199998));
#257621=CARTESIAN_POINT('Ctrl Pts',(-10.2396289140001,15.2,2.66151287899999));
#257622=CARTESIAN_POINT('Ctrl Pts',(-10.2396289140001,11.6,2.66151287899999));
#257623=CARTESIAN_POINT('Ctrl Pts',(-10.2416616380001,15.2,2.66159218399999));
#257624=CARTESIAN_POINT('Ctrl Pts',(-10.2416616380001,11.6,2.66159218399999));
#257625=CARTESIAN_POINT('Ctrl Pts',(-10.2437014030001,15.2,2.66166992699999));
#257626=CARTESIAN_POINT('Ctrl Pts',(-10.2437014030001,11.6,2.66166992699999));
#257627=CARTESIAN_POINT('Ctrl Pts',(-10.2457481980001,15.2,2.66174609399998));
#257628=CARTESIAN_POINT('Ctrl Pts',(-10.2457481980001,11.6,2.66174609399998));
#257629=CARTESIAN_POINT('Ctrl Pts',(-10.2478020060001,15.2,2.66182067599999));
#257630=CARTESIAN_POINT('Ctrl Pts',(-10.2478020060001,11.6,2.66182067599999));
#257631=CARTESIAN_POINT('Ctrl Pts',(-10.2498628120001,15.2,2.66189365799999));
#257632=CARTESIAN_POINT('Ctrl Pts',(-10.2498628120001,11.6,2.66189365799998));
#257633=CARTESIAN_POINT('Ctrl Pts',(-10.2519306040001,15.2,2.66196502999998));
#257634=CARTESIAN_POINT('Ctrl Pts',(-10.2519306040001,11.6,2.66196502999998));
#257635=CARTESIAN_POINT('Ctrl Pts',(-10.2540053660001,15.2,2.66203477999999));
#257636=CARTESIAN_POINT('Ctrl Pts',(-10.2540053660001,11.6,2.66203477999999));
#257637=CARTESIAN_POINT('Ctrl Pts',(-10.2560870840001,15.2,2.66210289699998));
#257638=CARTESIAN_POINT('Ctrl Pts',(-10.2560870840001,11.6,2.66210289699998));
#257639=CARTESIAN_POINT('Ctrl Pts',(-10.2581757450001,15.2,2.66216936899998));
#257640=CARTESIAN_POINT('Ctrl Pts',(-10.2581757450001,11.6,2.66216936899998));
#257641=CARTESIAN_POINT('Ctrl Pts',(-10.2602713320001,15.2,2.66223418299998));
#257642=CARTESIAN_POINT('Ctrl Pts',(-10.2602713320001,11.6,2.66223418299998));
#257643=CARTESIAN_POINT('Ctrl Pts',(-10.2623738330001,15.2,2.66229732999999));
#257644=CARTESIAN_POINT('Ctrl Pts',(-10.2623738330001,11.6,2.66229732999999));
#257645=CARTESIAN_POINT('Ctrl Pts',(-10.2644832330001,15.2,2.66235879699998));
#257646=CARTESIAN_POINT('Ctrl Pts',(-10.2644832330001,11.6,2.66235879699998));
#257647=CARTESIAN_POINT('Ctrl Pts',(-10.2665995190001,15.2,2.66241857399999));
#257648=CARTESIAN_POINT('Ctrl Pts',(-10.2665995190001,11.6,2.66241857399999));
#257649=CARTESIAN_POINT('Ctrl Pts',(-10.2687226760001,15.2,2.66247664899999));
#257650=CARTESIAN_POINT('Ctrl Pts',(-10.2687226760001,11.6,2.66247664899998));
#257651=CARTESIAN_POINT('Ctrl Pts',(-10.2708526900001,15.2,2.66253300899999));
#257652=CARTESIAN_POINT('Ctrl Pts',(-10.2708526900001,11.6,2.66253300899999));
#257653=CARTESIAN_POINT('Ctrl Pts',(-10.2729895460001,15.2,2.66258764499998));
#257654=CARTESIAN_POINT('Ctrl Pts',(-10.2729895460001,11.6,2.66258764499998));
#257655=CARTESIAN_POINT('Ctrl Pts',(-10.2751332320001,15.2,2.66264054599999));
#257656=CARTESIAN_POINT('Ctrl Pts',(-10.2751332320001,11.6,2.66264054599999));
#257657=CARTESIAN_POINT('Ctrl Pts',(-10.2772837330001,15.2,2.66269169899999));
#257658=CARTESIAN_POINT('Ctrl Pts',(-10.2772837330001,11.6,2.66269169899999));
#257659=CARTESIAN_POINT('Ctrl Pts',(-10.2794410340001,15.2,2.66274109399999));
#257660=CARTESIAN_POINT('Ctrl Pts',(-10.2794410340001,11.6,2.66274109399998));
#257661=CARTESIAN_POINT('Ctrl Pts',(-10.2816051240001,15.2,2.66278871999998));
#257662=CARTESIAN_POINT('Ctrl Pts',(-10.2816051240001,11.6,2.66278871999998));
#257663=CARTESIAN_POINT('Ctrl Pts',(-10.2837759870001,15.2,2.66283456499998));
#257664=CARTESIAN_POINT('Ctrl Pts',(-10.2837759870001,11.6,2.66283456499998));
#257665=CARTESIAN_POINT('Ctrl Pts',(-10.2859536100001,15.2,2.66287861899999));
#257666=CARTESIAN_POINT('Ctrl Pts',(-10.2859536100001,11.6,2.66287861899999));
#257667=CARTESIAN_POINT('Ctrl Pts',(-10.2881379790001,15.2,2.66292087099998));
#257668=CARTESIAN_POINT('Ctrl Pts',(-10.2881379790001,11.6,2.66292087099998));
#257669=CARTESIAN_POINT('Ctrl Pts',(-10.2903290790001,15.2,2.66296131099999));
#257670=CARTESIAN_POINT('Ctrl Pts',(-10.2903290790001,11.6,2.66296131099998));
#257671=CARTESIAN_POINT('Ctrl Pts',(-10.2925268990001,15.2,2.66299992599999));
#257672=CARTESIAN_POINT('Ctrl Pts',(-10.2925268990001,11.6,2.66299992599999));
#257673=CARTESIAN_POINT('Ctrl Pts',(-10.2947314240001,15.2,2.66303670599999));
#257674=CARTESIAN_POINT('Ctrl Pts',(-10.2947314240001,11.6,2.66303670599999));
#257675=CARTESIAN_POINT('Ctrl Pts',(-10.2969426400001,15.2,2.66307164099998));
#257676=CARTESIAN_POINT('Ctrl Pts',(-10.2969426400001,11.6,2.66307164099998));
#257677=CARTESIAN_POINT('Ctrl Pts',(-10.2991605340001,15.2,2.66310471999999));
#257678=CARTESIAN_POINT('Ctrl Pts',(-10.2991605340001,11.6,2.66310471999999));
#257679=CARTESIAN_POINT('Ctrl Pts',(-10.3013850920001,15.2,2.66313593099999));
#257680=CARTESIAN_POINT('Ctrl Pts',(-10.3013850920001,11.6,2.66313593099999));
#257681=CARTESIAN_POINT('Ctrl Pts',(-10.3036163000001,15.2,2.66316526499998));
#257682=CARTESIAN_POINT('Ctrl Pts',(-10.3036163000001,11.6,2.66316526499998));
#257683=CARTESIAN_POINT('Ctrl Pts',(-10.3058541460001,15.2,2.66319271199999));
#257684=CARTESIAN_POINT('Ctrl Pts',(-10.3058541460001,11.6,2.66319271199999));
#257685=CARTESIAN_POINT('Ctrl Pts',(-10.3080986170001,15.2,2.66321825899999));
#257686=CARTESIAN_POINT('Ctrl Pts',(-10.3080986170001,11.6,2.66321825899999));
#257687=CARTESIAN_POINT('Ctrl Pts',(-10.3103496970001,15.2,2.66324189799998));
#257688=CARTESIAN_POINT('Ctrl Pts',(-10.3103496970001,11.6,2.66324189799998));
#257689=CARTESIAN_POINT('Ctrl Pts',(-10.3126073740001,15.2,2.66326361599998));
#257690=CARTESIAN_POINT('Ctrl Pts',(-10.3126073740001,11.6,2.66326361599998));
#257691=CARTESIAN_POINT('Ctrl Pts',(-10.3148716350001,15.2,2.66328340499999));
#257692=CARTESIAN_POINT('Ctrl Pts',(-10.3148716350001,11.6,2.66328340499999));
#257693=CARTESIAN_POINT('Ctrl Pts',(-10.3171424670001,15.2,2.66330125299999));
#257694=CARTESIAN_POINT('Ctrl Pts',(-10.3171424670001,11.6,2.66330125299999));
#257695=CARTESIAN_POINT('Ctrl Pts',(-10.3194198560001,15.2,2.66331714999998));
#257696=CARTESIAN_POINT('Ctrl Pts',(-10.3194198560001,11.6,2.66331714999998));
#257697=CARTESIAN_POINT('Ctrl Pts',(-10.3217037880001,15.2,2.66333108599999));
#257698=CARTESIAN_POINT('Ctrl Pts',(-10.3217037880001,11.6,2.66333108599999));
#257699=CARTESIAN_POINT('Ctrl Pts',(-10.3239942520001,15.2,2.66334304999998));
#257700=CARTESIAN_POINT('Ctrl Pts',(-10.3239942520001,11.6,2.66334304999998));
#257701=CARTESIAN_POINT('Ctrl Pts',(-10.3262912330001,15.2,2.66335303299999));
#257702=CARTESIAN_POINT('Ctrl Pts',(-10.3262912330001,11.6,2.66335303299999));
#257703=CARTESIAN_POINT('Ctrl Pts',(-10.3285947190001,15.2,2.66336102499999));
#257704=CARTESIAN_POINT('Ctrl Pts',(-10.3285947190001,11.6,2.66336102499999));
#257705=CARTESIAN_POINT('Ctrl Pts',(-10.3309046950001,15.2,2.66336701399998));
#257706=CARTESIAN_POINT('Ctrl Pts',(-10.3309046950001,11.6,2.66336701399998));
#257707=CARTESIAN_POINT('Ctrl Pts',(-10.3332211510001,15.2,2.66337099099999));
#257708=CARTESIAN_POINT('Ctrl Pts',(-10.3332211510001,11.6,2.66337099099999));
#257709=CARTESIAN_POINT('Ctrl Pts',(-10.3355440700001,15.2,2.66337294499999));
#257710=CARTESIAN_POINT('Ctrl Pts',(-10.3355440700001,11.6,2.66337294499999));
#257711=CARTESIAN_POINT('Ctrl Pts',(-10.3378734430001,15.2,2.66337286799998));
#257712=CARTESIAN_POINT('Ctrl Pts',(-10.3378734430001,11.6,2.66337286799998));
#257713=CARTESIAN_POINT('Ctrl Pts',(-10.3402092540001,15.2,2.66337074899998));
#257714=CARTESIAN_POINT('Ctrl Pts',(-10.3402092540001,11.6,2.66337074899998));
#257715=CARTESIAN_POINT('Ctrl Pts',(-10.3425514920001,15.2,2.66336657699998));
#257716=CARTESIAN_POINT('Ctrl Pts',(-10.3425514920001,11.6,2.66336657699998));
#257717=CARTESIAN_POINT('Ctrl Pts',(-10.3449001440001,15.2,2.66336034399998));
#257718=CARTESIAN_POINT('Ctrl Pts',(-10.3449001440001,11.6,2.66336034399998));
#257719=CARTESIAN_POINT('Ctrl Pts',(-10.3472551960001,15.2,2.66335203799999));
#257720=CARTESIAN_POINT('Ctrl Pts',(-10.3472551960001,11.6,2.66335203799999));
#257721=CARTESIAN_POINT('Ctrl Pts',(-10.3496166340001,15.2,2.66334165099998));
#257722=CARTESIAN_POINT('Ctrl Pts',(-10.3496166340001,11.6,2.66334165099998));
#257723=CARTESIAN_POINT('Ctrl Pts',(-10.3519844490001,15.2,2.66332917099999));
#257724=CARTESIAN_POINT('Ctrl Pts',(-10.3519844490001,11.6,2.66332917099999));
#257725=CARTESIAN_POINT('Ctrl Pts',(-10.3543586250001,15.2,2.66331458999999));
#257726=CARTESIAN_POINT('Ctrl Pts',(-10.3543586250001,11.6,2.66331458999999));
#257727=CARTESIAN_POINT('Ctrl Pts',(-10.3567391510001,15.2,2.66329789899999));
#257728=CARTESIAN_POINT('Ctrl Pts',(-10.3567391510001,11.6,2.66329789899999));
#257729=CARTESIAN_POINT('Ctrl Pts',(-10.3591260120001,15.2,2.66327908699999));
#257730=CARTESIAN_POINT('Ctrl Pts',(-10.3591260120001,11.6,2.66327908699999));
#257731=CARTESIAN_POINT('Ctrl Pts',(-10.3615191980001,15.2,2.66325814399998));
#257732=CARTESIAN_POINT('Ctrl Pts',(-10.3615191980001,11.6,2.66325814399998));
#257733=CARTESIAN_POINT('Ctrl Pts',(-10.3639186950001,15.2,2.66323506099998));
#257734=CARTESIAN_POINT('Ctrl Pts',(-10.3639186950001,11.6,2.66323506099998));
#257735=CARTESIAN_POINT('Ctrl Pts',(-10.3663244900001,15.2,2.66320982799999));
#257736=CARTESIAN_POINT('Ctrl Pts',(-10.3663244900001,11.6,2.66320982799999));
#257737=CARTESIAN_POINT('Ctrl Pts',(-10.3687365710001,15.2,2.66318243599999));
#257738=CARTESIAN_POINT('Ctrl Pts',(-10.3687365710001,11.6,2.66318243599999));
#257739=CARTESIAN_POINT('Ctrl Pts',(-10.3711549250001,15.2,2.66315287599999));
#257740=CARTESIAN_POINT('Ctrl Pts',(-10.3711549250001,11.6,2.66315287599999));
#257741=CARTESIAN_POINT('Ctrl Pts',(-10.3735795410001,15.2,2.66312113599999));
#257742=CARTESIAN_POINT('Ctrl Pts',(-10.3735795410001,11.6,2.66312113599999));
#257743=CARTESIAN_POINT('Ctrl Pts',(-10.3760104050001,15.2,2.66308720999999));
#257744=CARTESIAN_POINT('Ctrl Pts',(-10.3760104050001,11.6,2.66308720999999));
#257745=CARTESIAN_POINT('Ctrl Pts',(-10.3784475030001,15.2,2.66305108599998));
#257746=CARTESIAN_POINT('Ctrl Pts',(-10.3784475030001,11.6,2.66305108599998));
#257747=CARTESIAN_POINT('Ctrl Pts',(-10.3808908260001,15.2,2.66301275499998));
#257748=CARTESIAN_POINT('Ctrl Pts',(-10.3808908260001,11.6,2.66301275499998));
#257749=CARTESIAN_POINT('Ctrl Pts',(-10.3833403590001,15.2,2.66297220899999));
#257750=CARTESIAN_POINT('Ctrl Pts',(-10.3833403590001,11.6,2.66297220899998));
#257751=CARTESIAN_POINT('Ctrl Pts',(-10.3857960910001,15.2,2.66292943799999));
#257752=CARTESIAN_POINT('Ctrl Pts',(-10.3857960910001,11.6,2.66292943799999));
#257753=CARTESIAN_POINT('Ctrl Pts',(-10.3882580090001,15.2,2.66288443299998));
#257754=CARTESIAN_POINT('Ctrl Pts',(-10.3882580090001,11.6,2.66288443299998));
#257755=CARTESIAN_POINT('Ctrl Pts',(-10.3907261000001,15.2,2.66283718399999));
#257756=CARTESIAN_POINT('Ctrl Pts',(-10.3907261000001,11.6,2.66283718399999));
#257757=CARTESIAN_POINT('Ctrl Pts',(-10.3932003530001,15.2,2.66278768199999));
#257758=CARTESIAN_POINT('Ctrl Pts',(-10.3932003530001,11.6,2.66278768199999));
#257759=CARTESIAN_POINT('Ctrl Pts',(-10.3956807540001,15.2,2.66273591899999));
#257760=CARTESIAN_POINT('Ctrl Pts',(-10.3956807540001,11.6,2.66273591899999));
#257761=CARTESIAN_POINT('Ctrl Pts',(-10.3981672930001,15.2,2.66268188399999));
#257762=CARTESIAN_POINT('Ctrl Pts',(-10.3981672930001,11.6,2.66268188399999));
#257763=CARTESIAN_POINT('Ctrl Pts',(-10.4006599560001,15.2,2.66262556899999));
#257764=CARTESIAN_POINT('Ctrl Pts',(-10.4006599560001,11.6,2.66262556899999));
#257765=CARTESIAN_POINT('Ctrl Pts',(-10.4031587310001,15.2,2.66256696399999));
#257766=CARTESIAN_POINT('Ctrl Pts',(-10.4031587310001,11.6,2.66256696399999));
#257767=CARTESIAN_POINT('Ctrl Pts',(-10.4056636070001,15.2,2.66250606099998));
#257768=CARTESIAN_POINT('Ctrl Pts',(-10.4056636070001,11.6,2.66250606099998));
#257769=CARTESIAN_POINT('Ctrl Pts',(-10.4081745700001,15.2,2.66244285099998));
#257770=CARTESIAN_POINT('Ctrl Pts',(-10.4081745700001,11.6,2.66244285099998));
#257771=CARTESIAN_POINT('Ctrl Pts',(-10.4106916090001,15.2,2.66237732499999));
#257772=CARTESIAN_POINT('Ctrl Pts',(-10.4106916090001,11.6,2.66237732499999));
#257773=CARTESIAN_POINT('Ctrl Pts',(-10.4132147120001,15.2,2.66230947299999));
#257774=CARTESIAN_POINT('Ctrl Pts',(-10.4132147120001,11.6,2.66230947299999));
#257775=CARTESIAN_POINT('Ctrl Pts',(-10.4157438670001,15.2,2.66223928799998));
#257776=CARTESIAN_POINT('Ctrl Pts',(-10.4157438670001,11.6,2.66223928799998));
#257777=CARTESIAN_POINT('Ctrl Pts',(-10.4182790610001,15.2,2.66216675899998));
#257778=CARTESIAN_POINT('Ctrl Pts',(-10.4182790610001,11.6,2.66216675899998));
#257779=CARTESIAN_POINT('Ctrl Pts',(-10.4208202830001,15.2,2.66209187899998));
#257780=CARTESIAN_POINT('Ctrl Pts',(-10.4208202830001,11.6,2.66209187899998));
#257781=CARTESIAN_POINT('Ctrl Pts',(-10.4233675200001,15.2,2.66201463899999));
#257782=CARTESIAN_POINT('Ctrl Pts',(-10.4233675200001,11.6,2.66201463899999));
#257783=CARTESIAN_POINT('Ctrl Pts',(-10.4259207610001,15.2,2.66193502899998));
#257784=CARTESIAN_POINT('Ctrl Pts',(-10.4259207610001,11.6,2.66193502899998));
#257785=CARTESIAN_POINT('Ctrl Pts',(-10.4284799940001,15.2,2.66185303999999));
#257786=CARTESIAN_POINT('Ctrl Pts',(-10.4284799940001,11.6,2.66185303999999));
#257787=CARTESIAN_POINT('Ctrl Pts',(-10.4310452060001,15.2,2.66176866499999));
#257788=CARTESIAN_POINT('Ctrl Pts',(-10.4310452060001,11.6,2.66176866499999));
#257789=CARTESIAN_POINT('Ctrl Pts',(-10.4336163860001,15.2,2.66168189499999));
#257790=CARTESIAN_POINT('Ctrl Pts',(-10.4336163860001,11.6,2.66168189499999));
#257791=CARTESIAN_POINT('Ctrl Pts',(-10.4361935220001,15.2,2.66159271999998));
#257792=CARTESIAN_POINT('Ctrl Pts',(-10.4361935220001,11.6,2.66159271999998));
#257793=CARTESIAN_POINT('Ctrl Pts',(-10.4387766020001,15.2,2.66150113299998));
#257794=CARTESIAN_POINT('Ctrl Pts',(-10.4387766020001,11.6,2.66150113299998));
#257795=CARTESIAN_POINT('Ctrl Pts',(-10.4413656150001,15.2,2.66140712399999));
#257796=CARTESIAN_POINT('Ctrl Pts',(-10.4413656150001,11.6,2.66140712399999));
#257797=CARTESIAN_POINT('Ctrl Pts',(-10.4439605480001,15.2,2.66131068599999));
#257798=CARTESIAN_POINT('Ctrl Pts',(-10.4439605480001,11.6,2.66131068599999));
#257799=CARTESIAN_POINT('Ctrl Pts',(-10.4465613900001,15.2,2.66121180899999));
#257800=CARTESIAN_POINT('Ctrl Pts',(-10.4465613900001,11.6,2.66121180899999));
#257801=CARTESIAN_POINT('Ctrl Pts',(-10.4491681290001,15.2,2.66111048599999));
#257802=CARTESIAN_POINT('Ctrl Pts',(-10.4491681290001,11.6,2.66111048599999));
#257803=CARTESIAN_POINT('Ctrl Pts',(-10.4517807530001,15.2,2.66100670699998));
#257804=CARTESIAN_POINT('Ctrl Pts',(-10.4517807530001,11.6,2.66100670699998));
#257805=CARTESIAN_POINT('Ctrl Pts',(-10.4543992500001,15.2,2.66090046499999));
#257806=CARTESIAN_POINT('Ctrl Pts',(-10.4543992500001,11.6,2.66090046499999));
#257807=CARTESIAN_POINT('Ctrl Pts',(-10.4570236090001,15.2,2.66079174999999));
#257808=CARTESIAN_POINT('Ctrl Pts',(-10.4570236090001,11.6,2.66079174999999));
#257809=CARTESIAN_POINT('Ctrl Pts',(-10.4596538190001,15.2,2.66068055499999));
#257810=CARTESIAN_POINT('Ctrl Pts',(-10.4596538190001,11.6,2.66068055499999));
#257811=CARTESIAN_POINT('Ctrl Pts',(-10.4622898670001,15.2,2.66056687199999));
#257812=CARTESIAN_POINT('Ctrl Pts',(-10.4622898670001,11.6,2.66056687199998));
#257813=CARTESIAN_POINT('Ctrl Pts',(-10.4649317430001,15.2,2.66045069099999));
#257814=CARTESIAN_POINT('Ctrl Pts',(-10.4649317430001,11.6,2.66045069099999));
#257815=CARTESIAN_POINT('Ctrl Pts',(-10.4675794330001,15.2,2.66033200499999));
#257816=CARTESIAN_POINT('Ctrl Pts',(-10.4675794330001,11.6,2.66033200499999));
#257817=CARTESIAN_POINT('Ctrl Pts',(-10.4702329280001,15.2,2.66021080599998));
#257818=CARTESIAN_POINT('Ctrl Pts',(-10.4702329280001,11.6,2.66021080599998));
#257819=CARTESIAN_POINT('Ctrl Pts',(-10.4728922150001,15.2,2.66008708399998));
#257820=CARTESIAN_POINT('Ctrl Pts',(-10.4728922150001,11.6,2.66008708399998));
#257821=CARTESIAN_POINT('Ctrl Pts',(-10.4755572830001,15.2,2.65996083299999));
#257822=CARTESIAN_POINT('Ctrl Pts',(-10.4755572830001,11.6,2.65996083299999));
#257823=CARTESIAN_POINT('Ctrl Pts',(-10.4782281200001,15.2,2.65983204299998));
#257824=CARTESIAN_POINT('Ctrl Pts',(-10.4782281200001,11.6,2.65983204299998));
#257825=CARTESIAN_POINT('Ctrl Pts',(-10.4809047160001,15.2,2.65970070699999));
#257826=CARTESIAN_POINT('Ctrl Pts',(-10.4809047160001,11.6,2.65970070699999));
#257827=CARTESIAN_POINT('Ctrl Pts',(-10.4835870570001,15.2,2.65956681699999));
#257828=CARTESIAN_POINT('Ctrl Pts',(-10.4835870570001,11.6,2.65956681699999));
#257829=CARTESIAN_POINT('Ctrl Pts',(-10.4862751350001,15.2,2.65943036399998));
#257830=CARTESIAN_POINT('Ctrl Pts',(-10.4862751350001,11.6,2.65943036399998));
#257831=CARTESIAN_POINT('Ctrl Pts',(-10.4889689350001,15.2,2.65929134099999));
#257832=CARTESIAN_POINT('Ctrl Pts',(-10.4889689350001,11.6,2.65929134099998));
#257833=CARTESIAN_POINT('Ctrl Pts',(-10.4916684480001,15.2,2.65914974099999));
#257834=CARTESIAN_POINT('Ctrl Pts',(-10.4916684480001,11.6,2.65914974099999));
#257835=CARTESIAN_POINT('Ctrl Pts',(-10.4943736620001,15.2,2.65900555299999));
#257836=CARTESIAN_POINT('Ctrl Pts',(-10.4943736620001,11.6,2.65900555299999));
#257837=CARTESIAN_POINT('Ctrl Pts',(-10.4970845660001,15.2,2.65885877099999));
#257838=CARTESIAN_POINT('Ctrl Pts',(-10.4970845660001,11.6,2.65885877099999));
#257839=CARTESIAN_POINT('Ctrl Pts',(-10.4998011490001,15.2,2.65870938599999));
#257840=CARTESIAN_POINT('Ctrl Pts',(-10.4998011490001,11.6,2.65870938599999));
#257841=CARTESIAN_POINT('Ctrl Pts',(-10.5025233980001,15.2,2.65855739099998));
#257842=CARTESIAN_POINT('Ctrl Pts',(-10.5025233980001,11.6,2.65855739099998));
#257843=CARTESIAN_POINT('Ctrl Pts',(-10.5052513030001,15.2,2.65840277799998));
#257844=CARTESIAN_POINT('Ctrl Pts',(-10.5052513030001,11.6,2.65840277799998));
#257845=CARTESIAN_POINT('Ctrl Pts',(-10.5079848540001,15.2,2.65824553999998));
#257846=CARTESIAN_POINT('Ctrl Pts',(-10.5079848540001,11.6,2.65824553999998));
#257847=CARTESIAN_POINT('Ctrl Pts',(-10.5107240380001,15.2,2.65808566799999));
#257848=CARTESIAN_POINT('Ctrl Pts',(-10.5107240380001,11.6,2.65808566799999));
#257849=CARTESIAN_POINT('Ctrl Pts',(-10.5134688430001,15.2,2.65792315499999));
#257850=CARTESIAN_POINT('Ctrl Pts',(-10.5134688430001,11.6,2.65792315499999));
#257851=CARTESIAN_POINT('Ctrl Pts',(-10.5162192600001,15.2,2.65775799199999));
#257852=CARTESIAN_POINT('Ctrl Pts',(-10.5162192600001,11.6,2.65775799199999));
#257853=CARTESIAN_POINT('Ctrl Pts',(-10.5189752770001,15.2,2.65759017199999));
#257854=CARTESIAN_POINT('Ctrl Pts',(-10.5189752770001,11.6,2.65759017199999));
#257855=CARTESIAN_POINT('Ctrl Pts',(-10.5217368840001,15.2,2.65741968699999));
#257856=CARTESIAN_POINT('Ctrl Pts',(-10.5217368840001,11.6,2.65741968699999));
#257857=CARTESIAN_POINT('Ctrl Pts',(-10.5245040670001,15.2,2.65724653099999));
#257858=CARTESIAN_POINT('Ctrl Pts',(-10.5245040670001,11.6,2.65724653099999));
#257859=CARTESIAN_POINT('Ctrl Pts',(-10.5272768180001,15.2,2.65707069399999));
#257860=CARTESIAN_POINT('Ctrl Pts',(-10.5272768180001,11.6,2.65707069399999));
#257861=CARTESIAN_POINT('Ctrl Pts',(-10.5300551240001,15.2,2.65689216899998));
#257862=CARTESIAN_POINT('Ctrl Pts',(-10.5300551240001,11.6,2.65689216899998));
#257863=CARTESIAN_POINT('Ctrl Pts',(-10.5328389750001,15.2,2.65671094999998));
#257864=CARTESIAN_POINT('Ctrl Pts',(-10.5328389750001,11.6,2.65671094999998));
#257865=CARTESIAN_POINT('Ctrl Pts',(-10.5356283600001,15.2,2.65652702799999));
#257866=CARTESIAN_POINT('Ctrl Pts',(-10.5356283600001,11.6,2.65652702799999));
#257867=CARTESIAN_POINT('Ctrl Pts',(-10.5384232670001,15.2,2.65634039599998));
#257868=CARTESIAN_POINT('Ctrl Pts',(-10.5384232670001,11.6,2.65634039599998));
#257869=CARTESIAN_POINT('Ctrl Pts',(-10.5412236860001,15.2,2.65615104599998));
#257870=CARTESIAN_POINT('Ctrl Pts',(-10.5412236860001,11.6,2.65615104599998));
#257871=CARTESIAN_POINT('Ctrl Pts',(-10.5440296060001,15.2,2.65595896999999));
#257872=CARTESIAN_POINT('Ctrl Pts',(-10.5440296060001,11.6,2.65595896999999));
#257873=CARTESIAN_POINT('Ctrl Pts',(-10.5468410160001,15.2,2.65576416199998));
#257874=CARTESIAN_POINT('Ctrl Pts',(-10.5468410160001,11.6,2.65576416199998));
#257875=CARTESIAN_POINT('Ctrl Pts',(-10.5496579050001,15.2,2.65556661399999));
#257876=CARTESIAN_POINT('Ctrl Pts',(-10.5496579050001,11.6,2.65556661399999));
#257877=CARTESIAN_POINT('Ctrl Pts',(-10.5524802620001,15.2,2.65536631799999));
#257878=CARTESIAN_POINT('Ctrl Pts',(-10.5524802620001,11.6,2.65536631799998));
#257879=CARTESIAN_POINT('Ctrl Pts',(-10.5553080750001,15.2,2.65516326799998));
#257880=CARTESIAN_POINT('Ctrl Pts',(-10.5553080750001,11.6,2.65516326799998));
#257881=CARTESIAN_POINT('Ctrl Pts',(-10.5581413360001,15.2,2.65495745499998));
#257882=CARTESIAN_POINT('Ctrl Pts',(-10.5581413360001,11.6,2.65495745499998));
#257883=CARTESIAN_POINT('Ctrl Pts',(-10.5609800320001,15.2,2.65474887199999));
#257884=CARTESIAN_POINT('Ctrl Pts',(-10.5609800320001,11.6,2.65474887199999));
#257885=CARTESIAN_POINT('Ctrl Pts',(-10.5638241530001,15.2,2.65453751199999));
#257886=CARTESIAN_POINT('Ctrl Pts',(-10.5638241530001,11.6,2.65453751199999));
#257887=CARTESIAN_POINT('Ctrl Pts',(-10.5666736870001,15.2,2.65432336899998));
#257888=CARTESIAN_POINT('Ctrl Pts',(-10.5666736870001,11.6,2.65432336899998));
#257889=CARTESIAN_POINT('Ctrl Pts',(-10.5695286260001,15.2,2.65410643399999));
#257890=CARTESIAN_POINT('Ctrl Pts',(-10.5695286260001,11.6,2.65410643399999));
#257891=CARTESIAN_POINT('Ctrl Pts',(-10.5723889570001,15.2,2.65388669999999));
#257892=CARTESIAN_POINT('Ctrl Pts',(-10.5723889570001,11.6,2.65388669999999));
#257893=CARTESIAN_POINT('Ctrl Pts',(-10.5752546690001,15.2,2.65366416099998));
#257894=CARTESIAN_POINT('Ctrl Pts',(-10.5752546690001,11.6,2.65366416099998));
#257895=CARTESIAN_POINT('Ctrl Pts',(-10.5781257530001,15.2,2.65343880799998));
#257896=CARTESIAN_POINT('Ctrl Pts',(-10.5781257530001,11.6,2.65343880799998));
#257897=CARTESIAN_POINT('Ctrl Pts',(-10.5810021970001,15.2,2.65321063499999));
#257898=CARTESIAN_POINT('Ctrl Pts',(-10.5810021970001,11.6,2.65321063499999));
#257899=CARTESIAN_POINT('Ctrl Pts',(-10.5838839910001,15.2,2.65297963599998));
#257900=CARTESIAN_POINT('Ctrl Pts',(-10.5838839910001,11.6,2.65297963599998));
#257901=CARTESIAN_POINT('Ctrl Pts',(-10.5867711240001,15.2,2.65274580099998));
#257902=CARTESIAN_POINT('Ctrl Pts',(-10.5867711240001,11.6,2.65274580099998));
#257903=CARTESIAN_POINT('Ctrl Pts',(-10.5896635860001,15.2,2.65250912599999));
#257904=CARTESIAN_POINT('Ctrl Pts',(-10.5896635860001,11.6,2.65250912599999));
#257905=CARTESIAN_POINT('Ctrl Pts',(-10.5925613650001,15.2,2.65226960099999));
#257906=CARTESIAN_POINT('Ctrl Pts',(-10.5925613650001,11.6,2.65226960099999));
#257907=CARTESIAN_POINT('Ctrl Pts',(-10.5954644520001,15.2,2.65202722099998));
#257908=CARTESIAN_POINT('Ctrl Pts',(-10.5954644520001,11.6,2.65202722099998));
#257909=CARTESIAN_POINT('Ctrl Pts',(-10.5983728360001,15.2,2.65178197799998));
#257910=CARTESIAN_POINT('Ctrl Pts',(-10.5983728360001,11.6,2.65178197799998));
#257911=CARTESIAN_POINT('Ctrl Pts',(-10.6012865070001,15.2,2.65153386599999));
#257912=CARTESIAN_POINT('Ctrl Pts',(-10.6012865070001,11.6,2.65153386599999));
#257913=CARTESIAN_POINT('Ctrl Pts',(-10.6042054530001,15.2,2.65128287899999));
#257914=CARTESIAN_POINT('Ctrl Pts',(-10.6042054530001,11.6,2.65128287899999));
#257915=CARTESIAN_POINT('Ctrl Pts',(-10.6071296640001,15.2,2.65102900599998));
#257916=CARTESIAN_POINT('Ctrl Pts',(-10.6071296640001,11.6,2.65102900599998));
#257917=CARTESIAN_POINT('Ctrl Pts',(-10.6100591290001,15.2,2.65077224399998));
#257918=CARTESIAN_POINT('Ctrl Pts',(-10.6100591290001,11.6,2.65077224399998));
#257919=CARTESIAN_POINT('Ctrl Pts',(-10.6129938410001,15.2,2.65051258599998));
#257920=CARTESIAN_POINT('Ctrl Pts',(-10.6129938410001,11.6,2.65051258599998));
#257921=CARTESIAN_POINT('Ctrl Pts',(-10.6159337850001,15.2,2.65025002199998));
#257922=CARTESIAN_POINT('Ctrl Pts',(-10.6159337850001,11.6,2.65025002199998));
#257923=CARTESIAN_POINT('Ctrl Pts',(-10.6188789520001,15.2,2.64998454799999));
#257924=CARTESIAN_POINT('Ctrl Pts',(-10.6188789520001,11.6,2.64998454799999));
#257925=CARTESIAN_POINT('Ctrl Pts',(-10.6218293330001,15.2,2.64971615699999));
#257926=CARTESIAN_POINT('Ctrl Pts',(-10.6218293330001,11.6,2.64971615699999));
#257927=CARTESIAN_POINT('Ctrl Pts',(-10.6247849170001,15.2,2.64944483999999));
#257928=CARTESIAN_POINT('Ctrl Pts',(-10.6247849170001,11.6,2.64944483999999));
#257929=CARTESIAN_POINT('Ctrl Pts',(-10.6277456920001,15.2,2.64917059199998));
#257930=CARTESIAN_POINT('Ctrl Pts',(-10.6277456920001,11.6,2.64917059199998));
#257931=CARTESIAN_POINT('Ctrl Pts',(-10.6307116510001,15.2,2.64889340699998));
#257932=CARTESIAN_POINT('Ctrl Pts',(-10.6307116510001,11.6,2.64889340699998));
#257933=CARTESIAN_POINT('Ctrl Pts',(-10.6336827810001,15.2,2.64861327699998));
#257934=CARTESIAN_POINT('Ctrl Pts',(-10.6336827810001,11.6,2.64861327699998));
#257935=CARTESIAN_POINT('Ctrl Pts',(-10.6366590710001,15.2,2.64833019599998));
#257936=CARTESIAN_POINT('Ctrl Pts',(-10.6366590710001,11.6,2.64833019599998));
#257937=CARTESIAN_POINT('Ctrl Pts',(-10.6396405130001,15.2,2.64804415599999));
#257938=CARTESIAN_POINT('Ctrl Pts',(-10.6396405130001,11.6,2.64804415599999));
#257939=CARTESIAN_POINT('Ctrl Pts',(-10.6426270960001,15.2,2.64775515199998));
#257940=CARTESIAN_POINT('Ctrl Pts',(-10.6426270960001,11.6,2.64775515199998));
#257941=CARTESIAN_POINT('Ctrl Pts',(-10.6456188090001,15.2,2.64746317599998));
#257942=CARTESIAN_POINT('Ctrl Pts',(-10.6456188090001,11.6,2.64746317599998));
#257943=CARTESIAN_POINT('Ctrl Pts',(-10.6486156430001,15.2,2.64716822299999));
#257944=CARTESIAN_POINT('Ctrl Pts',(-10.6486156430001,11.6,2.64716822299999));
#257945=CARTESIAN_POINT('Ctrl Pts',(-10.6516175860001,15.2,2.64687028499999));
#257946=CARTESIAN_POINT('Ctrl Pts',(-10.6516175860001,11.6,2.64687028499999));
#257947=CARTESIAN_POINT('Ctrl Pts',(-10.6546246300001,15.2,2.64656935599999));
#257948=CARTESIAN_POINT('Ctrl Pts',(-10.6546246300001,11.6,2.64656935599999));
#257949=CARTESIAN_POINT('Ctrl Pts',(-10.6576367620001,15.2,2.64626542899999));
#257950=CARTESIAN_POINT('Ctrl Pts',(-10.6576367620001,11.6,2.64626542899998));
#257951=CARTESIAN_POINT('Ctrl Pts',(-10.6606539750001,15.2,2.64595849899998));
#257952=CARTESIAN_POINT('Ctrl Pts',(-10.6606539750001,11.6,2.64595849899998));
#257953=CARTESIAN_POINT('Ctrl Pts',(-10.6636762580001,15.2,2.64564855699999));
#257954=CARTESIAN_POINT('Ctrl Pts',(-10.6636762580001,11.6,2.64564855699999));
#257955=CARTESIAN_POINT('Ctrl Pts',(-10.6667035990001,15.2,2.64533559999999));
#257956=CARTESIAN_POINT('Ctrl Pts',(-10.6667035990001,11.6,2.64533559999998));
#257957=CARTESIAN_POINT('Ctrl Pts',(-10.6697359890001,15.2,2.64501961799999));
#257958=CARTESIAN_POINT('Ctrl Pts',(-10.6697359890001,11.6,2.64501961799999));
#257959=CARTESIAN_POINT('Ctrl Pts',(-10.6727734180001,15.2,2.64470060699999));
#257960=CARTESIAN_POINT('Ctrl Pts',(-10.6727734180001,11.6,2.64470060699999));
#257961=CARTESIAN_POINT('Ctrl Pts',(-10.6758158770001,15.2,2.64437855899998));
#257962=CARTESIAN_POINT('Ctrl Pts',(-10.6758158770001,11.6,2.64437855899998));
#257963=CARTESIAN_POINT('Ctrl Pts',(-10.6788633540001,15.2,2.64405346799998));
#257964=CARTESIAN_POINT('Ctrl Pts',(-10.6788633540001,11.6,2.64405346799998));
#257965=CARTESIAN_POINT('Ctrl Pts',(-10.6819158400001,15.2,2.64372532899999));
#257966=CARTESIAN_POINT('Ctrl Pts',(-10.6819158400001,11.6,2.64372532899999));
#257967=CARTESIAN_POINT('Ctrl Pts',(-10.6849733260001,15.2,2.64339413399998));
#257968=CARTESIAN_POINT('Ctrl Pts',(-10.6849733260001,11.6,2.64339413399998));
#257969=CARTESIAN_POINT('Ctrl Pts',(-10.6880357990001,15.2,2.64305987699998));
#257970=CARTESIAN_POINT('Ctrl Pts',(-10.6880357990001,11.6,2.64305987699998));
#257971=CARTESIAN_POINT('Ctrl Pts',(-10.6911032520001,15.2,2.64272255199998));
#257972=CARTESIAN_POINT('Ctrl Pts',(-10.6911032520001,11.6,2.64272255199998));
#257973=CARTESIAN_POINT('Ctrl Pts',(-10.6941756740001,15.2,2.64238215299999));
#257974=CARTESIAN_POINT('Ctrl Pts',(-10.6941756740001,11.6,2.64238215299999));
#257975=CARTESIAN_POINT('Ctrl Pts',(-10.6972530540001,15.2,2.64203867399999));
#257976=CARTESIAN_POINT('Ctrl Pts',(-10.6972530540001,11.6,2.64203867399999));
#257977=CARTESIAN_POINT('Ctrl Pts',(-10.7003353830001,15.2,2.64169210799999));
#257978=CARTESIAN_POINT('Ctrl Pts',(-10.7003353830001,11.6,2.64169210799999));
#257979=CARTESIAN_POINT('Ctrl Pts',(-10.7034226510001,15.2,2.64134244899999));
#257980=CARTESIAN_POINT('Ctrl Pts',(-10.7034226510001,11.6,2.64134244899999));
#257981=CARTESIAN_POINT('Ctrl Pts',(-10.7065148490001,15.2,2.64098969099998));
#257982=CARTESIAN_POINT('Ctrl Pts',(-10.7065148490001,11.6,2.64098969099998));
#257983=CARTESIAN_POINT('Ctrl Pts',(-10.7096119650001,15.2,2.64063382799999));
#257984=CARTESIAN_POINT('Ctrl Pts',(-10.7096119650001,11.6,2.64063382799998));
#257985=CARTESIAN_POINT('Ctrl Pts',(-10.7127139910001,15.2,2.64027485299999));
#257986=CARTESIAN_POINT('Ctrl Pts',(-10.7127139910001,11.6,2.64027485299999));
#257987=CARTESIAN_POINT('Ctrl Pts',(-10.7158209160001,15.2,2.63991276099999));
#257988=CARTESIAN_POINT('Ctrl Pts',(-10.7158209160001,11.6,2.63991276099999));
#257989=CARTESIAN_POINT('Ctrl Pts',(-10.7189327310001,15.2,2.63954754399998));
#257990=CARTESIAN_POINT('Ctrl Pts',(-10.7189327310001,11.6,2.63954754399998));
#257991=CARTESIAN_POINT('Ctrl Pts',(-10.7220494270001,15.2,2.63917919899999));
#257992=CARTESIAN_POINT('Ctrl Pts',(-10.7220494270001,11.6,2.63917919899999));
#257993=CARTESIAN_POINT('Ctrl Pts',(-10.7251709920001,15.2,2.63880771699998));
#257994=CARTESIAN_POINT('Ctrl Pts',(-10.7251709920001,11.6,2.63880771699998));
#257995=CARTESIAN_POINT('Ctrl Pts',(-10.7282974160001,15.2,2.63843309399999));
#257996=CARTESIAN_POINT('Ctrl Pts',(-10.7282974160001,11.6,2.63843309399999));
#257997=CARTESIAN_POINT('Ctrl Pts',(-10.7314286920001,15.2,2.63805532299998));
#257998=CARTESIAN_POINT('Ctrl Pts',(-10.7314286920001,11.6,2.63805532299998));
#257999=CARTESIAN_POINT('Ctrl Pts',(-10.7345648080001,15.2,2.63767439799998));
#258000=CARTESIAN_POINT('Ctrl Pts',(-10.7345648080001,11.6,2.63767439799998));
#258001=CARTESIAN_POINT('Ctrl Pts',(-10.7377057560001,15.2,2.63729031299999));
#258002=CARTESIAN_POINT('Ctrl Pts',(-10.7377057560001,11.6,2.63729031299999));
#258003=CARTESIAN_POINT('Ctrl Pts',(-10.7408515230001,15.2,2.63690306299999));
#258004=CARTESIAN_POINT('Ctrl Pts',(-10.7408515230001,11.6,2.63690306299999));
#258005=CARTESIAN_POINT('Ctrl Pts',(-10.7440021030001,15.2,2.63651264099998));
#258006=CARTESIAN_POINT('Ctrl Pts',(-10.7440021030001,11.6,2.63651264099998));
#258007=CARTESIAN_POINT('Ctrl Pts',(-10.7471574850001,15.2,2.63611904099999));
#258008=CARTESIAN_POINT('Ctrl Pts',(-10.7471574850001,11.6,2.63611904099999));
#258009=CARTESIAN_POINT('Ctrl Pts',(-10.7503176590001,15.2,2.63572225799999));
#258010=CARTESIAN_POINT('Ctrl Pts',(-10.7503176590001,11.6,2.63572225799999));
#258011=CARTESIAN_POINT('Ctrl Pts',(-10.7534826150001,15.2,2.63532228399999));
#258012=CARTESIAN_POINT('Ctrl Pts',(-10.7534826150001,11.6,2.63532228399999));
#258013=CARTESIAN_POINT('Ctrl Pts',(-10.7566523440001,15.2,2.63491911599999));
#258014=CARTESIAN_POINT('Ctrl Pts',(-10.7566523440001,11.6,2.63491911599999));
#258015=CARTESIAN_POINT('Ctrl Pts',(-10.7598268370001,15.2,2.63451274799999));
#258016=CARTESIAN_POINT('Ctrl Pts',(-10.7598268370001,11.6,2.63451274799999));
#258017=CARTESIAN_POINT('Ctrl Pts',(-10.7630060830001,15.2,2.63410317099999));
#258018=CARTESIAN_POINT('Ctrl Pts',(-10.7630060830001,11.6,2.63410317099999));
#258019=CARTESIAN_POINT('Ctrl Pts',(-10.7661900720001,15.2,2.63369038299999));
#258020=CARTESIAN_POINT('Ctrl Pts',(-10.7661900720001,11.6,2.63369038299999));
#258021=CARTESIAN_POINT('Ctrl Pts',(-10.7693787950001,15.2,2.63327437599998));
#258022=CARTESIAN_POINT('Ctrl Pts',(-10.7693787950001,11.6,2.63327437599998));
#258023=CARTESIAN_POINT('Ctrl Pts',(-10.7725722440001,15.2,2.63285514399998));
#258024=CARTESIAN_POINT('Ctrl Pts',(-10.7725722440001,11.6,2.63285514399998));
#258025=CARTESIAN_POINT('Ctrl Pts',(-10.7757704090001,15.2,2.63243268299998));
#258026=CARTESIAN_POINT('Ctrl Pts',(-10.7757704090001,11.6,2.63243268299998));
#258027=CARTESIAN_POINT('Ctrl Pts',(-10.7789732780001,15.2,2.63200698499999));
#258028=CARTESIAN_POINT('Ctrl Pts',(-10.7789732780001,11.6,2.63200698499999));
#258029=CARTESIAN_POINT('Ctrl Pts',(-10.7821808440001,15.2,2.63157804699999));
#258030=CARTESIAN_POINT('Ctrl Pts',(-10.7821808440001,11.6,2.63157804699999));
#258031=CARTESIAN_POINT('Ctrl Pts',(-10.7853930960001,15.2,2.63114586099999));
#258032=CARTESIAN_POINT('Ctrl Pts',(-10.7853930960001,11.6,2.63114586099999));
#258033=CARTESIAN_POINT('Ctrl Pts',(-10.7886100260001,15.2,2.63071042299998));
#258034=CARTESIAN_POINT('Ctrl Pts',(-10.7886100260001,11.6,2.63071042299998));
#258035=CARTESIAN_POINT('Ctrl Pts',(-10.7918316230001,15.2,2.63027172599998));
#258036=CARTESIAN_POINT('Ctrl Pts',(-10.7918316230001,11.6,2.63027172599998));
#258037=CARTESIAN_POINT('Ctrl Pts',(-10.7950578790001,15.2,2.62982976599999));
#258038=CARTESIAN_POINT('Ctrl Pts',(-10.7950578790001,11.6,2.62982976599999));
#258039=CARTESIAN_POINT('Ctrl Pts',(-10.7982887820001,15.2,2.62938453599999));
#258040=CARTESIAN_POINT('Ctrl Pts',(-10.7982887820001,11.6,2.62938453599999));
#258041=CARTESIAN_POINT('Ctrl Pts',(-10.8015243260001,15.2,2.62893602899998));
#258042=CARTESIAN_POINT('Ctrl Pts',(-10.8015243260001,11.6,2.62893602899998));
#258043=CARTESIAN_POINT('Ctrl Pts',(-10.8047644990001,15.2,2.62848424299998));
#258044=CARTESIAN_POINT('Ctrl Pts',(-10.8047644990001,11.6,2.62848424299998));
#258045=CARTESIAN_POINT('Ctrl Pts',(-10.8080092930001,15.2,2.62802917099999));
#258046=CARTESIAN_POINT('Ctrl Pts',(-10.8080092930001,11.6,2.62802917099999));
#258047=CARTESIAN_POINT('Ctrl Pts',(-10.8112586980001,15.2,2.62757080599999));
#258048=CARTESIAN_POINT('Ctrl Pts',(-10.8112586980001,11.6,2.62757080599999));
#258049=CARTESIAN_POINT('Ctrl Pts',(-10.8145127050001,15.2,2.62710914399998));
#258050=CARTESIAN_POINT('Ctrl Pts',(-10.8145127050001,11.6,2.62710914399998));
#258051=CARTESIAN_POINT('Ctrl Pts',(-10.8177713030001,15.2,2.62664417899998));
#258052=CARTESIAN_POINT('Ctrl Pts',(-10.8177713030001,11.6,2.62664417899998));
#258053=CARTESIAN_POINT('Ctrl Pts',(-10.8210344850001,15.2,2.62617590599999));
#258054=CARTESIAN_POINT('Ctrl Pts',(-10.8210344850001,11.6,2.62617590599999));
#258055=CARTESIAN_POINT('Ctrl Pts',(-10.8243022400001,15.2,2.62570431899999));
#258056=CARTESIAN_POINT('Ctrl Pts',(-10.8243022400001,11.6,2.62570431899999));
#258057=CARTESIAN_POINT('Ctrl Pts',(-10.8275745600001,15.2,2.62522941199999));
#258058=CARTESIAN_POINT('Ctrl Pts',(-10.8275745600001,11.6,2.62522941199998));
#258059=CARTESIAN_POINT('Ctrl Pts',(-10.8308514350001,15.2,2.62475118099999));
#258060=CARTESIAN_POINT('Ctrl Pts',(-10.8308514350001,11.6,2.62475118099999));
#258061=CARTESIAN_POINT('Ctrl Pts',(-10.8341328550001,15.2,2.62426962099998));
#258062=CARTESIAN_POINT('Ctrl Pts',(-10.8341328550001,11.6,2.62426962099998));
#258063=CARTESIAN_POINT('Ctrl Pts',(-10.8374188130001,15.2,2.62378472399998));
#258064=CARTESIAN_POINT('Ctrl Pts',(-10.8374188130001,11.6,2.62378472399998));
#258065=CARTESIAN_POINT('Ctrl Pts',(-10.8407092960001,15.2,2.62329648699998));
#258066=CARTESIAN_POINT('Ctrl Pts',(-10.8407092960001,11.6,2.62329648699998));
#258067=CARTESIAN_POINT('Ctrl Pts',(-10.8440042990001,15.2,2.62280490399998));
#258068=CARTESIAN_POINT('Ctrl Pts',(-10.8440042990001,11.6,2.62280490399998));
#258069=CARTESIAN_POINT('Ctrl Pts',(-10.8473038090001,15.2,2.62230996899999));
#258070=CARTESIAN_POINT('Ctrl Pts',(-10.8473038090001,11.6,2.62230996899999));
#258071=CARTESIAN_POINT('Ctrl Pts',(-10.8506078190001,15.2,2.62181167699998));
#258072=CARTESIAN_POINT('Ctrl Pts',(-10.8506078190001,11.6,2.62181167699998));
#258073=CARTESIAN_POINT('Ctrl Pts',(-10.8539163200001,15.2,2.62131002399999));
#258074=CARTESIAN_POINT('Ctrl Pts',(-10.8539163200001,11.6,2.62131002399998));
#258075=CARTESIAN_POINT('Ctrl Pts',(-10.8572293010001,15.2,2.62080500299999));
#258076=CARTESIAN_POINT('Ctrl Pts',(-10.8572293010001,11.6,2.62080500299999));
#258077=CARTESIAN_POINT('Ctrl Pts',(-10.8605467540001,15.2,2.62029660899999));
#258078=CARTESIAN_POINT('Ctrl Pts',(-10.8605467540001,11.6,2.62029660899999));
#258079=CARTESIAN_POINT('Ctrl Pts',(-10.8638686700001,15.2,2.61978483699998));
#258080=CARTESIAN_POINT('Ctrl Pts',(-10.8638686700001,11.6,2.61978483699998));
#258081=CARTESIAN_POINT('Ctrl Pts',(-10.8671950400001,15.2,2.61926968199998));
#258082=CARTESIAN_POINT('Ctrl Pts',(-10.8671950400001,11.6,2.61926968199998));
#258083=CARTESIAN_POINT('Ctrl Pts',(-10.8705258540001,15.2,2.61875113999999));
#258084=CARTESIAN_POINT('Ctrl Pts',(-10.8705258540001,11.6,2.61875113999999));
#258085=CARTESIAN_POINT('Ctrl Pts',(-10.8738611030001,15.2,2.61822920299998));
#258086=CARTESIAN_POINT('Ctrl Pts',(-10.8738611030001,11.6,2.61822920299998));
#258087=CARTESIAN_POINT('Ctrl Pts',(-10.8772007790001,15.2,2.61770386799999));
#258088=CARTESIAN_POINT('Ctrl Pts',(-10.8772007790001,11.6,2.61770386799998));
#258089=CARTESIAN_POINT('Ctrl Pts',(-10.8805448720001,15.2,2.61717512899998));
#258090=CARTESIAN_POINT('Ctrl Pts',(-10.8805448720001,11.6,2.61717512899998));
#258091=CARTESIAN_POINT('Ctrl Pts',(-10.8838933720001,15.2,2.61664298099999));
#258092=CARTESIAN_POINT('Ctrl Pts',(-10.8838933720001,11.6,2.61664298099999));
#258093=CARTESIAN_POINT('Ctrl Pts',(-10.8872462720001,15.2,2.61610741899998));
#258094=CARTESIAN_POINT('Ctrl Pts',(-10.8872462720001,11.6,2.61610741899998));
#258095=CARTESIAN_POINT('Ctrl Pts',(-10.8906035620001,15.2,2.61556843799998));
#258096=CARTESIAN_POINT('Ctrl Pts',(-10.8906035620001,11.6,2.61556843799998));
#258097=CARTESIAN_POINT('Ctrl Pts',(-10.8939652320001,15.2,2.61502603199999));
#258098=CARTESIAN_POINT('Ctrl Pts',(-10.8939652320001,11.6,2.61502603199998));
#258099=CARTESIAN_POINT('Ctrl Pts',(-10.8973312750001,15.2,2.61448019799998));
#258100=CARTESIAN_POINT('Ctrl Pts',(-10.8973312750001,11.6,2.61448019799998));
#258101=CARTESIAN_POINT('Ctrl Pts',(-10.9007016800001,15.2,2.61393092799998));
#258102=CARTESIAN_POINT('Ctrl Pts',(-10.9007016800001,11.6,2.61393092799998));
#258103=CARTESIAN_POINT('Ctrl Pts',(-10.9040764380001,15.2,2.61337821999999));
#258104=CARTESIAN_POINT('Ctrl Pts',(-10.9040764380001,11.6,2.61337821999999));
#258105=CARTESIAN_POINT('Ctrl Pts',(-10.9074555420001,15.2,2.61282206699998));
#258106=CARTESIAN_POINT('Ctrl Pts',(-10.9074555420001,11.6,2.61282206699998));
#258107=CARTESIAN_POINT('Ctrl Pts',(-10.9108389810001,15.2,2.61226246499999));
#258108=CARTESIAN_POINT('Ctrl Pts',(-10.9108389810001,11.6,2.61226246499999));
#258109=CARTESIAN_POINT('Ctrl Pts',(-10.9142267470001,15.2,2.61169940799999));
#258110=CARTESIAN_POINT('Ctrl Pts',(-10.9142267470001,11.6,2.61169940799999));
#258111=CARTESIAN_POINT('Ctrl Pts',(-10.9176188310001,15.2,2.61113289199999));
#258112=CARTESIAN_POINT('Ctrl Pts',(-10.9176188310001,11.6,2.61113289199999));
#258113=CARTESIAN_POINT('Ctrl Pts',(-10.9210152230001,15.2,2.61056291099998));
#258114=CARTESIAN_POINT('Ctrl Pts',(-10.9210152230001,11.6,2.61056291099998));
#258115=CARTESIAN_POINT('Ctrl Pts',(-10.9244159170001,15.2,2.60998946099999));
#258116=CARTESIAN_POINT('Ctrl Pts',(-10.9244159170001,11.6,2.60998946099999));
#258117=CARTESIAN_POINT('Ctrl Pts',(-10.9278209010001,15.2,2.60941253699999));
#258118=CARTESIAN_POINT('Ctrl Pts',(-10.9278209010001,11.6,2.60941253699999));
#258119=CARTESIAN_POINT('Ctrl Pts',(-10.9312301670001,15.2,2.60883213399998));
#258120=CARTESIAN_POINT('Ctrl Pts',(-10.9312301670001,11.6,2.60883213399998));
#258121=CARTESIAN_POINT('Ctrl Pts',(-10.9346437070001,15.2,2.60824824699998));
#258122=CARTESIAN_POINT('Ctrl Pts',(-10.9346437070001,11.6,2.60824824699998));
#258123=CARTESIAN_POINT('Ctrl Pts',(-10.9380615100001,15.2,2.60766087099999));
#258124=CARTESIAN_POINT('Ctrl Pts',(-10.9380615100001,11.6,2.60766087099999));
#258125=CARTESIAN_POINT('Ctrl Pts',(-10.9414835700001,15.2,2.60707000099998));
#258126=CARTESIAN_POINT('Ctrl Pts',(-10.9414835700001,11.6,2.60707000099998));
#258127=CARTESIAN_POINT('Ctrl Pts',(-10.9449098760001,15.2,2.60647563299998));
#258128=CARTESIAN_POINT('Ctrl Pts',(-10.9449098760001,11.6,2.60647563299998));
#258129=CARTESIAN_POINT('Ctrl Pts',(-10.9483404200001,15.2,2.60587776099998));
#258130=CARTESIAN_POINT('Ctrl Pts',(-10.9483404200001,11.6,2.60587776099998));
#258131=CARTESIAN_POINT('Ctrl Pts',(-10.9517751930001,15.2,2.60527638199999));
#258132=CARTESIAN_POINT('Ctrl Pts',(-10.9517751930001,11.6,2.60527638199999));
#258133=CARTESIAN_POINT('Ctrl Pts',(-10.9552141870001,15.2,2.60467148899998));
#258134=CARTESIAN_POINT('Ctrl Pts',(-10.9552141870001,11.6,2.60467148899998));
#258135=CARTESIAN_POINT('Ctrl Pts',(-10.9586573930001,15.2,2.60406307899999));
#258136=CARTESIAN_POINT('Ctrl Pts',(-10.9586573930001,11.6,2.60406307899998));
#258137=CARTESIAN_POINT('Ctrl Pts',(-10.9621047990001,15.2,2.60345114599998));
#258138=CARTESIAN_POINT('Ctrl Pts',(-10.9621047990001,11.6,2.60345114599998));
#258139=CARTESIAN_POINT('Ctrl Pts',(-10.9655564020001,15.2,2.60283568599998));
#258140=CARTESIAN_POINT('Ctrl Pts',(-10.9655564020001,11.6,2.60283568599998));
#258141=CARTESIAN_POINT('Ctrl Pts',(-10.9690121870001,15.2,2.60221669399999));
#258142=CARTESIAN_POINT('Ctrl Pts',(-10.9690121870001,11.6,2.60221669399999));
#258143=CARTESIAN_POINT('Ctrl Pts',(-10.9724721500001,15.2,2.60159416599999));
#258144=CARTESIAN_POINT('Ctrl Pts',(-10.9724721500001,11.6,2.60159416599999));
#258145=CARTESIAN_POINT('Ctrl Pts',(-10.9759362810001,15.2,2.60096809599998));
#258146=CARTESIAN_POINT('Ctrl Pts',(-10.9759362810001,11.6,2.60096809599998));
#258147=CARTESIAN_POINT('Ctrl Pts',(-10.9794045700001,15.2,2.60033847899999));
#258148=CARTESIAN_POINT('Ctrl Pts',(-10.9794045700001,11.6,2.60033847899999));
#258149=CARTESIAN_POINT('Ctrl Pts',(-10.9828770100001,15.2,2.59970531199999));
#258150=CARTESIAN_POINT('Ctrl Pts',(-10.9828770100001,11.6,2.59970531199999));
#258151=CARTESIAN_POINT('Ctrl Pts',(-10.9863535920001,15.2,2.59906858999998));
#258152=CARTESIAN_POINT('Ctrl Pts',(-10.9863535920001,11.6,2.59906858999998));
#258153=CARTESIAN_POINT('Ctrl Pts',(-10.9898343060001,15.2,2.59842830899998));
#258154=CARTESIAN_POINT('Ctrl Pts',(-10.9898343060001,11.6,2.59842830899998));
#258155=CARTESIAN_POINT('Ctrl Pts',(-10.9933191440001,15.2,2.59778446199999));
#258156=CARTESIAN_POINT('Ctrl Pts',(-10.9933191440001,11.6,2.59778446199999));
#258157=CARTESIAN_POINT('Ctrl Pts',(-10.9968080970001,15.2,2.59713704699998));
#258158=CARTESIAN_POINT('Ctrl Pts',(-10.9968080970001,11.6,2.59713704699998));
#258159=CARTESIAN_POINT('Ctrl Pts',(-11.0003011580001,15.2,2.59648605699999));
#258160=CARTESIAN_POINT('Ctrl Pts',(-11.0003011580001,11.6,2.59648605699999));
#258161=CARTESIAN_POINT('Ctrl Pts',(-11.0037983160001,15.2,2.59583148899999));
#258162=CARTESIAN_POINT('Ctrl Pts',(-11.0037983160001,11.6,2.59583148899999));
#258163=CARTESIAN_POINT('Ctrl Pts',(-11.0072995640001,15.2,2.59517333899999));
#258164=CARTESIAN_POINT('Ctrl Pts',(-11.0072995640001,11.6,2.59517333899998));
#258165=CARTESIAN_POINT('Ctrl Pts',(-11.0108048930001,15.2,2.59451159999998));
#258166=CARTESIAN_POINT('Ctrl Pts',(-11.0108048930001,11.6,2.59451159999998));
#258167=CARTESIAN_POINT('Ctrl Pts',(-11.0143142940001,15.2,2.59384626999999));
#258168=CARTESIAN_POINT('Ctrl Pts',(-11.0143142940001,11.6,2.59384626999999));
#258169=CARTESIAN_POINT('Ctrl Pts',(-11.0178277600001,15.2,2.59317734299999));
#258170=CARTESIAN_POINT('Ctrl Pts',(-11.0178277600001,11.6,2.59317734299999));
#258171=CARTESIAN_POINT('Ctrl Pts',(-11.0213452790001,15.2,2.59250481599998));
#258172=CARTESIAN_POINT('Ctrl Pts',(-11.0213452790001,11.6,2.59250481599998));
#258173=CARTESIAN_POINT('Ctrl Pts',(-11.0248668450001,15.2,2.59182868299998));
#258174=CARTESIAN_POINT('Ctrl Pts',(-11.0248668450001,11.6,2.59182868299998));
#258175=CARTESIAN_POINT('Ctrl Pts',(-11.0283924510001,15.2,2.59114894099999));
#258176=CARTESIAN_POINT('Ctrl Pts',(-11.0283924510001,11.6,2.59114894099999));
#258177=CARTESIAN_POINT('Ctrl Pts',(-11.0319220850001,15.2,2.59046558299998));
#258178=CARTESIAN_POINT('Ctrl Pts',(-11.0319220850001,11.6,2.59046558299998));
#258179=CARTESIAN_POINT('Ctrl Pts',(-11.0354557400001,15.2,2.58977860699999));
#258180=CARTESIAN_POINT('Ctrl Pts',(-11.0354557400001,11.6,2.58977860699999));
#258181=CARTESIAN_POINT('Ctrl Pts',(-11.0389934070001,15.2,2.58908800799999));
#258182=CARTESIAN_POINT('Ctrl Pts',(-11.0389934070001,11.6,2.58908800799999));
#258183=CARTESIAN_POINT('Ctrl Pts',(-11.0425350780001,15.2,2.58839378199998));
#258184=CARTESIAN_POINT('Ctrl Pts',(-11.0425350780001,11.6,2.58839378199998));
#258185=CARTESIAN_POINT('Ctrl Pts',(-11.0460807450001,15.2,2.58769592199998));
#258186=CARTESIAN_POINT('Ctrl Pts',(-11.0460807450001,11.6,2.58769592199998));
#258187=CARTESIAN_POINT('Ctrl Pts',(-11.0496303980001,15.2,2.58699442799998));
#258188=CARTESIAN_POINT('Ctrl Pts',(-11.0496303980001,11.6,2.58699442799998));
#258189=CARTESIAN_POINT('Ctrl Pts',(-11.0531840300001,15.2,2.58628929099999));
#258190=CARTESIAN_POINT('Ctrl Pts',(-11.0531840300001,11.6,2.58628929099999));
#258191=CARTESIAN_POINT('Ctrl Pts',(-11.0567416320001,15.2,2.58558051099998));
#258192=CARTESIAN_POINT('Ctrl Pts',(-11.0567416320001,11.6,2.58558051099998));
#258193=CARTESIAN_POINT('Ctrl Pts',(-11.0603031950001,15.2,2.58486808099998));
#258194=CARTESIAN_POINT('Ctrl Pts',(-11.0603031950001,11.6,2.58486808099998));
#258195=CARTESIAN_POINT('Ctrl Pts',(-11.0638687110001,15.2,2.58415199699999));
#258196=CARTESIAN_POINT('Ctrl Pts',(-11.0638687110001,11.6,2.58415199699999));
#258197=CARTESIAN_POINT('Ctrl Pts',(-11.0674381720001,15.2,2.58343225399998));
#258198=CARTESIAN_POINT('Ctrl Pts',(-11.0674381720001,11.6,2.58343225399998));
#258199=CARTESIAN_POINT('Ctrl Pts',(-11.0710115690001,15.2,2.58270884999998));
#258200=CARTESIAN_POINT('Ctrl Pts',(-11.0710115690001,11.6,2.58270884999998));
#258201=CARTESIAN_POINT('Ctrl Pts',(-11.0745888930001,15.2,2.58198177899998));
#258202=CARTESIAN_POINT('Ctrl Pts',(-11.0745888930001,11.6,2.58198177899998));
#258203=CARTESIAN_POINT('Ctrl Pts',(-11.0781701370001,15.2,2.58125103699999));
#258204=CARTESIAN_POINT('Ctrl Pts',(-11.0781701370001,11.6,2.58125103699999));
#258205=CARTESIAN_POINT('Ctrl Pts',(-11.0817552930001,15.2,2.58051662099999));
#258206=CARTESIAN_POINT('Ctrl Pts',(-11.0817552930001,11.6,2.58051662099999));
#258207=CARTESIAN_POINT('Ctrl Pts',(-11.0853443500001,15.2,2.57977852499998));
#258208=CARTESIAN_POINT('Ctrl Pts',(-11.0853443500001,11.6,2.57977852499998));
#258209=CARTESIAN_POINT('Ctrl Pts',(-11.0889373030001,15.2,2.57903674599999));
#258210=CARTESIAN_POINT('Ctrl Pts',(-11.0889373030001,11.6,2.57903674599999));
#258211=CARTESIAN_POINT('Ctrl Pts',(-11.0925341410001,15.2,2.57829127899999));
#258212=CARTESIAN_POINT('Ctrl Pts',(-11.0925341410001,11.6,2.57829127899999));
#258213=CARTESIAN_POINT('Ctrl Pts',(-11.0961348560001,15.2,2.57754211899999));
#258214=CARTESIAN_POINT('Ctrl Pts',(-11.0961348560001,11.6,2.57754211899999));
#258215=CARTESIAN_POINT('Ctrl Pts',(-11.0997394400001,15.2,2.57678926399999));
#258216=CARTESIAN_POINT('Ctrl Pts',(-11.0997394400001,11.6,2.57678926399999));
#258217=CARTESIAN_POINT('Ctrl Pts',(-11.1033478850001,15.2,2.57603270799999));
#258218=CARTESIAN_POINT('Ctrl Pts',(-11.1033478850001,11.6,2.57603270799999));
#258219=CARTESIAN_POINT('Ctrl Pts',(-11.1069601830001,15.2,2.57527244799999));
#258220=CARTESIAN_POINT('Ctrl Pts',(-11.1069601830001,11.6,2.57527244799999));
#258221=CARTESIAN_POINT('Ctrl Pts',(-11.1105763250001,15.2,2.57450847999999));
#258222=CARTESIAN_POINT('Ctrl Pts',(-11.1105763250001,11.6,2.57450847999999));
#258223=CARTESIAN_POINT('Ctrl Pts',(-11.1141963030001,15.2,2.57374079699999));
#258224=CARTESIAN_POINT('Ctrl Pts',(-11.1141963030001,11.6,2.57374079699999));
#258225=CARTESIAN_POINT('Ctrl Pts',(-11.1178201080001,15.2,2.57296939999998));
#258226=CARTESIAN_POINT('Ctrl Pts',(-11.1178201080001,11.6,2.57296939999998));
#258227=CARTESIAN_POINT('Ctrl Pts',(-11.1214477320001,15.2,2.57219428099998));
#258228=CARTESIAN_POINT('Ctrl Pts',(-11.1214477320001,11.6,2.57219428099998));
#258229=CARTESIAN_POINT('Ctrl Pts',(-11.1250791700001,15.2,2.57141543699999));
#258230=CARTESIAN_POINT('Ctrl Pts',(-11.1250791700001,11.6,2.57141543699999));
#258231=CARTESIAN_POINT('Ctrl Pts',(-11.1287144100001,15.2,2.57063286499999));
#258232=CARTESIAN_POINT('Ctrl Pts',(-11.1287144100001,11.6,2.57063286499999));
#258233=CARTESIAN_POINT('Ctrl Pts',(-11.1323534440001,15.2,2.56984655999998));
#258234=CARTESIAN_POINT('Ctrl Pts',(-11.1323534440001,11.6,2.56984655999998));
#258235=CARTESIAN_POINT('Ctrl Pts',(-11.1359962660001,15.2,2.56905651699999));
#258236=CARTESIAN_POINT('Ctrl Pts',(-11.1359962660001,11.6,2.56905651699999));
#258237=CARTESIAN_POINT('Ctrl Pts',(-11.1396428650001,15.2,2.56826273399999));
#258238=CARTESIAN_POINT('Ctrl Pts',(-11.1396428650001,11.6,2.56826273399999));
#258239=CARTESIAN_POINT('Ctrl Pts',(-11.1432932330001,15.2,2.56746520399999));
#258240=CARTESIAN_POINT('Ctrl Pts',(-11.1432932330001,11.6,2.56746520399999));
#258241=CARTESIAN_POINT('Ctrl Pts',(-11.1469473610001,15.2,2.56666392599998));
#258242=CARTESIAN_POINT('Ctrl Pts',(-11.1469473610001,11.6,2.56666392599998));
#258243=CARTESIAN_POINT('Ctrl Pts',(-11.1506052430001,15.2,2.56585889299998));
#258244=CARTESIAN_POINT('Ctrl Pts',(-11.1506052430001,11.6,2.56585889299998));
#258245=CARTESIAN_POINT('Ctrl Pts',(-11.1542668700001,15.2,2.56505010399999));
#258246=CARTESIAN_POINT('Ctrl Pts',(-11.1542668700001,11.6,2.56505010399999));
#258247=CARTESIAN_POINT('Ctrl Pts',(-11.1579322340001,15.2,2.56423755399998));
#258248=CARTESIAN_POINT('Ctrl Pts',(-11.1579322340001,11.6,2.56423755399998));
#258249=CARTESIAN_POINT('Ctrl Pts',(-11.1616013300001,15.2,2.56342123899999));
#258250=CARTESIAN_POINT('Ctrl Pts',(-11.1616013300001,11.6,2.56342123899999));
#258251=CARTESIAN_POINT('Ctrl Pts',(-11.1652741470001,15.2,2.56260115599999));
#258252=CARTESIAN_POINT('Ctrl Pts',(-11.1652741470001,11.6,2.56260115599999));
#258253=CARTESIAN_POINT('Ctrl Pts',(-11.1689506800001,15.2,2.56177730199998));
#258254=CARTESIAN_POINT('Ctrl Pts',(-11.1689506800001,11.6,2.56177730199998));
#258255=CARTESIAN_POINT('Ctrl Pts',(-11.1726309200001,15.2,2.56094967199999));
#258256=CARTESIAN_POINT('Ctrl Pts',(-11.1726309200001,11.6,2.56094967199999));
#258257=CARTESIAN_POINT('Ctrl Pts',(-11.1763148560001,15.2,2.56011826199998));
#258258=CARTESIAN_POINT('Ctrl Pts',(-11.1763148560001,11.6,2.56011826199998));
#258259=CARTESIAN_POINT('Ctrl Pts',(-11.1800024800001,15.2,2.55928306599999));
#258260=CARTESIAN_POINT('Ctrl Pts',(-11.1800024800001,11.6,2.55928306599999));
#258261=CARTESIAN_POINT('Ctrl Pts',(-11.1836937810001,15.2,2.55844408099998));
#258262=CARTESIAN_POINT('Ctrl Pts',(-11.1836937810001,11.6,2.55844408099998));
#258263=CARTESIAN_POINT('Ctrl Pts',(-11.1873887500001,15.2,2.55760130099999));
#258264=CARTESIAN_POINT('Ctrl Pts',(-11.1873887500001,11.6,2.55760130099999));
#258265=CARTESIAN_POINT('Ctrl Pts',(-11.1910873770001,15.2,2.55675472199999));
#258266=CARTESIAN_POINT('Ctrl Pts',(-11.1910873770001,11.6,2.55675472199999));
#258267=CARTESIAN_POINT('Ctrl Pts',(-11.1947896560001,15.2,2.55590434099998));
#258268=CARTESIAN_POINT('Ctrl Pts',(-11.1947896560001,11.6,2.55590434099998));
#258269=CARTESIAN_POINT('Ctrl Pts',(-11.1984955800001,15.2,2.55505015599999));
#258270=CARTESIAN_POINT('Ctrl Pts',(-11.1984955800001,11.6,2.55505015599999));
#258271=CARTESIAN_POINT('Ctrl Pts',(-11.2022051470001,15.2,2.55419216399999));
#258272=CARTESIAN_POINT('Ctrl Pts',(-11.2022051470001,11.6,2.55419216399999));
#258273=CARTESIAN_POINT('Ctrl Pts',(-11.2059183540001,15.2,2.55333036499999));
#258274=CARTESIAN_POINT('Ctrl Pts',(-11.2059183540001,11.6,2.55333036499999));
#258275=CARTESIAN_POINT('Ctrl Pts',(-11.2088918300001,15.2,2.55263787899998));
#258276=CARTESIAN_POINT('Ctrl Pts',(-11.2088918300001,11.6,2.55263787899998));
#258277=CARTESIAN_POINT('Ctrl Pts',(-11.2111235750001,15.2,2.55211679999999));
#258278=CARTESIAN_POINT('Ctrl Pts',(-11.2111235750001,11.6,2.55211679999999));
#258279=CARTESIAN_POINT('Ctrl Pts',(-11.2126121320001,15.2,2.55176865399999));
#258280=CARTESIAN_POINT('Ctrl Pts',(-11.2126121320001,11.6,2.55176865399999));
#258281=CARTESIAN_POINT('Ctrl Pts',(-11.2133565920001,15.2,2.55159438999998));
#258282=CARTESIAN_POINT('Ctrl Pts',(-11.2133565920001,11.6,2.55159438999998));
#258283=CARTESIAN_POINT('Ctrl Pts',(-10.0330625580001,15.2,2.64164356399998));
#258284=CARTESIAN_POINT('Ctrl Pts',(-10.03482302717,15.2,2.64194831044285));
#258285=CARTESIAN_POINT('Ctrl Pts',(-10.0366407484416,15.2,2.64225751971682));
#258286=CARTESIAN_POINT('Ctrl Pts',(-10.0385148615364,15.2,2.64257038294905));
#258287=CARTESIAN_POINT('Ctrl Pts',(-10.0403980125518,15.2,2.64288475496593));
#258288=CARTESIAN_POINT('Ctrl Pts',(-10.0423381038147,15.2,2.64320281628067));
#258289=CARTESIAN_POINT('Ctrl Pts',(-10.0443343061932,15.2,2.64352378181437));
#258290=CARTESIAN_POINT('Ctrl Pts',(-10.0463305083903,15.2,2.64384474731891));
#258291=CARTESIAN_POINT('Ctrl Pts',(-10.0483828189766,15.2,2.64416861768683));
#258292=CARTESIAN_POINT('Ctrl Pts',(-10.0504904282333,15.2,2.64449462925831));
#258293=CARTESIAN_POINT('Ctrl Pts',(-10.05259803749,15.2,2.6448206408298));
#258294=CARTESIAN_POINT('Ctrl Pts',(-10.0547609456752,15.2,2.64514879427203));
#258295=CARTESIAN_POINT('Ctrl Pts',(-10.0569783630356,15.2,2.6454783536931));
#258296=CARTESIAN_POINT('Ctrl Pts',(-10.0591957805974,15.2,2.64580791314411));
#258297=CARTESIAN_POINT('Ctrl Pts',(-10.0614677060147,15.2,2.64613887440968));
#258298=CARTESIAN_POINT('Ctrl Pts',(-10.0637933707285,15.2,2.64647052701114));
#258299=CARTESIAN_POINT('Ctrl Pts',(-10.066506645911,15.2,2.64685745500097));
#258300=CARTESIAN_POINT('Ctrl Pts',(-10.0692930658019,15.2,2.64724531920595));
#258301=CARTESIAN_POINT('Ctrl Pts',(-10.0721514405131,15.2,2.64763302120117));
#258302=CARTESIAN_POINT('Ctrl Pts',(-10.0746014762659,15.2,2.64796533723589));
#258303=CARTESIAN_POINT('Ctrl Pts',(-10.077104375569,15.2,2.6482975368681));
#258304=CARTESIAN_POINT('Ctrl Pts',(-10.0796594095451,15.2,2.64862894605278));
#258305=CARTESIAN_POINT('Ctrl Pts',(-10.0826402821692,15.2,2.64901559005641));
#258306=CARTESIAN_POINT('Ctrl Pts',(-10.0856921168832,15.2,2.64940116149503));
#258307=CARTESIAN_POINT('Ctrl Pts',(-10.0888137817163,15.2,2.64978463072653));
#258308=CARTESIAN_POINT('Ctrl Pts',(-10.0914894947428,15.2,2.65011331867762));
#258309=CARTESIAN_POINT('Ctrl Pts',(-10.0942165130146,15.2,2.65044046151785));
#258310=CARTESIAN_POINT('Ctrl Pts',(-10.0969941418361,15.2,2.65076543253541));
#258311=CARTESIAN_POINT('Ctrl Pts',(-10.0997717704053,15.2,2.65109040352346));
#258312=CARTESIAN_POINT('Ctrl Pts',(-10.1026000079927,15.2,2.65141319986032));
#258313=CARTESIAN_POINT('Ctrl Pts',(-10.1054781797346,15.2,2.6517332150168));
#258314=CARTESIAN_POINT('Ctrl Pts',(-10.1083563514765,15.2,2.65205323017329));
#258315=CARTESIAN_POINT('Ctrl Pts',(-10.1112844546649,15.2,2.65237046014413));
#258316=CARTESIAN_POINT('Ctrl Pts',(-10.1142618273879,15.2,2.6526843154662));
#258317=CARTESIAN_POINT('Ctrl Pts',(-10.1172392003813,15.2,2.65299817081679));
#258318=CARTESIAN_POINT('Ctrl Pts',(-10.1202658403643,15.2,2.65330864964196));
#258319=CARTESIAN_POINT('Ctrl Pts',(-10.1233411005352,15.2,2.65361517507507));
#258320=CARTESIAN_POINT('Ctrl Pts',(-10.1264163604267,15.2,2.65392170048033));
#258321=CARTESIAN_POINT('Ctrl Pts',(-10.1295402396778,15.2,2.65422427246057));
#258322=CARTESIAN_POINT('Ctrl Pts',(-10.132712100648,15.2,2.65452233078288));
#258323=CARTESIAN_POINT('Ctrl Pts',(-10.1358839616182,15.2,2.6548203891052));
#258324=CARTESIAN_POINT('Ctrl Pts',(-10.1391038055679,15.2,2.65511393257785));
#258325=CARTESIAN_POINT('Ctrl Pts',(-10.1423710095304,15.2,2.65540241523425));
#258326=CARTESIAN_POINT('Ctrl Pts',(-10.1456382137898,15.2,2.65569089791686));
#258327=CARTESIAN_POINT('Ctrl Pts',(-10.14895277868,15.2,2.65597432189051));
#258328=CARTESIAN_POINT('Ctrl Pts',(-10.1523140903664,15.2,2.65625215348861));
#258329=CARTESIAN_POINT('Ctrl Pts',(-10.1556754017474,15.2,2.65652998506147));
#258330=CARTESIAN_POINT('Ctrl Pts',(-10.1590834649786,15.2,2.65680222564107));
#258331=CARTESIAN_POINT('Ctrl Pts',(-10.1625376761884,15.2,2.65706835629781));
#258332=CARTESIAN_POINT('Ctrl Pts',(-10.1659918873983,15.2,2.65733448695455));
#258333=CARTESIAN_POINT('Ctrl Pts',(-10.1694922497961,15.2,2.65759450932841));
#258334=CARTESIAN_POINT('Ctrl Pts',(-10.1730381740819,15.2,2.65784791815283));
#258335=CARTESIAN_POINT('Ctrl Pts',(-10.1771750859635,15.2,2.65814356179666));
#258336=CARTESIAN_POINT('Ctrl Pts',(-10.1813740127417,15.2,2.65843020520895));
#258337=CARTESIAN_POINT('Ctrl Pts',(-10.1856340416992,15.2,2.65870706775457));
#258338=CARTESIAN_POINT('Ctrl Pts',(-10.1892854949018,15.2,2.65894437849563));
#258339=CARTESIAN_POINT('Ctrl Pts',(-10.1929818390258,15.2,2.65917450500392));
#258340=CARTESIAN_POINT('Ctrl Pts',(-10.196722511138,15.2,2.65939697174618));
#258341=CARTESIAN_POINT('Ctrl Pts',(-10.2004631832501,15.2,2.65961943848842));
#258342=CARTESIAN_POINT('Ctrl Pts',(-10.2042481817748,15.2,2.65983424250942));
#258343=CARTESIAN_POINT('Ctrl Pts',(-10.2080769531327,15.2,2.66004092325247));
#258344=CARTESIAN_POINT('Ctrl Pts',(-10.2119057248383,15.2,2.66024760401429));
#258345=CARTESIAN_POINT('Ctrl Pts',(-10.2157782698399,15.2,2.660446157467));
#258346=CARTESIAN_POINT('Ctrl Pts',(-10.2196940444719,15.2,2.66063613431032));
#258347=CARTESIAN_POINT('Ctrl Pts',(-10.2242624476756,15.2,2.66085777393497));
#258348=CARTESIAN_POINT('Ctrl Pts',(-10.228889688663,15.2,2.66106773679313));
#258349=CARTESIAN_POINT('Ctrl Pts',(-10.2335749198123,15.2,2.66126532344821));
#258350=CARTESIAN_POINT('Ctrl Pts',(-10.2375908326949,15.2,2.66143468345806));
#258351=CARTESIAN_POINT('Ctrl Pts',(-10.2416493509317,15.2,2.66159495070038));
#258352=CARTESIAN_POINT('Ctrl Pts',(-10.2457499514903,15.2,2.66174569770818));
#258353=CARTESIAN_POINT('Ctrl Pts',(-10.2491671184363,15.2,2.66187132020783));
#258354=CARTESIAN_POINT('Ctrl Pts',(-10.2526135061945,15.2,2.66199032998565));
#258355=CARTESIAN_POINT('Ctrl Pts',(-10.2560888201202,15.2,2.66210248575466));
#258356=CARTESIAN_POINT('Ctrl Pts',(-10.2602591966794,15.2,2.66223707267259));
#258357=CARTESIAN_POINT('Ctrl Pts',(-10.2644712218128,15.2,2.66236178712083));
#258358=CARTESIAN_POINT('Ctrl Pts',(-10.2687243902416,15.2,2.66247622028334));
#258359=CARTESIAN_POINT('Ctrl Pts',(-10.2722686973944,15.2,2.66257158125556));
#258360=CARTESIAN_POINT('Ctrl Pts',(-10.2758415739022,15.2,2.66265980250525));
#258361=CARTESIAN_POINT('Ctrl Pts',(-10.2794427312103,15.2,2.66274065174171));
#258362=CARTESIAN_POINT('Ctrl Pts',(-10.283764119823,15.2,2.66283767082193));
#258363=CARTESIAN_POINT('Ctrl Pts',(-10.2881262325969,15.2,2.66292407391478));
#258364=CARTESIAN_POINT('Ctrl Pts',(-10.2925285750186,15.2,2.66299946724585));
#258365=CARTESIAN_POINT('Ctrl Pts',(-10.2961971938365,15.2,2.66306229502403));
#258366=CARTESIAN_POINT('Ctrl Pts',(-10.2998937493192,15.2,2.66311747731868));
#258367=CARTESIAN_POINT('Ctrl Pts',(-10.3036179592483,15.2,2.66316479322186));
#258368=CARTESIAN_POINT('Ctrl Pts',(-10.3088318532302,15.2,2.66323103548736));
#258369=CARTESIAN_POINT('Ctrl Pts',(-10.3140999532028,15.2,2.66328185661831));
#258370=CARTESIAN_POINT('Ctrl Pts',(-10.3194214920237,15.2,2.66331665974325));
#258371=CARTESIAN_POINT('Ctrl Pts',(-10.3262634701527,15.2,2.66336140661585));
#258372=CARTESIAN_POINT('Ctrl Pts',(-10.3331937896886,15.2,2.66337967464965));
#258373=CARTESIAN_POINT('Ctrl Pts',(-10.3402108602809,15.2,2.66337023577558));
#258374=CARTESIAN_POINT('Ctrl Pts',(-10.3441092329738,15.2,2.66336499195647));
#258375=CARTESIAN_POINT('Ctrl Pts',(-10.3480343817431,15.2,2.66335119775652));
#258376=CARTESIAN_POINT('Ctrl Pts',(-10.3519860390334,15.2,2.6633286457431));
#258377=CARTESIAN_POINT('Ctrl Pts',(-10.3559376963237,15.2,2.66330609372967));
#258378=CARTESIAN_POINT('Ctrl Pts',(-10.3599158609841,15.2,2.66327478816323));
#258379=CARTESIAN_POINT('Ctrl Pts',(-10.3639202692466,15.2,2.66323452351092));
#258380=CARTESIAN_POINT('Ctrl Pts',(-10.3679246775091,15.2,2.66319425885861));
#258381=CARTESIAN_POINT('Ctrl Pts',(-10.3719553298751,15.2,2.66314503698663));
#258382=CARTESIAN_POINT('Ctrl Pts',(-10.3760119632765,15.2,2.66308666052877));
#258383=CARTESIAN_POINT('Ctrl Pts',(-10.3800685966779,15.2,2.66302828407091));
#258384=CARTESIAN_POINT('Ctrl Pts',(-10.3841512130792,15.2,2.66296075166148));
#258385=CARTESIAN_POINT('Ctrl Pts',(-10.3882595522644,15.2,2.66288387200838));
#258386=CARTESIAN_POINT('Ctrl Pts',(-10.3948328948713,15.2,2.6627608645651));
#258387=CARTESIAN_POINT('Ctrl Pts',(-10.4014720887002,15.2,2.66261392210659));
#258388=CARTESIAN_POINT('Ctrl Pts',(-10.4081760887178,15.2,2.66244227199863));
#258389=CARTESIAN_POINT('Ctrl Pts',(-10.4115280889549,15.2,2.66235644693881));
#258390=CARTESIAN_POINT('Ctrl Pts',(-10.4148962921196,15.2,2.66226444478541));
#258391=CARTESIAN_POINT('Ctrl Pts',(-10.4182805684745,15.2,2.66216617121905));
#258392=CARTESIAN_POINT('Ctrl Pts',(-10.4216648443683,15.2,2.66206789766606));
#258393=CARTESIAN_POINT('Ctrl Pts',(-10.4250651934345,15.2,2.66196335370509));
#258394=CARTESIAN_POINT('Ctrl Pts',(-10.4284814884875,15.2,2.66185244349235));
#258395=CARTESIAN_POINT('Ctrl Pts',(-10.431897784006,15.2,2.6617415332645));
#258396=CARTESIAN_POINT('Ctrl Pts',(-10.4353300246598,15.2,2.66162425913311));
#258397=CARTESIAN_POINT('Ctrl Pts',(-10.4387780855154,15.2,2.66150052751483));
#258398=CARTESIAN_POINT('Ctrl Pts',(-10.44308816135,15.2,2.66134586300042));
#258399=CARTESIAN_POINT('Ctrl Pts',(-10.4474229556422,15.2,2.66118110989467));
#258400=CARTESIAN_POINT('Ctrl Pts',(-10.4517822217645,15.2,2.66100609120466));
#258401=CARTESIAN_POINT('Ctrl Pts',(-10.4552696343772,15.2,2.66086607626409));
#258402=CARTESIAN_POINT('Ctrl Pts',(-10.4587727093012,15.2,2.66071949113562));
#258403=CARTESIAN_POINT('Ctrl Pts',(-10.4622913236792,15.2,2.66056624753748));
#258404=CARTESIAN_POINT('Ctrl Pts',(-10.4658099385365,15.2,2.66041300391845));
#258405=CARTESIAN_POINT('Ctrl Pts',(-10.4693440916153,15.2,2.66025310126806));
#258406=CARTESIAN_POINT('Ctrl Pts',(-10.472893660532,15.2,2.66008645170299));
#258407=CARTESIAN_POINT('Ctrl Pts',(-10.476443228965,15.2,2.65991980216062));
#258408=CARTESIAN_POINT('Ctrl Pts',(-10.4800082127318,15.2,2.65974640584203));
#258409=CARTESIAN_POINT('Ctrl Pts',(-10.4835884906722,15.2,2.65956617629279));
#258410=CARTESIAN_POINT('Ctrl Pts',(-10.4880638384636,15.2,2.65934088933784));
#258411=CARTESIAN_POINT('Ctrl Pts',(-10.4925630812722,15.2,2.65910492722664));
#258412=CARTESIAN_POINT('Ctrl Pts',(-10.4970859854377,15.2,2.65885812028276));
#258413=CARTESIAN_POINT('Ctrl Pts',(-10.5016088896031,15.2,2.65861131333888));
#258414=CARTESIAN_POINT('Ctrl Pts',(-10.5061554536025,15.2,2.65835366302805));
#258415=CARTESIAN_POINT('Ctrl Pts',(-10.5107254429763,15.2,2.65808500775085));
#258416=CARTESIAN_POINT('Ctrl Pts',(-10.51529543235,15.2,2.65781635247365));
#258417=CARTESIAN_POINT('Ctrl Pts',(-10.5198888487266,15.2,2.65753668945702));
#258418=CARTESIAN_POINT('Ctrl Pts',(-10.5245054589558,15.2,2.65724586077517));
#258419=CARTESIAN_POINT('Ctrl Pts',(-10.5281987473405,15.2,2.65701319781701));
#258420=CARTESIAN_POINT('Ctrl Pts',(-10.5319068808099,15.2,2.65677338729882));
#258421=CARTESIAN_POINT('Ctrl Pts',(-10.5356297411254,15.2,2.65652635045129));
#258422=CARTESIAN_POINT('Ctrl Pts',(-10.5393526009336,15.2,2.65627931363741));
#258423=CARTESIAN_POINT('Ctrl Pts',(-10.54309018764,15.2,2.65602504855503));
#258424=CARTESIAN_POINT('Ctrl Pts',(-10.5468423854434,15.2,2.65576347702133));
#258425=CARTESIAN_POINT('Ctrl Pts',(-10.550594583758,15.2,2.65550190545199));
#258426=CARTESIAN_POINT('Ctrl Pts',(-10.5543613915386,15.2,2.65523302726716));
#258427=CARTESIAN_POINT('Ctrl Pts',(-10.5581426953238,15.2,2.65495676245988));
#258428=CARTESIAN_POINT('Ctrl Pts',(-10.5628693247976,15.2,2.6546114314696));
#258429=CARTESIAN_POINT('Ctrl Pts',(-10.5676186017778,15.2,2.65425456055276));
#258430=CARTESIAN_POINT('Ctrl Pts',(-10.5723903028908,15.2,2.6538859986768));
#258431=CARTESIAN_POINT('Ctrl Pts',(-10.5771620040038,15.2,2.65351743680084));
#258432=CARTESIAN_POINT('Ctrl Pts',(-10.5819561292227,15.2,2.65313718353857));
#258433=CARTESIAN_POINT('Ctrl Pts',(-10.5867724568633,15.2,2.65274509089872));
#258434=CARTESIAN_POINT('Ctrl Pts',(-10.591588783979,15.2,2.65235299830161));
#258435=CARTESIAN_POINT('Ctrl Pts',(-10.5964273130236,15.2,2.65194906423032));
#258436=CARTESIAN_POINT('Ctrl Pts',(-10.6012878251309,15.2,2.65153314726275));
#258437=CARTESIAN_POINT('Ctrl Pts',(-10.6080925429288,15.2,2.65095086343561));
#258438=CARTESIAN_POINT('Ctrl Pts',(-10.6149403430503,15.2,2.65034508626605));
#258439=CARTESIAN_POINT('Ctrl Pts',(-10.6218306334199,15.2,2.64971542556269));
#258440=CARTESIAN_POINT('Ctrl Pts',(-10.6267522693216,15.2,2.64926566792444));
#258441=CARTESIAN_POINT('Ctrl Pts',(-10.6316955836026,15.2,2.64880372468017));
#258442=CARTESIAN_POINT('Ctrl Pts',(-10.6366603589723,15.2,2.64832945627527));
#258443=CARTESIAN_POINT('Ctrl Pts',(-10.6406321794845,15.2,2.64795004153068));
#258444=CARTESIAN_POINT('Ctrl Pts',(-10.6446177371623,15.2,2.64756273816885));
#258445=CARTESIAN_POINT('Ctrl Pts',(-10.6486169209372,15.2,2.64716747670205));
#258446=CARTESIAN_POINT('Ctrl Pts',(-10.6526161041672,15.2,2.64677221528911));
#258447=CARTESIAN_POINT('Ctrl Pts',(-10.6566289131038,15.2,2.64636899471608));
#258448=CARTESIAN_POINT('Ctrl Pts',(-10.6606552421626,15.2,2.64595774608356));
#258449=CARTESIAN_POINT('Ctrl Pts',(-10.6656881538976,15.2,2.64544368525089));
#258450=CARTESIAN_POINT('Ctrl Pts',(-10.670742185986,15.2,2.64491708155677));
#258451=CARTESIAN_POINT('Ctrl Pts',(-10.6758171311932,15.2,2.64437779829354));
#258452=CARTESIAN_POINT('Ctrl Pts',(-10.6819070652207,15.2,2.64373065840118));
#258453=CARTESIAN_POINT('Ctrl Pts',(-10.6880271127384,15.2,2.64306526212345));
#258454=CARTESIAN_POINT('Ctrl Pts',(-10.6941769128464,15.2,2.64238138306622));
#258455=CARTESIAN_POINT('Ctrl Pts',(-10.6982767799574,15.2,2.64192546365333));
#258456=CARTESIAN_POINT('Ctrl Pts',(-10.7023898700862,15.2,2.64146132948965));
#258457=CARTESIAN_POINT('Ctrl Pts',(-10.7065160785333,15.2,2.64098891474169));
#258458=CARTESIAN_POINT('Ctrl Pts',(-10.7106422869804,15.2,2.64051649999372));
#258459=CARTESIAN_POINT('Ctrl Pts',(-10.7147816121763,15.2,2.64003580389756));
#258460=CARTESIAN_POINT('Ctrl Pts',(-10.7189339519039,15.2,2.63954676187006));
#258461=CARTESIAN_POINT('Ctrl Pts',(-10.7230862910658,15.2,2.63905771990918));
#258462=CARTESIAN_POINT('Ctrl Pts',(-10.7272516421309,15.2,2.63856033246128));
#258463=CARTESIAN_POINT('Ctrl Pts',(-10.7314299020305,15.2,2.63805453450036));
#258464=CARTESIAN_POINT('Ctrl Pts',(-10.7356081624993,15.2,2.63754873647052));
#258465=CARTESIAN_POINT('Ctrl Pts',(-10.7397993304653,15.2,2.63703452839668));
#258466=CARTESIAN_POINT('Ctrl Pts',(-10.7440033041957,15.2,2.63651184642289));
#258467=CARTESIAN_POINT('Ctrl Pts',(-10.7482072773533,15.2,2.6359891645203));
#258468=CARTESIAN_POINT('Ctrl Pts',(-10.7524240547621,15.2,2.63545800747438));
#258469=CARTESIAN_POINT('Ctrl Pts',(-10.7566535346377,15.2,2.63491831601906));
#258470=CARTESIAN_POINT('Ctrl Pts',(-10.7619403849144,15.2,2.63424370164476));
#258471=CARTESIAN_POINT('Ctrl Pts',(-10.7672470794841,15.2,2.63355574838688));
#258472=CARTESIAN_POINT('Ctrl Pts',(-10.7725734229804,15.2,2.63285433671706));
#258473=CARTESIAN_POINT('Ctrl Pts',(-10.7768344980098,15.2,2.63229320735063));
#258474=CARTESIAN_POINT('Ctrl Pts',(-10.7811081456632,15.2,2.63172346452397));
#258475=CARTESIAN_POINT('Ctrl Pts',(-10.7853942661758,15.2,2.63114504788044));
#258476=CARTESIAN_POINT('Ctrl Pts',(-10.7896803861045,15.2,2.63056663131573));
#258477=CARTESIAN_POINT('Ctrl Pts',(-10.7939789785343,15.2,2.6299795419577));
#258478=CARTESIAN_POINT('Ctrl Pts',(-10.7982899418477,15.2,2.62938371684031));
#258479=CARTESIAN_POINT('Ctrl Pts',(-10.80367864643,15.2,2.62863893538269));
#258480=CARTESIAN_POINT('Ctrl Pts',(-10.8090866831725,15.2,2.6278805081928));
#258481=CARTESIAN_POINT('Ctrl Pts',(-10.8145138527804,15.2,2.62710831825877));
#258482=CARTESIAN_POINT('Ctrl Pts',(-10.8188555887034,15.2,2.62649056627788));
#258483=CARTESIAN_POINT('Ctrl Pts',(-10.8232095703358,15.2,2.62586400675666));
#258484=CARTESIAN_POINT('Ctrl Pts',(-10.8275756994639,15.2,2.62522858088779));
#258485=CARTESIAN_POINT('Ctrl Pts',(-10.8330333605766,15.2,2.62443429859499));
#258486=CARTESIAN_POINT('Ctrl Pts',(-10.8385100004062,15.2,2.62362616499918));
#258487=CARTESIAN_POINT('Ctrl Pts',(-10.8440054265188,15.2,2.62280406590082));
#258488=CARTESIAN_POINT('Ctrl Pts',(-10.8473026820666,15.2,2.62231080645972));
#258489=CARTESIAN_POINT('Ctrl Pts',(-10.8506067004114,15.2,2.62181251942669));
#258490=CARTESIAN_POINT('Ctrl Pts',(-10.8539174406656,15.2,2.62130918191925));
#258491=CARTESIAN_POINT('Ctrl Pts',(-10.8572281809198,15.2,2.62080584441181));
#258492=CARTESIAN_POINT('Ctrl Pts',(-10.860545641766,15.2,2.62029745505909));
#258493=CARTESIAN_POINT('Ctrl Pts',(-10.8638697838541,15.2,2.6197839912023));
#258494=CARTESIAN_POINT('Ctrl Pts',(-10.8683019731037,15.2,2.61909937275767));
#258495=CARTESIAN_POINT('Ctrl Pts',(-10.8727460379981,15.2,2.61840573367598));
#258496=CARTESIAN_POINT('Ctrl Pts',(-10.8772018825215,15.2,2.61770301712324));
#258497=CARTESIAN_POINT('Ctrl Pts',(-10.8805437666729,15.2,2.61717597958901));
#258498=CARTESIAN_POINT('Ctrl Pts',(-10.8838922755763,15.2,2.61664383616167));
#258499=CARTESIAN_POINT('Ctrl Pts',(-10.8872473702314,15.2,2.61610656412456));
#258500=CARTESIAN_POINT('Ctrl Pts',(-10.8906024642771,15.2,2.61556929218505));
#258501=CARTESIAN_POINT('Ctrl Pts',(-10.8939641429551,15.2,2.61502689136876));
#258502=CARTESIAN_POINT('Ctrl Pts',(-10.8973323661684,15.2,2.61447933894403));
#258503=CARTESIAN_POINT('Ctrl Pts',(-10.9007005893817,15.2,2.6139317865193));
#258504=CARTESIAN_POINT('Ctrl Pts',(-10.9040753555576,15.2,2.61337908256931));
#258505=CARTESIAN_POINT('Ctrl Pts',(-10.9074566261437,15.2,2.61282120467246));
#258506=CARTESIAN_POINT('Ctrl Pts',(-10.9130920773252,15.2,2.61189140814393));
#258507=CARTESIAN_POINT('Ctrl Pts',(-10.918745592959,15.2,2.61094723813244));
#258508=CARTESIAN_POINT('Ctrl Pts',(-10.9244169899044,15.2,2.60998859243724));
#258509=CARTESIAN_POINT('Ctrl Pts',(-10.927819827948,15.2,2.60941340504101));
#258510=CARTESIAN_POINT('Ctrl Pts',(-10.9312291021117,15.2,2.60883300664756));
#258511=CARTESIAN_POINT('Ctrl Pts',(-10.9346447727948,15.2,2.60824737474949));
#258512=CARTESIAN_POINT('Ctrl Pts',(-10.9391990001654,15.2,2.60746653225419));
#258513=CARTESIAN_POINT('Ctrl Pts',(-10.9437645998298,15.2,2.6066763855033));
#258514=CARTESIAN_POINT('Ctrl Pts',(-10.94834147651,15.2,2.6058768843474));
#258515=CARTESIAN_POINT('Ctrl Pts',(-10.954062572828,15.2,2.60487750782083));
#258516=CARTESIAN_POINT('Ctrl Pts',(-10.959801291493,15.2,2.6038635137667));
#258517=CARTESIAN_POINT('Ctrl Pts',(-10.9655574468388,15.2,2.60283480314291));
#258518=CARTESIAN_POINT('Ctrl Pts',(-10.9690111405482,15.2,2.60221757667892));
#258519=CARTESIAN_POINT('Ctrl Pts',(-10.9724711114844,15.2,2.60159505305512));
#258520=CARTESIAN_POINT('Ctrl Pts',(-10.9759373212807,15.2,2.60096720912981));
#258521=CARTESIAN_POINT('Ctrl Pts',(-10.9817143361385,15.2,2.59992080285378));
#258522=CARTESIAN_POINT('Ctrl Pts',(-10.9875086812525,15.2,2.59885962227225));
#258523=CARTESIAN_POINT('Ctrl Pts',(-10.9933201720065,15.2,2.5977835700991));
#258524=CARTESIAN_POINT('Ctrl Pts',(-10.9968070673458,15.2,2.597137938631));
#258525=CARTESIAN_POINT('Ctrl Pts',(-11.0003001364035,15.2,2.59648695288639));
#258526=CARTESIAN_POINT('Ctrl Pts',(-11.0037993392462,15.2,2.59583059333193));
#258527=CARTESIAN_POINT('Ctrl Pts',(-11.008464941977,15.2,2.59495544745805));
#258528=CARTESIAN_POINT('Ctrl Pts',(-11.0131414509675,15.2,2.59407074614098));
#258529=CARTESIAN_POINT('Ctrl Pts',(-11.0178287729169,15.2,2.59317644304804));
#258530=CARTESIAN_POINT('Ctrl Pts',(-11.022516095505,15.2,2.59228213983327));
#258531=CARTESIAN_POINT('Ctrl Pts',(-11.0272142319166,15.2,2.59137823483956));
#258532=CARTESIAN_POINT('Ctrl Pts',(-11.0319230906184,15.2,2.59046467840025));
#258533=CARTESIAN_POINT('Ctrl Pts',(-11.0366319486786,15.2,2.58955112208541));
#258534=CARTESIAN_POINT('Ctrl Pts',(-11.0413515286011,15.2,2.5886279166965));
#258535=CARTESIAN_POINT('Ctrl Pts',(-11.0460817408387,15.2,2.58769501356034));
#258536=CARTESIAN_POINT('Ctrl Pts',(-11.0508119537207,15.2,2.58676211029707));
#258537=CARTESIAN_POINT('Ctrl Pts',(-11.0555527982678,15.2,2.58581951063295));
#258538=CARTESIAN_POINT('Ctrl Pts',(-11.0603041836385,15.2,2.58486716741374));
#258539=CARTESIAN_POINT('Ctrl Pts',(-11.0650555683619,15.2,2.58391482432429));
#258540=CARTESIAN_POINT('Ctrl Pts',(-11.0698174947693,15.2,2.58295273705902));
#258541=CARTESIAN_POINT('Ctrl Pts',(-11.0745898722114,15.2,2.58198086141725));
#258542=CARTESIAN_POINT('Ctrl Pts',(-11.0805553445017,15.2,2.58076601676573));
#258543=CARTESIAN_POINT('Ctrl Pts',(-11.086537149533,15.2,2.57953587896683));
#258544=CARTESIAN_POINT('Ctrl Pts',(-11.0925351095538,15.2,2.57829035591956));
#258545=CARTESIAN_POINT('Ctrl Pts',(-11.0961338854355,15.2,2.57754304211835));
#258546=CARTESIAN_POINT('Ctrl Pts',(-11.0997384767949,15.2,2.57679019042038));
#258547=CARTESIAN_POINT('Ctrl Pts',(-11.1033488474546,15.2,2.57603178215702));
#258548=CARTESIAN_POINT('Ctrl Pts',(-11.1069592187702,15.2,2.57527337375588));
#258549=CARTESIAN_POINT('Ctrl Pts',(-11.1105753692291,15.2,2.57450940866153));
#258550=CARTESIAN_POINT('Ctrl Pts',(-11.1141972605479,15.2,2.57373986825726));
#258551=CARTESIAN_POINT('Ctrl Pts',(-11.1178191512088,15.2,2.57297032799279));
#258552=CARTESIAN_POINT('Ctrl Pts',(-11.1214467828943,15.2,2.57219521320362));
#258553=CARTESIAN_POINT('Ctrl Pts',(-11.1250801209295,15.2,2.57141450489817));
#258554=CARTESIAN_POINT('Ctrl Pts',(-11.1287134589646,15.2,2.57063379659272));
#258555=CARTESIAN_POINT('Ctrl Pts',(-11.1323525006858,15.2,2.56984749530749));
#258556=CARTESIAN_POINT('Ctrl Pts',(-11.1359972102783,15.2,2.56905558195764));
#258557=CARTESIAN_POINT('Ctrl Pts',(-11.1396419198708,15.2,2.56826366860779));
#258558=CARTESIAN_POINT('Ctrl Pts',(-11.1432922952129,15.2,2.56746614310853));
#258559=CARTESIAN_POINT('Ctrl Pts',(-11.1469482994717,15.2,2.56666298730075));
#258560=CARTESIAN_POINT('Ctrl Pts',(-11.1518229722595,15.2,2.56559211279311));
#258561=CARTESIAN_POINT('Ctrl Pts',(-11.1567076530547,15.2,2.56451122921546));
#258562=CARTESIAN_POINT('Ctrl Pts',(-11.1616022611003,15.2,2.56342029682165));
#258563=CARTESIAN_POINT('Ctrl Pts',(-11.1664968684789,15.2,2.56232936457648));
#258564=CARTESIAN_POINT('Ctrl Pts',(-11.171401405698,15.2,2.56122838669093));
#258565=CARTESIAN_POINT('Ctrl Pts',(-11.1763157775734,15.2,2.56011731561576));
#258566=CARTESIAN_POINT('Ctrl Pts',(-11.1812301501183,15.2,2.5590062443892));
#258567=CARTESIAN_POINT('Ctrl Pts',(-11.1861543535804,15.2,2.55788507840765));
#258568=CARTESIAN_POINT('Ctrl Pts',(-11.1910882907077,15.2,2.55675377134414));
#258569=CARTESIAN_POINT('Ctrl Pts',(-11.1947887432171,15.2,2.55590529112359));
#258570=CARTESIAN_POINT('Ctrl Pts',(-11.1984946707624,15.2,2.55505110767388));
#258571=CARTESIAN_POINT('Ctrl Pts',(-11.2022060574113,15.2,2.5541912121441));
#258572=CARTESIAN_POINT('Ctrl Pts',(-11.2059174440601,15.2,2.55333131661431));
#258573=CARTESIAN_POINT('Ctrl Pts',(-11.209634289429,15.2,2.55246571060184));
#258574=CARTESIAN_POINT('Ctrl Pts',(-11.2133565920001,15.2,2.55159438999998));
#258575=CARTESIAN_POINT('Ctrl Pts',(-10.0330625580001,12.2,2.64164356399998));
#258576=CARTESIAN_POINT('Ctrl Pts',(-10.03482302717,12.2,2.64194831044285));
#258577=CARTESIAN_POINT('Ctrl Pts',(-10.0366407484416,12.2,2.64225751971682));
#258578=CARTESIAN_POINT('Ctrl Pts',(-10.0385148615364,12.2,2.64257038294905));
#258579=CARTESIAN_POINT('Ctrl Pts',(-10.0403980125518,12.2,2.64288475496593));
#258580=CARTESIAN_POINT('Ctrl Pts',(-10.0423381038147,12.2,2.64320281628067));
#258581=CARTESIAN_POINT('Ctrl Pts',(-10.0443343061932,12.2,2.64352378181437));
#258582=CARTESIAN_POINT('Ctrl Pts',(-10.0463305083903,12.2,2.64384474731891));
#258583=CARTESIAN_POINT('Ctrl Pts',(-10.0483828189766,12.2,2.64416861768683));
#258584=CARTESIAN_POINT('Ctrl Pts',(-10.0504904282333,12.2,2.64449462925831));
#258585=CARTESIAN_POINT('Ctrl Pts',(-10.05259803749,12.2,2.6448206408298));
#258586=CARTESIAN_POINT('Ctrl Pts',(-10.0547609456752,12.2,2.64514879427203));
#258587=CARTESIAN_POINT('Ctrl Pts',(-10.0569783630356,12.2,2.6454783536931));
#258588=CARTESIAN_POINT('Ctrl Pts',(-10.0591957805974,12.2,2.64580791314411));
#258589=CARTESIAN_POINT('Ctrl Pts',(-10.0614677060147,12.2,2.64613887440968));
#258590=CARTESIAN_POINT('Ctrl Pts',(-10.0637933707285,12.2,2.64647052701114));
#258591=CARTESIAN_POINT('Ctrl Pts',(-10.066119035231,12.2,2.64680217958246));
#258592=CARTESIAN_POINT('Ctrl Pts',(-10.0684984395783,12.2,2.64713451980237));
#258593=CARTESIAN_POINT('Ctrl Pts',(-10.0709308320011,12.2,2.6474668565418));
#258594=CARTESIAN_POINT('Ctrl Pts',(-10.0733632244239,12.2,2.64779919328124));
#258595=CARTESIAN_POINT('Ctrl Pts',(-10.0758486046314,12.2,2.64813152376893));
#258596=CARTESIAN_POINT('Ctrl Pts',(-10.0783862401202,12.2,2.64846317850691));
#258597=CARTESIAN_POINT('Ctrl Pts',(-10.0809238758396,12.2,2.648794833275));
#258598=CARTESIAN_POINT('Ctrl Pts',(-10.0835137669738,12.2,2.64912580913471));
#258599=CARTESIAN_POINT('Ctrl Pts',(-10.0861551977879,12.2,2.64945545331925));
#258600=CARTESIAN_POINT('Ctrl Pts',(-10.0892368667112,12.2,2.64984003815631));
#258601=CARTESIAN_POINT('Ctrl Pts',(-10.0923886860307,12.2,2.65022281240024));
#258602=CARTESIAN_POINT('Ctrl Pts',(-10.0956095477997,12.2,2.6506027689739));
#258603=CARTESIAN_POINT('Ctrl Pts',(-10.0983702867813,12.2,2.65092844607506));
#258604=CARTESIAN_POINT('Ctrl Pts',(-10.1011817504025,12.2,2.65125205333433));
#258605=CARTESIAN_POINT('Ctrl Pts',(-10.1040432585619,12.2,2.6515729785183));
#258606=CARTESIAN_POINT('Ctrl Pts',(-10.1069047664613,12.2,2.65189390367312));
#258607=CARTESIAN_POINT('Ctrl Pts',(-10.109816319292,12.2,2.6522121451454));
#258608=CARTESIAN_POINT('Ctrl Pts',(-10.1127772501032,12.2,2.65252710930047));
#258609=CARTESIAN_POINT('Ctrl Pts',(-10.1157381809144,12.2,2.65284207345556));
#258610=CARTESIAN_POINT('Ctrl Pts',(-10.118748489905,12.2,2.65315375821922));
#258611=CARTESIAN_POINT('Ctrl Pts',(-10.1218075248751,12.2,2.6534615854582));
#258612=CARTESIAN_POINT('Ctrl Pts',(-10.1248665598452,12.2,2.65376941269718));
#258613=CARTESIAN_POINT('Ctrl Pts',(-10.1279743222156,12.2,2.65407338062792));
#258614=CARTESIAN_POINT('Ctrl Pts',(-10.131130171181,12.2,2.65437292795067));
#258615=CARTESIAN_POINT('Ctrl Pts',(-10.1342860204331,12.2,2.65467247530064));
#258616=CARTESIAN_POINT('Ctrl Pts',(-10.1374899582731,12.2,2.65496760035852));
#258617=CARTESIAN_POINT('Ctrl Pts',(-10.1407413577024,12.2,2.65525775479079));
#258618=CARTESIAN_POINT('Ctrl Pts',(-10.1439927568363,12.2,2.65554790919669));
#258619=CARTESIAN_POINT('Ctrl Pts',(-10.1472916205581,12.2,2.65583309476966));
#258620=CARTESIAN_POINT('Ctrl Pts',(-10.1506373326012,12.2,2.65611277450973));
#258621=CARTESIAN_POINT('Ctrl Pts',(-10.1539830446442,12.2,2.6563924542498));
#258622=CARTESIAN_POINT('Ctrl Pts',(-10.1573756074199,12.2,2.65666663162176));
#258623=CARTESIAN_POINT('Ctrl Pts',(-10.1608144186252,12.2,2.65693478419576));
#258624=CARTESIAN_POINT('Ctrl Pts',(-10.1642532301428,12.2,2.65720293679412));
#258625=CARTESIAN_POINT('Ctrl Pts',(-10.1677382903315,12.2,2.65746506659192));
#258626=CARTESIAN_POINT('Ctrl Pts',(-10.1712690116926,12.2,2.65772066535557));
#258627=CARTESIAN_POINT('Ctrl Pts',(-10.1747997327329,12.2,2.65797626409599));
#258628=CARTESIAN_POINT('Ctrl Pts',(-10.1783761121886,12.2,2.65822533255757));
#258629=CARTESIAN_POINT('Ctrl Pts',(-10.18199757349,12.2,2.65846738004989));
#258630=CARTESIAN_POINT('Ctrl Pts',(-10.1862226118943,12.2,2.65874976880558));
#258631=CARTESIAN_POINT('Ctrl Pts',(-10.1905090113944,12.2,2.6590225943752));
#258632=CARTESIAN_POINT('Ctrl Pts',(-10.1948558718532,12.2,2.6592851022539));
#258633=CARTESIAN_POINT('Ctrl Pts',(-10.1992027319736,12.2,2.65954761011216));
#258634=CARTESIAN_POINT('Ctrl Pts',(-10.203610053331,12.2,2.65979979572518));
#258635=CARTESIAN_POINT('Ctrl Pts',(-10.2080769531326,12.2,2.66004092325247));
#258636=CARTESIAN_POINT('Ctrl Pts',(-10.2119057248383,12.2,2.66024760401429));
#258637=CARTESIAN_POINT('Ctrl Pts',(-10.2157782698399,12.2,2.660446157467));
#258638=CARTESIAN_POINT('Ctrl Pts',(-10.2196940444719,12.2,2.66063613431031));
#258639=CARTESIAN_POINT('Ctrl Pts',(-10.2242624476756,12.2,2.66085777393497));
#258640=CARTESIAN_POINT('Ctrl Pts',(-10.228889688663,12.2,2.66106773679313));
#258641=CARTESIAN_POINT('Ctrl Pts',(-10.2335749198123,12.2,2.66126532344821));
#258642=CARTESIAN_POINT('Ctrl Pts',(-10.2369215136987,12.2,2.66140645678205));
#258643=CARTESIAN_POINT('Ctrl Pts',(-10.2402976952847,12.2,2.66154127628825));
#258644=CARTESIAN_POINT('Ctrl Pts',(-10.2437031600046,12.2,2.66166953302489));
#258645=CARTESIAN_POINT('Ctrl Pts',(-10.2471086247244,12.2,2.66179778976154));
#258646=CARTESIAN_POINT('Ctrl Pts',(-10.250543372977,12.2,2.66191948415265));
#258647=CARTESIAN_POINT('Ctrl Pts',(-10.2540071046063,12.2,2.66203437172831));
#258648=CARTESIAN_POINT('Ctrl Pts',(-10.2574708362357,12.2,2.66214925930396));
#258649=CARTESIAN_POINT('Ctrl Pts',(-10.2609635511991,12.2,2.66225733933743));
#258650=CARTESIAN_POINT('Ctrl Pts',(-10.2644849542532,12.2,2.66235837447669));
#258651=CARTESIAN_POINT('Ctrl Pts',(-10.2680063573072,12.2,2.66245940961594));
#258652=CARTESIAN_POINT('Ctrl Pts',(-10.2715564484343,12.2,2.66255339894946));
#258653=CARTESIAN_POINT('Ctrl Pts',(-10.2751349355161,12.2,2.66264010901929));
#258654=CARTESIAN_POINT('Ctrl Pts',(-10.278713422598,12.2,2.66272681908912));
#258655=CARTESIAN_POINT('Ctrl Pts',(-10.2823203051538,12.2,2.66280624829962));
#258656=CARTESIAN_POINT('Ctrl Pts',(-10.2859552964897,12.2,2.6628781685083));
#258657=CARTESIAN_POINT('Ctrl Pts',(-10.2895902878256,12.2,2.66295008871698));
#258658=CARTESIAN_POINT('Ctrl Pts',(-10.2932533863666,12.2,2.66301450025556));
#258659=CARTESIAN_POINT('Ctrl Pts',(-10.2969443094916,12.2,2.66307117699167));
#258660=CARTESIAN_POINT('Ctrl Pts',(-10.3006352326166,12.2,2.66312785372779));
#258661=CARTESIAN_POINT('Ctrl Pts',(-10.3043539787127,12.2,2.6631767950832));
#258662=CARTESIAN_POINT('Ctrl Pts',(-10.3081002692854,12.2,2.66321778195836));
#258663=CARTESIAN_POINT('Ctrl Pts',(-10.311846559858,12.2,2.66325876883353));
#258664=CARTESIAN_POINT('Ctrl Pts',(-10.3156203929251,12.2,2.66329180036868));
#258665=CARTESIAN_POINT('Ctrl Pts',(-10.3194214920237,12.2,2.66331665974325));
#258666=CARTESIAN_POINT('Ctrl Pts',(-10.3232225911224,12.2,2.66334151911782));
#258667=CARTESIAN_POINT('Ctrl Pts',(-10.3270509570675,12.2,2.66335820737315));
#258668=CARTESIAN_POINT('Ctrl Pts',(-10.330906315194,12.2,2.66336651098383));
#258669=CARTESIAN_POINT('Ctrl Pts',(-10.3347616733204,12.2,2.66337481459451));
#258670=CARTESIAN_POINT('Ctrl Pts',(-10.3386440226234,12.2,2.66337473393888));
#258671=CARTESIAN_POINT('Ctrl Pts',(-10.3425530959455,12.2,2.66336606171563));
#258672=CARTESIAN_POINT('Ctrl Pts',(-10.3464621692677,12.2,2.66335738949238));
#258673=CARTESIAN_POINT('Ctrl Pts',(-10.3503979631216,12.2,2.66334012386954));
#258674=CARTESIAN_POINT('Ctrl Pts',(-10.3543602129849,12.2,2.66331406247993));
#258675=CARTESIAN_POINT('Ctrl Pts',(-10.3583224628482,12.2,2.66328800109032));
#258676=CARTESIAN_POINT('Ctrl Pts',(-10.3623111670841,12.2,2.66325314366167));
#258677=CARTESIAN_POINT('Ctrl Pts',(-10.3663260620168,12.2,2.66320928824427));
#258678=CARTESIAN_POINT('Ctrl Pts',(-10.3703409569495,12.2,2.66316543282687));
#258679=CARTESIAN_POINT('Ctrl Pts',(-10.3743820438965,12.2,2.66311258126487));
#258680=CARTESIAN_POINT('Ctrl Pts',(-10.378449059732,12.2,2.66305053425022));
#258681=CARTESIAN_POINT('Ctrl Pts',(-10.3825160751241,12.2,2.66298848724234));
#258682=CARTESIAN_POINT('Ctrl Pts',(-10.3866090221234,12.2,2.66291724777322));
#258683=CARTESIAN_POINT('Ctrl Pts',(-10.3907276399363,12.2,2.66283662076889));
#258684=CARTESIAN_POINT('Ctrl Pts',(-10.3948462581981,12.2,2.66275599375577));
#258685=CARTESIAN_POINT('Ctrl Pts',(-10.3989905482511,12.2,2.66266598068448));
#258686=CARTESIAN_POINT('Ctrl Pts',(-10.4031602556796,12.2,2.6625663895047));
#258687=CARTESIAN_POINT('Ctrl Pts',(-10.4064960218042,12.2,2.66248671655653));
#258688=CARTESIAN_POINT('Ctrl Pts',(-10.4098480541839,12.2,2.66240091538874));
#258689=CARTESIAN_POINT('Ctrl Pts',(-10.413216224994,12.2,2.66230888971661));
#258690=CARTESIAN_POINT('Ctrl Pts',(-10.417426438277,12.2,2.66219385763273));
#258691=CARTESIAN_POINT('Ctrl Pts',(-10.4216618660052,12.2,2.66206910120277));
#258692=CARTESIAN_POINT('Ctrl Pts',(-10.4259222592704,12.2,2.66193443425781));
#258693=CARTESIAN_POINT('Ctrl Pts',(-10.429330573604,12.2,2.66182670071065));
#258694=CARTESIAN_POINT('Ctrl Pts',(-10.4327548650065,12.2,2.66171262592865));
#258695=CARTESIAN_POINT('Ctrl Pts',(-10.4361950074459,12.2,2.66159211699471));
#258696=CARTESIAN_POINT('Ctrl Pts',(-10.439635150354,12.2,2.66147160804435));
#258697=CARTESIAN_POINT('Ctrl Pts',(-10.443091144714,12.2,2.66134466509394));
#258698=CARTESIAN_POINT('Ctrl Pts',(-10.4465628642524,12.2,2.66121119747492));
#258699=CARTESIAN_POINT('Ctrl Pts',(-10.4500345833177,12.2,2.66107772987409));
#258700=CARTESIAN_POINT('Ctrl Pts',(-10.4535220267819,12.2,2.66093773750299));
#258701=CARTESIAN_POINT('Ctrl Pts',(-10.4570250711606,12.2,2.66079113001565));
#258702=CARTESIAN_POINT('Ctrl Pts',(-10.4605281160166,12.2,2.66064452250833));
#258703=CARTESIAN_POINT('Ctrl Pts',(-10.4640467619129,12.2,2.6604913010754));
#258704=CARTESIAN_POINT('Ctrl Pts',(-10.4675808842167,12.2,2.66033137673335));
#258705=CARTESIAN_POINT('Ctrl Pts',(-10.4711150065204,12.2,2.6601714523913));
#258706=CARTESIAN_POINT('Ctrl Pts',(-10.4746646061037,12.2,2.66000482464013));
#258707=CARTESIAN_POINT('Ctrl Pts',(-10.4782295602995,12.2,2.65983140646332));
#258708=CARTESIAN_POINT('Ctrl Pts',(-10.4817945140097,12.2,2.65965798831013));
#258709=CARTESIAN_POINT('Ctrl Pts',(-10.4853748226669,12.2,2.65947777970233));
#258710=CARTESIAN_POINT('Ctrl Pts',(-10.4889703632225,12.2,2.65929069671681));
#258711=CARTESIAN_POINT('Ctrl Pts',(-10.4934647892845,12.2,2.65905684296577));
#258712=CARTESIAN_POINT('Ctrl Pts',(-10.4979830183889,12.2,2.65881224421668));
#258713=CARTESIAN_POINT('Ctrl Pts',(-10.502524812,12.2,2.65855673650835));
#258714=CARTESIAN_POINT('Ctrl Pts',(-10.5061582470869,12.2,2.65835233033054));
#258715=CARTESIAN_POINT('Ctrl Pts',(-10.5098067662061,12.2,2.65814094404915));
#258716=CARTESIAN_POINT('Ctrl Pts',(-10.513470246574,12.2,2.65792249248096));
#258717=CARTESIAN_POINT('Ctrl Pts',(-10.5171337264427,12.2,2.65770404094254));
#258718=CARTESIAN_POINT('Ctrl Pts',(-10.5208121710743,12.2,2.65747852370163));
#258719=CARTESIAN_POINT('Ctrl Pts',(-10.5245054589558,12.2,2.65724586077517));
#258720=CARTESIAN_POINT('Ctrl Pts',(-10.5281987473405,12.2,2.65701319781701));
#258721=CARTESIAN_POINT('Ctrl Pts',(-10.5319068808099,12.2,2.65677338729882));
#258722=CARTESIAN_POINT('Ctrl Pts',(-10.5356297411254,12.2,2.65652635045129));
#258723=CARTESIAN_POINT('Ctrl Pts',(-10.5393526009336,12.2,2.65627931363741));
#258724=CARTESIAN_POINT('Ctrl Pts',(-10.54309018764,12.2,2.65602504855502));
#258725=CARTESIAN_POINT('Ctrl Pts',(-10.5468423854434,12.2,2.65576347702133));
#258726=CARTESIAN_POINT('Ctrl Pts',(-10.550594583758,12.2,2.65550190545199));
#258727=CARTESIAN_POINT('Ctrl Pts',(-10.5543613915386,12.2,2.65523302726716));
#258728=CARTESIAN_POINT('Ctrl Pts',(-10.5581426953238,12.2,2.65495676245988));
#258729=CARTESIAN_POINT('Ctrl Pts',(-10.5619239985937,12.2,2.65468049769025));
#258730=CARTESIAN_POINT('Ctrl Pts',(-10.5657197953511,12.2,2.65439684764667));
#258731=CARTESIAN_POINT('Ctrl Pts',(-10.5695299737053,12.2,2.65410573428208));
#258732=CARTESIAN_POINT('Ctrl Pts',(-10.5733401525787,12.2,2.65381462087781));
#258733=CARTESIAN_POINT('Ctrl Pts',(-10.5771647104288,12.2,2.65351604401432));
#258734=CARTESIAN_POINT('Ctrl Pts',(-10.5810035348056,12.2,2.65320992844158));
#258735=CARTESIAN_POINT('Ctrl Pts',(-10.5848423586594,12.2,2.65290381291056));
#258736=CARTESIAN_POINT('Ctrl Pts',(-10.5886954486575,12.2,2.65259015798294));
#258737=CARTESIAN_POINT('Ctrl Pts',(-10.5925626914223,12.2,2.65226888727159));
#258738=CARTESIAN_POINT('Ctrl Pts',(-10.5973967452733,12.2,2.65186729884958));
#258739=CARTESIAN_POINT('Ctrl Pts',(-10.6022529151322,12.2,2.65145381360492));
#258740=CARTESIAN_POINT('Ctrl Pts',(-10.6071309772144,12.2,2.65102828374444));
#258741=CARTESIAN_POINT('Ctrl Pts',(-10.6110334270929,12.2,2.65068785983749));
#258742=CARTESIAN_POINT('Ctrl Pts',(-10.6149498913674,12.2,2.65033972961297));
#258743=CARTESIAN_POINT('Ctrl Pts',(-10.6188802558048,12.2,2.64998381870418));
#258744=CARTESIAN_POINT('Ctrl Pts',(-10.6228106197066,12.2,2.64962790784388));
#258745=CARTESIAN_POINT('Ctrl Pts',(-10.6267548853194,12.2,2.64926421491916));
#258746=CARTESIAN_POINT('Ctrl Pts',(-10.6307129431924,12.2,2.64889267082055));
#258747=CARTESIAN_POINT('Ctrl Pts',(-10.6346710016047,12.2,2.64852112667131));
#258748=CARTESIAN_POINT('Ctrl Pts',(-10.638642849069,12.2,2.64814172973713));
#258749=CARTESIAN_POINT('Ctrl Pts',(-10.6426283788426,12.2,2.64775440899328));
#258750=CARTESIAN_POINT('Ctrl Pts',(-10.6466139080733,12.2,2.6473670883022));
#258751=CARTESIAN_POINT('Ctrl Pts',(-10.6506131188344,12.2,2.64697184454883));
#258752=CARTESIAN_POINT('Ctrl Pts',(-10.6546259013939,12.2,2.64656860658261));
#258753=CARTESIAN_POINT('Ctrl Pts',(-10.6586386845001,12.2,2.64616536856145));
#258754=CARTESIAN_POINT('Ctrl Pts',(-10.6626650414104,12.2,2.64575413726732));
#258755=CARTESIAN_POINT('Ctrl Pts',(-10.6667048612417,12.2,2.64533484380002));
#258756=CARTESIAN_POINT('Ctrl Pts',(-10.670744681073,12.2,2.64491555033272));
#258757=CARTESIAN_POINT('Ctrl Pts',(-10.6747979656919,12.2,2.64448819331727));
#258758=CARTESIAN_POINT('Ctrl Pts',(-10.6788646069149,12.2,2.64405270590381));
#258759=CARTESIAN_POINT('Ctrl Pts',(-10.6829312475838,12.2,2.64361721854969));
#258760=CARTESIAN_POINT('Ctrl Pts',(-10.6870112457855,12.2,2.64317360013207));
#258761=CARTESIAN_POINT('Ctrl Pts',(-10.6911044942472,12.2,2.64272178350032));
#258762=CARTESIAN_POINT('Ctrl Pts',(-10.6951977432666,12.2,2.64226996680701));
#258763=CARTESIAN_POINT('Ctrl Pts',(-10.6993042410894,12.2,2.64180995286649));
#258764=CARTESIAN_POINT('Ctrl Pts',(-10.7034238841486,12.2,2.64134167417345));
#258765=CARTESIAN_POINT('Ctrl Pts',(-10.7075435266465,12.2,2.64087339554422));
#258766=CARTESIAN_POINT('Ctrl Pts',(-10.7116763128343,12.2,2.64039685306885));
#258767=CARTESIAN_POINT('Ctrl Pts',(-10.7158221381612,12.2,2.63991197983125));
#258768=CARTESIAN_POINT('Ctrl Pts',(-10.7210044202435,12.2,2.6393058882347));
#258769=CARTESIAN_POINT('Ctrl Pts',(-10.7262070767291,12.2,2.6386867820032));
#258770=CARTESIAN_POINT('Ctrl Pts',(-10.7314299020305,12.2,2.63805453450036));
#258771=CARTESIAN_POINT('Ctrl Pts',(-10.7356081624994,12.2,2.63754873647052));
#258772=CARTESIAN_POINT('Ctrl Pts',(-10.7397993304653,12.2,2.63703452839668));
#258773=CARTESIAN_POINT('Ctrl Pts',(-10.7440033041957,12.2,2.63651184642289));
#258774=CARTESIAN_POINT('Ctrl Pts',(-10.7482072773534,12.2,2.6359891645203));
#258775=CARTESIAN_POINT('Ctrl Pts',(-10.7524240547621,12.2,2.63545800747438));
#258776=CARTESIAN_POINT('Ctrl Pts',(-10.7566535346377,12.2,2.63491831601906));
#258777=CARTESIAN_POINT('Ctrl Pts',(-10.7608830150896,12.2,2.63437862449021));
#258778=CARTESIAN_POINT('Ctrl Pts',(-10.7651251963219,12.2,2.63383039630031));
#258779=CARTESIAN_POINT('Ctrl Pts',(-10.7693799771008,12.2,2.63327356968584));
#258780=CARTESIAN_POINT('Ctrl Pts',(-10.7736347573,12.2,2.63271674314724));
#258781=CARTESIAN_POINT('Ctrl Pts',(-10.7779021379148,12.2,2.63215131836604));
#258782=CARTESIAN_POINT('Ctrl Pts',(-10.7821820151752,12.2,2.6315772350802));
#258783=CARTESIAN_POINT('Ctrl Pts',(-10.7864618930188,12.2,2.63100315171615));
#258784=CARTESIAN_POINT('Ctrl Pts',(-10.79075426925,12.2,2.63042040926217));
#258785=CARTESIAN_POINT('Ctrl Pts',(-10.795059041152,12.2,2.62982894845158));
#258786=CARTESIAN_POINT('Ctrl Pts',(-10.7993638124676,12.2,2.62923748772159));
#258787=CARTESIAN_POINT('Ctrl Pts',(-10.8036809803244,12.2,2.62863730645432));
#258788=CARTESIAN_POINT('Ctrl Pts',(-10.8080104451302,12.2,2.62802834786334));
#258789=CARTESIAN_POINT('Ctrl Pts',(-10.8123399105258,12.2,2.62741938918938));
#258790=CARTESIAN_POINT('Ctrl Pts',(-10.8166816714485,12.2,2.62680165148344));
#258791=CARTESIAN_POINT('Ctrl Pts',(-10.8210356286311,12.2,2.62617507744871));
#258792=CARTESIAN_POINT('Ctrl Pts',(-10.8253895852204,12.2,2.62554850349936));
#258793=CARTESIAN_POINT('Ctrl Pts',(-10.8297557382045,12.2,2.62491309212122));
#258794=CARTESIAN_POINT('Ctrl Pts',(-10.8341339887342,12.2,2.62426878689703));
#258795=CARTESIAN_POINT('Ctrl Pts',(-10.8385122398604,12.2,2.62362448158504));
#258796=CARTESIAN_POINT('Ctrl Pts',(-10.8429025879486,12.2,2.62297128163036));
#258797=CARTESIAN_POINT('Ctrl Pts',(-10.8473049339863,12.2,2.6223091297579));
#258798=CARTESIAN_POINT('Ctrl Pts',(-10.8517072794243,12.2,2.62164697797566));
#258799=CARTESIAN_POINT('Ctrl Pts',(-10.8561216243894,12.2,2.62097587577692));
#258800=CARTESIAN_POINT('Ctrl Pts',(-10.8605478690263,12.2,2.62029576461122));
#258801=CARTESIAN_POINT('Ctrl Pts',(-10.8638675532579,12.2,2.61978568112111));
#258802=CARTESIAN_POINT('Ctrl Pts',(-10.867193932208,12.2,2.6192705312129));
#258803=CARTESIAN_POINT('Ctrl Pts',(-10.870526963485,12.2,2.61875029117827));
#258804=CARTESIAN_POINT('Ctrl Pts',(-10.8738599941564,12.2,2.61823005123815));
#258805=CARTESIAN_POINT('Ctrl Pts',(-10.8771996784692,12.2,2.61770472058996));
#258806=CARTESIAN_POINT('Ctrl Pts',(-10.8805459741399,12.2,2.61717427669212));
#258807=CARTESIAN_POINT('Ctrl Pts',(-10.8838922698105,12.2,2.61664383279428));
#258808=CARTESIAN_POINT('Ctrl Pts',(-10.8872451778432,12.2,2.61610827563236));
#258809=CARTESIAN_POINT('Ctrl Pts',(-10.8906046570281,12.2,2.61556758177453));
#258810=CARTESIAN_POINT('Ctrl Pts',(-10.893964136213,12.2,2.61502688791669));
#258811=CARTESIAN_POINT('Ctrl Pts',(-10.8973301875375,12.2,2.61448105781631));
#258812=CARTESIAN_POINT('Ctrl Pts',(-10.9007027682636,12.2,2.61393006845885));
#258813=CARTESIAN_POINT('Ctrl Pts',(-10.9040753489897,12.2,2.61337907910139));
#258814=CARTESIAN_POINT('Ctrl Pts',(-10.9074544607047,12.2,2.6128229312236));
#258815=CARTESIAN_POINT('Ctrl Pts',(-10.9108400623728,12.2,2.61226160132779));
#258816=CARTESIAN_POINT('Ctrl Pts',(-10.9142256640408,12.2,2.61170027143197));
#258817=CARTESIAN_POINT('Ctrl Pts',(-10.9176177555835,12.2,2.61113375971984));
#258818=CARTESIAN_POINT('Ctrl Pts',(-10.9210162977091,12.2,2.61056204386632));
#258819=CARTESIAN_POINT('Ctrl Pts',(-10.9244148404522,12.2,2.60999032790894));
#258820=CARTESIAN_POINT('Ctrl Pts',(-10.9278198335137,12.2,2.60941340837509));
#258821=CARTESIAN_POINT('Ctrl Pts',(-10.9312312362187,12.2,2.60883126287311));
#258822=CARTESIAN_POINT('Ctrl Pts',(-10.9346426383039,12.2,2.60824911747688));
#258823=CARTESIAN_POINT('Ctrl Pts',(-10.9380604499318,12.2,2.60766174579399));
#258824=CARTESIAN_POINT('Ctrl Pts',(-10.9414846321876,12.2,2.60706912636864));
#258825=CARTESIAN_POINT('Ctrl Pts',(-10.9449088144433,12.2,2.60647650694329));
#258826=CARTESIAN_POINT('Ctrl Pts',(-10.948339365949,12.2,2.60587863986274));
#258827=CARTESIAN_POINT('Ctrl Pts',(-10.9517762486164,12.2,2.60527550346752));
#258828=CARTESIAN_POINT('Ctrl Pts',(-10.9552131312838,12.2,2.60467236707231));
#258829=CARTESIAN_POINT('Ctrl Pts',(-10.9586563445253,12.2,2.60406396109439));
#258830=CARTESIAN_POINT('Ctrl Pts',(-10.96210584815,12.2,2.60345026424169));
#258831=CARTESIAN_POINT('Ctrl Pts',(-10.9655553517747,12.2,2.60283656738899));
#258832=CARTESIAN_POINT('Ctrl Pts',(-10.9690111455824,12.2,2.6022175800115));
#258833=CARTESIAN_POINT('Ctrl Pts',(-10.9724731916228,12.2,2.60159328057632));
#258834=CARTESIAN_POINT('Ctrl Pts',(-10.9759352376631,12.2,2.60096898114113));
#258835=CARTESIAN_POINT('Ctrl Pts',(-10.9794035345646,12.2,2.60033936826418));
#258836=CARTESIAN_POINT('Ctrl Pts',(-10.9828780448195,12.2,2.59970442338115));
#258837=CARTESIAN_POINT('Ctrl Pts',(-10.9863525550745,12.2,2.59906947849812));
#258838=CARTESIAN_POINT('Ctrl Pts',(-10.9898332773007,12.2,2.59842920144991));
#258839=CARTESIAN_POINT('Ctrl Pts',(-10.9933201720065,12.2,2.5977835700991));
#258840=CARTESIAN_POINT('Ctrl Pts',(-10.9968070673458,12.2,2.597137938631));
#258841=CARTESIAN_POINT('Ctrl Pts',(-11.0003001364035,12.2,2.59648695288639));
#258842=CARTESIAN_POINT('Ctrl Pts',(-11.0037993392462,12.2,2.59583059333193));
#258843=CARTESIAN_POINT('Ctrl Pts',(-11.0072985414532,12.2,2.59517423389671));
#258844=CARTESIAN_POINT('Ctrl Pts',(-11.0108038780099,12.2,2.59451249955344));
#258845=CARTESIAN_POINT('Ctrl Pts',(-11.0143153105912,12.2,2.59384537070222));
#258846=CARTESIAN_POINT('Ctrl Pts',(-11.0178267431725,12.2,2.59317824185099));
#258847=CARTESIAN_POINT('Ctrl Pts',(-11.021344269878,12.2,2.59250571860873));
#258848=CARTESIAN_POINT('Ctrl Pts',(-11.0248678549583,12.2,2.59182778071669));
#258849=CARTESIAN_POINT('Ctrl Pts',(-11.0283914400387,12.2,2.59114984282466));
#258850=CARTESIAN_POINT('Ctrl Pts',(-11.0319210824604,12.2,2.59046648918284));
#258851=CARTESIAN_POINT('Ctrl Pts',(-11.0354567426231,12.2,2.58977770133334));
#258852=CARTESIAN_POINT('Ctrl Pts',(-11.0389924027857,12.2,2.58908891348384));
#258853=CARTESIAN_POINT('Ctrl Pts',(-11.0425340814994,12.2,2.58839469094423));
#258854=CARTESIAN_POINT('Ctrl Pts',(-11.0460817408387,12.2,2.58769501356034));
#258855=CARTESIAN_POINT('Ctrl Pts',(-11.049629400178,12.2,2.58699533617644));
#258856=CARTESIAN_POINT('Ctrl Pts',(-11.0531830398208,12.2,2.5862902041117));
#258857=CARTESIAN_POINT('Ctrl Pts',(-11.0567426214824,12.2,2.58557959867993));
#258858=CARTESIAN_POINT('Ctrl Pts',(-11.0614887307955,12.2,2.58463212468484));
#258859=CARTESIAN_POINT('Ctrl Pts',(-11.0662454040624,12.2,2.58367491720828));
#258860=CARTESIAN_POINT('Ctrl Pts',(-11.0710125507667,12.2,2.58270793326669));
#258861=CARTESIAN_POINT('Ctrl Pts',(-11.0745879104701,12.2,2.58198269537637));
#258862=CARTESIAN_POINT('Ctrl Pts',(-11.0781691622066,12.2,2.58125195745296));
#258863=CARTESIAN_POINT('Ctrl Pts',(-11.0817562679091,12.2,2.58051570110518));
#258864=CARTESIAN_POINT('Ctrl Pts',(-11.0853433736116,12.2,2.57977944475741));
#258865=CARTESIAN_POINT('Ctrl Pts',(-11.0889363336721,12.2,2.57903766972076));
#258866=CARTESIAN_POINT('Ctrl Pts',(-11.0925351095538,12.2,2.57829035591956));
#258867=CARTESIAN_POINT('Ctrl Pts',(-11.0961338854355,12.2,2.57754304211835));
#258868=CARTESIAN_POINT('Ctrl Pts',(-11.0997384767949,12.2,2.57679019042038));
#258869=CARTESIAN_POINT('Ctrl Pts',(-11.1033488474546,12.2,2.57603178215702));
#258870=CARTESIAN_POINT('Ctrl Pts',(-11.1069592187702,12.2,2.57527337375588));
#258871=CARTESIAN_POINT('Ctrl Pts',(-11.1105753692291,12.2,2.57450940866153));
#258872=CARTESIAN_POINT('Ctrl Pts',(-11.1141972605479,12.2,2.57373986825726));
#258873=CARTESIAN_POINT('Ctrl Pts',(-11.1178191512088,12.2,2.57297032799279));
#258874=CARTESIAN_POINT('Ctrl Pts',(-11.1214467828943,12.2,2.57219521320362));
#258875=CARTESIAN_POINT('Ctrl Pts',(-11.1250801209295,12.2,2.57141450489817));
#258876=CARTESIAN_POINT('Ctrl Pts',(-11.1287134589646,12.2,2.57063379659272));
#258877=CARTESIAN_POINT('Ctrl Pts',(-11.1323525006858,12.2,2.56984749530749));
#258878=CARTESIAN_POINT('Ctrl Pts',(-11.1359972102783,12.2,2.56905558195764));
#258879=CARTESIAN_POINT('Ctrl Pts',(-11.1396419198708,12.2,2.56826366860779));
#258880=CARTESIAN_POINT('Ctrl Pts',(-11.1432922952129,12.2,2.56746614310853));
#258881=CARTESIAN_POINT('Ctrl Pts',(-11.1469482994717,12.2,2.56666298730075));
#258882=CARTESIAN_POINT('Ctrl Pts',(-11.1506043037305,12.2,2.56585983149297));
#258883=CARTESIAN_POINT('Ctrl Pts',(-11.1542659373508,12.2,2.56505104560862));
#258884=CARTESIAN_POINT('Ctrl Pts',(-11.1579331665504,12.2,2.56423661284704));
#258885=CARTESIAN_POINT('Ctrl Pts',(-11.1628228059273,12.2,2.56315070239962));
#258886=CARTESIAN_POINT('Ctrl Pts',(-11.1677223945472,12.2,2.562054754176));
#258887=CARTESIAN_POINT('Ctrl Pts',(-11.1726318444265,12.2,2.56094872689285));
#258888=CARTESIAN_POINT('Ctrl Pts',(-11.1775412936369,12.2,2.55984269976039));
#258889=CARTESIAN_POINT('Ctrl Pts',(-11.1824606008646,12.2,2.55872659110727));
#258890=CARTESIAN_POINT('Ctrl Pts',(-11.1873896638182,12.2,2.55760035142173));
#258891=CARTESIAN_POINT('Ctrl Pts',(-11.1910864612012,12.2,2.55675567161921));
#258892=CARTESIAN_POINT('Ctrl Pts',(-11.1947887447772,12.2,2.55590529305476));
#258893=CARTESIAN_POINT('Ctrl Pts',(-11.1984964899334,12.2,2.55504920446165));
#258894=CARTESIAN_POINT('Ctrl Pts',(-11.2034401505907,12.2,2.55390775290048));
#258895=CARTESIAN_POINT('Ctrl Pts',(-11.2083935214545,12.2,2.55275615090798));
#258896=CARTESIAN_POINT('Ctrl Pts',(-11.2133565920001,12.2,2.55159438999998));
#258897=CARTESIAN_POINT('Origin',(-5.66257110645729E-14,15.2,-1.77635683940025E-14));
#258898=CARTESIAN_POINT('',(-10.3068855240001,15.2,1.18690176599999));
#258899=CARTESIAN_POINT('',(-10.3068855240001,12.2,1.18690176599999));
#258900=CARTESIAN_POINT('',(-10.3068855240001,15.2,1.18690176599999));
#258901=CARTESIAN_POINT('Origin',(-5.66257110645729E-14,12.2,-1.77635683940025E-14));
#258902=CARTESIAN_POINT('Origin',(-5.66257110645729E-14,15.2,-1.77635683940025E-14));
#258903=CARTESIAN_POINT('Origin',(-5.66257110645729E-14,15.2,-1.77635683940025E-14));
#258904=CARTESIAN_POINT('',(-11.4623505340001,15.2,0.929795807999985));
#258905=CARTESIAN_POINT('',(-11.4869855320001,15.2,0.546958305999983));
#258906=CARTESIAN_POINT('Origin',(-5.66257110645729E-14,15.2,-1.77635683940025E-14));
#258907=CARTESIAN_POINT('',(-11.4869855320001,12.2,0.546958305999983));
#258908=CARTESIAN_POINT('',(-11.4869855320001,15.2,0.546958305999983));
#258909=CARTESIAN_POINT('',(-11.4623505340001,12.2,0.929795807999985));
#258910=CARTESIAN_POINT('Origin',(-5.66257110645729E-14,12.2,-1.77635683940025E-14));
#258911=CARTESIAN_POINT('',(-11.4623505340001,15.2,0.929795807999985));
#258912=CARTESIAN_POINT('Ctrl Pts',(-10.3068855240001,15.2,1.18690176599999));
#258913=CARTESIAN_POINT('Ctrl Pts',(-10.3068855240001,11.6,1.18690176599999));
#258914=CARTESIAN_POINT('Ctrl Pts',(-10.3070598110001,15.2,1.18690675299999));
#258915=CARTESIAN_POINT('Ctrl Pts',(-10.3070598110001,11.6,1.18690675299999));
#258916=CARTESIAN_POINT('Ctrl Pts',(-10.3074144740001,15.2,1.18691681599998));
#258917=CARTESIAN_POINT('Ctrl Pts',(-10.3074144740001,11.6,1.18691681599998));
#258918=CARTESIAN_POINT('Ctrl Pts',(-10.3079518810001,15.2,1.18693179799998));
#258919=CARTESIAN_POINT('Ctrl Pts',(-10.3079518810001,11.6,1.18693179799998));
#258920=CARTESIAN_POINT('Ctrl Pts',(-10.3086758300001,15.2,1.18695143999998));
#258921=CARTESIAN_POINT('Ctrl Pts',(-10.3086758300001,11.6,1.18695143999998));
#258922=CARTESIAN_POINT('Ctrl Pts',(-10.3095915440001,15.2,1.18697537099999));
#258923=CARTESIAN_POINT('Ctrl Pts',(-10.3095915440001,11.6,1.18697537099999));
#258924=CARTESIAN_POINT('Ctrl Pts',(-10.3105221240001,15.2,1.18699875499999));
#258925=CARTESIAN_POINT('Ctrl Pts',(-10.3105221240001,11.6,1.18699875499999));
#258926=CARTESIAN_POINT('Ctrl Pts',(-10.3114622390001,15.2,1.18702143499998));
#258927=CARTESIAN_POINT('Ctrl Pts',(-10.3114622390001,11.6,1.18702143499998));
#258928=CARTESIAN_POINT('Ctrl Pts',(-10.3124118610001,15.2,1.18704339399998));
#258929=CARTESIAN_POINT('Ctrl Pts',(-10.3124118610001,11.6,1.18704339399998));
#258930=CARTESIAN_POINT('Ctrl Pts',(-10.3133709660001,15.2,1.18706460899999));
#258931=CARTESIAN_POINT('Ctrl Pts',(-10.3133709660001,11.6,1.18706460899999));
#258932=CARTESIAN_POINT('Ctrl Pts',(-10.3143395250001,15.2,1.18708506599999));
#258933=CARTESIAN_POINT('Ctrl Pts',(-10.3143395250001,11.6,1.18708506599999));
#258934=CARTESIAN_POINT('Ctrl Pts',(-10.3153175130001,15.2,1.18710474299998));
#258935=CARTESIAN_POINT('Ctrl Pts',(-10.3153175130001,11.6,1.18710474299998));
#258936=CARTESIAN_POINT('Ctrl Pts',(-10.3163049050001,15.2,1.18712362399998));
#258937=CARTESIAN_POINT('Ctrl Pts',(-10.3163049050001,11.6,1.18712362399998));
#258938=CARTESIAN_POINT('Ctrl Pts',(-10.3173016730001,15.2,1.18714168899999));
#258939=CARTESIAN_POINT('Ctrl Pts',(-10.3173016730001,11.6,1.18714168899999));
#258940=CARTESIAN_POINT('Ctrl Pts',(-10.3183077930001,15.2,1.18715892099999));
#258941=CARTESIAN_POINT('Ctrl Pts',(-10.3183077930001,11.6,1.18715892099999));
#258942=CARTESIAN_POINT('Ctrl Pts',(-10.3193232400001,15.2,1.18717530199998));
#258943=CARTESIAN_POINT('Ctrl Pts',(-10.3193232400001,11.6,1.18717530199998));
#258944=CARTESIAN_POINT('Ctrl Pts',(-10.3203479850001,15.2,1.18719081299998));
#258945=CARTESIAN_POINT('Ctrl Pts',(-10.3203479850001,11.6,1.18719081299998));
#258946=CARTESIAN_POINT('Ctrl Pts',(-10.3213820050001,15.2,1.18720543699999));
#258947=CARTESIAN_POINT('Ctrl Pts',(-10.3213820050001,11.6,1.18720543699998));
#258948=CARTESIAN_POINT('Ctrl Pts',(-10.3224252740001,15.2,1.18721915599998));
#258949=CARTESIAN_POINT('Ctrl Pts',(-10.3224252740001,11.6,1.18721915599998));
#258950=CARTESIAN_POINT('Ctrl Pts',(-10.3234777680001,15.2,1.18723195099999));
#258951=CARTESIAN_POINT('Ctrl Pts',(-10.3234777680001,11.6,1.18723195099998));
#258952=CARTESIAN_POINT('Ctrl Pts',(-10.3245394590001,15.2,1.18724380599998));
#258953=CARTESIAN_POINT('Ctrl Pts',(-10.3245394590001,11.6,1.18724380599998));
#258954=CARTESIAN_POINT('Ctrl Pts',(-10.3256103250001,15.2,1.18725470399998));
#258955=CARTESIAN_POINT('Ctrl Pts',(-10.3256103250001,11.6,1.18725470399998));
#258956=CARTESIAN_POINT('Ctrl Pts',(-10.3266903400001,15.2,1.18726462499998));
#258957=CARTESIAN_POINT('Ctrl Pts',(-10.3266903400001,11.6,1.18726462499998));
#258958=CARTESIAN_POINT('Ctrl Pts',(-10.3277794780001,15.2,1.18727355499999));
#258959=CARTESIAN_POINT('Ctrl Pts',(-10.3277794780001,11.6,1.18727355499999));
#258960=CARTESIAN_POINT('Ctrl Pts',(-10.3288777160001,15.2,1.18728147399999));
#258961=CARTESIAN_POINT('Ctrl Pts',(-10.3288777160001,11.6,1.18728147399999));
#258962=CARTESIAN_POINT('Ctrl Pts',(-10.3299850290001,15.2,1.18728836599999));
#258963=CARTESIAN_POINT('Ctrl Pts',(-10.3299850290001,11.6,1.18728836599999));
#258964=CARTESIAN_POINT('Ctrl Pts',(-10.3311013920001,15.2,1.18729421399999));
#258965=CARTESIAN_POINT('Ctrl Pts',(-10.3311013920001,11.6,1.18729421399998));
#258966=CARTESIAN_POINT('Ctrl Pts',(-10.3322267810001,15.2,1.18729900199999));
#258967=CARTESIAN_POINT('Ctrl Pts',(-10.3322267810001,11.6,1.18729900199999));
#258968=CARTESIAN_POINT('Ctrl Pts',(-10.3333611710001,15.2,1.18730271099999));
#258969=CARTESIAN_POINT('Ctrl Pts',(-10.3333611710001,11.6,1.18730271099999));
#258970=CARTESIAN_POINT('Ctrl Pts',(-10.3345045400001,15.2,1.18730532599999));
#258971=CARTESIAN_POINT('Ctrl Pts',(-10.3345045400001,11.6,1.18730532599999));
#258972=CARTESIAN_POINT('Ctrl Pts',(-10.3356568620001,15.2,1.18730682999999));
#258973=CARTESIAN_POINT('Ctrl Pts',(-10.3356568620001,11.6,1.18730682999999));
#258974=CARTESIAN_POINT('Ctrl Pts',(-10.3368181130001,15.2,1.18730720599999));
#258975=CARTESIAN_POINT('Ctrl Pts',(-10.3368181130001,11.6,1.18730720599999));
#258976=CARTESIAN_POINT('Ctrl Pts',(-10.3379882700001,15.2,1.18730643699998));
#258977=CARTESIAN_POINT('Ctrl Pts',(-10.3379882700001,11.6,1.18730643699998));
#258978=CARTESIAN_POINT('Ctrl Pts',(-10.3391673090001,15.2,1.18730450799998));
#258979=CARTESIAN_POINT('Ctrl Pts',(-10.3391673090001,11.6,1.18730450799998));
#258980=CARTESIAN_POINT('Ctrl Pts',(-10.3403552060001,15.2,1.18730140199999));
#258981=CARTESIAN_POINT('Ctrl Pts',(-10.3403552060001,11.6,1.18730140199998));
#258982=CARTESIAN_POINT('Ctrl Pts',(-10.3415519380001,15.2,1.18729710199998));
#258983=CARTESIAN_POINT('Ctrl Pts',(-10.3415519380001,11.6,1.18729710199998));
#258984=CARTESIAN_POINT('Ctrl Pts',(-10.3427574820001,15.2,1.18729159399999));
#258985=CARTESIAN_POINT('Ctrl Pts',(-10.3427574820001,11.6,1.18729159399999));
#258986=CARTESIAN_POINT('Ctrl Pts',(-10.3439718130001,15.2,1.18728485899998));
#258987=CARTESIAN_POINT('Ctrl Pts',(-10.3439718130001,11.6,1.18728485899998));
#258988=CARTESIAN_POINT('Ctrl Pts',(-10.3451949090001,15.2,1.18727688299999));
#258989=CARTESIAN_POINT('Ctrl Pts',(-10.3451949090001,11.6,1.18727688299999));
#258990=CARTESIAN_POINT('Ctrl Pts',(-10.3464267470001,15.2,1.18726764999999));
#258991=CARTESIAN_POINT('Ctrl Pts',(-10.3464267470001,11.6,1.18726764999999));
#258992=CARTESIAN_POINT('Ctrl Pts',(-10.3476673040001,15.2,1.18725714299998));
#258993=CARTESIAN_POINT('Ctrl Pts',(-10.3476673040001,11.6,1.18725714299998));
#258994=CARTESIAN_POINT('Ctrl Pts',(-10.3489165560001,15.2,1.18724534699998));
#258995=CARTESIAN_POINT('Ctrl Pts',(-10.3489165560001,11.6,1.18724534699998));
#258996=CARTESIAN_POINT('Ctrl Pts',(-10.3501744810001,15.2,1.18723224699998));
#258997=CARTESIAN_POINT('Ctrl Pts',(-10.3501744810001,11.6,1.18723224699998));
#258998=CARTESIAN_POINT('Ctrl Pts',(-10.3514410560001,15.2,1.18721782799998));
#258999=CARTESIAN_POINT('Ctrl Pts',(-10.3514410560001,11.6,1.18721782799998));
#259000=CARTESIAN_POINT('Ctrl Pts',(-10.3527162580001,15.2,1.18720207199999));
#259001=CARTESIAN_POINT('Ctrl Pts',(-10.3527162580001,11.6,1.18720207199999));
#259002=CARTESIAN_POINT('Ctrl Pts',(-10.3540000650001,15.2,1.18718496499998));
#259003=CARTESIAN_POINT('Ctrl Pts',(-10.3540000650001,11.6,1.18718496499998));
#259004=CARTESIAN_POINT('Ctrl Pts',(-10.3552924550001,15.2,1.18716649199999));
#259005=CARTESIAN_POINT('Ctrl Pts',(-10.3552924550001,11.6,1.18716649199999));
#259006=CARTESIAN_POINT('Ctrl Pts',(-10.3565934040001,15.2,1.18714663699999));
#259007=CARTESIAN_POINT('Ctrl Pts',(-10.3565934040001,11.6,1.18714663699999));
#259008=CARTESIAN_POINT('Ctrl Pts',(-10.3579028900001,15.2,1.18712538499999));
#259009=CARTESIAN_POINT('Ctrl Pts',(-10.3579028900001,11.6,1.18712538499999));
#259010=CARTESIAN_POINT('Ctrl Pts',(-10.3592208920001,15.2,1.18710272199999));
#259011=CARTESIAN_POINT('Ctrl Pts',(-10.3592208920001,11.6,1.18710272199999));
#259012=CARTESIAN_POINT('Ctrl Pts',(-10.3605473870001,15.2,1.18707863099999));
#259013=CARTESIAN_POINT('Ctrl Pts',(-10.3605473870001,11.6,1.18707863099999));
#259014=CARTESIAN_POINT('Ctrl Pts',(-10.3618823540001,15.2,1.18705309899998));
#259015=CARTESIAN_POINT('Ctrl Pts',(-10.3618823540001,11.6,1.18705309899998));
#259016=CARTESIAN_POINT('Ctrl Pts',(-10.3632257690001,15.2,1.18702610999998));
#259017=CARTESIAN_POINT('Ctrl Pts',(-10.3632257690001,11.6,1.18702610999998));
#259018=CARTESIAN_POINT('Ctrl Pts',(-10.3645776120001,15.2,1.18699765099999));
#259019=CARTESIAN_POINT('Ctrl Pts',(-10.3645776120001,11.6,1.18699765099999));
#259020=CARTESIAN_POINT('Ctrl Pts',(-10.3659378610001,15.2,1.18696770399998));
#259021=CARTESIAN_POINT('Ctrl Pts',(-10.3659378610001,11.6,1.18696770399998));
#259022=CARTESIAN_POINT('Ctrl Pts',(-10.3673064940001,15.2,1.18693625599999));
#259023=CARTESIAN_POINT('Ctrl Pts',(-10.3673064940001,11.6,1.18693625599999));
#259024=CARTESIAN_POINT('Ctrl Pts',(-10.3686834880001,15.2,1.18690329399998));
#259025=CARTESIAN_POINT('Ctrl Pts',(-10.3686834880001,11.6,1.18690329399998));
#259026=CARTESIAN_POINT('Ctrl Pts',(-10.3700688240001,15.2,1.18686880099999));
#259027=CARTESIAN_POINT('Ctrl Pts',(-10.3700688240001,11.6,1.18686880099998));
#259028=CARTESIAN_POINT('Ctrl Pts',(-10.3714624790001,15.2,1.18683276399999));
#259029=CARTESIAN_POINT('Ctrl Pts',(-10.3714624790001,11.6,1.18683276399999));
#259030=CARTESIAN_POINT('Ctrl Pts',(-10.3728644310001,15.2,1.18679516799999));
#259031=CARTESIAN_POINT('Ctrl Pts',(-10.3728644310001,11.6,1.18679516799999));
#259032=CARTESIAN_POINT('Ctrl Pts',(-10.3742746610001,15.2,1.18675599899999));
#259033=CARTESIAN_POINT('Ctrl Pts',(-10.3742746610001,11.6,1.18675599899999));
#259034=CARTESIAN_POINT('Ctrl Pts',(-10.3756931460001,15.2,1.18671524399999));
#259035=CARTESIAN_POINT('Ctrl Pts',(-10.3756931460001,11.6,1.18671524399998));
#259036=CARTESIAN_POINT('Ctrl Pts',(-10.3771198660001,15.2,1.18667288599998));
#259037=CARTESIAN_POINT('Ctrl Pts',(-10.3771198660001,11.6,1.18667288599998));
#259038=CARTESIAN_POINT('Ctrl Pts',(-10.3785547980001,15.2,1.18662891399998));
#259039=CARTESIAN_POINT('Ctrl Pts',(-10.3785547980001,11.6,1.18662891399998));
#259040=CARTESIAN_POINT('Ctrl Pts',(-10.3799979240001,15.2,1.18658331299998));
#259041=CARTESIAN_POINT('Ctrl Pts',(-10.3799979240001,11.6,1.18658331299998));
#259042=CARTESIAN_POINT('Ctrl Pts',(-10.3814492210001,15.2,1.18653606699999));
#259043=CARTESIAN_POINT('Ctrl Pts',(-10.3814492210001,11.6,1.18653606699999));
#259044=CARTESIAN_POINT('Ctrl Pts',(-10.3829086680001,15.2,1.18648716499999));
#259045=CARTESIAN_POINT('Ctrl Pts',(-10.3829086680001,11.6,1.18648716499999));
#259046=CARTESIAN_POINT('Ctrl Pts',(-10.3843762450001,15.2,1.18643659199998));
#259047=CARTESIAN_POINT('Ctrl Pts',(-10.3843762450001,11.6,1.18643659199998));
#259048=CARTESIAN_POINT('Ctrl Pts',(-10.3858519330001,15.2,1.18638433399999));
#259049=CARTESIAN_POINT('Ctrl Pts',(-10.3858519330001,11.6,1.18638433399999));
#259050=CARTESIAN_POINT('Ctrl Pts',(-10.3873357080001,15.2,1.18633037799999));
#259051=CARTESIAN_POINT('Ctrl Pts',(-10.3873357080001,11.6,1.18633037799999));
#259052=CARTESIAN_POINT('Ctrl Pts',(-10.3888275530001,15.2,1.18627470999999));
#259053=CARTESIAN_POINT('Ctrl Pts',(-10.3888275530001,11.6,1.18627470999999));
#259054=CARTESIAN_POINT('Ctrl Pts',(-10.3903274450001,15.2,1.18621731599998));
#259055=CARTESIAN_POINT('Ctrl Pts',(-10.3903274450001,11.6,1.18621731599998));
#259056=CARTESIAN_POINT('Ctrl Pts',(-10.3918353650001,15.2,1.18615818399999));
#259057=CARTESIAN_POINT('Ctrl Pts',(-10.3918353650001,11.6,1.18615818399999));
#259058=CARTESIAN_POINT('Ctrl Pts',(-10.3933512920001,15.2,1.18609729999998));
#259059=CARTESIAN_POINT('Ctrl Pts',(-10.3933512920001,11.6,1.18609729999998));
#259060=CARTESIAN_POINT('Ctrl Pts',(-10.3948752070001,15.2,1.18603464899998));
#259061=CARTESIAN_POINT('Ctrl Pts',(-10.3948752070001,11.6,1.18603464899998));
#259062=CARTESIAN_POINT('Ctrl Pts',(-10.3964070880001,15.2,1.18597021999999));
#259063=CARTESIAN_POINT('Ctrl Pts',(-10.3964070880001,11.6,1.18597021999999));
#259064=CARTESIAN_POINT('Ctrl Pts',(-10.3979469170001,15.2,1.18590399899999));
#259065=CARTESIAN_POINT('Ctrl Pts',(-10.3979469170001,11.6,1.18590399899999));
#259066=CARTESIAN_POINT('Ctrl Pts',(-10.3994946730001,15.2,1.18583597199999));
#259067=CARTESIAN_POINT('Ctrl Pts',(-10.3994946730001,11.6,1.18583597199999));
#259068=CARTESIAN_POINT('Ctrl Pts',(-10.4010503360001,15.2,1.18576612699998));
#259069=CARTESIAN_POINT('Ctrl Pts',(-10.4010503360001,11.6,1.18576612699998));
#259070=CARTESIAN_POINT('Ctrl Pts',(-10.4026138870001,15.2,1.18569445199999));
#259071=CARTESIAN_POINT('Ctrl Pts',(-10.4026138870001,11.6,1.18569445199999));
#259072=CARTESIAN_POINT('Ctrl Pts',(-10.4041853050001,15.2,1.18562093199999));
#259073=CARTESIAN_POINT('Ctrl Pts',(-10.4041853050001,11.6,1.18562093199999));
#259074=CARTESIAN_POINT('Ctrl Pts',(-10.4057645710001,15.2,1.18554555499998));
#259075=CARTESIAN_POINT('Ctrl Pts',(-10.4057645710001,11.6,1.18554555499998));
#259076=CARTESIAN_POINT('Ctrl Pts',(-10.4073516650001,15.2,1.18546830799998));
#259077=CARTESIAN_POINT('Ctrl Pts',(-10.4073516650001,11.6,1.18546830799998));
#259078=CARTESIAN_POINT('Ctrl Pts',(-10.4089465690001,15.2,1.18538917799999));
#259079=CARTESIAN_POINT('Ctrl Pts',(-10.4089465690001,11.6,1.18538917799999));
#259080=CARTESIAN_POINT('Ctrl Pts',(-10.4105492620001,15.2,1.18530815299998));
#259081=CARTESIAN_POINT('Ctrl Pts',(-10.4105492620001,11.6,1.18530815299998));
#259082=CARTESIAN_POINT('Ctrl Pts',(-10.4121597240001,15.2,1.18522521999999));
#259083=CARTESIAN_POINT('Ctrl Pts',(-10.4121597240001,11.6,1.18522521999999));
#259084=CARTESIAN_POINT('Ctrl Pts',(-10.4137779370001,15.2,1.18514036599999));
#259085=CARTESIAN_POINT('Ctrl Pts',(-10.4137779370001,11.6,1.18514036599999));
#259086=CARTESIAN_POINT('Ctrl Pts',(-10.4154038820001,15.2,1.18505357999998));
#259087=CARTESIAN_POINT('Ctrl Pts',(-10.4154038820001,11.6,1.18505357999998));
#259088=CARTESIAN_POINT('Ctrl Pts',(-10.4170375390001,15.2,1.18496484799998));
#259089=CARTESIAN_POINT('Ctrl Pts',(-10.4170375390001,11.6,1.18496484799998));
#259090=CARTESIAN_POINT('Ctrl Pts',(-10.4186788900001,15.2,1.18487415599999));
#259091=CARTESIAN_POINT('Ctrl Pts',(-10.4186788900001,11.6,1.18487415599999));
#259092=CARTESIAN_POINT('Ctrl Pts',(-10.4203279130001,15.2,1.18478149699999));
#259093=CARTESIAN_POINT('Ctrl Pts',(-10.4203279130001,11.6,1.18478149699999));
#259094=CARTESIAN_POINT('Ctrl Pts',(-10.4219845930001,15.2,1.18468685399999));
#259095=CARTESIAN_POINT('Ctrl Pts',(-10.4219845930001,11.6,1.18468685399999));
#259096=CARTESIAN_POINT('Ctrl Pts',(-10.4236489080001,15.2,1.18459021499998));
#259097=CARTESIAN_POINT('Ctrl Pts',(-10.4236489080001,11.6,1.18459021499998));
#259098=CARTESIAN_POINT('Ctrl Pts',(-10.4253208410001,15.2,1.18449156999999));
#259099=CARTESIAN_POINT('Ctrl Pts',(-10.4253208410001,11.6,1.18449156999999));
#259100=CARTESIAN_POINT('Ctrl Pts',(-10.4270003720001,15.2,1.18439090599999));
#259101=CARTESIAN_POINT('Ctrl Pts',(-10.4270003720001,11.6,1.18439090599999));
#259102=CARTESIAN_POINT('Ctrl Pts',(-10.4286874830001,15.2,1.18428821199998));
#259103=CARTESIAN_POINT('Ctrl Pts',(-10.4286874830001,11.6,1.18428821199998));
#259104=CARTESIAN_POINT('Ctrl Pts',(-10.4303821540001,15.2,1.18418347399999));
#259105=CARTESIAN_POINT('Ctrl Pts',(-10.4303821540001,11.6,1.18418347399999));
#259106=CARTESIAN_POINT('Ctrl Pts',(-10.4320843690001,15.2,1.18407667999998));
#259107=CARTESIAN_POINT('Ctrl Pts',(-10.4320843690001,11.6,1.18407667999998));
#259108=CARTESIAN_POINT('Ctrl Pts',(-10.4337941070001,15.2,1.18396781999999));
#259109=CARTESIAN_POINT('Ctrl Pts',(-10.4337941070001,11.6,1.18396781999999));
#259110=CARTESIAN_POINT('Ctrl Pts',(-10.4355113520001,15.2,1.18385688099998));
#259111=CARTESIAN_POINT('Ctrl Pts',(-10.4355113520001,11.6,1.18385688099998));
#259112=CARTESIAN_POINT('Ctrl Pts',(-10.4372360820001,15.2,1.18374385099999));
#259113=CARTESIAN_POINT('Ctrl Pts',(-10.4372360820001,11.6,1.18374385099999));
#259114=CARTESIAN_POINT('Ctrl Pts',(-10.4389682810001,15.2,1.18362871999999));
#259115=CARTESIAN_POINT('Ctrl Pts',(-10.4389682810001,11.6,1.18362871999999));
#259116=CARTESIAN_POINT('Ctrl Pts',(-10.4407079310001,15.2,1.18351147399999));
#259117=CARTESIAN_POINT('Ctrl Pts',(-10.4407079310001,11.6,1.18351147399998));
#259118=CARTESIAN_POINT('Ctrl Pts',(-10.4424550130001,15.2,1.18339210299998));
#259119=CARTESIAN_POINT('Ctrl Pts',(-10.4424550130001,11.6,1.18339210299998));
#259120=CARTESIAN_POINT('Ctrl Pts',(-10.4442095090001,15.2,1.18327059399999));
#259121=CARTESIAN_POINT('Ctrl Pts',(-10.4442095090001,11.6,1.18327059399999));
#259122=CARTESIAN_POINT('Ctrl Pts',(-10.4459714000001,15.2,1.18314693699999));
#259123=CARTESIAN_POINT('Ctrl Pts',(-10.4459714000001,11.6,1.18314693699999));
#259124=CARTESIAN_POINT('Ctrl Pts',(-10.4477406700001,15.2,1.18302111899999));
#259125=CARTESIAN_POINT('Ctrl Pts',(-10.4477406700001,11.6,1.18302111899998));
#259126=CARTESIAN_POINT('Ctrl Pts',(-10.4495173000001,15.2,1.18289313099998));
#259127=CARTESIAN_POINT('Ctrl Pts',(-10.4495173000001,11.6,1.18289313099998));
#259128=CARTESIAN_POINT('Ctrl Pts',(-10.4513012710001,15.2,1.18276295899999));
#259129=CARTESIAN_POINT('Ctrl Pts',(-10.4513012710001,11.6,1.18276295899999));
#259130=CARTESIAN_POINT('Ctrl Pts',(-10.4530925660001,15.2,1.18263059399998));
#259131=CARTESIAN_POINT('Ctrl Pts',(-10.4530925660001,11.6,1.18263059399998));
#259132=CARTESIAN_POINT('Ctrl Pts',(-10.4548911670001,15.2,1.18249602199999));
#259133=CARTESIAN_POINT('Ctrl Pts',(-10.4548911670001,11.6,1.18249602199999));
#259134=CARTESIAN_POINT('Ctrl Pts',(-10.4566970570001,15.2,1.18235923399999));
#259135=CARTESIAN_POINT('Ctrl Pts',(-10.4566970570001,11.6,1.18235923399999));
#259136=CARTESIAN_POINT('Ctrl Pts',(-10.4585102170001,15.2,1.18222021899999));
#259137=CARTESIAN_POINT('Ctrl Pts',(-10.4585102170001,11.6,1.18222021899998));
#259138=CARTESIAN_POINT('Ctrl Pts',(-10.4603306310001,15.2,1.18207896399999));
#259139=CARTESIAN_POINT('Ctrl Pts',(-10.4603306310001,11.6,1.18207896399999));
#259140=CARTESIAN_POINT('Ctrl Pts',(-10.4621582800001,15.2,1.18193545999999));
#259141=CARTESIAN_POINT('Ctrl Pts',(-10.4621582800001,11.6,1.18193545999999));
#259142=CARTESIAN_POINT('Ctrl Pts',(-10.4639931470001,15.2,1.18178969599999));
#259143=CARTESIAN_POINT('Ctrl Pts',(-10.4639931470001,11.6,1.18178969599999));
#259144=CARTESIAN_POINT('Ctrl Pts',(-10.4658352150001,15.2,1.18164165899998));
#259145=CARTESIAN_POINT('Ctrl Pts',(-10.4658352150001,11.6,1.18164165899998));
#259146=CARTESIAN_POINT('Ctrl Pts',(-10.4676844650001,15.2,1.18149133999998));
#259147=CARTESIAN_POINT('Ctrl Pts',(-10.4676844650001,11.6,1.18149133999998));
#259148=CARTESIAN_POINT('Ctrl Pts',(-10.4695408810001,15.2,1.18133872599998));
#259149=CARTESIAN_POINT('Ctrl Pts',(-10.4695408810001,11.6,1.18133872599998));
#259150=CARTESIAN_POINT('Ctrl Pts',(-10.4714044460001,15.2,1.18118380899999));
#259151=CARTESIAN_POINT('Ctrl Pts',(-10.4714044460001,11.6,1.18118380899999));
#259152=CARTESIAN_POINT('Ctrl Pts',(-10.4732751410001,15.2,1.18102657599998));
#259153=CARTESIAN_POINT('Ctrl Pts',(-10.4732751410001,11.6,1.18102657599998));
#259154=CARTESIAN_POINT('Ctrl Pts',(-10.4751529500001,15.2,1.18086701799998));
#259155=CARTESIAN_POINT('Ctrl Pts',(-10.4751529500001,11.6,1.18086701799998));
#259156=CARTESIAN_POINT('Ctrl Pts',(-10.4770378570001,15.2,1.18070512399999));
#259157=CARTESIAN_POINT('Ctrl Pts',(-10.4770378570001,11.6,1.18070512399999));
#259158=CARTESIAN_POINT('Ctrl Pts',(-10.4789298430001,15.2,1.18054088199999));
#259159=CARTESIAN_POINT('Ctrl Pts',(-10.4789298430001,11.6,1.18054088199999));
#259160=CARTESIAN_POINT('Ctrl Pts',(-10.4808288920001,15.2,1.18037428299999));
#259161=CARTESIAN_POINT('Ctrl Pts',(-10.4808288920001,11.6,1.18037428299999));
#259162=CARTESIAN_POINT('Ctrl Pts',(-10.4827349850001,15.2,1.18020531599999));
#259163=CARTESIAN_POINT('Ctrl Pts',(-10.4827349850001,11.6,1.18020531599999));
#259164=CARTESIAN_POINT('Ctrl Pts',(-10.4846481080001,15.2,1.18003396999999));
#259165=CARTESIAN_POINT('Ctrl Pts',(-10.4846481080001,11.6,1.18003396999998));
#259166=CARTESIAN_POINT('Ctrl Pts',(-10.4865682440001,15.2,1.17986023499999));
#259167=CARTESIAN_POINT('Ctrl Pts',(-10.4865682440001,11.6,1.17986023499998));
#259168=CARTESIAN_POINT('Ctrl Pts',(-10.4884953720001,15.2,1.17968410099999));
#259169=CARTESIAN_POINT('Ctrl Pts',(-10.4884953720001,11.6,1.17968410099999));
#259170=CARTESIAN_POINT('Ctrl Pts',(-10.4904294800001,15.2,1.17950555699998));
#259171=CARTESIAN_POINT('Ctrl Pts',(-10.4904294800001,11.6,1.17950555699998));
#259172=CARTESIAN_POINT('Ctrl Pts',(-10.4923705490001,15.2,1.17932459399999));
#259173=CARTESIAN_POINT('Ctrl Pts',(-10.4923705490001,11.6,1.17932459399999));
#259174=CARTESIAN_POINT('Ctrl Pts',(-10.4943185630001,15.2,1.17914119999998));
#259175=CARTESIAN_POINT('Ctrl Pts',(-10.4943185630001,11.6,1.17914119999998));
#259176=CARTESIAN_POINT('Ctrl Pts',(-10.4962735060001,15.2,1.17895536499999));
#259177=CARTESIAN_POINT('Ctrl Pts',(-10.4962735060001,11.6,1.17895536499998));
#259178=CARTESIAN_POINT('Ctrl Pts',(-10.4982353590001,15.2,1.17876708099999));
#259179=CARTESIAN_POINT('Ctrl Pts',(-10.4982353590001,11.6,1.17876708099998));
#259180=CARTESIAN_POINT('Ctrl Pts',(-10.5002041080001,15.2,1.17857633499999));
#259181=CARTESIAN_POINT('Ctrl Pts',(-10.5002041080001,11.6,1.17857633499999));
#259182=CARTESIAN_POINT('Ctrl Pts',(-10.5021797350001,15.2,1.17838311899999));
#259183=CARTESIAN_POINT('Ctrl Pts',(-10.5021797350001,11.6,1.17838311899999));
#259184=CARTESIAN_POINT('Ctrl Pts',(-10.5041622250001,15.2,1.17818742199999));
#259185=CARTESIAN_POINT('Ctrl Pts',(-10.5041622250001,11.6,1.17818742199999));
#259186=CARTESIAN_POINT('Ctrl Pts',(-10.5061515600001,15.2,1.17798923599999));
#259187=CARTESIAN_POINT('Ctrl Pts',(-10.5061515600001,11.6,1.17798923599999));
#259188=CARTESIAN_POINT('Ctrl Pts',(-10.5081477230001,15.2,1.17778854799999));
#259189=CARTESIAN_POINT('Ctrl Pts',(-10.5081477230001,11.6,1.17778854799999));
#259190=CARTESIAN_POINT('Ctrl Pts',(-10.5101507010001,15.2,1.17758534999998));
#259191=CARTESIAN_POINT('Ctrl Pts',(-10.5101507010001,11.6,1.17758534999998));
#259192=CARTESIAN_POINT('Ctrl Pts',(-10.5121604750001,15.2,1.17737963099998));
#259193=CARTESIAN_POINT('Ctrl Pts',(-10.5121604750001,11.6,1.17737963099998));
#259194=CARTESIAN_POINT('Ctrl Pts',(-10.5141770310001,15.2,1.17717138199998));
#259195=CARTESIAN_POINT('Ctrl Pts',(-10.5141770310001,11.6,1.17717138199998));
#259196=CARTESIAN_POINT('Ctrl Pts',(-10.5162003510001,15.2,1.17696059399998));
#259197=CARTESIAN_POINT('Ctrl Pts',(-10.5162003510001,11.6,1.17696059399998));
#259198=CARTESIAN_POINT('Ctrl Pts',(-10.5182304190001,15.2,1.17674725699999));
#259199=CARTESIAN_POINT('Ctrl Pts',(-10.5182304190001,11.6,1.17674725699999));
#259200=CARTESIAN_POINT('Ctrl Pts',(-10.5202672190001,15.2,1.17653135999999));
#259201=CARTESIAN_POINT('Ctrl Pts',(-10.5202672190001,11.6,1.17653135999999));
#259202=CARTESIAN_POINT('Ctrl Pts',(-10.5223107360001,15.2,1.17631289399998));
#259203=CARTESIAN_POINT('Ctrl Pts',(-10.5223107360001,11.6,1.17631289399998));
#259204=CARTESIAN_POINT('Ctrl Pts',(-10.5243609530001,15.2,1.17609184999999));
#259205=CARTESIAN_POINT('Ctrl Pts',(-10.5243609530001,11.6,1.17609184999999));
#259206=CARTESIAN_POINT('Ctrl Pts',(-10.5264178550001,15.2,1.17586821899998));
#259207=CARTESIAN_POINT('Ctrl Pts',(-10.5264178550001,11.6,1.17586821899998));
#259208=CARTESIAN_POINT('Ctrl Pts',(-10.5284814260001,15.2,1.17564198999998));
#259209=CARTESIAN_POINT('Ctrl Pts',(-10.5284814260001,11.6,1.17564198999998));
#259210=CARTESIAN_POINT('Ctrl Pts',(-10.5305516490001,15.2,1.17541315299999));
#259211=CARTESIAN_POINT('Ctrl Pts',(-10.5305516490001,11.6,1.17541315299999));
#259212=CARTESIAN_POINT('Ctrl Pts',(-10.5326285090001,15.2,1.17518170099999));
#259213=CARTESIAN_POINT('Ctrl Pts',(-10.5326285090001,11.6,1.17518170099998));
#259214=CARTESIAN_POINT('Ctrl Pts',(-10.5347119910001,15.2,1.17494762299998));
#259215=CARTESIAN_POINT('Ctrl Pts',(-10.5347119910001,11.6,1.17494762299998));
#259216=CARTESIAN_POINT('Ctrl Pts',(-10.5368020780001,15.2,1.17471090999999));
#259217=CARTESIAN_POINT('Ctrl Pts',(-10.5368020780001,11.6,1.17471090999999));
#259218=CARTESIAN_POINT('Ctrl Pts',(-10.5388987570001,15.2,1.17447155299998));
#259219=CARTESIAN_POINT('Ctrl Pts',(-10.5388987570001,11.6,1.17447155299998));
#259220=CARTESIAN_POINT('Ctrl Pts',(-10.5410020080001,15.2,1.17422954199998));
#259221=CARTESIAN_POINT('Ctrl Pts',(-10.5410020080001,11.6,1.17422954199998));
#259222=CARTESIAN_POINT('Ctrl Pts',(-10.5431118190001,15.2,1.17398486899999));
#259223=CARTESIAN_POINT('Ctrl Pts',(-10.5431118190001,11.6,1.17398486899999));
#259224=CARTESIAN_POINT('Ctrl Pts',(-10.5452281730001,15.2,1.17373752299998));
#259225=CARTESIAN_POINT('Ctrl Pts',(-10.5452281730001,11.6,1.17373752299998));
#259226=CARTESIAN_POINT('Ctrl Pts',(-10.5473510550001,15.2,1.17348749699998));
#259227=CARTESIAN_POINT('Ctrl Pts',(-10.5473510550001,11.6,1.17348749699998));
#259228=CARTESIAN_POINT('Ctrl Pts',(-10.5494804500001,15.2,1.17323477999999));
#259229=CARTESIAN_POINT('Ctrl Pts',(-10.5494804500001,11.6,1.17323477999998));
#259230=CARTESIAN_POINT('Ctrl Pts',(-10.5516163410001,15.2,1.17297936399999));
#259231=CARTESIAN_POINT('Ctrl Pts',(-10.5516163410001,11.6,1.17297936399999));
#259232=CARTESIAN_POINT('Ctrl Pts',(-10.5537587150001,15.2,1.17272124099999));
#259233=CARTESIAN_POINT('Ctrl Pts',(-10.5537587150001,11.6,1.17272124099998));
#259234=CARTESIAN_POINT('Ctrl Pts',(-10.5559075550001,15.2,1.17246039999999));
#259235=CARTESIAN_POINT('Ctrl Pts',(-10.5559075550001,11.6,1.17246039999999));
#259236=CARTESIAN_POINT('Ctrl Pts',(-10.5580628460001,15.2,1.17219683299998));
#259237=CARTESIAN_POINT('Ctrl Pts',(-10.5580628460001,11.6,1.17219683299998));
#259238=CARTESIAN_POINT('Ctrl Pts',(-10.5602245730001,15.2,1.17193052999998));
#259239=CARTESIAN_POINT('Ctrl Pts',(-10.5602245730001,11.6,1.17193052999998));
#259240=CARTESIAN_POINT('Ctrl Pts',(-10.5623927210001,15.2,1.17166148499999));
#259241=CARTESIAN_POINT('Ctrl Pts',(-10.5623927210001,11.6,1.17166148499999));
#259242=CARTESIAN_POINT('Ctrl Pts',(-10.5645672750001,15.2,1.17138968599999));
#259243=CARTESIAN_POINT('Ctrl Pts',(-10.5645672750001,11.6,1.17138968599999));
#259244=CARTESIAN_POINT('Ctrl Pts',(-10.5667482200001,15.2,1.17111512499998));
#259245=CARTESIAN_POINT('Ctrl Pts',(-10.5667482200001,11.6,1.17111512499998));
#259246=CARTESIAN_POINT('Ctrl Pts',(-10.5689355400001,15.2,1.17083779399998));
#259247=CARTESIAN_POINT('Ctrl Pts',(-10.5689355400001,11.6,1.17083779399998));
#259248=CARTESIAN_POINT('Ctrl Pts',(-10.5711292210001,15.2,1.17055768399998));
#259249=CARTESIAN_POINT('Ctrl Pts',(-10.5711292210001,11.6,1.17055768399998));
#259250=CARTESIAN_POINT('Ctrl Pts',(-10.5733292470001,15.2,1.17027478699999));
#259251=CARTESIAN_POINT('Ctrl Pts',(-10.5733292470001,11.6,1.17027478699998));
#259252=CARTESIAN_POINT('Ctrl Pts',(-10.5755356040001,15.2,1.16998909399999));
#259253=CARTESIAN_POINT('Ctrl Pts',(-10.5755356040001,11.6,1.16998909399999));
#259254=CARTESIAN_POINT('Ctrl Pts',(-10.5777482770001,15.2,1.16970059599999));
#259255=CARTESIAN_POINT('Ctrl Pts',(-10.5777482770001,11.6,1.16970059599998));
#259256=CARTESIAN_POINT('Ctrl Pts',(-10.5799672510001,15.2,1.16940928399998));
#259257=CARTESIAN_POINT('Ctrl Pts',(-10.5799672510001,11.6,1.16940928399998));
#259258=CARTESIAN_POINT('Ctrl Pts',(-10.5821925120001,15.2,1.16911514999999));
#259259=CARTESIAN_POINT('Ctrl Pts',(-10.5821925120001,11.6,1.16911514999999));
#259260=CARTESIAN_POINT('Ctrl Pts',(-10.5844240430001,15.2,1.16881818499999));
#259261=CARTESIAN_POINT('Ctrl Pts',(-10.5844240430001,11.6,1.16881818499999));
#259262=CARTESIAN_POINT('Ctrl Pts',(-10.5866618310001,15.2,1.16851838199999));
#259263=CARTESIAN_POINT('Ctrl Pts',(-10.5866618310001,11.6,1.16851838199999));
#259264=CARTESIAN_POINT('Ctrl Pts',(-10.5889058620001,15.2,1.16821573099998));
#259265=CARTESIAN_POINT('Ctrl Pts',(-10.5889058620001,11.6,1.16821573099998));
#259266=CARTESIAN_POINT('Ctrl Pts',(-10.5911561200001,15.2,1.16791022399998));
#259267=CARTESIAN_POINT('Ctrl Pts',(-10.5911561200001,11.6,1.16791022399998));
#259268=CARTESIAN_POINT('Ctrl Pts',(-10.5934125910001,15.2,1.16760185399999));
#259269=CARTESIAN_POINT('Ctrl Pts',(-10.5934125910001,11.6,1.16760185399999));
#259270=CARTESIAN_POINT('Ctrl Pts',(-10.5956752600001,15.2,1.16729060999999));
#259271=CARTESIAN_POINT('Ctrl Pts',(-10.5956752600001,11.6,1.16729060999999));
#259272=CARTESIAN_POINT('Ctrl Pts',(-10.5979441110001,15.2,1.16697648599999));
#259273=CARTESIAN_POINT('Ctrl Pts',(-10.5979441110001,11.6,1.16697648599999));
#259274=CARTESIAN_POINT('Ctrl Pts',(-10.6002191330001,15.2,1.16665947299999));
#259275=CARTESIAN_POINT('Ctrl Pts',(-10.6002191330001,11.6,1.16665947299999));
#259276=CARTESIAN_POINT('Ctrl Pts',(-10.6025003100001,15.2,1.16633956299999));
#259277=CARTESIAN_POINT('Ctrl Pts',(-10.6025003100001,11.6,1.16633956299998));
#259278=CARTESIAN_POINT('Ctrl Pts',(-10.6047876270001,15.2,1.16601674699998));
#259279=CARTESIAN_POINT('Ctrl Pts',(-10.6047876270001,11.6,1.16601674699998));
#259280=CARTESIAN_POINT('Ctrl Pts',(-10.6070810700001,15.2,1.16569101799998));
#259281=CARTESIAN_POINT('Ctrl Pts',(-10.6070810700001,11.6,1.16569101799998));
#259282=CARTESIAN_POINT('Ctrl Pts',(-10.6093806240001,15.2,1.16536236699998));
#259283=CARTESIAN_POINT('Ctrl Pts',(-10.6093806240001,11.6,1.16536236699998));
#259284=CARTESIAN_POINT('Ctrl Pts',(-10.6116862760001,15.2,1.16503078599999));
#259285=CARTESIAN_POINT('Ctrl Pts',(-10.6116862760001,11.6,1.16503078599999));
#259286=CARTESIAN_POINT('Ctrl Pts',(-10.6139980110001,15.2,1.16469626699998));
#259287=CARTESIAN_POINT('Ctrl Pts',(-10.6139980110001,11.6,1.16469626699998));
#259288=CARTESIAN_POINT('Ctrl Pts',(-10.6163158140001,15.2,1.16435880299999));
#259289=CARTESIAN_POINT('Ctrl Pts',(-10.6163158140001,11.6,1.16435880299999));
#259290=CARTESIAN_POINT('Ctrl Pts',(-10.6186396720001,15.2,1.16401838499999));
#259291=CARTESIAN_POINT('Ctrl Pts',(-10.6186396720001,11.6,1.16401838499998));
#259292=CARTESIAN_POINT('Ctrl Pts',(-10.6209695720001,15.2,1.16367500499999));
#259293=CARTESIAN_POINT('Ctrl Pts',(-10.6209695720001,11.6,1.16367500499999));
#259294=CARTESIAN_POINT('Ctrl Pts',(-10.6233054970001,15.2,1.16332865499999));
#259295=CARTESIAN_POINT('Ctrl Pts',(-10.6233054970001,11.6,1.16332865499999));
#259296=CARTESIAN_POINT('Ctrl Pts',(-10.6256474340001,15.2,1.16297932799998));
#259297=CARTESIAN_POINT('Ctrl Pts',(-10.6256474340001,11.6,1.16297932799998));
#259298=CARTESIAN_POINT('Ctrl Pts',(-10.6279953690001,15.2,1.16262701499998));
#259299=CARTESIAN_POINT('Ctrl Pts',(-10.6279953690001,11.6,1.16262701499998));
#259300=CARTESIAN_POINT('Ctrl Pts',(-10.6303492890001,15.2,1.16227170999998));
#259301=CARTESIAN_POINT('Ctrl Pts',(-10.6303492890001,11.6,1.16227170999998));
#259302=CARTESIAN_POINT('Ctrl Pts',(-10.6327091780001,15.2,1.16191340299999));
#259303=CARTESIAN_POINT('Ctrl Pts',(-10.6327091780001,11.6,1.16191340299999));
#259304=CARTESIAN_POINT('Ctrl Pts',(-10.6350750250001,15.2,1.16155208699999));
#259305=CARTESIAN_POINT('Ctrl Pts',(-10.6350750250001,11.6,1.16155208699999));
#259306=CARTESIAN_POINT('Ctrl Pts',(-10.6374468130001,15.2,1.16118775499999));
#259307=CARTESIAN_POINT('Ctrl Pts',(-10.6374468130001,11.6,1.16118775499999));
#259308=CARTESIAN_POINT('Ctrl Pts',(-10.6398245300001,15.2,1.16082039899998));
#259309=CARTESIAN_POINT('Ctrl Pts',(-10.6398245300001,11.6,1.16082039899998));
#259310=CARTESIAN_POINT('Ctrl Pts',(-10.6422081610001,15.2,1.16045001099998));
#259311=CARTESIAN_POINT('Ctrl Pts',(-10.6422081610001,11.6,1.16045001099998));
#259312=CARTESIAN_POINT('Ctrl Pts',(-10.6445976930001,15.2,1.16007658299999));
#259313=CARTESIAN_POINT('Ctrl Pts',(-10.6445976930001,11.6,1.16007658299999));
#259314=CARTESIAN_POINT('Ctrl Pts',(-10.6469931120001,15.2,1.15970010799999));
#259315=CARTESIAN_POINT('Ctrl Pts',(-10.6469931120001,11.6,1.15970010799999));
#259316=CARTESIAN_POINT('Ctrl Pts',(-10.6493944050001,15.2,1.15932057999999));
#259317=CARTESIAN_POINT('Ctrl Pts',(-10.6493944050001,11.6,1.15932057999998));
#259318=CARTESIAN_POINT('Ctrl Pts',(-10.6518015570001,15.2,1.15893798799998));
#259319=CARTESIAN_POINT('Ctrl Pts',(-10.6518015570001,11.6,1.15893798799998));
#259320=CARTESIAN_POINT('Ctrl Pts',(-10.6542145550001,15.2,1.15855232699999));
#259321=CARTESIAN_POINT('Ctrl Pts',(-10.6542145550001,11.6,1.15855232699999));
#259322=CARTESIAN_POINT('Ctrl Pts',(-10.6566333850001,15.2,1.15816358799998));
#259323=CARTESIAN_POINT('Ctrl Pts',(-10.6566333850001,11.6,1.15816358799998));
#259324=CARTESIAN_POINT('Ctrl Pts',(-10.6590580340001,15.2,1.15777176599998));
#259325=CARTESIAN_POINT('Ctrl Pts',(-10.6590580340001,11.6,1.15777176599998));
#259326=CARTESIAN_POINT('Ctrl Pts',(-10.6614884880001,15.2,1.15737684999999));
#259327=CARTESIAN_POINT('Ctrl Pts',(-10.6614884880001,11.6,1.15737684999999));
#259328=CARTESIAN_POINT('Ctrl Pts',(-10.6639247340001,15.2,1.15697883699998));
#259329=CARTESIAN_POINT('Ctrl Pts',(-10.6639247340001,11.6,1.15697883699998));
#259330=CARTESIAN_POINT('Ctrl Pts',(-10.6663667570001,15.2,1.15657771499999));
#259331=CARTESIAN_POINT('Ctrl Pts',(-10.6663667570001,11.6,1.15657771499999));
#259332=CARTESIAN_POINT('Ctrl Pts',(-10.6688145450001,15.2,1.15617348099998));
#259333=CARTESIAN_POINT('Ctrl Pts',(-10.6688145450001,11.6,1.15617348099998));
#259334=CARTESIAN_POINT('Ctrl Pts',(-10.6712680840001,15.2,1.15576612499999));
#259335=CARTESIAN_POINT('Ctrl Pts',(-10.6712680840001,11.6,1.15576612499999));
#259336=CARTESIAN_POINT('Ctrl Pts',(-10.6737273610001,15.2,1.15535563899998));
#259337=CARTESIAN_POINT('Ctrl Pts',(-10.6737273610001,11.6,1.15535563899998));
#259338=CARTESIAN_POINT('Ctrl Pts',(-10.6761923620001,15.2,1.15494201899998));
#259339=CARTESIAN_POINT('Ctrl Pts',(-10.6761923620001,11.6,1.15494201899998));
#259340=CARTESIAN_POINT('Ctrl Pts',(-10.6786630740001,15.2,1.15452525499999));
#259341=CARTESIAN_POINT('Ctrl Pts',(-10.6786630740001,11.6,1.15452525499998));
#259342=CARTESIAN_POINT('Ctrl Pts',(-10.6811394830001,15.2,1.15410534099999));
#259343=CARTESIAN_POINT('Ctrl Pts',(-10.6811394830001,11.6,1.15410534099999));
#259344=CARTESIAN_POINT('Ctrl Pts',(-10.6836215780001,15.2,1.15368226999998));
#259345=CARTESIAN_POINT('Ctrl Pts',(-10.6836215780001,11.6,1.15368226999998));
#259346=CARTESIAN_POINT('Ctrl Pts',(-10.6861093440001,15.2,1.15325603399999));
#259347=CARTESIAN_POINT('Ctrl Pts',(-10.6861093440001,11.6,1.15325603399999));
#259348=CARTESIAN_POINT('Ctrl Pts',(-10.6886027670001,15.2,1.15282662699999));
#259349=CARTESIAN_POINT('Ctrl Pts',(-10.6886027670001,11.6,1.15282662699998));
#259350=CARTESIAN_POINT('Ctrl Pts',(-10.6911018330001,15.2,1.15239403999999));
#259351=CARTESIAN_POINT('Ctrl Pts',(-10.6911018330001,11.6,1.15239403999999));
#259352=CARTESIAN_POINT('Ctrl Pts',(-10.6936065330001,15.2,1.15195826999999));
#259353=CARTESIAN_POINT('Ctrl Pts',(-10.6936065330001,11.6,1.15195826999999));
#259354=CARTESIAN_POINT('Ctrl Pts',(-10.6961168510001,15.2,1.15151930499998));
#259355=CARTESIAN_POINT('Ctrl Pts',(-10.6961168510001,11.6,1.15151930499998));
#259356=CARTESIAN_POINT('Ctrl Pts',(-10.6986327730001,15.2,1.15107714099999));
#259357=CARTESIAN_POINT('Ctrl Pts',(-10.6986327730001,11.6,1.15107714099999));
#259358=CARTESIAN_POINT('Ctrl Pts',(-10.7011542890001,15.2,1.15063176999998));
#259359=CARTESIAN_POINT('Ctrl Pts',(-10.7011542890001,11.6,1.15063176999998));
#259360=CARTESIAN_POINT('Ctrl Pts',(-10.7036813830001,15.2,1.15018318599999));
#259361=CARTESIAN_POINT('Ctrl Pts',(-10.7036813830001,11.6,1.15018318599999));
#259362=CARTESIAN_POINT('Ctrl Pts',(-10.7062140430001,15.2,1.14973138199999));
#259363=CARTESIAN_POINT('Ctrl Pts',(-10.7062140430001,11.6,1.14973138199999));
#259364=CARTESIAN_POINT('Ctrl Pts',(-10.7087522570001,15.2,1.14927634999999));
#259365=CARTESIAN_POINT('Ctrl Pts',(-10.7087522570001,11.6,1.14927634999999));
#259366=CARTESIAN_POINT('Ctrl Pts',(-10.7112960120001,15.2,1.14881808499999));
#259367=CARTESIAN_POINT('Ctrl Pts',(-10.7112960120001,11.6,1.14881808499998));
#259368=CARTESIAN_POINT('Ctrl Pts',(-10.7138452930001,15.2,1.14835657899999));
#259369=CARTESIAN_POINT('Ctrl Pts',(-10.7138452930001,11.6,1.14835657899999));
#259370=CARTESIAN_POINT('Ctrl Pts',(-10.7164000880001,15.2,1.14789182399999));
#259371=CARTESIAN_POINT('Ctrl Pts',(-10.7164000880001,11.6,1.14789182399999));
#259372=CARTESIAN_POINT('Ctrl Pts',(-10.7189603860001,15.2,1.14742381499998));
#259373=CARTESIAN_POINT('Ctrl Pts',(-10.7189603860001,11.6,1.14742381499998));
#259374=CARTESIAN_POINT('Ctrl Pts',(-10.7215261720001,15.2,1.14695254599999));
#259375=CARTESIAN_POINT('Ctrl Pts',(-10.7215261720001,11.6,1.14695254599999));
#259376=CARTESIAN_POINT('Ctrl Pts',(-10.7240974330001,15.2,1.14647800799998));
#259377=CARTESIAN_POINT('Ctrl Pts',(-10.7240974330001,11.6,1.14647800799998));
#259378=CARTESIAN_POINT('Ctrl Pts',(-10.7266741590001,15.2,1.14600019699999));
#259379=CARTESIAN_POINT('Ctrl Pts',(-10.7266741590001,11.6,1.14600019699999));
#259380=CARTESIAN_POINT('Ctrl Pts',(-10.7292563340001,15.2,1.14551910299999));
#259381=CARTESIAN_POINT('Ctrl Pts',(-10.7292563340001,11.6,1.14551910299999));
#259382=CARTESIAN_POINT('Ctrl Pts',(-10.7318439480001,15.2,1.14503472299999));
#259383=CARTESIAN_POINT('Ctrl Pts',(-10.7318439480001,11.6,1.14503472299999));
#259384=CARTESIAN_POINT('Ctrl Pts',(-10.7344369860001,15.2,1.14454704699999));
#259385=CARTESIAN_POINT('Ctrl Pts',(-10.7344369860001,11.6,1.14454704699999));
#259386=CARTESIAN_POINT('Ctrl Pts',(-10.7370354360001,15.2,1.14405607099998));
#259387=CARTESIAN_POINT('Ctrl Pts',(-10.7370354360001,11.6,1.14405607099998));
#259388=CARTESIAN_POINT('Ctrl Pts',(-10.7396392860001,15.2,1.14356178699999));
#259389=CARTESIAN_POINT('Ctrl Pts',(-10.7396392860001,11.6,1.14356178699999));
#259390=CARTESIAN_POINT('Ctrl Pts',(-10.7422485240001,15.2,1.14306418899998));
#259391=CARTESIAN_POINT('Ctrl Pts',(-10.7422485240001,11.6,1.14306418899998));
#259392=CARTESIAN_POINT('Ctrl Pts',(-10.7448631370001,15.2,1.14256327099998));
#259393=CARTESIAN_POINT('Ctrl Pts',(-10.7448631370001,11.6,1.14256327099998));
#259394=CARTESIAN_POINT('Ctrl Pts',(-10.7474831100001,15.2,1.14205902499998));
#259395=CARTESIAN_POINT('Ctrl Pts',(-10.7474831100001,11.6,1.14205902499998));
#259396=CARTESIAN_POINT('Ctrl Pts',(-10.7501084340001,15.2,1.14155144699998));
#259397=CARTESIAN_POINT('Ctrl Pts',(-10.7501084340001,11.6,1.14155144699998));
#259398=CARTESIAN_POINT('Ctrl Pts',(-10.7527390940001,15.2,1.14104052899998));
#259399=CARTESIAN_POINT('Ctrl Pts',(-10.7527390940001,11.6,1.14104052899998));
#259400=CARTESIAN_POINT('Ctrl Pts',(-10.7553750790001,15.2,1.14052626499999));
#259401=CARTESIAN_POINT('Ctrl Pts',(-10.7553750790001,11.6,1.14052626499999));
#259402=CARTESIAN_POINT('Ctrl Pts',(-10.7580163760001,15.2,1.14000864899999));
#259403=CARTESIAN_POINT('Ctrl Pts',(-10.7580163760001,11.6,1.14000864899999));
#259404=CARTESIAN_POINT('Ctrl Pts',(-10.7606629730001,15.2,1.13948767199998));
#259405=CARTESIAN_POINT('Ctrl Pts',(-10.7606629730001,11.6,1.13948767199998));
#259406=CARTESIAN_POINT('Ctrl Pts',(-10.7633148570001,15.2,1.13896333199999));
#259407=CARTESIAN_POINT('Ctrl Pts',(-10.7633148570001,11.6,1.13896333199999));
#259408=CARTESIAN_POINT('Ctrl Pts',(-10.7659720160001,15.2,1.13843561899999));
#259409=CARTESIAN_POINT('Ctrl Pts',(-10.7659720160001,11.6,1.13843561899999));
#259410=CARTESIAN_POINT('Ctrl Pts',(-10.7686344370001,15.2,1.13790452999998));
#259411=CARTESIAN_POINT('Ctrl Pts',(-10.7686344370001,11.6,1.13790452999998));
#259412=CARTESIAN_POINT('Ctrl Pts',(-10.7713021080001,15.2,1.13737005599999));
#259413=CARTESIAN_POINT('Ctrl Pts',(-10.7713021080001,11.6,1.13737005599999));
#259414=CARTESIAN_POINT('Ctrl Pts',(-10.7739750180001,15.2,1.13683219199999));
#259415=CARTESIAN_POINT('Ctrl Pts',(-10.7739750180001,11.6,1.13683219199999));
#259416=CARTESIAN_POINT('Ctrl Pts',(-10.7766531540001,15.2,1.13629093099998));
#259417=CARTESIAN_POINT('Ctrl Pts',(-10.7766531540001,11.6,1.13629093099998));
#259418=CARTESIAN_POINT('Ctrl Pts',(-10.7793365030001,15.2,1.13574626899998));
#259419=CARTESIAN_POINT('Ctrl Pts',(-10.7793365030001,11.6,1.13574626899998));
#259420=CARTESIAN_POINT('Ctrl Pts',(-10.7820250540001,15.2,1.13519819699999));
#259421=CARTESIAN_POINT('Ctrl Pts',(-10.7820250540001,11.6,1.13519819699999));
#259422=CARTESIAN_POINT('Ctrl Pts',(-10.7847187940001,15.2,1.13464671099999));
#259423=CARTESIAN_POINT('Ctrl Pts',(-10.7847187940001,11.6,1.13464671099999));
#259424=CARTESIAN_POINT('Ctrl Pts',(-10.7874177100001,15.2,1.13409180499998));
#259425=CARTESIAN_POINT('Ctrl Pts',(-10.7874177100001,11.6,1.13409180499998));
#259426=CARTESIAN_POINT('Ctrl Pts',(-10.7901217920001,15.2,1.13353347099999));
#259427=CARTESIAN_POINT('Ctrl Pts',(-10.7901217920001,11.6,1.13353347099999));
#259428=CARTESIAN_POINT('Ctrl Pts',(-10.7928310260001,15.2,1.13297170399999));
#259429=CARTESIAN_POINT('Ctrl Pts',(-10.7928310260001,11.6,1.13297170399999));
#259430=CARTESIAN_POINT('Ctrl Pts',(-10.7955454010001,15.2,1.13240649799998));
#259431=CARTESIAN_POINT('Ctrl Pts',(-10.7955454010001,11.6,1.13240649799998));
#259432=CARTESIAN_POINT('Ctrl Pts',(-10.7982649040001,15.2,1.13183784699999));
#259433=CARTESIAN_POINT('Ctrl Pts',(-10.7982649040001,11.6,1.13183784699999));
#259434=CARTESIAN_POINT('Ctrl Pts',(-10.8009895250001,15.2,1.13126574599999));
#259435=CARTESIAN_POINT('Ctrl Pts',(-10.8009895250001,11.6,1.13126574599998));
#259436=CARTESIAN_POINT('Ctrl Pts',(-10.8037192500001,15.2,1.13069018799999));
#259437=CARTESIAN_POINT('Ctrl Pts',(-10.8037192500001,11.6,1.13069018799999));
#259438=CARTESIAN_POINT('Ctrl Pts',(-10.8064540680001,15.2,1.13011116799999));
#259439=CARTESIAN_POINT('Ctrl Pts',(-10.8064540680001,11.6,1.13011116799999));
#259440=CARTESIAN_POINT('Ctrl Pts',(-10.8091939670001,15.2,1.12952867799998));
#259441=CARTESIAN_POINT('Ctrl Pts',(-10.8091939670001,11.6,1.12952867799998));
#259442=CARTESIAN_POINT('Ctrl Pts',(-10.8119389340001,15.2,1.12894271399998));
#259443=CARTESIAN_POINT('Ctrl Pts',(-10.8119389340001,11.6,1.12894271399998));
#259444=CARTESIAN_POINT('Ctrl Pts',(-10.8146889590001,15.2,1.12835326899999));
#259445=CARTESIAN_POINT('Ctrl Pts',(-10.8146889590001,11.6,1.12835326899999));
#259446=CARTESIAN_POINT('Ctrl Pts',(-10.8174440290001,15.2,1.12776033899999));
#259447=CARTESIAN_POINT('Ctrl Pts',(-10.8174440290001,11.6,1.12776033899999));
#259448=CARTESIAN_POINT('Ctrl Pts',(-10.8202041310001,15.2,1.12716391599998));
#259449=CARTESIAN_POINT('Ctrl Pts',(-10.8202041310001,11.6,1.12716391599998));
#259450=CARTESIAN_POINT('Ctrl Pts',(-10.8229692560001,15.2,1.12656399699999));
#259451=CARTESIAN_POINT('Ctrl Pts',(-10.8229692560001,11.6,1.12656399699999));
#259452=CARTESIAN_POINT('Ctrl Pts',(-10.8257393900001,15.2,1.12596057199998));
#259453=CARTESIAN_POINT('Ctrl Pts',(-10.8257393900001,11.6,1.12596057199998));
#259454=CARTESIAN_POINT('Ctrl Pts',(-10.8285145220001,15.2,1.12535363899998));
#259455=CARTESIAN_POINT('Ctrl Pts',(-10.8285145220001,11.6,1.12535363899998));
#259456=CARTESIAN_POINT('Ctrl Pts',(-10.8312946400001,15.2,1.12474319099999));
#259457=CARTESIAN_POINT('Ctrl Pts',(-10.8312946400001,11.6,1.12474319099999));
#259458=CARTESIAN_POINT('Ctrl Pts',(-10.8340797320001,15.2,1.12412922199999));
#259459=CARTESIAN_POINT('Ctrl Pts',(-10.8340797320001,11.6,1.12412922199998));
#259460=CARTESIAN_POINT('Ctrl Pts',(-10.8368697870001,15.2,1.12351172799999));
#259461=CARTESIAN_POINT('Ctrl Pts',(-10.8368697870001,11.6,1.12351172799999));
#259462=CARTESIAN_POINT('Ctrl Pts',(-10.8396647920001,15.2,1.12289069999999));
#259463=CARTESIAN_POINT('Ctrl Pts',(-10.8396647920001,11.6,1.12289069999999));
#259464=CARTESIAN_POINT('Ctrl Pts',(-10.8424647370001,15.2,1.12226613499999));
#259465=CARTESIAN_POINT('Ctrl Pts',(-10.8424647370001,11.6,1.12226613499998));
#259466=CARTESIAN_POINT('Ctrl Pts',(-10.8452696110001,15.2,1.12163802799999));
#259467=CARTESIAN_POINT('Ctrl Pts',(-10.8452696110001,11.6,1.12163802799999));
#259468=CARTESIAN_POINT('Ctrl Pts',(-10.8480794000001,15.2,1.12100637199998));
#259469=CARTESIAN_POINT('Ctrl Pts',(-10.8480794000001,11.6,1.12100637199998));
#259470=CARTESIAN_POINT('Ctrl Pts',(-10.8508940940001,15.2,1.12037116099998));
#259471=CARTESIAN_POINT('Ctrl Pts',(-10.8508940940001,11.6,1.12037116099998));
#259472=CARTESIAN_POINT('Ctrl Pts',(-10.8537136800001,15.2,1.11973238999999));
#259473=CARTESIAN_POINT('Ctrl Pts',(-10.8537136800001,11.6,1.11973238999999));
#259474=CARTESIAN_POINT('Ctrl Pts',(-10.8565381480001,15.2,1.11909005299998));
#259475=CARTESIAN_POINT('Ctrl Pts',(-10.8565381480001,11.6,1.11909005299998));
#259476=CARTESIAN_POINT('Ctrl Pts',(-10.8593674860001,15.2,1.11844414699998));
#259477=CARTESIAN_POINT('Ctrl Pts',(-10.8593674860001,11.6,1.11844414699998));
#259478=CARTESIAN_POINT('Ctrl Pts',(-10.8622016830001,15.2,1.11779466399998));
#259479=CARTESIAN_POINT('Ctrl Pts',(-10.8622016830001,11.6,1.11779466399998));
#259480=CARTESIAN_POINT('Ctrl Pts',(-10.8650407270001,15.2,1.11714159799998));
#259481=CARTESIAN_POINT('Ctrl Pts',(-10.8650407270001,11.6,1.11714159799998));
#259482=CARTESIAN_POINT('Ctrl Pts',(-10.8678846060001,15.2,1.11648494599998));
#259483=CARTESIAN_POINT('Ctrl Pts',(-10.8678846060001,11.6,1.11648494599998));
#259484=CARTESIAN_POINT('Ctrl Pts',(-10.8707333090001,15.2,1.11582469999998));
#259485=CARTESIAN_POINT('Ctrl Pts',(-10.8707333090001,11.6,1.11582469999998));
#259486=CARTESIAN_POINT('Ctrl Pts',(-10.8735868260001,15.2,1.11516085799999));
#259487=CARTESIAN_POINT('Ctrl Pts',(-10.8735868260001,11.6,1.11516085799999));
#259488=CARTESIAN_POINT('Ctrl Pts',(-10.8764451420001,15.2,1.11449341099998));
#259489=CARTESIAN_POINT('Ctrl Pts',(-10.8764451420001,11.6,1.11449341099998));
#259490=CARTESIAN_POINT('Ctrl Pts',(-10.8793082490001,15.2,1.11382235599998));
#259491=CARTESIAN_POINT('Ctrl Pts',(-10.8793082490001,11.6,1.11382235599998));
#259492=CARTESIAN_POINT('Ctrl Pts',(-10.8821761360001,15.2,1.11314768799998));
#259493=CARTESIAN_POINT('Ctrl Pts',(-10.8821761360001,11.6,1.11314768799998));
#259494=CARTESIAN_POINT('Ctrl Pts',(-10.8850487880001,15.2,1.11246939899999));
#259495=CARTESIAN_POINT('Ctrl Pts',(-10.8850487880001,11.6,1.11246939899999));
#259496=CARTESIAN_POINT('Ctrl Pts',(-10.8879261980001,15.2,1.11178748499999));
#259497=CARTESIAN_POINT('Ctrl Pts',(-10.8879261980001,11.6,1.11178748499999));
#259498=CARTESIAN_POINT('Ctrl Pts',(-10.8908083520001,15.2,1.11110194299998));
#259499=CARTESIAN_POINT('Ctrl Pts',(-10.8908083520001,11.6,1.11110194299998));
#259500=CARTESIAN_POINT('Ctrl Pts',(-10.8936952400001,15.2,1.11041276499999));
#259501=CARTESIAN_POINT('Ctrl Pts',(-10.8936952400001,11.6,1.11041276499999));
#259502=CARTESIAN_POINT('Ctrl Pts',(-10.8965868490001,15.2,1.10971994599999));
#259503=CARTESIAN_POINT('Ctrl Pts',(-10.8965868490001,11.6,1.10971994599998));
#259504=CARTESIAN_POINT('Ctrl Pts',(-10.8994831710001,15.2,1.10902348199998));
#259505=CARTESIAN_POINT('Ctrl Pts',(-10.8994831710001,11.6,1.10902348199998));
#259506=CARTESIAN_POINT('Ctrl Pts',(-10.9023841920001,15.2,1.10832336799998));
#259507=CARTESIAN_POINT('Ctrl Pts',(-10.9023841920001,11.6,1.10832336799998));
#259508=CARTESIAN_POINT('Ctrl Pts',(-10.9052899020001,15.2,1.10761959699999));
#259509=CARTESIAN_POINT('Ctrl Pts',(-10.9052899020001,11.6,1.10761959699999));
#259510=CARTESIAN_POINT('Ctrl Pts',(-10.9082002890001,15.2,1.10691216599998));
#259511=CARTESIAN_POINT('Ctrl Pts',(-10.9082002890001,11.6,1.10691216599998));
#259512=CARTESIAN_POINT('Ctrl Pts',(-10.9111153440001,15.2,1.10620106799999));
#259513=CARTESIAN_POINT('Ctrl Pts',(-10.9111153440001,11.6,1.10620106799999));
#259514=CARTESIAN_POINT('Ctrl Pts',(-10.9140350530001,15.2,1.10548629899998));
#259515=CARTESIAN_POINT('Ctrl Pts',(-10.9140350530001,11.6,1.10548629899998));
#259516=CARTESIAN_POINT('Ctrl Pts',(-10.9169594070001,15.2,1.10476785399999));
#259517=CARTESIAN_POINT('Ctrl Pts',(-10.9169594070001,11.6,1.10476785399999));
#259518=CARTESIAN_POINT('Ctrl Pts',(-10.9198883940001,15.2,1.10404572799998));
#259519=CARTESIAN_POINT('Ctrl Pts',(-10.9198883940001,11.6,1.10404572799998));
#259520=CARTESIAN_POINT('Ctrl Pts',(-10.9228220030001,15.2,1.10331991499999));
#259521=CARTESIAN_POINT('Ctrl Pts',(-10.9228220030001,11.6,1.10331991499998));
#259522=CARTESIAN_POINT('Ctrl Pts',(-10.9257602240001,15.2,1.10259041099999));
#259523=CARTESIAN_POINT('Ctrl Pts',(-10.9257602240001,11.6,1.10259041099999));
#259524=CARTESIAN_POINT('Ctrl Pts',(-10.9287030450001,15.2,1.10185720999999));
#259525=CARTESIAN_POINT('Ctrl Pts',(-10.9287030450001,11.6,1.10185720999999));
#259526=CARTESIAN_POINT('Ctrl Pts',(-10.9316504550001,15.2,1.10112030799999));
#259527=CARTESIAN_POINT('Ctrl Pts',(-10.9316504550001,11.6,1.10112030799998));
#259528=CARTESIAN_POINT('Ctrl Pts',(-10.9346024440001,15.2,1.10037969999999));
#259529=CARTESIAN_POINT('Ctrl Pts',(-10.9346024440001,11.6,1.10037969999999));
#259530=CARTESIAN_POINT('Ctrl Pts',(-10.9375590010001,15.2,1.09963537999999));
#259531=CARTESIAN_POINT('Ctrl Pts',(-10.9375590010001,11.6,1.09963537999999));
#259532=CARTESIAN_POINT('Ctrl Pts',(-10.9405201130001,15.2,1.09888734399998));
#259533=CARTESIAN_POINT('Ctrl Pts',(-10.9405201130001,11.6,1.09888734399998));
#259534=CARTESIAN_POINT('Ctrl Pts',(-10.9434857720001,15.2,1.09813558799999));
#259535=CARTESIAN_POINT('Ctrl Pts',(-10.9434857720001,11.6,1.09813558799999));
#259536=CARTESIAN_POINT('Ctrl Pts',(-10.9464559650001,15.2,1.09738010499999));
#259537=CARTESIAN_POINT('Ctrl Pts',(-10.9464559650001,11.6,1.09738010499999));
#259538=CARTESIAN_POINT('Ctrl Pts',(-10.9494306820001,15.2,1.09662089099999));
#259539=CARTESIAN_POINT('Ctrl Pts',(-10.9494306820001,11.6,1.09662089099999));
#259540=CARTESIAN_POINT('Ctrl Pts',(-10.9524099120001,15.2,1.09585794199999));
#259541=CARTESIAN_POINT('Ctrl Pts',(-10.9524099120001,11.6,1.09585794199999));
#259542=CARTESIAN_POINT('Ctrl Pts',(-10.9553936450001,15.2,1.09509125199999));
#259543=CARTESIAN_POINT('Ctrl Pts',(-10.9553936450001,11.6,1.09509125199999));
#259544=CARTESIAN_POINT('Ctrl Pts',(-10.9583818690001,15.2,1.09432081699998));
#259545=CARTESIAN_POINT('Ctrl Pts',(-10.9583818690001,11.6,1.09432081699998));
#259546=CARTESIAN_POINT('Ctrl Pts',(-10.9613745740001,15.2,1.09354663099999));
#259547=CARTESIAN_POINT('Ctrl Pts',(-10.9613745740001,11.6,1.09354663099999));
#259548=CARTESIAN_POINT('Ctrl Pts',(-10.9643717480001,15.2,1.09276869099999));
#259549=CARTESIAN_POINT('Ctrl Pts',(-10.9643717480001,11.6,1.09276869099999));
#259550=CARTESIAN_POINT('Ctrl Pts',(-10.9673733820001,15.2,1.09198699199998));
#259551=CARTESIAN_POINT('Ctrl Pts',(-10.9673733820001,11.6,1.09198699199998));
#259552=CARTESIAN_POINT('Ctrl Pts',(-10.9703794650001,15.2,1.09120152799999));
#259553=CARTESIAN_POINT('Ctrl Pts',(-10.9703794650001,11.6,1.09120152799999));
#259554=CARTESIAN_POINT('Ctrl Pts',(-10.9733899850001,15.2,1.09041229499999));
#259555=CARTESIAN_POINT('Ctrl Pts',(-10.9733899850001,11.6,1.09041229499998));
#259556=CARTESIAN_POINT('Ctrl Pts',(-10.9764049340001,15.2,1.08961928699999));
#259557=CARTESIAN_POINT('Ctrl Pts',(-10.9764049340001,11.6,1.08961928699999));
#259558=CARTESIAN_POINT('Ctrl Pts',(-10.9794242980001,15.2,1.08882250199999));
#259559=CARTESIAN_POINT('Ctrl Pts',(-10.9794242980001,11.6,1.08882250199999));
#259560=CARTESIAN_POINT('Ctrl Pts',(-10.9824480680001,15.2,1.08802193399999));
#259561=CARTESIAN_POINT('Ctrl Pts',(-10.9824480680001,11.6,1.08802193399998));
#259562=CARTESIAN_POINT('Ctrl Pts',(-10.9854762340001,15.2,1.08721757799998));
#259563=CARTESIAN_POINT('Ctrl Pts',(-10.9854762340001,11.6,1.08721757799998));
#259564=CARTESIAN_POINT('Ctrl Pts',(-10.9885087840001,15.2,1.08640942999998));
#259565=CARTESIAN_POINT('Ctrl Pts',(-10.9885087840001,11.6,1.08640942999998));
#259566=CARTESIAN_POINT('Ctrl Pts',(-10.9915457090001,15.2,1.08559748499998));
#259567=CARTESIAN_POINT('Ctrl Pts',(-10.9915457090001,11.6,1.08559748499998));
#259568=CARTESIAN_POINT('Ctrl Pts',(-10.9945869970001,15.2,1.08478173799998));
#259569=CARTESIAN_POINT('Ctrl Pts',(-10.9945869970001,11.6,1.08478173799998));
#259570=CARTESIAN_POINT('Ctrl Pts',(-10.9976326380001,15.2,1.08396218499998));
#259571=CARTESIAN_POINT('Ctrl Pts',(-10.9976326380001,11.6,1.08396218499998));
#259572=CARTESIAN_POINT('Ctrl Pts',(-11.0006826220001,15.2,1.08313882099999));
#259573=CARTESIAN_POINT('Ctrl Pts',(-11.0006826220001,11.6,1.08313882099999));
#259574=CARTESIAN_POINT('Ctrl Pts',(-11.0037369370001,15.2,1.08231164299998));
#259575=CARTESIAN_POINT('Ctrl Pts',(-11.0037369370001,11.6,1.08231164299998));
#259576=CARTESIAN_POINT('Ctrl Pts',(-11.0067955760001,15.2,1.08148064399999));
#259577=CARTESIAN_POINT('Ctrl Pts',(-11.0067955760001,11.6,1.08148064399999));
#259578=CARTESIAN_POINT('Ctrl Pts',(-11.0098585240001,15.2,1.08064582099999));
#259579=CARTESIAN_POINT('Ctrl Pts',(-11.0098585240001,11.6,1.08064582099999));
#259580=CARTESIAN_POINT('Ctrl Pts',(-11.0129257730001,15.2,1.07980717099998));
#259581=CARTESIAN_POINT('Ctrl Pts',(-11.0129257730001,11.6,1.07980717099998));
#259582=CARTESIAN_POINT('Ctrl Pts',(-11.0159973130001,15.2,1.07896468599999));
#259583=CARTESIAN_POINT('Ctrl Pts',(-11.0159973130001,11.6,1.07896468599999));
#259584=CARTESIAN_POINT('Ctrl Pts',(-11.0190731330001,15.2,1.07811836399998));
#259585=CARTESIAN_POINT('Ctrl Pts',(-11.0190731330001,11.6,1.07811836399998));
#259586=CARTESIAN_POINT('Ctrl Pts',(-11.0221532220001,15.2,1.07726820099999));
#259587=CARTESIAN_POINT('Ctrl Pts',(-11.0221532220001,11.6,1.07726820099999));
#259588=CARTESIAN_POINT('Ctrl Pts',(-11.0252375700001,15.2,1.07641418999998));
#259589=CARTESIAN_POINT('Ctrl Pts',(-11.0252375700001,11.6,1.07641418999998));
#259590=CARTESIAN_POINT('Ctrl Pts',(-11.0283261660001,15.2,1.07555632999999));
#259591=CARTESIAN_POINT('Ctrl Pts',(-11.0283261660001,11.6,1.07555632999999));
#259592=CARTESIAN_POINT('Ctrl Pts',(-11.0314190020001,15.2,1.07469461299999));
#259593=CARTESIAN_POINT('Ctrl Pts',(-11.0314190020001,11.6,1.07469461299999));
#259594=CARTESIAN_POINT('Ctrl Pts',(-11.0345160640001,15.2,1.07382903799999));
#259595=CARTESIAN_POINT('Ctrl Pts',(-11.0345160640001,11.6,1.07382903799999));
#259596=CARTESIAN_POINT('Ctrl Pts',(-11.0376173460001,15.2,1.07295959799998));
#259597=CARTESIAN_POINT('Ctrl Pts',(-11.0376173460001,11.6,1.07295959799998));
#259598=CARTESIAN_POINT('Ctrl Pts',(-11.0407228350001,15.2,1.07208629099999));
#259599=CARTESIAN_POINT('Ctrl Pts',(-11.0407228350001,11.6,1.07208629099999));
#259600=CARTESIAN_POINT('Ctrl Pts',(-11.0438325210001,15.2,1.07120911099999));
#259601=CARTESIAN_POINT('Ctrl Pts',(-11.0438325210001,11.6,1.07120911099999));
#259602=CARTESIAN_POINT('Ctrl Pts',(-11.0469463940001,15.2,1.07032805399998));
#259603=CARTESIAN_POINT('Ctrl Pts',(-11.0469463940001,11.6,1.07032805399998));
#259604=CARTESIAN_POINT('Ctrl Pts',(-11.0500644440001,15.2,1.06944311599999));
#259605=CARTESIAN_POINT('Ctrl Pts',(-11.0500644440001,11.6,1.06944311599999));
#259606=CARTESIAN_POINT('Ctrl Pts',(-11.0531866600001,15.2,1.06855429399999));
#259607=CARTESIAN_POINT('Ctrl Pts',(-11.0531866600001,11.6,1.06855429399999));
#259608=CARTESIAN_POINT('Ctrl Pts',(-11.0563130330001,15.2,1.06766158099999));
#259609=CARTESIAN_POINT('Ctrl Pts',(-11.0563130330001,11.6,1.06766158099999));
#259610=CARTESIAN_POINT('Ctrl Pts',(-11.0594435520001,15.2,1.06676497499999));
#259611=CARTESIAN_POINT('Ctrl Pts',(-11.0594435520001,11.6,1.06676497499999));
#259612=CARTESIAN_POINT('Ctrl Pts',(-11.0625782070001,15.2,1.06586446999998));
#259613=CARTESIAN_POINT('Ctrl Pts',(-11.0625782070001,11.6,1.06586446999998));
#259614=CARTESIAN_POINT('Ctrl Pts',(-11.0657169880001,15.2,1.06496006399999));
#259615=CARTESIAN_POINT('Ctrl Pts',(-11.0657169880001,11.6,1.06496006399999));
#259616=CARTESIAN_POINT('Ctrl Pts',(-11.0688598860001,15.2,1.06405175099999));
#259617=CARTESIAN_POINT('Ctrl Pts',(-11.0688598860001,11.6,1.06405175099999));
#259618=CARTESIAN_POINT('Ctrl Pts',(-11.0720068880001,15.2,1.06313952799999));
#259619=CARTESIAN_POINT('Ctrl Pts',(-11.0720068880001,11.6,1.06313952799999));
#259620=CARTESIAN_POINT('Ctrl Pts',(-11.0751579870001,15.2,1.06222338999999));
#259621=CARTESIAN_POINT('Ctrl Pts',(-11.0751579870001,11.6,1.06222338999999));
#259622=CARTESIAN_POINT('Ctrl Pts',(-11.0783131710001,15.2,1.06130333499999));
#259623=CARTESIAN_POINT('Ctrl Pts',(-11.0783131710001,11.6,1.06130333499999));
#259624=CARTESIAN_POINT('Ctrl Pts',(-11.0814724300001,15.2,1.06037935499999));
#259625=CARTESIAN_POINT('Ctrl Pts',(-11.0814724300001,11.6,1.06037935499998));
#259626=CARTESIAN_POINT('Ctrl Pts',(-11.0846357550001,15.2,1.05945144899998));
#259627=CARTESIAN_POINT('Ctrl Pts',(-11.0846357550001,11.6,1.05945144899998));
#259628=CARTESIAN_POINT('Ctrl Pts',(-11.0878031360001,15.2,1.05851961199999));
#259629=CARTESIAN_POINT('Ctrl Pts',(-11.0878031360001,11.6,1.05851961199999));
#259630=CARTESIAN_POINT('Ctrl Pts',(-11.0909745620001,15.2,1.05758383999999));
#259631=CARTESIAN_POINT('Ctrl Pts',(-11.0909745620001,11.6,1.05758383999999));
#259632=CARTESIAN_POINT('Ctrl Pts',(-11.0941500240001,15.2,1.05664412899999));
#259633=CARTESIAN_POINT('Ctrl Pts',(-11.0941500240001,11.6,1.05664412899999));
#259634=CARTESIAN_POINT('Ctrl Pts',(-11.0973295110001,15.2,1.05570047499999));
#259635=CARTESIAN_POINT('Ctrl Pts',(-11.0973295110001,11.6,1.05570047499999));
#259636=CARTESIAN_POINT('Ctrl Pts',(-11.1005130140001,15.2,1.05475287299999));
#259637=CARTESIAN_POINT('Ctrl Pts',(-11.1005130140001,11.6,1.05475287299999));
#259638=CARTESIAN_POINT('Ctrl Pts',(-11.1037005220001,15.2,1.05380132099999));
#259639=CARTESIAN_POINT('Ctrl Pts',(-11.1037005220001,11.6,1.05380132099999));
#259640=CARTESIAN_POINT('Ctrl Pts',(-11.1068920250001,15.2,1.05284581399999));
#259641=CARTESIAN_POINT('Ctrl Pts',(-11.1068920250001,11.6,1.05284581399998));
#259642=CARTESIAN_POINT('Ctrl Pts',(-11.1100875160001,15.2,1.05188634799998));
#259643=CARTESIAN_POINT('Ctrl Pts',(-11.1100875160001,11.6,1.05188634799998));
#259644=CARTESIAN_POINT('Ctrl Pts',(-11.1132869810001,15.2,1.05092291799998));
#259645=CARTESIAN_POINT('Ctrl Pts',(-11.1132869810001,11.6,1.05092291799998));
#259646=CARTESIAN_POINT('Ctrl Pts',(-11.1164904140001,15.2,1.04995552199998));
#259647=CARTESIAN_POINT('Ctrl Pts',(-11.1164904140001,11.6,1.04995552199998));
#259648=CARTESIAN_POINT('Ctrl Pts',(-11.1196978020001,15.2,1.04898415499999));
#259649=CARTESIAN_POINT('Ctrl Pts',(-11.1196978020001,11.6,1.04898415499999));
#259650=CARTESIAN_POINT('Ctrl Pts',(-11.1229091360001,15.2,1.04800881199999));
#259651=CARTESIAN_POINT('Ctrl Pts',(-11.1229091360001,11.6,1.04800881199999));
#259652=CARTESIAN_POINT('Ctrl Pts',(-11.1261244080001,15.2,1.04702949099998));
#259653=CARTESIAN_POINT('Ctrl Pts',(-11.1261244080001,11.6,1.04702949099998));
#259654=CARTESIAN_POINT('Ctrl Pts',(-11.1293436050001,15.2,1.04604618899999));
#259655=CARTESIAN_POINT('Ctrl Pts',(-11.1293436050001,11.6,1.04604618899998));
#259656=CARTESIAN_POINT('Ctrl Pts',(-11.1325667200001,15.2,1.04505889899999));
#259657=CARTESIAN_POINT('Ctrl Pts',(-11.1325667200001,11.6,1.04505889899999));
#259658=CARTESIAN_POINT('Ctrl Pts',(-11.1357937420001,15.2,1.04406762099998));
#259659=CARTESIAN_POINT('Ctrl Pts',(-11.1357937420001,11.6,1.04406762099998));
#259660=CARTESIAN_POINT('Ctrl Pts',(-11.1390246620001,15.2,1.04307234699998));
#259661=CARTESIAN_POINT('Ctrl Pts',(-11.1390246620001,11.6,1.04307234699998));
#259662=CARTESIAN_POINT('Ctrl Pts',(-11.1422594690001,15.2,1.04207307599999));
#259663=CARTESIAN_POINT('Ctrl Pts',(-11.1422594690001,11.6,1.04207307599998));
#259664=CARTESIAN_POINT('Ctrl Pts',(-11.1454981540001,15.2,1.04106980299999));
#259665=CARTESIAN_POINT('Ctrl Pts',(-11.1454981540001,11.6,1.04106980299999));
#259666=CARTESIAN_POINT('Ctrl Pts',(-11.1487407070001,15.2,1.04006252499998));
#259667=CARTESIAN_POINT('Ctrl Pts',(-11.1487407070001,11.6,1.04006252499998));
#259668=CARTESIAN_POINT('Ctrl Pts',(-11.1519871190001,15.2,1.03905123799999));
#259669=CARTESIAN_POINT('Ctrl Pts',(-11.1519871190001,11.6,1.03905123799999));
#259670=CARTESIAN_POINT('Ctrl Pts',(-11.1552373810001,15.2,1.03803593699999));
#259671=CARTESIAN_POINT('Ctrl Pts',(-11.1552373810001,11.6,1.03803593699999));
#259672=CARTESIAN_POINT('Ctrl Pts',(-11.1584914810001,15.2,1.03701662199999));
#259673=CARTESIAN_POINT('Ctrl Pts',(-11.1584914810001,11.6,1.03701662199999));
#259674=CARTESIAN_POINT('Ctrl Pts',(-11.1617494110001,15.2,1.03599328399998));
#259675=CARTESIAN_POINT('Ctrl Pts',(-11.1617494110001,11.6,1.03599328399998));
#259676=CARTESIAN_POINT('Ctrl Pts',(-11.1650111610001,15.2,1.03496592399999));
#259677=CARTESIAN_POINT('Ctrl Pts',(-11.1650111610001,11.6,1.03496592399999));
#259678=CARTESIAN_POINT('Ctrl Pts',(-11.1682767210001,15.2,1.03393453499999));
#259679=CARTESIAN_POINT('Ctrl Pts',(-11.1682767210001,11.6,1.03393453499998));
#259680=CARTESIAN_POINT('Ctrl Pts',(-11.1715460820001,15.2,1.03289911399999));
#259681=CARTESIAN_POINT('Ctrl Pts',(-11.1715460820001,11.6,1.03289911399999));
#259682=CARTESIAN_POINT('Ctrl Pts',(-11.1748192350001,15.2,1.03185965899999));
#259683=CARTESIAN_POINT('Ctrl Pts',(-11.1748192350001,11.6,1.03185965899998));
#259684=CARTESIAN_POINT('Ctrl Pts',(-11.1780961680001,15.2,1.03081616499999));
#259685=CARTESIAN_POINT('Ctrl Pts',(-11.1780961680001,11.6,1.03081616499999));
#259686=CARTESIAN_POINT('Ctrl Pts',(-11.1813768730001,15.2,1.02976862899999));
#259687=CARTESIAN_POINT('Ctrl Pts',(-11.1813768730001,11.6,1.02976862899998));
#259688=CARTESIAN_POINT('Ctrl Pts',(-11.1846613420001,15.2,1.02871704699998));
#259689=CARTESIAN_POINT('Ctrl Pts',(-11.1846613420001,11.6,1.02871704699998));
#259690=CARTESIAN_POINT('Ctrl Pts',(-11.1879495640001,15.2,1.02766141599998));
#259691=CARTESIAN_POINT('Ctrl Pts',(-11.1879495640001,11.6,1.02766141599998));
#259692=CARTESIAN_POINT('Ctrl Pts',(-11.1912415290001,15.2,1.02660173099999));
#259693=CARTESIAN_POINT('Ctrl Pts',(-11.1912415290001,11.6,1.02660173099998));
#259694=CARTESIAN_POINT('Ctrl Pts',(-11.1945372270001,15.2,1.02553798999999));
#259695=CARTESIAN_POINT('Ctrl Pts',(-11.1945372270001,11.6,1.02553798999998));
#259696=CARTESIAN_POINT('Ctrl Pts',(-11.1978366510001,15.2,1.02447018799999));
#259697=CARTESIAN_POINT('Ctrl Pts',(-11.1978366510001,11.6,1.02447018799999));
#259698=CARTESIAN_POINT('Ctrl Pts',(-11.2011397890001,15.2,1.02339832299998));
#259699=CARTESIAN_POINT('Ctrl Pts',(-11.2011397890001,11.6,1.02339832299998));
#259700=CARTESIAN_POINT('Ctrl Pts',(-11.2044466330001,15.2,1.02232238999999));
#259701=CARTESIAN_POINT('Ctrl Pts',(-11.2044466330001,11.6,1.02232238999999));
#259702=CARTESIAN_POINT('Ctrl Pts',(-11.2077571730001,15.2,1.02124238699998));
#259703=CARTESIAN_POINT('Ctrl Pts',(-11.2077571730001,11.6,1.02124238699998));
#259704=CARTESIAN_POINT('Ctrl Pts',(-11.2110714010001,15.2,1.02015830899999));
#259705=CARTESIAN_POINT('Ctrl Pts',(-11.2110714010001,11.6,1.02015830899999));
#259706=CARTESIAN_POINT('Ctrl Pts',(-11.2143893040001,15.2,1.01907015299998));
#259707=CARTESIAN_POINT('Ctrl Pts',(-11.2143893040001,11.6,1.01907015299998));
#259708=CARTESIAN_POINT('Ctrl Pts',(-11.2177108770001,15.2,1.01797791699999));
#259709=CARTESIAN_POINT('Ctrl Pts',(-11.2177108770001,11.6,1.01797791699999));
#259710=CARTESIAN_POINT('Ctrl Pts',(-11.2210361080001,15.2,1.01688159599998));
#259711=CARTESIAN_POINT('Ctrl Pts',(-11.2210361080001,11.6,1.01688159599998));
#259712=CARTESIAN_POINT('Ctrl Pts',(-11.2243649880001,15.2,1.01578118599999));
#259713=CARTESIAN_POINT('Ctrl Pts',(-11.2243649880001,11.6,1.01578118599999));
#259714=CARTESIAN_POINT('Ctrl Pts',(-11.2276975070001,15.2,1.01467668399998));
#259715=CARTESIAN_POINT('Ctrl Pts',(-11.2276975070001,11.6,1.01467668399998));
#259716=CARTESIAN_POINT('Ctrl Pts',(-11.2310336580001,15.2,1.01356808799999));
#259717=CARTESIAN_POINT('Ctrl Pts',(-11.2310336580001,11.6,1.01356808799998));
#259718=CARTESIAN_POINT('Ctrl Pts',(-11.2343734290001,15.2,1.01245539299998));
#259719=CARTESIAN_POINT('Ctrl Pts',(-11.2343734290001,11.6,1.01245539299998));
#259720=CARTESIAN_POINT('Ctrl Pts',(-11.2377168140001,15.2,1.01133859799999));
#259721=CARTESIAN_POINT('Ctrl Pts',(-11.2377168140001,11.6,1.01133859799999));
#259722=CARTESIAN_POINT('Ctrl Pts',(-11.2410637990001,15.2,1.01021769499999));
#259723=CARTESIAN_POINT('Ctrl Pts',(-11.2410637990001,11.6,1.01021769499999));
#259724=CARTESIAN_POINT('Ctrl Pts',(-11.2444143790001,15.2,1.00909268499999));
#259725=CARTESIAN_POINT('Ctrl Pts',(-11.2444143790001,11.6,1.00909268499999));
#259726=CARTESIAN_POINT('Ctrl Pts',(-11.2477685430001,15.2,1.00796356299998));
#259727=CARTESIAN_POINT('Ctrl Pts',(-11.2477685430001,11.6,1.00796356299998));
#259728=CARTESIAN_POINT('Ctrl Pts',(-11.2511262810001,15.2,1.00683032499999));
#259729=CARTESIAN_POINT('Ctrl Pts',(-11.2511262810001,11.6,1.00683032499999));
#259730=CARTESIAN_POINT('Ctrl Pts',(-11.2544875850001,15.2,1.00569296999999));
#259731=CARTESIAN_POINT('Ctrl Pts',(-11.2544875850001,11.6,1.00569296999998));
#259732=CARTESIAN_POINT('Ctrl Pts',(-11.2578524460001,15.2,1.00455149199998));
#259733=CARTESIAN_POINT('Ctrl Pts',(-11.2578524460001,11.6,1.00455149199998));
#259734=CARTESIAN_POINT('Ctrl Pts',(-11.2612208540001,15.2,1.00340588999998));
#259735=CARTESIAN_POINT('Ctrl Pts',(-11.2612208540001,11.6,1.00340588999998));
#259736=CARTESIAN_POINT('Ctrl Pts',(-11.2645927990001,15.2,1.00225615799999));
#259737=CARTESIAN_POINT('Ctrl Pts',(-11.2645927990001,11.6,1.00225615799999));
#259738=CARTESIAN_POINT('Ctrl Pts',(-11.2679682740001,15.2,1.00110229499998));
#259739=CARTESIAN_POINT('Ctrl Pts',(-11.2679682740001,11.6,1.00110229499998));
#259740=CARTESIAN_POINT('Ctrl Pts',(-11.2713472680001,15.2,0.999944296999988));
#259741=CARTESIAN_POINT('Ctrl Pts',(-11.2713472680001,11.6,0.999944296999988));
#259742=CARTESIAN_POINT('Ctrl Pts',(-11.2747297730001,15.2,0.998782160999987));
#259743=CARTESIAN_POINT('Ctrl Pts',(-11.2747297730001,11.6,0.998782160999987));
#259744=CARTESIAN_POINT('Ctrl Pts',(-11.2781157800001,15.2,0.997615882999985));
#259745=CARTESIAN_POINT('Ctrl Pts',(-11.2781157800001,11.6,0.997615882999984));
#259746=CARTESIAN_POINT('Ctrl Pts',(-11.2815052780001,15.2,0.996445461999986));
#259747=CARTESIAN_POINT('Ctrl Pts',(-11.2815052780001,11.6,0.996445461999986));
#259748=CARTESIAN_POINT('Ctrl Pts',(-11.2848982590001,15.2,0.995270892999987));
#259749=CARTESIAN_POINT('Ctrl Pts',(-11.2848982590001,11.6,0.995270892999986));
#259750=CARTESIAN_POINT('Ctrl Pts',(-11.2882947150001,15.2,0.994092171999985));
#259751=CARTESIAN_POINT('Ctrl Pts',(-11.2882947150001,11.6,0.994092171999985));
#259752=CARTESIAN_POINT('Ctrl Pts',(-11.2916946350001,15.2,0.992909295999986));
#259753=CARTESIAN_POINT('Ctrl Pts',(-11.2916946350001,11.6,0.992909295999986));
#259754=CARTESIAN_POINT('Ctrl Pts',(-11.2950980120001,15.2,0.991722263999986));
#259755=CARTESIAN_POINT('Ctrl Pts',(-11.2950980120001,11.6,0.991722263999985));
#259756=CARTESIAN_POINT('Ctrl Pts',(-11.2985048360001,15.2,0.990531070999987));
#259757=CARTESIAN_POINT('Ctrl Pts',(-11.2985048360001,11.6,0.990531070999987));
#259758=CARTESIAN_POINT('Ctrl Pts',(-11.3019150960001,15.2,0.989335713999986));
#259759=CARTESIAN_POINT('Ctrl Pts',(-11.3019150960001,11.6,0.989335713999985));
#259760=CARTESIAN_POINT('Ctrl Pts',(-11.3053287860001,15.2,0.988136191999986));
#259761=CARTESIAN_POINT('Ctrl Pts',(-11.3053287860001,11.6,0.988136191999986));
#259762=CARTESIAN_POINT('Ctrl Pts',(-11.3087458960001,15.2,0.986932498999984));
#259763=CARTESIAN_POINT('Ctrl Pts',(-11.3087458960001,11.6,0.986932498999983));
#259764=CARTESIAN_POINT('Ctrl Pts',(-11.3121664170001,15.2,0.985724631999982));
#259765=CARTESIAN_POINT('Ctrl Pts',(-11.3121664170001,11.6,0.985724631999982));
#259766=CARTESIAN_POINT('Ctrl Pts',(-11.3155903390001,15.2,0.984512589999986));
#259767=CARTESIAN_POINT('Ctrl Pts',(-11.3155903390001,11.6,0.984512589999986));
#259768=CARTESIAN_POINT('Ctrl Pts',(-11.3190176540001,15.2,0.983296368999986));
#259769=CARTESIAN_POINT('Ctrl Pts',(-11.3190176540001,11.6,0.983296368999986));
#259770=CARTESIAN_POINT('Ctrl Pts',(-11.3224483530001,15.2,0.982075965999982));
#259771=CARTESIAN_POINT('Ctrl Pts',(-11.3224483530001,11.6,0.982075965999982));
#259772=CARTESIAN_POINT('Ctrl Pts',(-11.3258824260001,15.2,0.980851377999983));
#259773=CARTESIAN_POINT('Ctrl Pts',(-11.3258824260001,11.6,0.980851377999982));
#259774=CARTESIAN_POINT('Ctrl Pts',(-11.3293198660001,15.2,0.979622600999988));
#259775=CARTESIAN_POINT('Ctrl Pts',(-11.3293198660001,11.6,0.979622600999987));
#259776=CARTESIAN_POINT('Ctrl Pts',(-11.3327606630001,15.2,0.978389632999987));
#259777=CARTESIAN_POINT('Ctrl Pts',(-11.3327606630001,11.6,0.978389632999987));
#259778=CARTESIAN_POINT('Ctrl Pts',(-11.3362048080001,15.2,0.977152470999982));
#259779=CARTESIAN_POINT('Ctrl Pts',(-11.3362048080001,11.6,0.977152470999982));
#259780=CARTESIAN_POINT('Ctrl Pts',(-11.3396522920001,15.2,0.975911110999985));
#259781=CARTESIAN_POINT('Ctrl Pts',(-11.3396522920001,11.6,0.975911110999985));
#259782=CARTESIAN_POINT('Ctrl Pts',(-11.3431031070001,15.2,0.974665550999987));
#259783=CARTESIAN_POINT('Ctrl Pts',(-11.3431031070001,11.6,0.974665550999986));
#259784=CARTESIAN_POINT('Ctrl Pts',(-11.3465572430001,15.2,0.973415788999983));
#259785=CARTESIAN_POINT('Ctrl Pts',(-11.3465572430001,11.6,0.973415788999982));
#259786=CARTESIAN_POINT('Ctrl Pts',(-11.3500146920001,15.2,0.972161818999986));
#259787=CARTESIAN_POINT('Ctrl Pts',(-11.3500146920001,11.6,0.972161818999985));
#259788=CARTESIAN_POINT('Ctrl Pts',(-11.3534754440001,15.2,0.970903640999987));
#259789=CARTESIAN_POINT('Ctrl Pts',(-11.3534754440001,11.6,0.970903640999987));
#259790=CARTESIAN_POINT('Ctrl Pts',(-11.3569394920001,15.2,0.969641250999986));
#259791=CARTESIAN_POINT('Ctrl Pts',(-11.3569394920001,11.6,0.969641250999986));
#259792=CARTESIAN_POINT('Ctrl Pts',(-11.3604068260001,15.2,0.968374645999983));
#259793=CARTESIAN_POINT('Ctrl Pts',(-11.3604068260001,11.6,0.968374645999983));
#259794=CARTESIAN_POINT('Ctrl Pts',(-11.3638774360001,15.2,0.967103821999986));
#259795=CARTESIAN_POINT('Ctrl Pts',(-11.3638774360001,11.6,0.967103821999986));
#259796=CARTESIAN_POINT('Ctrl Pts',(-11.3673513150001,15.2,0.965828777999986));
#259797=CARTESIAN_POINT('Ctrl Pts',(-11.3673513150001,11.6,0.965828777999986));
#259798=CARTESIAN_POINT('Ctrl Pts',(-11.3708284530001,15.2,0.964549509999983));
#259799=CARTESIAN_POINT('Ctrl Pts',(-11.3708284530001,11.6,0.964549509999983));
#259800=CARTESIAN_POINT('Ctrl Pts',(-11.3743088440001,15.2,0.963266015999986));
#259801=CARTESIAN_POINT('Ctrl Pts',(-11.3743088440001,11.6,0.963266015999986));
#259802=CARTESIAN_POINT('Ctrl Pts',(-11.3777924770001,15.2,0.961978291999985));
#259803=CARTESIAN_POINT('Ctrl Pts',(-11.3777924770001,11.6,0.961978291999985));
#259804=CARTESIAN_POINT('Ctrl Pts',(-11.3812793430001,15.2,0.960686337999985));
#259805=CARTESIAN_POINT('Ctrl Pts',(-11.3812793430001,11.6,0.960686337999985));
#259806=CARTESIAN_POINT('Ctrl Pts',(-11.3847694350001,15.2,0.959390146999985));
#259807=CARTESIAN_POINT('Ctrl Pts',(-11.3847694350001,11.6,0.959390146999985));
#259808=CARTESIAN_POINT('Ctrl Pts',(-11.3882627430001,15.2,0.958089718999986));
#259809=CARTESIAN_POINT('Ctrl Pts',(-11.3882627430001,11.6,0.958089718999986));
#259810=CARTESIAN_POINT('Ctrl Pts',(-11.3917592580001,15.2,0.956785048999986));
#259811=CARTESIAN_POINT('Ctrl Pts',(-11.3917592580001,11.6,0.956785048999986));
#259812=CARTESIAN_POINT('Ctrl Pts',(-11.3952589700001,15.2,0.955476136999986));
#259813=CARTESIAN_POINT('Ctrl Pts',(-11.3952589700001,11.6,0.955476136999986));
#259814=CARTESIAN_POINT('Ctrl Pts',(-11.3987618720001,15.2,0.954162976999986));
#259815=CARTESIAN_POINT('Ctrl Pts',(-11.3987618720001,11.6,0.954162976999986));
#259816=CARTESIAN_POINT('Ctrl Pts',(-11.4022679530001,15.2,0.952845567999985));
#259817=CARTESIAN_POINT('Ctrl Pts',(-11.4022679530001,11.6,0.952845567999984));
#259818=CARTESIAN_POINT('Ctrl Pts',(-11.4057772070001,15.2,0.951523905999987));
#259819=CARTESIAN_POINT('Ctrl Pts',(-11.4057772070001,11.6,0.951523905999986));
#259820=CARTESIAN_POINT('Ctrl Pts',(-11.4092896250001,15.2,0.950197990999988));
#259821=CARTESIAN_POINT('Ctrl Pts',(-11.4092896250001,11.6,0.950197990999988));
#259822=CARTESIAN_POINT('Ctrl Pts',(-11.4128052000001,15.2,0.948867817999983));
#259823=CARTESIAN_POINT('Ctrl Pts',(-11.4128052000001,11.6,0.948867817999983));
#259824=CARTESIAN_POINT('Ctrl Pts',(-11.4163239240001,15.2,0.947533386999986));
#259825=CARTESIAN_POINT('Ctrl Pts',(-11.4163239240001,11.6,0.947533386999985));
#259826=CARTESIAN_POINT('Ctrl Pts',(-11.4198457890001,15.2,0.946194692999986));
#259827=CARTESIAN_POINT('Ctrl Pts',(-11.4198457890001,11.6,0.946194692999986));
#259828=CARTESIAN_POINT('Ctrl Pts',(-11.4233707840001,15.2,0.944851733999985));
#259829=CARTESIAN_POINT('Ctrl Pts',(-11.4233707840001,11.6,0.944851733999985));
#259830=CARTESIAN_POINT('Ctrl Pts',(-11.4268989030001,15.2,0.943504507999986));
#259831=CARTESIAN_POINT('Ctrl Pts',(-11.4268989030001,11.6,0.943504507999986));
#259832=CARTESIAN_POINT('Ctrl Pts',(-11.4304301310001,15.2,0.942153010999984));
#259833=CARTESIAN_POINT('Ctrl Pts',(-11.4304301310001,11.6,0.942153010999984));
#259834=CARTESIAN_POINT('Ctrl Pts',(-11.4339644600001,15.2,0.940797237999984));
#259835=CARTESIAN_POINT('Ctrl Pts',(-11.4339644600001,11.6,0.940797237999984));
#259836=CARTESIAN_POINT('Ctrl Pts',(-11.4375018800001,15.2,0.939437186999985));
#259837=CARTESIAN_POINT('Ctrl Pts',(-11.4375018800001,11.6,0.939437186999985));
#259838=CARTESIAN_POINT('Ctrl Pts',(-11.4410423790001,15.2,0.938072855999987));
#259839=CARTESIAN_POINT('Ctrl Pts',(-11.4410423790001,11.6,0.938072855999987));
#259840=CARTESIAN_POINT('Ctrl Pts',(-11.4445859520001,15.2,0.936704240999986));
#259841=CARTESIAN_POINT('Ctrl Pts',(-11.4445859520001,11.6,0.936704240999986));
#259842=CARTESIAN_POINT('Ctrl Pts',(-11.4481325920001,15.2,0.935331340999985));
#259843=CARTESIAN_POINT('Ctrl Pts',(-11.4481325920001,11.6,0.935331340999985));
#259844=CARTESIAN_POINT('Ctrl Pts',(-11.4516822960001,15.2,0.933954156999985));
#259845=CARTESIAN_POINT('Ctrl Pts',(-11.4516822960001,11.6,0.933954156999985));
#259846=CARTESIAN_POINT('Ctrl Pts',(-11.4552350600001,15.2,0.932572684999986));
#259847=CARTESIAN_POINT('Ctrl Pts',(-11.4552350600001,11.6,0.932572684999986));
#259848=CARTESIAN_POINT('Ctrl Pts',(-11.4580797200001,15.2,0.931464077999986));
#259849=CARTESIAN_POINT('Ctrl Pts',(-11.4580797200001,11.6,0.931464077999986));
#259850=CARTESIAN_POINT('Ctrl Pts',(-11.4602145910001,15.2,0.930630692999985));
#259851=CARTESIAN_POINT('Ctrl Pts',(-11.4602145910001,11.6,0.930630692999985));
#259852=CARTESIAN_POINT('Ctrl Pts',(-11.4616384500001,15.2,0.930074245999983));
#259853=CARTESIAN_POINT('Ctrl Pts',(-11.4616384500001,11.6,0.930074245999983));
#259854=CARTESIAN_POINT('Ctrl Pts',(-11.4623505340001,15.2,0.929795807999985));
#259855=CARTESIAN_POINT('Ctrl Pts',(-11.4623505340001,11.6,0.929795807999984));
#259856=CARTESIAN_POINT('Ctrl Pts',(-10.3068855240001,15.2,1.18690176599999));
#259857=CARTESIAN_POINT('Ctrl Pts',(-10.3070598110001,15.2,1.18690675299999));
#259858=CARTESIAN_POINT('Ctrl Pts',(-10.3074144740001,15.2,1.18691681599998));
#259859=CARTESIAN_POINT('Ctrl Pts',(-10.3079518800001,15.2,1.18693179799998));
#259860=CARTESIAN_POINT('Ctrl Pts',(-10.3086758300001,15.2,1.18695143999998));
#259861=CARTESIAN_POINT('Ctrl Pts',(-10.3095915440001,15.2,1.18697537099999));
#259862=CARTESIAN_POINT('Ctrl Pts',(-10.3105221240001,15.2,1.18699875499999));
#259863=CARTESIAN_POINT('Ctrl Pts',(-10.3114622390001,15.2,1.18702143499998));
#259864=CARTESIAN_POINT('Ctrl Pts',(-10.3124118610001,15.2,1.18704339399998));
#259865=CARTESIAN_POINT('Ctrl Pts',(-10.3133709660001,15.2,1.18706460899999));
#259866=CARTESIAN_POINT('Ctrl Pts',(-10.3143395250001,15.2,1.18708506599999));
#259867=CARTESIAN_POINT('Ctrl Pts',(-10.3153175130001,15.2,1.18710474299998));
#259868=CARTESIAN_POINT('Ctrl Pts',(-10.3163049050001,15.2,1.18712362399998));
#259869=CARTESIAN_POINT('Ctrl Pts',(-10.3173016730001,15.2,1.18714168899999));
#259870=CARTESIAN_POINT('Ctrl Pts',(-10.3183077930001,15.2,1.18715892099999));
#259871=CARTESIAN_POINT('Ctrl Pts',(-10.3193232400001,15.2,1.18717530199998));
#259872=CARTESIAN_POINT('Ctrl Pts',(-10.3203479850001,15.2,1.18719081299998));
#259873=CARTESIAN_POINT('Ctrl Pts',(-10.3213820050001,15.2,1.18720543699999));
#259874=CARTESIAN_POINT('Ctrl Pts',(-10.3224252740001,15.2,1.18721915599998));
#259875=CARTESIAN_POINT('Ctrl Pts',(-10.3234777680001,15.2,1.18723195099999));
#259876=CARTESIAN_POINT('Ctrl Pts',(-10.3245394590001,15.2,1.18724380599998));
#259877=CARTESIAN_POINT('Ctrl Pts',(-10.3256103250001,15.2,1.18725470399998));
#259878=CARTESIAN_POINT('Ctrl Pts',(-10.3266903400001,15.2,1.18726462499998));
#259879=CARTESIAN_POINT('Ctrl Pts',(-10.3277794780001,15.2,1.18727355499999));
#259880=CARTESIAN_POINT('Ctrl Pts',(-10.3288777160001,15.2,1.18728147399999));
#259881=CARTESIAN_POINT('Ctrl Pts',(-10.3299850290001,15.2,1.18728836599999));
#259882=CARTESIAN_POINT('Ctrl Pts',(-10.3311013920001,15.2,1.18729421399999));
#259883=CARTESIAN_POINT('Ctrl Pts',(-10.3322267810001,15.2,1.18729900199999));
#259884=CARTESIAN_POINT('Ctrl Pts',(-10.3333611710001,15.2,1.18730271099999));
#259885=CARTESIAN_POINT('Ctrl Pts',(-10.3345045400001,15.2,1.18730532599999));
#259886=CARTESIAN_POINT('Ctrl Pts',(-10.3356568620001,15.2,1.18730682999999));
#259887=CARTESIAN_POINT('Ctrl Pts',(-10.3368181130001,15.2,1.18730720599999));
#259888=CARTESIAN_POINT('Ctrl Pts',(-10.3379882700001,15.2,1.18730643699998));
#259889=CARTESIAN_POINT('Ctrl Pts',(-10.3391673090001,15.2,1.18730450799998));
#259890=CARTESIAN_POINT('Ctrl Pts',(-10.3403552060001,15.2,1.18730140199999));
#259891=CARTESIAN_POINT('Ctrl Pts',(-10.3415519380001,15.2,1.18729710199998));
#259892=CARTESIAN_POINT('Ctrl Pts',(-10.3427574820001,15.2,1.18729159399999));
#259893=CARTESIAN_POINT('Ctrl Pts',(-10.3439718130001,15.2,1.18728485899998));
#259894=CARTESIAN_POINT('Ctrl Pts',(-10.3451949090001,15.2,1.18727688299999));
#259895=CARTESIAN_POINT('Ctrl Pts',(-10.3464267470001,15.2,1.18726764999999));
#259896=CARTESIAN_POINT('Ctrl Pts',(-10.3476673040001,15.2,1.18725714299998));
#259897=CARTESIAN_POINT('Ctrl Pts',(-10.3489165560001,15.2,1.18724534699998));
#259898=CARTESIAN_POINT('Ctrl Pts',(-10.3501744810001,15.2,1.18723224699998));
#259899=CARTESIAN_POINT('Ctrl Pts',(-10.3514410560001,15.2,1.18721782799998));
#259900=CARTESIAN_POINT('Ctrl Pts',(-10.3527162580001,15.2,1.18720207199999));
#259901=CARTESIAN_POINT('Ctrl Pts',(-10.3540000650001,15.2,1.18718496499998));
#259902=CARTESIAN_POINT('Ctrl Pts',(-10.3552924550001,15.2,1.18716649199999));
#259903=CARTESIAN_POINT('Ctrl Pts',(-10.3565934040001,15.2,1.18714663699999));
#259904=CARTESIAN_POINT('Ctrl Pts',(-10.3579028900001,15.2,1.18712538499999));
#259905=CARTESIAN_POINT('Ctrl Pts',(-10.3592208920001,15.2,1.18710272199999));
#259906=CARTESIAN_POINT('Ctrl Pts',(-10.3605473870001,15.2,1.18707863099999));
#259907=CARTESIAN_POINT('Ctrl Pts',(-10.3618823540001,15.2,1.18705309899998));
#259908=CARTESIAN_POINT('Ctrl Pts',(-10.3632257690001,15.2,1.18702610999998));
#259909=CARTESIAN_POINT('Ctrl Pts',(-10.3645776120001,15.2,1.18699765099999));
#259910=CARTESIAN_POINT('Ctrl Pts',(-10.3659378610001,15.2,1.18696770399998));
#259911=CARTESIAN_POINT('Ctrl Pts',(-10.3673064940001,15.2,1.18693625599999));
#259912=CARTESIAN_POINT('Ctrl Pts',(-10.3686834880001,15.2,1.18690329399998));
#259913=CARTESIAN_POINT('Ctrl Pts',(-10.3700688240001,15.2,1.18686880099999));
#259914=CARTESIAN_POINT('Ctrl Pts',(-10.3714624790001,15.2,1.18683276399999));
#259915=CARTESIAN_POINT('Ctrl Pts',(-10.3728644310001,15.2,1.18679516799999));
#259916=CARTESIAN_POINT('Ctrl Pts',(-10.3742746610001,15.2,1.18675599899999));
#259917=CARTESIAN_POINT('Ctrl Pts',(-10.3756931460001,15.2,1.18671524399999));
#259918=CARTESIAN_POINT('Ctrl Pts',(-10.3771198660001,15.2,1.18667288599998));
#259919=CARTESIAN_POINT('Ctrl Pts',(-10.3785547980001,15.2,1.18662891399998));
#259920=CARTESIAN_POINT('Ctrl Pts',(-10.3799979240001,15.2,1.18658331299998));
#259921=CARTESIAN_POINT('Ctrl Pts',(-10.3814492210001,15.2,1.18653606699999));
#259922=CARTESIAN_POINT('Ctrl Pts',(-10.3829086680001,15.2,1.18648716499999));
#259923=CARTESIAN_POINT('Ctrl Pts',(-10.3843762450001,15.2,1.18643659199998));
#259924=CARTESIAN_POINT('Ctrl Pts',(-10.3858519330001,15.2,1.18638433399999));
#259925=CARTESIAN_POINT('Ctrl Pts',(-10.3873357080001,15.2,1.18633037799999));
#259926=CARTESIAN_POINT('Ctrl Pts',(-10.3888275530001,15.2,1.18627470999999));
#259927=CARTESIAN_POINT('Ctrl Pts',(-10.3903274450001,15.2,1.18621731599998));
#259928=CARTESIAN_POINT('Ctrl Pts',(-10.3918353650001,15.2,1.18615818399999));
#259929=CARTESIAN_POINT('Ctrl Pts',(-10.3933512920001,15.2,1.18609729999998));
#259930=CARTESIAN_POINT('Ctrl Pts',(-10.3948752070001,15.2,1.18603464899998));
#259931=CARTESIAN_POINT('Ctrl Pts',(-10.3964070880001,15.2,1.18597021999999));
#259932=CARTESIAN_POINT('Ctrl Pts',(-10.3979469170001,15.2,1.18590399899999));
#259933=CARTESIAN_POINT('Ctrl Pts',(-10.3994946730001,15.2,1.18583597199999));
#259934=CARTESIAN_POINT('Ctrl Pts',(-10.4010503360001,15.2,1.18576612699998));
#259935=CARTESIAN_POINT('Ctrl Pts',(-10.4026138870001,15.2,1.18569445199999));
#259936=CARTESIAN_POINT('Ctrl Pts',(-10.4041853050001,15.2,1.18562093199999));
#259937=CARTESIAN_POINT('Ctrl Pts',(-10.4057645710001,15.2,1.18554555499998));
#259938=CARTESIAN_POINT('Ctrl Pts',(-10.4073516650001,15.2,1.18546830799998));
#259939=CARTESIAN_POINT('Ctrl Pts',(-10.4089465690001,15.2,1.18538917799999));
#259940=CARTESIAN_POINT('Ctrl Pts',(-10.4105492620001,15.2,1.18530815299998));
#259941=CARTESIAN_POINT('Ctrl Pts',(-10.4121597240001,15.2,1.18522521999999));
#259942=CARTESIAN_POINT('Ctrl Pts',(-10.4137779370001,15.2,1.18514036599999));
#259943=CARTESIAN_POINT('Ctrl Pts',(-10.4154038820001,15.2,1.18505357999998));
#259944=CARTESIAN_POINT('Ctrl Pts',(-10.4170375390001,15.2,1.18496484799998));
#259945=CARTESIAN_POINT('Ctrl Pts',(-10.4186788900001,15.2,1.18487415599999));
#259946=CARTESIAN_POINT('Ctrl Pts',(-10.4203279130001,15.2,1.18478149699999));
#259947=CARTESIAN_POINT('Ctrl Pts',(-10.4219845930001,15.2,1.18468685399999));
#259948=CARTESIAN_POINT('Ctrl Pts',(-10.4236489080001,15.2,1.18459021499998));
#259949=CARTESIAN_POINT('Ctrl Pts',(-10.4253208410001,15.2,1.18449156999999));
#259950=CARTESIAN_POINT('Ctrl Pts',(-10.4270003720001,15.2,1.18439090599999));
#259951=CARTESIAN_POINT('Ctrl Pts',(-10.4286874830001,15.2,1.18428821199998));
#259952=CARTESIAN_POINT('Ctrl Pts',(-10.4303821540001,15.2,1.18418347399999));
#259953=CARTESIAN_POINT('Ctrl Pts',(-10.4320843690001,15.2,1.18407667999998));
#259954=CARTESIAN_POINT('Ctrl Pts',(-10.4337941070001,15.2,1.18396781999999));
#259955=CARTESIAN_POINT('Ctrl Pts',(-10.4355113520001,15.2,1.18385688099998));
#259956=CARTESIAN_POINT('Ctrl Pts',(-10.4372360820001,15.2,1.18374385099999));
#259957=CARTESIAN_POINT('Ctrl Pts',(-10.4389682810001,15.2,1.18362871999999));
#259958=CARTESIAN_POINT('Ctrl Pts',(-10.4407079310001,15.2,1.18351147399999));
#259959=CARTESIAN_POINT('Ctrl Pts',(-10.4424550130001,15.2,1.18339210299998));
#259960=CARTESIAN_POINT('Ctrl Pts',(-10.4442095090001,15.2,1.18327059399999));
#259961=CARTESIAN_POINT('Ctrl Pts',(-10.4459714000001,15.2,1.18314693699999));
#259962=CARTESIAN_POINT('Ctrl Pts',(-10.4477406700001,15.2,1.18302111899999));
#259963=CARTESIAN_POINT('Ctrl Pts',(-10.4495173000001,15.2,1.18289313099998));
#259964=CARTESIAN_POINT('Ctrl Pts',(-10.4513012710001,15.2,1.18276295899999));
#259965=CARTESIAN_POINT('Ctrl Pts',(-10.4530925660001,15.2,1.18263059399998));
#259966=CARTESIAN_POINT('Ctrl Pts',(-10.4548911670001,15.2,1.18249602199999));
#259967=CARTESIAN_POINT('Ctrl Pts',(-10.4566970570001,15.2,1.18235923399999));
#259968=CARTESIAN_POINT('Ctrl Pts',(-10.4585102170001,15.2,1.18222021899999));
#259969=CARTESIAN_POINT('Ctrl Pts',(-10.4603306310001,15.2,1.18207896399999));
#259970=CARTESIAN_POINT('Ctrl Pts',(-10.4621582800001,15.2,1.18193545999999));
#259971=CARTESIAN_POINT('Ctrl Pts',(-10.4639931470001,15.2,1.18178969599999));
#259972=CARTESIAN_POINT('Ctrl Pts',(-10.4658352150001,15.2,1.18164165899998));
#259973=CARTESIAN_POINT('Ctrl Pts',(-10.4676844650001,15.2,1.18149133999998));
#259974=CARTESIAN_POINT('Ctrl Pts',(-10.4695408810001,15.2,1.18133872599998));
#259975=CARTESIAN_POINT('Ctrl Pts',(-10.4714044460001,15.2,1.18118380899999));
#259976=CARTESIAN_POINT('Ctrl Pts',(-10.4732751410001,15.2,1.18102657599998));
#259977=CARTESIAN_POINT('Ctrl Pts',(-10.4751529500001,15.2,1.18086701799998));
#259978=CARTESIAN_POINT('Ctrl Pts',(-10.4770378570001,15.2,1.18070512399999));
#259979=CARTESIAN_POINT('Ctrl Pts',(-10.4789298430001,15.2,1.18054088199999));
#259980=CARTESIAN_POINT('Ctrl Pts',(-10.4808288920001,15.2,1.18037428299999));
#259981=CARTESIAN_POINT('Ctrl Pts',(-10.4827349850001,15.2,1.18020531599999));
#259982=CARTESIAN_POINT('Ctrl Pts',(-10.4846481080001,15.2,1.18003396999999));
#259983=CARTESIAN_POINT('Ctrl Pts',(-10.4865682440001,15.2,1.17986023499999));
#259984=CARTESIAN_POINT('Ctrl Pts',(-10.4884953720001,15.2,1.17968410099999));
#259985=CARTESIAN_POINT('Ctrl Pts',(-10.4904294800001,15.2,1.17950555699998));
#259986=CARTESIAN_POINT('Ctrl Pts',(-10.4923705490001,15.2,1.17932459399999));
#259987=CARTESIAN_POINT('Ctrl Pts',(-10.4943185630001,15.2,1.17914119999998));
#259988=CARTESIAN_POINT('Ctrl Pts',(-10.4962735060001,15.2,1.17895536499999));
#259989=CARTESIAN_POINT('Ctrl Pts',(-10.4982353590001,15.2,1.17876708099999));
#259990=CARTESIAN_POINT('Ctrl Pts',(-10.5002041080001,15.2,1.17857633499999));
#259991=CARTESIAN_POINT('Ctrl Pts',(-10.5021797350001,15.2,1.17838311899999));
#259992=CARTESIAN_POINT('Ctrl Pts',(-10.5041622250001,15.2,1.17818742199999));
#259993=CARTESIAN_POINT('Ctrl Pts',(-10.5061515600001,15.2,1.17798923599999));
#259994=CARTESIAN_POINT('Ctrl Pts',(-10.5081477230001,15.2,1.17778854799999));
#259995=CARTESIAN_POINT('Ctrl Pts',(-10.5101507010001,15.2,1.17758534999998));
#259996=CARTESIAN_POINT('Ctrl Pts',(-10.5121604750001,15.2,1.17737963099998));
#259997=CARTESIAN_POINT('Ctrl Pts',(-10.5141770310001,15.2,1.17717138199998));
#259998=CARTESIAN_POINT('Ctrl Pts',(-10.5162003510001,15.2,1.17696059399998));
#259999=CARTESIAN_POINT('Ctrl Pts',(-10.5182304190001,15.2,1.17674725699999));
#260000=CARTESIAN_POINT('Ctrl Pts',(-10.5202672190001,15.2,1.17653135999999));
#260001=CARTESIAN_POINT('Ctrl Pts',(-10.5223107360001,15.2,1.17631289399998));
#260002=CARTESIAN_POINT('Ctrl Pts',(-10.5243609530001,15.2,1.17609184999999));
#260003=CARTESIAN_POINT('Ctrl Pts',(-10.5264178550001,15.2,1.17586821899998));
#260004=CARTESIAN_POINT('Ctrl Pts',(-10.5284814260001,15.2,1.17564198999998));
#260005=CARTESIAN_POINT('Ctrl Pts',(-10.5305516490001,15.2,1.17541315299999));
#260006=CARTESIAN_POINT('Ctrl Pts',(-10.5326285090001,15.2,1.17518170099999));
#260007=CARTESIAN_POINT('Ctrl Pts',(-10.5347119910001,15.2,1.17494762299998));
#260008=CARTESIAN_POINT('Ctrl Pts',(-10.5368020780001,15.2,1.17471090999999));
#260009=CARTESIAN_POINT('Ctrl Pts',(-10.5388987570001,15.2,1.17447155299998));
#260010=CARTESIAN_POINT('Ctrl Pts',(-10.5410020080001,15.2,1.17422954199998));
#260011=CARTESIAN_POINT('Ctrl Pts',(-10.5431118190001,15.2,1.17398486899999));
#260012=CARTESIAN_POINT('Ctrl Pts',(-10.5452281730001,15.2,1.17373752299998));
#260013=CARTESIAN_POINT('Ctrl Pts',(-10.5473510550001,15.2,1.17348749699998));
#260014=CARTESIAN_POINT('Ctrl Pts',(-10.5494804500001,15.2,1.17323477999999));
#260015=CARTESIAN_POINT('Ctrl Pts',(-10.5516163410001,15.2,1.17297936399999));
#260016=CARTESIAN_POINT('Ctrl Pts',(-10.5537587150001,15.2,1.17272124099999));
#260017=CARTESIAN_POINT('Ctrl Pts',(-10.5559075550001,15.2,1.17246039999999));
#260018=CARTESIAN_POINT('Ctrl Pts',(-10.5580628460001,15.2,1.17219683299998));
#260019=CARTESIAN_POINT('Ctrl Pts',(-10.5602245730001,15.2,1.17193052999998));
#260020=CARTESIAN_POINT('Ctrl Pts',(-10.5623927210001,15.2,1.17166148499999));
#260021=CARTESIAN_POINT('Ctrl Pts',(-10.5645672750001,15.2,1.17138968599999));
#260022=CARTESIAN_POINT('Ctrl Pts',(-10.5667482200001,15.2,1.17111512499998));
#260023=CARTESIAN_POINT('Ctrl Pts',(-10.5689355400001,15.2,1.17083779399998));
#260024=CARTESIAN_POINT('Ctrl Pts',(-10.5711292210001,15.2,1.17055768399998));
#260025=CARTESIAN_POINT('Ctrl Pts',(-10.5733292470001,15.2,1.17027478699999));
#260026=CARTESIAN_POINT('Ctrl Pts',(-10.5755356040001,15.2,1.16998909399999));
#260027=CARTESIAN_POINT('Ctrl Pts',(-10.5777482770001,15.2,1.16970059599999));
#260028=CARTESIAN_POINT('Ctrl Pts',(-10.5799672510001,15.2,1.16940928399998));
#260029=CARTESIAN_POINT('Ctrl Pts',(-10.5821925120001,15.2,1.16911514999999));
#260030=CARTESIAN_POINT('Ctrl Pts',(-10.5844240430001,15.2,1.16881818499999));
#260031=CARTESIAN_POINT('Ctrl Pts',(-10.5866618310001,15.2,1.16851838199999));
#260032=CARTESIAN_POINT('Ctrl Pts',(-10.5889058620001,15.2,1.16821573099998));
#260033=CARTESIAN_POINT('Ctrl Pts',(-10.5911561200001,15.2,1.16791022399998));
#260034=CARTESIAN_POINT('Ctrl Pts',(-10.5934125910001,15.2,1.16760185399999));
#260035=CARTESIAN_POINT('Ctrl Pts',(-10.5956752600001,15.2,1.16729060999999));
#260036=CARTESIAN_POINT('Ctrl Pts',(-10.5979441110001,15.2,1.16697648599999));
#260037=CARTESIAN_POINT('Ctrl Pts',(-10.6002191330001,15.2,1.16665947299999));
#260038=CARTESIAN_POINT('Ctrl Pts',(-10.6025003100001,15.2,1.16633956299999));
#260039=CARTESIAN_POINT('Ctrl Pts',(-10.6047876270001,15.2,1.16601674699998));
#260040=CARTESIAN_POINT('Ctrl Pts',(-10.6070810700001,15.2,1.16569101799998));
#260041=CARTESIAN_POINT('Ctrl Pts',(-10.6093806240001,15.2,1.16536236699998));
#260042=CARTESIAN_POINT('Ctrl Pts',(-10.6116862760001,15.2,1.16503078599999));
#260043=CARTESIAN_POINT('Ctrl Pts',(-10.6139980110001,15.2,1.16469626699998));
#260044=CARTESIAN_POINT('Ctrl Pts',(-10.6163158140001,15.2,1.16435880299999));
#260045=CARTESIAN_POINT('Ctrl Pts',(-10.6186396720001,15.2,1.16401838499999));
#260046=CARTESIAN_POINT('Ctrl Pts',(-10.6209695720001,15.2,1.16367500499999));
#260047=CARTESIAN_POINT('Ctrl Pts',(-10.6233054970001,15.2,1.16332865499999));
#260048=CARTESIAN_POINT('Ctrl Pts',(-10.6256474340001,15.2,1.16297932799998));
#260049=CARTESIAN_POINT('Ctrl Pts',(-10.6279953690001,15.2,1.16262701499998));
#260050=CARTESIAN_POINT('Ctrl Pts',(-10.6303492890001,15.2,1.16227170999998));
#260051=CARTESIAN_POINT('Ctrl Pts',(-10.6327091780001,15.2,1.16191340299999));
#260052=CARTESIAN_POINT('Ctrl Pts',(-10.6350750250001,15.2,1.16155208699999));
#260053=CARTESIAN_POINT('Ctrl Pts',(-10.6374468130001,15.2,1.16118775499999));
#260054=CARTESIAN_POINT('Ctrl Pts',(-10.6398245300001,15.2,1.16082039899998));
#260055=CARTESIAN_POINT('Ctrl Pts',(-10.6422081610001,15.2,1.16045001099998));
#260056=CARTESIAN_POINT('Ctrl Pts',(-10.6445976930001,15.2,1.16007658299999));
#260057=CARTESIAN_POINT('Ctrl Pts',(-10.6469931120001,15.2,1.15970010799999));
#260058=CARTESIAN_POINT('Ctrl Pts',(-10.6493944050001,15.2,1.15932057999999));
#260059=CARTESIAN_POINT('Ctrl Pts',(-10.6518015570001,15.2,1.15893798799998));
#260060=CARTESIAN_POINT('Ctrl Pts',(-10.6542145550001,15.2,1.15855232699999));
#260061=CARTESIAN_POINT('Ctrl Pts',(-10.6566333850001,15.2,1.15816358799998));
#260062=CARTESIAN_POINT('Ctrl Pts',(-10.6590580340001,15.2,1.15777176599998));
#260063=CARTESIAN_POINT('Ctrl Pts',(-10.6614884880001,15.2,1.15737684999999));
#260064=CARTESIAN_POINT('Ctrl Pts',(-10.6639247340001,15.2,1.15697883699998));
#260065=CARTESIAN_POINT('Ctrl Pts',(-10.6663667570001,15.2,1.15657771499999));
#260066=CARTESIAN_POINT('Ctrl Pts',(-10.6688145450001,15.2,1.15617348099998));
#260067=CARTESIAN_POINT('Ctrl Pts',(-10.6712680840001,15.2,1.15576612499999));
#260068=CARTESIAN_POINT('Ctrl Pts',(-10.6737273610001,15.2,1.15535563899998));
#260069=CARTESIAN_POINT('Ctrl Pts',(-10.6761923620001,15.2,1.15494201899998));
#260070=CARTESIAN_POINT('Ctrl Pts',(-10.6786630740001,15.2,1.15452525499999));
#260071=CARTESIAN_POINT('Ctrl Pts',(-10.6811394830001,15.2,1.15410534099999));
#260072=CARTESIAN_POINT('Ctrl Pts',(-10.6836215780001,15.2,1.15368226999998));
#260073=CARTESIAN_POINT('Ctrl Pts',(-10.6861093440001,15.2,1.15325603399999));
#260074=CARTESIAN_POINT('Ctrl Pts',(-10.6886027670001,15.2,1.15282662699999));
#260075=CARTESIAN_POINT('Ctrl Pts',(-10.6911018330001,15.2,1.15239403999999));
#260076=CARTESIAN_POINT('Ctrl Pts',(-10.6936065330001,15.2,1.15195826999999));
#260077=CARTESIAN_POINT('Ctrl Pts',(-10.6961168510001,15.2,1.15151930499998));
#260078=CARTESIAN_POINT('Ctrl Pts',(-10.6986327730001,15.2,1.15107714099999));
#260079=CARTESIAN_POINT('Ctrl Pts',(-10.7011542890001,15.2,1.15063176999998));
#260080=CARTESIAN_POINT('Ctrl Pts',(-10.7036813830001,15.2,1.15018318599999));
#260081=CARTESIAN_POINT('Ctrl Pts',(-10.7062140430001,15.2,1.14973138199999));
#260082=CARTESIAN_POINT('Ctrl Pts',(-10.7087522570001,15.2,1.14927634999999));
#260083=CARTESIAN_POINT('Ctrl Pts',(-10.7112960120001,15.2,1.14881808499999));
#260084=CARTESIAN_POINT('Ctrl Pts',(-10.7138452930001,15.2,1.14835657899999));
#260085=CARTESIAN_POINT('Ctrl Pts',(-10.7164000880001,15.2,1.14789182399999));
#260086=CARTESIAN_POINT('Ctrl Pts',(-10.7189603860001,15.2,1.14742381499998));
#260087=CARTESIAN_POINT('Ctrl Pts',(-10.7215261720001,15.2,1.14695254599999));
#260088=CARTESIAN_POINT('Ctrl Pts',(-10.7240974330001,15.2,1.14647800799998));
#260089=CARTESIAN_POINT('Ctrl Pts',(-10.7266741590001,15.2,1.14600019699999));
#260090=CARTESIAN_POINT('Ctrl Pts',(-10.7292563340001,15.2,1.14551910299999));
#260091=CARTESIAN_POINT('Ctrl Pts',(-10.7318439480001,15.2,1.14503472299999));
#260092=CARTESIAN_POINT('Ctrl Pts',(-10.734955593487,15.2,1.14444951182125));
#260093=CARTESIAN_POINT('Ctrl Pts',(-10.7380753572566,15.2,1.14385935058935));
#260094=CARTESIAN_POINT('Ctrl Pts',(-10.7412032147435,15.2,1.14326422341062));
#260095=CARTESIAN_POINT('Ctrl Pts',(-10.7443391425131,15.2,1.1426641201787));
#260096=CARTESIAN_POINT('Ctrl Pts',(-10.7474831100001,15.2,1.14205902499998));
#260097=CARTESIAN_POINT('Ctrl Pts',(-10.7501084340001,15.2,1.14155144699998));
#260098=CARTESIAN_POINT('Ctrl Pts',(-10.7527390940001,15.2,1.14104052899998));
#260099=CARTESIAN_POINT('Ctrl Pts',(-10.7553750790001,15.2,1.14052626499999));
#260100=CARTESIAN_POINT('Ctrl Pts',(-10.7580163760001,15.2,1.14000864899999));
#260101=CARTESIAN_POINT('Ctrl Pts',(-10.7606629730001,15.2,1.13948767199998));
#260102=CARTESIAN_POINT('Ctrl Pts',(-10.7633148570001,15.2,1.13896333199999));
#260103=CARTESIAN_POINT('Ctrl Pts',(-10.7659720160001,15.2,1.13843561899999));
#260104=CARTESIAN_POINT('Ctrl Pts',(-10.7686344370001,15.2,1.13790452999998));
#260105=CARTESIAN_POINT('Ctrl Pts',(-10.7713021080001,15.2,1.13737005599999));
#260106=CARTESIAN_POINT('Ctrl Pts',(-10.7739750180001,15.2,1.13683219199999));
#260107=CARTESIAN_POINT('Ctrl Pts',(-10.7766531540001,15.2,1.13629093099998));
#260108=CARTESIAN_POINT('Ctrl Pts',(-10.7793365030001,15.2,1.13574626899998));
#260109=CARTESIAN_POINT('Ctrl Pts',(-10.7820250540001,15.2,1.13519819699999));
#260110=CARTESIAN_POINT('Ctrl Pts',(-10.7847187940001,15.2,1.13464671099999));
#260111=CARTESIAN_POINT('Ctrl Pts',(-10.7874177100001,15.2,1.13409180499998));
#260112=CARTESIAN_POINT('Ctrl Pts',(-10.7901217920001,15.2,1.13353347099999));
#260113=CARTESIAN_POINT('Ctrl Pts',(-10.7928310260001,15.2,1.13297170399999));
#260114=CARTESIAN_POINT('Ctrl Pts',(-10.7955454010001,15.2,1.13240649799998));
#260115=CARTESIAN_POINT('Ctrl Pts',(-10.7982649040001,15.2,1.13183784699999));
#260116=CARTESIAN_POINT('Ctrl Pts',(-10.8009895250001,15.2,1.13126574599999));
#260117=CARTESIAN_POINT('Ctrl Pts',(-10.8037192500001,15.2,1.13069018799999));
#260118=CARTESIAN_POINT('Ctrl Pts',(-10.8064540680001,15.2,1.13011116799999));
#260119=CARTESIAN_POINT('Ctrl Pts',(-10.8091939670001,15.2,1.12952867799998));
#260120=CARTESIAN_POINT('Ctrl Pts',(-10.8119389340001,15.2,1.12894271399998));
#260121=CARTESIAN_POINT('Ctrl Pts',(-10.8146889590001,15.2,1.12835326899999));
#260122=CARTESIAN_POINT('Ctrl Pts',(-10.8174440290001,15.2,1.12776033899999));
#260123=CARTESIAN_POINT('Ctrl Pts',(-10.8202041310001,15.2,1.12716391599998));
#260124=CARTESIAN_POINT('Ctrl Pts',(-10.8229692560001,15.2,1.12656399699999));
#260125=CARTESIAN_POINT('Ctrl Pts',(-10.8257393900001,15.2,1.12596057199998));
#260126=CARTESIAN_POINT('Ctrl Pts',(-10.8285145220001,15.2,1.12535363899998));
#260127=CARTESIAN_POINT('Ctrl Pts',(-10.8312946400001,15.2,1.12474319099999));
#260128=CARTESIAN_POINT('Ctrl Pts',(-10.8340797320001,15.2,1.12412922199999));
#260129=CARTESIAN_POINT('Ctrl Pts',(-10.8368697870001,15.2,1.12351172799999));
#260130=CARTESIAN_POINT('Ctrl Pts',(-10.8396647920001,15.2,1.12289069999999));
#260131=CARTESIAN_POINT('Ctrl Pts',(-10.8424647370001,15.2,1.12226613499999));
#260132=CARTESIAN_POINT('Ctrl Pts',(-10.8452696110001,15.2,1.12163802799999));
#260133=CARTESIAN_POINT('Ctrl Pts',(-10.8480794000001,15.2,1.12100637199998));
#260134=CARTESIAN_POINT('Ctrl Pts',(-10.8508940940001,15.2,1.12037116099998));
#260135=CARTESIAN_POINT('Ctrl Pts',(-10.8537136800001,15.2,1.11973238999999));
#260136=CARTESIAN_POINT('Ctrl Pts',(-10.8565381480001,15.2,1.11909005299998));
#260137=CARTESIAN_POINT('Ctrl Pts',(-10.8593674860001,15.2,1.11844414699998));
#260138=CARTESIAN_POINT('Ctrl Pts',(-10.8622016830001,15.2,1.11779466399998));
#260139=CARTESIAN_POINT('Ctrl Pts',(-10.8650407270001,15.2,1.11714159799998));
#260140=CARTESIAN_POINT('Ctrl Pts',(-10.8678846060001,15.2,1.11648494599998));
#260141=CARTESIAN_POINT('Ctrl Pts',(-10.8707333090001,15.2,1.11582469999998));
#260142=CARTESIAN_POINT('Ctrl Pts',(-10.8735868260001,15.2,1.11516085799999));
#260143=CARTESIAN_POINT('Ctrl Pts',(-10.8764451420001,15.2,1.11449341099998));
#260144=CARTESIAN_POINT('Ctrl Pts',(-10.8793082490001,15.2,1.11382235599998));
#260145=CARTESIAN_POINT('Ctrl Pts',(-10.8821761360001,15.2,1.11314768799998));
#260146=CARTESIAN_POINT('Ctrl Pts',(-10.8850487880001,15.2,1.11246939899999));
#260147=CARTESIAN_POINT('Ctrl Pts',(-10.8879261980001,15.2,1.11178748499999));
#260148=CARTESIAN_POINT('Ctrl Pts',(-10.8908083520001,15.2,1.11110194299998));
#260149=CARTESIAN_POINT('Ctrl Pts',(-10.8936952400001,15.2,1.11041276499999));
#260150=CARTESIAN_POINT('Ctrl Pts',(-10.8965868490001,15.2,1.10971994599999));
#260151=CARTESIAN_POINT('Ctrl Pts',(-10.8994831710001,15.2,1.10902348199998));
#260152=CARTESIAN_POINT('Ctrl Pts',(-10.9023841920001,15.2,1.10832336799998));
#260153=CARTESIAN_POINT('Ctrl Pts',(-10.9052899020001,15.2,1.10761959699999));
#260154=CARTESIAN_POINT('Ctrl Pts',(-10.9082002890001,15.2,1.10691216599998));
#260155=CARTESIAN_POINT('Ctrl Pts',(-10.9111153440001,15.2,1.10620106799999));
#260156=CARTESIAN_POINT('Ctrl Pts',(-10.9140350530001,15.2,1.10548629899998));
#260157=CARTESIAN_POINT('Ctrl Pts',(-10.9169594070001,15.2,1.10476785399999));
#260158=CARTESIAN_POINT('Ctrl Pts',(-10.9198883940001,15.2,1.10404572799998));
#260159=CARTESIAN_POINT('Ctrl Pts',(-10.9228220030001,15.2,1.10331991499999));
#260160=CARTESIAN_POINT('Ctrl Pts',(-10.9257602240001,15.2,1.10259041099999));
#260161=CARTESIAN_POINT('Ctrl Pts',(-10.9287030450001,15.2,1.10185720999999));
#260162=CARTESIAN_POINT('Ctrl Pts',(-10.9316504550001,15.2,1.10112030799999));
#260163=CARTESIAN_POINT('Ctrl Pts',(-10.9346024440001,15.2,1.10037969999999));
#260164=CARTESIAN_POINT('Ctrl Pts',(-10.9375590010001,15.2,1.09963537999999));
#260165=CARTESIAN_POINT('Ctrl Pts',(-10.9405201130001,15.2,1.09888734399998));
#260166=CARTESIAN_POINT('Ctrl Pts',(-10.9434857720001,15.2,1.09813558799999));
#260167=CARTESIAN_POINT('Ctrl Pts',(-10.9464559650001,15.2,1.09738010499999));
#260168=CARTESIAN_POINT('Ctrl Pts',(-10.9494306820001,15.2,1.09662089099999));
#260169=CARTESIAN_POINT('Ctrl Pts',(-10.9524099120001,15.2,1.09585794199999));
#260170=CARTESIAN_POINT('Ctrl Pts',(-10.9553936450001,15.2,1.09509125199999));
#260171=CARTESIAN_POINT('Ctrl Pts',(-10.9583818690001,15.2,1.09432081699998));
#260172=CARTESIAN_POINT('Ctrl Pts',(-10.9613745740001,15.2,1.09354663099999));
#260173=CARTESIAN_POINT('Ctrl Pts',(-10.9643717480001,15.2,1.09276869099999));
#260174=CARTESIAN_POINT('Ctrl Pts',(-10.9673733820001,15.2,1.09198699199998));
#260175=CARTESIAN_POINT('Ctrl Pts',(-10.9703794650001,15.2,1.09120152799999));
#260176=CARTESIAN_POINT('Ctrl Pts',(-10.9733899850001,15.2,1.09041229499999));
#260177=CARTESIAN_POINT('Ctrl Pts',(-10.9764049340001,15.2,1.08961928699999));
#260178=CARTESIAN_POINT('Ctrl Pts',(-10.9794242980001,15.2,1.08882250199999));
#260179=CARTESIAN_POINT('Ctrl Pts',(-10.9824480680001,15.2,1.08802193399999));
#260180=CARTESIAN_POINT('Ctrl Pts',(-10.9854762340001,15.2,1.08721757799998));
#260181=CARTESIAN_POINT('Ctrl Pts',(-10.9885087840001,15.2,1.08640942999998));
#260182=CARTESIAN_POINT('Ctrl Pts',(-10.9915457090001,15.2,1.08559748499998));
#260183=CARTESIAN_POINT('Ctrl Pts',(-10.9945869970001,15.2,1.08478173799998));
#260184=CARTESIAN_POINT('Ctrl Pts',(-10.9976326380001,15.2,1.08396218499998));
#260185=CARTESIAN_POINT('Ctrl Pts',(-11.0006826220001,15.2,1.08313882099999));
#260186=CARTESIAN_POINT('Ctrl Pts',(-11.0037369370001,15.2,1.08231164299998));
#260187=CARTESIAN_POINT('Ctrl Pts',(-11.0067955760001,15.2,1.08148064399999));
#260188=CARTESIAN_POINT('Ctrl Pts',(-11.0098585240001,15.2,1.08064582099999));
#260189=CARTESIAN_POINT('Ctrl Pts',(-11.0129257730001,15.2,1.07980717099998));
#260190=CARTESIAN_POINT('Ctrl Pts',(-11.0159973130001,15.2,1.07896468599999));
#260191=CARTESIAN_POINT('Ctrl Pts',(-11.0190731330001,15.2,1.07811836399998));
#260192=CARTESIAN_POINT('Ctrl Pts',(-11.0221532220001,15.2,1.07726820099999));
#260193=CARTESIAN_POINT('Ctrl Pts',(-11.0252375700001,15.2,1.07641418999998));
#260194=CARTESIAN_POINT('Ctrl Pts',(-11.0283261660001,15.2,1.07555632999999));
#260195=CARTESIAN_POINT('Ctrl Pts',(-11.0314190020001,15.2,1.07469461299999));
#260196=CARTESIAN_POINT('Ctrl Pts',(-11.0345160640001,15.2,1.07382903799999));
#260197=CARTESIAN_POINT('Ctrl Pts',(-11.0376173460001,15.2,1.07295959799998));
#260198=CARTESIAN_POINT('Ctrl Pts',(-11.0407228350001,15.2,1.07208629099999));
#260199=CARTESIAN_POINT('Ctrl Pts',(-11.0438325210001,15.2,1.07120911099999));
#260200=CARTESIAN_POINT('Ctrl Pts',(-11.0469463940001,15.2,1.07032805399998));
#260201=CARTESIAN_POINT('Ctrl Pts',(-11.0500644440001,15.2,1.06944311599999));
#260202=CARTESIAN_POINT('Ctrl Pts',(-11.0531866600001,15.2,1.06855429399999));
#260203=CARTESIAN_POINT('Ctrl Pts',(-11.0563130330001,15.2,1.06766158099999));
#260204=CARTESIAN_POINT('Ctrl Pts',(-11.0594435520001,15.2,1.06676497499999));
#260205=CARTESIAN_POINT('Ctrl Pts',(-11.0625782070001,15.2,1.06586446999998));
#260206=CARTESIAN_POINT('Ctrl Pts',(-11.0657169880001,15.2,1.06496006399999));
#260207=CARTESIAN_POINT('Ctrl Pts',(-11.0688598860001,15.2,1.06405175099999));
#260208=CARTESIAN_POINT('Ctrl Pts',(-11.0720068880001,15.2,1.06313952799999));
#260209=CARTESIAN_POINT('Ctrl Pts',(-11.0751579870001,15.2,1.06222338999999));
#260210=CARTESIAN_POINT('Ctrl Pts',(-11.0783131710001,15.2,1.06130333499999));
#260211=CARTESIAN_POINT('Ctrl Pts',(-11.0814724300001,15.2,1.06037935499999));
#260212=CARTESIAN_POINT('Ctrl Pts',(-11.0846357550001,15.2,1.05945144899998));
#260213=CARTESIAN_POINT('Ctrl Pts',(-11.0878031360001,15.2,1.05851961199999));
#260214=CARTESIAN_POINT('Ctrl Pts',(-11.0909745620001,15.2,1.05758383999999));
#260215=CARTESIAN_POINT('Ctrl Pts',(-11.0941500240001,15.2,1.05664412899999));
#260216=CARTESIAN_POINT('Ctrl Pts',(-11.0973295110001,15.2,1.05570047499999));
#260217=CARTESIAN_POINT('Ctrl Pts',(-11.1005130140001,15.2,1.05475287299999));
#260218=CARTESIAN_POINT('Ctrl Pts',(-11.1037005220001,15.2,1.05380132099999));
#260219=CARTESIAN_POINT('Ctrl Pts',(-11.1068920250001,15.2,1.05284581399999));
#260220=CARTESIAN_POINT('Ctrl Pts',(-11.1100875160001,15.2,1.05188634799998));
#260221=CARTESIAN_POINT('Ctrl Pts',(-11.1132869810001,15.2,1.05092291799998));
#260222=CARTESIAN_POINT('Ctrl Pts',(-11.1164904140001,15.2,1.04995552199998));
#260223=CARTESIAN_POINT('Ctrl Pts',(-11.1196978020001,15.2,1.04898415499999));
#260224=CARTESIAN_POINT('Ctrl Pts',(-11.1229091360001,15.2,1.04800881199999));
#260225=CARTESIAN_POINT('Ctrl Pts',(-11.1261244080001,15.2,1.04702949099998));
#260226=CARTESIAN_POINT('Ctrl Pts',(-11.1293436050001,15.2,1.04604618899999));
#260227=CARTESIAN_POINT('Ctrl Pts',(-11.1325667200001,15.2,1.04505889899999));
#260228=CARTESIAN_POINT('Ctrl Pts',(-11.1357937420001,15.2,1.04406762099998));
#260229=CARTESIAN_POINT('Ctrl Pts',(-11.1390246620001,15.2,1.04307234699998));
#260230=CARTESIAN_POINT('Ctrl Pts',(-11.1422594690001,15.2,1.04207307599999));
#260231=CARTESIAN_POINT('Ctrl Pts',(-11.1454981540001,15.2,1.04106980299999));
#260232=CARTESIAN_POINT('Ctrl Pts',(-11.1487407070001,15.2,1.04006252499998));
#260233=CARTESIAN_POINT('Ctrl Pts',(-11.1519871190001,15.2,1.03905123799999));
#260234=CARTESIAN_POINT('Ctrl Pts',(-11.1552373810001,15.2,1.03803593699999));
#260235=CARTESIAN_POINT('Ctrl Pts',(-11.1584914810001,15.2,1.03701662199999));
#260236=CARTESIAN_POINT('Ctrl Pts',(-11.1617494110001,15.2,1.03599328399998));
#260237=CARTESIAN_POINT('Ctrl Pts',(-11.1650111610001,15.2,1.03496592399999));
#260238=CARTESIAN_POINT('Ctrl Pts',(-11.1682767210001,15.2,1.03393453499999));
#260239=CARTESIAN_POINT('Ctrl Pts',(-11.1715460820001,15.2,1.03289911399999));
#260240=CARTESIAN_POINT('Ctrl Pts',(-11.1748192350001,15.2,1.03185965899999));
#260241=CARTESIAN_POINT('Ctrl Pts',(-11.1780961680001,15.2,1.03081616499999));
#260242=CARTESIAN_POINT('Ctrl Pts',(-11.1813768730001,15.2,1.02976862899999));
#260243=CARTESIAN_POINT('Ctrl Pts',(-11.1846613420001,15.2,1.02871704699998));
#260244=CARTESIAN_POINT('Ctrl Pts',(-11.1879495640001,15.2,1.02766141599998));
#260245=CARTESIAN_POINT('Ctrl Pts',(-11.1912415290001,15.2,1.02660173099999));
#260246=CARTESIAN_POINT('Ctrl Pts',(-11.1945372270001,15.2,1.02553798999999));
#260247=CARTESIAN_POINT('Ctrl Pts',(-11.1978366510001,15.2,1.02447018799999));
#260248=CARTESIAN_POINT('Ctrl Pts',(-11.2011397890001,15.2,1.02339832299998));
#260249=CARTESIAN_POINT('Ctrl Pts',(-11.2044466330001,15.2,1.02232238999999));
#260250=CARTESIAN_POINT('Ctrl Pts',(-11.2077571730001,15.2,1.02124238699998));
#260251=CARTESIAN_POINT('Ctrl Pts',(-11.2110714010001,15.2,1.02015830899999));
#260252=CARTESIAN_POINT('Ctrl Pts',(-11.2143893040001,15.2,1.01907015299998));
#260253=CARTESIAN_POINT('Ctrl Pts',(-11.2177108770001,15.2,1.01797791699999));
#260254=CARTESIAN_POINT('Ctrl Pts',(-11.2210361080001,15.2,1.01688159599998));
#260255=CARTESIAN_POINT('Ctrl Pts',(-11.2243649880001,15.2,1.01578118599999));
#260256=CARTESIAN_POINT('Ctrl Pts',(-11.2276975070001,15.2,1.01467668399998));
#260257=CARTESIAN_POINT('Ctrl Pts',(-11.2310336580001,15.2,1.01356808799999));
#260258=CARTESIAN_POINT('Ctrl Pts',(-11.2343734290001,15.2,1.01245539299998));
#260259=CARTESIAN_POINT('Ctrl Pts',(-11.2377168140001,15.2,1.01133859799999));
#260260=CARTESIAN_POINT('Ctrl Pts',(-11.2410637990001,15.2,1.01021769499999));
#260261=CARTESIAN_POINT('Ctrl Pts',(-11.2444143790001,15.2,1.00909268499999));
#260262=CARTESIAN_POINT('Ctrl Pts',(-11.2477685430001,15.2,1.00796356299998));
#260263=CARTESIAN_POINT('Ctrl Pts',(-11.2511262810001,15.2,1.00683032499999));
#260264=CARTESIAN_POINT('Ctrl Pts',(-11.2544875850001,15.2,1.00569296999999));
#260265=CARTESIAN_POINT('Ctrl Pts',(-11.2578524460001,15.2,1.00455149199998));
#260266=CARTESIAN_POINT('Ctrl Pts',(-11.2612208540001,15.2,1.00340588999998));
#260267=CARTESIAN_POINT('Ctrl Pts',(-11.2645927990001,15.2,1.00225615799999));
#260268=CARTESIAN_POINT('Ctrl Pts',(-11.2679682740001,15.2,1.00110229499998));
#260269=CARTESIAN_POINT('Ctrl Pts',(-11.2713472680001,15.2,0.999944296999988));
#260270=CARTESIAN_POINT('Ctrl Pts',(-11.2747297730001,15.2,0.998782160999987));
#260271=CARTESIAN_POINT('Ctrl Pts',(-11.2781157800001,15.2,0.997615882999985));
#260272=CARTESIAN_POINT('Ctrl Pts',(-11.2815052780001,15.2,0.996445461999986));
#260273=CARTESIAN_POINT('Ctrl Pts',(-11.2848982590001,15.2,0.995270892999987));
#260274=CARTESIAN_POINT('Ctrl Pts',(-11.2882947150001,15.2,0.994092171999985));
#260275=CARTESIAN_POINT('Ctrl Pts',(-11.2916946350001,15.2,0.992909295999986));
#260276=CARTESIAN_POINT('Ctrl Pts',(-11.2950980120001,15.2,0.991722263999986));
#260277=CARTESIAN_POINT('Ctrl Pts',(-11.2985048360001,15.2,0.990531070999987));
#260278=CARTESIAN_POINT('Ctrl Pts',(-11.3019150960001,15.2,0.989335713999986));
#260279=CARTESIAN_POINT('Ctrl Pts',(-11.3053287860001,15.2,0.988136191999986));
#260280=CARTESIAN_POINT('Ctrl Pts',(-11.3087458960001,15.2,0.986932498999984));
#260281=CARTESIAN_POINT('Ctrl Pts',(-11.3121664170001,15.2,0.985724631999982));
#260282=CARTESIAN_POINT('Ctrl Pts',(-11.3155903390001,15.2,0.984512589999986));
#260283=CARTESIAN_POINT('Ctrl Pts',(-11.3190176540001,15.2,0.983296368999986));
#260284=CARTESIAN_POINT('Ctrl Pts',(-11.3224483530001,15.2,0.982075965999982));
#260285=CARTESIAN_POINT('Ctrl Pts',(-11.3258824260001,15.2,0.980851377999983));
#260286=CARTESIAN_POINT('Ctrl Pts',(-11.3293198660001,15.2,0.979622600999988));
#260287=CARTESIAN_POINT('Ctrl Pts',(-11.3327606630001,15.2,0.978389632999987));
#260288=CARTESIAN_POINT('Ctrl Pts',(-11.3362048080001,15.2,0.977152470999982));
#260289=CARTESIAN_POINT('Ctrl Pts',(-11.3396522920001,15.2,0.975911110999985));
#260290=CARTESIAN_POINT('Ctrl Pts',(-11.3431031070001,15.2,0.974665550999987));
#260291=CARTESIAN_POINT('Ctrl Pts',(-11.3465572430001,15.2,0.973415788999983));
#260292=CARTESIAN_POINT('Ctrl Pts',(-11.3500146920001,15.2,0.972161818999986));
#260293=CARTESIAN_POINT('Ctrl Pts',(-11.3534754440001,15.2,0.970903640999987));
#260294=CARTESIAN_POINT('Ctrl Pts',(-11.3569394920001,15.2,0.969641250999986));
#260295=CARTESIAN_POINT('Ctrl Pts',(-11.3604068260001,15.2,0.968374645999983));
#260296=CARTESIAN_POINT('Ctrl Pts',(-11.3638774360001,15.2,0.967103821999986));
#260297=CARTESIAN_POINT('Ctrl Pts',(-11.3673513150001,15.2,0.965828777999986));
#260298=CARTESIAN_POINT('Ctrl Pts',(-11.3708284530001,15.2,0.964549509999983));
#260299=CARTESIAN_POINT('Ctrl Pts',(-11.3743088440001,15.2,0.963266015999986));
#260300=CARTESIAN_POINT('Ctrl Pts',(-11.3777924770001,15.2,0.961978291999985));
#260301=CARTESIAN_POINT('Ctrl Pts',(-11.3812793430001,15.2,0.960686337999985));
#260302=CARTESIAN_POINT('Ctrl Pts',(-11.3847694350001,15.2,0.959390146999985));
#260303=CARTESIAN_POINT('Ctrl Pts',(-11.3882627430001,15.2,0.958089718999986));
#260304=CARTESIAN_POINT('Ctrl Pts',(-11.3917592580001,15.2,0.956785048999986));
#260305=CARTESIAN_POINT('Ctrl Pts',(-11.3952589700001,15.2,0.955476136999986));
#260306=CARTESIAN_POINT('Ctrl Pts',(-11.3987618720001,15.2,0.954162976999986));
#260307=CARTESIAN_POINT('Ctrl Pts',(-11.4022679530001,15.2,0.952845567999985));
#260308=CARTESIAN_POINT('Ctrl Pts',(-11.4057772070001,15.2,0.951523905999987));
#260309=CARTESIAN_POINT('Ctrl Pts',(-11.4092896250001,15.2,0.950197990999988));
#260310=CARTESIAN_POINT('Ctrl Pts',(-11.4128052000001,15.2,0.948867817999983));
#260311=CARTESIAN_POINT('Ctrl Pts',(-11.4163239240001,15.2,0.947533386999986));
#260312=CARTESIAN_POINT('Ctrl Pts',(-11.4198457890001,15.2,0.946194692999986));
#260313=CARTESIAN_POINT('Ctrl Pts',(-11.4233707840001,15.2,0.944851733999985));
#260314=CARTESIAN_POINT('Ctrl Pts',(-11.4268989030001,15.2,0.943504507999986));
#260315=CARTESIAN_POINT('Ctrl Pts',(-11.4304301310001,15.2,0.942153010999984));
#260316=CARTESIAN_POINT('Ctrl Pts',(-11.4339644600001,15.2,0.940797237999984));
#260317=CARTESIAN_POINT('Ctrl Pts',(-11.4375018800001,15.2,0.939437186999985));
#260318=CARTESIAN_POINT('Ctrl Pts',(-11.4410423790001,15.2,0.938072855999987));
#260319=CARTESIAN_POINT('Ctrl Pts',(-11.4445859520001,15.2,0.936704240999986));
#260320=CARTESIAN_POINT('Ctrl Pts',(-11.4481325920001,15.2,0.935331340999985));
#260321=CARTESIAN_POINT('Ctrl Pts',(-11.4516822960001,15.2,0.933954156999985));
#260322=CARTESIAN_POINT('Ctrl Pts',(-11.4552350600001,15.2,0.932572684999986));
#260323=CARTESIAN_POINT('Ctrl Pts',(-11.4580797200001,15.2,0.931464077999986));
#260324=CARTESIAN_POINT('Ctrl Pts',(-11.4602145910001,15.2,0.930630692999985));
#260325=CARTESIAN_POINT('Ctrl Pts',(-11.4616384500001,15.2,0.930074245999983));
#260326=CARTESIAN_POINT('Ctrl Pts',(-11.4623505340001,15.2,0.929795807999985));
#260327=CARTESIAN_POINT('Ctrl Pts',(-10.3068855240001,12.2,1.18690176599999));
#260328=CARTESIAN_POINT('Ctrl Pts',(-10.3070598110001,12.2,1.18690675299999));
#260329=CARTESIAN_POINT('Ctrl Pts',(-10.3074144740001,12.2,1.18691681599998));
#260330=CARTESIAN_POINT('Ctrl Pts',(-10.3079518800001,12.2,1.18693179799998));
#260331=CARTESIAN_POINT('Ctrl Pts',(-10.3086758300001,12.2,1.18695143999998));
#260332=CARTESIAN_POINT('Ctrl Pts',(-10.3095915440001,12.2,1.18697537099999));
#260333=CARTESIAN_POINT('Ctrl Pts',(-10.3105221240001,12.2,1.18699875499999));
#260334=CARTESIAN_POINT('Ctrl Pts',(-10.3114622390001,12.2,1.18702143499998));
#260335=CARTESIAN_POINT('Ctrl Pts',(-10.3124118610001,12.2,1.18704339399998));
#260336=CARTESIAN_POINT('Ctrl Pts',(-10.3133709660001,12.2,1.18706460899999));
#260337=CARTESIAN_POINT('Ctrl Pts',(-10.3143395250001,12.2,1.18708506599999));
#260338=CARTESIAN_POINT('Ctrl Pts',(-10.3153175130001,12.2,1.18710474299998));
#260339=CARTESIAN_POINT('Ctrl Pts',(-10.3163049050001,12.2,1.18712362399998));
#260340=CARTESIAN_POINT('Ctrl Pts',(-10.3173016730001,12.2,1.18714168899999));
#260341=CARTESIAN_POINT('Ctrl Pts',(-10.3183077930001,12.2,1.18715892099999));
#260342=CARTESIAN_POINT('Ctrl Pts',(-10.3193232400001,12.2,1.18717530199998));
#260343=CARTESIAN_POINT('Ctrl Pts',(-10.3203479850001,12.2,1.18719081299998));
#260344=CARTESIAN_POINT('Ctrl Pts',(-10.3213820050001,12.2,1.18720543699999));
#260345=CARTESIAN_POINT('Ctrl Pts',(-10.3224252740001,12.2,1.18721915599998));
#260346=CARTESIAN_POINT('Ctrl Pts',(-10.3234777680001,12.2,1.18723195099999));
#260347=CARTESIAN_POINT('Ctrl Pts',(-10.3245394590001,12.2,1.18724380599998));
#260348=CARTESIAN_POINT('Ctrl Pts',(-10.3256103250001,12.2,1.18725470399998));
#260349=CARTESIAN_POINT('Ctrl Pts',(-10.3266903400001,12.2,1.18726462499998));
#260350=CARTESIAN_POINT('Ctrl Pts',(-10.3277794780001,12.2,1.18727355499999));
#260351=CARTESIAN_POINT('Ctrl Pts',(-10.3288777160001,12.2,1.18728147399999));
#260352=CARTESIAN_POINT('Ctrl Pts',(-10.3299850290001,12.2,1.18728836599999));
#260353=CARTESIAN_POINT('Ctrl Pts',(-10.3311013920001,12.2,1.18729421399999));
#260354=CARTESIAN_POINT('Ctrl Pts',(-10.3322267810001,12.2,1.18729900199999));
#260355=CARTESIAN_POINT('Ctrl Pts',(-10.3333611710001,12.2,1.18730271099999));
#260356=CARTESIAN_POINT('Ctrl Pts',(-10.3345045400001,12.2,1.18730532599999));
#260357=CARTESIAN_POINT('Ctrl Pts',(-10.3356568620001,12.2,1.18730682999999));
#260358=CARTESIAN_POINT('Ctrl Pts',(-10.3368181130001,12.2,1.18730720599999));
#260359=CARTESIAN_POINT('Ctrl Pts',(-10.3379882700001,12.2,1.18730643699998));
#260360=CARTESIAN_POINT('Ctrl Pts',(-10.3391673090001,12.2,1.18730450799998));
#260361=CARTESIAN_POINT('Ctrl Pts',(-10.3403552060001,12.2,1.18730140199999));
#260362=CARTESIAN_POINT('Ctrl Pts',(-10.3415519380001,12.2,1.18729710199998));
#260363=CARTESIAN_POINT('Ctrl Pts',(-10.3427574820001,12.2,1.18729159399999));
#260364=CARTESIAN_POINT('Ctrl Pts',(-10.3439718130001,12.2,1.18728485899998));
#260365=CARTESIAN_POINT('Ctrl Pts',(-10.3451949090001,12.2,1.18727688299999));
#260366=CARTESIAN_POINT('Ctrl Pts',(-10.3464267470001,12.2,1.18726764999999));
#260367=CARTESIAN_POINT('Ctrl Pts',(-10.3476673040001,12.2,1.18725714299998));
#260368=CARTESIAN_POINT('Ctrl Pts',(-10.3489165560001,12.2,1.18724534699998));
#260369=CARTESIAN_POINT('Ctrl Pts',(-10.3501744810001,12.2,1.18723224699998));
#260370=CARTESIAN_POINT('Ctrl Pts',(-10.3514410560001,12.2,1.18721782799998));
#260371=CARTESIAN_POINT('Ctrl Pts',(-10.3527162580001,12.2,1.18720207199999));
#260372=CARTESIAN_POINT('Ctrl Pts',(-10.3540000650001,12.2,1.18718496499998));
#260373=CARTESIAN_POINT('Ctrl Pts',(-10.3552924550001,12.2,1.18716649199999));
#260374=CARTESIAN_POINT('Ctrl Pts',(-10.3565934040001,12.2,1.18714663699999));
#260375=CARTESIAN_POINT('Ctrl Pts',(-10.3579028900001,12.2,1.18712538499999));
#260376=CARTESIAN_POINT('Ctrl Pts',(-10.3592208920001,12.2,1.18710272199999));
#260377=CARTESIAN_POINT('Ctrl Pts',(-10.3605473870001,12.2,1.18707863099999));
#260378=CARTESIAN_POINT('Ctrl Pts',(-10.3618823540001,12.2,1.18705309899998));
#260379=CARTESIAN_POINT('Ctrl Pts',(-10.3632257690001,12.2,1.18702610999998));
#260380=CARTESIAN_POINT('Ctrl Pts',(-10.3645776120001,12.2,1.18699765099999));
#260381=CARTESIAN_POINT('Ctrl Pts',(-10.3659378610001,12.2,1.18696770399998));
#260382=CARTESIAN_POINT('Ctrl Pts',(-10.3673064940001,12.2,1.18693625599999));
#260383=CARTESIAN_POINT('Ctrl Pts',(-10.3686834880001,12.2,1.18690329399998));
#260384=CARTESIAN_POINT('Ctrl Pts',(-10.3700688240001,12.2,1.18686880099999));
#260385=CARTESIAN_POINT('Ctrl Pts',(-10.3714624790001,12.2,1.18683276399999));
#260386=CARTESIAN_POINT('Ctrl Pts',(-10.3728644310001,12.2,1.18679516799999));
#260387=CARTESIAN_POINT('Ctrl Pts',(-10.3742746610001,12.2,1.18675599899999));
#260388=CARTESIAN_POINT('Ctrl Pts',(-10.3756931460001,12.2,1.18671524399999));
#260389=CARTESIAN_POINT('Ctrl Pts',(-10.3771198660001,12.2,1.18667288599998));
#260390=CARTESIAN_POINT('Ctrl Pts',(-10.3785547980001,12.2,1.18662891399998));
#260391=CARTESIAN_POINT('Ctrl Pts',(-10.3799979240001,12.2,1.18658331299998));
#260392=CARTESIAN_POINT('Ctrl Pts',(-10.3814492210001,12.2,1.18653606699999));
#260393=CARTESIAN_POINT('Ctrl Pts',(-10.3829086680001,12.2,1.18648716499999));
#260394=CARTESIAN_POINT('Ctrl Pts',(-10.3843762450001,12.2,1.18643659199998));
#260395=CARTESIAN_POINT('Ctrl Pts',(-10.3858519330001,12.2,1.18638433399999));
#260396=CARTESIAN_POINT('Ctrl Pts',(-10.3873357080001,12.2,1.18633037799999));
#260397=CARTESIAN_POINT('Ctrl Pts',(-10.3888275530001,12.2,1.18627470999999));
#260398=CARTESIAN_POINT('Ctrl Pts',(-10.3903274450001,12.2,1.18621731599998));
#260399=CARTESIAN_POINT('Ctrl Pts',(-10.3918353650001,12.2,1.18615818399999));
#260400=CARTESIAN_POINT('Ctrl Pts',(-10.3933512920001,12.2,1.18609729999998));
#260401=CARTESIAN_POINT('Ctrl Pts',(-10.3948752070001,12.2,1.18603464899998));
#260402=CARTESIAN_POINT('Ctrl Pts',(-10.3964070880001,12.2,1.18597021999999));
#260403=CARTESIAN_POINT('Ctrl Pts',(-10.3979469170001,12.2,1.18590399899999));
#260404=CARTESIAN_POINT('Ctrl Pts',(-10.3994946730001,12.2,1.18583597199999));
#260405=CARTESIAN_POINT('Ctrl Pts',(-10.4010503360001,12.2,1.18576612699998));
#260406=CARTESIAN_POINT('Ctrl Pts',(-10.4026138870001,12.2,1.18569445199999));
#260407=CARTESIAN_POINT('Ctrl Pts',(-10.4041853050001,12.2,1.18562093199999));
#260408=CARTESIAN_POINT('Ctrl Pts',(-10.4057645710001,12.2,1.18554555499998));
#260409=CARTESIAN_POINT('Ctrl Pts',(-10.4073516650001,12.2,1.18546830799998));
#260410=CARTESIAN_POINT('Ctrl Pts',(-10.4089465690001,12.2,1.18538917799999));
#260411=CARTESIAN_POINT('Ctrl Pts',(-10.4105492620001,12.2,1.18530815299998));
#260412=CARTESIAN_POINT('Ctrl Pts',(-10.4121597240001,12.2,1.18522521999999));
#260413=CARTESIAN_POINT('Ctrl Pts',(-10.4137779370001,12.2,1.18514036599999));
#260414=CARTESIAN_POINT('Ctrl Pts',(-10.4154038820001,12.2,1.18505357999998));
#260415=CARTESIAN_POINT('Ctrl Pts',(-10.4170375390001,12.2,1.18496484799998));
#260416=CARTESIAN_POINT('Ctrl Pts',(-10.4186788900001,12.2,1.18487415599999));
#260417=CARTESIAN_POINT('Ctrl Pts',(-10.4203279130001,12.2,1.18478149699999));
#260418=CARTESIAN_POINT('Ctrl Pts',(-10.4219845930001,12.2,1.18468685399999));
#260419=CARTESIAN_POINT('Ctrl Pts',(-10.4236489080001,12.2,1.18459021499998));
#260420=CARTESIAN_POINT('Ctrl Pts',(-10.4253208410001,12.2,1.18449156999999));
#260421=CARTESIAN_POINT('Ctrl Pts',(-10.4270003720001,12.2,1.18439090599999));
#260422=CARTESIAN_POINT('Ctrl Pts',(-10.4286874830001,12.2,1.18428821199998));
#260423=CARTESIAN_POINT('Ctrl Pts',(-10.4303821540001,12.2,1.18418347399999));
#260424=CARTESIAN_POINT('Ctrl Pts',(-10.4320843690001,12.2,1.18407667999998));
#260425=CARTESIAN_POINT('Ctrl Pts',(-10.4337941070001,12.2,1.18396781999999));
#260426=CARTESIAN_POINT('Ctrl Pts',(-10.4355113520001,12.2,1.18385688099998));
#260427=CARTESIAN_POINT('Ctrl Pts',(-10.4372360820001,12.2,1.18374385099999));
#260428=CARTESIAN_POINT('Ctrl Pts',(-10.4389682810001,12.2,1.18362871999999));
#260429=CARTESIAN_POINT('Ctrl Pts',(-10.4407079310001,12.2,1.18351147399999));
#260430=CARTESIAN_POINT('Ctrl Pts',(-10.4424550130001,12.2,1.18339210299998));
#260431=CARTESIAN_POINT('Ctrl Pts',(-10.4442095090001,12.2,1.18327059399999));
#260432=CARTESIAN_POINT('Ctrl Pts',(-10.4459714000001,12.2,1.18314693699999));
#260433=CARTESIAN_POINT('Ctrl Pts',(-10.4477406700001,12.2,1.18302111899999));
#260434=CARTESIAN_POINT('Ctrl Pts',(-10.4495173000001,12.2,1.18289313099998));
#260435=CARTESIAN_POINT('Ctrl Pts',(-10.4513012710001,12.2,1.18276295899999));
#260436=CARTESIAN_POINT('Ctrl Pts',(-10.4530925660001,12.2,1.18263059399998));
#260437=CARTESIAN_POINT('Ctrl Pts',(-10.4548911670001,12.2,1.18249602199999));
#260438=CARTESIAN_POINT('Ctrl Pts',(-10.4566970570001,12.2,1.18235923399999));
#260439=CARTESIAN_POINT('Ctrl Pts',(-10.4585102170001,12.2,1.18222021899999));
#260440=CARTESIAN_POINT('Ctrl Pts',(-10.4603306310001,12.2,1.18207896399999));
#260441=CARTESIAN_POINT('Ctrl Pts',(-10.4621582800001,12.2,1.18193545999999));
#260442=CARTESIAN_POINT('Ctrl Pts',(-10.4639931470001,12.2,1.18178969599999));
#260443=CARTESIAN_POINT('Ctrl Pts',(-10.4658352150001,12.2,1.18164165899998));
#260444=CARTESIAN_POINT('Ctrl Pts',(-10.4676844650001,12.2,1.18149133999998));
#260445=CARTESIAN_POINT('Ctrl Pts',(-10.4695408810001,12.2,1.18133872599998));
#260446=CARTESIAN_POINT('Ctrl Pts',(-10.4714044460001,12.2,1.18118380899999));
#260447=CARTESIAN_POINT('Ctrl Pts',(-10.4732751410001,12.2,1.18102657599998));
#260448=CARTESIAN_POINT('Ctrl Pts',(-10.4751529500001,12.2,1.18086701799998));
#260449=CARTESIAN_POINT('Ctrl Pts',(-10.4770378570001,12.2,1.18070512399999));
#260450=CARTESIAN_POINT('Ctrl Pts',(-10.4789298430001,12.2,1.18054088199999));
#260451=CARTESIAN_POINT('Ctrl Pts',(-10.4808288920001,12.2,1.18037428299999));
#260452=CARTESIAN_POINT('Ctrl Pts',(-10.4827349850001,12.2,1.18020531599999));
#260453=CARTESIAN_POINT('Ctrl Pts',(-10.4846481080001,12.2,1.18003396999999));
#260454=CARTESIAN_POINT('Ctrl Pts',(-10.4865682440001,12.2,1.17986023499999));
#260455=CARTESIAN_POINT('Ctrl Pts',(-10.4884953720001,12.2,1.17968410099999));
#260456=CARTESIAN_POINT('Ctrl Pts',(-10.4904294800001,12.2,1.17950555699998));
#260457=CARTESIAN_POINT('Ctrl Pts',(-10.4923705490001,12.2,1.17932459399999));
#260458=CARTESIAN_POINT('Ctrl Pts',(-10.4943185630001,12.2,1.17914119999998));
#260459=CARTESIAN_POINT('Ctrl Pts',(-10.4962735060001,12.2,1.17895536499999));
#260460=CARTESIAN_POINT('Ctrl Pts',(-10.4982353590001,12.2,1.17876708099999));
#260461=CARTESIAN_POINT('Ctrl Pts',(-10.5002041080001,12.2,1.17857633499999));
#260462=CARTESIAN_POINT('Ctrl Pts',(-10.5021797350001,12.2,1.17838311899999));
#260463=CARTESIAN_POINT('Ctrl Pts',(-10.5041622250001,12.2,1.17818742199999));
#260464=CARTESIAN_POINT('Ctrl Pts',(-10.5061515600001,12.2,1.17798923599999));
#260465=CARTESIAN_POINT('Ctrl Pts',(-10.5081477230001,12.2,1.17778854799999));
#260466=CARTESIAN_POINT('Ctrl Pts',(-10.5101507010001,12.2,1.17758534999998));
#260467=CARTESIAN_POINT('Ctrl Pts',(-10.5121604750001,12.2,1.17737963099998));
#260468=CARTESIAN_POINT('Ctrl Pts',(-10.5141770310001,12.2,1.17717138199998));
#260469=CARTESIAN_POINT('Ctrl Pts',(-10.5162003510001,12.2,1.17696059399998));
#260470=CARTESIAN_POINT('Ctrl Pts',(-10.5182304190001,12.2,1.17674725699999));
#260471=CARTESIAN_POINT('Ctrl Pts',(-10.5202672190001,12.2,1.17653135999999));
#260472=CARTESIAN_POINT('Ctrl Pts',(-10.5223107360001,12.2,1.17631289399998));
#260473=CARTESIAN_POINT('Ctrl Pts',(-10.5243609530001,12.2,1.17609184999999));
#260474=CARTESIAN_POINT('Ctrl Pts',(-10.5264178550001,12.2,1.17586821899998));
#260475=CARTESIAN_POINT('Ctrl Pts',(-10.5284814260001,12.2,1.17564198999998));
#260476=CARTESIAN_POINT('Ctrl Pts',(-10.5305516490001,12.2,1.17541315299999));
#260477=CARTESIAN_POINT('Ctrl Pts',(-10.5326285090001,12.2,1.17518170099999));
#260478=CARTESIAN_POINT('Ctrl Pts',(-10.5347119910001,12.2,1.17494762299998));
#260479=CARTESIAN_POINT('Ctrl Pts',(-10.5368020780001,12.2,1.17471090999999));
#260480=CARTESIAN_POINT('Ctrl Pts',(-10.5388987570001,12.2,1.17447155299998));
#260481=CARTESIAN_POINT('Ctrl Pts',(-10.5410020080001,12.2,1.17422954199998));
#260482=CARTESIAN_POINT('Ctrl Pts',(-10.5431118190001,12.2,1.17398486899999));
#260483=CARTESIAN_POINT('Ctrl Pts',(-10.5452281730001,12.2,1.17373752299998));
#260484=CARTESIAN_POINT('Ctrl Pts',(-10.5473510550001,12.2,1.17348749699998));
#260485=CARTESIAN_POINT('Ctrl Pts',(-10.5494804500001,12.2,1.17323477999999));
#260486=CARTESIAN_POINT('Ctrl Pts',(-10.5516163410001,12.2,1.17297936399999));
#260487=CARTESIAN_POINT('Ctrl Pts',(-10.5537587150001,12.2,1.17272124099999));
#260488=CARTESIAN_POINT('Ctrl Pts',(-10.5559075550001,12.2,1.17246039999999));
#260489=CARTESIAN_POINT('Ctrl Pts',(-10.5580628460001,12.2,1.17219683299998));
#260490=CARTESIAN_POINT('Ctrl Pts',(-10.5602245730001,12.2,1.17193052999998));
#260491=CARTESIAN_POINT('Ctrl Pts',(-10.5623927210001,12.2,1.17166148499999));
#260492=CARTESIAN_POINT('Ctrl Pts',(-10.5645672750001,12.2,1.17138968599999));
#260493=CARTESIAN_POINT('Ctrl Pts',(-10.5667482200001,12.2,1.17111512499998));
#260494=CARTESIAN_POINT('Ctrl Pts',(-10.5689355400001,12.2,1.17083779399998));
#260495=CARTESIAN_POINT('Ctrl Pts',(-10.5711292210001,12.2,1.17055768399998));
#260496=CARTESIAN_POINT('Ctrl Pts',(-10.5733292470001,12.2,1.17027478699999));
#260497=CARTESIAN_POINT('Ctrl Pts',(-10.5755356040001,12.2,1.16998909399999));
#260498=CARTESIAN_POINT('Ctrl Pts',(-10.5777482770001,12.2,1.16970059599999));
#260499=CARTESIAN_POINT('Ctrl Pts',(-10.5799672510001,12.2,1.16940928399998));
#260500=CARTESIAN_POINT('Ctrl Pts',(-10.5821925120001,12.2,1.16911514999999));
#260501=CARTESIAN_POINT('Ctrl Pts',(-10.5844240430001,12.2,1.16881818499999));
#260502=CARTESIAN_POINT('Ctrl Pts',(-10.5866618310001,12.2,1.16851838199999));
#260503=CARTESIAN_POINT('Ctrl Pts',(-10.5889058620001,12.2,1.16821573099998));
#260504=CARTESIAN_POINT('Ctrl Pts',(-10.5911561200001,12.2,1.16791022399998));
#260505=CARTESIAN_POINT('Ctrl Pts',(-10.5934125910001,12.2,1.16760185399999));
#260506=CARTESIAN_POINT('Ctrl Pts',(-10.5956752600001,12.2,1.16729060999999));
#260507=CARTESIAN_POINT('Ctrl Pts',(-10.5979441110001,12.2,1.16697648599999));
#260508=CARTESIAN_POINT('Ctrl Pts',(-10.6002191330001,12.2,1.16665947299999));
#260509=CARTESIAN_POINT('Ctrl Pts',(-10.6025003100001,12.2,1.16633956299999));
#260510=CARTESIAN_POINT('Ctrl Pts',(-10.6047876270001,12.2,1.16601674699998));
#260511=CARTESIAN_POINT('Ctrl Pts',(-10.6070810700001,12.2,1.16569101799998));
#260512=CARTESIAN_POINT('Ctrl Pts',(-10.6093806240001,12.2,1.16536236699998));
#260513=CARTESIAN_POINT('Ctrl Pts',(-10.6116862760001,12.2,1.16503078599999));
#260514=CARTESIAN_POINT('Ctrl Pts',(-10.6139980110001,12.2,1.16469626699998));
#260515=CARTESIAN_POINT('Ctrl Pts',(-10.6163158140001,12.2,1.16435880299999));
#260516=CARTESIAN_POINT('Ctrl Pts',(-10.6186396720001,12.2,1.16401838499999));
#260517=CARTESIAN_POINT('Ctrl Pts',(-10.6209695720001,12.2,1.16367500499999));
#260518=CARTESIAN_POINT('Ctrl Pts',(-10.6233054970001,12.2,1.16332865499999));
#260519=CARTESIAN_POINT('Ctrl Pts',(-10.6256474340001,12.2,1.16297932799998));
#260520=CARTESIAN_POINT('Ctrl Pts',(-10.6279953690001,12.2,1.16262701499998));
#260521=CARTESIAN_POINT('Ctrl Pts',(-10.6303492890001,12.2,1.16227170999998));
#260522=CARTESIAN_POINT('Ctrl Pts',(-10.6327091780001,12.2,1.16191340299999));
#260523=CARTESIAN_POINT('Ctrl Pts',(-10.6350750250001,12.2,1.16155208699999));
#260524=CARTESIAN_POINT('Ctrl Pts',(-10.6374468130001,12.2,1.16118775499999));
#260525=CARTESIAN_POINT('Ctrl Pts',(-10.6398245300001,12.2,1.16082039899998));
#260526=CARTESIAN_POINT('Ctrl Pts',(-10.6422081610001,12.2,1.16045001099998));
#260527=CARTESIAN_POINT('Ctrl Pts',(-10.6445976930001,12.2,1.16007658299999));
#260528=CARTESIAN_POINT('Ctrl Pts',(-10.6469931120001,12.2,1.15970010799999));
#260529=CARTESIAN_POINT('Ctrl Pts',(-10.6493944050001,12.2,1.15932057999999));
#260530=CARTESIAN_POINT('Ctrl Pts',(-10.6518015570001,12.2,1.15893798799998));
#260531=CARTESIAN_POINT('Ctrl Pts',(-10.6542145550001,12.2,1.15855232699999));
#260532=CARTESIAN_POINT('Ctrl Pts',(-10.6566333850001,12.2,1.15816358799998));
#260533=CARTESIAN_POINT('Ctrl Pts',(-10.6590580340001,12.2,1.15777176599998));
#260534=CARTESIAN_POINT('Ctrl Pts',(-10.6614884880001,12.2,1.15737684999999));
#260535=CARTESIAN_POINT('Ctrl Pts',(-10.6639247340001,12.2,1.15697883699998));
#260536=CARTESIAN_POINT('Ctrl Pts',(-10.6663667570001,12.2,1.15657771499999));
#260537=CARTESIAN_POINT('Ctrl Pts',(-10.6688145450001,12.2,1.15617348099998));
#260538=CARTESIAN_POINT('Ctrl Pts',(-10.6712680840001,12.2,1.15576612499999));
#260539=CARTESIAN_POINT('Ctrl Pts',(-10.6737273610001,12.2,1.15535563899998));
#260540=CARTESIAN_POINT('Ctrl Pts',(-10.6761923620001,12.2,1.15494201899998));
#260541=CARTESIAN_POINT('Ctrl Pts',(-10.6786630740001,12.2,1.15452525499999));
#260542=CARTESIAN_POINT('Ctrl Pts',(-10.6811394830001,12.2,1.15410534099999));
#260543=CARTESIAN_POINT('Ctrl Pts',(-10.6836215780001,12.2,1.15368226999998));
#260544=CARTESIAN_POINT('Ctrl Pts',(-10.6861093440001,12.2,1.15325603399999));
#260545=CARTESIAN_POINT('Ctrl Pts',(-10.6886027670001,12.2,1.15282662699999));
#260546=CARTESIAN_POINT('Ctrl Pts',(-10.6911018330001,12.2,1.15239403999999));
#260547=CARTESIAN_POINT('Ctrl Pts',(-10.6936065330001,12.2,1.15195826999999));
#260548=CARTESIAN_POINT('Ctrl Pts',(-10.6961168510001,12.2,1.15151930499998));
#260549=CARTESIAN_POINT('Ctrl Pts',(-10.6986327730001,12.2,1.15107714099999));
#260550=CARTESIAN_POINT('Ctrl Pts',(-10.7011542890001,12.2,1.15063176999998));
#260551=CARTESIAN_POINT('Ctrl Pts',(-10.7036813830001,12.2,1.15018318599999));
#260552=CARTESIAN_POINT('Ctrl Pts',(-10.7062140430001,12.2,1.14973138199999));
#260553=CARTESIAN_POINT('Ctrl Pts',(-10.7087522570001,12.2,1.14927634999999));
#260554=CARTESIAN_POINT('Ctrl Pts',(-10.7112960120001,12.2,1.14881808499999));
#260555=CARTESIAN_POINT('Ctrl Pts',(-10.7138452930001,12.2,1.14835657899999));
#260556=CARTESIAN_POINT('Ctrl Pts',(-10.7164000880001,12.2,1.14789182399999));
#260557=CARTESIAN_POINT('Ctrl Pts',(-10.7189603860001,12.2,1.14742381499998));
#260558=CARTESIAN_POINT('Ctrl Pts',(-10.7215261720001,12.2,1.14695254599999));
#260559=CARTESIAN_POINT('Ctrl Pts',(-10.7240974330001,12.2,1.14647800799998));
#260560=CARTESIAN_POINT('Ctrl Pts',(-10.7266741590001,12.2,1.14600019699999));
#260561=CARTESIAN_POINT('Ctrl Pts',(-10.7292563340001,12.2,1.14551910299999));
#260562=CARTESIAN_POINT('Ctrl Pts',(-10.7318439480001,12.2,1.14503472299999));
#260563=CARTESIAN_POINT('Ctrl Pts',(-10.734955593487,12.2,1.14444951182125));
#260564=CARTESIAN_POINT('Ctrl Pts',(-10.7380753572566,12.2,1.14385935058935));
#260565=CARTESIAN_POINT('Ctrl Pts',(-10.7412032147435,12.2,1.14326422341062));
#260566=CARTESIAN_POINT('Ctrl Pts',(-10.7443391425131,12.2,1.1426641201787));
#260567=CARTESIAN_POINT('Ctrl Pts',(-10.7474831100001,12.2,1.14205902499998));
#260568=CARTESIAN_POINT('Ctrl Pts',(-10.7501084340001,12.2,1.14155144699998));
#260569=CARTESIAN_POINT('Ctrl Pts',(-10.7527390940001,12.2,1.14104052899998));
#260570=CARTESIAN_POINT('Ctrl Pts',(-10.7553750790001,12.2,1.14052626499999));
#260571=CARTESIAN_POINT('Ctrl Pts',(-10.7580163760001,12.2,1.14000864899999));
#260572=CARTESIAN_POINT('Ctrl Pts',(-10.7606629730001,12.2,1.13948767199998));
#260573=CARTESIAN_POINT('Ctrl Pts',(-10.7633148570001,12.2,1.13896333199999));
#260574=CARTESIAN_POINT('Ctrl Pts',(-10.7659720160001,12.2,1.13843561899999));
#260575=CARTESIAN_POINT('Ctrl Pts',(-10.7686344370001,12.2,1.13790452999998));
#260576=CARTESIAN_POINT('Ctrl Pts',(-10.7713021080001,12.2,1.13737005599999));
#260577=CARTESIAN_POINT('Ctrl Pts',(-10.7739750180001,12.2,1.13683219199999));
#260578=CARTESIAN_POINT('Ctrl Pts',(-10.7766531540001,12.2,1.13629093099998));
#260579=CARTESIAN_POINT('Ctrl Pts',(-10.7793365030001,12.2,1.13574626899998));
#260580=CARTESIAN_POINT('Ctrl Pts',(-10.7820250540001,12.2,1.13519819699999));
#260581=CARTESIAN_POINT('Ctrl Pts',(-10.7847187940001,12.2,1.13464671099999));
#260582=CARTESIAN_POINT('Ctrl Pts',(-10.7874177100001,12.2,1.13409180499998));
#260583=CARTESIAN_POINT('Ctrl Pts',(-10.7901217920001,12.2,1.13353347099999));
#260584=CARTESIAN_POINT('Ctrl Pts',(-10.7928310260001,12.2,1.13297170399999));
#260585=CARTESIAN_POINT('Ctrl Pts',(-10.7955454010001,12.2,1.13240649799998));
#260586=CARTESIAN_POINT('Ctrl Pts',(-10.7982649040001,12.2,1.13183784699999));
#260587=CARTESIAN_POINT('Ctrl Pts',(-10.8009895250001,12.2,1.13126574599999));
#260588=CARTESIAN_POINT('Ctrl Pts',(-10.8037192500001,12.2,1.13069018799999));
#260589=CARTESIAN_POINT('Ctrl Pts',(-10.8064540680001,12.2,1.13011116799999));
#260590=CARTESIAN_POINT('Ctrl Pts',(-10.8091939670001,12.2,1.12952867799998));
#260591=CARTESIAN_POINT('Ctrl Pts',(-10.8119389340001,12.2,1.12894271399998));
#260592=CARTESIAN_POINT('Ctrl Pts',(-10.8146889590001,12.2,1.12835326899999));
#260593=CARTESIAN_POINT('Ctrl Pts',(-10.8174440290001,12.2,1.12776033899999));
#260594=CARTESIAN_POINT('Ctrl Pts',(-10.8202041310001,12.2,1.12716391599998));
#260595=CARTESIAN_POINT('Ctrl Pts',(-10.8229692560001,12.2,1.12656399699999));
#260596=CARTESIAN_POINT('Ctrl Pts',(-10.8257393900001,12.2,1.12596057199998));
#260597=CARTESIAN_POINT('Ctrl Pts',(-10.8285145220001,12.2,1.12535363899998));
#260598=CARTESIAN_POINT('Ctrl Pts',(-10.8312946400001,12.2,1.12474319099999));
#260599=CARTESIAN_POINT('Ctrl Pts',(-10.8340797320001,12.2,1.12412922199999));
#260600=CARTESIAN_POINT('Ctrl Pts',(-10.8368697870001,12.2,1.12351172799999));
#260601=CARTESIAN_POINT('Ctrl Pts',(-10.8396647920001,12.2,1.12289069999999));
#260602=CARTESIAN_POINT('Ctrl Pts',(-10.8424647370001,12.2,1.12226613499999));
#260603=CARTESIAN_POINT('Ctrl Pts',(-10.8452696110001,12.2,1.12163802799999));
#260604=CARTESIAN_POINT('Ctrl Pts',(-10.8480794000001,12.2,1.12100637199998));
#260605=CARTESIAN_POINT('Ctrl Pts',(-10.8508940940001,12.2,1.12037116099998));
#260606=CARTESIAN_POINT('Ctrl Pts',(-10.8537136800001,12.2,1.11973238999999));
#260607=CARTESIAN_POINT('Ctrl Pts',(-10.8565381480001,12.2,1.11909005299998));
#260608=CARTESIAN_POINT('Ctrl Pts',(-10.8593674860001,12.2,1.11844414699998));
#260609=CARTESIAN_POINT('Ctrl Pts',(-10.8622016830001,12.2,1.11779466399998));
#260610=CARTESIAN_POINT('Ctrl Pts',(-10.8650407270001,12.2,1.11714159799998));
#260611=CARTESIAN_POINT('Ctrl Pts',(-10.8678846060001,12.2,1.11648494599998));
#260612=CARTESIAN_POINT('Ctrl Pts',(-10.8707333090001,12.2,1.11582469999998));
#260613=CARTESIAN_POINT('Ctrl Pts',(-10.8735868260001,12.2,1.11516085799999));
#260614=CARTESIAN_POINT('Ctrl Pts',(-10.8764451420001,12.2,1.11449341099998));
#260615=CARTESIAN_POINT('Ctrl Pts',(-10.8793082490001,12.2,1.11382235599998));
#260616=CARTESIAN_POINT('Ctrl Pts',(-10.8821761360001,12.2,1.11314768799998));
#260617=CARTESIAN_POINT('Ctrl Pts',(-10.8850487880001,12.2,1.11246939899999));
#260618=CARTESIAN_POINT('Ctrl Pts',(-10.8879261980001,12.2,1.11178748499999));
#260619=CARTESIAN_POINT('Ctrl Pts',(-10.8908083520001,12.2,1.11110194299998));
#260620=CARTESIAN_POINT('Ctrl Pts',(-10.8936952400001,12.2,1.11041276499999));
#260621=CARTESIAN_POINT('Ctrl Pts',(-10.8965868490001,12.2,1.10971994599999));
#260622=CARTESIAN_POINT('Ctrl Pts',(-10.8994831710001,12.2,1.10902348199998));
#260623=CARTESIAN_POINT('Ctrl Pts',(-10.9023841920001,12.2,1.10832336799998));
#260624=CARTESIAN_POINT('Ctrl Pts',(-10.9052899020001,12.2,1.10761959699999));
#260625=CARTESIAN_POINT('Ctrl Pts',(-10.9082002890001,12.2,1.10691216599998));
#260626=CARTESIAN_POINT('Ctrl Pts',(-10.9111153440001,12.2,1.10620106799999));
#260627=CARTESIAN_POINT('Ctrl Pts',(-10.9140350530001,12.2,1.10548629899998));
#260628=CARTESIAN_POINT('Ctrl Pts',(-10.9169594070001,12.2,1.10476785399999));
#260629=CARTESIAN_POINT('Ctrl Pts',(-10.9198883940001,12.2,1.10404572799998));
#260630=CARTESIAN_POINT('Ctrl Pts',(-10.9228220030001,12.2,1.10331991499999));
#260631=CARTESIAN_POINT('Ctrl Pts',(-10.9257602240001,12.2,1.10259041099999));
#260632=CARTESIAN_POINT('Ctrl Pts',(-10.9287030450001,12.2,1.10185720999999));
#260633=CARTESIAN_POINT('Ctrl Pts',(-10.9316504550001,12.2,1.10112030799999));
#260634=CARTESIAN_POINT('Ctrl Pts',(-10.9346024440001,12.2,1.10037969999999));
#260635=CARTESIAN_POINT('Ctrl Pts',(-10.9375590010001,12.2,1.09963537999999));
#260636=CARTESIAN_POINT('Ctrl Pts',(-10.9405201130001,12.2,1.09888734399998));
#260637=CARTESIAN_POINT('Ctrl Pts',(-10.9434857720001,12.2,1.09813558799999));
#260638=CARTESIAN_POINT('Ctrl Pts',(-10.9464559650001,12.2,1.09738010499999));
#260639=CARTESIAN_POINT('Ctrl Pts',(-10.9494306820001,12.2,1.09662089099999));
#260640=CARTESIAN_POINT('Ctrl Pts',(-10.9524099120001,12.2,1.09585794199999));
#260641=CARTESIAN_POINT('Ctrl Pts',(-10.9553936450001,12.2,1.09509125199999));
#260642=CARTESIAN_POINT('Ctrl Pts',(-10.9583818690001,12.2,1.09432081699998));
#260643=CARTESIAN_POINT('Ctrl Pts',(-10.9613745740001,12.2,1.09354663099999));
#260644=CARTESIAN_POINT('Ctrl Pts',(-10.9643717480001,12.2,1.09276869099999));
#260645=CARTESIAN_POINT('Ctrl Pts',(-10.9673733820001,12.2,1.09198699199998));
#260646=CARTESIAN_POINT('Ctrl Pts',(-10.9703794650001,12.2,1.09120152799999));
#260647=CARTESIAN_POINT('Ctrl Pts',(-10.9733899850001,12.2,1.09041229499999));
#260648=CARTESIAN_POINT('Ctrl Pts',(-10.9764049340001,12.2,1.08961928699999));
#260649=CARTESIAN_POINT('Ctrl Pts',(-10.9794242980001,12.2,1.08882250199999));
#260650=CARTESIAN_POINT('Ctrl Pts',(-10.9824480680001,12.2,1.08802193399999));
#260651=CARTESIAN_POINT('Ctrl Pts',(-10.9854762340001,12.2,1.08721757799998));
#260652=CARTESIAN_POINT('Ctrl Pts',(-10.9885087840001,12.2,1.08640942999998));
#260653=CARTESIAN_POINT('Ctrl Pts',(-10.9915457090001,12.2,1.08559748499998));
#260654=CARTESIAN_POINT('Ctrl Pts',(-10.9945869970001,12.2,1.08478173799998));
#260655=CARTESIAN_POINT('Ctrl Pts',(-10.9976326380001,12.2,1.08396218499998));
#260656=CARTESIAN_POINT('Ctrl Pts',(-11.0006826220001,12.2,1.08313882099999));
#260657=CARTESIAN_POINT('Ctrl Pts',(-11.0037369370001,12.2,1.08231164299998));
#260658=CARTESIAN_POINT('Ctrl Pts',(-11.0067955760001,12.2,1.08148064399999));
#260659=CARTESIAN_POINT('Ctrl Pts',(-11.0098585240001,12.2,1.08064582099999));
#260660=CARTESIAN_POINT('Ctrl Pts',(-11.0129257730001,12.2,1.07980717099998));
#260661=CARTESIAN_POINT('Ctrl Pts',(-11.0159973130001,12.2,1.07896468599999));
#260662=CARTESIAN_POINT('Ctrl Pts',(-11.0190731330001,12.2,1.07811836399998));
#260663=CARTESIAN_POINT('Ctrl Pts',(-11.0221532220001,12.2,1.07726820099999));
#260664=CARTESIAN_POINT('Ctrl Pts',(-11.0252375700001,12.2,1.07641418999998));
#260665=CARTESIAN_POINT('Ctrl Pts',(-11.0283261660001,12.2,1.07555632999999));
#260666=CARTESIAN_POINT('Ctrl Pts',(-11.0314190020001,12.2,1.07469461299999));
#260667=CARTESIAN_POINT('Ctrl Pts',(-11.0345160640001,12.2,1.07382903799999));
#260668=CARTESIAN_POINT('Ctrl Pts',(-11.0376173460001,12.2,1.07295959799998));
#260669=CARTESIAN_POINT('Ctrl Pts',(-11.0407228350001,12.2,1.07208629099999));
#260670=CARTESIAN_POINT('Ctrl Pts',(-11.0438325210001,12.2,1.07120911099999));
#260671=CARTESIAN_POINT('Ctrl Pts',(-11.0469463940001,12.2,1.07032805399998));
#260672=CARTESIAN_POINT('Ctrl Pts',(-11.0500644440001,12.2,1.06944311599999));
#260673=CARTESIAN_POINT('Ctrl Pts',(-11.0531866600001,12.2,1.06855429399999));
#260674=CARTESIAN_POINT('Ctrl Pts',(-11.0563130330001,12.2,1.06766158099999));
#260675=CARTESIAN_POINT('Ctrl Pts',(-11.0594435520001,12.2,1.06676497499999));
#260676=CARTESIAN_POINT('Ctrl Pts',(-11.0625782070001,12.2,1.06586446999998));
#260677=CARTESIAN_POINT('Ctrl Pts',(-11.0657169880001,12.2,1.06496006399999));
#260678=CARTESIAN_POINT('Ctrl Pts',(-11.0688598860001,12.2,1.06405175099999));
#260679=CARTESIAN_POINT('Ctrl Pts',(-11.0720068880001,12.2,1.06313952799999));
#260680=CARTESIAN_POINT('Ctrl Pts',(-11.0751579870001,12.2,1.06222338999999));
#260681=CARTESIAN_POINT('Ctrl Pts',(-11.0783131710001,12.2,1.06130333499999));
#260682=CARTESIAN_POINT('Ctrl Pts',(-11.0814724300001,12.2,1.06037935499999));
#260683=CARTESIAN_POINT('Ctrl Pts',(-11.0846357550001,12.2,1.05945144899998));
#260684=CARTESIAN_POINT('Ctrl Pts',(-11.0878031360001,12.2,1.05851961199999));
#260685=CARTESIAN_POINT('Ctrl Pts',(-11.0909745620001,12.2,1.05758383999999));
#260686=CARTESIAN_POINT('Ctrl Pts',(-11.0941500240001,12.2,1.05664412899999));
#260687=CARTESIAN_POINT('Ctrl Pts',(-11.0973295110001,12.2,1.05570047499999));
#260688=CARTESIAN_POINT('Ctrl Pts',(-11.1005130140001,12.2,1.05475287299999));
#260689=CARTESIAN_POINT('Ctrl Pts',(-11.1037005220001,12.2,1.05380132099999));
#260690=CARTESIAN_POINT('Ctrl Pts',(-11.1068920250001,12.2,1.05284581399999));
#260691=CARTESIAN_POINT('Ctrl Pts',(-11.1100875160001,12.2,1.05188634799998));
#260692=CARTESIAN_POINT('Ctrl Pts',(-11.1132869810001,12.2,1.05092291799998));
#260693=CARTESIAN_POINT('Ctrl Pts',(-11.1164904140001,12.2,1.04995552199998));
#260694=CARTESIAN_POINT('Ctrl Pts',(-11.1196978020001,12.2,1.04898415499999));
#260695=CARTESIAN_POINT('Ctrl Pts',(-11.1229091360001,12.2,1.04800881199999));
#260696=CARTESIAN_POINT('Ctrl Pts',(-11.1261244080001,12.2,1.04702949099998));
#260697=CARTESIAN_POINT('Ctrl Pts',(-11.1293436050001,12.2,1.04604618899999));
#260698=CARTESIAN_POINT('Ctrl Pts',(-11.1325667200001,12.2,1.04505889899999));
#260699=CARTESIAN_POINT('Ctrl Pts',(-11.1357937420001,12.2,1.04406762099998));
#260700=CARTESIAN_POINT('Ctrl Pts',(-11.1390246620001,12.2,1.04307234699998));
#260701=CARTESIAN_POINT('Ctrl Pts',(-11.1422594690001,12.2,1.04207307599999));
#260702=CARTESIAN_POINT('Ctrl Pts',(-11.1454981540001,12.2,1.04106980299999));
#260703=CARTESIAN_POINT('Ctrl Pts',(-11.1487407070001,12.2,1.04006252499998));
#260704=CARTESIAN_POINT('Ctrl Pts',(-11.1519871190001,12.2,1.03905123799999));
#260705=CARTESIAN_POINT('Ctrl Pts',(-11.1552373810001,12.2,1.03803593699999));
#260706=CARTESIAN_POINT('Ctrl Pts',(-11.1584914810001,12.2,1.03701662199999));
#260707=CARTESIAN_POINT('Ctrl Pts',(-11.1617494110001,12.2,1.03599328399998));
#260708=CARTESIAN_POINT('Ctrl Pts',(-11.1650111610001,12.2,1.03496592399999));
#260709=CARTESIAN_POINT('Ctrl Pts',(-11.1682767210001,12.2,1.03393453499999));
#260710=CARTESIAN_POINT('Ctrl Pts',(-11.1715460820001,12.2,1.03289911399999));
#260711=CARTESIAN_POINT('Ctrl Pts',(-11.1748192350001,12.2,1.03185965899999));
#260712=CARTESIAN_POINT('Ctrl Pts',(-11.1780961680001,12.2,1.03081616499999));
#260713=CARTESIAN_POINT('Ctrl Pts',(-11.1813768730001,12.2,1.02976862899999));
#260714=CARTESIAN_POINT('Ctrl Pts',(-11.1846613420001,12.2,1.02871704699998));
#260715=CARTESIAN_POINT('Ctrl Pts',(-11.1879495640001,12.2,1.02766141599998));
#260716=CARTESIAN_POINT('Ctrl Pts',(-11.1912415290001,12.2,1.02660173099999));
#260717=CARTESIAN_POINT('Ctrl Pts',(-11.1945372270001,12.2,1.02553798999999));
#260718=CARTESIAN_POINT('Ctrl Pts',(-11.1978366510001,12.2,1.02447018799999));
#260719=CARTESIAN_POINT('Ctrl Pts',(-11.2011397890001,12.2,1.02339832299998));
#260720=CARTESIAN_POINT('Ctrl Pts',(-11.2044466330001,12.2,1.02232238999999));
#260721=CARTESIAN_POINT('Ctrl Pts',(-11.2077571730001,12.2,1.02124238699998));
#260722=CARTESIAN_POINT('Ctrl Pts',(-11.2110714010001,12.2,1.02015830899999));
#260723=CARTESIAN_POINT('Ctrl Pts',(-11.2143893040001,12.2,1.01907015299998));
#260724=CARTESIAN_POINT('Ctrl Pts',(-11.2177108770001,12.2,1.01797791699999));
#260725=CARTESIAN_POINT('Ctrl Pts',(-11.2210361080001,12.2,1.01688159599998));
#260726=CARTESIAN_POINT('Ctrl Pts',(-11.2243649880001,12.2,1.01578118599999));
#260727=CARTESIAN_POINT('Ctrl Pts',(-11.2276975070001,12.2,1.01467668399998));
#260728=CARTESIAN_POINT('Ctrl Pts',(-11.2310336580001,12.2,1.01356808799999));
#260729=CARTESIAN_POINT('Ctrl Pts',(-11.2343734290001,12.2,1.01245539299998));
#260730=CARTESIAN_POINT('Ctrl Pts',(-11.2377168140001,12.2,1.01133859799999));
#260731=CARTESIAN_POINT('Ctrl Pts',(-11.2410637990001,12.2,1.01021769499999));
#260732=CARTESIAN_POINT('Ctrl Pts',(-11.2444143790001,12.2,1.00909268499999));
#260733=CARTESIAN_POINT('Ctrl Pts',(-11.2477685430001,12.2,1.00796356299998));
#260734=CARTESIAN_POINT('Ctrl Pts',(-11.2511262810001,12.2,1.00683032499999));
#260735=CARTESIAN_POINT('Ctrl Pts',(-11.2544875850001,12.2,1.00569296999999));
#260736=CARTESIAN_POINT('Ctrl Pts',(-11.2578524460001,12.2,1.00455149199998));
#260737=CARTESIAN_POINT('Ctrl Pts',(-11.2612208540001,12.2,1.00340588999998));
#260738=CARTESIAN_POINT('Ctrl Pts',(-11.2645927990001,12.2,1.00225615799999));
#260739=CARTESIAN_POINT('Ctrl Pts',(-11.2679682740001,12.2,1.00110229499998));
#260740=CARTESIAN_POINT('Ctrl Pts',(-11.2713472680001,12.2,0.999944296999988));
#260741=CARTESIAN_POINT('Ctrl Pts',(-11.2747297730001,12.2,0.998782160999987));
#260742=CARTESIAN_POINT('Ctrl Pts',(-11.2781157800001,12.2,0.997615882999985));
#260743=CARTESIAN_POINT('Ctrl Pts',(-11.2815052780001,12.2,0.996445461999986));
#260744=CARTESIAN_POINT('Ctrl Pts',(-11.2848982590001,12.2,0.995270892999987));
#260745=CARTESIAN_POINT('Ctrl Pts',(-11.2882947150001,12.2,0.994092171999985));
#260746=CARTESIAN_POINT('Ctrl Pts',(-11.2916946350001,12.2,0.992909295999986));
#260747=CARTESIAN_POINT('Ctrl Pts',(-11.2950980120001,12.2,0.991722263999986));
#260748=CARTESIAN_POINT('Ctrl Pts',(-11.2985048360001,12.2,0.990531070999987));
#260749=CARTESIAN_POINT('Ctrl Pts',(-11.3019150960001,12.2,0.989335713999986));
#260750=CARTESIAN_POINT('Ctrl Pts',(-11.3053287860001,12.2,0.988136191999986));
#260751=CARTESIAN_POINT('Ctrl Pts',(-11.3087458960001,12.2,0.986932498999984));
#260752=CARTESIAN_POINT('Ctrl Pts',(-11.3121664170001,12.2,0.985724631999982));
#260753=CARTESIAN_POINT('Ctrl Pts',(-11.3155903390001,12.2,0.984512589999986));
#260754=CARTESIAN_POINT('Ctrl Pts',(-11.3190176540001,12.2,0.983296368999986));
#260755=CARTESIAN_POINT('Ctrl Pts',(-11.3224483530001,12.2,0.982075965999982));
#260756=CARTESIAN_POINT('Ctrl Pts',(-11.3258824260001,12.2,0.980851377999983));
#260757=CARTESIAN_POINT('Ctrl Pts',(-11.3293198660001,12.2,0.979622600999988));
#260758=CARTESIAN_POINT('Ctrl Pts',(-11.3327606630001,12.2,0.978389632999987));
#260759=CARTESIAN_POINT('Ctrl Pts',(-11.3362048080001,12.2,0.977152470999982));
#260760=CARTESIAN_POINT('Ctrl Pts',(-11.3396522920001,12.2,0.975911110999985));
#260761=CARTESIAN_POINT('Ctrl Pts',(-11.3431031070001,12.2,0.974665550999987));
#260762=CARTESIAN_POINT('Ctrl Pts',(-11.3465572430001,12.2,0.973415788999983));
#260763=CARTESIAN_POINT('Ctrl Pts',(-11.3500146920001,12.2,0.972161818999986));
#260764=CARTESIAN_POINT('Ctrl Pts',(-11.3534754440001,12.2,0.970903640999987));
#260765=CARTESIAN_POINT('Ctrl Pts',(-11.3569394920001,12.2,0.969641250999986));
#260766=CARTESIAN_POINT('Ctrl Pts',(-11.3604068260001,12.2,0.968374645999983));
#260767=CARTESIAN_POINT('Ctrl Pts',(-11.3638774360001,12.2,0.967103821999986));
#260768=CARTESIAN_POINT('Ctrl Pts',(-11.3673513150001,12.2,0.965828777999986));
#260769=CARTESIAN_POINT('Ctrl Pts',(-11.3708284530001,12.2,0.964549509999983));
#260770=CARTESIAN_POINT('Ctrl Pts',(-11.3743088440001,12.2,0.963266015999986));
#260771=CARTESIAN_POINT('Ctrl Pts',(-11.3777924770001,12.2,0.961978291999985));
#260772=CARTESIAN_POINT('Ctrl Pts',(-11.3812793430001,12.2,0.960686337999985));
#260773=CARTESIAN_POINT('Ctrl Pts',(-11.3847694350001,12.2,0.959390146999985));
#260774=CARTESIAN_POINT('Ctrl Pts',(-11.3882627430001,12.2,0.958089718999986));
#260775=CARTESIAN_POINT('Ctrl Pts',(-11.3917592580001,12.2,0.956785048999986));
#260776=CARTESIAN_POINT('Ctrl Pts',(-11.3952589700001,12.2,0.955476136999986));
#260777=CARTESIAN_POINT('Ctrl Pts',(-11.3987618720001,12.2,0.954162976999986));
#260778=CARTESIAN_POINT('Ctrl Pts',(-11.4022679530001,12.2,0.952845567999985));
#260779=CARTESIAN_POINT('Ctrl Pts',(-11.4057772070001,12.2,0.951523905999987));
#260780=CARTESIAN_POINT('Ctrl Pts',(-11.4092896250001,12.2,0.950197990999988));
#260781=CARTESIAN_POINT('Ctrl Pts',(-11.4128052000001,12.2,0.948867817999983));
#260782=CARTESIAN_POINT('Ctrl Pts',(-11.4163239240001,12.2,0.947533386999986));
#260783=CARTESIAN_POINT('Ctrl Pts',(-11.4198457890001,12.2,0.946194692999986));
#260784=CARTESIAN_POINT('Ctrl Pts',(-11.4233707840001,12.2,0.944851733999985));
#260785=CARTESIAN_POINT('Ctrl Pts',(-11.4268989030001,12.2,0.943504507999986));
#260786=CARTESIAN_POINT('Ctrl Pts',(-11.4304301310001,12.2,0.942153010999984));
#260787=CARTESIAN_POINT('Ctrl Pts',(-11.4339644600001,12.2,0.940797237999984));
#260788=CARTESIAN_POINT('Ctrl Pts',(-11.4375018800001,12.2,0.939437186999985));
#260789=CARTESIAN_POINT('Ctrl Pts',(-11.4410423790001,12.2,0.938072855999987));
#260790=CARTESIAN_POINT('Ctrl Pts',(-11.4445859520001,12.2,0.936704240999986));
#260791=CARTESIAN_POINT('Ctrl Pts',(-11.4481325920001,12.2,0.935331340999985));
#260792=CARTESIAN_POINT('Ctrl Pts',(-11.4516822960001,12.2,0.933954156999985));
#260793=CARTESIAN_POINT('Ctrl Pts',(-11.4552350600001,12.2,0.932572684999986));
#260794=CARTESIAN_POINT('Ctrl Pts',(-11.4580797200001,12.2,0.931464077999986));
#260795=CARTESIAN_POINT('Ctrl Pts',(-11.4602145910001,12.2,0.930630692999985));
#260796=CARTESIAN_POINT('Ctrl Pts',(-11.4616384500001,12.2,0.930074245999983));
#260797=CARTESIAN_POINT('Ctrl Pts',(-11.4623505340001,12.2,0.929795807999985));
#260798=CARTESIAN_POINT('Ctrl Pts',(-11.4869855320001,15.2,0.546958305999983));
#260799=CARTESIAN_POINT('Ctrl Pts',(-11.4869855320001,11.6,0.546958305999982));
#260800=CARTESIAN_POINT('Ctrl Pts',(-11.4863150090001,15.2,0.546590898999986));
#260801=CARTESIAN_POINT('Ctrl Pts',(-11.4863150090001,11.6,0.546590898999985));
#260802=CARTESIAN_POINT('Ctrl Pts',(-11.4849742100001,15.2,0.545856550999986));
#260803=CARTESIAN_POINT('Ctrl Pts',(-11.4849742100001,11.6,0.545856550999985));
#260804=CARTESIAN_POINT('Ctrl Pts',(-11.4829637560001,15.2,0.544756421999986));
#260805=CARTESIAN_POINT('Ctrl Pts',(-11.4829637560001,11.6,0.544756421999985));
#260806=CARTESIAN_POINT('Ctrl Pts',(-11.4802846430001,15.2,0.543292367999988));
#260807=CARTESIAN_POINT('Ctrl Pts',(-11.4802846430001,11.6,0.543292367999987));
#260808=CARTESIAN_POINT('Ctrl Pts',(-11.4769382380001,15.2,0.541466945999982));
#260809=CARTESIAN_POINT('Ctrl Pts',(-11.4769382380001,11.6,0.541466945999982));
#260810=CARTESIAN_POINT('Ctrl Pts',(-11.4735943180001,15.2,0.539646165999983));
#260811=CARTESIAN_POINT('Ctrl Pts',(-11.4735943180001,11.6,0.539646165999982));
#260812=CARTESIAN_POINT('Ctrl Pts',(-11.4702528880001,15.2,0.537830029999986));
#260813=CARTESIAN_POINT('Ctrl Pts',(-11.4702528880001,11.6,0.537830029999986));
#260814=CARTESIAN_POINT('Ctrl Pts',(-11.4669139500001,15.2,0.536018536999983));
#260815=CARTESIAN_POINT('Ctrl Pts',(-11.4669139500001,11.6,0.536018536999982));
#260816=CARTESIAN_POINT('Ctrl Pts',(-11.4635775100001,15.2,0.534211684999986));
#260817=CARTESIAN_POINT('Ctrl Pts',(-11.4635775100001,11.6,0.534211684999985));
#260818=CARTESIAN_POINT('Ctrl Pts',(-11.4602435780001,15.2,0.532409473999986));
#260819=CARTESIAN_POINT('Ctrl Pts',(-11.4602435780001,11.6,0.532409473999986));
#260820=CARTESIAN_POINT('Ctrl Pts',(-11.4569121620001,15.2,0.530611900999984));
#260821=CARTESIAN_POINT('Ctrl Pts',(-11.4569121620001,11.6,0.530611900999984));
#260822=CARTESIAN_POINT('Ctrl Pts',(-11.4535832720001,15.2,0.528818965999989));
#260823=CARTESIAN_POINT('Ctrl Pts',(-11.4535832720001,11.6,0.528818965999988));
#260824=CARTESIAN_POINT('Ctrl Pts',(-11.4502569220001,15.2,0.527030663999986));
#260825=CARTESIAN_POINT('Ctrl Pts',(-11.4502569220001,11.6,0.527030663999985));
#260826=CARTESIAN_POINT('Ctrl Pts',(-11.4469331180001,15.2,0.525246995999984));
#260827=CARTESIAN_POINT('Ctrl Pts',(-11.4469331180001,11.6,0.525246995999983));
#260828=CARTESIAN_POINT('Ctrl Pts',(-11.4436118760001,15.2,0.523467958999984));
#260829=CARTESIAN_POINT('Ctrl Pts',(-11.4436118760001,11.6,0.523467958999983));
#260830=CARTESIAN_POINT('Ctrl Pts',(-11.4402932010001,15.2,0.521693550999984));
#260831=CARTESIAN_POINT('Ctrl Pts',(-11.4402932010001,11.6,0.521693550999984));
#260832=CARTESIAN_POINT('Ctrl Pts',(-11.4369771030001,15.2,0.519923770999986));
#260833=CARTESIAN_POINT('Ctrl Pts',(-11.4369771030001,11.6,0.519923770999986));
#260834=CARTESIAN_POINT('Ctrl Pts',(-11.4336635900001,15.2,0.518158617999984));
#260835=CARTESIAN_POINT('Ctrl Pts',(-11.4336635900001,11.6,0.518158617999984));
#260836=CARTESIAN_POINT('Ctrl Pts',(-11.4303526710001,15.2,0.516398088999988));
#260837=CARTESIAN_POINT('Ctrl Pts',(-11.4303526710001,11.6,0.516398088999987));
#260838=CARTESIAN_POINT('Ctrl Pts',(-11.4270443520001,15.2,0.514642183999987));
#260839=CARTESIAN_POINT('Ctrl Pts',(-11.4270443520001,11.6,0.514642183999987));
#260840=CARTESIAN_POINT('Ctrl Pts',(-11.4237386430001,15.2,0.512890900999987));
#260841=CARTESIAN_POINT('Ctrl Pts',(-11.4237386430001,11.6,0.512890900999987));
#260842=CARTESIAN_POINT('Ctrl Pts',(-11.4204355510001,15.2,0.511144238999983));
#260843=CARTESIAN_POINT('Ctrl Pts',(-11.4204355510001,11.6,0.511144238999983));
#260844=CARTESIAN_POINT('Ctrl Pts',(-11.4171350880001,15.2,0.509402193999984));
#260845=CARTESIAN_POINT('Ctrl Pts',(-11.4171350880001,11.6,0.509402193999983));
#260846=CARTESIAN_POINT('Ctrl Pts',(-11.4138372610001,15.2,0.507664766999985));
#260847=CARTESIAN_POINT('Ctrl Pts',(-11.4138372610001,11.6,0.507664766999984));
#260848=CARTESIAN_POINT('Ctrl Pts',(-11.4105420820001,15.2,0.505931953999985));
#260849=CARTESIAN_POINT('Ctrl Pts',(-11.4105420820001,11.6,0.505931953999985));
#260850=CARTESIAN_POINT('Ctrl Pts',(-11.4072495570001,15.2,0.504203755999986));
#260851=CARTESIAN_POINT('Ctrl Pts',(-11.4072495570001,11.6,0.504203755999985));
#260852=CARTESIAN_POINT('Ctrl Pts',(-11.4039596970001,15.2,0.502480167999986));
#260853=CARTESIAN_POINT('Ctrl Pts',(-11.4039596970001,11.6,0.502480167999985));
#260854=CARTESIAN_POINT('Ctrl Pts',(-11.4006725110001,15.2,0.500761190999985));
#260855=CARTESIAN_POINT('Ctrl Pts',(-11.4006725110001,11.6,0.500761190999985));
#260856=CARTESIAN_POINT('Ctrl Pts',(-11.3973880080001,15.2,0.499046821999984));
#260857=CARTESIAN_POINT('Ctrl Pts',(-11.3973880080001,11.6,0.499046821999984));
#260858=CARTESIAN_POINT('Ctrl Pts',(-11.3941061970001,15.2,0.497337060999987));
#260859=CARTESIAN_POINT('Ctrl Pts',(-11.3941061970001,11.6,0.497337060999987));
#260860=CARTESIAN_POINT('Ctrl Pts',(-11.3908270860001,15.2,0.495631902999989));
#260861=CARTESIAN_POINT('Ctrl Pts',(-11.3908270860001,11.6,0.495631902999988));
#260862=CARTESIAN_POINT('Ctrl Pts',(-11.3875506850001,15.2,0.493931348999985));
#260863=CARTESIAN_POINT('Ctrl Pts',(-11.3875506850001,11.6,0.493931348999985));
#260864=CARTESIAN_POINT('Ctrl Pts',(-11.3842770020001,15.2,0.492235395999985));
#260865=CARTESIAN_POINT('Ctrl Pts',(-11.3842770020001,11.6,0.492235395999984));
#260866=CARTESIAN_POINT('Ctrl Pts',(-11.3810060480001,15.2,0.490544042999983));
#260867=CARTESIAN_POINT('Ctrl Pts',(-11.3810060480001,11.6,0.490544042999983));
#260868=CARTESIAN_POINT('Ctrl Pts',(-11.3777378300001,15.2,0.488857287999984));
#260869=CARTESIAN_POINT('Ctrl Pts',(-11.3777378300001,11.6,0.488857287999984));
#260870=CARTESIAN_POINT('Ctrl Pts',(-11.3744723580001,15.2,0.487175127999984));
#260871=CARTESIAN_POINT('Ctrl Pts',(-11.3744723580001,11.6,0.487175127999983));
#260872=CARTESIAN_POINT('Ctrl Pts',(-11.3712096420001,15.2,0.485497562999986));
#260873=CARTESIAN_POINT('Ctrl Pts',(-11.3712096420001,11.6,0.485497562999985));
#260874=CARTESIAN_POINT('Ctrl Pts',(-11.3679496900001,15.2,0.483824590999986));
#260875=CARTESIAN_POINT('Ctrl Pts',(-11.3679496900001,11.6,0.483824590999986));
#260876=CARTESIAN_POINT('Ctrl Pts',(-11.3646925130001,15.2,0.482156208999989));
#260877=CARTESIAN_POINT('Ctrl Pts',(-11.3646925130001,11.6,0.482156208999988));
#260878=CARTESIAN_POINT('Ctrl Pts',(-11.3614381180001,15.2,0.480492415999985));
#260879=CARTESIAN_POINT('Ctrl Pts',(-11.3614381180001,11.6,0.480492415999984));
#260880=CARTESIAN_POINT('Ctrl Pts',(-11.3581865150001,15.2,0.478833208999987));
#260881=CARTESIAN_POINT('Ctrl Pts',(-11.3581865150001,11.6,0.478833208999986));
#260882=CARTESIAN_POINT('Ctrl Pts',(-11.3549377140001,15.2,0.477178588999987));
#260883=CARTESIAN_POINT('Ctrl Pts',(-11.3549377140001,11.6,0.477178588999986));
#260884=CARTESIAN_POINT('Ctrl Pts',(-11.3516917240001,15.2,0.475528550999984));
#260885=CARTESIAN_POINT('Ctrl Pts',(-11.3516917240001,11.6,0.475528550999984));
#260886=CARTESIAN_POINT('Ctrl Pts',(-11.3484485530001,15.2,0.473883093999987));
#260887=CARTESIAN_POINT('Ctrl Pts',(-11.3484485530001,11.6,0.473883093999987));
#260888=CARTESIAN_POINT('Ctrl Pts',(-11.3452082120001,15.2,0.472242216999987));
#260889=CARTESIAN_POINT('Ctrl Pts',(-11.3452082120001,11.6,0.472242216999987));
#260890=CARTESIAN_POINT('Ctrl Pts',(-11.3419707090001,15.2,0.470605916999984));
#260891=CARTESIAN_POINT('Ctrl Pts',(-11.3419707090001,11.6,0.470605916999984));
#260892=CARTESIAN_POINT('Ctrl Pts',(-11.3387360540001,15.2,0.468974193999987));
#260893=CARTESIAN_POINT('Ctrl Pts',(-11.3387360540001,11.6,0.468974193999987));
#260894=CARTESIAN_POINT('Ctrl Pts',(-11.3355042560001,15.2,0.467347044999986));
#260895=CARTESIAN_POINT('Ctrl Pts',(-11.3355042560001,11.6,0.467347044999986));
#260896=CARTESIAN_POINT('Ctrl Pts',(-11.3322753250001,15.2,0.465724465999986));
#260897=CARTESIAN_POINT('Ctrl Pts',(-11.3322753250001,11.6,0.465724465999986));
#260898=CARTESIAN_POINT('Ctrl Pts',(-11.3290492700001,15.2,0.464106457999982));
#260899=CARTESIAN_POINT('Ctrl Pts',(-11.3290492700001,11.6,0.464106457999982));
#260900=CARTESIAN_POINT('Ctrl Pts',(-11.3258260990001,15.2,0.462493017999983));
#260901=CARTESIAN_POINT('Ctrl Pts',(-11.3258260990001,11.6,0.462493017999983));
#260902=CARTESIAN_POINT('Ctrl Pts',(-11.3226058230001,15.2,0.460884142999984));
#260903=CARTESIAN_POINT('Ctrl Pts',(-11.3226058230001,11.6,0.460884142999984));
#260904=CARTESIAN_POINT('Ctrl Pts',(-11.3193884510001,15.2,0.459279831999986));
#260905=CARTESIAN_POINT('Ctrl Pts',(-11.3193884510001,11.6,0.459279831999985));
#260906=CARTESIAN_POINT('Ctrl Pts',(-11.3161739920001,15.2,0.457680083999983));
#260907=CARTESIAN_POINT('Ctrl Pts',(-11.3161739920001,11.6,0.457680083999982));
#260908=CARTESIAN_POINT('Ctrl Pts',(-11.3129624580001,15.2,0.456084895999984));
#260909=CARTESIAN_POINT('Ctrl Pts',(-11.3129624580001,11.6,0.456084895999984));
#260910=CARTESIAN_POINT('Ctrl Pts',(-11.3097538530001,15.2,0.454494265999985));
#260911=CARTESIAN_POINT('Ctrl Pts',(-11.3097538530001,11.6,0.454494265999985));
#260912=CARTESIAN_POINT('Ctrl Pts',(-11.3065481920001,15.2,0.452908190999985));
#260913=CARTESIAN_POINT('Ctrl Pts',(-11.3065481920001,11.6,0.452908190999985));
#260914=CARTESIAN_POINT('Ctrl Pts',(-11.3033454810001,15.2,0.451326670999985));
#260915=CARTESIAN_POINT('Ctrl Pts',(-11.3033454810001,11.6,0.451326670999985));
#260916=CARTESIAN_POINT('Ctrl Pts',(-11.3001457320001,15.2,0.449749702999984));
#260917=CARTESIAN_POINT('Ctrl Pts',(-11.3001457320001,11.6,0.449749702999984));
#260918=CARTESIAN_POINT('Ctrl Pts',(-11.2969489510001,15.2,0.448177283999982));
#260919=CARTESIAN_POINT('Ctrl Pts',(-11.2969489510001,11.6,0.448177283999982));
#260920=CARTESIAN_POINT('Ctrl Pts',(-11.2937551520001,15.2,0.446609412999983));
#260921=CARTESIAN_POINT('Ctrl Pts',(-11.2937551520001,11.6,0.446609412999983));
#260922=CARTESIAN_POINT('Ctrl Pts',(-11.2905643410001,15.2,0.445046087999987));
#260923=CARTESIAN_POINT('Ctrl Pts',(-11.2905643410001,11.6,0.445046087999987));
#260924=CARTESIAN_POINT('Ctrl Pts',(-11.2873765290001,15.2,0.443487306999986));
#260925=CARTESIAN_POINT('Ctrl Pts',(-11.2873765290001,11.6,0.443487306999985));
#260926=CARTESIAN_POINT('Ctrl Pts',(-11.2841917260001,15.2,0.441933066999987));
#260927=CARTESIAN_POINT('Ctrl Pts',(-11.2841917260001,11.6,0.441933066999986));
#260928=CARTESIAN_POINT('Ctrl Pts',(-11.2810099400001,15.2,0.440383366999986));
#260929=CARTESIAN_POINT('Ctrl Pts',(-11.2810099400001,11.6,0.440383366999985));
#260930=CARTESIAN_POINT('Ctrl Pts',(-11.2778311820001,15.2,0.438838203999987));
#260931=CARTESIAN_POINT('Ctrl Pts',(-11.2778311820001,11.6,0.438838203999987));
#260932=CARTESIAN_POINT('Ctrl Pts',(-11.2746554610001,15.2,0.437297575999986));
#260933=CARTESIAN_POINT('Ctrl Pts',(-11.2746554610001,11.6,0.437297575999986));
#260934=CARTESIAN_POINT('Ctrl Pts',(-11.2714827870001,15.2,0.435761481999983));
#260935=CARTESIAN_POINT('Ctrl Pts',(-11.2714827870001,11.6,0.435761481999983));
#260936=CARTESIAN_POINT('Ctrl Pts',(-11.2683131690001,15.2,0.434229917999982));
#260937=CARTESIAN_POINT('Ctrl Pts',(-11.2683131690001,11.6,0.434229917999982));
#260938=CARTESIAN_POINT('Ctrl Pts',(-11.2651466170001,15.2,0.432702882999987));
#260939=CARTESIAN_POINT('Ctrl Pts',(-11.2651466170001,11.6,0.432702882999986));
#260940=CARTESIAN_POINT('Ctrl Pts',(-11.2619831420001,15.2,0.431180374999984));
#260941=CARTESIAN_POINT('Ctrl Pts',(-11.2619831420001,11.6,0.431180374999984));
#260942=CARTESIAN_POINT('Ctrl Pts',(-11.2588227510001,15.2,0.429662389999983));
#260943=CARTESIAN_POINT('Ctrl Pts',(-11.2588227510001,11.6,0.429662389999983));
#260944=CARTESIAN_POINT('Ctrl Pts',(-11.2556654560001,15.2,0.428148927999987));
#260945=CARTESIAN_POINT('Ctrl Pts',(-11.2556654560001,11.6,0.428148927999987));
#260946=CARTESIAN_POINT('Ctrl Pts',(-11.2525112650001,15.2,0.426639985999984));
#260947=CARTESIAN_POINT('Ctrl Pts',(-11.2525112650001,11.6,0.426639985999983));
#260948=CARTESIAN_POINT('Ctrl Pts',(-11.2493601900001,15.2,0.425135561999985));
#260949=CARTESIAN_POINT('Ctrl Pts',(-11.2493601900001,11.6,0.425135561999985));
#260950=CARTESIAN_POINT('Ctrl Pts',(-11.2462122380001,15.2,0.423635652999987));
#260951=CARTESIAN_POINT('Ctrl Pts',(-11.2462122380001,11.6,0.423635652999987));
#260952=CARTESIAN_POINT('Ctrl Pts',(-11.2430674210001,15.2,0.422140256999985));
#260953=CARTESIAN_POINT('Ctrl Pts',(-11.2430674210001,11.6,0.422140256999985));
#260954=CARTESIAN_POINT('Ctrl Pts',(-11.2399257470001,15.2,0.420649372999984));
#260955=CARTESIAN_POINT('Ctrl Pts',(-11.2399257470001,11.6,0.420649372999983));
#260956=CARTESIAN_POINT('Ctrl Pts',(-11.2367872280001,15.2,0.419162996999987));
#260957=CARTESIAN_POINT('Ctrl Pts',(-11.2367872280001,11.6,0.419162996999986));
#260958=CARTESIAN_POINT('Ctrl Pts',(-11.2336518720001,15.2,0.417681126999985));
#260959=CARTESIAN_POINT('Ctrl Pts',(-11.2336518720001,11.6,0.417681126999984));
#260960=CARTESIAN_POINT('Ctrl Pts',(-11.2305196890001,15.2,0.416203761999987));
#260961=CARTESIAN_POINT('Ctrl Pts',(-11.2305196890001,11.6,0.416203761999987));
#260962=CARTESIAN_POINT('Ctrl Pts',(-11.2273906900001,15.2,0.414730897999984));
#260963=CARTESIAN_POINT('Ctrl Pts',(-11.2273906900001,11.6,0.414730897999984));
#260964=CARTESIAN_POINT('Ctrl Pts',(-11.2242648840001,15.2,0.413262533999985));
#260965=CARTESIAN_POINT('Ctrl Pts',(-11.2242648840001,11.6,0.413262533999985));
#260966=CARTESIAN_POINT('Ctrl Pts',(-11.2211422810001,15.2,0.411798666999985));
#260967=CARTESIAN_POINT('Ctrl Pts',(-11.2211422810001,11.6,0.411798666999985));
#260968=CARTESIAN_POINT('Ctrl Pts',(-11.2180228910001,15.2,0.410339293999984));
#260969=CARTESIAN_POINT('Ctrl Pts',(-11.2180228910001,11.6,0.410339293999983));
#260970=CARTESIAN_POINT('Ctrl Pts',(-11.2149067230001,15.2,0.408884414999986));
#260971=CARTESIAN_POINT('Ctrl Pts',(-11.2149067230001,11.6,0.408884414999986));
#260972=CARTESIAN_POINT('Ctrl Pts',(-11.2117937880001,15.2,0.407434024999986));
#260973=CARTESIAN_POINT('Ctrl Pts',(-11.2117937880001,11.6,0.407434024999986));
#260974=CARTESIAN_POINT('Ctrl Pts',(-11.2086840970001,15.2,0.405988122999985));
#260975=CARTESIAN_POINT('Ctrl Pts',(-11.2086840970001,11.6,0.405988122999985));
#260976=CARTESIAN_POINT('Ctrl Pts',(-11.2055776580001,15.2,0.404546704999986));
#260977=CARTESIAN_POINT('Ctrl Pts',(-11.2055776580001,11.6,0.404546704999986));
#260978=CARTESIAN_POINT('Ctrl Pts',(-11.2024744820001,15.2,0.403109771999985));
#260979=CARTESIAN_POINT('Ctrl Pts',(-11.2024744820001,11.6,0.403109771999985));
#260980=CARTESIAN_POINT('Ctrl Pts',(-11.1993745780001,15.2,0.401677316999987));
#260981=CARTESIAN_POINT('Ctrl Pts',(-11.1993745780001,11.6,0.401677316999986));
#260982=CARTESIAN_POINT('Ctrl Pts',(-11.1962779570001,15.2,0.400249341999985));
#260983=CARTESIAN_POINT('Ctrl Pts',(-11.1962779570001,11.6,0.400249341999985));
#260984=CARTESIAN_POINT('Ctrl Pts',(-11.1931846300001,15.2,0.398825840999986));
#260985=CARTESIAN_POINT('Ctrl Pts',(-11.1931846300001,11.6,0.398825840999985));
#260986=CARTESIAN_POINT('Ctrl Pts',(-11.1900946040001,15.2,0.397406813999983));
#260987=CARTESIAN_POINT('Ctrl Pts',(-11.1900946040001,11.6,0.397406813999983));
#260988=CARTESIAN_POINT('Ctrl Pts',(-11.1870078920001,15.2,0.395992257999982));
#260989=CARTESIAN_POINT('Ctrl Pts',(-11.1870078920001,11.6,0.395992257999982));
#260990=CARTESIAN_POINT('Ctrl Pts',(-11.1839245020001,15.2,0.394582169999986));
#260991=CARTESIAN_POINT('Ctrl Pts',(-11.1839245020001,11.6,0.394582169999986));
#260992=CARTESIAN_POINT('Ctrl Pts',(-11.1808444470001,15.2,0.393176545999987));
#260993=CARTESIAN_POINT('Ctrl Pts',(-11.1808444470001,11.6,0.393176545999987));
#260994=CARTESIAN_POINT('Ctrl Pts',(-11.1777677340001,15.2,0.391775386999988));
#260995=CARTESIAN_POINT('Ctrl Pts',(-11.1777677340001,11.6,0.391775386999988));
#260996=CARTESIAN_POINT('Ctrl Pts',(-11.1746943740001,15.2,0.390378687999986));
#260997=CARTESIAN_POINT('Ctrl Pts',(-11.1746943740001,11.6,0.390378687999986));
#260998=CARTESIAN_POINT('Ctrl Pts',(-11.1716243780001,15.2,0.388986446999984));
#260999=CARTESIAN_POINT('Ctrl Pts',(-11.1716243780001,11.6,0.388986446999983));
#261000=CARTESIAN_POINT('Ctrl Pts',(-11.1685577570001,15.2,0.387598660999986));
#261001=CARTESIAN_POINT('Ctrl Pts',(-11.1685577570001,11.6,0.387598660999986));
#261002=CARTESIAN_POINT('Ctrl Pts',(-11.1654945190001,15.2,0.386215327999988));
#261003=CARTESIAN_POINT('Ctrl Pts',(-11.1654945190001,11.6,0.386215327999988));
#261004=CARTESIAN_POINT('Ctrl Pts',(-11.1624346740001,15.2,0.384836445999985));
#261005=CARTESIAN_POINT('Ctrl Pts',(-11.1624346740001,11.6,0.384836445999985));
#261006=CARTESIAN_POINT('Ctrl Pts',(-11.1593782350001,15.2,0.383462010999986));
#261007=CARTESIAN_POINT('Ctrl Pts',(-11.1593782350001,11.6,0.383462010999986));
#261008=CARTESIAN_POINT('Ctrl Pts',(-11.1563252100001,15.2,0.382092021999987));
#261009=CARTESIAN_POINT('Ctrl Pts',(-11.1563252100001,11.6,0.382092021999986));
#261010=CARTESIAN_POINT('Ctrl Pts',(-11.1532756110001,15.2,0.380726473999986));
#261011=CARTESIAN_POINT('Ctrl Pts',(-11.1532756110001,11.6,0.380726473999986));
#261012=CARTESIAN_POINT('Ctrl Pts',(-11.1502294460001,15.2,0.379365366999984));
#261013=CARTESIAN_POINT('Ctrl Pts',(-11.1502294460001,11.6,0.379365366999984));
#261014=CARTESIAN_POINT('Ctrl Pts',(-11.1471867270001,15.2,0.378008696999985));
#261015=CARTESIAN_POINT('Ctrl Pts',(-11.1471867270001,11.6,0.378008696999985));
#261016=CARTESIAN_POINT('Ctrl Pts',(-11.1441474640001,15.2,0.376656461999989));
#261017=CARTESIAN_POINT('Ctrl Pts',(-11.1441474640001,11.6,0.376656461999989));
#261018=CARTESIAN_POINT('Ctrl Pts',(-11.1411116670001,15.2,0.375308657999986));
#261019=CARTESIAN_POINT('Ctrl Pts',(-11.1411116670001,11.6,0.375308657999986));
#261020=CARTESIAN_POINT('Ctrl Pts',(-11.1380793470001,15.2,0.373965283999986));
#261021=CARTESIAN_POINT('Ctrl Pts',(-11.1380793470001,11.6,0.373965283999986));
#261022=CARTESIAN_POINT('Ctrl Pts',(-11.1350505130001,15.2,0.372626335999984));
#261023=CARTESIAN_POINT('Ctrl Pts',(-11.1350505130001,11.6,0.372626335999983));
#261024=CARTESIAN_POINT('Ctrl Pts',(-11.1320251780001,15.2,0.371291811999988));
#261025=CARTESIAN_POINT('Ctrl Pts',(-11.1320251780001,11.6,0.371291811999987));
#261026=CARTESIAN_POINT('Ctrl Pts',(-11.1290033490001,15.2,0.369961708999984));
#261027=CARTESIAN_POINT('Ctrl Pts',(-11.1290033490001,11.6,0.369961708999984));
#261028=CARTESIAN_POINT('Ctrl Pts',(-11.1259850390001,15.2,0.368636023999986));
#261029=CARTESIAN_POINT('Ctrl Pts',(-11.1259850390001,11.6,0.368636023999986));
#261030=CARTESIAN_POINT('Ctrl Pts',(-11.1229702580001,15.2,0.367314754999986));
#261031=CARTESIAN_POINT('Ctrl Pts',(-11.1229702580001,11.6,0.367314754999985));
#261032=CARTESIAN_POINT('Ctrl Pts',(-11.1199590150001,15.2,0.365997898999986));
#261033=CARTESIAN_POINT('Ctrl Pts',(-11.1199590150001,11.6,0.365997898999985));
#261034=CARTESIAN_POINT('Ctrl Pts',(-11.1169513230001,15.2,0.364685452999982));
#261035=CARTESIAN_POINT('Ctrl Pts',(-11.1169513230001,11.6,0.364685452999982));
#261036=CARTESIAN_POINT('Ctrl Pts',(-11.1139471900001,15.2,0.363377413999988));
#261037=CARTESIAN_POINT('Ctrl Pts',(-11.1139471900001,11.6,0.363377413999987));
#261038=CARTESIAN_POINT('Ctrl Pts',(-11.1109466290001,15.2,0.362073778999985));
#261039=CARTESIAN_POINT('Ctrl Pts',(-11.1109466290001,11.6,0.362073778999985));
#261040=CARTESIAN_POINT('Ctrl Pts',(-11.1079496490001,15.2,0.360774545999987));
#261041=CARTESIAN_POINT('Ctrl Pts',(-11.1079496490001,11.6,0.360774545999986));
#261042=CARTESIAN_POINT('Ctrl Pts',(-11.1049562600001,15.2,0.359479711999988));
#261043=CARTESIAN_POINT('Ctrl Pts',(-11.1049562600001,11.6,0.359479711999988));
#261044=CARTESIAN_POINT('Ctrl Pts',(-11.1019664740001,15.2,0.358189272999985));
#261045=CARTESIAN_POINT('Ctrl Pts',(-11.1019664740001,11.6,0.358189272999984));
#261046=CARTESIAN_POINT('Ctrl Pts',(-11.0989803000001,15.2,0.356903227999985));
#261047=CARTESIAN_POINT('Ctrl Pts',(-11.0989803000001,11.6,0.356903227999985));
#261048=CARTESIAN_POINT('Ctrl Pts',(-11.0959977500001,15.2,0.355621572999985));
#261049=CARTESIAN_POINT('Ctrl Pts',(-11.0959977500001,11.6,0.355621572999984));
#261050=CARTESIAN_POINT('Ctrl Pts',(-11.0930188360001,15.2,0.354344304999987));
#261051=CARTESIAN_POINT('Ctrl Pts',(-11.0930188360001,11.6,0.354344304999987));
#261052=CARTESIAN_POINT('Ctrl Pts',(-11.0900435650001,15.2,0.353071420999989));
#261053=CARTESIAN_POINT('Ctrl Pts',(-11.0900435650001,11.6,0.353071420999988));
#261054=CARTESIAN_POINT('Ctrl Pts',(-11.0870719500001,15.2,0.351802918999984));
#261055=CARTESIAN_POINT('Ctrl Pts',(-11.0870719500001,11.6,0.351802918999983));
#261056=CARTESIAN_POINT('Ctrl Pts',(-11.0841040020001,15.2,0.350538794999986));
#261057=CARTESIAN_POINT('Ctrl Pts',(-11.0841040020001,11.6,0.350538794999986));
#261058=CARTESIAN_POINT('Ctrl Pts',(-11.0811397300001,15.2,0.349279046999986));
#261059=CARTESIAN_POINT('Ctrl Pts',(-11.0811397300001,11.6,0.349279046999986));
#261060=CARTESIAN_POINT('Ctrl Pts',(-11.0781791480001,15.2,0.348023670999984));
#261061=CARTESIAN_POINT('Ctrl Pts',(-11.0781791480001,11.6,0.348023670999984));
#261062=CARTESIAN_POINT('Ctrl Pts',(-11.0752222620001,15.2,0.346772664999988));
#261063=CARTESIAN_POINT('Ctrl Pts',(-11.0752222620001,11.6,0.346772664999988));
#261064=CARTESIAN_POINT('Ctrl Pts',(-11.0722690870001,15.2,0.345526024999985));
#261065=CARTESIAN_POINT('Ctrl Pts',(-11.0722690870001,11.6,0.345526024999984));
#261066=CARTESIAN_POINT('Ctrl Pts',(-11.0693196320001,15.2,0.344283748999987));
#261067=CARTESIAN_POINT('Ctrl Pts',(-11.0693196320001,11.6,0.344283748999987));
#261068=CARTESIAN_POINT('Ctrl Pts',(-11.0663739070001,15.2,0.343045833999986));
#261069=CARTESIAN_POINT('Ctrl Pts',(-11.0663739070001,11.6,0.343045833999986));
#261070=CARTESIAN_POINT('Ctrl Pts',(-11.0634319250001,15.2,0.341812274999986));
#261071=CARTESIAN_POINT('Ctrl Pts',(-11.0634319250001,11.6,0.341812274999986));
#261072=CARTESIAN_POINT('Ctrl Pts',(-11.0604936960001,15.2,0.340583071999987));
#261073=CARTESIAN_POINT('Ctrl Pts',(-11.0604936960001,11.6,0.340583071999986));
#261074=CARTESIAN_POINT('Ctrl Pts',(-11.0575592300001,15.2,0.339358219999983));
#261075=CARTESIAN_POINT('Ctrl Pts',(-11.0575592300001,11.6,0.339358219999983));
#261076=CARTESIAN_POINT('Ctrl Pts',(-11.0546285370001,15.2,0.338137715999984));
#261077=CARTESIAN_POINT('Ctrl Pts',(-11.0546285370001,11.6,0.338137715999984));
#261078=CARTESIAN_POINT('Ctrl Pts',(-11.0517016320001,15.2,0.336921557999985));
#261079=CARTESIAN_POINT('Ctrl Pts',(-11.0517016320001,11.6,0.336921557999985));
#261080=CARTESIAN_POINT('Ctrl Pts',(-11.0487785220001,15.2,0.335709739999985));
#261081=CARTESIAN_POINT('Ctrl Pts',(-11.0487785220001,11.6,0.335709739999985));
#261082=CARTESIAN_POINT('Ctrl Pts',(-11.0458592200001,15.2,0.334502262999985));
#261083=CARTESIAN_POINT('Ctrl Pts',(-11.0458592200001,11.6,0.334502262999985));
#261084=CARTESIAN_POINT('Ctrl Pts',(-11.0429437360001,15.2,0.333299120999988));
#261085=CARTESIAN_POINT('Ctrl Pts',(-11.0429437360001,11.6,0.333299120999988));
#261086=CARTESIAN_POINT('Ctrl Pts',(-11.0400320810001,15.2,0.332100310999985));
#261087=CARTESIAN_POINT('Ctrl Pts',(-11.0400320810001,11.6,0.332100310999985));
#261088=CARTESIAN_POINT('Ctrl Pts',(-11.0371242670001,15.2,0.330905830999986));
#261089=CARTESIAN_POINT('Ctrl Pts',(-11.0371242670001,11.6,0.330905830999985));
#261090=CARTESIAN_POINT('Ctrl Pts',(-11.0342203030001,15.2,0.329715676999989));
#261091=CARTESIAN_POINT('Ctrl Pts',(-11.0342203030001,11.6,0.329715676999988));
#261092=CARTESIAN_POINT('Ctrl Pts',(-11.0313202040001,15.2,0.328529845999985));
#261093=CARTESIAN_POINT('Ctrl Pts',(-11.0313202040001,11.6,0.328529845999985));
#261094=CARTESIAN_POINT('Ctrl Pts',(-11.0284239770001,15.2,0.327348335999984));
#261095=CARTESIAN_POINT('Ctrl Pts',(-11.0284239770001,11.6,0.327348335999984));
#261096=CARTESIAN_POINT('Ctrl Pts',(-11.0255316350001,15.2,0.326171140999989));
#261097=CARTESIAN_POINT('Ctrl Pts',(-11.0255316350001,11.6,0.326171140999989));
#261098=CARTESIAN_POINT('Ctrl Pts',(-11.0226431890001,15.2,0.324998259999987));
#261099=CARTESIAN_POINT('Ctrl Pts',(-11.0226431890001,11.6,0.324998259999986));
#261100=CARTESIAN_POINT('Ctrl Pts',(-11.0197586510001,15.2,0.323829688999986));
#261101=CARTESIAN_POINT('Ctrl Pts',(-11.0197586510001,11.6,0.323829688999985));
#261102=CARTESIAN_POINT('Ctrl Pts',(-11.0168780300001,15.2,0.322665424999986));
#261103=CARTESIAN_POINT('Ctrl Pts',(-11.0168780300001,11.6,0.322665424999986));
#261104=CARTESIAN_POINT('Ctrl Pts',(-11.0140013380001,15.2,0.321505463999987));
#261105=CARTESIAN_POINT('Ctrl Pts',(-11.0140013380001,11.6,0.321505463999987));
#261106=CARTESIAN_POINT('Ctrl Pts',(-11.0111285880001,15.2,0.320349803999989));
#261107=CARTESIAN_POINT('Ctrl Pts',(-11.0111285880001,11.6,0.320349803999988));
#261108=CARTESIAN_POINT('Ctrl Pts',(-11.0082597890001,15.2,0.319198439999986));
#261109=CARTESIAN_POINT('Ctrl Pts',(-11.0082597890001,11.6,0.319198439999985));
#261110=CARTESIAN_POINT('Ctrl Pts',(-11.0053949540001,15.2,0.318051369999988));
#261111=CARTESIAN_POINT('Ctrl Pts',(-11.0053949540001,11.6,0.318051369999987));
#261112=CARTESIAN_POINT('Ctrl Pts',(-11.0025340930001,15.2,0.316908588999985));
#261113=CARTESIAN_POINT('Ctrl Pts',(-11.0025340930001,11.6,0.316908588999984));
#261114=CARTESIAN_POINT('Ctrl Pts',(-10.9996772170001,15.2,0.315770094999985));
#261115=CARTESIAN_POINT('Ctrl Pts',(-10.9996772170001,11.6,0.315770094999985));
#261116=CARTESIAN_POINT('Ctrl Pts',(-10.9968243390001,15.2,0.314635884999985));
#261117=CARTESIAN_POINT('Ctrl Pts',(-10.9968243390001,11.6,0.314635884999985));
#261118=CARTESIAN_POINT('Ctrl Pts',(-10.9939754690001,15.2,0.313505953999984));
#261119=CARTESIAN_POINT('Ctrl Pts',(-10.9939754690001,11.6,0.313505953999984));
#261120=CARTESIAN_POINT('Ctrl Pts',(-10.9911306190001,15.2,0.312380299999986));
#261121=CARTESIAN_POINT('Ctrl Pts',(-10.9911306190001,11.6,0.312380299999985));
#261122=CARTESIAN_POINT('Ctrl Pts',(-10.9882898000001,15.2,0.311258919999986));
#261123=CARTESIAN_POINT('Ctrl Pts',(-10.9882898000001,11.6,0.311258919999986));
#261124=CARTESIAN_POINT('Ctrl Pts',(-10.9854530250001,15.2,0.310141807999984));
#261125=CARTESIAN_POINT('Ctrl Pts',(-10.9854530250001,11.6,0.310141807999984));
#261126=CARTESIAN_POINT('Ctrl Pts',(-10.9826203020001,15.2,0.309028961999989));
#261127=CARTESIAN_POINT('Ctrl Pts',(-10.9826203020001,11.6,0.309028961999988));
#261128=CARTESIAN_POINT('Ctrl Pts',(-10.9797916470001,15.2,0.307920378999986));
#261129=CARTESIAN_POINT('Ctrl Pts',(-10.9797916470001,11.6,0.307920378999986));
#261130=CARTESIAN_POINT('Ctrl Pts',(-10.9769670670001,15.2,0.306816054999985));
#261131=CARTESIAN_POINT('Ctrl Pts',(-10.9769670670001,11.6,0.306816054999985));
#261132=CARTESIAN_POINT('Ctrl Pts',(-10.9741465770001,15.2,0.305715986999986));
#261133=CARTESIAN_POINT('Ctrl Pts',(-10.9741465770001,11.6,0.305715986999985));
#261134=CARTESIAN_POINT('Ctrl Pts',(-10.9713301870001,15.2,0.304620170999983));
#261135=CARTESIAN_POINT('Ctrl Pts',(-10.9713301870001,11.6,0.304620170999983));
#261136=CARTESIAN_POINT('Ctrl Pts',(-10.9685179070001,15.2,0.303528602999985));
#261137=CARTESIAN_POINT('Ctrl Pts',(-10.9685179070001,11.6,0.303528602999985));
#261138=CARTESIAN_POINT('Ctrl Pts',(-10.9657097520001,15.2,0.302441278999983));
#261139=CARTESIAN_POINT('Ctrl Pts',(-10.9657097520001,11.6,0.302441278999983));
#261140=CARTESIAN_POINT('Ctrl Pts',(-10.9629057310001,15.2,0.301358197999986));
#261141=CARTESIAN_POINT('Ctrl Pts',(-10.9629057310001,11.6,0.301358197999985));
#261142=CARTESIAN_POINT('Ctrl Pts',(-10.9601058580001,15.2,0.300279352999984));
#261143=CARTESIAN_POINT('Ctrl Pts',(-10.9601058580001,11.6,0.300279352999983));
#261144=CARTESIAN_POINT('Ctrl Pts',(-10.9573101410001,15.2,0.299204742999986));
#261145=CARTESIAN_POINT('Ctrl Pts',(-10.9573101410001,11.6,0.299204742999985));
#261146=CARTESIAN_POINT('Ctrl Pts',(-10.9545185950001,15.2,0.298134361999987));
#261147=CARTESIAN_POINT('Ctrl Pts',(-10.9545185950001,11.6,0.298134361999986));
#261148=CARTESIAN_POINT('Ctrl Pts',(-10.9517312310001,15.2,0.297068208999987));
#261149=CARTESIAN_POINT('Ctrl Pts',(-10.9517312310001,11.6,0.297068208999986));
#261150=CARTESIAN_POINT('Ctrl Pts',(-10.9489480600001,15.2,0.296006278999985));
#261151=CARTESIAN_POINT('Ctrl Pts',(-10.9489480600001,11.6,0.296006278999985));
#261152=CARTESIAN_POINT('Ctrl Pts',(-10.9461690940001,15.2,0.294948567999986));
#261153=CARTESIAN_POINT('Ctrl Pts',(-10.9461690940001,11.6,0.294948567999986));
#261154=CARTESIAN_POINT('Ctrl Pts',(-10.9433943440001,15.2,0.293895071999986));
#261155=CARTESIAN_POINT('Ctrl Pts',(-10.9433943440001,11.6,0.293895071999985));
#261156=CARTESIAN_POINT('Ctrl Pts',(-10.9406238230001,15.2,0.292845787999987));
#261157=CARTESIAN_POINT('Ctrl Pts',(-10.9406238230001,11.6,0.292845787999986));
#261158=CARTESIAN_POINT('Ctrl Pts',(-10.9378575430001,15.2,0.291800712999986));
#261159=CARTESIAN_POINT('Ctrl Pts',(-10.9378575430001,11.6,0.291800712999985));
#261160=CARTESIAN_POINT('Ctrl Pts',(-10.9350955160001,15.2,0.290759840999986));
#261161=CARTESIAN_POINT('Ctrl Pts',(-10.9350955160001,11.6,0.290759840999985));
#261162=CARTESIAN_POINT('Ctrl Pts',(-10.9323377520001,15.2,0.289723170999987));
#261163=CARTESIAN_POINT('Ctrl Pts',(-10.9323377520001,11.6,0.289723170999987));
#261164=CARTESIAN_POINT('Ctrl Pts',(-10.9295842640001,15.2,0.288690695999985));
#261165=CARTESIAN_POINT('Ctrl Pts',(-10.9295842640001,11.6,0.288690695999984));
#261166=CARTESIAN_POINT('Ctrl Pts',(-10.9268350640001,15.2,0.287662414999983));
#261167=CARTESIAN_POINT('Ctrl Pts',(-10.9268350640001,11.6,0.287662414999982));
#261168=CARTESIAN_POINT('Ctrl Pts',(-10.9240901640001,15.2,0.286638322999986));
#261169=CARTESIAN_POINT('Ctrl Pts',(-10.9240901640001,11.6,0.286638322999985));
#261170=CARTESIAN_POINT('Ctrl Pts',(-10.9213495760001,15.2,0.285618414999984));
#261171=CARTESIAN_POINT('Ctrl Pts',(-10.9213495760001,11.6,0.285618414999984));
#261172=CARTESIAN_POINT('Ctrl Pts',(-10.9186133120001,15.2,0.284602688999982));
#261173=CARTESIAN_POINT('Ctrl Pts',(-10.9186133120001,11.6,0.284602688999982));
#261174=CARTESIAN_POINT('Ctrl Pts',(-10.9158813840001,15.2,0.283591140999988));
#261175=CARTESIAN_POINT('Ctrl Pts',(-10.9158813840001,11.6,0.283591140999988));
#261176=CARTESIAN_POINT('Ctrl Pts',(-10.9131538030001,15.2,0.282583765999984));
#261177=CARTESIAN_POINT('Ctrl Pts',(-10.9131538030001,11.6,0.282583765999984));
#261178=CARTESIAN_POINT('Ctrl Pts',(-10.9104305830001,15.2,0.281580559999988));
#261179=CARTESIAN_POINT('Ctrl Pts',(-10.9104305830001,11.6,0.281580559999987));
#261180=CARTESIAN_POINT('Ctrl Pts',(-10.9077117350001,15.2,0.280581520999985));
#261181=CARTESIAN_POINT('Ctrl Pts',(-10.9077117350001,11.6,0.280581520999985));
#261182=CARTESIAN_POINT('Ctrl Pts',(-10.9049972710001,15.2,0.279586640999985));
#261183=CARTESIAN_POINT('Ctrl Pts',(-10.9049972710001,11.6,0.279586640999984));
#261184=CARTESIAN_POINT('Ctrl Pts',(-10.9022872040001,15.2,0.278595920999987));
#261185=CARTESIAN_POINT('Ctrl Pts',(-10.9022872040001,11.6,0.278595920999986));
#261186=CARTESIAN_POINT('Ctrl Pts',(-10.8995815450001,15.2,0.277609353999986));
#261187=CARTESIAN_POINT('Ctrl Pts',(-10.8995815450001,11.6,0.277609353999985));
#261188=CARTESIAN_POINT('Ctrl Pts',(-10.8968803070001,15.2,0.276626936999986));
#261189=CARTESIAN_POINT('Ctrl Pts',(-10.8968803070001,11.6,0.276626936999986));
#261190=CARTESIAN_POINT('Ctrl Pts',(-10.8941835000001,15.2,0.275648664999988));
#261191=CARTESIAN_POINT('Ctrl Pts',(-10.8941835000001,11.6,0.275648664999987));
#261192=CARTESIAN_POINT('Ctrl Pts',(-10.8914911410001,15.2,0.274674534999986));
#261193=CARTESIAN_POINT('Ctrl Pts',(-10.8914911410001,11.6,0.274674534999985));
#261194=CARTESIAN_POINT('Ctrl Pts',(-10.8888032380001,15.2,0.273704540999984));
#261195=CARTESIAN_POINT('Ctrl Pts',(-10.8888032380001,11.6,0.273704540999983));
#261196=CARTESIAN_POINT('Ctrl Pts',(-10.8861198050001,15.2,0.272738680999982));
#261197=CARTESIAN_POINT('Ctrl Pts',(-10.8861198050001,11.6,0.272738680999982));
#261198=CARTESIAN_POINT('Ctrl Pts',(-10.8834408550001,15.2,0.271776950999989));
#261199=CARTESIAN_POINT('Ctrl Pts',(-10.8834408550001,11.6,0.271776950999989));
#261200=CARTESIAN_POINT('Ctrl Pts',(-10.8807663990001,15.2,0.270819344999986));
#261201=CARTESIAN_POINT('Ctrl Pts',(-10.8807663990001,11.6,0.270819344999986));
#261202=CARTESIAN_POINT('Ctrl Pts',(-10.8780964490001,15.2,0.269865860999987));
#261203=CARTESIAN_POINT('Ctrl Pts',(-10.8780964490001,11.6,0.269865860999987));
#261204=CARTESIAN_POINT('Ctrl Pts',(-10.8754310200001,15.2,0.268916491999986));
#261205=CARTESIAN_POINT('Ctrl Pts',(-10.8754310200001,11.6,0.268916491999986));
#261206=CARTESIAN_POINT('Ctrl Pts',(-10.8727701220001,15.2,0.267971236999984));
#261207=CARTESIAN_POINT('Ctrl Pts',(-10.8727701220001,11.6,0.267971236999984));
#261208=CARTESIAN_POINT('Ctrl Pts',(-10.8701137680001,15.2,0.267030089999984));
#261209=CARTESIAN_POINT('Ctrl Pts',(-10.8701137680001,11.6,0.267030089999984));
#261210=CARTESIAN_POINT('Ctrl Pts',(-10.8674619700001,15.2,0.266093045999987));
#261211=CARTESIAN_POINT('Ctrl Pts',(-10.8674619700001,11.6,0.266093045999986));
#261212=CARTESIAN_POINT('Ctrl Pts',(-10.8648147410001,15.2,0.265160102999986));
#261213=CARTESIAN_POINT('Ctrl Pts',(-10.8648147410001,11.6,0.265160102999986));
#261214=CARTESIAN_POINT('Ctrl Pts',(-10.8621720950001,15.2,0.264231254999987));
#261215=CARTESIAN_POINT('Ctrl Pts',(-10.8621720950001,11.6,0.264231254999987));
#261216=CARTESIAN_POINT('Ctrl Pts',(-10.8595340430001,15.2,0.263306497999984));
#261217=CARTESIAN_POINT('Ctrl Pts',(-10.8595340430001,11.6,0.263306497999984));
#261218=CARTESIAN_POINT('Ctrl Pts',(-10.8569005980001,15.2,0.262385827999987));
#261219=CARTESIAN_POINT('Ctrl Pts',(-10.8569005980001,11.6,0.262385827999986));
#261220=CARTESIAN_POINT('Ctrl Pts',(-10.8542717720001,15.2,0.261469240999985));
#261221=CARTESIAN_POINT('Ctrl Pts',(-10.8542717720001,11.6,0.261469240999985));
#261222=CARTESIAN_POINT('Ctrl Pts',(-10.8516475780001,15.2,0.260556731999984));
#261223=CARTESIAN_POINT('Ctrl Pts',(-10.8516475780001,11.6,0.260556731999983));
#261224=CARTESIAN_POINT('Ctrl Pts',(-10.8490280300001,15.2,0.259648296999986));
#261225=CARTESIAN_POINT('Ctrl Pts',(-10.8490280300001,11.6,0.259648296999985));
#261226=CARTESIAN_POINT('Ctrl Pts',(-10.8464131390001,15.2,0.258743930999987));
#261227=CARTESIAN_POINT('Ctrl Pts',(-10.8464131390001,11.6,0.258743930999987));
#261228=CARTESIAN_POINT('Ctrl Pts',(-10.8438029180001,15.2,0.257843629999983));
#261229=CARTESIAN_POINT('Ctrl Pts',(-10.8438029180001,11.6,0.257843629999983));
#261230=CARTESIAN_POINT('Ctrl Pts',(-10.8411973810001,15.2,0.256947389999986));
#261231=CARTESIAN_POINT('Ctrl Pts',(-10.8411973810001,11.6,0.256947389999986));
#261232=CARTESIAN_POINT('Ctrl Pts',(-10.8385965390001,15.2,0.256055205999988));
#261233=CARTESIAN_POINT('Ctrl Pts',(-10.8385965390001,11.6,0.256055205999987));
#261234=CARTESIAN_POINT('Ctrl Pts',(-10.8360004070001,15.2,0.255167072999987));
#261235=CARTESIAN_POINT('Ctrl Pts',(-10.8360004070001,11.6,0.255167072999986));
#261236=CARTESIAN_POINT('Ctrl Pts',(-10.8334089940001,15.2,0.254282987999983));
#261237=CARTESIAN_POINT('Ctrl Pts',(-10.8334089940001,11.6,0.254282987999983));
#261238=CARTESIAN_POINT('Ctrl Pts',(-10.8308223180001,15.2,0.253402943999985));
#261239=CARTESIAN_POINT('Ctrl Pts',(-10.8308223180001,11.6,0.253402943999985));
#261240=CARTESIAN_POINT('Ctrl Pts',(-10.8282403890001,15.2,0.252526939999989));
#261241=CARTESIAN_POINT('Ctrl Pts',(-10.8282403890001,11.6,0.252526939999988));
#261242=CARTESIAN_POINT('Ctrl Pts',(-10.8256632200001,15.2,0.251654968999984));
#261243=CARTESIAN_POINT('Ctrl Pts',(-10.8256632200001,11.6,0.251654968999983));
#261244=CARTESIAN_POINT('Ctrl Pts',(-10.8230908230001,15.2,0.250787025999983));
#261245=CARTESIAN_POINT('Ctrl Pts',(-10.8230908230001,11.6,0.250787025999983));
#261246=CARTESIAN_POINT('Ctrl Pts',(-10.8205232130001,15.2,0.249923108999983));
#261247=CARTESIAN_POINT('Ctrl Pts',(-10.8205232130001,11.6,0.249923108999983));
#261248=CARTESIAN_POINT('Ctrl Pts',(-10.8179604030001,15.2,0.249063209999987));
#261249=CARTESIAN_POINT('Ctrl Pts',(-10.8179604030001,11.6,0.249063209999986));
#261250=CARTESIAN_POINT('Ctrl Pts',(-10.8154024050001,15.2,0.248207326999985));
#261251=CARTESIAN_POINT('Ctrl Pts',(-10.8154024050001,11.6,0.248207326999985));
#261252=CARTESIAN_POINT('Ctrl Pts',(-10.8128492330001,15.2,0.247355453999987));
#261253=CARTESIAN_POINT('Ctrl Pts',(-10.8128492330001,11.6,0.247355453999986));
#261254=CARTESIAN_POINT('Ctrl Pts',(-10.8103008990001,15.2,0.246507586999982));
#261255=CARTESIAN_POINT('Ctrl Pts',(-10.8103008990001,11.6,0.246507586999982));
#261256=CARTESIAN_POINT('Ctrl Pts',(-10.8077574170001,15.2,0.245663720999989));
#261257=CARTESIAN_POINT('Ctrl Pts',(-10.8077574170001,11.6,0.245663720999989));
#261258=CARTESIAN_POINT('Ctrl Pts',(-10.8052187990001,15.2,0.244823850999989));
#261259=CARTESIAN_POINT('Ctrl Pts',(-10.8052187990001,11.6,0.244823850999988));
#261260=CARTESIAN_POINT('Ctrl Pts',(-10.8026850610001,15.2,0.243987971999986));
#261261=CARTESIAN_POINT('Ctrl Pts',(-10.8026850610001,11.6,0.243987971999986));
#261262=CARTESIAN_POINT('Ctrl Pts',(-10.8001562130001,15.2,0.243156080999984));
#261263=CARTESIAN_POINT('Ctrl Pts',(-10.8001562130001,11.6,0.243156080999984));
#261264=CARTESIAN_POINT('Ctrl Pts',(-10.7976322700001,15.2,0.242328170999984));
#261265=CARTESIAN_POINT('Ctrl Pts',(-10.7976322700001,11.6,0.242328170999983));
#261266=CARTESIAN_POINT('Ctrl Pts',(-10.7951132440001,15.2,0.241504237999983));
#261267=CARTESIAN_POINT('Ctrl Pts',(-10.7951132440001,11.6,0.241504237999983));
#261268=CARTESIAN_POINT('Ctrl Pts',(-10.7925991510001,15.2,0.240684276999983));
#261269=CARTESIAN_POINT('Ctrl Pts',(-10.7925991510001,11.6,0.240684276999982));
#261270=CARTESIAN_POINT('Ctrl Pts',(-10.7900900010001,15.2,0.239868283999982));
#261271=CARTESIAN_POINT('Ctrl Pts',(-10.7900900010001,11.6,0.239868283999982));
#261272=CARTESIAN_POINT('Ctrl Pts',(-10.7875858100001,15.2,0.239056253999985));
#261273=CARTESIAN_POINT('Ctrl Pts',(-10.7875858100001,11.6,0.239056253999985));
#261274=CARTESIAN_POINT('Ctrl Pts',(-10.7850865910001,15.2,0.238248179999987));
#261275=CARTESIAN_POINT('Ctrl Pts',(-10.7850865910001,11.6,0.238248179999986));
#261276=CARTESIAN_POINT('Ctrl Pts',(-10.7825923560001,15.2,0.237444060999987));
#261277=CARTESIAN_POINT('Ctrl Pts',(-10.7825923560001,11.6,0.237444060999987));
#261278=CARTESIAN_POINT('Ctrl Pts',(-10.7801031190001,15.2,0.236643886999985));
#261279=CARTESIAN_POINT('Ctrl Pts',(-10.7801031190001,11.6,0.236643886999985));
#261280=CARTESIAN_POINT('Ctrl Pts',(-10.7776188950001,15.2,0.235847656999986));
#261281=CARTESIAN_POINT('Ctrl Pts',(-10.7776188950001,11.6,0.235847656999985));
#261282=CARTESIAN_POINT('Ctrl Pts',(-10.7751396960001,15.2,0.235055364999983));
#261283=CARTESIAN_POINT('Ctrl Pts',(-10.7751396960001,11.6,0.235055364999983));
#261284=CARTESIAN_POINT('Ctrl Pts',(-10.7726655360001,15.2,0.234267004999986));
#261285=CARTESIAN_POINT('Ctrl Pts',(-10.7726655360001,11.6,0.234267004999986));
#261286=CARTESIAN_POINT('Ctrl Pts',(-10.7701964290001,15.2,0.233482572999986));
#261287=CARTESIAN_POINT('Ctrl Pts',(-10.7701964290001,11.6,0.233482572999985));
#261288=CARTESIAN_POINT('Ctrl Pts',(-10.7677323890001,15.2,0.232702063999985));
#261289=CARTESIAN_POINT('Ctrl Pts',(-10.7677323890001,11.6,0.232702063999985));
#261290=CARTESIAN_POINT('Ctrl Pts',(-10.7652734280001,15.2,0.231925471999985));
#261291=CARTESIAN_POINT('Ctrl Pts',(-10.7652734280001,11.6,0.231925471999985));
#261292=CARTESIAN_POINT('Ctrl Pts',(-10.7628195610001,15.2,0.231152792999989));
#261293=CARTESIAN_POINT('Ctrl Pts',(-10.7628195610001,11.6,0.231152792999989));
#261294=CARTESIAN_POINT('Ctrl Pts',(-10.7603708020001,15.2,0.230384019999987));
#261295=CARTESIAN_POINT('Ctrl Pts',(-10.7603708020001,11.6,0.230384019999987));
#261296=CARTESIAN_POINT('Ctrl Pts',(-10.7579271630001,15.2,0.229619148999984));
#261297=CARTESIAN_POINT('Ctrl Pts',(-10.7579271630001,11.6,0.229619148999984));
#261298=CARTESIAN_POINT('Ctrl Pts',(-10.7554886610001,15.2,0.228858175999989));
#261299=CARTESIAN_POINT('Ctrl Pts',(-10.7554886610001,11.6,0.228858175999988));
#261300=CARTESIAN_POINT('Ctrl Pts',(-10.7530553070001,15.2,0.228101093999986));
#261301=CARTESIAN_POINT('Ctrl Pts',(-10.7530553070001,11.6,0.228101093999986));
#261302=CARTESIAN_POINT('Ctrl Pts',(-10.7506271160001,15.2,0.227347897999985));
#261303=CARTESIAN_POINT('Ctrl Pts',(-10.7506271160001,11.6,0.227347897999985));
#261304=CARTESIAN_POINT('Ctrl Pts',(-10.7482041010001,15.2,0.226598583999986));
#261305=CARTESIAN_POINT('Ctrl Pts',(-10.7482041010001,11.6,0.226598583999986));
#261306=CARTESIAN_POINT('Ctrl Pts',(-10.7457862770001,15.2,0.225853145999988));
#261307=CARTESIAN_POINT('Ctrl Pts',(-10.7457862770001,11.6,0.225853145999988));
#261308=CARTESIAN_POINT('Ctrl Pts',(-10.7433736600001,15.2,0.225111577999986));
#261309=CARTESIAN_POINT('Ctrl Pts',(-10.7433736600001,11.6,0.225111577999985));
#261310=CARTESIAN_POINT('Ctrl Pts',(-10.7409662590001,15.2,0.224373874999984));
#261311=CARTESIAN_POINT('Ctrl Pts',(-10.7409662590001,11.6,0.224373874999983));
#261312=CARTESIAN_POINT('Ctrl Pts',(-10.7385640920001,15.2,0.223640032999985));
#261313=CARTESIAN_POINT('Ctrl Pts',(-10.7385640920001,11.6,0.223640032999985));
#261314=CARTESIAN_POINT('Ctrl Pts',(-10.7361671710001,15.2,0.222910043999986));
#261315=CARTESIAN_POINT('Ctrl Pts',(-10.7361671710001,11.6,0.222910043999986));
#261316=CARTESIAN_POINT('Ctrl Pts',(-10.7337755120001,15.2,0.222183903999986));
#261317=CARTESIAN_POINT('Ctrl Pts',(-10.7337755120001,11.6,0.222183903999986));
#261318=CARTESIAN_POINT('Ctrl Pts',(-10.7313891280001,15.2,0.221461608999984));
#261319=CARTESIAN_POINT('Ctrl Pts',(-10.7313891280001,11.6,0.221461608999984));
#261320=CARTESIAN_POINT('Ctrl Pts',(-10.7290080330001,15.2,0.220743150999985));
#261321=CARTESIAN_POINT('Ctrl Pts',(-10.7290080330001,11.6,0.220743150999984));
#261322=CARTESIAN_POINT('Ctrl Pts',(-10.7266322420001,15.2,0.220028526999982));
#261323=CARTESIAN_POINT('Ctrl Pts',(-10.7266322420001,11.6,0.220028526999982));
#261324=CARTESIAN_POINT('Ctrl Pts',(-10.7242617690001,15.2,0.219317729999986));
#261325=CARTESIAN_POINT('Ctrl Pts',(-10.7242617690001,11.6,0.219317729999986));
#261326=CARTESIAN_POINT('Ctrl Pts',(-10.7218966280001,15.2,0.218610753999986));
#261327=CARTESIAN_POINT('Ctrl Pts',(-10.7218966280001,11.6,0.218610753999986));
#261328=CARTESIAN_POINT('Ctrl Pts',(-10.7195368330001,15.2,0.217907592999986));
#261329=CARTESIAN_POINT('Ctrl Pts',(-10.7195368330001,11.6,0.217907592999986));
#261330=CARTESIAN_POINT('Ctrl Pts',(-10.7171823990001,15.2,0.217208243999987));
#261331=CARTESIAN_POINT('Ctrl Pts',(-10.7171823990001,11.6,0.217208243999986));
#261332=CARTESIAN_POINT('Ctrl Pts',(-10.7148333410001,15.2,0.216512699999987));
#261333=CARTESIAN_POINT('Ctrl Pts',(-10.7148333410001,11.6,0.216512699999986));
#261334=CARTESIAN_POINT('Ctrl Pts',(-10.7124896730001,15.2,0.215820953999986));
#261335=CARTESIAN_POINT('Ctrl Pts',(-10.7124896730001,11.6,0.215820953999985));
#261336=CARTESIAN_POINT('Ctrl Pts',(-10.7101514080001,15.2,0.215133002999988));
#261337=CARTESIAN_POINT('Ctrl Pts',(-10.7101514080001,11.6,0.215133002999987));
#261338=CARTESIAN_POINT('Ctrl Pts',(-10.7078185620001,15.2,0.214448838999988));
#261339=CARTESIAN_POINT('Ctrl Pts',(-10.7078185620001,11.6,0.214448838999987));
#261340=CARTESIAN_POINT('Ctrl Pts',(-10.7054911500001,15.2,0.213768457999985));
#261341=CARTESIAN_POINT('Ctrl Pts',(-10.7054911500001,11.6,0.213768457999985));
#261342=CARTESIAN_POINT('Ctrl Pts',(-10.7031691860001,15.2,0.213091852999985));
#261343=CARTESIAN_POINT('Ctrl Pts',(-10.7031691860001,11.6,0.213091852999984));
#261344=CARTESIAN_POINT('Ctrl Pts',(-10.7008526850001,15.2,0.212419018999985));
#261345=CARTESIAN_POINT('Ctrl Pts',(-10.7008526850001,11.6,0.212419018999985));
#261346=CARTESIAN_POINT('Ctrl Pts',(-10.6985416600001,15.2,0.211749948999986));
#261347=CARTESIAN_POINT('Ctrl Pts',(-10.6985416600001,11.6,0.211749948999986));
#261348=CARTESIAN_POINT('Ctrl Pts',(-10.6962361280001,15.2,0.211084637999988));
#261349=CARTESIAN_POINT('Ctrl Pts',(-10.6962361280001,11.6,0.211084637999987));
#261350=CARTESIAN_POINT('Ctrl Pts',(-10.6939361020001,15.2,0.210423081999984));
#261351=CARTESIAN_POINT('Ctrl Pts',(-10.6939361020001,11.6,0.210423081999984));
#261352=CARTESIAN_POINT('Ctrl Pts',(-10.6916415980001,15.2,0.209765271999984));
#261353=CARTESIAN_POINT('Ctrl Pts',(-10.6916415980001,11.6,0.209765271999984));
#261354=CARTESIAN_POINT('Ctrl Pts',(-10.6893526300001,15.2,0.209111201999987));
#261355=CARTESIAN_POINT('Ctrl Pts',(-10.6893526300001,11.6,0.209111201999987));
#261356=CARTESIAN_POINT('Ctrl Pts',(-10.6870692130001,15.2,0.208460869999989));
#261357=CARTESIAN_POINT('Ctrl Pts',(-10.6870692130001,11.6,0.208460869999989));
#261358=CARTESIAN_POINT('Ctrl Pts',(-10.6847913630001,15.2,0.207814266999984));
#261359=CARTESIAN_POINT('Ctrl Pts',(-10.6847913630001,11.6,0.207814266999983));
#261360=CARTESIAN_POINT('Ctrl Pts',(-10.6825190920001,15.2,0.207171386999985));
#261361=CARTESIAN_POINT('Ctrl Pts',(-10.6825190920001,11.6,0.207171386999984));
#261362=CARTESIAN_POINT('Ctrl Pts',(-10.6802524190001,15.2,0.206532224999982));
#261363=CARTESIAN_POINT('Ctrl Pts',(-10.6802524190001,11.6,0.206532224999982));
#261364=CARTESIAN_POINT('Ctrl Pts',(-10.6779913570001,15.2,0.205896773999985));
#261365=CARTESIAN_POINT('Ctrl Pts',(-10.6779913570001,11.6,0.205896773999985));
#261366=CARTESIAN_POINT('Ctrl Pts',(-10.6757359200001,15.2,0.205265028999988));
#261367=CARTESIAN_POINT('Ctrl Pts',(-10.6757359200001,11.6,0.205265028999988));
#261368=CARTESIAN_POINT('Ctrl Pts',(-10.6734861240001,15.2,0.204636982999986));
#261369=CARTESIAN_POINT('Ctrl Pts',(-10.6734861240001,11.6,0.204636982999986));
#261370=CARTESIAN_POINT('Ctrl Pts',(-10.6712419860001,15.2,0.204012629999983));
#261371=CARTESIAN_POINT('Ctrl Pts',(-10.6712419860001,11.6,0.204012629999983));
#261372=CARTESIAN_POINT('Ctrl Pts',(-10.6690035190001,15.2,0.203391963999984));
#261373=CARTESIAN_POINT('Ctrl Pts',(-10.6690035190001,11.6,0.203391963999983));
#261374=CARTESIAN_POINT('Ctrl Pts',(-10.6667707370001,15.2,0.202774979999987));
#261375=CARTESIAN_POINT('Ctrl Pts',(-10.6667707370001,11.6,0.202774979999986));
#261376=CARTESIAN_POINT('Ctrl Pts',(-10.6645436590001,15.2,0.202161669999987));
#261377=CARTESIAN_POINT('Ctrl Pts',(-10.6645436590001,11.6,0.202161669999987));
#261378=CARTESIAN_POINT('Ctrl Pts',(-10.6623222980001,15.2,0.201552028999985));
#261379=CARTESIAN_POINT('Ctrl Pts',(-10.6623222980001,11.6,0.201552028999985));
#261380=CARTESIAN_POINT('Ctrl Pts',(-10.6601066700001,15.2,0.200946048999988));
#261381=CARTESIAN_POINT('Ctrl Pts',(-10.6601066700001,11.6,0.200946048999988));
#261382=CARTESIAN_POINT('Ctrl Pts',(-10.6578967890001,15.2,0.200343724999983));
#261383=CARTESIAN_POINT('Ctrl Pts',(-10.6578967890001,11.6,0.200343724999982));
#261384=CARTESIAN_POINT('Ctrl Pts',(-10.6556926720001,15.2,0.199745050999987));
#261385=CARTESIAN_POINT('Ctrl Pts',(-10.6556926720001,11.6,0.199745050999986));
#261386=CARTESIAN_POINT('Ctrl Pts',(-10.6534943330001,15.2,0.199150019999985));
#261387=CARTESIAN_POINT('Ctrl Pts',(-10.6534943330001,11.6,0.199150019999985));
#261388=CARTESIAN_POINT('Ctrl Pts',(-10.6513017900001,15.2,0.198558625999983));
#261389=CARTESIAN_POINT('Ctrl Pts',(-10.6513017900001,11.6,0.198558625999982));
#261390=CARTESIAN_POINT('Ctrl Pts',(-10.6491150560001,15.2,0.197970862999988));
#261391=CARTESIAN_POINT('Ctrl Pts',(-10.6491150560001,11.6,0.197970862999987));
#261392=CARTESIAN_POINT('Ctrl Pts',(-10.6469341480001,15.2,0.197386722999986));
#261393=CARTESIAN_POINT('Ctrl Pts',(-10.6469341480001,11.6,0.197386722999985));
#261394=CARTESIAN_POINT('Ctrl Pts',(-10.6447590820001,15.2,0.196806200999986));
#261395=CARTESIAN_POINT('Ctrl Pts',(-10.6447590820001,11.6,0.196806200999986));
#261396=CARTESIAN_POINT('Ctrl Pts',(-10.6425898720001,15.2,0.196229288999987));
#261397=CARTESIAN_POINT('Ctrl Pts',(-10.6425898720001,11.6,0.196229288999987));
#261398=CARTESIAN_POINT('Ctrl Pts',(-10.6404265340001,15.2,0.195655982999985));
#261399=CARTESIAN_POINT('Ctrl Pts',(-10.6404265340001,11.6,0.195655982999984));
#261400=CARTESIAN_POINT('Ctrl Pts',(-10.6382690860001,15.2,0.195086272999987));
#261401=CARTESIAN_POINT('Ctrl Pts',(-10.6382690860001,11.6,0.195086272999986));
#261402=CARTESIAN_POINT('Ctrl Pts',(-10.6361175410001,15.2,0.194520154999989));
#261403=CARTESIAN_POINT('Ctrl Pts',(-10.6361175410001,11.6,0.194520154999988));
#261404=CARTESIAN_POINT('Ctrl Pts',(-10.6339719170001,15.2,0.193957621999985));
#261405=CARTESIAN_POINT('Ctrl Pts',(-10.6339719170001,11.6,0.193957621999985));
#261406=CARTESIAN_POINT('Ctrl Pts',(-10.6318322290001,15.2,0.193398666999984));
#261407=CARTESIAN_POINT('Ctrl Pts',(-10.6318322290001,11.6,0.193398666999984));
#261408=CARTESIAN_POINT('Ctrl Pts',(-10.6296984920001,15.2,0.192843283999986));
#261409=CARTESIAN_POINT('Ctrl Pts',(-10.6296984920001,11.6,0.192843283999986));
#261410=CARTESIAN_POINT('Ctrl Pts',(-10.6275707240001,15.2,0.192291463999985));
#261411=CARTESIAN_POINT('Ctrl Pts',(-10.6275707240001,11.6,0.192291463999985));
#261412=CARTESIAN_POINT('Ctrl Pts',(-10.6254489400001,15.2,0.191743201999985));
#261413=CARTESIAN_POINT('Ctrl Pts',(-10.6254489400001,11.6,0.191743201999985));
#261414=CARTESIAN_POINT('Ctrl Pts',(-10.6233331560001,15.2,0.191198491999987));
#261415=CARTESIAN_POINT('Ctrl Pts',(-10.6233331560001,11.6,0.191198491999986));
#261416=CARTESIAN_POINT('Ctrl Pts',(-10.6212233880001,15.2,0.190657325999983));
#261417=CARTESIAN_POINT('Ctrl Pts',(-10.6212233880001,11.6,0.190657325999983));
#261418=CARTESIAN_POINT('Ctrl Pts',(-10.6191196530001,15.2,0.190119695999984));
#261419=CARTESIAN_POINT('Ctrl Pts',(-10.6191196530001,11.6,0.190119695999984));
#261420=CARTESIAN_POINT('Ctrl Pts',(-10.6170219660001,15.2,0.189585598999984));
#261421=CARTESIAN_POINT('Ctrl Pts',(-10.6170219660001,11.6,0.189585598999984));
#261422=CARTESIAN_POINT('Ctrl Pts',(-10.6149303440001,15.2,0.189055023999987));
#261423=CARTESIAN_POINT('Ctrl Pts',(-10.6149303440001,11.6,0.189055023999986));
#261424=CARTESIAN_POINT('Ctrl Pts',(-10.6128448030001,15.2,0.188527964999987));
#261425=CARTESIAN_POINT('Ctrl Pts',(-10.6128448030001,11.6,0.188527964999987));
#261426=CARTESIAN_POINT('Ctrl Pts',(-10.6107653600001,15.2,0.188004416999985));
#261427=CARTESIAN_POINT('Ctrl Pts',(-10.6107653600001,11.6,0.188004416999985));
#261428=CARTESIAN_POINT('Ctrl Pts',(-10.6086920310001,15.2,0.187484370999984));
#261429=CARTESIAN_POINT('Ctrl Pts',(-10.6086920310001,11.6,0.187484370999984));
#261430=CARTESIAN_POINT('Ctrl Pts',(-10.6066248330001,15.2,0.186967819999988));
#261431=CARTESIAN_POINT('Ctrl Pts',(-10.6066248330001,11.6,0.186967819999988));
#261432=CARTESIAN_POINT('Ctrl Pts',(-10.6045637800001,15.2,0.186454757999983));
#261433=CARTESIAN_POINT('Ctrl Pts',(-10.6045637800001,11.6,0.186454757999983));
#261434=CARTESIAN_POINT('Ctrl Pts',(-10.6025088930001,15.2,0.185945177999987));
#261435=CARTESIAN_POINT('Ctrl Pts',(-10.6025088930001,11.6,0.185945177999986));
#261436=CARTESIAN_POINT('Ctrl Pts',(-10.6004601840001,15.2,0.185439070999984));
#261437=CARTESIAN_POINT('Ctrl Pts',(-10.6004601840001,11.6,0.185439070999984));
#261438=CARTESIAN_POINT('Ctrl Pts',(-10.5984176730001,15.2,0.184936432999985));
#261439=CARTESIAN_POINT('Ctrl Pts',(-10.5984176730001,11.6,0.184936432999984));
#261440=CARTESIAN_POINT('Ctrl Pts',(-10.5963813760001,15.2,0.184437252999987));
#261441=CARTESIAN_POINT('Ctrl Pts',(-10.5963813760001,11.6,0.184437252999987));
#261442=CARTESIAN_POINT('Ctrl Pts',(-10.5943513080001,15.2,0.183941525999987));
#261443=CARTESIAN_POINT('Ctrl Pts',(-10.5943513080001,11.6,0.183941525999986));
#261444=CARTESIAN_POINT('Ctrl Pts',(-10.5923274870001,15.2,0.183449243999987));
#261445=CARTESIAN_POINT('Ctrl Pts',(-10.5923274870001,11.6,0.183449243999986));
#261446=CARTESIAN_POINT('Ctrl Pts',(-10.5903099300001,15.2,0.182960399999987));
#261447=CARTESIAN_POINT('Ctrl Pts',(-10.5903099300001,11.6,0.182960399999987));
#261448=CARTESIAN_POINT('Ctrl Pts',(-10.5882986550001,15.2,0.182474987999988));
#261449=CARTESIAN_POINT('Ctrl Pts',(-10.5882986550001,11.6,0.182474987999987));
#261450=CARTESIAN_POINT('Ctrl Pts',(-10.5862936760001,15.2,0.181992998999987));
#261451=CARTESIAN_POINT('Ctrl Pts',(-10.5862936760001,11.6,0.181992998999986));
#261452=CARTESIAN_POINT('Ctrl Pts',(-10.5842950130001,15.2,0.181514424999989));
#261453=CARTESIAN_POINT('Ctrl Pts',(-10.5842950130001,11.6,0.181514424999988));
#261454=CARTESIAN_POINT('Ctrl Pts',(-10.5823026810001,15.2,0.181039259999984));
#261455=CARTESIAN_POINT('Ctrl Pts',(-10.5823026810001,11.6,0.181039259999984));
#261456=CARTESIAN_POINT('Ctrl Pts',(-10.5803166980001,15.2,0.180567494999986));
#261457=CARTESIAN_POINT('Ctrl Pts',(-10.5803166980001,11.6,0.180567494999985));
#261458=CARTESIAN_POINT('Ctrl Pts',(-10.5783370810001,15.2,0.180099124999984));
#261459=CARTESIAN_POINT('Ctrl Pts',(-10.5783370810001,11.6,0.180099124999983));
#261460=CARTESIAN_POINT('Ctrl Pts',(-10.5763638480001,15.2,0.179634139999987));
#261461=CARTESIAN_POINT('Ctrl Pts',(-10.5763638480001,11.6,0.179634139999986));
#261462=CARTESIAN_POINT('Ctrl Pts',(-10.5743970150001,15.2,0.179172532999985));
#261463=CARTESIAN_POINT('Ctrl Pts',(-10.5743970150001,11.6,0.179172532999984));
#261464=CARTESIAN_POINT('Ctrl Pts',(-10.5724365990001,15.2,0.178714295999987));
#261465=CARTESIAN_POINT('Ctrl Pts',(-10.5724365990001,11.6,0.178714295999986));
#261466=CARTESIAN_POINT('Ctrl Pts',(-10.5704826190001,15.2,0.178259422999982));
#261467=CARTESIAN_POINT('Ctrl Pts',(-10.5704826190001,11.6,0.178259422999982));
#261468=CARTESIAN_POINT('Ctrl Pts',(-10.5685350920001,15.2,0.177807903999985));
#261469=CARTESIAN_POINT('Ctrl Pts',(-10.5685350920001,11.6,0.177807903999984));
#261470=CARTESIAN_POINT('Ctrl Pts',(-10.5665940340001,15.2,0.177359733999989));
#261471=CARTESIAN_POINT('Ctrl Pts',(-10.5665940340001,11.6,0.177359733999988));
#261472=CARTESIAN_POINT('Ctrl Pts',(-10.5646594650001,15.2,0.176914901999985));
#261473=CARTESIAN_POINT('Ctrl Pts',(-10.5646594650001,11.6,0.176914901999984));
#261474=CARTESIAN_POINT('Ctrl Pts',(-10.5627314000001,15.2,0.176473403999986));
#261475=CARTESIAN_POINT('Ctrl Pts',(-10.5627314000001,11.6,0.176473403999986));
#261476=CARTESIAN_POINT('Ctrl Pts',(-10.5608098580001,15.2,0.176035227999982));
#261477=CARTESIAN_POINT('Ctrl Pts',(-10.5608098580001,11.6,0.176035227999982));
#261478=CARTESIAN_POINT('Ctrl Pts',(-10.5588948570001,15.2,0.175600368999986));
#261479=CARTESIAN_POINT('Ctrl Pts',(-10.5588948570001,11.6,0.175600368999986));
#261480=CARTESIAN_POINT('Ctrl Pts',(-10.5569864130001,15.2,0.175168818999989));
#261481=CARTESIAN_POINT('Ctrl Pts',(-10.5569864130001,11.6,0.175168818999988));
#261482=CARTESIAN_POINT('Ctrl Pts',(-10.5550845460001,15.2,0.174740567999985));
#261483=CARTESIAN_POINT('Ctrl Pts',(-10.5550845460001,11.6,0.174740567999984));
#261484=CARTESIAN_POINT('Ctrl Pts',(-10.5531892730001,15.2,0.174315608999986));
#261485=CARTESIAN_POINT('Ctrl Pts',(-10.5531892730001,11.6,0.174315608999986));
#261486=CARTESIAN_POINT('Ctrl Pts',(-10.5513006120001,15.2,0.173893933999985));
#261487=CARTESIAN_POINT('Ctrl Pts',(-10.5513006120001,11.6,0.173893933999984));
#261488=CARTESIAN_POINT('Ctrl Pts',(-10.5494185790001,15.2,0.173475535999987));
#261489=CARTESIAN_POINT('Ctrl Pts',(-10.5494185790001,11.6,0.173475535999987));
#261490=CARTESIAN_POINT('Ctrl Pts',(-10.5475431950001,15.2,0.173060405999985));
#261491=CARTESIAN_POINT('Ctrl Pts',(-10.5475431950001,11.6,0.173060405999985));
#261492=CARTESIAN_POINT('Ctrl Pts',(-10.5456744770001,15.2,0.172648534999986));
#261493=CARTESIAN_POINT('Ctrl Pts',(-10.5456744770001,11.6,0.172648534999986));
#261494=CARTESIAN_POINT('Ctrl Pts',(-10.5438124430001,15.2,0.172239915999985));
#261495=CARTESIAN_POINT('Ctrl Pts',(-10.5438124430001,11.6,0.172239915999985));
#261496=CARTESIAN_POINT('Ctrl Pts',(-10.5419571120001,15.2,0.171834540999987));
#261497=CARTESIAN_POINT('Ctrl Pts',(-10.5419571120001,11.6,0.171834540999986));
#261498=CARTESIAN_POINT('Ctrl Pts',(-10.5401085000001,15.2,0.171432399999984));
#261499=CARTESIAN_POINT('Ctrl Pts',(-10.5401085000001,11.6,0.171432399999984));
#261500=CARTESIAN_POINT('Ctrl Pts',(-10.5382666270001,15.2,0.171033485999987));
#261501=CARTESIAN_POINT('Ctrl Pts',(-10.5382666270001,11.6,0.171033485999987));
#261502=CARTESIAN_POINT('Ctrl Pts',(-10.5364315110001,15.2,0.170637790999986));
#261503=CARTESIAN_POINT('Ctrl Pts',(-10.5364315110001,11.6,0.170637790999985));
#261504=CARTESIAN_POINT('Ctrl Pts',(-10.5346031720001,15.2,0.170245304999987));
#261505=CARTESIAN_POINT('Ctrl Pts',(-10.5346031720001,11.6,0.170245304999987));
#261506=CARTESIAN_POINT('Ctrl Pts',(-10.5327816250001,15.2,0.169856020999983));
#261507=CARTESIAN_POINT('Ctrl Pts',(-10.5327816250001,11.6,0.169856020999983));
#261508=CARTESIAN_POINT('Ctrl Pts',(-10.5309668930001,15.2,0.169469929999986));
#261509=CARTESIAN_POINT('Ctrl Pts',(-10.5309668930001,11.6,0.169469929999985));
#261510=CARTESIAN_POINT('Ctrl Pts',(-10.5291589900001,15.2,0.169087022999985));
#261511=CARTESIAN_POINT('Ctrl Pts',(-10.5291589900001,11.6,0.169087022999985));
#261512=CARTESIAN_POINT('Ctrl Pts',(-10.5273579390001,15.2,0.168707291999985));
#261513=CARTESIAN_POINT('Ctrl Pts',(-10.5273579390001,11.6,0.168707291999985));
#261514=CARTESIAN_POINT('Ctrl Pts',(-10.5255637550001,15.2,0.168330728999986));
#261515=CARTESIAN_POINT('Ctrl Pts',(-10.5255637550001,11.6,0.168330728999985));
#261516=CARTESIAN_POINT('Ctrl Pts',(-10.5237764590001,15.2,0.167957323999985));
#261517=CARTESIAN_POINT('Ctrl Pts',(-10.5237764590001,11.6,0.167957323999985));
#261518=CARTESIAN_POINT('Ctrl Pts',(-10.5219960680001,15.2,0.167587068999988));
#261519=CARTESIAN_POINT('Ctrl Pts',(-10.5219960680001,11.6,0.167587068999988));
#261520=CARTESIAN_POINT('Ctrl Pts',(-10.5202226040001,15.2,0.167219955999984));
#261521=CARTESIAN_POINT('Ctrl Pts',(-10.5202226040001,11.6,0.167219955999984));
#261522=CARTESIAN_POINT('Ctrl Pts',(-10.5184560840001,15.2,0.166855974999987));
#261523=CARTESIAN_POINT('Ctrl Pts',(-10.5184560840001,11.6,0.166855974999986));
#261524=CARTESIAN_POINT('Ctrl Pts',(-10.5166965270001,15.2,0.166495116999985));
#261525=CARTESIAN_POINT('Ctrl Pts',(-10.5166965270001,11.6,0.166495116999985));
#261526=CARTESIAN_POINT('Ctrl Pts',(-10.5149439520001,15.2,0.166137374999984));
#261527=CARTESIAN_POINT('Ctrl Pts',(-10.5149439520001,11.6,0.166137374999983));
#261528=CARTESIAN_POINT('Ctrl Pts',(-10.5131983790001,15.2,0.165782736999986));
#261529=CARTESIAN_POINT('Ctrl Pts',(-10.5131983790001,11.6,0.165782736999986));
#261530=CARTESIAN_POINT('Ctrl Pts',(-10.5114598270001,15.2,0.165431196999983));
#261531=CARTESIAN_POINT('Ctrl Pts',(-10.5114598270001,11.6,0.165431196999983));
#261532=CARTESIAN_POINT('Ctrl Pts',(-10.5097283150001,15.2,0.165082744999987));
#261533=CARTESIAN_POINT('Ctrl Pts',(-10.5097283150001,11.6,0.165082744999987));
#261534=CARTESIAN_POINT('Ctrl Pts',(-10.5080038620001,15.2,0.164737371999983));
#261535=CARTESIAN_POINT('Ctrl Pts',(-10.5080038620001,11.6,0.164737371999983));
#261536=CARTESIAN_POINT('Ctrl Pts',(-10.5062864880001,15.2,0.164395067999985));
#261537=CARTESIAN_POINT('Ctrl Pts',(-10.5062864880001,11.6,0.164395067999985));
#261538=CARTESIAN_POINT('Ctrl Pts',(-10.5045762130001,15.2,0.164055823999987));
#261539=CARTESIAN_POINT('Ctrl Pts',(-10.5045762130001,11.6,0.164055823999986));
#261540=CARTESIAN_POINT('Ctrl Pts',(-10.5028730550001,15.2,0.163719632999988));
#261541=CARTESIAN_POINT('Ctrl Pts',(-10.5028730550001,11.6,0.163719632999987));
#261542=CARTESIAN_POINT('Ctrl Pts',(-10.5011770350001,15.2,0.163386482999983));
#261543=CARTESIAN_POINT('Ctrl Pts',(-10.5011770350001,11.6,0.163386482999983));
#261544=CARTESIAN_POINT('Ctrl Pts',(-10.4994881720001,15.2,0.163056365999985));
#261545=CARTESIAN_POINT('Ctrl Pts',(-10.4994881720001,11.6,0.163056365999985));
#261546=CARTESIAN_POINT('Ctrl Pts',(-10.4978064870001,15.2,0.162729272999984));
#261547=CARTESIAN_POINT('Ctrl Pts',(-10.4978064870001,11.6,0.162729272999984));
#261548=CARTESIAN_POINT('Ctrl Pts',(-10.4961320000001,15.2,0.162405193999984));
#261549=CARTESIAN_POINT('Ctrl Pts',(-10.4961320000001,11.6,0.162405193999983));
#261550=CARTESIAN_POINT('Ctrl Pts',(-10.4944647280001,15.2,0.162084120999988));
#261551=CARTESIAN_POINT('Ctrl Pts',(-10.4944647280001,11.6,0.162084120999987));
#261552=CARTESIAN_POINT('Ctrl Pts',(-10.4928046930001,15.2,0.161766040999982));
#261553=CARTESIAN_POINT('Ctrl Pts',(-10.4928046930001,11.6,0.161766040999982));
#261554=CARTESIAN_POINT('Ctrl Pts',(-10.4911519150001,15.2,0.161450947999988));
#261555=CARTESIAN_POINT('Ctrl Pts',(-10.4911519150001,11.6,0.161450947999988));
#261556=CARTESIAN_POINT('Ctrl Pts',(-10.4895064150001,15.2,0.161138831999987));
#261557=CARTESIAN_POINT('Ctrl Pts',(-10.4895064150001,11.6,0.161138831999987));
#261558=CARTESIAN_POINT('Ctrl Pts',(-10.4878682100001,15.2,0.160829682999988));
#261559=CARTESIAN_POINT('Ctrl Pts',(-10.4878682100001,11.6,0.160829682999987));
#261560=CARTESIAN_POINT('Ctrl Pts',(-10.4862373250001,15.2,0.160523489999989));
#261561=CARTESIAN_POINT('Ctrl Pts',(-10.4862373250001,11.6,0.160523489999988));
#261562=CARTESIAN_POINT('Ctrl Pts',(-10.4846137770001,15.2,0.160220243999984));
#261563=CARTESIAN_POINT('Ctrl Pts',(-10.4846137770001,11.6,0.160220243999984));
#261564=CARTESIAN_POINT('Ctrl Pts',(-10.4829975860001,15.2,0.159919936999984));
#261565=CARTESIAN_POINT('Ctrl Pts',(-10.4829975860001,11.6,0.159919936999983));
#261566=CARTESIAN_POINT('Ctrl Pts',(-10.4813887750001,15.2,0.159622555999985));
#261567=CARTESIAN_POINT('Ctrl Pts',(-10.4813887750001,11.6,0.159622555999985));
#261568=CARTESIAN_POINT('Ctrl Pts',(-10.4797873630001,15.2,0.159328093999989));
#261569=CARTESIAN_POINT('Ctrl Pts',(-10.4797873630001,11.6,0.159328093999988));
#261570=CARTESIAN_POINT('Ctrl Pts',(-10.4781933710001,15.2,0.159036539999988));
#261571=CARTESIAN_POINT('Ctrl Pts',(-10.4781933710001,11.6,0.159036539999988));
#261572=CARTESIAN_POINT('Ctrl Pts',(-10.4766068200001,15.2,0.158747883999983));
#261573=CARTESIAN_POINT('Ctrl Pts',(-10.4766068200001,11.6,0.158747883999983));
#261574=CARTESIAN_POINT('Ctrl Pts',(-10.4750277290001,15.2,0.158462115999987));
#261575=CARTESIAN_POINT('Ctrl Pts',(-10.4750277290001,11.6,0.158462115999986));
#261576=CARTESIAN_POINT('Ctrl Pts',(-10.4734561210001,15.2,0.158179226999984));
#261577=CARTESIAN_POINT('Ctrl Pts',(-10.4734561210001,11.6,0.158179226999983));
#261578=CARTESIAN_POINT('Ctrl Pts',(-10.4718920160001,15.2,0.157899203999987));
#261579=CARTESIAN_POINT('Ctrl Pts',(-10.4718920160001,11.6,0.157899203999987));
#261580=CARTESIAN_POINT('Ctrl Pts',(-10.4703354350001,15.2,0.157622039999987));
#261581=CARTESIAN_POINT('Ctrl Pts',(-10.4703354350001,11.6,0.157622039999987));
#261582=CARTESIAN_POINT('Ctrl Pts',(-10.4687864010001,15.2,0.157347723999983));
#261583=CARTESIAN_POINT('Ctrl Pts',(-10.4687864010001,11.6,0.157347723999983));
#261584=CARTESIAN_POINT('Ctrl Pts',(-10.4672449310001,15.2,0.157076244999987));
#261585=CARTESIAN_POINT('Ctrl Pts',(-10.4672449310001,11.6,0.157076244999987));
#261586=CARTESIAN_POINT('Ctrl Pts',(-10.4657110500001,15.2,0.156807592999986));
#261587=CARTESIAN_POINT('Ctrl Pts',(-10.4657110500001,11.6,0.156807592999985));
#261588=CARTESIAN_POINT('Ctrl Pts',(-10.4641847780001,15.2,0.156541757999986));
#261589=CARTESIAN_POINT('Ctrl Pts',(-10.4641847780001,11.6,0.156541757999986));
#261590=CARTESIAN_POINT('Ctrl Pts',(-10.4626661360001,15.2,0.156278728999983));
#261591=CARTESIAN_POINT('Ctrl Pts',(-10.4626661360001,11.6,0.156278728999983));
#261592=CARTESIAN_POINT('Ctrl Pts',(-10.4611551460001,15.2,0.156018495999986));
#261593=CARTESIAN_POINT('Ctrl Pts',(-10.4611551460001,11.6,0.156018495999985));
#261594=CARTESIAN_POINT('Ctrl Pts',(-10.4596518290001,15.2,0.155761047999987));
#261595=CARTESIAN_POINT('Ctrl Pts',(-10.4596518290001,11.6,0.155761047999987));
#261596=CARTESIAN_POINT('Ctrl Pts',(-10.4581562070001,15.2,0.155506375999988));
#261597=CARTESIAN_POINT('Ctrl Pts',(-10.4581562070001,11.6,0.155506375999987));
#261598=CARTESIAN_POINT('Ctrl Pts',(-10.4566683020001,15.2,0.155254465999985));
#261599=CARTESIAN_POINT('Ctrl Pts',(-10.4566683020001,11.6,0.155254465999985));
#261600=CARTESIAN_POINT('Ctrl Pts',(-10.4551881360001,15.2,0.155005310999985));
#261601=CARTESIAN_POINT('Ctrl Pts',(-10.4551881360001,11.6,0.155005310999984));
#261602=CARTESIAN_POINT('Ctrl Pts',(-10.4537157300001,15.2,0.154758897999985));
#261603=CARTESIAN_POINT('Ctrl Pts',(-10.4537157300001,11.6,0.154758897999984));
#261604=CARTESIAN_POINT('Ctrl Pts',(-10.4522511070001,15.2,0.154515216999984));
#261605=CARTESIAN_POINT('Ctrl Pts',(-10.4522511070001,11.6,0.154515216999984));
#261606=CARTESIAN_POINT('Ctrl Pts',(-10.4507942880001,15.2,0.154274255999987));
#261607=CARTESIAN_POINT('Ctrl Pts',(-10.4507942880001,11.6,0.154274255999986));
#261608=CARTESIAN_POINT('Ctrl Pts',(-10.4493452950001,15.2,0.154036006999987));
#261609=CARTESIAN_POINT('Ctrl Pts',(-10.4493452950001,11.6,0.154036006999986));
#261610=CARTESIAN_POINT('Ctrl Pts',(-10.4479041520001,15.2,0.153800454999988));
#261611=CARTESIAN_POINT('Ctrl Pts',(-10.4479041520001,11.6,0.153800454999988));
#261612=CARTESIAN_POINT('Ctrl Pts',(-10.4464708800001,15.2,0.153567592999986));
#261613=CARTESIAN_POINT('Ctrl Pts',(-10.4464708800001,11.6,0.153567592999985));
#261614=CARTESIAN_POINT('Ctrl Pts',(-10.4450455010001,15.2,0.153337406999987));
#261615=CARTESIAN_POINT('Ctrl Pts',(-10.4450455010001,11.6,0.153337406999987));
#261616=CARTESIAN_POINT('Ctrl Pts',(-10.4436280380001,15.2,0.153109886999987));
#261617=CARTESIAN_POINT('Ctrl Pts',(-10.4436280380001,11.6,0.153109886999987));
#261618=CARTESIAN_POINT('Ctrl Pts',(-10.4422185140001,15.2,0.152885022999989));
#261619=CARTESIAN_POINT('Ctrl Pts',(-10.4422185140001,11.6,0.152885022999989));
#261620=CARTESIAN_POINT('Ctrl Pts',(-10.4408169510001,15.2,0.152662800999988));
#261621=CARTESIAN_POINT('Ctrl Pts',(-10.4408169510001,11.6,0.152662800999987));
#261622=CARTESIAN_POINT('Ctrl Pts',(-10.4394233720001,15.2,0.152443211999986));
#261623=CARTESIAN_POINT('Ctrl Pts',(-10.4394233720001,11.6,0.152443211999986));
#261624=CARTESIAN_POINT('Ctrl Pts',(-10.4380378000001,15.2,0.152226242999984));
#261625=CARTESIAN_POINT('Ctrl Pts',(-10.4380378000001,11.6,0.152226242999984));
#261626=CARTESIAN_POINT('Ctrl Pts',(-10.4366602580001,15.2,0.152011882999985));
#261627=CARTESIAN_POINT('Ctrl Pts',(-10.4366602580001,11.6,0.152011882999985));
#261628=CARTESIAN_POINT('Ctrl Pts',(-10.4352907680001,15.2,0.151800122999983));
#261629=CARTESIAN_POINT('Ctrl Pts',(-10.4352907680001,11.6,0.151800122999983));
#261630=CARTESIAN_POINT('Ctrl Pts',(-10.4339293550001,15.2,0.151590946999987));
#261631=CARTESIAN_POINT('Ctrl Pts',(-10.4339293550001,11.6,0.151590946999986));
#261632=CARTESIAN_POINT('Ctrl Pts',(-10.4325760410001,15.2,0.151384346999985));
#261633=CARTESIAN_POINT('Ctrl Pts',(-10.4325760410001,11.6,0.151384346999985));
#261634=CARTESIAN_POINT('Ctrl Pts',(-10.4312308480001,15.2,0.151180308999983));
#261635=CARTESIAN_POINT('Ctrl Pts',(-10.4312308480001,11.6,0.151180308999983));
#261636=CARTESIAN_POINT('Ctrl Pts',(-10.4298938030001,15.2,0.150978822999988));
#261637=CARTESIAN_POINT('Ctrl Pts',(-10.4298938030001,11.6,0.150978822999987));
#261638=CARTESIAN_POINT('Ctrl Pts',(-10.4285649260001,15.2,0.150779875999985));
#261639=CARTESIAN_POINT('Ctrl Pts',(-10.4285649260001,11.6,0.150779875999984));
#261640=CARTESIAN_POINT('Ctrl Pts',(-10.4272442410001,15.2,0.150583456999982));
#261641=CARTESIAN_POINT('Ctrl Pts',(-10.4272442410001,11.6,0.150583456999982));
#261642=CARTESIAN_POINT('Ctrl Pts',(-10.4259317730001,15.2,0.150389553999983));
#261643=CARTESIAN_POINT('Ctrl Pts',(-10.4259317730001,11.6,0.150389553999983));
#261644=CARTESIAN_POINT('Ctrl Pts',(-10.4246275460001,15.2,0.150198153999987));
#261645=CARTESIAN_POINT('Ctrl Pts',(-10.4246275460001,11.6,0.150198153999987));
#261646=CARTESIAN_POINT('Ctrl Pts',(-10.4233315830001,15.2,0.150009245999985));
#261647=CARTESIAN_POINT('Ctrl Pts',(-10.4233315830001,11.6,0.150009245999984));
#261648=CARTESIAN_POINT('Ctrl Pts',(-10.4220439070001,15.2,0.149822816999983));
#261649=CARTESIAN_POINT('Ctrl Pts',(-10.4220439070001,11.6,0.149822816999982));
#261650=CARTESIAN_POINT('Ctrl Pts',(-10.4207645450001,15.2,0.149638854999985));
#261651=CARTESIAN_POINT('Ctrl Pts',(-10.4207645450001,11.6,0.149638854999985));
#261652=CARTESIAN_POINT('Ctrl Pts',(-10.4194935180001,15.2,0.149457348999986));
#261653=CARTESIAN_POINT('Ctrl Pts',(-10.4194935180001,11.6,0.149457348999986));
#261654=CARTESIAN_POINT('Ctrl Pts',(-10.4182308520001,15.2,0.149278284999985));
#261655=CARTESIAN_POINT('Ctrl Pts',(-10.4182308520001,11.6,0.149278284999985));
#261656=CARTESIAN_POINT('Ctrl Pts',(-10.4169765720001,15.2,0.149101651999985));
#261657=CARTESIAN_POINT('Ctrl Pts',(-10.4169765720001,11.6,0.149101651999985));
#261658=CARTESIAN_POINT('Ctrl Pts',(-10.4157307010001,15.2,0.148927436999986));
#261659=CARTESIAN_POINT('Ctrl Pts',(-10.4157307010001,11.6,0.148927436999986));
#261660=CARTESIAN_POINT('Ctrl Pts',(-10.4144932620001,15.2,0.148755626999986));
#261661=CARTESIAN_POINT('Ctrl Pts',(-10.4144932620001,11.6,0.148755626999985));
#261662=CARTESIAN_POINT('Ctrl Pts',(-10.4132642840001,15.2,0.148586209999984));
#261663=CARTESIAN_POINT('Ctrl Pts',(-10.4132642840001,11.6,0.148586209999983));
#261664=CARTESIAN_POINT('Ctrl Pts',(-10.4120437890001,15.2,0.148419172999983));
#261665=CARTESIAN_POINT('Ctrl Pts',(-10.4120437890001,11.6,0.148419172999982));
#261666=CARTESIAN_POINT('Ctrl Pts',(-10.4108318020001,15.2,0.148254502999983));
#261667=CARTESIAN_POINT('Ctrl Pts',(-10.4108318020001,11.6,0.148254502999982));
#261668=CARTESIAN_POINT('Ctrl Pts',(-10.4096283490001,15.2,0.148092186999986));
#261669=CARTESIAN_POINT('Ctrl Pts',(-10.4096283490001,11.6,0.148092186999986));
#261670=CARTESIAN_POINT('Ctrl Pts',(-10.4084334530001,15.2,0.147932213999984));
#261671=CARTESIAN_POINT('Ctrl Pts',(-10.4084334530001,11.6,0.147932213999983));
#261672=CARTESIAN_POINT('Ctrl Pts',(-10.4072471420001,15.2,0.147774568999988));
#261673=CARTESIAN_POINT('Ctrl Pts',(-10.4072471420001,11.6,0.147774568999987));
#261674=CARTESIAN_POINT('Ctrl Pts',(-10.4060694410001,15.2,0.147619239999983));
#261675=CARTESIAN_POINT('Ctrl Pts',(-10.4060694410001,11.6,0.147619239999983));
#261676=CARTESIAN_POINT('Ctrl Pts',(-10.4049003720001,15.2,0.147466213999987));
#261677=CARTESIAN_POINT('Ctrl Pts',(-10.4049003720001,11.6,0.147466213999987));
#261678=CARTESIAN_POINT('Ctrl Pts',(-10.4037399650001,15.2,0.147315476999985));
#261679=CARTESIAN_POINT('Ctrl Pts',(-10.4037399650001,11.6,0.147315476999985));
#261680=CARTESIAN_POINT('Ctrl Pts',(-10.4025882420001,15.2,0.147167016999985));
#261681=CARTESIAN_POINT('Ctrl Pts',(-10.4025882420001,11.6,0.147167016999985));
#261682=CARTESIAN_POINT('Ctrl Pts',(-10.4014452320001,15.2,0.147020818999986));
#261683=CARTESIAN_POINT('Ctrl Pts',(-10.4014452320001,11.6,0.147020818999985));
#261684=CARTESIAN_POINT('Ctrl Pts',(-10.4003109570001,15.2,0.146876870999986));
#261685=CARTESIAN_POINT('Ctrl Pts',(-10.4003109570001,11.6,0.146876870999985));
#261686=CARTESIAN_POINT('Ctrl Pts',(-10.3991854470001,15.2,0.146735159999984));
#261687=CARTESIAN_POINT('Ctrl Pts',(-10.3991854470001,11.6,0.146735159999984));
#261688=CARTESIAN_POINT('Ctrl Pts',(-10.3980687260001,15.2,0.146595670999985));
#261689=CARTESIAN_POINT('Ctrl Pts',(-10.3980687260001,11.6,0.146595670999984));
#261690=CARTESIAN_POINT('Ctrl Pts',(-10.3969608200001,15.2,0.146458390999986));
#261691=CARTESIAN_POINT('Ctrl Pts',(-10.3969608200001,11.6,0.146458390999986));
#261692=CARTESIAN_POINT('Ctrl Pts',(-10.3958617570001,15.2,0.146323306999987));
#261693=CARTESIAN_POINT('Ctrl Pts',(-10.3958617570001,11.6,0.146323306999987));
#261694=CARTESIAN_POINT('Ctrl Pts',(-10.3947715610001,15.2,0.146190402999986));
#261695=CARTESIAN_POINT('Ctrl Pts',(-10.3947715610001,11.6,0.146190402999986));
#261696=CARTESIAN_POINT('Ctrl Pts',(-10.3936902610001,15.2,0.146059668999987));
#261697=CARTESIAN_POINT('Ctrl Pts',(-10.3936902610001,11.6,0.146059668999987));
#261698=CARTESIAN_POINT('Ctrl Pts',(-10.3926178820001,15.2,0.145931086999984));
#261699=CARTESIAN_POINT('Ctrl Pts',(-10.3926178820001,11.6,0.145931086999984));
#261700=CARTESIAN_POINT('Ctrl Pts',(-10.3915544510001,15.2,0.145804645999985));
#261701=CARTESIAN_POINT('Ctrl Pts',(-10.3915544510001,11.6,0.145804645999985));
#261702=CARTESIAN_POINT('Ctrl Pts',(-10.3904999960001,15.2,0.145680330999984));
#261703=CARTESIAN_POINT('Ctrl Pts',(-10.3904999960001,11.6,0.145680330999984));
#261704=CARTESIAN_POINT('Ctrl Pts',(-10.3894545430001,15.2,0.145558126999985));
#261705=CARTESIAN_POINT('Ctrl Pts',(-10.3894545430001,11.6,0.145558126999985));
#261706=CARTESIAN_POINT('Ctrl Pts',(-10.3884181200001,15.2,0.145438019999986));
#261707=CARTESIAN_POINT('Ctrl Pts',(-10.3884181200001,11.6,0.145438019999986));
#261708=CARTESIAN_POINT('Ctrl Pts',(-10.3873907530001,15.2,0.145319995999986));
#261709=CARTESIAN_POINT('Ctrl Pts',(-10.3873907530001,11.6,0.145319995999986));
#261710=CARTESIAN_POINT('Ctrl Pts',(-10.3863724700001,15.2,0.145204041999989));
#261711=CARTESIAN_POINT('Ctrl Pts',(-10.3863724700001,11.6,0.145204041999988));
#261712=CARTESIAN_POINT('Ctrl Pts',(-10.3853633010001,15.2,0.145090140999984));
#261713=CARTESIAN_POINT('Ctrl Pts',(-10.3853633010001,11.6,0.145090140999983));
#261714=CARTESIAN_POINT('Ctrl Pts',(-10.3843632700001,15.2,0.144978280999983));
#261715=CARTESIAN_POINT('Ctrl Pts',(-10.3843632700001,11.6,0.144978280999983));
#261716=CARTESIAN_POINT('Ctrl Pts',(-10.3833724070001,15.2,0.144868444999986));
#261717=CARTESIAN_POINT('Ctrl Pts',(-10.3833724070001,11.6,0.144868444999986));
#261718=CARTESIAN_POINT('Ctrl Pts',(-10.3823907380001,15.2,0.144760619999986));
#261719=CARTESIAN_POINT('Ctrl Pts',(-10.3823907380001,11.6,0.144760619999986));
#261720=CARTESIAN_POINT('Ctrl Pts',(-10.3814182930001,15.2,0.144654789999983));
#261721=CARTESIAN_POINT('Ctrl Pts',(-10.3814182930001,11.6,0.144654789999982));
#261722=CARTESIAN_POINT('Ctrl Pts',(-10.3804551000001,15.2,0.144550940999988));
#261723=CARTESIAN_POINT('Ctrl Pts',(-10.3804551000001,11.6,0.144550940999987));
#261724=CARTESIAN_POINT('Ctrl Pts',(-10.3795011870001,15.2,0.144449057999987));
#261725=CARTESIAN_POINT('Ctrl Pts',(-10.3795011870001,11.6,0.144449057999986));
#261726=CARTESIAN_POINT('Ctrl Pts',(-10.3785565820001,15.2,0.144349124999987));
#261727=CARTESIAN_POINT('Ctrl Pts',(-10.3785565820001,11.6,0.144349124999987));
#261728=CARTESIAN_POINT('Ctrl Pts',(-10.3776213140001,15.2,0.144251127999984));
#261729=CARTESIAN_POINT('Ctrl Pts',(-10.3776213140001,11.6,0.144251127999983));
#261730=CARTESIAN_POINT('Ctrl Pts',(-10.3766954110001,15.2,0.144155049999988));
#261731=CARTESIAN_POINT('Ctrl Pts',(-10.3766954110001,11.6,0.144155049999987));
#261732=CARTESIAN_POINT('Ctrl Pts',(-10.3757841830001,15.2,0.144061419999986));
#261733=CARTESIAN_POINT('Ctrl Pts',(-10.3757841830001,11.6,0.144061419999985));
#261734=CARTESIAN_POINT('Ctrl Pts',(-10.3750636860001,15.2,0.143988113999987));
#261735=CARTESIAN_POINT('Ctrl Pts',(-10.3750636860001,11.6,0.143988113999986));
#261736=CARTESIAN_POINT('Ctrl Pts',(-10.3745287910001,15.2,0.143934095999985));
#261737=CARTESIAN_POINT('Ctrl Pts',(-10.3745287910001,11.6,0.143934095999984));
#261738=CARTESIAN_POINT('Ctrl Pts',(-10.3741757630001,15.2,0.143898618999985));
#261739=CARTESIAN_POINT('Ctrl Pts',(-10.3741757630001,11.6,0.143898618999984));
#261740=CARTESIAN_POINT('Ctrl Pts',(-10.3740022750001,15.2,0.143881226999985));
#261741=CARTESIAN_POINT('Ctrl Pts',(-10.3740022750001,11.6,0.143881226999984));
#261742=CARTESIAN_POINT('',(-10.3740022750001,12.2,0.143881226999985));
#261743=CARTESIAN_POINT('',(-10.3740022750001,15.2,0.143881226999985));
#261744=CARTESIAN_POINT('',(-10.3740022750001,12.2,0.143881226999985));
#261745=CARTESIAN_POINT('Ctrl Pts',(-11.4869855320001,12.2,0.546958305999983));
#261746=CARTESIAN_POINT('Ctrl Pts',(-11.4863150090001,12.2,0.546590898999986));
#261747=CARTESIAN_POINT('Ctrl Pts',(-11.4849742100001,12.2,0.545856550999986));
#261748=CARTESIAN_POINT('Ctrl Pts',(-11.4829637560001,12.2,0.544756421999986));
#261749=CARTESIAN_POINT('Ctrl Pts',(-11.4802846430001,12.2,0.543292367999988));
#261750=CARTESIAN_POINT('Ctrl Pts',(-11.4769382380001,12.2,0.541466945999982));
#261751=CARTESIAN_POINT('Ctrl Pts',(-11.4735943180001,12.2,0.539646165999983));
#261752=CARTESIAN_POINT('Ctrl Pts',(-11.4702528880001,12.2,0.537830029999986));
#261753=CARTESIAN_POINT('Ctrl Pts',(-11.4669139500001,12.2,0.536018536999983));
#261754=CARTESIAN_POINT('Ctrl Pts',(-11.4635775100001,12.2,0.534211684999986));
#261755=CARTESIAN_POINT('Ctrl Pts',(-11.4602435780001,12.2,0.532409473999986));
#261756=CARTESIAN_POINT('Ctrl Pts',(-11.4569121620001,12.2,0.530611900999984));
#261757=CARTESIAN_POINT('Ctrl Pts',(-11.4535832720001,12.2,0.528818965999989));
#261758=CARTESIAN_POINT('Ctrl Pts',(-11.4502569220001,12.2,0.527030663999986));
#261759=CARTESIAN_POINT('Ctrl Pts',(-11.4469331180001,12.2,0.525246995999984));
#261760=CARTESIAN_POINT('Ctrl Pts',(-11.4436118760001,12.2,0.523467958999984));
#261761=CARTESIAN_POINT('Ctrl Pts',(-11.4402932010001,12.2,0.521693550999984));
#261762=CARTESIAN_POINT('Ctrl Pts',(-11.4369771030001,12.2,0.519923770999986));
#261763=CARTESIAN_POINT('Ctrl Pts',(-11.4336635900001,12.2,0.518158617999984));
#261764=CARTESIAN_POINT('Ctrl Pts',(-11.4303526710001,12.2,0.516398088999988));
#261765=CARTESIAN_POINT('Ctrl Pts',(-11.4270443520001,12.2,0.514642183999987));
#261766=CARTESIAN_POINT('Ctrl Pts',(-11.4237386430001,12.2,0.512890900999987));
#261767=CARTESIAN_POINT('Ctrl Pts',(-11.4204355510001,12.2,0.511144238999983));
#261768=CARTESIAN_POINT('Ctrl Pts',(-11.4171350880001,12.2,0.509402193999984));
#261769=CARTESIAN_POINT('Ctrl Pts',(-11.4138372610001,12.2,0.507664766999985));
#261770=CARTESIAN_POINT('Ctrl Pts',(-11.4105420820001,12.2,0.505931953999985));
#261771=CARTESIAN_POINT('Ctrl Pts',(-11.4072495570001,12.2,0.504203755999986));
#261772=CARTESIAN_POINT('Ctrl Pts',(-11.4039596970001,12.2,0.502480167999986));
#261773=CARTESIAN_POINT('Ctrl Pts',(-11.4006725110001,12.2,0.500761190999985));
#261774=CARTESIAN_POINT('Ctrl Pts',(-11.3973880080001,12.2,0.499046821999984));
#261775=CARTESIAN_POINT('Ctrl Pts',(-11.3941061970001,12.2,0.497337060999987));
#261776=CARTESIAN_POINT('Ctrl Pts',(-11.3908270860001,12.2,0.495631902999989));
#261777=CARTESIAN_POINT('Ctrl Pts',(-11.3875506850001,12.2,0.493931348999985));
#261778=CARTESIAN_POINT('Ctrl Pts',(-11.3842770020001,12.2,0.492235395999985));
#261779=CARTESIAN_POINT('Ctrl Pts',(-11.3810060480001,12.2,0.490544042999983));
#261780=CARTESIAN_POINT('Ctrl Pts',(-11.3777378300001,12.2,0.488857287999984));
#261781=CARTESIAN_POINT('Ctrl Pts',(-11.3744723580001,12.2,0.487175127999984));
#261782=CARTESIAN_POINT('Ctrl Pts',(-11.3712096420001,12.2,0.485497562999986));
#261783=CARTESIAN_POINT('Ctrl Pts',(-11.3679496900001,12.2,0.483824590999986));
#261784=CARTESIAN_POINT('Ctrl Pts',(-11.3646925130001,12.2,0.482156208999989));
#261785=CARTESIAN_POINT('Ctrl Pts',(-11.3614381180001,12.2,0.480492415999985));
#261786=CARTESIAN_POINT('Ctrl Pts',(-11.3581865150001,12.2,0.478833208999987));
#261787=CARTESIAN_POINT('Ctrl Pts',(-11.3549377140001,12.2,0.477178588999987));
#261788=CARTESIAN_POINT('Ctrl Pts',(-11.3516917240001,12.2,0.475528550999984));
#261789=CARTESIAN_POINT('Ctrl Pts',(-11.3484485530001,12.2,0.473883093999987));
#261790=CARTESIAN_POINT('Ctrl Pts',(-11.3452082120001,12.2,0.472242216999987));
#261791=CARTESIAN_POINT('Ctrl Pts',(-11.3419707090001,12.2,0.470605916999984));
#261792=CARTESIAN_POINT('Ctrl Pts',(-11.3387360540001,12.2,0.468974193999987));
#261793=CARTESIAN_POINT('Ctrl Pts',(-11.3355042560001,12.2,0.467347044999986));
#261794=CARTESIAN_POINT('Ctrl Pts',(-11.3322753250001,12.2,0.465724465999986));
#261795=CARTESIAN_POINT('Ctrl Pts',(-11.3290492700001,12.2,0.464106457999982));
#261796=CARTESIAN_POINT('Ctrl Pts',(-11.3258260990001,12.2,0.462493017999983));
#261797=CARTESIAN_POINT('Ctrl Pts',(-11.3226058230001,12.2,0.460884142999984));
#261798=CARTESIAN_POINT('Ctrl Pts',(-11.3193884510001,12.2,0.459279831999986));
#261799=CARTESIAN_POINT('Ctrl Pts',(-11.3161739920001,12.2,0.457680083999983));
#261800=CARTESIAN_POINT('Ctrl Pts',(-11.3129624580001,12.2,0.456084895999984));
#261801=CARTESIAN_POINT('Ctrl Pts',(-11.3097538530001,12.2,0.454494265999985));
#261802=CARTESIAN_POINT('Ctrl Pts',(-11.3065481920001,12.2,0.452908190999985));
#261803=CARTESIAN_POINT('Ctrl Pts',(-11.3033454810001,12.2,0.451326670999985));
#261804=CARTESIAN_POINT('Ctrl Pts',(-11.3001457320001,12.2,0.449749702999984));
#261805=CARTESIAN_POINT('Ctrl Pts',(-11.2969489510001,12.2,0.448177283999982));
#261806=CARTESIAN_POINT('Ctrl Pts',(-11.2937551520001,12.2,0.446609412999983));
#261807=CARTESIAN_POINT('Ctrl Pts',(-11.2905643410001,12.2,0.445046087999987));
#261808=CARTESIAN_POINT('Ctrl Pts',(-11.2873765290001,12.2,0.443487306999986));
#261809=CARTESIAN_POINT('Ctrl Pts',(-11.2841917260001,12.2,0.441933066999987));
#261810=CARTESIAN_POINT('Ctrl Pts',(-11.2810099400001,12.2,0.440383366999986));
#261811=CARTESIAN_POINT('Ctrl Pts',(-11.2778311820001,12.2,0.438838203999987));
#261812=CARTESIAN_POINT('Ctrl Pts',(-11.2746554610001,12.2,0.437297575999986));
#261813=CARTESIAN_POINT('Ctrl Pts',(-11.2714827870001,12.2,0.435761481999983));
#261814=CARTESIAN_POINT('Ctrl Pts',(-11.2683131690001,12.2,0.434229917999982));
#261815=CARTESIAN_POINT('Ctrl Pts',(-11.2651466170001,12.2,0.432702882999987));
#261816=CARTESIAN_POINT('Ctrl Pts',(-11.2619831420001,12.2,0.431180374999984));
#261817=CARTESIAN_POINT('Ctrl Pts',(-11.2588227510001,12.2,0.429662389999983));
#261818=CARTESIAN_POINT('Ctrl Pts',(-11.2556654560001,12.2,0.428148927999987));
#261819=CARTESIAN_POINT('Ctrl Pts',(-11.2525112650001,12.2,0.426639985999984));
#261820=CARTESIAN_POINT('Ctrl Pts',(-11.2493601900001,12.2,0.425135561999985));
#261821=CARTESIAN_POINT('Ctrl Pts',(-11.2462122380001,12.2,0.423635652999987));
#261822=CARTESIAN_POINT('Ctrl Pts',(-11.2430674210001,12.2,0.422140256999985));
#261823=CARTESIAN_POINT('Ctrl Pts',(-11.2399257470001,12.2,0.420649372999984));
#261824=CARTESIAN_POINT('Ctrl Pts',(-11.2367872280001,12.2,0.419162996999987));
#261825=CARTESIAN_POINT('Ctrl Pts',(-11.2336518720001,12.2,0.417681126999985));
#261826=CARTESIAN_POINT('Ctrl Pts',(-11.2305196890001,12.2,0.416203761999987));
#261827=CARTESIAN_POINT('Ctrl Pts',(-11.2273906900001,12.2,0.414730897999984));
#261828=CARTESIAN_POINT('Ctrl Pts',(-11.2242648840001,12.2,0.413262533999985));
#261829=CARTESIAN_POINT('Ctrl Pts',(-11.2211422810001,12.2,0.411798666999985));
#261830=CARTESIAN_POINT('Ctrl Pts',(-11.2180228910001,12.2,0.410339293999984));
#261831=CARTESIAN_POINT('Ctrl Pts',(-11.2149067230001,12.2,0.408884414999986));
#261832=CARTESIAN_POINT('Ctrl Pts',(-11.2117937880001,12.2,0.407434024999986));
#261833=CARTESIAN_POINT('Ctrl Pts',(-11.2086840970001,12.2,0.405988122999985));
#261834=CARTESIAN_POINT('Ctrl Pts',(-11.2055776580001,12.2,0.404546704999986));
#261835=CARTESIAN_POINT('Ctrl Pts',(-11.2024744820001,12.2,0.403109771999985));
#261836=CARTESIAN_POINT('Ctrl Pts',(-11.1993745780001,12.2,0.401677316999987));
#261837=CARTESIAN_POINT('Ctrl Pts',(-11.1962779570001,12.2,0.400249341999985));
#261838=CARTESIAN_POINT('Ctrl Pts',(-11.1931846300001,12.2,0.398825840999986));
#261839=CARTESIAN_POINT('Ctrl Pts',(-11.1900946040001,12.2,0.397406813999983));
#261840=CARTESIAN_POINT('Ctrl Pts',(-11.1870078920001,12.2,0.395992257999982));
#261841=CARTESIAN_POINT('Ctrl Pts',(-11.1839245020001,12.2,0.394582169999986));
#261842=CARTESIAN_POINT('Ctrl Pts',(-11.1808444470001,12.2,0.393176545999987));
#261843=CARTESIAN_POINT('Ctrl Pts',(-11.1777677340001,12.2,0.391775386999988));
#261844=CARTESIAN_POINT('Ctrl Pts',(-11.1746943740001,12.2,0.390378687999986));
#261845=CARTESIAN_POINT('Ctrl Pts',(-11.1716243780001,12.2,0.388986446999984));
#261846=CARTESIAN_POINT('Ctrl Pts',(-11.1685577570001,12.2,0.387598660999986));
#261847=CARTESIAN_POINT('Ctrl Pts',(-11.1654945190001,12.2,0.386215327999988));
#261848=CARTESIAN_POINT('Ctrl Pts',(-11.1624346740001,12.2,0.384836445999985));
#261849=CARTESIAN_POINT('Ctrl Pts',(-11.1593782350001,12.2,0.383462010999986));
#261850=CARTESIAN_POINT('Ctrl Pts',(-11.1563252100001,12.2,0.382092021999987));
#261851=CARTESIAN_POINT('Ctrl Pts',(-11.1532756110001,12.2,0.380726473999986));
#261852=CARTESIAN_POINT('Ctrl Pts',(-11.1502294460001,12.2,0.379365366999984));
#261853=CARTESIAN_POINT('Ctrl Pts',(-11.1471867270001,12.2,0.378008696999985));
#261854=CARTESIAN_POINT('Ctrl Pts',(-11.1441474640001,12.2,0.376656461999989));
#261855=CARTESIAN_POINT('Ctrl Pts',(-11.1411116670001,12.2,0.375308657999986));
#261856=CARTESIAN_POINT('Ctrl Pts',(-11.1380793470001,12.2,0.373965283999986));
#261857=CARTESIAN_POINT('Ctrl Pts',(-11.1350505130001,12.2,0.372626335999984));
#261858=CARTESIAN_POINT('Ctrl Pts',(-11.1320251780001,12.2,0.371291811999988));
#261859=CARTESIAN_POINT('Ctrl Pts',(-11.1290033490001,12.2,0.369961708999984));
#261860=CARTESIAN_POINT('Ctrl Pts',(-11.1259850390001,12.2,0.368636023999986));
#261861=CARTESIAN_POINT('Ctrl Pts',(-11.1229702580001,12.2,0.367314754999986));
#261862=CARTESIAN_POINT('Ctrl Pts',(-11.1199590150001,12.2,0.365997898999986));
#261863=CARTESIAN_POINT('Ctrl Pts',(-11.1169513230001,12.2,0.364685452999982));
#261864=CARTESIAN_POINT('Ctrl Pts',(-11.1139471900001,12.2,0.363377413999988));
#261865=CARTESIAN_POINT('Ctrl Pts',(-11.1109466290001,12.2,0.362073778999985));
#261866=CARTESIAN_POINT('Ctrl Pts',(-11.1079496490001,12.2,0.360774545999987));
#261867=CARTESIAN_POINT('Ctrl Pts',(-11.1049562600001,12.2,0.359479711999988));
#261868=CARTESIAN_POINT('Ctrl Pts',(-11.1019664740001,12.2,0.358189272999985));
#261869=CARTESIAN_POINT('Ctrl Pts',(-11.0989803000001,12.2,0.356903227999985));
#261870=CARTESIAN_POINT('Ctrl Pts',(-11.0959977500001,12.2,0.355621572999985));
#261871=CARTESIAN_POINT('Ctrl Pts',(-11.0930188360001,12.2,0.354344304999987));
#261872=CARTESIAN_POINT('Ctrl Pts',(-11.0900435650001,12.2,0.353071420999989));
#261873=CARTESIAN_POINT('Ctrl Pts',(-11.0870719500001,12.2,0.351802918999984));
#261874=CARTESIAN_POINT('Ctrl Pts',(-11.0841040020001,12.2,0.350538794999986));
#261875=CARTESIAN_POINT('Ctrl Pts',(-11.0811397300001,12.2,0.349279046999986));
#261876=CARTESIAN_POINT('Ctrl Pts',(-11.0781791480001,12.2,0.348023670999984));
#261877=CARTESIAN_POINT('Ctrl Pts',(-11.0752222620001,12.2,0.346772664999988));
#261878=CARTESIAN_POINT('Ctrl Pts',(-11.0722690870001,12.2,0.345526024999985));
#261879=CARTESIAN_POINT('Ctrl Pts',(-11.0693196320001,12.2,0.344283748999987));
#261880=CARTESIAN_POINT('Ctrl Pts',(-11.0663739070001,12.2,0.343045833999986));
#261881=CARTESIAN_POINT('Ctrl Pts',(-11.0634319250001,12.2,0.341812274999986));
#261882=CARTESIAN_POINT('Ctrl Pts',(-11.0604936960001,12.2,0.340583071999987));
#261883=CARTESIAN_POINT('Ctrl Pts',(-11.0575592300001,12.2,0.339358219999983));
#261884=CARTESIAN_POINT('Ctrl Pts',(-11.0546285370001,12.2,0.338137715999984));
#261885=CARTESIAN_POINT('Ctrl Pts',(-11.0517016320001,12.2,0.336921557999985));
#261886=CARTESIAN_POINT('Ctrl Pts',(-11.0487785220001,12.2,0.335709739999985));
#261887=CARTESIAN_POINT('Ctrl Pts',(-11.0458592200001,12.2,0.334502262999985));
#261888=CARTESIAN_POINT('Ctrl Pts',(-11.0429437360001,12.2,0.333299120999988));
#261889=CARTESIAN_POINT('Ctrl Pts',(-11.0400320810001,12.2,0.332100310999985));
#261890=CARTESIAN_POINT('Ctrl Pts',(-11.0371242670001,12.2,0.330905830999986));
#261891=CARTESIAN_POINT('Ctrl Pts',(-11.0342203030001,12.2,0.329715676999989));
#261892=CARTESIAN_POINT('Ctrl Pts',(-11.0313202040001,12.2,0.328529845999985));
#261893=CARTESIAN_POINT('Ctrl Pts',(-11.0284239770001,12.2,0.327348335999984));
#261894=CARTESIAN_POINT('Ctrl Pts',(-11.0255316350001,12.2,0.326171140999989));
#261895=CARTESIAN_POINT('Ctrl Pts',(-11.0226431890001,12.2,0.324998259999987));
#261896=CARTESIAN_POINT('Ctrl Pts',(-11.0197586510001,12.2,0.323829688999986));
#261897=CARTESIAN_POINT('Ctrl Pts',(-11.0168780300001,12.2,0.322665424999986));
#261898=CARTESIAN_POINT('Ctrl Pts',(-11.0140013380001,12.2,0.321505463999987));
#261899=CARTESIAN_POINT('Ctrl Pts',(-11.0111285880001,12.2,0.320349803999989));
#261900=CARTESIAN_POINT('Ctrl Pts',(-11.0082597890001,12.2,0.319198439999986));
#261901=CARTESIAN_POINT('Ctrl Pts',(-11.0053949540001,12.2,0.318051369999988));
#261902=CARTESIAN_POINT('Ctrl Pts',(-11.0025340930001,12.2,0.316908588999985));
#261903=CARTESIAN_POINT('Ctrl Pts',(-10.9996772170001,12.2,0.315770094999985));
#261904=CARTESIAN_POINT('Ctrl Pts',(-10.9968243390001,12.2,0.314635884999985));
#261905=CARTESIAN_POINT('Ctrl Pts',(-10.9939754690001,12.2,0.313505953999984));
#261906=CARTESIAN_POINT('Ctrl Pts',(-10.9911306190001,12.2,0.312380299999986));
#261907=CARTESIAN_POINT('Ctrl Pts',(-10.9882898000001,12.2,0.311258919999986));
#261908=CARTESIAN_POINT('Ctrl Pts',(-10.9854530250001,12.2,0.310141807999984));
#261909=CARTESIAN_POINT('Ctrl Pts',(-10.9826203020001,12.2,0.309028961999989));
#261910=CARTESIAN_POINT('Ctrl Pts',(-10.9797916470001,12.2,0.307920378999986));
#261911=CARTESIAN_POINT('Ctrl Pts',(-10.9769670670001,12.2,0.306816054999985));
#261912=CARTESIAN_POINT('Ctrl Pts',(-10.9741465770001,12.2,0.305715986999986));
#261913=CARTESIAN_POINT('Ctrl Pts',(-10.9713301870001,12.2,0.304620170999983));
#261914=CARTESIAN_POINT('Ctrl Pts',(-10.9685179070001,12.2,0.303528602999985));
#261915=CARTESIAN_POINT('Ctrl Pts',(-10.9657097520001,12.2,0.302441278999983));
#261916=CARTESIAN_POINT('Ctrl Pts',(-10.9629057310001,12.2,0.301358197999986));
#261917=CARTESIAN_POINT('Ctrl Pts',(-10.9601058580001,12.2,0.300279352999984));
#261918=CARTESIAN_POINT('Ctrl Pts',(-10.9573101410001,12.2,0.299204742999986));
#261919=CARTESIAN_POINT('Ctrl Pts',(-10.9545185950001,12.2,0.298134361999987));
#261920=CARTESIAN_POINT('Ctrl Pts',(-10.9517312310001,12.2,0.297068208999987));
#261921=CARTESIAN_POINT('Ctrl Pts',(-10.9489480600001,12.2,0.296006278999985));
#261922=CARTESIAN_POINT('Ctrl Pts',(-10.9461690940001,12.2,0.294948567999986));
#261923=CARTESIAN_POINT('Ctrl Pts',(-10.9433943440001,12.2,0.293895071999986));
#261924=CARTESIAN_POINT('Ctrl Pts',(-10.9406238230001,12.2,0.292845787999987));
#261925=CARTESIAN_POINT('Ctrl Pts',(-10.9378575430001,12.2,0.291800712999986));
#261926=CARTESIAN_POINT('Ctrl Pts',(-10.9350955160001,12.2,0.290759840999986));
#261927=CARTESIAN_POINT('Ctrl Pts',(-10.9323377520001,12.2,0.289723170999987));
#261928=CARTESIAN_POINT('Ctrl Pts',(-10.9295842640001,12.2,0.288690695999985));
#261929=CARTESIAN_POINT('Ctrl Pts',(-10.9268350640001,12.2,0.287662414999983));
#261930=CARTESIAN_POINT('Ctrl Pts',(-10.9240901640001,12.2,0.286638322999986));
#261931=CARTESIAN_POINT('Ctrl Pts',(-10.9213495760001,12.2,0.285618414999984));
#261932=CARTESIAN_POINT('Ctrl Pts',(-10.9186133120001,12.2,0.284602688999982));
#261933=CARTESIAN_POINT('Ctrl Pts',(-10.9158813840001,12.2,0.283591140999988));
#261934=CARTESIAN_POINT('Ctrl Pts',(-10.9131538030001,12.2,0.282583765999984));
#261935=CARTESIAN_POINT('Ctrl Pts',(-10.9104305830001,12.2,0.281580559999988));
#261936=CARTESIAN_POINT('Ctrl Pts',(-10.9077117350001,12.2,0.280581520999985));
#261937=CARTESIAN_POINT('Ctrl Pts',(-10.9049972710001,12.2,0.279586640999985));
#261938=CARTESIAN_POINT('Ctrl Pts',(-10.9022872040001,12.2,0.278595920999987));
#261939=CARTESIAN_POINT('Ctrl Pts',(-10.8995815450001,12.2,0.277609353999986));
#261940=CARTESIAN_POINT('Ctrl Pts',(-10.8968803070001,12.2,0.276626936999986));
#261941=CARTESIAN_POINT('Ctrl Pts',(-10.8941835000001,12.2,0.275648664999988));
#261942=CARTESIAN_POINT('Ctrl Pts',(-10.8914911410001,12.2,0.274674534999986));
#261943=CARTESIAN_POINT('Ctrl Pts',(-10.8888032380001,12.2,0.273704540999984));
#261944=CARTESIAN_POINT('Ctrl Pts',(-10.8861198050001,12.2,0.272738680999982));
#261945=CARTESIAN_POINT('Ctrl Pts',(-10.8834408550001,12.2,0.271776950999989));
#261946=CARTESIAN_POINT('Ctrl Pts',(-10.8807663990001,12.2,0.270819344999986));
#261947=CARTESIAN_POINT('Ctrl Pts',(-10.8780964490001,12.2,0.269865860999987));
#261948=CARTESIAN_POINT('Ctrl Pts',(-10.8754310200001,12.2,0.268916491999986));
#261949=CARTESIAN_POINT('Ctrl Pts',(-10.8727701220001,12.2,0.267971236999984));
#261950=CARTESIAN_POINT('Ctrl Pts',(-10.8701137680001,12.2,0.267030089999984));
#261951=CARTESIAN_POINT('Ctrl Pts',(-10.8674619700001,12.2,0.266093045999987));
#261952=CARTESIAN_POINT('Ctrl Pts',(-10.8648147410001,12.2,0.265160102999986));
#261953=CARTESIAN_POINT('Ctrl Pts',(-10.8621720950001,12.2,0.264231254999987));
#261954=CARTESIAN_POINT('Ctrl Pts',(-10.8595340430001,12.2,0.263306497999984));
#261955=CARTESIAN_POINT('Ctrl Pts',(-10.8569005980001,12.2,0.262385827999987));
#261956=CARTESIAN_POINT('Ctrl Pts',(-10.8542717720001,12.2,0.261469240999985));
#261957=CARTESIAN_POINT('Ctrl Pts',(-10.8516475780001,12.2,0.260556731999984));
#261958=CARTESIAN_POINT('Ctrl Pts',(-10.8490280300001,12.2,0.259648296999986));
#261959=CARTESIAN_POINT('Ctrl Pts',(-10.8464131390001,12.2,0.258743930999987));
#261960=CARTESIAN_POINT('Ctrl Pts',(-10.8438029180001,12.2,0.257843629999983));
#261961=CARTESIAN_POINT('Ctrl Pts',(-10.8411973810001,12.2,0.256947389999986));
#261962=CARTESIAN_POINT('Ctrl Pts',(-10.8385965390001,12.2,0.256055205999988));
#261963=CARTESIAN_POINT('Ctrl Pts',(-10.8360004070001,12.2,0.255167072999987));
#261964=CARTESIAN_POINT('Ctrl Pts',(-10.8334089940001,12.2,0.254282987999983));
#261965=CARTESIAN_POINT('Ctrl Pts',(-10.8308223180001,12.2,0.253402943999985));
#261966=CARTESIAN_POINT('Ctrl Pts',(-10.8282403890001,12.2,0.252526939999989));
#261967=CARTESIAN_POINT('Ctrl Pts',(-10.8256632200001,12.2,0.251654968999984));
#261968=CARTESIAN_POINT('Ctrl Pts',(-10.8230908230001,12.2,0.250787025999983));
#261969=CARTESIAN_POINT('Ctrl Pts',(-10.8205232130001,12.2,0.249923108999983));
#261970=CARTESIAN_POINT('Ctrl Pts',(-10.8179604030001,12.2,0.249063209999987));
#261971=CARTESIAN_POINT('Ctrl Pts',(-10.8154024050001,12.2,0.248207326999985));
#261972=CARTESIAN_POINT('Ctrl Pts',(-10.8128492330001,12.2,0.247355453999987));
#261973=CARTESIAN_POINT('Ctrl Pts',(-10.8103008990001,12.2,0.246507586999982));
#261974=CARTESIAN_POINT('Ctrl Pts',(-10.8077574170001,12.2,0.245663720999989));
#261975=CARTESIAN_POINT('Ctrl Pts',(-10.8052187990001,12.2,0.244823850999989));
#261976=CARTESIAN_POINT('Ctrl Pts',(-10.8026850610001,12.2,0.243987971999986));
#261977=CARTESIAN_POINT('Ctrl Pts',(-10.8001562130001,12.2,0.243156080999984));
#261978=CARTESIAN_POINT('Ctrl Pts',(-10.7976322700001,12.2,0.242328170999984));
#261979=CARTESIAN_POINT('Ctrl Pts',(-10.7951132440001,12.2,0.241504237999983));
#261980=CARTESIAN_POINT('Ctrl Pts',(-10.7925991510001,12.2,0.240684276999983));
#261981=CARTESIAN_POINT('Ctrl Pts',(-10.7900900010001,12.2,0.239868283999982));
#261982=CARTESIAN_POINT('Ctrl Pts',(-10.7875858100001,12.2,0.239056253999985));
#261983=CARTESIAN_POINT('Ctrl Pts',(-10.7850865910001,12.2,0.238248179999987));
#261984=CARTESIAN_POINT('Ctrl Pts',(-10.7825923560001,12.2,0.237444060999987));
#261985=CARTESIAN_POINT('Ctrl Pts',(-10.7801031190001,12.2,0.236643886999985));
#261986=CARTESIAN_POINT('Ctrl Pts',(-10.7776188950001,12.2,0.235847656999986));
#261987=CARTESIAN_POINT('Ctrl Pts',(-10.7751396960001,12.2,0.235055364999983));
#261988=CARTESIAN_POINT('Ctrl Pts',(-10.7726655360001,12.2,0.234267004999986));
#261989=CARTESIAN_POINT('Ctrl Pts',(-10.7701964290001,12.2,0.233482572999986));
#261990=CARTESIAN_POINT('Ctrl Pts',(-10.7677323890001,12.2,0.232702063999985));
#261991=CARTESIAN_POINT('Ctrl Pts',(-10.7652734280001,12.2,0.231925471999985));
#261992=CARTESIAN_POINT('Ctrl Pts',(-10.7628195610001,12.2,0.231152792999989));
#261993=CARTESIAN_POINT('Ctrl Pts',(-10.7603708020001,12.2,0.230384019999987));
#261994=CARTESIAN_POINT('Ctrl Pts',(-10.7579271630001,12.2,0.229619148999984));
#261995=CARTESIAN_POINT('Ctrl Pts',(-10.7554886610001,12.2,0.228858175999989));
#261996=CARTESIAN_POINT('Ctrl Pts',(-10.7530553070001,12.2,0.228101093999986));
#261997=CARTESIAN_POINT('Ctrl Pts',(-10.7506271160001,12.2,0.227347897999985));
#261998=CARTESIAN_POINT('Ctrl Pts',(-10.7482041010001,12.2,0.226598583999986));
#261999=CARTESIAN_POINT('Ctrl Pts',(-10.7457862770001,12.2,0.225853145999988));
#262000=CARTESIAN_POINT('Ctrl Pts',(-10.7433736600001,12.2,0.225111577999986));
#262001=CARTESIAN_POINT('Ctrl Pts',(-10.7409662590001,12.2,0.224373874999984));
#262002=CARTESIAN_POINT('Ctrl Pts',(-10.7385640920001,12.2,0.223640032999985));
#262003=CARTESIAN_POINT('Ctrl Pts',(-10.7361671710001,12.2,0.222910043999986));
#262004=CARTESIAN_POINT('Ctrl Pts',(-10.7337755120001,12.2,0.222183903999986));
#262005=CARTESIAN_POINT('Ctrl Pts',(-10.7313891280001,12.2,0.221461608999984));
#262006=CARTESIAN_POINT('Ctrl Pts',(-10.7290080330001,12.2,0.220743150999985));
#262007=CARTESIAN_POINT('Ctrl Pts',(-10.7266322420001,12.2,0.220028526999982));
#262008=CARTESIAN_POINT('Ctrl Pts',(-10.7242617690001,12.2,0.219317729999986));
#262009=CARTESIAN_POINT('Ctrl Pts',(-10.7218966280001,12.2,0.218610753999986));
#262010=CARTESIAN_POINT('Ctrl Pts',(-10.7195368330001,12.2,0.217907592999986));
#262011=CARTESIAN_POINT('Ctrl Pts',(-10.7171823990001,12.2,0.217208243999987));
#262012=CARTESIAN_POINT('Ctrl Pts',(-10.7148333410001,12.2,0.216512699999987));
#262013=CARTESIAN_POINT('Ctrl Pts',(-10.7124896730001,12.2,0.215820953999986));
#262014=CARTESIAN_POINT('Ctrl Pts',(-10.7101514080001,12.2,0.215133002999988));
#262015=CARTESIAN_POINT('Ctrl Pts',(-10.7078185620001,12.2,0.214448838999988));
#262016=CARTESIAN_POINT('Ctrl Pts',(-10.7054911500001,12.2,0.213768457999985));
#262017=CARTESIAN_POINT('Ctrl Pts',(-10.7031691860001,12.2,0.213091852999985));
#262018=CARTESIAN_POINT('Ctrl Pts',(-10.7008526850001,12.2,0.212419018999985));
#262019=CARTESIAN_POINT('Ctrl Pts',(-10.6985416600001,12.2,0.211749948999986));
#262020=CARTESIAN_POINT('Ctrl Pts',(-10.6962361280001,12.2,0.211084637999988));
#262021=CARTESIAN_POINT('Ctrl Pts',(-10.6939361020001,12.2,0.210423081999984));
#262022=CARTESIAN_POINT('Ctrl Pts',(-10.6916415980001,12.2,0.209765271999984));
#262023=CARTESIAN_POINT('Ctrl Pts',(-10.6893526300001,12.2,0.209111201999987));
#262024=CARTESIAN_POINT('Ctrl Pts',(-10.6870692130001,12.2,0.208460869999989));
#262025=CARTESIAN_POINT('Ctrl Pts',(-10.6847913630001,12.2,0.207814266999984));
#262026=CARTESIAN_POINT('Ctrl Pts',(-10.6825190920001,12.2,0.207171386999985));
#262027=CARTESIAN_POINT('Ctrl Pts',(-10.6802524190001,12.2,0.206532224999982));
#262028=CARTESIAN_POINT('Ctrl Pts',(-10.6779913570001,12.2,0.205896773999985));
#262029=CARTESIAN_POINT('Ctrl Pts',(-10.6757359200001,12.2,0.205265028999988));
#262030=CARTESIAN_POINT('Ctrl Pts',(-10.6734861240001,12.2,0.204636982999986));
#262031=CARTESIAN_POINT('Ctrl Pts',(-10.6712419860001,12.2,0.204012629999983));
#262032=CARTESIAN_POINT('Ctrl Pts',(-10.6690035190001,12.2,0.203391963999984));
#262033=CARTESIAN_POINT('Ctrl Pts',(-10.6667707370001,12.2,0.202774979999987));
#262034=CARTESIAN_POINT('Ctrl Pts',(-10.6645436590001,12.2,0.202161669999987));
#262035=CARTESIAN_POINT('Ctrl Pts',(-10.6623222980001,12.2,0.201552028999985));
#262036=CARTESIAN_POINT('Ctrl Pts',(-10.6601066700001,12.2,0.200946048999988));
#262037=CARTESIAN_POINT('Ctrl Pts',(-10.6578967890001,12.2,0.200343724999983));
#262038=CARTESIAN_POINT('Ctrl Pts',(-10.6556926720001,12.2,0.199745050999987));
#262039=CARTESIAN_POINT('Ctrl Pts',(-10.6534943330001,12.2,0.199150019999985));
#262040=CARTESIAN_POINT('Ctrl Pts',(-10.6513017900001,12.2,0.198558625999983));
#262041=CARTESIAN_POINT('Ctrl Pts',(-10.6491150560001,12.2,0.197970862999988));
#262042=CARTESIAN_POINT('Ctrl Pts',(-10.6469341480001,12.2,0.197386722999986));
#262043=CARTESIAN_POINT('Ctrl Pts',(-10.6447590820001,12.2,0.196806200999986));
#262044=CARTESIAN_POINT('Ctrl Pts',(-10.6425898720001,12.2,0.196229288999987));
#262045=CARTESIAN_POINT('Ctrl Pts',(-10.6404265340001,12.2,0.195655982999985));
#262046=CARTESIAN_POINT('Ctrl Pts',(-10.6382690860001,12.2,0.195086272999987));
#262047=CARTESIAN_POINT('Ctrl Pts',(-10.6361175410001,12.2,0.194520154999989));
#262048=CARTESIAN_POINT('Ctrl Pts',(-10.6339719170001,12.2,0.193957621999985));
#262049=CARTESIAN_POINT('Ctrl Pts',(-10.6318322290001,12.2,0.193398666999984));
#262050=CARTESIAN_POINT('Ctrl Pts',(-10.6296984920001,12.2,0.192843283999986));
#262051=CARTESIAN_POINT('Ctrl Pts',(-10.6275707240001,12.2,0.192291463999985));
#262052=CARTESIAN_POINT('Ctrl Pts',(-10.6254489400001,12.2,0.191743201999985));
#262053=CARTESIAN_POINT('Ctrl Pts',(-10.6233331560001,12.2,0.191198491999987));
#262054=CARTESIAN_POINT('Ctrl Pts',(-10.6212233880001,12.2,0.190657325999983));
#262055=CARTESIAN_POINT('Ctrl Pts',(-10.6191196530001,12.2,0.190119695999984));
#262056=CARTESIAN_POINT('Ctrl Pts',(-10.6170219660001,12.2,0.189585598999984));
#262057=CARTESIAN_POINT('Ctrl Pts',(-10.6149303440001,12.2,0.189055023999987));
#262058=CARTESIAN_POINT('Ctrl Pts',(-10.6128448030001,12.2,0.188527964999987));
#262059=CARTESIAN_POINT('Ctrl Pts',(-10.6107653600001,12.2,0.188004416999985));
#262060=CARTESIAN_POINT('Ctrl Pts',(-10.6086920310001,12.2,0.187484370999984));
#262061=CARTESIAN_POINT('Ctrl Pts',(-10.6066248330001,12.2,0.186967819999988));
#262062=CARTESIAN_POINT('Ctrl Pts',(-10.6045637800001,12.2,0.186454757999983));
#262063=CARTESIAN_POINT('Ctrl Pts',(-10.6025088930001,12.2,0.185945177999987));
#262064=CARTESIAN_POINT('Ctrl Pts',(-10.6004601840001,12.2,0.185439070999984));
#262065=CARTESIAN_POINT('Ctrl Pts',(-10.5984176730001,12.2,0.184936432999985));
#262066=CARTESIAN_POINT('Ctrl Pts',(-10.5963813760001,12.2,0.184437252999987));
#262067=CARTESIAN_POINT('Ctrl Pts',(-10.5943513080001,12.2,0.183941525999987));
#262068=CARTESIAN_POINT('Ctrl Pts',(-10.5923274870001,12.2,0.183449243999987));
#262069=CARTESIAN_POINT('Ctrl Pts',(-10.5903099300001,12.2,0.182960399999987));
#262070=CARTESIAN_POINT('Ctrl Pts',(-10.5882986550001,12.2,0.182474987999988));
#262071=CARTESIAN_POINT('Ctrl Pts',(-10.5862936760001,12.2,0.181992998999987));
#262072=CARTESIAN_POINT('Ctrl Pts',(-10.5842950130001,12.2,0.181514424999989));
#262073=CARTESIAN_POINT('Ctrl Pts',(-10.5823026810001,12.2,0.181039259999984));
#262074=CARTESIAN_POINT('Ctrl Pts',(-10.5803166980001,12.2,0.180567494999986));
#262075=CARTESIAN_POINT('Ctrl Pts',(-10.5783370810001,12.2,0.180099124999984));
#262076=CARTESIAN_POINT('Ctrl Pts',(-10.5763638480001,12.2,0.179634139999987));
#262077=CARTESIAN_POINT('Ctrl Pts',(-10.5743970150001,12.2,0.179172532999985));
#262078=CARTESIAN_POINT('Ctrl Pts',(-10.5724365990001,12.2,0.178714295999987));
#262079=CARTESIAN_POINT('Ctrl Pts',(-10.5704826190001,12.2,0.178259422999982));
#262080=CARTESIAN_POINT('Ctrl Pts',(-10.5685350920001,12.2,0.177807903999985));
#262081=CARTESIAN_POINT('Ctrl Pts',(-10.5665940340001,12.2,0.177359733999989));
#262082=CARTESIAN_POINT('Ctrl Pts',(-10.5646594650001,12.2,0.176914901999985));
#262083=CARTESIAN_POINT('Ctrl Pts',(-10.5627314000001,12.2,0.176473403999986));
#262084=CARTESIAN_POINT('Ctrl Pts',(-10.5608098580001,12.2,0.176035227999982));
#262085=CARTESIAN_POINT('Ctrl Pts',(-10.5588948570001,12.2,0.175600368999986));
#262086=CARTESIAN_POINT('Ctrl Pts',(-10.5569864130001,12.2,0.175168818999989));
#262087=CARTESIAN_POINT('Ctrl Pts',(-10.5550845460001,12.2,0.174740567999985));
#262088=CARTESIAN_POINT('Ctrl Pts',(-10.5531892730001,12.2,0.174315608999986));
#262089=CARTESIAN_POINT('Ctrl Pts',(-10.5513006120001,12.2,0.173893933999985));
#262090=CARTESIAN_POINT('Ctrl Pts',(-10.5494185790001,12.2,0.173475535999987));
#262091=CARTESIAN_POINT('Ctrl Pts',(-10.5475431950001,12.2,0.173060405999985));
#262092=CARTESIAN_POINT('Ctrl Pts',(-10.5456744770001,12.2,0.172648534999986));
#262093=CARTESIAN_POINT('Ctrl Pts',(-10.5438124430001,12.2,0.172239915999985));
#262094=CARTESIAN_POINT('Ctrl Pts',(-10.5419571120001,12.2,0.171834540999987));
#262095=CARTESIAN_POINT('Ctrl Pts',(-10.5401085000001,12.2,0.171432399999984));
#262096=CARTESIAN_POINT('Ctrl Pts',(-10.5382666270001,12.2,0.171033485999987));
#262097=CARTESIAN_POINT('Ctrl Pts',(-10.5364315110001,12.2,0.170637790999986));
#262098=CARTESIAN_POINT('Ctrl Pts',(-10.5346031720001,12.2,0.170245304999987));
#262099=CARTESIAN_POINT('Ctrl Pts',(-10.5327816250001,12.2,0.169856020999983));
#262100=CARTESIAN_POINT('Ctrl Pts',(-10.5309668930001,12.2,0.169469929999986));
#262101=CARTESIAN_POINT('Ctrl Pts',(-10.5291589900001,12.2,0.169087022999985));
#262102=CARTESIAN_POINT('Ctrl Pts',(-10.5273579390001,12.2,0.168707291999985));
#262103=CARTESIAN_POINT('Ctrl Pts',(-10.5255637550001,12.2,0.168330728999986));
#262104=CARTESIAN_POINT('Ctrl Pts',(-10.5237764590001,12.2,0.167957323999985));
#262105=CARTESIAN_POINT('Ctrl Pts',(-10.5219960680001,12.2,0.167587068999988));
#262106=CARTESIAN_POINT('Ctrl Pts',(-10.5202226040001,12.2,0.167219955999984));
#262107=CARTESIAN_POINT('Ctrl Pts',(-10.5184560840001,12.2,0.166855974999987));
#262108=CARTESIAN_POINT('Ctrl Pts',(-10.5166965270001,12.2,0.166495116999985));
#262109=CARTESIAN_POINT('Ctrl Pts',(-10.5149439520001,12.2,0.166137374999984));
#262110=CARTESIAN_POINT('Ctrl Pts',(-10.5131983790001,12.2,0.165782736999986));
#262111=CARTESIAN_POINT('Ctrl Pts',(-10.5114598270001,12.2,0.165431196999983));
#262112=CARTESIAN_POINT('Ctrl Pts',(-10.5097283150001,12.2,0.165082744999987));
#262113=CARTESIAN_POINT('Ctrl Pts',(-10.5080038620001,12.2,0.164737371999983));
#262114=CARTESIAN_POINT('Ctrl Pts',(-10.5062864880001,12.2,0.164395067999985));
#262115=CARTESIAN_POINT('Ctrl Pts',(-10.5045762130001,12.2,0.164055823999987));
#262116=CARTESIAN_POINT('Ctrl Pts',(-10.5028730550001,12.2,0.163719632999988));
#262117=CARTESIAN_POINT('Ctrl Pts',(-10.5011770350001,12.2,0.163386482999983));
#262118=CARTESIAN_POINT('Ctrl Pts',(-10.4994881720001,12.2,0.163056365999985));
#262119=CARTESIAN_POINT('Ctrl Pts',(-10.4978064870001,12.2,0.162729272999984));
#262120=CARTESIAN_POINT('Ctrl Pts',(-10.4961320000001,12.2,0.162405193999984));
#262121=CARTESIAN_POINT('Ctrl Pts',(-10.4944647280001,12.2,0.162084120999988));
#262122=CARTESIAN_POINT('Ctrl Pts',(-10.4928046930001,12.2,0.161766040999982));
#262123=CARTESIAN_POINT('Ctrl Pts',(-10.4911519150001,12.2,0.161450947999988));
#262124=CARTESIAN_POINT('Ctrl Pts',(-10.4895064150001,12.2,0.161138831999987));
#262125=CARTESIAN_POINT('Ctrl Pts',(-10.4878682100001,12.2,0.160829682999988));
#262126=CARTESIAN_POINT('Ctrl Pts',(-10.4862373250001,12.2,0.160523489999989));
#262127=CARTESIAN_POINT('Ctrl Pts',(-10.4846137770001,12.2,0.160220243999984));
#262128=CARTESIAN_POINT('Ctrl Pts',(-10.4829975860001,12.2,0.159919936999984));
#262129=CARTESIAN_POINT('Ctrl Pts',(-10.4813887750001,12.2,0.159622555999985));
#262130=CARTESIAN_POINT('Ctrl Pts',(-10.4797873630001,12.2,0.159328093999989));
#262131=CARTESIAN_POINT('Ctrl Pts',(-10.4781933710001,12.2,0.159036539999988));
#262132=CARTESIAN_POINT('Ctrl Pts',(-10.4766068200001,12.2,0.158747883999983));
#262133=CARTESIAN_POINT('Ctrl Pts',(-10.4750277290001,12.2,0.158462115999987));
#262134=CARTESIAN_POINT('Ctrl Pts',(-10.4734561210001,12.2,0.158179226999984));
#262135=CARTESIAN_POINT('Ctrl Pts',(-10.4718920160001,12.2,0.157899203999987));
#262136=CARTESIAN_POINT('Ctrl Pts',(-10.4703354350001,12.2,0.157622039999987));
#262137=CARTESIAN_POINT('Ctrl Pts',(-10.4687864010001,12.2,0.157347723999983));
#262138=CARTESIAN_POINT('Ctrl Pts',(-10.4672449310001,12.2,0.157076244999987));
#262139=CARTESIAN_POINT('Ctrl Pts',(-10.4657110500001,12.2,0.156807592999986));
#262140=CARTESIAN_POINT('Ctrl Pts',(-10.4641847780001,12.2,0.156541757999986));
#262141=CARTESIAN_POINT('Ctrl Pts',(-10.4626661360001,12.2,0.156278728999983));
#262142=CARTESIAN_POINT('Ctrl Pts',(-10.4611551460001,12.2,0.156018495999986));
#262143=CARTESIAN_POINT('Ctrl Pts',(-10.4596518290001,12.2,0.155761047999987));
#262144=CARTESIAN_POINT('Ctrl Pts',(-10.4581562070001,12.2,0.155506375999988));
#262145=CARTESIAN_POINT('Ctrl Pts',(-10.4566683020001,12.2,0.155254465999985));
#262146=CARTESIAN_POINT('Ctrl Pts',(-10.4551881360001,12.2,0.155005310999985));
#262147=CARTESIAN_POINT('Ctrl Pts',(-10.4537157300001,12.2,0.154758897999985));
#262148=CARTESIAN_POINT('Ctrl Pts',(-10.4522511070001,12.2,0.154515216999984));
#262149=CARTESIAN_POINT('Ctrl Pts',(-10.4507942880001,12.2,0.154274255999987));
#262150=CARTESIAN_POINT('Ctrl Pts',(-10.4493452950001,12.2,0.154036006999987));
#262151=CARTESIAN_POINT('Ctrl Pts',(-10.4479041520001,12.2,0.153800454999988));
#262152=CARTESIAN_POINT('Ctrl Pts',(-10.4464708800001,12.2,0.153567592999986));
#262153=CARTESIAN_POINT('Ctrl Pts',(-10.4450455010001,12.2,0.153337406999987));
#262154=CARTESIAN_POINT('Ctrl Pts',(-10.4436280380001,12.2,0.153109886999987));
#262155=CARTESIAN_POINT('Ctrl Pts',(-10.4422185140001,12.2,0.152885022999989));
#262156=CARTESIAN_POINT('Ctrl Pts',(-10.4408169510001,12.2,0.152662800999988));
#262157=CARTESIAN_POINT('Ctrl Pts',(-10.4394233720001,12.2,0.152443211999986));
#262158=CARTESIAN_POINT('Ctrl Pts',(-10.4380378000001,12.2,0.152226242999984));
#262159=CARTESIAN_POINT('Ctrl Pts',(-10.4366602580001,12.2,0.152011882999985));
#262160=CARTESIAN_POINT('Ctrl Pts',(-10.4352907680001,12.2,0.151800122999983));
#262161=CARTESIAN_POINT('Ctrl Pts',(-10.4339293550001,12.2,0.151590946999987));
#262162=CARTESIAN_POINT('Ctrl Pts',(-10.4325760410001,12.2,0.151384346999985));
#262163=CARTESIAN_POINT('Ctrl Pts',(-10.4312308480001,12.2,0.151180308999983));
#262164=CARTESIAN_POINT('Ctrl Pts',(-10.4298938030001,12.2,0.150978822999988));
#262165=CARTESIAN_POINT('Ctrl Pts',(-10.4285649260001,12.2,0.150779875999985));
#262166=CARTESIAN_POINT('Ctrl Pts',(-10.4272442410001,12.2,0.150583456999982));
#262167=CARTESIAN_POINT('Ctrl Pts',(-10.4259317730001,12.2,0.150389553999983));
#262168=CARTESIAN_POINT('Ctrl Pts',(-10.4246275460001,12.2,0.150198153999987));
#262169=CARTESIAN_POINT('Ctrl Pts',(-10.4233315830001,12.2,0.150009245999985));
#262170=CARTESIAN_POINT('Ctrl Pts',(-10.4220439070001,12.2,0.149822816999983));
#262171=CARTESIAN_POINT('Ctrl Pts',(-10.4207645450001,12.2,0.149638854999985));
#262172=CARTESIAN_POINT('Ctrl Pts',(-10.4194935180001,12.2,0.149457348999986));
#262173=CARTESIAN_POINT('Ctrl Pts',(-10.4182308520001,12.2,0.149278284999985));
#262174=CARTESIAN_POINT('Ctrl Pts',(-10.4169765720001,12.2,0.149101651999985));
#262175=CARTESIAN_POINT('Ctrl Pts',(-10.4157307010001,12.2,0.148927436999986));
#262176=CARTESIAN_POINT('Ctrl Pts',(-10.4144932620001,12.2,0.148755626999986));
#262177=CARTESIAN_POINT('Ctrl Pts',(-10.4132642840001,12.2,0.148586209999984));
#262178=CARTESIAN_POINT('Ctrl Pts',(-10.4120437890001,12.2,0.148419172999983));
#262179=CARTESIAN_POINT('Ctrl Pts',(-10.4108318020001,12.2,0.148254502999983));
#262180=CARTESIAN_POINT('Ctrl Pts',(-10.4096283490001,12.2,0.148092186999986));
#262181=CARTESIAN_POINT('Ctrl Pts',(-10.4084334530001,12.2,0.147932213999984));
#262182=CARTESIAN_POINT('Ctrl Pts',(-10.4072471420001,12.2,0.147774568999988));
#262183=CARTESIAN_POINT('Ctrl Pts',(-10.4060694410001,12.2,0.147619239999983));
#262184=CARTESIAN_POINT('Ctrl Pts',(-10.4049003720001,12.2,0.147466213999987));
#262185=CARTESIAN_POINT('Ctrl Pts',(-10.4037399650001,12.2,0.147315476999985));
#262186=CARTESIAN_POINT('Ctrl Pts',(-10.4025882420001,12.2,0.147167016999985));
#262187=CARTESIAN_POINT('Ctrl Pts',(-10.4014452320001,12.2,0.147020818999986));
#262188=CARTESIAN_POINT('Ctrl Pts',(-10.4003109570001,12.2,0.146876870999986));
#262189=CARTESIAN_POINT('Ctrl Pts',(-10.3991854470001,12.2,0.146735159999984));
#262190=CARTESIAN_POINT('Ctrl Pts',(-10.3980687260001,12.2,0.146595670999985));
#262191=CARTESIAN_POINT('Ctrl Pts',(-10.3969608200001,12.2,0.146458390999986));
#262192=CARTESIAN_POINT('Ctrl Pts',(-10.3958617570001,12.2,0.146323306999987));
#262193=CARTESIAN_POINT('Ctrl Pts',(-10.3947715610001,12.2,0.146190402999986));
#262194=CARTESIAN_POINT('Ctrl Pts',(-10.3936902610001,12.2,0.146059668999987));
#262195=CARTESIAN_POINT('Ctrl Pts',(-10.3926178820001,12.2,0.145931086999984));
#262196=CARTESIAN_POINT('Ctrl Pts',(-10.3915544510001,12.2,0.145804645999985));
#262197=CARTESIAN_POINT('Ctrl Pts',(-10.3904999960001,12.2,0.145680330999984));
#262198=CARTESIAN_POINT('Ctrl Pts',(-10.3894545430001,12.2,0.145558126999985));
#262199=CARTESIAN_POINT('Ctrl Pts',(-10.3884181200001,12.2,0.145438019999986));
#262200=CARTESIAN_POINT('Ctrl Pts',(-10.3873907530001,12.2,0.145319995999986));
#262201=CARTESIAN_POINT('Ctrl Pts',(-10.3863724700001,12.2,0.145204041999989));
#262202=CARTESIAN_POINT('Ctrl Pts',(-10.3853633010001,12.2,0.145090140999984));
#262203=CARTESIAN_POINT('Ctrl Pts',(-10.3843632700001,12.2,0.144978280999983));
#262204=CARTESIAN_POINT('Ctrl Pts',(-10.3833724070001,12.2,0.144868444999986));
#262205=CARTESIAN_POINT('Ctrl Pts',(-10.3823907380001,12.2,0.144760619999986));
#262206=CARTESIAN_POINT('Ctrl Pts',(-10.3814182930001,12.2,0.144654789999983));
#262207=CARTESIAN_POINT('Ctrl Pts',(-10.3804551000001,12.2,0.144550940999988));
#262208=CARTESIAN_POINT('Ctrl Pts',(-10.3795011870001,12.2,0.144449057999987));
#262209=CARTESIAN_POINT('Ctrl Pts',(-10.3785565820001,12.2,0.144349124999987));
#262210=CARTESIAN_POINT('Ctrl Pts',(-10.3776213140001,12.2,0.144251127999984));
#262211=CARTESIAN_POINT('Ctrl Pts',(-10.3766954110001,12.2,0.144155049999988));
#262212=CARTESIAN_POINT('Ctrl Pts',(-10.3757841820001,12.2,0.144061419999986));
#262213=CARTESIAN_POINT('Ctrl Pts',(-10.3750636860001,12.2,0.143988113999987));
#262214=CARTESIAN_POINT('Ctrl Pts',(-10.3745287910001,12.2,0.143934095999985));
#262215=CARTESIAN_POINT('Ctrl Pts',(-10.3741757630001,12.2,0.143898618999985));
#262216=CARTESIAN_POINT('Ctrl Pts',(-10.3740022750001,12.2,0.143881226999985));
#262217=CARTESIAN_POINT('Ctrl Pts',(-10.3740022750001,15.2,0.143881226999985));
#262218=CARTESIAN_POINT('Ctrl Pts',(-10.3741757630001,15.2,0.143898618999985));
#262219=CARTESIAN_POINT('Ctrl Pts',(-10.3745287910001,15.2,0.143934095999985));
#262220=CARTESIAN_POINT('Ctrl Pts',(-10.3750636860001,15.2,0.143988113999987));
#262221=CARTESIAN_POINT('Ctrl Pts',(-10.3757841820001,15.2,0.144061419999986));
#262222=CARTESIAN_POINT('Ctrl Pts',(-10.3766954110001,15.2,0.144155049999988));
#262223=CARTESIAN_POINT('Ctrl Pts',(-10.3776213140001,15.2,0.144251127999984));
#262224=CARTESIAN_POINT('Ctrl Pts',(-10.3785565820001,15.2,0.144349124999987));
#262225=CARTESIAN_POINT('Ctrl Pts',(-10.3795011870001,15.2,0.144449057999987));
#262226=CARTESIAN_POINT('Ctrl Pts',(-10.3804551000001,15.2,0.144550940999988));
#262227=CARTESIAN_POINT('Ctrl Pts',(-10.3814182930001,15.2,0.144654789999983));
#262228=CARTESIAN_POINT('Ctrl Pts',(-10.3823907380001,15.2,0.144760619999986));
#262229=CARTESIAN_POINT('Ctrl Pts',(-10.3833724070001,15.2,0.144868444999986));
#262230=CARTESIAN_POINT('Ctrl Pts',(-10.3843632700001,15.2,0.144978280999983));
#262231=CARTESIAN_POINT('Ctrl Pts',(-10.3853633010001,15.2,0.145090140999984));
#262232=CARTESIAN_POINT('Ctrl Pts',(-10.3863724700001,15.2,0.145204041999989));
#262233=CARTESIAN_POINT('Ctrl Pts',(-10.3873907530001,15.2,0.145319995999986));
#262234=CARTESIAN_POINT('Ctrl Pts',(-10.3884181200001,15.2,0.145438019999986));
#262235=CARTESIAN_POINT('Ctrl Pts',(-10.3894545430001,15.2,0.145558126999985));
#262236=CARTESIAN_POINT('Ctrl Pts',(-10.3904999960001,15.2,0.145680330999984));
#262237=CARTESIAN_POINT('Ctrl Pts',(-10.3915544510001,15.2,0.145804645999985));
#262238=CARTESIAN_POINT('Ctrl Pts',(-10.3926178820001,15.2,0.145931086999984));
#262239=CARTESIAN_POINT('Ctrl Pts',(-10.3936902610001,15.2,0.146059668999987));
#262240=CARTESIAN_POINT('Ctrl Pts',(-10.3947715610001,15.2,0.146190402999986));
#262241=CARTESIAN_POINT('Ctrl Pts',(-10.3958617570001,15.2,0.146323306999987));
#262242=CARTESIAN_POINT('Ctrl Pts',(-10.3969608200001,15.2,0.146458390999986));
#262243=CARTESIAN_POINT('Ctrl Pts',(-10.3980687260001,15.2,0.146595670999985));
#262244=CARTESIAN_POINT('Ctrl Pts',(-10.3991854470001,15.2,0.146735159999984));
#262245=CARTESIAN_POINT('Ctrl Pts',(-10.4003109570001,15.2,0.146876870999986));
#262246=CARTESIAN_POINT('Ctrl Pts',(-10.4014452320001,15.2,0.147020818999986));
#262247=CARTESIAN_POINT('Ctrl Pts',(-10.4025882420001,15.2,0.147167016999985));
#262248=CARTESIAN_POINT('Ctrl Pts',(-10.4037399650001,15.2,0.147315476999985));
#262249=CARTESIAN_POINT('Ctrl Pts',(-10.4049003720001,15.2,0.147466213999987));
#262250=CARTESIAN_POINT('Ctrl Pts',(-10.4060694410001,15.2,0.147619239999983));
#262251=CARTESIAN_POINT('Ctrl Pts',(-10.4072471420001,15.2,0.147774568999988));
#262252=CARTESIAN_POINT('Ctrl Pts',(-10.4084334530001,15.2,0.147932213999984));
#262253=CARTESIAN_POINT('Ctrl Pts',(-10.4096283490001,15.2,0.148092186999986));
#262254=CARTESIAN_POINT('Ctrl Pts',(-10.4108318020001,15.2,0.148254502999983));
#262255=CARTESIAN_POINT('Ctrl Pts',(-10.4120437890001,15.2,0.148419172999983));
#262256=CARTESIAN_POINT('Ctrl Pts',(-10.4132642840001,15.2,0.148586209999984));
#262257=CARTESIAN_POINT('Ctrl Pts',(-10.4144932620001,15.2,0.148755626999986));
#262258=CARTESIAN_POINT('Ctrl Pts',(-10.4157307010001,15.2,0.148927436999986));
#262259=CARTESIAN_POINT('Ctrl Pts',(-10.4169765720001,15.2,0.149101651999985));
#262260=CARTESIAN_POINT('Ctrl Pts',(-10.4182308520001,15.2,0.149278284999985));
#262261=CARTESIAN_POINT('Ctrl Pts',(-10.4194935180001,15.2,0.149457348999986));
#262262=CARTESIAN_POINT('Ctrl Pts',(-10.4207645450001,15.2,0.149638854999985));
#262263=CARTESIAN_POINT('Ctrl Pts',(-10.4220439070001,15.2,0.149822816999983));
#262264=CARTESIAN_POINT('Ctrl Pts',(-10.4233315830001,15.2,0.150009245999985));
#262265=CARTESIAN_POINT('Ctrl Pts',(-10.4246275460001,15.2,0.150198153999987));
#262266=CARTESIAN_POINT('Ctrl Pts',(-10.4259317730001,15.2,0.150389553999983));
#262267=CARTESIAN_POINT('Ctrl Pts',(-10.4272442410001,15.2,0.150583456999982));
#262268=CARTESIAN_POINT('Ctrl Pts',(-10.4285649260001,15.2,0.150779875999985));
#262269=CARTESIAN_POINT('Ctrl Pts',(-10.4298938030001,15.2,0.150978822999988));
#262270=CARTESIAN_POINT('Ctrl Pts',(-10.4312308480001,15.2,0.151180308999983));
#262271=CARTESIAN_POINT('Ctrl Pts',(-10.4325760410001,15.2,0.151384346999985));
#262272=CARTESIAN_POINT('Ctrl Pts',(-10.4339293550001,15.2,0.151590946999987));
#262273=CARTESIAN_POINT('Ctrl Pts',(-10.4352907680001,15.2,0.151800122999983));
#262274=CARTESIAN_POINT('Ctrl Pts',(-10.4366602580001,15.2,0.152011882999985));
#262275=CARTESIAN_POINT('Ctrl Pts',(-10.4380378000001,15.2,0.152226242999984));
#262276=CARTESIAN_POINT('Ctrl Pts',(-10.4394233720001,15.2,0.152443211999986));
#262277=CARTESIAN_POINT('Ctrl Pts',(-10.4408169510001,15.2,0.152662800999988));
#262278=CARTESIAN_POINT('Ctrl Pts',(-10.4422185140001,15.2,0.152885022999989));
#262279=CARTESIAN_POINT('Ctrl Pts',(-10.4436280380001,15.2,0.153109886999987));
#262280=CARTESIAN_POINT('Ctrl Pts',(-10.4450455010001,15.2,0.153337406999987));
#262281=CARTESIAN_POINT('Ctrl Pts',(-10.4464708800001,15.2,0.153567592999986));
#262282=CARTESIAN_POINT('Ctrl Pts',(-10.4479041520001,15.2,0.153800454999988));
#262283=CARTESIAN_POINT('Ctrl Pts',(-10.4493452950001,15.2,0.154036006999987));
#262284=CARTESIAN_POINT('Ctrl Pts',(-10.4507942880001,15.2,0.154274255999987));
#262285=CARTESIAN_POINT('Ctrl Pts',(-10.4522511070001,15.2,0.154515216999984));
#262286=CARTESIAN_POINT('Ctrl Pts',(-10.4537157300001,15.2,0.154758897999985));
#262287=CARTESIAN_POINT('Ctrl Pts',(-10.4551881360001,15.2,0.155005310999985));
#262288=CARTESIAN_POINT('Ctrl Pts',(-10.4566683020001,15.2,0.155254465999985));
#262289=CARTESIAN_POINT('Ctrl Pts',(-10.4581562070001,15.2,0.155506375999988));
#262290=CARTESIAN_POINT('Ctrl Pts',(-10.4596518290001,15.2,0.155761047999987));
#262291=CARTESIAN_POINT('Ctrl Pts',(-10.4611551460001,15.2,0.156018495999986));
#262292=CARTESIAN_POINT('Ctrl Pts',(-10.4626661360001,15.2,0.156278728999983));
#262293=CARTESIAN_POINT('Ctrl Pts',(-10.4641847780001,15.2,0.156541757999986));
#262294=CARTESIAN_POINT('Ctrl Pts',(-10.4657110500001,15.2,0.156807592999986));
#262295=CARTESIAN_POINT('Ctrl Pts',(-10.4672449310001,15.2,0.157076244999987));
#262296=CARTESIAN_POINT('Ctrl Pts',(-10.4687864010001,15.2,0.157347723999983));
#262297=CARTESIAN_POINT('Ctrl Pts',(-10.4703354350001,15.2,0.157622039999987));
#262298=CARTESIAN_POINT('Ctrl Pts',(-10.4718920160001,15.2,0.157899203999987));
#262299=CARTESIAN_POINT('Ctrl Pts',(-10.4734561210001,15.2,0.158179226999984));
#262300=CARTESIAN_POINT('Ctrl Pts',(-10.4750277290001,15.2,0.158462115999987));
#262301=CARTESIAN_POINT('Ctrl Pts',(-10.4766068200001,15.2,0.158747883999983));
#262302=CARTESIAN_POINT('Ctrl Pts',(-10.4781933710001,15.2,0.159036539999988));
#262303=CARTESIAN_POINT('Ctrl Pts',(-10.4797873630001,15.2,0.159328093999989));
#262304=CARTESIAN_POINT('Ctrl Pts',(-10.4813887750001,15.2,0.159622555999985));
#262305=CARTESIAN_POINT('Ctrl Pts',(-10.4829975860001,15.2,0.159919936999984));
#262306=CARTESIAN_POINT('Ctrl Pts',(-10.4846137770001,15.2,0.160220243999984));
#262307=CARTESIAN_POINT('Ctrl Pts',(-10.4862373250001,15.2,0.160523489999989));
#262308=CARTESIAN_POINT('Ctrl Pts',(-10.4878682100001,15.2,0.160829682999988));
#262309=CARTESIAN_POINT('Ctrl Pts',(-10.4895064150001,15.2,0.161138831999987));
#262310=CARTESIAN_POINT('Ctrl Pts',(-10.4911519150001,15.2,0.161450947999988));
#262311=CARTESIAN_POINT('Ctrl Pts',(-10.4928046930001,15.2,0.161766040999982));
#262312=CARTESIAN_POINT('Ctrl Pts',(-10.4944647280001,15.2,0.162084120999988));
#262313=CARTESIAN_POINT('Ctrl Pts',(-10.4961320000001,15.2,0.162405193999984));
#262314=CARTESIAN_POINT('Ctrl Pts',(-10.4978064870001,15.2,0.162729272999984));
#262315=CARTESIAN_POINT('Ctrl Pts',(-10.4994881720001,15.2,0.163056365999985));
#262316=CARTESIAN_POINT('Ctrl Pts',(-10.5011770350001,15.2,0.163386482999983));
#262317=CARTESIAN_POINT('Ctrl Pts',(-10.5028730550001,15.2,0.163719632999988));
#262318=CARTESIAN_POINT('Ctrl Pts',(-10.5045762130001,15.2,0.164055823999987));
#262319=CARTESIAN_POINT('Ctrl Pts',(-10.5062864880001,15.2,0.164395067999985));
#262320=CARTESIAN_POINT('Ctrl Pts',(-10.5080038620001,15.2,0.164737371999983));
#262321=CARTESIAN_POINT('Ctrl Pts',(-10.5097283150001,15.2,0.165082744999987));
#262322=CARTESIAN_POINT('Ctrl Pts',(-10.5114598270001,15.2,0.165431196999983));
#262323=CARTESIAN_POINT('Ctrl Pts',(-10.5131983790001,15.2,0.165782736999986));
#262324=CARTESIAN_POINT('Ctrl Pts',(-10.5149439520001,15.2,0.166137374999984));
#262325=CARTESIAN_POINT('Ctrl Pts',(-10.5166965270001,15.2,0.166495116999985));
#262326=CARTESIAN_POINT('Ctrl Pts',(-10.5184560840001,15.2,0.166855974999987));
#262327=CARTESIAN_POINT('Ctrl Pts',(-10.5202226040001,15.2,0.167219955999984));
#262328=CARTESIAN_POINT('Ctrl Pts',(-10.5219960680001,15.2,0.167587068999988));
#262329=CARTESIAN_POINT('Ctrl Pts',(-10.5237764590001,15.2,0.167957323999985));
#262330=CARTESIAN_POINT('Ctrl Pts',(-10.5255637550001,15.2,0.168330728999986));
#262331=CARTESIAN_POINT('Ctrl Pts',(-10.5273579390001,15.2,0.168707291999985));
#262332=CARTESIAN_POINT('Ctrl Pts',(-10.5291589900001,15.2,0.169087022999985));
#262333=CARTESIAN_POINT('Ctrl Pts',(-10.5309668930001,15.2,0.169469929999986));
#262334=CARTESIAN_POINT('Ctrl Pts',(-10.5327816250001,15.2,0.169856020999983));
#262335=CARTESIAN_POINT('Ctrl Pts',(-10.5346031720001,15.2,0.170245304999987));
#262336=CARTESIAN_POINT('Ctrl Pts',(-10.5364315110001,15.2,0.170637790999986));
#262337=CARTESIAN_POINT('Ctrl Pts',(-10.5382666270001,15.2,0.171033485999987));
#262338=CARTESIAN_POINT('Ctrl Pts',(-10.5401085000001,15.2,0.171432399999984));
#262339=CARTESIAN_POINT('Ctrl Pts',(-10.5419571120001,15.2,0.171834540999987));
#262340=CARTESIAN_POINT('Ctrl Pts',(-10.5438124430001,15.2,0.172239915999985));
#262341=CARTESIAN_POINT('Ctrl Pts',(-10.5456744770001,15.2,0.172648534999986));
#262342=CARTESIAN_POINT('Ctrl Pts',(-10.5475431950001,15.2,0.173060405999985));
#262343=CARTESIAN_POINT('Ctrl Pts',(-10.5494185790001,15.2,0.173475535999987));
#262344=CARTESIAN_POINT('Ctrl Pts',(-10.5513006120001,15.2,0.173893933999985));
#262345=CARTESIAN_POINT('Ctrl Pts',(-10.5531892730001,15.2,0.174315608999986));
#262346=CARTESIAN_POINT('Ctrl Pts',(-10.5550845460001,15.2,0.174740567999985));
#262347=CARTESIAN_POINT('Ctrl Pts',(-10.5569864130001,15.2,0.175168818999989));
#262348=CARTESIAN_POINT('Ctrl Pts',(-10.5588948570001,15.2,0.175600368999986));
#262349=CARTESIAN_POINT('Ctrl Pts',(-10.5608098580001,15.2,0.176035227999982));
#262350=CARTESIAN_POINT('Ctrl Pts',(-10.5627314000001,15.2,0.176473403999986));
#262351=CARTESIAN_POINT('Ctrl Pts',(-10.5646594650001,15.2,0.176914901999985));
#262352=CARTESIAN_POINT('Ctrl Pts',(-10.5665940340001,15.2,0.177359733999989));
#262353=CARTESIAN_POINT('Ctrl Pts',(-10.5685350920001,15.2,0.177807903999985));
#262354=CARTESIAN_POINT('Ctrl Pts',(-10.5704826190001,15.2,0.178259422999982));
#262355=CARTESIAN_POINT('Ctrl Pts',(-10.5724365990001,15.2,0.178714295999987));
#262356=CARTESIAN_POINT('Ctrl Pts',(-10.5743970150001,15.2,0.179172532999985));
#262357=CARTESIAN_POINT('Ctrl Pts',(-10.5763638480001,15.2,0.179634139999987));
#262358=CARTESIAN_POINT('Ctrl Pts',(-10.5783370810001,15.2,0.180099124999984));
#262359=CARTESIAN_POINT('Ctrl Pts',(-10.5803166980001,15.2,0.180567494999986));
#262360=CARTESIAN_POINT('Ctrl Pts',(-10.5823026810001,15.2,0.181039259999984));
#262361=CARTESIAN_POINT('Ctrl Pts',(-10.5842950130001,15.2,0.181514424999989));
#262362=CARTESIAN_POINT('Ctrl Pts',(-10.5862936760001,15.2,0.181992998999987));
#262363=CARTESIAN_POINT('Ctrl Pts',(-10.5882986550001,15.2,0.182474987999988));
#262364=CARTESIAN_POINT('Ctrl Pts',(-10.5903099300001,15.2,0.182960399999987));
#262365=CARTESIAN_POINT('Ctrl Pts',(-10.5923274870001,15.2,0.183449243999987));
#262366=CARTESIAN_POINT('Ctrl Pts',(-10.5943513080001,15.2,0.183941525999987));
#262367=CARTESIAN_POINT('Ctrl Pts',(-10.5963813760001,15.2,0.184437252999987));
#262368=CARTESIAN_POINT('Ctrl Pts',(-10.5984176730001,15.2,0.184936432999985));
#262369=CARTESIAN_POINT('Ctrl Pts',(-10.6004601840001,15.2,0.185439070999984));
#262370=CARTESIAN_POINT('Ctrl Pts',(-10.6025088930001,15.2,0.185945177999987));
#262371=CARTESIAN_POINT('Ctrl Pts',(-10.6045637800001,15.2,0.186454757999983));
#262372=CARTESIAN_POINT('Ctrl Pts',(-10.6066248330001,15.2,0.186967819999988));
#262373=CARTESIAN_POINT('Ctrl Pts',(-10.6086920310001,15.2,0.187484370999984));
#262374=CARTESIAN_POINT('Ctrl Pts',(-10.6107653600001,15.2,0.188004416999985));
#262375=CARTESIAN_POINT('Ctrl Pts',(-10.6128448030001,15.2,0.188527964999987));
#262376=CARTESIAN_POINT('Ctrl Pts',(-10.6149303440001,15.2,0.189055023999987));
#262377=CARTESIAN_POINT('Ctrl Pts',(-10.6170219660001,15.2,0.189585598999984));
#262378=CARTESIAN_POINT('Ctrl Pts',(-10.6191196530001,15.2,0.190119695999984));
#262379=CARTESIAN_POINT('Ctrl Pts',(-10.6212233880001,15.2,0.190657325999983));
#262380=CARTESIAN_POINT('Ctrl Pts',(-10.6233331560001,15.2,0.191198491999987));
#262381=CARTESIAN_POINT('Ctrl Pts',(-10.6254489400001,15.2,0.191743201999985));
#262382=CARTESIAN_POINT('Ctrl Pts',(-10.6275707240001,15.2,0.192291463999985));
#262383=CARTESIAN_POINT('Ctrl Pts',(-10.6296984920001,15.2,0.192843283999986));
#262384=CARTESIAN_POINT('Ctrl Pts',(-10.6318322290001,15.2,0.193398666999984));
#262385=CARTESIAN_POINT('Ctrl Pts',(-10.6339719170001,15.2,0.193957621999985));
#262386=CARTESIAN_POINT('Ctrl Pts',(-10.6361175410001,15.2,0.194520154999989));
#262387=CARTESIAN_POINT('Ctrl Pts',(-10.6382690860001,15.2,0.195086272999987));
#262388=CARTESIAN_POINT('Ctrl Pts',(-10.6404265340001,15.2,0.195655982999985));
#262389=CARTESIAN_POINT('Ctrl Pts',(-10.6425898720001,15.2,0.196229288999987));
#262390=CARTESIAN_POINT('Ctrl Pts',(-10.6447590820001,15.2,0.196806200999986));
#262391=CARTESIAN_POINT('Ctrl Pts',(-10.6469341480001,15.2,0.197386722999986));
#262392=CARTESIAN_POINT('Ctrl Pts',(-10.6491150560001,15.2,0.197970862999988));
#262393=CARTESIAN_POINT('Ctrl Pts',(-10.6513017900001,15.2,0.198558625999983));
#262394=CARTESIAN_POINT('Ctrl Pts',(-10.6534943330001,15.2,0.199150019999985));
#262395=CARTESIAN_POINT('Ctrl Pts',(-10.6556926720001,15.2,0.199745050999987));
#262396=CARTESIAN_POINT('Ctrl Pts',(-10.6578967890001,15.2,0.200343724999983));
#262397=CARTESIAN_POINT('Ctrl Pts',(-10.6601066700001,15.2,0.200946048999988));
#262398=CARTESIAN_POINT('Ctrl Pts',(-10.6623222980001,15.2,0.201552028999985));
#262399=CARTESIAN_POINT('Ctrl Pts',(-10.6645436590001,15.2,0.202161669999987));
#262400=CARTESIAN_POINT('Ctrl Pts',(-10.6667707370001,15.2,0.202774979999987));
#262401=CARTESIAN_POINT('Ctrl Pts',(-10.6690035190001,15.2,0.203391963999984));
#262402=CARTESIAN_POINT('Ctrl Pts',(-10.6712419860001,15.2,0.204012629999983));
#262403=CARTESIAN_POINT('Ctrl Pts',(-10.6734861240001,15.2,0.204636982999986));
#262404=CARTESIAN_POINT('Ctrl Pts',(-10.6757359200001,15.2,0.205265028999988));
#262405=CARTESIAN_POINT('Ctrl Pts',(-10.6779913570001,15.2,0.205896773999985));
#262406=CARTESIAN_POINT('Ctrl Pts',(-10.6802524190001,15.2,0.206532224999982));
#262407=CARTESIAN_POINT('Ctrl Pts',(-10.6825190920001,15.2,0.207171386999985));
#262408=CARTESIAN_POINT('Ctrl Pts',(-10.6847913630001,15.2,0.207814266999984));
#262409=CARTESIAN_POINT('Ctrl Pts',(-10.6870692130001,15.2,0.208460869999989));
#262410=CARTESIAN_POINT('Ctrl Pts',(-10.6893526300001,15.2,0.209111201999987));
#262411=CARTESIAN_POINT('Ctrl Pts',(-10.6916415980001,15.2,0.209765271999984));
#262412=CARTESIAN_POINT('Ctrl Pts',(-10.6939361020001,15.2,0.210423081999984));
#262413=CARTESIAN_POINT('Ctrl Pts',(-10.6962361280001,15.2,0.211084637999988));
#262414=CARTESIAN_POINT('Ctrl Pts',(-10.6985416600001,15.2,0.211749948999986));
#262415=CARTESIAN_POINT('Ctrl Pts',(-10.7008526850001,15.2,0.212419018999985));
#262416=CARTESIAN_POINT('Ctrl Pts',(-10.7031691860001,15.2,0.213091852999985));
#262417=CARTESIAN_POINT('Ctrl Pts',(-10.7054911500001,15.2,0.213768457999985));
#262418=CARTESIAN_POINT('Ctrl Pts',(-10.7078185620001,15.2,0.214448838999988));
#262419=CARTESIAN_POINT('Ctrl Pts',(-10.7101514080001,15.2,0.215133002999988));
#262420=CARTESIAN_POINT('Ctrl Pts',(-10.7124896730001,15.2,0.215820953999986));
#262421=CARTESIAN_POINT('Ctrl Pts',(-10.7148333410001,15.2,0.216512699999987));
#262422=CARTESIAN_POINT('Ctrl Pts',(-10.7171823990001,15.2,0.217208243999987));
#262423=CARTESIAN_POINT('Ctrl Pts',(-10.7195368330001,15.2,0.217907592999986));
#262424=CARTESIAN_POINT('Ctrl Pts',(-10.7218966280001,15.2,0.218610753999986));
#262425=CARTESIAN_POINT('Ctrl Pts',(-10.7242617690001,15.2,0.219317729999986));
#262426=CARTESIAN_POINT('Ctrl Pts',(-10.7266322420001,15.2,0.220028526999982));
#262427=CARTESIAN_POINT('Ctrl Pts',(-10.7290080330001,15.2,0.220743150999985));
#262428=CARTESIAN_POINT('Ctrl Pts',(-10.7313891280001,15.2,0.221461608999984));
#262429=CARTESIAN_POINT('Ctrl Pts',(-10.7337755120001,15.2,0.222183903999986));
#262430=CARTESIAN_POINT('Ctrl Pts',(-10.7361671710001,15.2,0.222910043999986));
#262431=CARTESIAN_POINT('Ctrl Pts',(-10.7385640920001,15.2,0.223640032999985));
#262432=CARTESIAN_POINT('Ctrl Pts',(-10.7409662590001,15.2,0.224373874999984));
#262433=CARTESIAN_POINT('Ctrl Pts',(-10.7433736600001,15.2,0.225111577999986));
#262434=CARTESIAN_POINT('Ctrl Pts',(-10.7457862770001,15.2,0.225853145999988));
#262435=CARTESIAN_POINT('Ctrl Pts',(-10.7482041010001,15.2,0.226598583999986));
#262436=CARTESIAN_POINT('Ctrl Pts',(-10.7506271160001,15.2,0.227347897999985));
#262437=CARTESIAN_POINT('Ctrl Pts',(-10.7530553070001,15.2,0.228101093999986));
#262438=CARTESIAN_POINT('Ctrl Pts',(-10.7554886610001,15.2,0.228858175999989));
#262439=CARTESIAN_POINT('Ctrl Pts',(-10.7579271630001,15.2,0.229619148999984));
#262440=CARTESIAN_POINT('Ctrl Pts',(-10.7603708020001,15.2,0.230384019999987));
#262441=CARTESIAN_POINT('Ctrl Pts',(-10.7628195610001,15.2,0.231152792999989));
#262442=CARTESIAN_POINT('Ctrl Pts',(-10.7652734280001,15.2,0.231925471999985));
#262443=CARTESIAN_POINT('Ctrl Pts',(-10.7677323890001,15.2,0.232702063999985));
#262444=CARTESIAN_POINT('Ctrl Pts',(-10.7701964290001,15.2,0.233482572999986));
#262445=CARTESIAN_POINT('Ctrl Pts',(-10.7726655360001,15.2,0.234267004999986));
#262446=CARTESIAN_POINT('Ctrl Pts',(-10.7751396960001,15.2,0.235055364999983));
#262447=CARTESIAN_POINT('Ctrl Pts',(-10.7776188950001,15.2,0.235847656999986));
#262448=CARTESIAN_POINT('Ctrl Pts',(-10.7801031190001,15.2,0.236643886999985));
#262449=CARTESIAN_POINT('Ctrl Pts',(-10.7825923560001,15.2,0.237444060999987));
#262450=CARTESIAN_POINT('Ctrl Pts',(-10.7850865910001,15.2,0.238248179999987));
#262451=CARTESIAN_POINT('Ctrl Pts',(-10.7875858100001,15.2,0.239056253999985));
#262452=CARTESIAN_POINT('Ctrl Pts',(-10.7900900010001,15.2,0.239868283999982));
#262453=CARTESIAN_POINT('Ctrl Pts',(-10.7925991510001,15.2,0.240684276999983));
#262454=CARTESIAN_POINT('Ctrl Pts',(-10.7951132440001,15.2,0.241504237999983));
#262455=CARTESIAN_POINT('Ctrl Pts',(-10.7976322700001,15.2,0.242328170999984));
#262456=CARTESIAN_POINT('Ctrl Pts',(-10.8001562130001,15.2,0.243156080999984));
#262457=CARTESIAN_POINT('Ctrl Pts',(-10.8026850610001,15.2,0.243987971999986));
#262458=CARTESIAN_POINT('Ctrl Pts',(-10.8052187990001,15.2,0.244823850999989));
#262459=CARTESIAN_POINT('Ctrl Pts',(-10.8077574170001,15.2,0.245663720999989));
#262460=CARTESIAN_POINT('Ctrl Pts',(-10.8103008990001,15.2,0.246507586999982));
#262461=CARTESIAN_POINT('Ctrl Pts',(-10.8128492330001,15.2,0.247355453999987));
#262462=CARTESIAN_POINT('Ctrl Pts',(-10.8154024050001,15.2,0.248207326999985));
#262463=CARTESIAN_POINT('Ctrl Pts',(-10.8179604030001,15.2,0.249063209999987));
#262464=CARTESIAN_POINT('Ctrl Pts',(-10.8205232130001,15.2,0.249923108999983));
#262465=CARTESIAN_POINT('Ctrl Pts',(-10.8230908230001,15.2,0.250787025999983));
#262466=CARTESIAN_POINT('Ctrl Pts',(-10.8256632200001,15.2,0.251654968999984));
#262467=CARTESIAN_POINT('Ctrl Pts',(-10.8282403890001,15.2,0.252526939999989));
#262468=CARTESIAN_POINT('Ctrl Pts',(-10.8308223180001,15.2,0.253402943999985));
#262469=CARTESIAN_POINT('Ctrl Pts',(-10.8334089940001,15.2,0.254282987999983));
#262470=CARTESIAN_POINT('Ctrl Pts',(-10.8360004070001,15.2,0.255167072999987));
#262471=CARTESIAN_POINT('Ctrl Pts',(-10.8385965390001,15.2,0.256055205999988));
#262472=CARTESIAN_POINT('Ctrl Pts',(-10.8411973810001,15.2,0.256947389999986));
#262473=CARTESIAN_POINT('Ctrl Pts',(-10.8438029180001,15.2,0.257843629999983));
#262474=CARTESIAN_POINT('Ctrl Pts',(-10.8464131390001,15.2,0.258743930999987));
#262475=CARTESIAN_POINT('Ctrl Pts',(-10.8490280300001,15.2,0.259648296999986));
#262476=CARTESIAN_POINT('Ctrl Pts',(-10.8516475780001,15.2,0.260556731999984));
#262477=CARTESIAN_POINT('Ctrl Pts',(-10.8542717720001,15.2,0.261469240999985));
#262478=CARTESIAN_POINT('Ctrl Pts',(-10.8569005980001,15.2,0.262385827999987));
#262479=CARTESIAN_POINT('Ctrl Pts',(-10.8595340430001,15.2,0.263306497999984));
#262480=CARTESIAN_POINT('Ctrl Pts',(-10.8621720950001,15.2,0.264231254999987));
#262481=CARTESIAN_POINT('Ctrl Pts',(-10.8648147410001,15.2,0.265160102999986));
#262482=CARTESIAN_POINT('Ctrl Pts',(-10.8674619700001,15.2,0.266093045999987));
#262483=CARTESIAN_POINT('Ctrl Pts',(-10.8701137680001,15.2,0.267030089999984));
#262484=CARTESIAN_POINT('Ctrl Pts',(-10.8727701220001,15.2,0.267971236999984));
#262485=CARTESIAN_POINT('Ctrl Pts',(-10.8754310200001,15.2,0.268916491999986));
#262486=CARTESIAN_POINT('Ctrl Pts',(-10.8780964490001,15.2,0.269865860999987));
#262487=CARTESIAN_POINT('Ctrl Pts',(-10.8807663990001,15.2,0.270819344999986));
#262488=CARTESIAN_POINT('Ctrl Pts',(-10.8834408550001,15.2,0.271776950999989));
#262489=CARTESIAN_POINT('Ctrl Pts',(-10.8861198050001,15.2,0.272738680999982));
#262490=CARTESIAN_POINT('Ctrl Pts',(-10.8888032380001,15.2,0.273704540999984));
#262491=CARTESIAN_POINT('Ctrl Pts',(-10.8914911410001,15.2,0.274674534999986));
#262492=CARTESIAN_POINT('Ctrl Pts',(-10.8941835000001,15.2,0.275648664999988));
#262493=CARTESIAN_POINT('Ctrl Pts',(-10.8968803070001,15.2,0.276626936999986));
#262494=CARTESIAN_POINT('Ctrl Pts',(-10.8995815450001,15.2,0.277609353999986));
#262495=CARTESIAN_POINT('Ctrl Pts',(-10.9022872040001,15.2,0.278595920999987));
#262496=CARTESIAN_POINT('Ctrl Pts',(-10.9049972710001,15.2,0.279586640999985));
#262497=CARTESIAN_POINT('Ctrl Pts',(-10.9077117350001,15.2,0.280581520999985));
#262498=CARTESIAN_POINT('Ctrl Pts',(-10.9104305830001,15.2,0.281580559999988));
#262499=CARTESIAN_POINT('Ctrl Pts',(-10.9131538030001,15.2,0.282583765999984));
#262500=CARTESIAN_POINT('Ctrl Pts',(-10.9158813840001,15.2,0.283591140999988));
#262501=CARTESIAN_POINT('Ctrl Pts',(-10.9186133120001,15.2,0.284602688999982));
#262502=CARTESIAN_POINT('Ctrl Pts',(-10.9213495760001,15.2,0.285618414999984));
#262503=CARTESIAN_POINT('Ctrl Pts',(-10.9240901640001,15.2,0.286638322999986));
#262504=CARTESIAN_POINT('Ctrl Pts',(-10.9268350640001,15.2,0.287662414999983));
#262505=CARTESIAN_POINT('Ctrl Pts',(-10.9295842640001,15.2,0.288690695999985));
#262506=CARTESIAN_POINT('Ctrl Pts',(-10.9323377520001,15.2,0.289723170999987));
#262507=CARTESIAN_POINT('Ctrl Pts',(-10.9350955160001,15.2,0.290759840999986));
#262508=CARTESIAN_POINT('Ctrl Pts',(-10.9378575430001,15.2,0.291800712999986));
#262509=CARTESIAN_POINT('Ctrl Pts',(-10.9406238230001,15.2,0.292845787999987));
#262510=CARTESIAN_POINT('Ctrl Pts',(-10.9433943440001,15.2,0.293895071999986));
#262511=CARTESIAN_POINT('Ctrl Pts',(-10.9461690940001,15.2,0.294948567999986));
#262512=CARTESIAN_POINT('Ctrl Pts',(-10.9489480600001,15.2,0.296006278999985));
#262513=CARTESIAN_POINT('Ctrl Pts',(-10.9517312310001,15.2,0.297068208999987));
#262514=CARTESIAN_POINT('Ctrl Pts',(-10.9545185950001,15.2,0.298134361999987));
#262515=CARTESIAN_POINT('Ctrl Pts',(-10.9573101410001,15.2,0.299204742999986));
#262516=CARTESIAN_POINT('Ctrl Pts',(-10.9601058580001,15.2,0.300279352999984));
#262517=CARTESIAN_POINT('Ctrl Pts',(-10.9629057310001,15.2,0.301358197999986));
#262518=CARTESIAN_POINT('Ctrl Pts',(-10.9657097520001,15.2,0.302441278999983));
#262519=CARTESIAN_POINT('Ctrl Pts',(-10.9685179070001,15.2,0.303528602999985));
#262520=CARTESIAN_POINT('Ctrl Pts',(-10.9713301870001,15.2,0.304620170999983));
#262521=CARTESIAN_POINT('Ctrl Pts',(-10.9741465770001,15.2,0.305715986999986));
#262522=CARTESIAN_POINT('Ctrl Pts',(-10.9769670670001,15.2,0.306816054999985));
#262523=CARTESIAN_POINT('Ctrl Pts',(-10.9797916470001,15.2,0.307920378999986));
#262524=CARTESIAN_POINT('Ctrl Pts',(-10.9826203020001,15.2,0.309028961999989));
#262525=CARTESIAN_POINT('Ctrl Pts',(-10.9854530250001,15.2,0.310141807999984));
#262526=CARTESIAN_POINT('Ctrl Pts',(-10.9882898000001,15.2,0.311258919999986));
#262527=CARTESIAN_POINT('Ctrl Pts',(-10.9911306190001,15.2,0.312380299999986));
#262528=CARTESIAN_POINT('Ctrl Pts',(-10.9939754690001,15.2,0.313505953999984));
#262529=CARTESIAN_POINT('Ctrl Pts',(-10.9968243390001,15.2,0.314635884999985));
#262530=CARTESIAN_POINT('Ctrl Pts',(-10.9996772170001,15.2,0.315770094999985));
#262531=CARTESIAN_POINT('Ctrl Pts',(-11.0025340930001,15.2,0.316908588999985));
#262532=CARTESIAN_POINT('Ctrl Pts',(-11.0053949540001,15.2,0.318051369999988));
#262533=CARTESIAN_POINT('Ctrl Pts',(-11.0082597890001,15.2,0.319198439999986));
#262534=CARTESIAN_POINT('Ctrl Pts',(-11.0111285880001,15.2,0.320349803999989));
#262535=CARTESIAN_POINT('Ctrl Pts',(-11.0140013380001,15.2,0.321505463999987));
#262536=CARTESIAN_POINT('Ctrl Pts',(-11.0168780300001,15.2,0.322665424999986));
#262537=CARTESIAN_POINT('Ctrl Pts',(-11.0197586510001,15.2,0.323829688999986));
#262538=CARTESIAN_POINT('Ctrl Pts',(-11.0226431890001,15.2,0.324998259999987));
#262539=CARTESIAN_POINT('Ctrl Pts',(-11.0255316350001,15.2,0.326171140999989));
#262540=CARTESIAN_POINT('Ctrl Pts',(-11.0284239770001,15.2,0.327348335999984));
#262541=CARTESIAN_POINT('Ctrl Pts',(-11.0313202040001,15.2,0.328529845999985));
#262542=CARTESIAN_POINT('Ctrl Pts',(-11.0342203030001,15.2,0.329715676999989));
#262543=CARTESIAN_POINT('Ctrl Pts',(-11.0371242670001,15.2,0.330905830999986));
#262544=CARTESIAN_POINT('Ctrl Pts',(-11.0400320810001,15.2,0.332100310999985));
#262545=CARTESIAN_POINT('Ctrl Pts',(-11.0429437360001,15.2,0.333299120999988));
#262546=CARTESIAN_POINT('Ctrl Pts',(-11.0458592200001,15.2,0.334502262999985));
#262547=CARTESIAN_POINT('Ctrl Pts',(-11.0487785220001,15.2,0.335709739999985));
#262548=CARTESIAN_POINT('Ctrl Pts',(-11.0517016320001,15.2,0.336921557999985));
#262549=CARTESIAN_POINT('Ctrl Pts',(-11.0546285370001,15.2,0.338137715999984));
#262550=CARTESIAN_POINT('Ctrl Pts',(-11.0575592300001,15.2,0.339358219999983));
#262551=CARTESIAN_POINT('Ctrl Pts',(-11.0604936960001,15.2,0.340583071999987));
#262552=CARTESIAN_POINT('Ctrl Pts',(-11.0634319250001,15.2,0.341812274999986));
#262553=CARTESIAN_POINT('Ctrl Pts',(-11.0663739070001,15.2,0.343045833999986));
#262554=CARTESIAN_POINT('Ctrl Pts',(-11.0693196320001,15.2,0.344283748999987));
#262555=CARTESIAN_POINT('Ctrl Pts',(-11.0722690870001,15.2,0.345526024999985));
#262556=CARTESIAN_POINT('Ctrl Pts',(-11.0752222620001,15.2,0.346772664999988));
#262557=CARTESIAN_POINT('Ctrl Pts',(-11.0781791480001,15.2,0.348023670999984));
#262558=CARTESIAN_POINT('Ctrl Pts',(-11.0811397300001,15.2,0.349279046999986));
#262559=CARTESIAN_POINT('Ctrl Pts',(-11.0841040020001,15.2,0.350538794999986));
#262560=CARTESIAN_POINT('Ctrl Pts',(-11.0870719500001,15.2,0.351802918999984));
#262561=CARTESIAN_POINT('Ctrl Pts',(-11.0900435650001,15.2,0.353071420999989));
#262562=CARTESIAN_POINT('Ctrl Pts',(-11.0930188360001,15.2,0.354344304999987));
#262563=CARTESIAN_POINT('Ctrl Pts',(-11.0959977500001,15.2,0.355621572999985));
#262564=CARTESIAN_POINT('Ctrl Pts',(-11.0989803000001,15.2,0.356903227999985));
#262565=CARTESIAN_POINT('Ctrl Pts',(-11.1019664740001,15.2,0.358189272999985));
#262566=CARTESIAN_POINT('Ctrl Pts',(-11.1049562600001,15.2,0.359479711999988));
#262567=CARTESIAN_POINT('Ctrl Pts',(-11.1079496490001,15.2,0.360774545999987));
#262568=CARTESIAN_POINT('Ctrl Pts',(-11.1109466290001,15.2,0.362073778999985));
#262569=CARTESIAN_POINT('Ctrl Pts',(-11.1139471900001,15.2,0.363377413999988));
#262570=CARTESIAN_POINT('Ctrl Pts',(-11.1169513230001,15.2,0.364685452999982));
#262571=CARTESIAN_POINT('Ctrl Pts',(-11.1199590150001,15.2,0.365997898999986));
#262572=CARTESIAN_POINT('Ctrl Pts',(-11.1229702580001,15.2,0.367314754999986));
#262573=CARTESIAN_POINT('Ctrl Pts',(-11.1259850390001,15.2,0.368636023999986));
#262574=CARTESIAN_POINT('Ctrl Pts',(-11.1290033490001,15.2,0.369961708999984));
#262575=CARTESIAN_POINT('Ctrl Pts',(-11.1320251780001,15.2,0.371291811999988));
#262576=CARTESIAN_POINT('Ctrl Pts',(-11.1350505130001,15.2,0.372626335999984));
#262577=CARTESIAN_POINT('Ctrl Pts',(-11.1380793470001,15.2,0.373965283999986));
#262578=CARTESIAN_POINT('Ctrl Pts',(-11.1411116670001,15.2,0.375308657999986));
#262579=CARTESIAN_POINT('Ctrl Pts',(-11.1441474640001,15.2,0.376656461999989));
#262580=CARTESIAN_POINT('Ctrl Pts',(-11.1471867270001,15.2,0.378008696999985));
#262581=CARTESIAN_POINT('Ctrl Pts',(-11.1502294460001,15.2,0.379365366999984));
#262582=CARTESIAN_POINT('Ctrl Pts',(-11.1532756110001,15.2,0.380726473999986));
#262583=CARTESIAN_POINT('Ctrl Pts',(-11.1563252100001,15.2,0.382092021999987));
#262584=CARTESIAN_POINT('Ctrl Pts',(-11.1593782350001,15.2,0.383462010999986));
#262585=CARTESIAN_POINT('Ctrl Pts',(-11.1624346740001,15.2,0.384836445999985));
#262586=CARTESIAN_POINT('Ctrl Pts',(-11.1654945190001,15.2,0.386215327999988));
#262587=CARTESIAN_POINT('Ctrl Pts',(-11.1685577570001,15.2,0.387598660999986));
#262588=CARTESIAN_POINT('Ctrl Pts',(-11.1716243780001,15.2,0.388986446999984));
#262589=CARTESIAN_POINT('Ctrl Pts',(-11.1746943740001,15.2,0.390378687999986));
#262590=CARTESIAN_POINT('Ctrl Pts',(-11.1777677340001,15.2,0.391775386999988));
#262591=CARTESIAN_POINT('Ctrl Pts',(-11.1808444470001,15.2,0.393176545999987));
#262592=CARTESIAN_POINT('Ctrl Pts',(-11.1839245020001,15.2,0.394582169999986));
#262593=CARTESIAN_POINT('Ctrl Pts',(-11.1870078920001,15.2,0.395992257999982));
#262594=CARTESIAN_POINT('Ctrl Pts',(-11.1900946040001,15.2,0.397406813999983));
#262595=CARTESIAN_POINT('Ctrl Pts',(-11.1931846300001,15.2,0.398825840999986));
#262596=CARTESIAN_POINT('Ctrl Pts',(-11.1962779570001,15.2,0.400249341999985));
#262597=CARTESIAN_POINT('Ctrl Pts',(-11.1993745780001,15.2,0.401677316999987));
#262598=CARTESIAN_POINT('Ctrl Pts',(-11.2024744820001,15.2,0.403109771999985));
#262599=CARTESIAN_POINT('Ctrl Pts',(-11.2055776580001,15.2,0.404546704999986));
#262600=CARTESIAN_POINT('Ctrl Pts',(-11.2086840970001,15.2,0.405988122999985));
#262601=CARTESIAN_POINT('Ctrl Pts',(-11.2117937880001,15.2,0.407434024999986));
#262602=CARTESIAN_POINT('Ctrl Pts',(-11.2149067230001,15.2,0.408884414999986));
#262603=CARTESIAN_POINT('Ctrl Pts',(-11.2180228910001,15.2,0.410339293999984));
#262604=CARTESIAN_POINT('Ctrl Pts',(-11.2211422810001,15.2,0.411798666999985));
#262605=CARTESIAN_POINT('Ctrl Pts',(-11.2242648840001,15.2,0.413262533999985));
#262606=CARTESIAN_POINT('Ctrl Pts',(-11.2273906900001,15.2,0.414730897999984));
#262607=CARTESIAN_POINT('Ctrl Pts',(-11.2305196890001,15.2,0.416203761999987));
#262608=CARTESIAN_POINT('Ctrl Pts',(-11.2336518720001,15.2,0.417681126999985));
#262609=CARTESIAN_POINT('Ctrl Pts',(-11.2367872280001,15.2,0.419162996999987));
#262610=CARTESIAN_POINT('Ctrl Pts',(-11.2399257470001,15.2,0.420649372999984));
#262611=CARTESIAN_POINT('Ctrl Pts',(-11.2430674210001,15.2,0.422140256999985));
#262612=CARTESIAN_POINT('Ctrl Pts',(-11.2462122380001,15.2,0.423635652999987));
#262613=CARTESIAN_POINT('Ctrl Pts',(-11.2493601900001,15.2,0.425135561999985));
#262614=CARTESIAN_POINT('Ctrl Pts',(-11.2525112650001,15.2,0.426639985999984));
#262615=CARTESIAN_POINT('Ctrl Pts',(-11.2556654560001,15.2,0.428148927999987));
#262616=CARTESIAN_POINT('Ctrl Pts',(-11.2588227510001,15.2,0.429662389999983));
#262617=CARTESIAN_POINT('Ctrl Pts',(-11.2619831420001,15.2,0.431180374999984));
#262618=CARTESIAN_POINT('Ctrl Pts',(-11.2651466170001,15.2,0.432702882999987));
#262619=CARTESIAN_POINT('Ctrl Pts',(-11.2683131690001,15.2,0.434229917999982));
#262620=CARTESIAN_POINT('Ctrl Pts',(-11.2714827870001,15.2,0.435761481999983));
#262621=CARTESIAN_POINT('Ctrl Pts',(-11.2746554610001,15.2,0.437297575999986));
#262622=CARTESIAN_POINT('Ctrl Pts',(-11.2778311820001,15.2,0.438838203999987));
#262623=CARTESIAN_POINT('Ctrl Pts',(-11.2810099400001,15.2,0.440383366999986));
#262624=CARTESIAN_POINT('Ctrl Pts',(-11.2841917260001,15.2,0.441933066999987));
#262625=CARTESIAN_POINT('Ctrl Pts',(-11.2873765290001,15.2,0.443487306999986));
#262626=CARTESIAN_POINT('Ctrl Pts',(-11.2905643410001,15.2,0.445046087999987));
#262627=CARTESIAN_POINT('Ctrl Pts',(-11.2937551520001,15.2,0.446609412999983));
#262628=CARTESIAN_POINT('Ctrl Pts',(-11.2969489510001,15.2,0.448177283999982));
#262629=CARTESIAN_POINT('Ctrl Pts',(-11.3001457320001,15.2,0.449749702999984));
#262630=CARTESIAN_POINT('Ctrl Pts',(-11.3033454810001,15.2,0.451326670999985));
#262631=CARTESIAN_POINT('Ctrl Pts',(-11.3065481920001,15.2,0.452908190999985));
#262632=CARTESIAN_POINT('Ctrl Pts',(-11.3097538530001,15.2,0.454494265999985));
#262633=CARTESIAN_POINT('Ctrl Pts',(-11.3129624580001,15.2,0.456084895999984));
#262634=CARTESIAN_POINT('Ctrl Pts',(-11.3161739920001,15.2,0.457680083999983));
#262635=CARTESIAN_POINT('Ctrl Pts',(-11.3193884510001,15.2,0.459279831999986));
#262636=CARTESIAN_POINT('Ctrl Pts',(-11.3226058230001,15.2,0.460884142999984));
#262637=CARTESIAN_POINT('Ctrl Pts',(-11.3258260990001,15.2,0.462493017999983));
#262638=CARTESIAN_POINT('Ctrl Pts',(-11.3290492700001,15.2,0.464106457999982));
#262639=CARTESIAN_POINT('Ctrl Pts',(-11.3322753250001,15.2,0.465724465999986));
#262640=CARTESIAN_POINT('Ctrl Pts',(-11.3355042560001,15.2,0.467347044999986));
#262641=CARTESIAN_POINT('Ctrl Pts',(-11.3387360540001,15.2,0.468974193999987));
#262642=CARTESIAN_POINT('Ctrl Pts',(-11.3419707090001,15.2,0.470605916999984));
#262643=CARTESIAN_POINT('Ctrl Pts',(-11.3452082120001,15.2,0.472242216999987));
#262644=CARTESIAN_POINT('Ctrl Pts',(-11.3484485530001,15.2,0.473883093999987));
#262645=CARTESIAN_POINT('Ctrl Pts',(-11.3516917240001,15.2,0.475528550999984));
#262646=CARTESIAN_POINT('Ctrl Pts',(-11.3549377140001,15.2,0.477178588999987));
#262647=CARTESIAN_POINT('Ctrl Pts',(-11.3581865150001,15.2,0.478833208999987));
#262648=CARTESIAN_POINT('Ctrl Pts',(-11.3614381180001,15.2,0.480492415999985));
#262649=CARTESIAN_POINT('Ctrl Pts',(-11.3646925130001,15.2,0.482156208999989));
#262650=CARTESIAN_POINT('Ctrl Pts',(-11.3679496900001,15.2,0.483824590999986));
#262651=CARTESIAN_POINT('Ctrl Pts',(-11.3712096420001,15.2,0.485497562999986));
#262652=CARTESIAN_POINT('Ctrl Pts',(-11.3744723580001,15.2,0.487175127999984));
#262653=CARTESIAN_POINT('Ctrl Pts',(-11.3777378300001,15.2,0.488857287999984));
#262654=CARTESIAN_POINT('Ctrl Pts',(-11.3810060480001,15.2,0.490544042999983));
#262655=CARTESIAN_POINT('Ctrl Pts',(-11.3842770020001,15.2,0.492235395999985));
#262656=CARTESIAN_POINT('Ctrl Pts',(-11.3875506850001,15.2,0.493931348999985));
#262657=CARTESIAN_POINT('Ctrl Pts',(-11.3908270860001,15.2,0.495631902999989));
#262658=CARTESIAN_POINT('Ctrl Pts',(-11.3941061970001,15.2,0.497337060999987));
#262659=CARTESIAN_POINT('Ctrl Pts',(-11.3973880080001,15.2,0.499046821999984));
#262660=CARTESIAN_POINT('Ctrl Pts',(-11.4006725110001,15.2,0.500761190999985));
#262661=CARTESIAN_POINT('Ctrl Pts',(-11.4039596970001,15.2,0.502480167999986));
#262662=CARTESIAN_POINT('Ctrl Pts',(-11.4072495570001,15.2,0.504203755999986));
#262663=CARTESIAN_POINT('Ctrl Pts',(-11.4105420820001,15.2,0.505931953999985));
#262664=CARTESIAN_POINT('Ctrl Pts',(-11.4138372610001,15.2,0.507664766999985));
#262665=CARTESIAN_POINT('Ctrl Pts',(-11.4171350880001,15.2,0.509402193999984));
#262666=CARTESIAN_POINT('Ctrl Pts',(-11.4204355510001,15.2,0.511144238999983));
#262667=CARTESIAN_POINT('Ctrl Pts',(-11.4237386430001,15.2,0.512890900999987));
#262668=CARTESIAN_POINT('Ctrl Pts',(-11.4270443520001,15.2,0.514642183999987));
#262669=CARTESIAN_POINT('Ctrl Pts',(-11.4303526710001,15.2,0.516398088999988));
#262670=CARTESIAN_POINT('Ctrl Pts',(-11.4336635900001,15.2,0.518158617999984));
#262671=CARTESIAN_POINT('Ctrl Pts',(-11.4369771030001,15.2,0.519923770999986));
#262672=CARTESIAN_POINT('Ctrl Pts',(-11.4402932010001,15.2,0.521693550999984));
#262673=CARTESIAN_POINT('Ctrl Pts',(-11.4436118760001,15.2,0.523467958999984));
#262674=CARTESIAN_POINT('Ctrl Pts',(-11.4469331180001,15.2,0.525246995999984));
#262675=CARTESIAN_POINT('Ctrl Pts',(-11.4502569220001,15.2,0.527030663999986));
#262676=CARTESIAN_POINT('Ctrl Pts',(-11.4535832720001,15.2,0.528818965999989));
#262677=CARTESIAN_POINT('Ctrl Pts',(-11.4569121620001,15.2,0.530611900999984));
#262678=CARTESIAN_POINT('Ctrl Pts',(-11.4602435780001,15.2,0.532409473999986));
#262679=CARTESIAN_POINT('Ctrl Pts',(-11.4635775100001,15.2,0.534211684999986));
#262680=CARTESIAN_POINT('Ctrl Pts',(-11.4669139500001,15.2,0.536018536999983));
#262681=CARTESIAN_POINT('Ctrl Pts',(-11.4702528880001,15.2,0.537830029999986));
#262682=CARTESIAN_POINT('Ctrl Pts',(-11.4735943180001,15.2,0.539646165999983));
#262683=CARTESIAN_POINT('Ctrl Pts',(-11.4769382380001,15.2,0.541466945999982));
#262684=CARTESIAN_POINT('Ctrl Pts',(-11.4802846430001,15.2,0.543292367999988));
#262685=CARTESIAN_POINT('Ctrl Pts',(-11.4829637560001,15.2,0.544756421999986));
#262686=CARTESIAN_POINT('Ctrl Pts',(-11.4849742100001,15.2,0.545856550999986));
#262687=CARTESIAN_POINT('Ctrl Pts',(-11.4863150090001,15.2,0.546590898999986));
#262688=CARTESIAN_POINT('Ctrl Pts',(-11.4869855320001,15.2,0.546958305999983));
#262689=CARTESIAN_POINT('Origin',(-5.66257110645729E-14,15.2,-1.77635683940025E-14));
#262690=CARTESIAN_POINT('',(-10.3708900234024,15.2,-0.292001929001953));
#262691=CARTESIAN_POINT('',(-10.3708900234024,12.2,-0.292001929001953));
#262692=CARTESIAN_POINT('',(-10.3708900230001,15.2,-0.292001929000012));
#262693=CARTESIAN_POINT('Origin',(-5.66257110645729E-14,12.2,-1.77635683940025E-14));
#262694=CARTESIAN_POINT('Origin',(-5.66257110645729E-14,15.2,-1.77635683940025E-14));
#262695=CARTESIAN_POINT('Origin',(-5.66257110645729E-14,15.2,-1.77635683940025E-14));
#262696=CARTESIAN_POINT('',(-11.4780040730001,15.2,-0.710930734000015));
#262697=CARTESIAN_POINT('',(-11.4479048650001,15.2,-1.09337742900002));
#262698=CARTESIAN_POINT('Origin',(-5.66257110645729E-14,15.2,-1.77635683940025E-14));
#262699=CARTESIAN_POINT('',(-11.4479048650001,12.2,-1.09337742900002));
#262700=CARTESIAN_POINT('',(-11.4479048650001,15.2,-1.09337742900002));
#262701=CARTESIAN_POINT('',(-11.4780040730001,12.2,-0.710930734000015));
#262702=CARTESIAN_POINT('Origin',(-5.66257110645729E-14,12.2,-1.77635683940025E-14));
#262703=CARTESIAN_POINT('',(-11.4780040730001,15.2,-0.710930734000015));
#262704=CARTESIAN_POINT('Ctrl Pts',(-11.4479048650001,15.2,-1.09337742900002));
#262705=CARTESIAN_POINT('Ctrl Pts',(-11.4479048650001,11.6,-1.09337742900002));
#262706=CARTESIAN_POINT('Ctrl Pts',(-11.4471888790001,15.2,-1.09364567100001));
#262707=CARTESIAN_POINT('Ctrl Pts',(-11.4471888790001,11.6,-1.09364567100001));
#262708=CARTESIAN_POINT('Ctrl Pts',(-11.4457572180001,15.2,-1.09418172800002));
#262709=CARTESIAN_POINT('Ctrl Pts',(-11.4457572180001,11.6,-1.09418172800002));
#262710=CARTESIAN_POINT('Ctrl Pts',(-11.4436106650001,15.2,-1.09498454300001));
#262711=CARTESIAN_POINT('Ctrl Pts',(-11.4436106650001,11.6,-1.09498454300002));
#262712=CARTESIAN_POINT('Ctrl Pts',(-11.4407504650001,15.2,-1.09605241700002));
#262713=CARTESIAN_POINT('Ctrl Pts',(-11.4407504650001,11.6,-1.09605241700002));
#262714=CARTESIAN_POINT('Ctrl Pts',(-11.4371783360001,15.2,-1.09738301600002));
#262715=CARTESIAN_POINT('Ctrl Pts',(-11.4371783360001,11.6,-1.09738301600002));
#262716=CARTESIAN_POINT('Ctrl Pts',(-11.4336093280001,15.2,-1.09870937400002));
#262717=CARTESIAN_POINT('Ctrl Pts',(-11.4336093280001,11.6,-1.09870937400002));
#262718=CARTESIAN_POINT('Ctrl Pts',(-11.4300434450001,15.2,-1.10003148800002));
#262719=CARTESIAN_POINT('Ctrl Pts',(-11.4300434450001,11.6,-1.10003148800002));
#262720=CARTESIAN_POINT('Ctrl Pts',(-11.4264806910001,15.2,-1.10134936300001));
#262721=CARTESIAN_POINT('Ctrl Pts',(-11.4264806910001,11.6,-1.10134936300002));
#262722=CARTESIAN_POINT('Ctrl Pts',(-11.4229210700001,15.2,-1.10266299900001));
#262723=CARTESIAN_POINT('Ctrl Pts',(-11.4229210700001,11.6,-1.10266299900002));
#262724=CARTESIAN_POINT('Ctrl Pts',(-11.4193645910001,15.2,-1.10397239900001));
#262725=CARTESIAN_POINT('Ctrl Pts',(-11.4193645910001,11.6,-1.10397239900002));
#262726=CARTESIAN_POINT('Ctrl Pts',(-11.4158112620001,15.2,-1.10527756400002));
#262727=CARTESIAN_POINT('Ctrl Pts',(-11.4158112620001,11.6,-1.10527756400002));
#262728=CARTESIAN_POINT('Ctrl Pts',(-11.4122610950001,15.2,-1.10657850000001));
#262729=CARTESIAN_POINT('Ctrl Pts',(-11.4122610950001,11.6,-1.10657850000001));
#262730=CARTESIAN_POINT('Ctrl Pts',(-11.4087141000001,15.2,-1.10787520900002));
#262731=CARTESIAN_POINT('Ctrl Pts',(-11.4087141000001,11.6,-1.10787520900002));
#262732=CARTESIAN_POINT('Ctrl Pts',(-11.4051702860001,15.2,-1.10916769600002));
#262733=CARTESIAN_POINT('Ctrl Pts',(-11.4051702860001,11.6,-1.10916769600002));
#262734=CARTESIAN_POINT('Ctrl Pts',(-11.4016296650001,15.2,-1.11045596300002));
#262735=CARTESIAN_POINT('Ctrl Pts',(-11.4016296650001,11.6,-1.11045596300002));
#262736=CARTESIAN_POINT('Ctrl Pts',(-11.3980922450001,15.2,-1.11174001300002));
#262737=CARTESIAN_POINT('Ctrl Pts',(-11.3980922450001,11.6,-1.11174001300002));
#262738=CARTESIAN_POINT('Ctrl Pts',(-11.3945580340001,15.2,-1.11301985000001));
#262739=CARTESIAN_POINT('Ctrl Pts',(-11.3945580340001,11.6,-1.11301985000001));
#262740=CARTESIAN_POINT('Ctrl Pts',(-11.3910270410001,15.2,-1.11429547400002));
#262741=CARTESIAN_POINT('Ctrl Pts',(-11.3910270410001,11.6,-1.11429547400002));
#262742=CARTESIAN_POINT('Ctrl Pts',(-11.3874992720001,15.2,-1.11556689000002));
#262743=CARTESIAN_POINT('Ctrl Pts',(-11.3874992720001,11.6,-1.11556689000002));
#262744=CARTESIAN_POINT('Ctrl Pts',(-11.3839747360001,15.2,-1.11683410000001));
#262745=CARTESIAN_POINT('Ctrl Pts',(-11.3839747360001,11.6,-1.11683410000001));
#262746=CARTESIAN_POINT('Ctrl Pts',(-11.3804534400001,15.2,-1.11809710600001));
#262747=CARTESIAN_POINT('Ctrl Pts',(-11.3804534400001,11.6,-1.11809710600001));
#262748=CARTESIAN_POINT('Ctrl Pts',(-11.3769353940001,15.2,-1.11935591200002));
#262749=CARTESIAN_POINT('Ctrl Pts',(-11.3769353940001,11.6,-1.11935591200002));
#262750=CARTESIAN_POINT('Ctrl Pts',(-11.3734206060001,15.2,-1.12061052000001));
#262751=CARTESIAN_POINT('Ctrl Pts',(-11.3734206060001,11.6,-1.12061052000001));
#262752=CARTESIAN_POINT('Ctrl Pts',(-11.3699090850001,15.2,-1.12186093300001));
#262753=CARTESIAN_POINT('Ctrl Pts',(-11.3699090850001,11.6,-1.12186093300001));
#262754=CARTESIAN_POINT('Ctrl Pts',(-11.3664008400001,15.2,-1.12310715400001));
#262755=CARTESIAN_POINT('Ctrl Pts',(-11.3664008400001,11.6,-1.12310715400001));
#262756=CARTESIAN_POINT('Ctrl Pts',(-11.3628958810001,15.2,-1.12434918700002));
#262757=CARTESIAN_POINT('Ctrl Pts',(-11.3628958810001,11.6,-1.12434918700002));
#262758=CARTESIAN_POINT('Ctrl Pts',(-11.3593942150001,15.2,-1.12558703500001));
#262759=CARTESIAN_POINT('Ctrl Pts',(-11.3593942150001,11.6,-1.12558703500001));
#262760=CARTESIAN_POINT('Ctrl Pts',(-11.3558958510001,15.2,-1.12682069900002));
#262761=CARTESIAN_POINT('Ctrl Pts',(-11.3558958510001,11.6,-1.12682069900002));
#262762=CARTESIAN_POINT('Ctrl Pts',(-11.3524008000001,15.2,-1.12805018600001));
#262763=CARTESIAN_POINT('Ctrl Pts',(-11.3524008000001,11.6,-1.12805018600001));
#262764=CARTESIAN_POINT('Ctrl Pts',(-11.3489090690001,15.2,-1.12927549400001));
#262765=CARTESIAN_POINT('Ctrl Pts',(-11.3489090690001,11.6,-1.12927549400002));
#262766=CARTESIAN_POINT('Ctrl Pts',(-11.3454206650001,15.2,-1.13049662900002));
#262767=CARTESIAN_POINT('Ctrl Pts',(-11.3454206650001,11.6,-1.13049662900002));
#262768=CARTESIAN_POINT('Ctrl Pts',(-11.3419355990001,15.2,-1.13171359300001));
#262769=CARTESIAN_POINT('Ctrl Pts',(-11.3419355990001,11.6,-1.13171359300001));
#262770=CARTESIAN_POINT('Ctrl Pts',(-11.3384538780001,15.2,-1.13292639100001));
#262771=CARTESIAN_POINT('Ctrl Pts',(-11.3384538780001,11.6,-1.13292639100001));
#262772=CARTESIAN_POINT('Ctrl Pts',(-11.3349755130001,15.2,-1.13413502300002));
#262773=CARTESIAN_POINT('Ctrl Pts',(-11.3349755130001,11.6,-1.13413502300002));
#262774=CARTESIAN_POINT('Ctrl Pts',(-11.3315005100001,15.2,-1.13533949300002));
#262775=CARTESIAN_POINT('Ctrl Pts',(-11.3315005100001,11.6,-1.13533949300002));
#262776=CARTESIAN_POINT('Ctrl Pts',(-11.3280288800001,15.2,-1.13653980600001));
#262777=CARTESIAN_POINT('Ctrl Pts',(-11.3280288800001,11.6,-1.13653980600001));
#262778=CARTESIAN_POINT('Ctrl Pts',(-11.3245606310001,15.2,-1.13773596300002));
#262779=CARTESIAN_POINT('Ctrl Pts',(-11.3245606310001,11.6,-1.13773596300002));
#262780=CARTESIAN_POINT('Ctrl Pts',(-11.3210957720001,15.2,-1.13892796700001));
#262781=CARTESIAN_POINT('Ctrl Pts',(-11.3210957720001,11.6,-1.13892796700001));
#262782=CARTESIAN_POINT('Ctrl Pts',(-11.3176343120001,15.2,-1.14011582200002));
#262783=CARTESIAN_POINT('Ctrl Pts',(-11.3176343120001,11.6,-1.14011582200002));
#262784=CARTESIAN_POINT('Ctrl Pts',(-11.3141762600001,15.2,-1.14129953200001));
#262785=CARTESIAN_POINT('Ctrl Pts',(-11.3141762600001,11.6,-1.14129953200001));
#262786=CARTESIAN_POINT('Ctrl Pts',(-11.3107216250001,15.2,-1.14247909900001));
#262787=CARTESIAN_POINT('Ctrl Pts',(-11.3107216250001,11.6,-1.14247909900001));
#262788=CARTESIAN_POINT('Ctrl Pts',(-11.3072704150001,15.2,-1.14365452600001));
#262789=CARTESIAN_POINT('Ctrl Pts',(-11.3072704150001,11.6,-1.14365452600001));
#262790=CARTESIAN_POINT('Ctrl Pts',(-11.3038226390001,15.2,-1.14482581600001));
#262791=CARTESIAN_POINT('Ctrl Pts',(-11.3038226390001,11.6,-1.14482581600001));
#262792=CARTESIAN_POINT('Ctrl Pts',(-11.3003783060001,15.2,-1.14599297300002));
#262793=CARTESIAN_POINT('Ctrl Pts',(-11.3003783060001,11.6,-1.14599297300002));
#262794=CARTESIAN_POINT('Ctrl Pts',(-11.2969374260001,15.2,-1.14715599900002));
#262795=CARTESIAN_POINT('Ctrl Pts',(-11.2969374260001,11.6,-1.14715599900002));
#262796=CARTESIAN_POINT('Ctrl Pts',(-11.2935000060001,15.2,-1.14831489900002));
#262797=CARTESIAN_POINT('Ctrl Pts',(-11.2935000060001,11.6,-1.14831489900002));
#262798=CARTESIAN_POINT('Ctrl Pts',(-11.2900660570001,15.2,-1.14946967500002));
#262799=CARTESIAN_POINT('Ctrl Pts',(-11.2900660570001,11.6,-1.14946967500002));
#262800=CARTESIAN_POINT('Ctrl Pts',(-11.2866355860001,15.2,-1.15062033000001));
#262801=CARTESIAN_POINT('Ctrl Pts',(-11.2866355860001,11.6,-1.15062033000001));
#262802=CARTESIAN_POINT('Ctrl Pts',(-11.2832086040001,15.2,-1.15176686800002));
#262803=CARTESIAN_POINT('Ctrl Pts',(-11.2832086040001,11.6,-1.15176686800002));
#262804=CARTESIAN_POINT('Ctrl Pts',(-11.2797851190001,15.2,-1.15290929100002));
#262805=CARTESIAN_POINT('Ctrl Pts',(-11.2797851190001,11.6,-1.15290929100002));
#262806=CARTESIAN_POINT('Ctrl Pts',(-11.2763651390001,15.2,-1.15404760400001));
#262807=CARTESIAN_POINT('Ctrl Pts',(-11.2763651390001,11.6,-1.15404760400002));
#262808=CARTESIAN_POINT('Ctrl Pts',(-11.2729486730001,15.2,-1.15518181000001));
#262809=CARTESIAN_POINT('Ctrl Pts',(-11.2729486730001,11.6,-1.15518181000001));
#262810=CARTESIAN_POINT('Ctrl Pts',(-11.2695357330001,15.2,-1.15631191100002));
#262811=CARTESIAN_POINT('Ctrl Pts',(-11.2695357330001,11.6,-1.15631191100002));
#262812=CARTESIAN_POINT('Ctrl Pts',(-11.2661263250001,15.2,-1.15743791100002));
#262813=CARTESIAN_POINT('Ctrl Pts',(-11.2661263250001,11.6,-1.15743791100002));
#262814=CARTESIAN_POINT('Ctrl Pts',(-11.2627204590001,15.2,-1.15855981300002));
#262815=CARTESIAN_POINT('Ctrl Pts',(-11.2627204590001,11.6,-1.15855981300002));
#262816=CARTESIAN_POINT('Ctrl Pts',(-11.2593181450001,15.2,-1.15967762100002));
#262817=CARTESIAN_POINT('Ctrl Pts',(-11.2593181450001,11.6,-1.15967762100002));
#262818=CARTESIAN_POINT('Ctrl Pts',(-11.2559193900001,15.2,-1.16079133800001));
#262819=CARTESIAN_POINT('Ctrl Pts',(-11.2559193900001,11.6,-1.16079133800001));
#262820=CARTESIAN_POINT('Ctrl Pts',(-11.2525242050001,15.2,-1.16190096800001));
#262821=CARTESIAN_POINT('Ctrl Pts',(-11.2525242050001,11.6,-1.16190096800001));
#262822=CARTESIAN_POINT('Ctrl Pts',(-11.2491325970001,15.2,-1.16300651300001));
#262823=CARTESIAN_POINT('Ctrl Pts',(-11.2491325970001,11.6,-1.16300651300001));
#262824=CARTESIAN_POINT('Ctrl Pts',(-11.2457445790001,15.2,-1.16410797700001));
#262825=CARTESIAN_POINT('Ctrl Pts',(-11.2457445790001,11.6,-1.16410797700001));
#262826=CARTESIAN_POINT('Ctrl Pts',(-11.2423601550001,15.2,-1.16520536500001));
#262827=CARTESIAN_POINT('Ctrl Pts',(-11.2423601550001,11.6,-1.16520536500001));
#262828=CARTESIAN_POINT('Ctrl Pts',(-11.2389793380001,15.2,-1.16629867700001));
#262829=CARTESIAN_POINT('Ctrl Pts',(-11.2389793380001,11.6,-1.16629867700001));
#262830=CARTESIAN_POINT('Ctrl Pts',(-11.2356021350001,15.2,-1.16738791900001));
#262831=CARTESIAN_POINT('Ctrl Pts',(-11.2356021350001,11.6,-1.16738791900001));
#262832=CARTESIAN_POINT('Ctrl Pts',(-11.2322285580001,15.2,-1.16847309500002));
#262833=CARTESIAN_POINT('Ctrl Pts',(-11.2322285580001,11.6,-1.16847309500002));
#262834=CARTESIAN_POINT('Ctrl Pts',(-11.2288586130001,15.2,-1.16955420600001));
#262835=CARTESIAN_POINT('Ctrl Pts',(-11.2288586130001,11.6,-1.16955420600001));
#262836=CARTESIAN_POINT('Ctrl Pts',(-11.2254923100001,15.2,-1.17063125600001));
#262837=CARTESIAN_POINT('Ctrl Pts',(-11.2254923100001,11.6,-1.17063125600001));
#262838=CARTESIAN_POINT('Ctrl Pts',(-11.2221296590001,15.2,-1.17170425100001));
#262839=CARTESIAN_POINT('Ctrl Pts',(-11.2221296590001,11.6,-1.17170425100001));
#262840=CARTESIAN_POINT('Ctrl Pts',(-11.2187706690001,15.2,-1.17277319100001));
#262841=CARTESIAN_POINT('Ctrl Pts',(-11.2187706690001,11.6,-1.17277319100001));
#262842=CARTESIAN_POINT('Ctrl Pts',(-11.2154153490001,15.2,-1.17383808300001));
#262843=CARTESIAN_POINT('Ctrl Pts',(-11.2154153490001,11.6,-1.17383808300001));
#262844=CARTESIAN_POINT('Ctrl Pts',(-11.2120637080001,15.2,-1.17489892700001));
#262845=CARTESIAN_POINT('Ctrl Pts',(-11.2120637080001,11.6,-1.17489892700001));
#262846=CARTESIAN_POINT('Ctrl Pts',(-11.2087157570001,15.2,-1.17595572900001));
#262847=CARTESIAN_POINT('Ctrl Pts',(-11.2087157570001,11.6,-1.17595572900001));
#262848=CARTESIAN_POINT('Ctrl Pts',(-11.2053715030001,15.2,-1.17700849300002));
#262849=CARTESIAN_POINT('Ctrl Pts',(-11.2053715030001,11.6,-1.17700849300002));
#262850=CARTESIAN_POINT('Ctrl Pts',(-11.2020309560001,15.2,-1.17805721900002));
#262851=CARTESIAN_POINT('Ctrl Pts',(-11.2020309560001,11.6,-1.17805721900002));
#262852=CARTESIAN_POINT('Ctrl Pts',(-11.1986941260001,15.2,-1.17910191500001));
#262853=CARTESIAN_POINT('Ctrl Pts',(-11.1986941260001,11.6,-1.17910191500001));
#262854=CARTESIAN_POINT('Ctrl Pts',(-11.1953610220001,15.2,-1.18014258100001));
#262855=CARTESIAN_POINT('Ctrl Pts',(-11.1953610220001,11.6,-1.18014258100001));
#262856=CARTESIAN_POINT('Ctrl Pts',(-11.1920316530001,15.2,-1.18117922300002));
#262857=CARTESIAN_POINT('Ctrl Pts',(-11.1920316530001,11.6,-1.18117922300002));
#262858=CARTESIAN_POINT('Ctrl Pts',(-11.1887060280001,15.2,-1.18221184300001));
#262859=CARTESIAN_POINT('Ctrl Pts',(-11.1887060280001,11.6,-1.18221184300001));
#262860=CARTESIAN_POINT('Ctrl Pts',(-11.1853841570001,15.2,-1.18324044600001));
#262861=CARTESIAN_POINT('Ctrl Pts',(-11.1853841570001,11.6,-1.18324044600001));
#262862=CARTESIAN_POINT('Ctrl Pts',(-11.1820660500001,15.2,-1.18426503500002));
#262863=CARTESIAN_POINT('Ctrl Pts',(-11.1820660500001,11.6,-1.18426503500002));
#262864=CARTESIAN_POINT('Ctrl Pts',(-11.1787517160001,15.2,-1.18528561300002));
#262865=CARTESIAN_POINT('Ctrl Pts',(-11.1787517160001,11.6,-1.18528561300002));
#262866=CARTESIAN_POINT('Ctrl Pts',(-11.1754411630001,15.2,-1.18630218500002));
#262867=CARTESIAN_POINT('Ctrl Pts',(-11.1754411630001,11.6,-1.18630218500002));
#262868=CARTESIAN_POINT('Ctrl Pts',(-11.1721344020001,15.2,-1.18731475500002));
#262869=CARTESIAN_POINT('Ctrl Pts',(-11.1721344020001,11.6,-1.18731475500002));
#262870=CARTESIAN_POINT('Ctrl Pts',(-11.1688314420001,15.2,-1.18832332500002));
#262871=CARTESIAN_POINT('Ctrl Pts',(-11.1688314420001,11.6,-1.18832332500002));
#262872=CARTESIAN_POINT('Ctrl Pts',(-11.1655322930001,15.2,-1.18932789900001));
#262873=CARTESIAN_POINT('Ctrl Pts',(-11.1655322930001,11.6,-1.18932789900001));
#262874=CARTESIAN_POINT('Ctrl Pts',(-11.1622369630001,15.2,-1.19032848100002));
#262875=CARTESIAN_POINT('Ctrl Pts',(-11.1622369630001,11.6,-1.19032848100002));
#262876=CARTESIAN_POINT('Ctrl Pts',(-11.1589454620001,15.2,-1.19132507600002));
#262877=CARTESIAN_POINT('Ctrl Pts',(-11.1589454620001,11.6,-1.19132507600002));
#262878=CARTESIAN_POINT('Ctrl Pts',(-11.1556578010001,15.2,-1.19231768700002));
#262879=CARTESIAN_POINT('Ctrl Pts',(-11.1556578010001,11.6,-1.19231768700002));
#262880=CARTESIAN_POINT('Ctrl Pts',(-11.1523739880001,15.2,-1.19330631600001));
#262881=CARTESIAN_POINT('Ctrl Pts',(-11.1523739880001,11.6,-1.19330631600001));
#262882=CARTESIAN_POINT('Ctrl Pts',(-11.1490940330001,15.2,-1.19429096900001));
#262883=CARTESIAN_POINT('Ctrl Pts',(-11.1490940330001,11.6,-1.19429096900001));
#262884=CARTESIAN_POINT('Ctrl Pts',(-11.1458179460001,15.2,-1.19527164900001));
#262885=CARTESIAN_POINT('Ctrl Pts',(-11.1458179460001,11.6,-1.19527164900001));
#262886=CARTESIAN_POINT('Ctrl Pts',(-11.1425457350001,15.2,-1.19624836000002));
#262887=CARTESIAN_POINT('Ctrl Pts',(-11.1425457350001,11.6,-1.19624836000002));
#262888=CARTESIAN_POINT('Ctrl Pts',(-11.1392774120001,15.2,-1.19722110600001));
#262889=CARTESIAN_POINT('Ctrl Pts',(-11.1392774120001,11.6,-1.19722110600002));
#262890=CARTESIAN_POINT('Ctrl Pts',(-11.1360129840001,15.2,-1.19818989000001));
#262891=CARTESIAN_POINT('Ctrl Pts',(-11.1360129840001,11.6,-1.19818989000001));
#262892=CARTESIAN_POINT('Ctrl Pts',(-11.1327524620001,15.2,-1.19915471800002));
#262893=CARTESIAN_POINT('Ctrl Pts',(-11.1327524620001,11.6,-1.19915471800002));
#262894=CARTESIAN_POINT('Ctrl Pts',(-11.1294958560001,15.2,-1.20011559100002));
#262895=CARTESIAN_POINT('Ctrl Pts',(-11.1294958560001,11.6,-1.20011559100002));
#262896=CARTESIAN_POINT('Ctrl Pts',(-11.1262431750001,15.2,-1.20107251400002));
#262897=CARTESIAN_POINT('Ctrl Pts',(-11.1262431750001,11.6,-1.20107251400002));
#262898=CARTESIAN_POINT('Ctrl Pts',(-11.1229944280001,15.2,-1.20202549200001));
#262899=CARTESIAN_POINT('Ctrl Pts',(-11.1229944280001,11.6,-1.20202549200001));
#262900=CARTESIAN_POINT('Ctrl Pts',(-11.1197496260001,15.2,-1.20297452800001));
#262901=CARTESIAN_POINT('Ctrl Pts',(-11.1197496260001,11.6,-1.20297452800001));
#262902=CARTESIAN_POINT('Ctrl Pts',(-11.1165087780001,15.2,-1.20391962700001));
#262903=CARTESIAN_POINT('Ctrl Pts',(-11.1165087780001,11.6,-1.20391962700001));
#262904=CARTESIAN_POINT('Ctrl Pts',(-11.1132718940001,15.2,-1.20486079100001));
#262905=CARTESIAN_POINT('Ctrl Pts',(-11.1132718940001,11.6,-1.20486079100001));
#262906=CARTESIAN_POINT('Ctrl Pts',(-11.1100389830001,15.2,-1.20579802500002));
#262907=CARTESIAN_POINT('Ctrl Pts',(-11.1100389830001,11.6,-1.20579802500002));
#262908=CARTESIAN_POINT('Ctrl Pts',(-11.1068100550001,15.2,-1.20673133400001));
#262909=CARTESIAN_POINT('Ctrl Pts',(-11.1068100550001,11.6,-1.20673133400001));
#262910=CARTESIAN_POINT('Ctrl Pts',(-11.1035851210001,15.2,-1.20766072000002));
#262911=CARTESIAN_POINT('Ctrl Pts',(-11.1035851210001,11.6,-1.20766072000002));
#262912=CARTESIAN_POINT('Ctrl Pts',(-11.1003641890001,15.2,-1.20858618800002));
#262913=CARTESIAN_POINT('Ctrl Pts',(-11.1003641890001,11.6,-1.20858618800002));
#262914=CARTESIAN_POINT('Ctrl Pts',(-11.0971472700001,15.2,-1.20950774300002));
#262915=CARTESIAN_POINT('Ctrl Pts',(-11.0971472700001,11.6,-1.20950774300002));
#262916=CARTESIAN_POINT('Ctrl Pts',(-11.0939343730001,15.2,-1.21042538700001));
#262917=CARTESIAN_POINT('Ctrl Pts',(-11.0939343730001,11.6,-1.21042538700001));
#262918=CARTESIAN_POINT('Ctrl Pts',(-11.0907255090001,15.2,-1.21133912600001));
#262919=CARTESIAN_POINT('Ctrl Pts',(-11.0907255090001,11.6,-1.21133912600001));
#262920=CARTESIAN_POINT('Ctrl Pts',(-11.0875206860001,15.2,-1.21224896200001));
#262921=CARTESIAN_POINT('Ctrl Pts',(-11.0875206860001,11.6,-1.21224896200001));
#262922=CARTESIAN_POINT('Ctrl Pts',(-11.0843199150001,15.2,-1.21315490200002));
#262923=CARTESIAN_POINT('Ctrl Pts',(-11.0843199150001,11.6,-1.21315490200002));
#262924=CARTESIAN_POINT('Ctrl Pts',(-11.0811232050001,15.2,-1.21405694800002));
#262925=CARTESIAN_POINT('Ctrl Pts',(-11.0811232050001,11.6,-1.21405694800002));
#262926=CARTESIAN_POINT('Ctrl Pts',(-11.0779305680001,15.2,-1.21495510400001));
#262927=CARTESIAN_POINT('Ctrl Pts',(-11.0779305680001,11.6,-1.21495510400001));
#262928=CARTESIAN_POINT('Ctrl Pts',(-11.0747420110001,15.2,-1.21584937600002));
#262929=CARTESIAN_POINT('Ctrl Pts',(-11.0747420110001,11.6,-1.21584937600002));
#262930=CARTESIAN_POINT('Ctrl Pts',(-11.0715575460001,15.2,-1.21673976600002));
#262931=CARTESIAN_POINT('Ctrl Pts',(-11.0715575460001,11.6,-1.21673976600002));
#262932=CARTESIAN_POINT('Ctrl Pts',(-11.0683771820001,15.2,-1.21762628000001));
#262933=CARTESIAN_POINT('Ctrl Pts',(-11.0683771820001,11.6,-1.21762628000001));
#262934=CARTESIAN_POINT('Ctrl Pts',(-11.0652009300001,15.2,-1.21850892000001));
#262935=CARTESIAN_POINT('Ctrl Pts',(-11.0652009300001,11.6,-1.21850892000001));
#262936=CARTESIAN_POINT('Ctrl Pts',(-11.0620287980001,15.2,-1.21938769300002));
#262937=CARTESIAN_POINT('Ctrl Pts',(-11.0620287980001,11.6,-1.21938769300002));
#262938=CARTESIAN_POINT('Ctrl Pts',(-11.0588607980001,15.2,-1.22026260000001));
#262939=CARTESIAN_POINT('Ctrl Pts',(-11.0588607980001,11.6,-1.22026260000002));
#262940=CARTESIAN_POINT('Ctrl Pts',(-11.0556969390001,15.2,-1.22113364900001));
#262941=CARTESIAN_POINT('Ctrl Pts',(-11.0556969390001,11.6,-1.22113364900002));
#262942=CARTESIAN_POINT('Ctrl Pts',(-11.0525372310001,15.2,-1.22200084200002));
#262943=CARTESIAN_POINT('Ctrl Pts',(-11.0525372310001,11.6,-1.22200084200002));
#262944=CARTESIAN_POINT('Ctrl Pts',(-11.0493816840001,15.2,-1.22286418300002));
#262945=CARTESIAN_POINT('Ctrl Pts',(-11.0493816840001,11.6,-1.22286418300002));
#262946=CARTESIAN_POINT('Ctrl Pts',(-11.0462303080001,15.2,-1.22372367600001));
#262947=CARTESIAN_POINT('Ctrl Pts',(-11.0462303080001,11.6,-1.22372367600002));
#262948=CARTESIAN_POINT('Ctrl Pts',(-11.0430831140001,15.2,-1.22457932800002));
#262949=CARTESIAN_POINT('Ctrl Pts',(-11.0430831140001,11.6,-1.22457932800002));
#262950=CARTESIAN_POINT('Ctrl Pts',(-11.0399401110001,15.2,-1.22543114000001));
#262951=CARTESIAN_POINT('Ctrl Pts',(-11.0399401110001,11.6,-1.22543114000001));
#262952=CARTESIAN_POINT('Ctrl Pts',(-11.0368013090001,15.2,-1.22627911900001));
#262953=CARTESIAN_POINT('Ctrl Pts',(-11.0368013090001,11.6,-1.22627911900001));
#262954=CARTESIAN_POINT('Ctrl Pts',(-11.0336667190001,15.2,-1.22712326700002));
#262955=CARTESIAN_POINT('Ctrl Pts',(-11.0336667190001,11.6,-1.22712326700002));
#262956=CARTESIAN_POINT('Ctrl Pts',(-11.0305363500001,15.2,-1.22796359100001));
#262957=CARTESIAN_POINT('Ctrl Pts',(-11.0305363500001,11.6,-1.22796359100001));
#262958=CARTESIAN_POINT('Ctrl Pts',(-11.0274102140001,15.2,-1.22880009400001));
#262959=CARTESIAN_POINT('Ctrl Pts',(-11.0274102140001,11.6,-1.22880009400001));
#262960=CARTESIAN_POINT('Ctrl Pts',(-11.0242883200001,15.2,-1.22963277900002));
#262961=CARTESIAN_POINT('Ctrl Pts',(-11.0242883200001,11.6,-1.22963277900002));
#262962=CARTESIAN_POINT('Ctrl Pts',(-11.0211706780001,15.2,-1.23046165300002));
#262963=CARTESIAN_POINT('Ctrl Pts',(-11.0211706780001,11.6,-1.23046165300002));
#262964=CARTESIAN_POINT('Ctrl Pts',(-11.0180572970001,15.2,-1.23128671800002));
#262965=CARTESIAN_POINT('Ctrl Pts',(-11.0180572970001,11.6,-1.23128671800002));
#262966=CARTESIAN_POINT('Ctrl Pts',(-11.0149481890001,15.2,-1.23210798200001));
#262967=CARTESIAN_POINT('Ctrl Pts',(-11.0149481890001,11.6,-1.23210798200002));
#262968=CARTESIAN_POINT('Ctrl Pts',(-11.0118433650001,15.2,-1.23292544600002));
#262969=CARTESIAN_POINT('Ctrl Pts',(-11.0118433650001,11.6,-1.23292544600002));
#262970=CARTESIAN_POINT('Ctrl Pts',(-11.0087428330001,15.2,-1.23373911600002));
#262971=CARTESIAN_POINT('Ctrl Pts',(-11.0087428330001,11.6,-1.23373911600002));
#262972=CARTESIAN_POINT('Ctrl Pts',(-11.0056466050001,15.2,-1.23454899600001));
#262973=CARTESIAN_POINT('Ctrl Pts',(-11.0056466050001,11.6,-1.23454899600001));
#262974=CARTESIAN_POINT('Ctrl Pts',(-11.0025546900001,15.2,-1.23535509100002));
#262975=CARTESIAN_POINT('Ctrl Pts',(-11.0025546900001,11.6,-1.23535509100002));
#262976=CARTESIAN_POINT('Ctrl Pts',(-10.9994670990001,15.2,-1.23615740600002));
#262977=CARTESIAN_POINT('Ctrl Pts',(-10.9994670990001,11.6,-1.23615740600002));
#262978=CARTESIAN_POINT('Ctrl Pts',(-10.9963838420001,15.2,-1.23695594400001));
#262979=CARTESIAN_POINT('Ctrl Pts',(-10.9963838420001,11.6,-1.23695594400001));
#262980=CARTESIAN_POINT('Ctrl Pts',(-10.9933049300001,15.2,-1.23775071100001));
#262981=CARTESIAN_POINT('Ctrl Pts',(-10.9933049300001,11.6,-1.23775071100001));
#262982=CARTESIAN_POINT('Ctrl Pts',(-10.9902303730001,15.2,-1.23854171100001));
#262983=CARTESIAN_POINT('Ctrl Pts',(-10.9902303730001,11.6,-1.23854171100001));
#262984=CARTESIAN_POINT('Ctrl Pts',(-10.9871601810001,15.2,-1.23932894900001));
#262985=CARTESIAN_POINT('Ctrl Pts',(-10.9871601810001,11.6,-1.23932894900001));
#262986=CARTESIAN_POINT('Ctrl Pts',(-10.9840943650001,15.2,-1.24011242900002));
#262987=CARTESIAN_POINT('Ctrl Pts',(-10.9840943650001,11.6,-1.24011242900002));
#262988=CARTESIAN_POINT('Ctrl Pts',(-10.9810329350001,15.2,-1.24089215700002));
#262989=CARTESIAN_POINT('Ctrl Pts',(-10.9810329350001,11.6,-1.24089215700002));
#262990=CARTESIAN_POINT('Ctrl Pts',(-10.9779759010001,15.2,-1.24166813600001));
#262991=CARTESIAN_POINT('Ctrl Pts',(-10.9779759010001,11.6,-1.24166813600001));
#262992=CARTESIAN_POINT('Ctrl Pts',(-10.9749232750001,15.2,-1.24244037200001));
#262993=CARTESIAN_POINT('Ctrl Pts',(-10.9749232750001,11.6,-1.24244037200001));
#262994=CARTESIAN_POINT('Ctrl Pts',(-10.9718750660001,15.2,-1.24320886800001));
#262995=CARTESIAN_POINT('Ctrl Pts',(-10.9718750660001,11.6,-1.24320886800001));
#262996=CARTESIAN_POINT('Ctrl Pts',(-10.9688312840001,15.2,-1.24397363100002));
#262997=CARTESIAN_POINT('Ctrl Pts',(-10.9688312840001,11.6,-1.24397363100002));
#262998=CARTESIAN_POINT('Ctrl Pts',(-10.9657919420001,15.2,-1.24473466500001));
#262999=CARTESIAN_POINT('Ctrl Pts',(-10.9657919420001,11.6,-1.24473466500001));
#263000=CARTESIAN_POINT('Ctrl Pts',(-10.9627570480001,15.2,-1.24549197300002));
#263001=CARTESIAN_POINT('Ctrl Pts',(-10.9627570480001,11.6,-1.24549197300002));
#263002=CARTESIAN_POINT('Ctrl Pts',(-10.9597266140001,15.2,-1.24624556300001));
#263003=CARTESIAN_POINT('Ctrl Pts',(-10.9597266140001,11.6,-1.24624556300002));
#263004=CARTESIAN_POINT('Ctrl Pts',(-10.9567006500001,15.2,-1.24699543600002));
#263005=CARTESIAN_POINT('Ctrl Pts',(-10.9567006500001,11.6,-1.24699543600002));
#263006=CARTESIAN_POINT('Ctrl Pts',(-10.9536791670001,15.2,-1.24774160000001));
#263007=CARTESIAN_POINT('Ctrl Pts',(-10.9536791670001,11.6,-1.24774160000001));
#263008=CARTESIAN_POINT('Ctrl Pts',(-10.9506621740001,15.2,-1.24848405800002));
#263009=CARTESIAN_POINT('Ctrl Pts',(-10.9506621740001,11.6,-1.24848405800002));
#263010=CARTESIAN_POINT('Ctrl Pts',(-10.9476496840001,15.2,-1.24922281700002));
#263011=CARTESIAN_POINT('Ctrl Pts',(-10.9476496840001,11.6,-1.24922281700002));
#263012=CARTESIAN_POINT('Ctrl Pts',(-10.9446417060001,15.2,-1.24995787900001));
#263013=CARTESIAN_POINT('Ctrl Pts',(-10.9446417060001,11.6,-1.24995787900001));
#263014=CARTESIAN_POINT('Ctrl Pts',(-10.9416382510001,15.2,-1.25068925100001));
#263015=CARTESIAN_POINT('Ctrl Pts',(-10.9416382510001,11.6,-1.25068925100001));
#263016=CARTESIAN_POINT('Ctrl Pts',(-10.9386393310001,15.2,-1.25141693800002));
#263017=CARTESIAN_POINT('Ctrl Pts',(-10.9386393310001,11.6,-1.25141693800002));
#263018=CARTESIAN_POINT('Ctrl Pts',(-10.9356449540001,15.2,-1.25214094400001));
#263019=CARTESIAN_POINT('Ctrl Pts',(-10.9356449540001,11.6,-1.25214094400001));
#263020=CARTESIAN_POINT('Ctrl Pts',(-10.9326551340001,15.2,-1.25286127300001));
#263021=CARTESIAN_POINT('Ctrl Pts',(-10.9326551340001,11.6,-1.25286127300001));
#263022=CARTESIAN_POINT('Ctrl Pts',(-10.9296698780001,15.2,-1.25357793200001));
#263023=CARTESIAN_POINT('Ctrl Pts',(-10.9296698780001,11.6,-1.25357793200001));
#263024=CARTESIAN_POINT('Ctrl Pts',(-10.9266892000001,15.2,-1.25429092500001));
#263025=CARTESIAN_POINT('Ctrl Pts',(-10.9266892000001,11.6,-1.25429092500001));
#263026=CARTESIAN_POINT('Ctrl Pts',(-10.9237131090001,15.2,-1.25500025700001));
#263027=CARTESIAN_POINT('Ctrl Pts',(-10.9237131090001,11.6,-1.25500025700001));
#263028=CARTESIAN_POINT('Ctrl Pts',(-10.9207416170001,15.2,-1.25570593300001));
#263029=CARTESIAN_POINT('Ctrl Pts',(-10.9207416170001,11.6,-1.25570593300001));
#263030=CARTESIAN_POINT('Ctrl Pts',(-10.9177747340001,15.2,-1.25640795900001));
#263031=CARTESIAN_POINT('Ctrl Pts',(-10.9177747340001,11.6,-1.25640795900001));
#263032=CARTESIAN_POINT('Ctrl Pts',(-10.9148124710001,15.2,-1.25710633900002));
#263033=CARTESIAN_POINT('Ctrl Pts',(-10.9148124710001,11.6,-1.25710633900002));
#263034=CARTESIAN_POINT('Ctrl Pts',(-10.9118548380001,15.2,-1.25780107900002));
#263035=CARTESIAN_POINT('Ctrl Pts',(-10.9118548380001,11.6,-1.25780107900002));
#263036=CARTESIAN_POINT('Ctrl Pts',(-10.9089018470001,15.2,-1.25849218200001));
#263037=CARTESIAN_POINT('Ctrl Pts',(-10.9089018470001,11.6,-1.25849218200001));
#263038=CARTESIAN_POINT('Ctrl Pts',(-10.9059535100001,15.2,-1.25917965600001));
#263039=CARTESIAN_POINT('Ctrl Pts',(-10.9059535100001,11.6,-1.25917965600001));
#263040=CARTESIAN_POINT('Ctrl Pts',(-10.9030098350001,15.2,-1.25986350400002));
#263041=CARTESIAN_POINT('Ctrl Pts',(-10.9030098350001,11.6,-1.25986350400002));
#263042=CARTESIAN_POINT('Ctrl Pts',(-10.9000708340001,15.2,-1.26054373200001));
#263043=CARTESIAN_POINT('Ctrl Pts',(-10.9000708340001,11.6,-1.26054373200002));
#263044=CARTESIAN_POINT('Ctrl Pts',(-10.8971365200001,15.2,-1.26122034700002));
#263045=CARTESIAN_POINT('Ctrl Pts',(-10.8971365200001,11.6,-1.26122034700002));
#263046=CARTESIAN_POINT('Ctrl Pts',(-10.8942069010001,15.2,-1.26189335000001));
#263047=CARTESIAN_POINT('Ctrl Pts',(-10.8942069010001,11.6,-1.26189335000001));
#263048=CARTESIAN_POINT('Ctrl Pts',(-10.8912819900001,15.2,-1.26256275000001));
#263049=CARTESIAN_POINT('Ctrl Pts',(-10.8912819900001,11.6,-1.26256275000001));
#263050=CARTESIAN_POINT('Ctrl Pts',(-10.8883617980001,15.2,-1.26322855100002));
#263051=CARTESIAN_POINT('Ctrl Pts',(-10.8883617980001,11.6,-1.26322855100002));
#263052=CARTESIAN_POINT('Ctrl Pts',(-10.8854463350001,15.2,-1.26389075700001));
#263053=CARTESIAN_POINT('Ctrl Pts',(-10.8854463350001,11.6,-1.26389075700002));
#263054=CARTESIAN_POINT('Ctrl Pts',(-10.8825356130001,15.2,-1.26454937500001));
#263055=CARTESIAN_POINT('Ctrl Pts',(-10.8825356130001,11.6,-1.26454937500002));
#263056=CARTESIAN_POINT('Ctrl Pts',(-10.8796296420001,15.2,-1.26520441000002));
#263057=CARTESIAN_POINT('Ctrl Pts',(-10.8796296420001,11.6,-1.26520441000002));
#263058=CARTESIAN_POINT('Ctrl Pts',(-10.8767284330001,15.2,-1.26585586700001));
#263059=CARTESIAN_POINT('Ctrl Pts',(-10.8767284330001,11.6,-1.26585586700001));
#263060=CARTESIAN_POINT('Ctrl Pts',(-10.8738319990001,15.2,-1.26650375200001));
#263061=CARTESIAN_POINT('Ctrl Pts',(-10.8738319990001,11.6,-1.26650375200001));
#263062=CARTESIAN_POINT('Ctrl Pts',(-10.8709403490001,15.2,-1.26714806900001));
#263063=CARTESIAN_POINT('Ctrl Pts',(-10.8709403490001,11.6,-1.26714806900001));
#263064=CARTESIAN_POINT('Ctrl Pts',(-10.8680534960001,15.2,-1.26778882500002));
#263065=CARTESIAN_POINT('Ctrl Pts',(-10.8680534960001,11.6,-1.26778882500002));
#263066=CARTESIAN_POINT('Ctrl Pts',(-10.8651714500001,15.2,-1.26842602400002));
#263067=CARTESIAN_POINT('Ctrl Pts',(-10.8651714500001,11.6,-1.26842602400002));
#263068=CARTESIAN_POINT('Ctrl Pts',(-10.8622942230001,15.2,-1.26905967200001));
#263069=CARTESIAN_POINT('Ctrl Pts',(-10.8622942230001,11.6,-1.26905967200001));
#263070=CARTESIAN_POINT('Ctrl Pts',(-10.8594218250001,15.2,-1.26968977500002));
#263071=CARTESIAN_POINT('Ctrl Pts',(-10.8594218250001,11.6,-1.26968977500002));
#263072=CARTESIAN_POINT('Ctrl Pts',(-10.8565542680001,15.2,-1.27031633800001));
#263073=CARTESIAN_POINT('Ctrl Pts',(-10.8565542680001,11.6,-1.27031633800002));
#263074=CARTESIAN_POINT('Ctrl Pts',(-10.8536915640001,15.2,-1.27093936700001));
#263075=CARTESIAN_POINT('Ctrl Pts',(-10.8536915640001,11.6,-1.27093936700002));
#263076=CARTESIAN_POINT('Ctrl Pts',(-10.8508337230001,15.2,-1.27155886700002));
#263077=CARTESIAN_POINT('Ctrl Pts',(-10.8508337230001,11.6,-1.27155886700002));
#263078=CARTESIAN_POINT('Ctrl Pts',(-10.8479807570001,15.2,-1.27217484400001));
#263079=CARTESIAN_POINT('Ctrl Pts',(-10.8479807570001,11.6,-1.27217484400001));
#263080=CARTESIAN_POINT('Ctrl Pts',(-10.8451326780001,15.2,-1.27278730200001));
#263081=CARTESIAN_POINT('Ctrl Pts',(-10.8451326780001,11.6,-1.27278730200001));
#263082=CARTESIAN_POINT('Ctrl Pts',(-10.8422894960001,15.2,-1.27339624800001));
#263083=CARTESIAN_POINT('Ctrl Pts',(-10.8422894960001,11.6,-1.27339624800001));
#263084=CARTESIAN_POINT('Ctrl Pts',(-10.8394512230001,15.2,-1.27400168700001));
#263085=CARTESIAN_POINT('Ctrl Pts',(-10.8394512230001,11.6,-1.27400168700001));
#263086=CARTESIAN_POINT('Ctrl Pts',(-10.8366178710001,15.2,-1.27460362600001));
#263087=CARTESIAN_POINT('Ctrl Pts',(-10.8366178710001,11.6,-1.27460362600001));
#263088=CARTESIAN_POINT('Ctrl Pts',(-10.8337894500001,15.2,-1.27520207000002));
#263089=CARTESIAN_POINT('Ctrl Pts',(-10.8337894500001,11.6,-1.27520207000002));
#263090=CARTESIAN_POINT('Ctrl Pts',(-10.8309659720001,15.2,-1.27579702400002));
#263091=CARTESIAN_POINT('Ctrl Pts',(-10.8309659720001,11.6,-1.27579702400002));
#263092=CARTESIAN_POINT('Ctrl Pts',(-10.8281474500001,15.2,-1.27638849300002));
#263093=CARTESIAN_POINT('Ctrl Pts',(-10.8281474500001,11.6,-1.27638849300002));
#263094=CARTESIAN_POINT('Ctrl Pts',(-10.8253338940001,15.2,-1.27697648500002));
#263095=CARTESIAN_POINT('Ctrl Pts',(-10.8253338940001,11.6,-1.27697648500002));
#263096=CARTESIAN_POINT('Ctrl Pts',(-10.8225253160001,15.2,-1.27756100400001));
#263097=CARTESIAN_POINT('Ctrl Pts',(-10.8225253160001,11.6,-1.27756100400001));
#263098=CARTESIAN_POINT('Ctrl Pts',(-10.8197217270001,15.2,-1.27814205700002));
#263099=CARTESIAN_POINT('Ctrl Pts',(-10.8197217270001,11.6,-1.27814205700002));
#263100=CARTESIAN_POINT('Ctrl Pts',(-10.8169231390001,15.2,-1.27871964900002));
#263101=CARTESIAN_POINT('Ctrl Pts',(-10.8169231390001,11.6,-1.27871964900002));
#263102=CARTESIAN_POINT('Ctrl Pts',(-10.8141295640001,15.2,-1.27929378400002));
#263103=CARTESIAN_POINT('Ctrl Pts',(-10.8141295640001,11.6,-1.27929378400002));
#263104=CARTESIAN_POINT('Ctrl Pts',(-10.8113410120001,15.2,-1.27986447200001));
#263105=CARTESIAN_POINT('Ctrl Pts',(-10.8113410120001,11.6,-1.27986447200001));
#263106=CARTESIAN_POINT('Ctrl Pts',(-10.8085574970001,15.2,-1.28043171600002));
#263107=CARTESIAN_POINT('Ctrl Pts',(-10.8085574970001,11.6,-1.28043171600002));
#263108=CARTESIAN_POINT('Ctrl Pts',(-10.8057790290001,15.2,-1.28099552100001));
#263109=CARTESIAN_POINT('Ctrl Pts',(-10.8057790290001,11.6,-1.28099552100002));
#263110=CARTESIAN_POINT('Ctrl Pts',(-10.8030056200001,15.2,-1.28155589700001));
#263111=CARTESIAN_POINT('Ctrl Pts',(-10.8030056200001,11.6,-1.28155589700001));
#263112=CARTESIAN_POINT('Ctrl Pts',(-10.8002372820001,15.2,-1.28211284500001));
#263113=CARTESIAN_POINT('Ctrl Pts',(-10.8002372820001,11.6,-1.28211284500001));
#263114=CARTESIAN_POINT('Ctrl Pts',(-10.7974740270001,15.2,-1.28266637400001));
#263115=CARTESIAN_POINT('Ctrl Pts',(-10.7974740270001,11.6,-1.28266637400001));
#263116=CARTESIAN_POINT('Ctrl Pts',(-10.7947158660001,15.2,-1.28321649000001));
#263117=CARTESIAN_POINT('Ctrl Pts',(-10.7947158660001,11.6,-1.28321649000001));
#263118=CARTESIAN_POINT('Ctrl Pts',(-10.7919628110001,15.2,-1.28376319800001));
#263119=CARTESIAN_POINT('Ctrl Pts',(-10.7919628110001,11.6,-1.28376319800001));
#263120=CARTESIAN_POINT('Ctrl Pts',(-10.7892148740001,15.2,-1.28430650300002));
#263121=CARTESIAN_POINT('Ctrl Pts',(-10.7892148740001,11.6,-1.28430650300002));
#263122=CARTESIAN_POINT('Ctrl Pts',(-10.7864720660001,15.2,-1.28484641300001));
#263123=CARTESIAN_POINT('Ctrl Pts',(-10.7864720660001,11.6,-1.28484641300001));
#263124=CARTESIAN_POINT('Ctrl Pts',(-10.7837344010001,15.2,-1.28538293400001));
#263125=CARTESIAN_POINT('Ctrl Pts',(-10.7837344010001,11.6,-1.28538293400001));
#263126=CARTESIAN_POINT('Ctrl Pts',(-10.7810018880001,15.2,-1.28591607100002));
#263127=CARTESIAN_POINT('Ctrl Pts',(-10.7810018880001,11.6,-1.28591607100002));
#263128=CARTESIAN_POINT('Ctrl Pts',(-10.7782745420001,15.2,-1.28644583000002));
#263129=CARTESIAN_POINT('Ctrl Pts',(-10.7782745420001,11.6,-1.28644583000002));
#263130=CARTESIAN_POINT('Ctrl Pts',(-10.7755523730001,15.2,-1.28697221800001));
#263131=CARTESIAN_POINT('Ctrl Pts',(-10.7755523730001,11.6,-1.28697221800001));
#263132=CARTESIAN_POINT('Ctrl Pts',(-10.7728353940001,15.2,-1.28749524100002));
#263133=CARTESIAN_POINT('Ctrl Pts',(-10.7728353940001,11.6,-1.28749524100002));
#263134=CARTESIAN_POINT('Ctrl Pts',(-10.7701236150001,15.2,-1.28801490500001));
#263135=CARTESIAN_POINT('Ctrl Pts',(-10.7701236150001,11.6,-1.28801490500001));
#263136=CARTESIAN_POINT('Ctrl Pts',(-10.7674170490001,15.2,-1.28853121600002));
#263137=CARTESIAN_POINT('Ctrl Pts',(-10.7674170490001,11.6,-1.28853121600002));
#263138=CARTESIAN_POINT('Ctrl Pts',(-10.7647157090001,15.2,-1.28904418000001));
#263139=CARTESIAN_POINT('Ctrl Pts',(-10.7647157090001,11.6,-1.28904418000001));
#263140=CARTESIAN_POINT('Ctrl Pts',(-10.7620196070001,15.2,-1.28955380500001));
#263141=CARTESIAN_POINT('Ctrl Pts',(-10.7620196070001,11.6,-1.28955380500001));
#263142=CARTESIAN_POINT('Ctrl Pts',(-10.7593287540001,15.2,-1.29006009500001));
#263143=CARTESIAN_POINT('Ctrl Pts',(-10.7593287540001,11.6,-1.29006009500001));
#263144=CARTESIAN_POINT('Ctrl Pts',(-10.7566431620001,15.2,-1.29056305800002));
#263145=CARTESIAN_POINT('Ctrl Pts',(-10.7566431620001,11.6,-1.29056305800002));
#263146=CARTESIAN_POINT('Ctrl Pts',(-10.7539628450001,15.2,-1.29106270000001));
#263147=CARTESIAN_POINT('Ctrl Pts',(-10.7539628450001,11.6,-1.29106270000001));
#263148=CARTESIAN_POINT('Ctrl Pts',(-10.7512878130001,15.2,-1.29155902600001));
#263149=CARTESIAN_POINT('Ctrl Pts',(-10.7512878130001,11.6,-1.29155902600001));
#263150=CARTESIAN_POINT('Ctrl Pts',(-10.7486180790001,15.2,-1.29205204400002));
#263151=CARTESIAN_POINT('Ctrl Pts',(-10.7486180790001,11.6,-1.29205204400002));
#263152=CARTESIAN_POINT('Ctrl Pts',(-10.7459536560001,15.2,-1.29254175900002));
#263153=CARTESIAN_POINT('Ctrl Pts',(-10.7459536560001,11.6,-1.29254175900002));
#263154=CARTESIAN_POINT('Ctrl Pts',(-10.7432945550001,15.2,-1.29302817900002));
#263155=CARTESIAN_POINT('Ctrl Pts',(-10.7432945550001,11.6,-1.29302817900002));
#263156=CARTESIAN_POINT('Ctrl Pts',(-10.7406407890001,15.2,-1.29351131000002));
#263157=CARTESIAN_POINT('Ctrl Pts',(-10.7406407890001,11.6,-1.29351131000002));
#263158=CARTESIAN_POINT('Ctrl Pts',(-10.7379923700001,15.2,-1.29399115700001));
#263159=CARTESIAN_POINT('Ctrl Pts',(-10.7379923700001,11.6,-1.29399115700001));
#263160=CARTESIAN_POINT('Ctrl Pts',(-10.7353493100001,15.2,-1.29446772800001));
#263161=CARTESIAN_POINT('Ctrl Pts',(-10.7353493100001,11.6,-1.29446772800002));
#263162=CARTESIAN_POINT('Ctrl Pts',(-10.7327116220001,15.2,-1.29494103100001));
#263163=CARTESIAN_POINT('Ctrl Pts',(-10.7327116220001,11.6,-1.29494103100001));
#263164=CARTESIAN_POINT('Ctrl Pts',(-10.7300793190001,15.2,-1.29541106900001));
#263165=CARTESIAN_POINT('Ctrl Pts',(-10.7300793190001,11.6,-1.29541106900001));
#263166=CARTESIAN_POINT('Ctrl Pts',(-10.7274524110001,15.2,-1.29587785100002));
#263167=CARTESIAN_POINT('Ctrl Pts',(-10.7274524110001,11.6,-1.29587785100002));
#263168=CARTESIAN_POINT('Ctrl Pts',(-10.7248309140001,15.2,-1.29634138200001));
#263169=CARTESIAN_POINT('Ctrl Pts',(-10.7248309140001,11.6,-1.29634138200002));
#263170=CARTESIAN_POINT('Ctrl Pts',(-10.7222148360001,15.2,-1.29680167100001));
#263171=CARTESIAN_POINT('Ctrl Pts',(-10.7222148360001,11.6,-1.29680167100001));
#263172=CARTESIAN_POINT('Ctrl Pts',(-10.7196041930001,15.2,-1.29725872300002));
#263173=CARTESIAN_POINT('Ctrl Pts',(-10.7196041930001,11.6,-1.29725872300002));
#263174=CARTESIAN_POINT('Ctrl Pts',(-10.7169989970001,15.2,-1.29771254400001));
#263175=CARTESIAN_POINT('Ctrl Pts',(-10.7169989970001,11.6,-1.29771254400001));
#263176=CARTESIAN_POINT('Ctrl Pts',(-10.7143992590001,15.2,-1.29816314300002));
#263177=CARTESIAN_POINT('Ctrl Pts',(-10.7143992590001,11.6,-1.29816314300002));
#263178=CARTESIAN_POINT('Ctrl Pts',(-10.7118049930001,15.2,-1.29861052400001));
#263179=CARTESIAN_POINT('Ctrl Pts',(-10.7118049930001,11.6,-1.29861052400001));
#263180=CARTESIAN_POINT('Ctrl Pts',(-10.7092162110001,15.2,-1.29905469600001));
#263181=CARTESIAN_POINT('Ctrl Pts',(-10.7092162110001,11.6,-1.29905469600002));
#263182=CARTESIAN_POINT('Ctrl Pts',(-10.7066329250001,15.2,-1.29949566500001));
#263183=CARTESIAN_POINT('Ctrl Pts',(-10.7066329250001,11.6,-1.29949566500001));
#263184=CARTESIAN_POINT('Ctrl Pts',(-10.7040551500001,15.2,-1.29993343800002));
#263185=CARTESIAN_POINT('Ctrl Pts',(-10.7040551500001,11.6,-1.29993343800002));
#263186=CARTESIAN_POINT('Ctrl Pts',(-10.7014828960001,15.2,-1.30036802200001));
#263187=CARTESIAN_POINT('Ctrl Pts',(-10.7014828960001,11.6,-1.30036802200001));
#263188=CARTESIAN_POINT('Ctrl Pts',(-10.6989161770001,15.2,-1.30079942300001));
#263189=CARTESIAN_POINT('Ctrl Pts',(-10.6989161770001,11.6,-1.30079942300001));
#263190=CARTESIAN_POINT('Ctrl Pts',(-10.6963550050001,15.2,-1.30122764900001));
#263191=CARTESIAN_POINT('Ctrl Pts',(-10.6963550050001,11.6,-1.30122764900001));
#263192=CARTESIAN_POINT('Ctrl Pts',(-10.6937993940001,15.2,-1.30165270500001));
#263193=CARTESIAN_POINT('Ctrl Pts',(-10.6937993940001,11.6,-1.30165270500001));
#263194=CARTESIAN_POINT('Ctrl Pts',(-10.6912493550001,15.2,-1.30207460100001));
#263195=CARTESIAN_POINT('Ctrl Pts',(-10.6912493550001,11.6,-1.30207460100001));
#263196=CARTESIAN_POINT('Ctrl Pts',(-10.6887049020001,15.2,-1.30249334200002));
#263197=CARTESIAN_POINT('Ctrl Pts',(-10.6887049020001,11.6,-1.30249334200002));
#263198=CARTESIAN_POINT('Ctrl Pts',(-10.6861660490001,15.2,-1.30290893500002));
#263199=CARTESIAN_POINT('Ctrl Pts',(-10.6861660490001,11.6,-1.30290893500002));
#263200=CARTESIAN_POINT('Ctrl Pts',(-10.6836328060001,15.2,-1.30332138700001));
#263201=CARTESIAN_POINT('Ctrl Pts',(-10.6836328060001,11.6,-1.30332138700001));
#263202=CARTESIAN_POINT('Ctrl Pts',(-10.6811051890001,15.2,-1.30373070700001));
#263203=CARTESIAN_POINT('Ctrl Pts',(-10.6811051890001,11.6,-1.30373070700002));
#263204=CARTESIAN_POINT('Ctrl Pts',(-10.6785832090001,15.2,-1.30413690000001));
#263205=CARTESIAN_POINT('Ctrl Pts',(-10.6785832090001,11.6,-1.30413690000002));
#263206=CARTESIAN_POINT('Ctrl Pts',(-10.6760668780001,15.2,-1.30453997300001));
#263207=CARTESIAN_POINT('Ctrl Pts',(-10.6760668780001,11.6,-1.30453997300001));
#263208=CARTESIAN_POINT('Ctrl Pts',(-10.6735562130001,15.2,-1.30493993500002));
#263209=CARTESIAN_POINT('Ctrl Pts',(-10.6735562130001,11.6,-1.30493993500002));
#263210=CARTESIAN_POINT('Ctrl Pts',(-10.6710512220001,15.2,-1.30533679100001));
#263211=CARTESIAN_POINT('Ctrl Pts',(-10.6710512220001,11.6,-1.30533679100001));
#263212=CARTESIAN_POINT('Ctrl Pts',(-10.6685519220001,15.2,-1.30573054900001));
#263213=CARTESIAN_POINT('Ctrl Pts',(-10.6685519220001,11.6,-1.30573054900002));
#263214=CARTESIAN_POINT('Ctrl Pts',(-10.6660583240001,15.2,-1.30612121800001));
#263215=CARTESIAN_POINT('Ctrl Pts',(-10.6660583240001,11.6,-1.30612121800001));
#263216=CARTESIAN_POINT('Ctrl Pts',(-10.6635704410001,15.2,-1.30650880300001));
#263217=CARTESIAN_POINT('Ctrl Pts',(-10.6635704410001,11.6,-1.30650880300002));
#263218=CARTESIAN_POINT('Ctrl Pts',(-10.6610882880001,15.2,-1.30689331200001));
#263219=CARTESIAN_POINT('Ctrl Pts',(-10.6610882880001,11.6,-1.30689331200002));
#263220=CARTESIAN_POINT('Ctrl Pts',(-10.6586118770001,15.2,-1.30727475400001));
#263221=CARTESIAN_POINT('Ctrl Pts',(-10.6586118770001,11.6,-1.30727475400001));
#263222=CARTESIAN_POINT('Ctrl Pts',(-10.6561412200001,15.2,-1.30765313300001));
#263223=CARTESIAN_POINT('Ctrl Pts',(-10.6561412200001,11.6,-1.30765313300001));
#263224=CARTESIAN_POINT('Ctrl Pts',(-10.6536763330001,15.2,-1.30802845900002));
#263225=CARTESIAN_POINT('Ctrl Pts',(-10.6536763330001,11.6,-1.30802845900002));
#263226=CARTESIAN_POINT('Ctrl Pts',(-10.6512172270001,15.2,-1.30840073900002));
#263227=CARTESIAN_POINT('Ctrl Pts',(-10.6512172270001,11.6,-1.30840073900002));
#263228=CARTESIAN_POINT('Ctrl Pts',(-10.6487639160001,15.2,-1.30876997900002));
#263229=CARTESIAN_POINT('Ctrl Pts',(-10.6487639160001,11.6,-1.30876997900002));
#263230=CARTESIAN_POINT('Ctrl Pts',(-10.6463164150001,15.2,-1.30913618800002));
#263231=CARTESIAN_POINT('Ctrl Pts',(-10.6463164150001,11.6,-1.30913618800002));
#263232=CARTESIAN_POINT('Ctrl Pts',(-10.6438747330001,15.2,-1.30949937400001));
#263233=CARTESIAN_POINT('Ctrl Pts',(-10.6438747330001,11.6,-1.30949937400001));
#263234=CARTESIAN_POINT('Ctrl Pts',(-10.6414388880001,15.2,-1.30985954200002));
#263235=CARTESIAN_POINT('Ctrl Pts',(-10.6414388880001,11.6,-1.30985954200002));
#263236=CARTESIAN_POINT('Ctrl Pts',(-10.6390088920001,15.2,-1.31021670200001));
#263237=CARTESIAN_POINT('Ctrl Pts',(-10.6390088920001,11.6,-1.31021670200001));
#263238=CARTESIAN_POINT('Ctrl Pts',(-10.6365847570001,15.2,-1.31057086100002));
#263239=CARTESIAN_POINT('Ctrl Pts',(-10.6365847570001,11.6,-1.31057086100002));
#263240=CARTESIAN_POINT('Ctrl Pts',(-10.6341664980001,15.2,-1.31092202700001));
#263241=CARTESIAN_POINT('Ctrl Pts',(-10.6341664980001,11.6,-1.31092202700001));
#263242=CARTESIAN_POINT('Ctrl Pts',(-10.6317541280001,15.2,-1.31127020600001));
#263243=CARTESIAN_POINT('Ctrl Pts',(-10.6317541280001,11.6,-1.31127020600002));
#263244=CARTESIAN_POINT('Ctrl Pts',(-10.6293476610001,15.2,-1.31161540800001));
#263245=CARTESIAN_POINT('Ctrl Pts',(-10.6293476610001,11.6,-1.31161540800001));
#263246=CARTESIAN_POINT('Ctrl Pts',(-10.6269471100001,15.2,-1.31195763900001));
#263247=CARTESIAN_POINT('Ctrl Pts',(-10.6269471100001,11.6,-1.31195763900001));
#263248=CARTESIAN_POINT('Ctrl Pts',(-10.6245524890001,15.2,-1.31229690700001));
#263249=CARTESIAN_POINT('Ctrl Pts',(-10.6245524890001,11.6,-1.31229690700002));
#263250=CARTESIAN_POINT('Ctrl Pts',(-10.6221638120001,15.2,-1.31263322000001));
#263251=CARTESIAN_POINT('Ctrl Pts',(-10.6221638120001,11.6,-1.31263322000002));
#263252=CARTESIAN_POINT('Ctrl Pts',(-10.6197810910001,15.2,-1.31296658600002));
#263253=CARTESIAN_POINT('Ctrl Pts',(-10.6197810910001,11.6,-1.31296658600002));
#263254=CARTESIAN_POINT('Ctrl Pts',(-10.6174043430001,15.2,-1.31329701400002));
#263255=CARTESIAN_POINT('Ctrl Pts',(-10.6174043430001,11.6,-1.31329701400002));
#263256=CARTESIAN_POINT('Ctrl Pts',(-10.6150335790001,15.2,-1.31362450900002));
#263257=CARTESIAN_POINT('Ctrl Pts',(-10.6150335790001,11.6,-1.31362450900002));
#263258=CARTESIAN_POINT('Ctrl Pts',(-10.6126688130001,15.2,-1.31394908200001));
#263259=CARTESIAN_POINT('Ctrl Pts',(-10.6126688130001,11.6,-1.31394908200001));
#263260=CARTESIAN_POINT('Ctrl Pts',(-10.6103100600001,15.2,-1.31427073900001));
#263261=CARTESIAN_POINT('Ctrl Pts',(-10.6103100600001,11.6,-1.31427073900001));
#263262=CARTESIAN_POINT('Ctrl Pts',(-10.6079573330001,15.2,-1.31458948800002));
#263263=CARTESIAN_POINT('Ctrl Pts',(-10.6079573330001,11.6,-1.31458948800002));
#263264=CARTESIAN_POINT('Ctrl Pts',(-10.6056106460001,15.2,-1.31490533800001));
#263265=CARTESIAN_POINT('Ctrl Pts',(-10.6056106460001,11.6,-1.31490533800001));
#263266=CARTESIAN_POINT('Ctrl Pts',(-10.6032700140001,15.2,-1.31521829600001));
#263267=CARTESIAN_POINT('Ctrl Pts',(-10.6032700140001,11.6,-1.31521829600001));
#263268=CARTESIAN_POINT('Ctrl Pts',(-10.6009354490001,15.2,-1.31552837200001));
#263269=CARTESIAN_POINT('Ctrl Pts',(-10.6009354490001,11.6,-1.31552837200001));
#263270=CARTESIAN_POINT('Ctrl Pts',(-10.5986069670001,15.2,-1.31583557100001));
#263271=CARTESIAN_POINT('Ctrl Pts',(-10.5986069670001,11.6,-1.31583557100001));
#263272=CARTESIAN_POINT('Ctrl Pts',(-10.5962845810001,15.2,-1.31613990400002));
#263273=CARTESIAN_POINT('Ctrl Pts',(-10.5962845810001,11.6,-1.31613990400002));
#263274=CARTESIAN_POINT('Ctrl Pts',(-10.5939683050001,15.2,-1.31644137800001));
#263275=CARTESIAN_POINT('Ctrl Pts',(-10.5939683050001,11.6,-1.31644137800001));
#263276=CARTESIAN_POINT('Ctrl Pts',(-10.5916581540001,15.2,-1.31674000200002));
#263277=CARTESIAN_POINT('Ctrl Pts',(-10.5916581540001,11.6,-1.31674000200002));
#263278=CARTESIAN_POINT('Ctrl Pts',(-10.5893541410001,15.2,-1.31703578300002));
#263279=CARTESIAN_POINT('Ctrl Pts',(-10.5893541410001,11.6,-1.31703578300002));
#263280=CARTESIAN_POINT('Ctrl Pts',(-10.5870562810001,15.2,-1.31732872900002));
#263281=CARTESIAN_POINT('Ctrl Pts',(-10.5870562810001,11.6,-1.31732872900002));
#263282=CARTESIAN_POINT('Ctrl Pts',(-10.5847645880001,15.2,-1.31761885100001));
#263283=CARTESIAN_POINT('Ctrl Pts',(-10.5847645880001,11.6,-1.31761885100001));
#263284=CARTESIAN_POINT('Ctrl Pts',(-10.5824790750001,15.2,-1.31790615500002));
#263285=CARTESIAN_POINT('Ctrl Pts',(-10.5824790750001,11.6,-1.31790615500002));
#263286=CARTESIAN_POINT('Ctrl Pts',(-10.5801997580001,15.2,-1.31819064900002));
#263287=CARTESIAN_POINT('Ctrl Pts',(-10.5801997580001,11.6,-1.31819064900002));
#263288=CARTESIAN_POINT('Ctrl Pts',(-10.5779266520001,15.2,-1.31847234300002));
#263289=CARTESIAN_POINT('Ctrl Pts',(-10.5779266520001,11.6,-1.31847234300002));
#263290=CARTESIAN_POINT('Ctrl Pts',(-10.5756597690001,15.2,-1.31875124500001));
#263291=CARTESIAN_POINT('Ctrl Pts',(-10.5756597690001,11.6,-1.31875124500001));
#263292=CARTESIAN_POINT('Ctrl Pts',(-10.5733991250001,15.2,-1.31902736300002));
#263293=CARTESIAN_POINT('Ctrl Pts',(-10.5733991250001,11.6,-1.31902736300002));
#263294=CARTESIAN_POINT('Ctrl Pts',(-10.5711447350001,15.2,-1.31930070600002));
#263295=CARTESIAN_POINT('Ctrl Pts',(-10.5711447350001,11.6,-1.31930070600002));
#263296=CARTESIAN_POINT('Ctrl Pts',(-10.5688966110001,15.2,-1.31957128200002));
#263297=CARTESIAN_POINT('Ctrl Pts',(-10.5688966110001,11.6,-1.31957128200002));
#263298=CARTESIAN_POINT('Ctrl Pts',(-10.5666547700001,15.2,-1.31983910100002));
#263299=CARTESIAN_POINT('Ctrl Pts',(-10.5666547700001,11.6,-1.31983910100002));
#263300=CARTESIAN_POINT('Ctrl Pts',(-10.5644192250001,15.2,-1.32010417000001));
#263301=CARTESIAN_POINT('Ctrl Pts',(-10.5644192250001,11.6,-1.32010417000001));
#263302=CARTESIAN_POINT('Ctrl Pts',(-10.5621899910001,15.2,-1.32036649800002));
#263303=CARTESIAN_POINT('Ctrl Pts',(-10.5621899910001,11.6,-1.32036649800002));
#263304=CARTESIAN_POINT('Ctrl Pts',(-10.5599670840001,15.2,-1.32062609500001));
#263305=CARTESIAN_POINT('Ctrl Pts',(-10.5599670840001,11.6,-1.32062609500002));
#263306=CARTESIAN_POINT('Ctrl Pts',(-10.5577505170001,15.2,-1.32088296800001));
#263307=CARTESIAN_POINT('Ctrl Pts',(-10.5577505170001,11.6,-1.32088296800001));
#263308=CARTESIAN_POINT('Ctrl Pts',(-10.5555403050001,15.2,-1.32113712700002));
#263309=CARTESIAN_POINT('Ctrl Pts',(-10.5555403050001,11.6,-1.32113712700002));
#263310=CARTESIAN_POINT('Ctrl Pts',(-10.5533364630001,15.2,-1.32138858100001));
#263311=CARTESIAN_POINT('Ctrl Pts',(-10.5533364630001,11.6,-1.32138858100001));
#263312=CARTESIAN_POINT('Ctrl Pts',(-10.5511390070001,15.2,-1.32163733700001));
#263313=CARTESIAN_POINT('Ctrl Pts',(-10.5511390070001,11.6,-1.32163733700001));
#263314=CARTESIAN_POINT('Ctrl Pts',(-10.5489479500001,15.2,-1.32188340500001));
#263315=CARTESIAN_POINT('Ctrl Pts',(-10.5489479500001,11.6,-1.32188340500001));
#263316=CARTESIAN_POINT('Ctrl Pts',(-10.5467633070001,15.2,-1.32212679400002));
#263317=CARTESIAN_POINT('Ctrl Pts',(-10.5467633070001,11.6,-1.32212679400002));
#263318=CARTESIAN_POINT('Ctrl Pts',(-10.5445850930001,15.2,-1.32236751500002));
#263319=CARTESIAN_POINT('Ctrl Pts',(-10.5445850930001,11.6,-1.32236751500002));
#263320=CARTESIAN_POINT('Ctrl Pts',(-10.5424133250001,15.2,-1.32260557300001));
#263321=CARTESIAN_POINT('Ctrl Pts',(-10.5424133250001,11.6,-1.32260557300001));
#263322=CARTESIAN_POINT('Ctrl Pts',(-10.5402480150001,15.2,-1.32284098000001));
#263323=CARTESIAN_POINT('Ctrl Pts',(-10.5402480150001,11.6,-1.32284098000001));
#263324=CARTESIAN_POINT('Ctrl Pts',(-10.5380891800001,15.2,-1.32307374300002));
#263325=CARTESIAN_POINT('Ctrl Pts',(-10.5380891800001,11.6,-1.32307374300002));
#263326=CARTESIAN_POINT('Ctrl Pts',(-10.5359368350001,15.2,-1.32330387300001));
#263327=CARTESIAN_POINT('Ctrl Pts',(-10.5359368350001,11.6,-1.32330387300002));
#263328=CARTESIAN_POINT('Ctrl Pts',(-10.5337909930001,15.2,-1.32353137900001));
#263329=CARTESIAN_POINT('Ctrl Pts',(-10.5337909930001,11.6,-1.32353137900001));
#263330=CARTESIAN_POINT('Ctrl Pts',(-10.5316516720001,15.2,-1.32375626900001));
#263331=CARTESIAN_POINT('Ctrl Pts',(-10.5316516720001,11.6,-1.32375626900001));
#263332=CARTESIAN_POINT('Ctrl Pts',(-10.5295188860001,15.2,-1.32397855400002));
#263333=CARTESIAN_POINT('Ctrl Pts',(-10.5295188860001,11.6,-1.32397855400002));
#263334=CARTESIAN_POINT('Ctrl Pts',(-10.5273926510001,15.2,-1.32419824100001));
#263335=CARTESIAN_POINT('Ctrl Pts',(-10.5273926510001,11.6,-1.32419824100001));
#263336=CARTESIAN_POINT('Ctrl Pts',(-10.5252729800001,15.2,-1.32441534000002));
#263337=CARTESIAN_POINT('Ctrl Pts',(-10.5252729800001,11.6,-1.32441534000002));
#263338=CARTESIAN_POINT('Ctrl Pts',(-10.5231598910001,15.2,-1.32462986200002));
#263339=CARTESIAN_POINT('Ctrl Pts',(-10.5231598910001,11.6,-1.32462986200002));
#263340=CARTESIAN_POINT('Ctrl Pts',(-10.5210533970001,15.2,-1.32484181400002));
#263341=CARTESIAN_POINT('Ctrl Pts',(-10.5210533970001,11.6,-1.32484181400002));
#263342=CARTESIAN_POINT('Ctrl Pts',(-10.5189535150001,15.2,-1.32505120800001));
#263343=CARTESIAN_POINT('Ctrl Pts',(-10.5189535150001,11.6,-1.32505120800001));
#263344=CARTESIAN_POINT('Ctrl Pts',(-10.5168602610001,15.2,-1.32525805100002));
#263345=CARTESIAN_POINT('Ctrl Pts',(-10.5168602610001,11.6,-1.32525805100002));
#263346=CARTESIAN_POINT('Ctrl Pts',(-10.5147736500001,15.2,-1.32546235400001));
#263347=CARTESIAN_POINT('Ctrl Pts',(-10.5147736500001,11.6,-1.32546235400001));
#263348=CARTESIAN_POINT('Ctrl Pts',(-10.5126936960001,15.2,-1.32566412600001));
#263349=CARTESIAN_POINT('Ctrl Pts',(-10.5126936960001,11.6,-1.32566412600002));
#263350=CARTESIAN_POINT('Ctrl Pts',(-10.5106204160001,15.2,-1.32586337800001));
#263351=CARTESIAN_POINT('Ctrl Pts',(-10.5106204160001,11.6,-1.32586337800001));
#263352=CARTESIAN_POINT('Ctrl Pts',(-10.5085538250001,15.2,-1.32606011700001));
#263353=CARTESIAN_POINT('Ctrl Pts',(-10.5085538250001,11.6,-1.32606011700001));
#263354=CARTESIAN_POINT('Ctrl Pts',(-10.5064939400001,15.2,-1.32625435500001));
#263355=CARTESIAN_POINT('Ctrl Pts',(-10.5064939400001,11.6,-1.32625435500001));
#263356=CARTESIAN_POINT('Ctrl Pts',(-10.5044407750001,15.2,-1.32644610000002));
#263357=CARTESIAN_POINT('Ctrl Pts',(-10.5044407750001,11.6,-1.32644610000002));
#263358=CARTESIAN_POINT('Ctrl Pts',(-10.5023943470001,15.2,-1.32663536300001));
#263359=CARTESIAN_POINT('Ctrl Pts',(-10.5023943470001,11.6,-1.32663536300001));
#263360=CARTESIAN_POINT('Ctrl Pts',(-10.5003546710001,15.2,-1.32682215400001));
#263361=CARTESIAN_POINT('Ctrl Pts',(-10.5003546710001,11.6,-1.32682215400001));
#263362=CARTESIAN_POINT('Ctrl Pts',(-10.4983217640001,15.2,-1.32700648100001));
#263363=CARTESIAN_POINT('Ctrl Pts',(-10.4983217640001,11.6,-1.32700648100002));
#263364=CARTESIAN_POINT('Ctrl Pts',(-10.4962956400001,15.2,-1.32718835600001));
#263365=CARTESIAN_POINT('Ctrl Pts',(-10.4962956400001,11.6,-1.32718835600001));
#263366=CARTESIAN_POINT('Ctrl Pts',(-10.4942763170001,15.2,-1.32736778800002));
#263367=CARTESIAN_POINT('Ctrl Pts',(-10.4942763170001,11.6,-1.32736778800002));
#263368=CARTESIAN_POINT('Ctrl Pts',(-10.4922638100001,15.2,-1.32754478700001));
#263369=CARTESIAN_POINT('Ctrl Pts',(-10.4922638100001,11.6,-1.32754478700001));
#263370=CARTESIAN_POINT('Ctrl Pts',(-10.4902581350001,15.2,-1.32771936200001));
#263371=CARTESIAN_POINT('Ctrl Pts',(-10.4902581350001,11.6,-1.32771936200002));
#263372=CARTESIAN_POINT('Ctrl Pts',(-10.4882593090001,15.2,-1.32789152500001));
#263373=CARTESIAN_POINT('Ctrl Pts',(-10.4882593090001,11.6,-1.32789152500001));
#263374=CARTESIAN_POINT('Ctrl Pts',(-10.4862673460001,15.2,-1.32806128600001));
#263375=CARTESIAN_POINT('Ctrl Pts',(-10.4862673460001,11.6,-1.32806128600001));
#263376=CARTESIAN_POINT('Ctrl Pts',(-10.4842822650001,15.2,-1.32822865400001));
#263377=CARTESIAN_POINT('Ctrl Pts',(-10.4842822650001,11.6,-1.32822865400001));
#263378=CARTESIAN_POINT('Ctrl Pts',(-10.4823040800001,15.2,-1.32839363900001));
#263379=CARTESIAN_POINT('Ctrl Pts',(-10.4823040800001,11.6,-1.32839363900001));
#263380=CARTESIAN_POINT('Ctrl Pts',(-10.4803328080001,15.2,-1.32855625200001));
#263381=CARTESIAN_POINT('Ctrl Pts',(-10.4803328080001,11.6,-1.32855625200001));
#263382=CARTESIAN_POINT('Ctrl Pts',(-10.4783684660001,15.2,-1.32871650300002));
#263383=CARTESIAN_POINT('Ctrl Pts',(-10.4783684660001,11.6,-1.32871650300002));
#263384=CARTESIAN_POINT('Ctrl Pts',(-10.4764110690001,15.2,-1.32887440400001));
#263385=CARTESIAN_POINT('Ctrl Pts',(-10.4764110690001,11.6,-1.32887440400001));
#263386=CARTESIAN_POINT('Ctrl Pts',(-10.4744606350001,15.2,-1.32902996200002));
#263387=CARTESIAN_POINT('Ctrl Pts',(-10.4744606350001,11.6,-1.32902996200002));
#263388=CARTESIAN_POINT('Ctrl Pts',(-10.4725171800001,15.2,-1.32918319000002));
#263389=CARTESIAN_POINT('Ctrl Pts',(-10.4725171800001,11.6,-1.32918319000002));
#263390=CARTESIAN_POINT('Ctrl Pts',(-10.4705807200001,15.2,-1.32933409700001));
#263391=CARTESIAN_POINT('Ctrl Pts',(-10.4705807200001,11.6,-1.32933409700001));
#263392=CARTESIAN_POINT('Ctrl Pts',(-10.4686512720001,15.2,-1.32948269500002));
#263393=CARTESIAN_POINT('Ctrl Pts',(-10.4686512720001,11.6,-1.32948269500002));
#263394=CARTESIAN_POINT('Ctrl Pts',(-10.4667288520001,15.2,-1.32962899400002));
#263395=CARTESIAN_POINT('Ctrl Pts',(-10.4667288520001,11.6,-1.32962899400002));
#263396=CARTESIAN_POINT('Ctrl Pts',(-10.4648134780001,15.2,-1.32977300400002));
#263397=CARTESIAN_POINT('Ctrl Pts',(-10.4648134780001,11.6,-1.32977300400002));
#263398=CARTESIAN_POINT('Ctrl Pts',(-10.4629051650001,15.2,-1.32991473500002));
#263399=CARTESIAN_POINT('Ctrl Pts',(-10.4629051650001,11.6,-1.32991473500002));
#263400=CARTESIAN_POINT('Ctrl Pts',(-10.4610039310001,15.2,-1.33005420000002));
#263401=CARTESIAN_POINT('Ctrl Pts',(-10.4610039310001,11.6,-1.33005420000002));
#263402=CARTESIAN_POINT('Ctrl Pts',(-10.4591097930001,15.2,-1.33019140900001));
#263403=CARTESIAN_POINT('Ctrl Pts',(-10.4591097930001,11.6,-1.33019140900001));
#263404=CARTESIAN_POINT('Ctrl Pts',(-10.4572227670001,15.2,-1.33032637100001));
#263405=CARTESIAN_POINT('Ctrl Pts',(-10.4572227670001,11.6,-1.33032637100001));
#263406=CARTESIAN_POINT('Ctrl Pts',(-10.4553428710001,15.2,-1.33045909900002));
#263407=CARTESIAN_POINT('Ctrl Pts',(-10.4553428710001,11.6,-1.33045909900002));
#263408=CARTESIAN_POINT('Ctrl Pts',(-10.4534701210001,15.2,-1.33058960200001));
#263409=CARTESIAN_POINT('Ctrl Pts',(-10.4534701210001,11.6,-1.33058960200001));
#263410=CARTESIAN_POINT('Ctrl Pts',(-10.4516045340001,15.2,-1.33071789400002));
#263411=CARTESIAN_POINT('Ctrl Pts',(-10.4516045340001,11.6,-1.33071789400002));
#263412=CARTESIAN_POINT('Ctrl Pts',(-10.4497461280001,15.2,-1.33084398300001));
#263413=CARTESIAN_POINT('Ctrl Pts',(-10.4497461280001,11.6,-1.33084398300001));
#263414=CARTESIAN_POINT('Ctrl Pts',(-10.4478949200001,15.2,-1.33096788000001));
#263415=CARTESIAN_POINT('Ctrl Pts',(-10.4478949200001,11.6,-1.33096788000001));
#263416=CARTESIAN_POINT('Ctrl Pts',(-10.4460509260001,15.2,-1.33108959700001));
#263417=CARTESIAN_POINT('Ctrl Pts',(-10.4460509260001,11.6,-1.33108959700001));
#263418=CARTESIAN_POINT('Ctrl Pts',(-10.4442141650001,15.2,-1.33120914700001));
#263419=CARTESIAN_POINT('Ctrl Pts',(-10.4442141650001,11.6,-1.33120914700001));
#263420=CARTESIAN_POINT('Ctrl Pts',(-10.4423846530001,15.2,-1.33132653900002));
#263421=CARTESIAN_POINT('Ctrl Pts',(-10.4423846530001,11.6,-1.33132653900002));
#263422=CARTESIAN_POINT('Ctrl Pts',(-10.4405624080001,15.2,-1.33144178400002));
#263423=CARTESIAN_POINT('Ctrl Pts',(-10.4405624080001,11.6,-1.33144178400002));
#263424=CARTESIAN_POINT('Ctrl Pts',(-10.4387474470001,15.2,-1.33155489400002));
#263425=CARTESIAN_POINT('Ctrl Pts',(-10.4387474470001,11.6,-1.33155489400002));
#263426=CARTESIAN_POINT('Ctrl Pts',(-10.4369397880001,15.2,-1.33166588100002));
#263427=CARTESIAN_POINT('Ctrl Pts',(-10.4369397880001,11.6,-1.33166588100002));
#263428=CARTESIAN_POINT('Ctrl Pts',(-10.4351394480001,15.2,-1.33177475500001));
#263429=CARTESIAN_POINT('Ctrl Pts',(-10.4351394480001,11.6,-1.33177475500002));
#263430=CARTESIAN_POINT('Ctrl Pts',(-10.4333464460001,15.2,-1.33188152900001));
#263431=CARTESIAN_POINT('Ctrl Pts',(-10.4333464460001,11.6,-1.33188152900001));
#263432=CARTESIAN_POINT('Ctrl Pts',(-10.4315607980001,15.2,-1.33198621200001));
#263433=CARTESIAN_POINT('Ctrl Pts',(-10.4315607980001,11.6,-1.33198621200001));
#263434=CARTESIAN_POINT('Ctrl Pts',(-10.4297825220001,15.2,-1.33208881900002));
#263435=CARTESIAN_POINT('Ctrl Pts',(-10.4297825220001,11.6,-1.33208881900002));
#263436=CARTESIAN_POINT('Ctrl Pts',(-10.4280116360001,15.2,-1.33218936000001));
#263437=CARTESIAN_POINT('Ctrl Pts',(-10.4280116360001,11.6,-1.33218936000001));
#263438=CARTESIAN_POINT('Ctrl Pts',(-10.4262481590001,15.2,-1.33228784500002));
#263439=CARTESIAN_POINT('Ctrl Pts',(-10.4262481590001,11.6,-1.33228784500002));
#263440=CARTESIAN_POINT('Ctrl Pts',(-10.4244921060001,15.2,-1.33238428800002));
#263441=CARTESIAN_POINT('Ctrl Pts',(-10.4244921060001,11.6,-1.33238428800002));
#263442=CARTESIAN_POINT('Ctrl Pts',(-10.4227434980001,15.2,-1.33247870000002));
#263443=CARTESIAN_POINT('Ctrl Pts',(-10.4227434980001,11.6,-1.33247870000002));
#263444=CARTESIAN_POINT('Ctrl Pts',(-10.4210023520001,15.2,-1.33257109300001));
#263445=CARTESIAN_POINT('Ctrl Pts',(-10.4210023520001,11.6,-1.33257109300001));
#263446=CARTESIAN_POINT('Ctrl Pts',(-10.4192686840001,15.2,-1.33266147700001));
#263447=CARTESIAN_POINT('Ctrl Pts',(-10.4192686840001,11.6,-1.33266147700001));
#263448=CARTESIAN_POINT('Ctrl Pts',(-10.4175425150001,15.2,-1.33274986700001));
#263449=CARTESIAN_POINT('Ctrl Pts',(-10.4175425150001,11.6,-1.33274986700001));
#263450=CARTESIAN_POINT('Ctrl Pts',(-10.4158238630001,15.2,-1.33283627400001));
#263451=CARTESIAN_POINT('Ctrl Pts',(-10.4158238630001,11.6,-1.33283627400001));
#263452=CARTESIAN_POINT('Ctrl Pts',(-10.4141127450001,15.2,-1.33292070900001));
#263453=CARTESIAN_POINT('Ctrl Pts',(-10.4141127450001,11.6,-1.33292070900001));
#263454=CARTESIAN_POINT('Ctrl Pts',(-10.4124091790001,15.2,-1.33300318500002));
#263455=CARTESIAN_POINT('Ctrl Pts',(-10.4124091790001,11.6,-1.33300318500002));
#263456=CARTESIAN_POINT('Ctrl Pts',(-10.4107131830001,15.2,-1.33308371300001));
#263457=CARTESIAN_POINT('Ctrl Pts',(-10.4107131830001,11.6,-1.33308371300001));
#263458=CARTESIAN_POINT('Ctrl Pts',(-10.4090247790001,15.2,-1.33316230600002));
#263459=CARTESIAN_POINT('Ctrl Pts',(-10.4090247790001,11.6,-1.33316230600002));
#263460=CARTESIAN_POINT('Ctrl Pts',(-10.4073439810001,15.2,-1.33323897700001));
#263461=CARTESIAN_POINT('Ctrl Pts',(-10.4073439810001,11.6,-1.33323897700001));
#263462=CARTESIAN_POINT('Ctrl Pts',(-10.4056708110001,15.2,-1.33331373800001));
#263463=CARTESIAN_POINT('Ctrl Pts',(-10.4056708110001,11.6,-1.33331373800001));
#263464=CARTESIAN_POINT('Ctrl Pts',(-10.4040052850001,15.2,-1.33338660100002));
#263465=CARTESIAN_POINT('Ctrl Pts',(-10.4040052850001,11.6,-1.33338660100002));
#263466=CARTESIAN_POINT('Ctrl Pts',(-10.4023474230001,15.2,-1.33345757700001));
#263467=CARTESIAN_POINT('Ctrl Pts',(-10.4023474230001,11.6,-1.33345757700001));
#263468=CARTESIAN_POINT('Ctrl Pts',(-10.4006972440001,15.2,-1.33352668100001));
#263469=CARTESIAN_POINT('Ctrl Pts',(-10.4006972440001,11.6,-1.33352668100002));
#263470=CARTESIAN_POINT('Ctrl Pts',(-10.3990547660001,15.2,-1.33359392500001));
#263471=CARTESIAN_POINT('Ctrl Pts',(-10.3990547660001,11.6,-1.33359392500001));
#263472=CARTESIAN_POINT('Ctrl Pts',(-10.3974200090001,15.2,-1.33365931900002));
#263473=CARTESIAN_POINT('Ctrl Pts',(-10.3974200090001,11.6,-1.33365931900002));
#263474=CARTESIAN_POINT('Ctrl Pts',(-10.3957929910001,15.2,-1.33372288000002));
#263475=CARTESIAN_POINT('Ctrl Pts',(-10.3957929910001,11.6,-1.33372288000002));
#263476=CARTESIAN_POINT('Ctrl Pts',(-10.3941737300001,15.2,-1.33378461700001));
#263477=CARTESIAN_POINT('Ctrl Pts',(-10.3941737300001,11.6,-1.33378461700001));
#263478=CARTESIAN_POINT('Ctrl Pts',(-10.3925622480001,15.2,-1.33384454600002));
#263479=CARTESIAN_POINT('Ctrl Pts',(-10.3925622480001,11.6,-1.33384454600002));
#263480=CARTESIAN_POINT('Ctrl Pts',(-10.3909585610001,15.2,-1.33390267600001));
#263481=CARTESIAN_POINT('Ctrl Pts',(-10.3909585610001,11.6,-1.33390267600001));
#263482=CARTESIAN_POINT('Ctrl Pts',(-10.3893626900001,15.2,-1.33395902400002));
#263483=CARTESIAN_POINT('Ctrl Pts',(-10.3893626900001,11.6,-1.33395902400002));
#263484=CARTESIAN_POINT('Ctrl Pts',(-10.3877746550001,15.2,-1.33401360000001));
#263485=CARTESIAN_POINT('Ctrl Pts',(-10.3877746550001,11.6,-1.33401360000002));
#263486=CARTESIAN_POINT('Ctrl Pts',(-10.3861944730001,15.2,-1.33406641800002));
#263487=CARTESIAN_POINT('Ctrl Pts',(-10.3861944730001,11.6,-1.33406641800002));
#263488=CARTESIAN_POINT('Ctrl Pts',(-10.3846221650001,15.2,-1.33411749200001));
#263489=CARTESIAN_POINT('Ctrl Pts',(-10.3846221650001,11.6,-1.33411749200001));
#263490=CARTESIAN_POINT('Ctrl Pts',(-10.3830577510001,15.2,-1.33416683400001));
#263491=CARTESIAN_POINT('Ctrl Pts',(-10.3830577510001,11.6,-1.33416683400002));
#263492=CARTESIAN_POINT('Ctrl Pts',(-10.3815012490001,15.2,-1.33421445700002));
#263493=CARTESIAN_POINT('Ctrl Pts',(-10.3815012490001,11.6,-1.33421445700002));
#263494=CARTESIAN_POINT('Ctrl Pts',(-10.3799526800001,15.2,-1.33426037500001));
#263495=CARTESIAN_POINT('Ctrl Pts',(-10.3799526800001,11.6,-1.33426037500001));
#263496=CARTESIAN_POINT('Ctrl Pts',(-10.3784120630001,15.2,-1.33430460200001));
#263497=CARTESIAN_POINT('Ctrl Pts',(-10.3784120630001,11.6,-1.33430460200001));
#263498=CARTESIAN_POINT('Ctrl Pts',(-10.3768794170001,15.2,-1.33434714900002));
#263499=CARTESIAN_POINT('Ctrl Pts',(-10.3768794170001,11.6,-1.33434714900002));
#263500=CARTESIAN_POINT('Ctrl Pts',(-10.3753547630001,15.2,-1.33438803300002));
#263501=CARTESIAN_POINT('Ctrl Pts',(-10.3753547630001,11.6,-1.33438803300002));
#263502=CARTESIAN_POINT('Ctrl Pts',(-10.3738381210001,15.2,-1.33442726500002));
#263503=CARTESIAN_POINT('Ctrl Pts',(-10.3738381210001,11.6,-1.33442726500002));
#263504=CARTESIAN_POINT('Ctrl Pts',(-10.3723295110001,15.2,-1.33446485900001));
#263505=CARTESIAN_POINT('Ctrl Pts',(-10.3723295110001,11.6,-1.33446485900001));
#263506=CARTESIAN_POINT('Ctrl Pts',(-10.3708289520001,15.2,-1.33450082900001));
#263507=CARTESIAN_POINT('Ctrl Pts',(-10.3708289520001,11.6,-1.33450082900001));
#263508=CARTESIAN_POINT('Ctrl Pts',(-10.3693364650001,15.2,-1.33453518900001));
#263509=CARTESIAN_POINT('Ctrl Pts',(-10.3693364650001,11.6,-1.33453518900001));
#263510=CARTESIAN_POINT('Ctrl Pts',(-10.3678520690001,15.2,-1.33456795200001));
#263511=CARTESIAN_POINT('Ctrl Pts',(-10.3678520690001,11.6,-1.33456795200001));
#263512=CARTESIAN_POINT('Ctrl Pts',(-10.3663757870001,15.2,-1.33459913200001));
#263513=CARTESIAN_POINT('Ctrl Pts',(-10.3663757870001,11.6,-1.33459913200001));
#263514=CARTESIAN_POINT('Ctrl Pts',(-10.3649076360001,15.2,-1.33462874400001));
#263515=CARTESIAN_POINT('Ctrl Pts',(-10.3649076360001,11.6,-1.33462874400002));
#263516=CARTESIAN_POINT('Ctrl Pts',(-10.3634476390001,15.2,-1.33465680100001));
#263517=CARTESIAN_POINT('Ctrl Pts',(-10.3634476390001,11.6,-1.33465680100001));
#263518=CARTESIAN_POINT('Ctrl Pts',(-10.3619958160001,15.2,-1.33468331700001));
#263519=CARTESIAN_POINT('Ctrl Pts',(-10.3619958160001,11.6,-1.33468331700001));
#263520=CARTESIAN_POINT('Ctrl Pts',(-10.3605521870001,15.2,-1.33470830800002));
#263521=CARTESIAN_POINT('Ctrl Pts',(-10.3605521870001,11.6,-1.33470830800002));
#263522=CARTESIAN_POINT('Ctrl Pts',(-10.3591167720001,15.2,-1.33473178600001));
#263523=CARTESIAN_POINT('Ctrl Pts',(-10.3591167720001,11.6,-1.33473178600001));
#263524=CARTESIAN_POINT('Ctrl Pts',(-10.3576895940001,15.2,-1.33475376600002));
#263525=CARTESIAN_POINT('Ctrl Pts',(-10.3576895940001,11.6,-1.33475376600002));
#263526=CARTESIAN_POINT('Ctrl Pts',(-10.3562706710001,15.2,-1.33477426200002));
#263527=CARTESIAN_POINT('Ctrl Pts',(-10.3562706710001,11.6,-1.33477426200002));
#263528=CARTESIAN_POINT('Ctrl Pts',(-10.3548600260001,15.2,-1.33479329000001));
#263529=CARTESIAN_POINT('Ctrl Pts',(-10.3548600260001,11.6,-1.33479329000001));
#263530=CARTESIAN_POINT('Ctrl Pts',(-10.3534576790001,15.2,-1.33481086200002));
#263531=CARTESIAN_POINT('Ctrl Pts',(-10.3534576790001,11.6,-1.33481086200002));
#263532=CARTESIAN_POINT('Ctrl Pts',(-10.3520636520001,15.2,-1.33482699500002));
#263533=CARTESIAN_POINT('Ctrl Pts',(-10.3520636520001,11.6,-1.33482699500002));
#263534=CARTESIAN_POINT('Ctrl Pts',(-10.3506779650001,15.2,-1.33484170200001));
#263535=CARTESIAN_POINT('Ctrl Pts',(-10.3506779650001,11.6,-1.33484170200001));
#263536=CARTESIAN_POINT('Ctrl Pts',(-10.3493006400001,15.2,-1.33485499900001));
#263537=CARTESIAN_POINT('Ctrl Pts',(-10.3493006400001,11.6,-1.33485499900001));
#263538=CARTESIAN_POINT('Ctrl Pts',(-10.3479316980001,15.2,-1.33486689900002));
#263539=CARTESIAN_POINT('Ctrl Pts',(-10.3479316980001,11.6,-1.33486689900002));
#263540=CARTESIAN_POINT('Ctrl Pts',(-10.3465711600001,15.2,-1.33487741900002));
#263541=CARTESIAN_POINT('Ctrl Pts',(-10.3465711600001,11.6,-1.33487741900002));
#263542=CARTESIAN_POINT('Ctrl Pts',(-10.3452190490001,15.2,-1.33488657300001));
#263543=CARTESIAN_POINT('Ctrl Pts',(-10.3452190490001,11.6,-1.33488657300001));
#263544=CARTESIAN_POINT('Ctrl Pts',(-10.3438753840001,15.2,-1.33489437600002));
#263545=CARTESIAN_POINT('Ctrl Pts',(-10.3438753840001,11.6,-1.33489437600002));
#263546=CARTESIAN_POINT('Ctrl Pts',(-10.3425401900001,15.2,-1.33490084300002));
#263547=CARTESIAN_POINT('Ctrl Pts',(-10.3425401900001,11.6,-1.33490084300002));
#263548=CARTESIAN_POINT('Ctrl Pts',(-10.3412134860001,15.2,-1.33490598900002));
#263549=CARTESIAN_POINT('Ctrl Pts',(-10.3412134860001,11.6,-1.33490598900002));
#263550=CARTESIAN_POINT('Ctrl Pts',(-10.3398952940001,15.2,-1.33490982900001));
#263551=CARTESIAN_POINT('Ctrl Pts',(-10.3398952940001,11.6,-1.33490982900002));
#263552=CARTESIAN_POINT('Ctrl Pts',(-10.3385856380001,15.2,-1.33491238000001));
#263553=CARTESIAN_POINT('Ctrl Pts',(-10.3385856380001,11.6,-1.33491238000001));
#263554=CARTESIAN_POINT('Ctrl Pts',(-10.3372845370001,15.2,-1.33491365700001));
#263555=CARTESIAN_POINT('Ctrl Pts',(-10.3372845370001,11.6,-1.33491365700001));
#263556=CARTESIAN_POINT('Ctrl Pts',(-10.3359920170001,15.2,-1.33491367300001));
#263557=CARTESIAN_POINT('Ctrl Pts',(-10.3359920170001,11.6,-1.33491367300001));
#263558=CARTESIAN_POINT('Ctrl Pts',(-10.3347080960001,15.2,-1.33491244600001));
#263559=CARTESIAN_POINT('Ctrl Pts',(-10.3347080960001,11.6,-1.33491244600001));
#263560=CARTESIAN_POINT('Ctrl Pts',(-10.3334327990001,15.2,-1.33490999100002));
#263561=CARTESIAN_POINT('Ctrl Pts',(-10.3334327990001,11.6,-1.33490999100002));
#263562=CARTESIAN_POINT('Ctrl Pts',(-10.3321661480001,15.2,-1.33490632400001));
#263563=CARTESIAN_POINT('Ctrl Pts',(-10.3321661480001,11.6,-1.33490632400001));
#263564=CARTESIAN_POINT('Ctrl Pts',(-10.3309081640001,15.2,-1.33490146000002));
#263565=CARTESIAN_POINT('Ctrl Pts',(-10.3309081640001,11.6,-1.33490146000002));
#263566=CARTESIAN_POINT('Ctrl Pts',(-10.3296588710001,15.2,-1.33489541500001));
#263567=CARTESIAN_POINT('Ctrl Pts',(-10.3296588710001,11.6,-1.33489541500001));
#263568=CARTESIAN_POINT('Ctrl Pts',(-10.3284182910001,15.2,-1.33488820600002));
#263569=CARTESIAN_POINT('Ctrl Pts',(-10.3284182910001,11.6,-1.33488820600002));
#263570=CARTESIAN_POINT('Ctrl Pts',(-10.3271864460001,15.2,-1.33487984800002));
#263571=CARTESIAN_POINT('Ctrl Pts',(-10.3271864460001,11.6,-1.33487984800002));
#263572=CARTESIAN_POINT('Ctrl Pts',(-10.3259633610001,15.2,-1.33487035800002));
#263573=CARTESIAN_POINT('Ctrl Pts',(-10.3259633610001,11.6,-1.33487035800002));
#263574=CARTESIAN_POINT('Ctrl Pts',(-10.3247490570001,15.2,-1.33485975200001));
#263575=CARTESIAN_POINT('Ctrl Pts',(-10.3247490570001,11.6,-1.33485975200002));
#263576=CARTESIAN_POINT('Ctrl Pts',(-10.3235435580001,15.2,-1.33484804600001));
#263577=CARTESIAN_POINT('Ctrl Pts',(-10.3235435580001,11.6,-1.33484804600001));
#263578=CARTESIAN_POINT('Ctrl Pts',(-10.3223468860001,15.2,-1.33483525700001));
#263579=CARTESIAN_POINT('Ctrl Pts',(-10.3223468860001,11.6,-1.33483525700001));
#263580=CARTESIAN_POINT('Ctrl Pts',(-10.3211590660001,15.2,-1.33482140000002));
#263581=CARTESIAN_POINT('Ctrl Pts',(-10.3211590660001,11.6,-1.33482140000002));
#263582=CARTESIAN_POINT('Ctrl Pts',(-10.3199801190001,15.2,-1.33480649300001));
#263583=CARTESIAN_POINT('Ctrl Pts',(-10.3199801190001,11.6,-1.33480649300001));
#263584=CARTESIAN_POINT('Ctrl Pts',(-10.3188100710001,15.2,-1.33479055200001));
#263585=CARTESIAN_POINT('Ctrl Pts',(-10.3188100710001,11.6,-1.33479055200001));
#263586=CARTESIAN_POINT('Ctrl Pts',(-10.3176489430001,15.2,-1.33477359400001));
#263587=CARTESIAN_POINT('Ctrl Pts',(-10.3176489430001,11.6,-1.33477359400001));
#263588=CARTESIAN_POINT('Ctrl Pts',(-10.3164967600001,15.2,-1.33475563600001));
#263589=CARTESIAN_POINT('Ctrl Pts',(-10.3164967600001,11.6,-1.33475563600001));
#263590=CARTESIAN_POINT('Ctrl Pts',(-10.3153535460001,15.2,-1.33473669500002));
#263591=CARTESIAN_POINT('Ctrl Pts',(-10.3153535460001,11.6,-1.33473669500002));
#263592=CARTESIAN_POINT('Ctrl Pts',(-10.3142193240001,15.2,-1.33471678800001));
#263593=CARTESIAN_POINT('Ctrl Pts',(-10.3142193240001,11.6,-1.33471678800001));
#263594=CARTESIAN_POINT('Ctrl Pts',(-10.3130941180001,15.2,-1.33469593100001));
#263595=CARTESIAN_POINT('Ctrl Pts',(-10.3130941180001,11.6,-1.33469593100001));
#263596=CARTESIAN_POINT('Ctrl Pts',(-10.3119779530001,15.2,-1.33467414100001));
#263597=CARTESIAN_POINT('Ctrl Pts',(-10.3119779530001,11.6,-1.33467414100001));
#263598=CARTESIAN_POINT('Ctrl Pts',(-10.3108708510001,15.2,-1.33465143800001));
#263599=CARTESIAN_POINT('Ctrl Pts',(-10.3108708510001,11.6,-1.33465143800001));
#263600=CARTESIAN_POINT('Ctrl Pts',(-10.3097728380001,15.2,-1.33462783700002));
#263601=CARTESIAN_POINT('Ctrl Pts',(-10.3097728380001,11.6,-1.33462783700002));
#263602=CARTESIAN_POINT('Ctrl Pts',(-10.3086839380001,15.2,-1.33460335600001));
#263603=CARTESIAN_POINT('Ctrl Pts',(-10.3086839380001,11.6,-1.33460335600002));
#263604=CARTESIAN_POINT('Ctrl Pts',(-10.3076041750001,15.2,-1.33457801300001));
#263605=CARTESIAN_POINT('Ctrl Pts',(-10.3076041750001,11.6,-1.33457801300001));
#263606=CARTESIAN_POINT('Ctrl Pts',(-10.3065335750001,15.2,-1.33455182600001));
#263607=CARTESIAN_POINT('Ctrl Pts',(-10.3065335750001,11.6,-1.33455182600001));
#263608=CARTESIAN_POINT('Ctrl Pts',(-10.3054721600001,15.2,-1.33452481200001));
#263609=CARTESIAN_POINT('Ctrl Pts',(-10.3054721600001,11.6,-1.33452481200001));
#263610=CARTESIAN_POINT('Ctrl Pts',(-10.3044199570001,15.2,-1.33449698800002));
#263611=CARTESIAN_POINT('Ctrl Pts',(-10.3044199570001,11.6,-1.33449698800002));
#263612=CARTESIAN_POINT('Ctrl Pts',(-10.3033769900001,15.2,-1.33446837400002));
#263613=CARTESIAN_POINT('Ctrl Pts',(-10.3033769900001,11.6,-1.33446837400002));
#263614=CARTESIAN_POINT('Ctrl Pts',(-10.3023432850001,15.2,-1.33443898600001));
#263615=CARTESIAN_POINT('Ctrl Pts',(-10.3023432850001,11.6,-1.33443898600001));
#263616=CARTESIAN_POINT('Ctrl Pts',(-10.3013188650001,15.2,-1.33440884400001));
#263617=CARTESIAN_POINT('Ctrl Pts',(-10.3013188650001,11.6,-1.33440884400002));
#263618=CARTESIAN_POINT('Ctrl Pts',(-10.3003037570001,15.2,-1.33437796600001));
#263619=CARTESIAN_POINT('Ctrl Pts',(-10.3003037570001,11.6,-1.33437796600001));
#263620=CARTESIAN_POINT('Ctrl Pts',(-10.2992979850001,15.2,-1.33434636800001));
#263621=CARTESIAN_POINT('Ctrl Pts',(-10.2992979850001,11.6,-1.33434636800001));
#263622=CARTESIAN_POINT('Ctrl Pts',(-10.2983015770001,15.2,-1.33431407100002));
#263623=CARTESIAN_POINT('Ctrl Pts',(-10.2983015770001,11.6,-1.33431407100002));
#263624=CARTESIAN_POINT('Ctrl Pts',(-10.2973145550001,15.2,-1.33428109300001));
#263625=CARTESIAN_POINT('Ctrl Pts',(-10.2973145550001,11.6,-1.33428109300001));
#263626=CARTESIAN_POINT('Ctrl Pts',(-10.2963369470001,15.2,-1.33424745200001));
#263627=CARTESIAN_POINT('Ctrl Pts',(-10.2963369470001,11.6,-1.33424745200002));
#263628=CARTESIAN_POINT('Ctrl Pts',(-10.2953687780001,15.2,-1.33421316700002));
#263629=CARTESIAN_POINT('Ctrl Pts',(-10.2953687780001,11.6,-1.33421316700002));
#263630=CARTESIAN_POINT('Ctrl Pts',(-10.2944100750001,15.2,-1.33417825800001));
#263631=CARTESIAN_POINT('Ctrl Pts',(-10.2944100750001,11.6,-1.33417825800001));
#263632=CARTESIAN_POINT('Ctrl Pts',(-10.2934608630001,15.2,-1.33414274200002));
#263633=CARTESIAN_POINT('Ctrl Pts',(-10.2934608630001,11.6,-1.33414274200002));
#263634=CARTESIAN_POINT('Ctrl Pts',(-10.2925211680001,15.2,-1.33410664000001));
#263635=CARTESIAN_POINT('Ctrl Pts',(-10.2925211680001,11.6,-1.33410664000001));
#263636=CARTESIAN_POINT('Ctrl Pts',(-10.2915910170001,15.2,-1.33406997000002));
#263637=CARTESIAN_POINT('Ctrl Pts',(-10.2915910170001,11.6,-1.33406997000002));
#263638=CARTESIAN_POINT('Ctrl Pts',(-10.2906757380001,15.2,-1.33403296500001));
#263639=CARTESIAN_POINT('Ctrl Pts',(-10.2906757380001,11.6,-1.33403296500001));
#263640=CARTESIAN_POINT('Ctrl Pts',(-10.2899521420001,15.2,-1.33400298800002));
#263641=CARTESIAN_POINT('Ctrl Pts',(-10.2899521420001,11.6,-1.33400298800002));
#263642=CARTESIAN_POINT('Ctrl Pts',(-10.2894150050001,15.2,-1.33398033400002));
#263643=CARTESIAN_POINT('Ctrl Pts',(-10.2894150050001,11.6,-1.33398033400002));
#263644=CARTESIAN_POINT('Ctrl Pts',(-10.2890605210001,15.2,-1.33396520700002));
#263645=CARTESIAN_POINT('Ctrl Pts',(-10.2890605210001,11.6,-1.33396520700002));
#263646=CARTESIAN_POINT('Ctrl Pts',(-10.2888863240001,15.2,-1.33395773200002));
#263647=CARTESIAN_POINT('Ctrl Pts',(-10.2888863240001,11.6,-1.33395773200002));
#263648=CARTESIAN_POINT('',(-10.2888863233592,12.2,-1.33395773200336));
#263649=CARTESIAN_POINT('',(-10.2888863233592,15.2,-1.33395773200336));
#263650=CARTESIAN_POINT('',(-10.2888863230001,12.2,-1.33395773200002));
#263651=CARTESIAN_POINT('Ctrl Pts',(-11.4479048650001,12.2,-1.09337742900002));
#263652=CARTESIAN_POINT('Ctrl Pts',(-11.4443249343497,12.2,-1.09471863924366));
#263653=CARTESIAN_POINT('Ctrl Pts',(-11.4407496848669,12.2,-1.0960534771315));
#263654=CARTESIAN_POINT('Ctrl Pts',(-11.437179116671,12.2,-1.09738195555992));
#263655=CARTESIAN_POINT('Ctrl Pts',(-11.4336085484751,12.2,-1.09871043398834));
#263656=CARTESIAN_POINT('Ctrl Pts',(-11.4300426619881,12.2,-1.10003254737677));
#263657=CARTESIAN_POINT('Ctrl Pts',(-11.4264814749807,12.2,-1.10134830302043));
#263658=CARTESIAN_POINT('Ctrl Pts',(-11.4217332252062,12.2,-1.103102644038));
#263659=CARTESIAN_POINT('Ctrl Pts',(-11.4169933281401,12.2,-1.10484567960066));
#263660=CARTESIAN_POINT('Ctrl Pts',(-11.412261887605,12.2,-1.10657744341652));
#263661=CARTESIAN_POINT('Ctrl Pts',(-11.408713307526,12.2,-1.10787626616044));
#263662=CARTESIAN_POINT('Ctrl Pts',(-11.4051694849548,12.2,-1.10916875001346));
#263663=CARTESIAN_POINT('Ctrl Pts',(-11.40163046525,12.2,-1.1104549087584));
#263664=CARTESIAN_POINT('Ctrl Pts',(-11.3980914455453,12.2,-1.11174106750334));
#263665=CARTESIAN_POINT('Ctrl Pts',(-11.394557227657,12.2,-1.1130209015902));
#263666=CARTESIAN_POINT('Ctrl Pts',(-11.3910278474098,12.2,-1.11429442183614));
#263667=CARTESIAN_POINT('Ctrl Pts',(-11.3874984671626,12.2,-1.11556794208209));
#263668=CARTESIAN_POINT('Ctrl Pts',(-11.3839739234629,12.2,-1.11683514947146));
#263669=CARTESIAN_POINT('Ctrl Pts',(-11.3804542531644,12.2,-1.11809605573938));
#263670=CARTESIAN_POINT('Ctrl Pts',(-11.3769345828659,12.2,-1.11935696200729));
#263671=CARTESIAN_POINT('Ctrl Pts',(-11.373419786855,12.2,-1.12061156748908));
#263672=CARTESIAN_POINT('Ctrl Pts',(-11.3699099047735,12.2,-1.12185988473625));
#263673=CARTESIAN_POINT('Ctrl Pts',(-11.3664000220544,12.2,-1.1231082022102));
#263674=CARTESIAN_POINT('Ctrl Pts',(-11.3628950544283,12.2,-1.12435023280738));
#263675=CARTESIAN_POINT('Ctrl Pts',(-11.3593950397537,12.2,-1.12558598931945));
#263676=CARTESIAN_POINT('Ctrl Pts',(-11.3558950257149,12.2,-1.12682174560702));
#263677=CARTESIAN_POINT('Ctrl Pts',(-11.3523999670258,12.2,-1.12805122906161));
#263678=CARTESIAN_POINT('Ctrl Pts',(-11.348909900403,12.2,-1.12927445084995));
#263679=CARTESIAN_POINT('Ctrl Pts',(-11.3454198337803,12.2,-1.13049767263829));
#263680=CARTESIAN_POINT('Ctrl Pts',(-11.3419347591362,12.2,-1.13171463440634));
#263681=CARTESIAN_POINT('Ctrl Pts',(-11.3384547169552,12.2,-1.13292534953449));
#263682=CARTESIAN_POINT('Ctrl Pts',(-11.3349746747742,12.2,-1.13413606466264));
#263683=CARTESIAN_POINT('Ctrl Pts',(-11.3314996639429,12.2,-1.13534053188703));
#263684=CARTESIAN_POINT('Ctrl Pts',(-11.3280297252615,12.2,-1.13653876701564));
#263685=CARTESIAN_POINT('Ctrl Pts',(-11.3245597865801,12.2,-1.13773700214424));
#263686=CARTESIAN_POINT('Ctrl Pts',(-11.321094919502,12.2,-1.13892900289658));
#263687=CARTESIAN_POINT('Ctrl Pts',(-11.3176351643772,12.2,-1.14011478560404));
#263688=CARTESIAN_POINT('Ctrl Pts',(-11.3141754092525,12.2,-1.1413005683115));
#263689=CARTESIAN_POINT('Ctrl Pts',(-11.3107207663774,12.2,-1.14248013275271));
#263690=CARTESIAN_POINT('Ctrl Pts',(-11.307271274252,12.2,-1.14365349150259));
#263691=CARTESIAN_POINT('Ctrl Pts',(-11.3038217815,12.2,-1.14482685046563));
#263692=CARTESIAN_POINT('Ctrl Pts',(-11.3003774400327,12.2,-1.14599400426859));
#263693=CARTESIAN_POINT('Ctrl Pts',(-11.2969382902836,12.2,-1.14715496772814));
#263694=CARTESIAN_POINT('Ctrl Pts',(-11.2923527583261,12.2,-1.14870291865603));
#263695=CARTESIAN_POINT('Ctrl Pts',(-11.2877764550117,12.2,-1.15023986500291));
#263696=CARTESIAN_POINT('Ctrl Pts',(-11.2832094782531,12.2,-1.15176583927402));
#263697=CARTESIAN_POINT('Ctrl Pts',(-11.2797842455287,12.2,-1.15291032002932));
#263698=CARTESIAN_POINT('Ctrl Pts',(-11.2763642569487,12.2,-1.15404862993381));
#263699=CARTESIAN_POINT('Ctrl Pts',(-11.2729495548223,12.2,-1.15518078364322));
#263700=CARTESIAN_POINT('Ctrl Pts',(-11.2683966182402,12.2,-1.15669032205955));
#263701=CARTESIAN_POINT('Ctrl Pts',(-11.2638530796593,12.2,-1.15818891457732));
#263702=CARTESIAN_POINT('Ctrl Pts',(-11.2593190344128,12.2,-1.15967659837991));
#263703=CARTESIAN_POINT('Ctrl Pts',(-11.2559185007868,12.2,-1.1607923611305));
#263704=CARTESIAN_POINT('Ctrl Pts',(-11.2525233065935,12.2,-1.16190198792349));
#263705=CARTESIAN_POINT('Ctrl Pts',(-11.249133494425,12.2,-1.16300549275839));
#263706=CARTESIAN_POINT('Ctrl Pts',(-11.2457436822565,12.2,-1.1641089975933));
#263707=CARTESIAN_POINT('Ctrl Pts',(-11.2423592509961,12.2,-1.16520638198679));
#263708=CARTESIAN_POINT('Ctrl Pts',(-11.2389802419101,12.2,-1.16629765936434));
#263709=CARTESIAN_POINT('Ctrl Pts',(-11.235601232824,12.2,-1.16738893674189));
#263710=CARTESIAN_POINT('Ctrl Pts',(-11.2322276473649,12.2,-1.16847410962581));
#263711=CARTESIAN_POINT('Ctrl Pts',(-11.2288595241517,12.2,-1.16955319055789));
#263712=CARTESIAN_POINT('Ctrl Pts',(-11.2254914009385,12.2,-1.17063227148996));
#263713=CARTESIAN_POINT('Ctrl Pts',(-11.2221287413606,12.2,-1.1717052624554));
#263714=CARTESIAN_POINT('Ctrl Pts',(-11.2187715872319,12.2,-1.17277217870913));
#263715=CARTESIAN_POINT('Ctrl Pts',(-11.2154144324932,12.2,-1.17383909515668));
#263716=CARTESIAN_POINT('Ctrl Pts',(-11.2120627828228,12.2,-1.17489993637752));
#263717=CARTESIAN_POINT('Ctrl Pts',(-11.2087166805456,12.2,-1.17595471969666));
#263718=CARTESIAN_POINT('Ctrl Pts',(-11.2053705788762,12.2,-1.17700950282418));
#263719=CARTESIAN_POINT('Ctrl Pts',(-11.2020300232649,12.2,-1.17805822645202));
#263720=CARTESIAN_POINT('Ctrl Pts',(-11.1986950571366,12.2,-1.17910090766361));
#263721=CARTESIAN_POINT('Ctrl Pts',(-11.1942484358341,12.2,-1.18049114921591));
#263722=CARTESIAN_POINT('Ctrl Pts',(-11.1898117494387,12.2,-1.18187064734396));
#263723=CARTESIAN_POINT('Ctrl Pts',(-11.1853850986341,12.2,-1.18323944230138));
#263724=CARTESIAN_POINT('Ctrl Pts',(-11.1820651103798,12.2,-1.18426603856607));
#263725=CARTESIAN_POINT('Ctrl Pts',(-11.1787507677519,12.2,-1.18528661304825));
#263726=CARTESIAN_POINT('Ctrl Pts',(-11.1754421117046,12.2,-1.18630118426221));
#263727=CARTESIAN_POINT('Ctrl Pts',(-11.1721334550563,12.2,-1.18731575566048));
#263728=CARTESIAN_POINT('Ctrl Pts',(-11.1688304862763,12.2,-1.18832432270706));
#263729=CARTESIAN_POINT('Ctrl Pts',(-11.1655332470479,12.2,-1.18932690122695));
#263730=CARTESIAN_POINT('Ctrl Pts',(-11.1622360084185,12.2,-1.1903294795647));
#263731=CARTESIAN_POINT('Ctrl Pts',(-11.1589444987887,12.2,-1.19132607134445));
#263732=CARTESIAN_POINT('Ctrl Pts',(-11.1556587626586,12.2,-1.19231669164127));
#263733=CARTESIAN_POINT('Ctrl Pts',(-11.1523730265285,12.2,-1.19330731193808));
#263734=CARTESIAN_POINT('Ctrl Pts',(-11.1490930630929,12.2,-1.19429196094875));
#263735=CARTESIAN_POINT('Ctrl Pts',(-11.1458189150304,12.2,-1.19527065675094));
#263736=CARTESIAN_POINT('Ctrl Pts',(-11.1425447669678,12.2,-1.19624935255314));
#263737=CARTESIAN_POINT('Ctrl Pts',(-11.1392764345159,12.2,-1.19722209469656));
#263738=CARTESIAN_POINT('Ctrl Pts',(-11.1360139604947,12.2,-1.19818890095751));
#263739=CARTESIAN_POINT('Ctrl Pts',(-11.1327514864734,12.2,-1.19915570721846));
#263740=CARTESIAN_POINT('Ctrl Pts',(-11.1294948719202,12.2,-1.20011657683005));
#263741=CARTESIAN_POINT('Ctrl Pts',(-11.1262441588711,12.2,-1.2010715276292));
#263742=CARTESIAN_POINT('Ctrl Pts',(-11.122993445822,12.2,-1.20202647842836));
#263743=CARTESIAN_POINT('Ctrl Pts',(-11.1197486347892,12.2,-1.20297551131124));
#263744=CARTESIAN_POINT('Ctrl Pts',(-11.1165097696978,12.2,-1.20391864306945));
#263745=CARTESIAN_POINT('Ctrl Pts',(-11.1132709040179,12.2,-1.20486177499899));
#263746=CARTESIAN_POINT('Ctrl Pts',(-11.1100379834481,12.2,-1.20579900555186));
#263747=CARTESIAN_POINT('Ctrl Pts',(-11.1068110527716,12.2,-1.20673035347808));
#263748=CARTESIAN_POINT('Ctrl Pts',(-11.1025084795132,12.2,-1.20797215043106));
#263749=CARTESIAN_POINT('Ctrl Pts',(-11.0982165538419,12.2,-1.20920348836568));
#263750=CARTESIAN_POINT('Ctrl Pts',(-11.0939353812279,12.2,-1.21042441071589));
#263751=CARTESIAN_POINT('Ctrl Pts',(-11.088583915023,12.2,-1.21195056377841));
#263752=CARTESIAN_POINT('Ctrl Pts',(-11.0832492483889,12.2,-1.21346044241117));
#263753=CARTESIAN_POINT('Ctrl Pts',(-11.0779315880417,12.2,-1.21495413296672));
#263754=CARTESIAN_POINT('Ctrl Pts',(-11.0736774595321,12.2,-1.21614908547629));
#263755=CARTESIAN_POINT('Ctrl Pts',(-11.0694342144598,12.2,-1.21733367755132));
#263756=CARTESIAN_POINT('Ctrl Pts',(-11.0652019593414,12.2,-1.21850795339204));
#263757=CARTESIAN_POINT('Ctrl Pts',(-11.0599116413083,12.2,-1.21997579795295));
#263758=CARTESIAN_POINT('Ctrl Pts',(-11.0546384945827,12.2,-1.22142752522855));
#263759=CARTESIAN_POINT('Ctrl Pts',(-11.0493827274458,12.2,-1.22286322083726));
#263760=CARTESIAN_POINT('Ctrl Pts',(-11.0441269597361,12.2,-1.22429891660247));
#263761=CARTESIAN_POINT('Ctrl Pts',(-11.0388885726677,12.2,-1.2257185834207));
#263762=CARTESIAN_POINT('Ctrl Pts',(-11.0336677749579,12.2,-1.22712231078311));
#263763=CARTESIAN_POINT('Ctrl Pts',(-11.0294911365625,12.2,-1.22824529273425));
#263764=CARTESIAN_POINT('Ctrl Pts',(-11.0253257576841,12.2,-1.22935807418019));
#263765=CARTESIAN_POINT('Ctrl Pts',(-11.0211717432722,12.2,-1.2304607008008));
#263766=CARTESIAN_POINT('Ctrl Pts',(-11.0170177294263,12.2,-1.23156332727119));
#263767=CARTESIAN_POINT('Ctrl Pts',(-11.0128750814806,12.2,-1.2326558012522));
#263768=CARTESIAN_POINT('Ctrl Pts',(-11.0087439096505,12.2,-1.23373816833142));
#263769=CARTESIAN_POINT('Ctrl Pts',(-11.0046127372575,12.2,-1.23482053555811));
#263770=CARTESIAN_POINT('Ctrl Pts',(-11.0004930399656,12.2,-1.23589279728661));
#263771=CARTESIAN_POINT('Ctrl Pts',(-10.9963849282417,12.2,-1.23695500123339));
#263772=CARTESIAN_POINT('Ctrl Pts',(-10.9922768165178,12.2,-1.23801720518017));
#263773=CARTESIAN_POINT('Ctrl Pts',(-10.9881802906091,12.2,-1.239069351923));
#263774=CARTESIAN_POINT('Ctrl Pts',(-10.9840954608322,12.2,-1.24011149114544));
#263775=CARTESIAN_POINT('Ctrl Pts',(-10.9800106316117,12.2,-1.24115363022589));
#263776=CARTESIAN_POINT('Ctrl Pts',(-10.9759374985198,12.2,-1.24218576152546));
#263777=CARTESIAN_POINT('Ctrl Pts',(-10.9718761727778,12.2,-1.24320793472435));
#263778=CARTESIAN_POINT('Ctrl Pts',(-10.9667995151852,12.2,-1.24448565132742));
#263779=CARTESIAN_POINT('Ctrl Pts',(-10.9617413080111,12.2,-1.24574781044451));
#263780=CARTESIAN_POINT('Ctrl Pts',(-10.9567017702333,12.2,-1.24699450870839));
#263781=CARTESIAN_POINT('Ctrl Pts',(-10.9526701397914,12.2,-1.24799186737385));
#263782=CARTESIAN_POINT('Ctrl Pts',(-10.9486504570425,12.2,-1.24897933325762));
#263783=CARTESIAN_POINT('Ctrl Pts',(-10.9446428361031,12.2,-1.24995695664322));
#263784=CARTESIAN_POINT('Ctrl Pts',(-10.9396333107479,12.2,-1.25117898567543));
#263785=CARTESIAN_POINT('Ctrl Pts',(-10.9346426326377,12.2,-1.25238563818949));
#263786=CARTESIAN_POINT('Ctrl Pts',(-10.9296710231086,12.2,-1.25357701535255));
#263787=CARTESIAN_POINT('Ctrl Pts',(-10.925693734835,12.2,-1.25453011723883));
#263788=CARTESIAN_POINT('Ctrl Pts',(-10.9217286520404,12.2,-1.25547344291028));
#263789=CARTESIAN_POINT('Ctrl Pts',(-10.9177758889917,12.2,-1.25640704751672));
#263790=CARTESIAN_POINT('Ctrl Pts',(-10.9138231259429,12.2,-1.25734065212316));
#263791=CARTESIAN_POINT('Ctrl Pts',(-10.9098826819928,12.2,-1.25826453445901));
#263792=CARTESIAN_POINT('Ctrl Pts',(-10.9059546748911,12.2,-1.25917874967452));
#263793=CARTESIAN_POINT('Ctrl Pts',(-10.9020266683246,12.2,-1.26009296476547));
#263794=CARTESIAN_POINT('Ctrl Pts',(-10.898111096651,12.2,-1.26099751315211));
#263795=CARTESIAN_POINT('Ctrl Pts',(-10.8942080783025,12.2,-1.26189244913513));
#263796=CARTESIAN_POINT('Ctrl Pts',(-10.8903050594223,12.2,-1.26278738524009));
#263797=CARTESIAN_POINT('Ctrl Pts',(-10.8864145947664,12.2,-1.26367271006421));
#263798=CARTESIAN_POINT('Ctrl Pts',(-10.8825368001957,12.2,-1.26454847937708));
#263799=CARTESIAN_POINT('Ctrl Pts',(-10.8786590061534,12.2,-1.26542424857063));
#263800=CARTESIAN_POINT('Ctrl Pts',(-10.8747938822815,12.2,-1.2662904627799));
#263801=CARTESIAN_POINT('Ctrl Pts',(-10.8709415485401,12.2,-1.26714717865493));
#263802=CARTESIAN_POINT('Ctrl Pts',(-10.8670892142737,12.2,-1.26800389464668));
#263803=CARTESIAN_POINT('Ctrl Pts',(-10.8632496704783,12.2,-1.2688511120873));
#263804=CARTESIAN_POINT('Ctrl Pts',(-10.8594230349373,12.2,-1.26968889007678));
#263805=CARTESIAN_POINT('Ctrl Pts',(-10.8555963999176,12.2,-1.27052666795213));
#263806=CARTESIAN_POINT('Ctrl Pts',(-10.8517826746097,12.2,-1.27135500690361));
#263807=CARTESIAN_POINT('Ctrl Pts',(-10.8479819792849,12.2,-1.27217396415616));
#263808=CARTESIAN_POINT('Ctrl Pts',(-10.8441812834423,12.2,-1.2729929215203));
#263809=CARTESIAN_POINT('Ctrl Pts',(-10.8403936177742,12.2,-1.27380249638349));
#263810=CARTESIAN_POINT('Ctrl Pts',(-10.8366191034582,12.2,-1.27460275231538));
#263811=CARTESIAN_POINT('Ctrl Pts',(-10.8319009608204,12.2,-1.27560307217574));
#263812=CARTESIAN_POINT('Ctrl Pts',(-10.8272033671876,12.2,-1.27658882671425));
#263813=CARTESIAN_POINT('Ctrl Pts',(-10.8225265629526,12.2,-1.27756013754682));
#263814=CARTESIAN_POINT('Ctrl Pts',(-10.8187851198705,12.2,-1.27833718614936));
#263815=CARTESIAN_POINT('Ctrl Pts',(-10.8150569816388,12.2,-1.27910498915213));
#263816=CARTESIAN_POINT('Ctrl Pts',(-10.8113422717558,12.2,-1.27986361090659));
#263817=CARTESIAN_POINT('Ctrl Pts',(-10.8066988840224,12.2,-1.28081188817718));
#263818=CARTESIAN_POINT('Ctrl Pts',(-10.8020764792133,12.2,-1.28174581575018));
#263819=CARTESIAN_POINT('Ctrl Pts',(-10.7974753008094,12.2,-1.28266552068148));
#263820=CARTESIAN_POINT('Ctrl Pts',(-10.7937943578857,12.2,-1.28340128466662));
#263821=CARTESIAN_POINT('Ctrl Pts',(-10.7901269989969,12.2,-1.284127944484));
#263822=CARTESIAN_POINT('Ctrl Pts',(-10.7864733514098,12.2,-1.2848455658003));
#263823=CARTESIAN_POINT('Ctrl Pts',(-10.7828197043205,12.2,-1.28556318701882));
#263824=CARTESIAN_POINT('Ctrl Pts',(-10.7791797682761,12.2,-1.28627176866994));
#263825=CARTESIAN_POINT('Ctrl Pts',(-10.7755536710012,12.2,-1.28697137664848));
#263826=CARTESIAN_POINT('Ctrl Pts',(-10.7719275732324,12.2,-1.28767098472235));
#263827=CARTESIAN_POINT('Ctrl Pts',(-10.7683153117817,12.2,-1.28836161856912));
#263828=CARTESIAN_POINT('Ctrl Pts',(-10.7647170181976,12.2,-1.28904334527236));
#263829=CARTESIAN_POINT('Ctrl Pts',(-10.7611187251038,12.2,-1.28972507188272));
#263830=CARTESIAN_POINT('Ctrl Pts',(-10.7575343979572,12.2,-1.29039789158097));
#263831=CARTESIAN_POINT('Ctrl Pts',(-10.7539641668588,12.2,-1.29106187091648));
#263832=CARTESIAN_POINT('Ctrl Pts',(-10.7503939352738,12.2,-1.29172585034246));
#263833=CARTESIAN_POINT('Ctrl Pts',(-10.7468377988928,12.2,-1.29238098875958));
#263834=CARTESIAN_POINT('Ctrl Pts',(-10.7432958887393,12.2,-1.29302735674216));
#263835=CARTESIAN_POINT('Ctrl Pts',(-10.7397539790683,12.2,-1.29367372463666));
#263836=CARTESIAN_POINT('Ctrl Pts',(-10.7362262945692,12.2,-1.29431132008108));
#263837=CARTESIAN_POINT('Ctrl Pts',(-10.7327129687994,12.2,-1.29494021469722));
#263838=CARTESIAN_POINT('Ctrl Pts',(-10.7291996425509,12.2,-1.29556910939905));
#263839=CARTESIAN_POINT('Ctrl Pts',(-10.7257006740177,12.2,-1.29618930044728));
#263840=CARTESIAN_POINT('Ctrl Pts',(-10.7222161947167,12.2,-1.29680086175838));
#263841=CARTESIAN_POINT('Ctrl Pts',(-10.7187317154157,12.2,-1.29741242306949));
#263842=CARTESIAN_POINT('Ctrl Pts',(-10.7152617276219,12.2,-1.2980153522907));
#263843=CARTESIAN_POINT('Ctrl Pts',(-10.7118063634351,12.2,-1.29860972182222));
#263844=CARTESIAN_POINT('Ctrl Pts',(-10.708350999719,12.2,-1.29920409127276));
#263845=CARTESIAN_POINT('Ctrl Pts',(-10.7049102600267,12.2,-1.29978990219976));
#263846=CARTESIAN_POINT('Ctrl Pts',(-10.7014842797357,12.2,-1.30036722626632));
#263847=CARTESIAN_POINT('Ctrl Pts',(-10.6980582989778,12.2,-1.30094455041154));
#263848=CARTESIAN_POINT('Ctrl Pts',(-10.6946470775727,12.2,-1.30151338699532));
#263849=CARTESIAN_POINT('Ctrl Pts',(-10.6912507509447,12.2,-1.30207381235834));
#263850=CARTESIAN_POINT('Ctrl Pts',(-10.6878544247794,12.2,-1.302634237645));
#263851=CARTESIAN_POINT('Ctrl Pts',(-10.6844729949817,12.2,-1.30318624926609));
#263852=CARTESIAN_POINT('Ctrl Pts',(-10.6811065985337,12.2,-1.30372992522219));
#263853=CARTESIAN_POINT('Ctrl Pts',(-10.677740201627,12.2,-1.30427360125237));
#263854=CARTESIAN_POINT('Ctrl Pts',(-10.6743888370076,12.2,-1.30480893958603));
#263855=CARTESIAN_POINT('Ctrl Pts',(-10.671052644216,12.2,-1.30533601658482));
#263856=CARTESIAN_POINT('Ctrl Pts',(-10.6677164518789,12.2,-1.30586309351179));
#263857=CARTESIAN_POINT('Ctrl Pts',(-10.6643954315011,12.2,-1.30638191048555));
#263858=CARTESIAN_POINT('Ctrl Pts',(-10.6610897237704,12.2,-1.30689254516656));
#263859=CARTESIAN_POINT('Ctrl Pts',(-10.6569575887691,12.2,-1.30753083857));
#263860=CARTESIAN_POINT('Ctrl Pts',(-10.6528493770518,12.2,-1.30815634585368));
#263861=CARTESIAN_POINT('Ctrl Pts',(-10.6487653687172,12.2,-1.30876922120156));
#263862=CARTESIAN_POINT('Ctrl Pts',(-10.6446813603826,12.2,-1.30938209654944));
#263863=CARTESIAN_POINT('Ctrl Pts',(-10.6406215523928,12.2,-1.3099823409248));
#263864=CARTESIAN_POINT('Ctrl Pts',(-10.6365862259855,12.2,-1.31057011273306));
#263865=CARTESIAN_POINT('Ctrl Pts',(-10.6325508995783,12.2,-1.31115788454132));
#263866=CARTESIAN_POINT('Ctrl Pts',(-10.6285400548445,12.2,-1.31173318297227));
#263867=CARTESIAN_POINT('Ctrl Pts',(-10.6245539749833,12.2,-1.31229616825005));
#263868=CARTESIAN_POINT('Ctrl Pts',(-10.6205678951222,12.2,-1.31285915352783));
#263869=CARTESIAN_POINT('Ctrl Pts',(-10.6166065801222,12.2,-1.31340982704449));
#263870=CARTESIAN_POINT('Ctrl Pts',(-10.6126703162333,12.2,-1.31394835301671));
#263871=CARTESIAN_POINT('Ctrl Pts',(-10.6087340523445,12.2,-1.31448687898893));
#263872=CARTESIAN_POINT('Ctrl Pts',(-10.6048228402266,12.2,-1.31501325585358));
#263873=CARTESIAN_POINT('Ctrl Pts',(-10.6009369697229,12.2,-1.31552765280032));
#263874=CARTESIAN_POINT('Ctrl Pts',(-10.5970510992192,12.2,-1.31604204974707));
#263875=CARTESIAN_POINT('Ctrl Pts',(-10.5931905711424,12.2,-1.3165444671549));
#263876=CARTESIAN_POINT('Ctrl Pts',(-10.589355678991,12.2,-1.31703507430706));
#263877=CARTESIAN_POINT('Ctrl Pts',(-10.5847538085765,12.2,-1.31762380286826));
#263878=CARTESIAN_POINT('Ctrl Pts',(-10.5801888532424,12.2,-1.31819552758083));
#263879=CARTESIAN_POINT('Ctrl Pts',(-10.5756613289886,12.2,-1.31875054897806));
#263880=CARTESIAN_POINT('Ctrl Pts',(-10.5711338047347,12.2,-1.31930557037529));
#263881=CARTESIAN_POINT('Ctrl Pts',(-10.5666437116344,12.2,-1.31984388876933));
#263882=CARTESIAN_POINT('Ctrl Pts',(-10.5621915732103,12.2,-1.32036581516815));
#263883=CARTESIAN_POINT('Ctrl Pts',(-10.5569974114458,12.2,-1.32097472933171));
#263884=CARTESIAN_POINT('Ctrl Pts',(-10.551854911308,12.2,-1.32156133035842));
#263885=CARTESIAN_POINT('Ctrl Pts',(-10.5467649145046,12.2,-1.32212612692359));
#263886=CARTESIAN_POINT('Ctrl Pts',(-10.5431292025587,12.2,-1.32252955303529));
#263887=CARTESIAN_POINT('Ctrl Pts',(-10.5395202811572,12.2,-1.32292185247585));
#263888=CARTESIAN_POINT('Ctrl Pts',(-10.5359384607936,12.2,-1.3233032169915));
#263889=CARTESIAN_POINT('Ctrl Pts',(-10.5309239122065,12.2,-1.32383712732172));
#263890=CARTESIAN_POINT('Ctrl Pts',(-10.5259624852953,12.2,-1.32434960229385));
#263891=CARTESIAN_POINT('Ctrl Pts',(-10.5210550497626,12.2,-1.32484117448127));
#263892=CARTESIAN_POINT('Ctrl Pts',(-10.5175497387223,12.2,-1.32519229746683));
#263893=CARTESIAN_POINT('Ctrl Pts',(-10.5140719783145,12.2,-1.32553275599477));
#263894=CARTESIAN_POINT('Ctrl Pts',(-10.5106220878663,12.2,-1.32586274982998));
#263895=CARTESIAN_POINT('Ctrl Pts',(-10.5071721974181,12.2,-1.32619274366518));
#263896=CARTESIAN_POINT('Ctrl Pts',(-10.5037501797926,12.2,-1.32651227168577));
#263897=CARTESIAN_POINT('Ctrl Pts',(-10.5003563627811,12.2,-1.32682153807382));
#263898=CARTESIAN_POINT('Ctrl Pts',(-10.4969625457695,12.2,-1.32713080446187));
#263899=CARTESIAN_POINT('Ctrl Pts',(-10.4935969288001,12.2,-1.32742980916087));
#263900=CARTESIAN_POINT('Ctrl Pts',(-10.4902598467885,12.2,-1.32771875902116));
#263901=CARTESIAN_POINT('Ctrl Pts',(-10.4862553485201,12.2,-1.32806549884092));
#263902=CARTESIAN_POINT('Ctrl Pts',(-10.4822919381671,12.2,-1.32839776190449));
#263903=CARTESIAN_POINT('Ctrl Pts',(-10.4783702020614,12.2,-1.32871591547565));
#263904=CARTESIAN_POINT('Ctrl Pts',(-10.4744484659558,12.2,-1.32903406904681));
#263905=CARTESIAN_POINT('Ctrl Pts',(-10.4705684047967,12.2,-1.32933811107744));
#263906=CARTESIAN_POINT('Ctrl Pts',(-10.4667306136843,12.2,-1.32962842173416));
#263907=CARTESIAN_POINT('Ctrl Pts',(-10.4628928225719,12.2,-1.32991873239088));
#263908=CARTESIAN_POINT('Ctrl Pts',(-10.4590973010339,12.2,-1.330195309855));
#263909=CARTESIAN_POINT('Ctrl Pts',(-10.4553446579174,12.2,-1.33045854276301));
#263910=CARTESIAN_POINT('Ctrl Pts',(-10.4515920144599,12.2,-1.33072177569494));
#263911=CARTESIAN_POINT('Ctrl Pts',(-10.4478822474316,12.2,-1.33097166385054));
#263912=CARTESIAN_POINT('Ctrl Pts',(-10.444215977067,12.2,-1.33120860752956));
#263913=CARTESIAN_POINT('Ctrl Pts',(-10.4405497070355,12.2,-1.33144555118706));
#263914=CARTESIAN_POINT('Ctrl Pts',(-10.4369269315713,12.2,-1.33166954730663));
#263915=CARTESIAN_POINT('Ctrl Pts',(-10.4333482845183,12.2,-1.33188100629994));
#263916=CARTESIAN_POINT('Ctrl Pts',(-10.429173196073,12.2,-1.3321277084716));
#263917=CARTESIAN_POINT('Ctrl Pts',(-10.4250581674828,12.2,-1.33235734853502));
#263918=CARTESIAN_POINT('Ctrl Pts',(-10.4210042213525,12.2,-1.33257059080161));
#263919=CARTESIAN_POINT('Ctrl Pts',(-10.417529410564,12.2,-1.33275336987778));
#263920=CARTESIAN_POINT('Ctrl Pts',(-10.4140994778273,12.2,-1.33292410608833));
#263921=CARTESIAN_POINT('Ctrl Pts',(-10.4107150809348,12.2,-1.33308322924996));
#263922=CARTESIAN_POINT('Ctrl Pts',(-10.4073306840424,12.2,-1.33324235241159));
#263923=CARTESIAN_POINT('Ctrl Pts',(-10.4039918233424,12.2,-1.33338986613936));
#263924=CARTESIAN_POINT('Ctrl Pts',(-10.4006991696256,12.2,-1.3335262159685));
#263925=CARTESIAN_POINT('Ctrl Pts',(-10.3974065156096,12.2,-1.33366256581003));
#263926=CARTESIAN_POINT('Ctrl Pts',(-10.3941600695731,12.2,-1.33378775019212));
#263927=CARTESIAN_POINT('Ctrl Pts',(-10.3909605148175,12.2,-1.33390223044789));
#263928=CARTESIAN_POINT('Ctrl Pts',(-10.3877609603524,12.2,-1.33401671069327));
#263929=CARTESIAN_POINT('Ctrl Pts',(-10.3846082998028,12.2,-1.33412048741961));
#263930=CARTESIAN_POINT('Ctrl Pts',(-10.3815032322347,12.2,-1.33421403074999));
#263931=CARTESIAN_POINT('Ctrl Pts',(-10.3783981646667,12.2,-1.33430757408037));
#263932=CARTESIAN_POINT('Ctrl Pts',(-10.3753406896553,12.2,-1.33439088666069));
#263933=CARTESIAN_POINT('Ctrl Pts',(-10.3723315240947,12.2,-1.33446445299201));
#263934=CARTESIAN_POINT('Ctrl Pts',(-10.3688208307584,12.2,-1.33455028038301));
#263935=CARTESIAN_POINT('Ctrl Pts',(-10.3653758880138,12.2,-1.33462284149322));
#263936=CARTESIAN_POINT('Ctrl Pts',(-10.3619978645013,12.2,-1.33468293571667));
#263937=CARTESIAN_POINT('Ctrl Pts',(-10.358137266314,12.2,-1.33475161482719));
#263938=CARTESIAN_POINT('Ctrl Pts',(-10.3543640668174,12.2,-1.3348040075846));
#263939=CARTESIAN_POINT('Ctrl Pts',(-10.3506800556424,12.2,-1.33484134947347));
#263940=CARTESIAN_POINT('Ctrl Pts',(-10.347917047324,12.2,-1.33486935588948));
#263941=CARTESIAN_POINT('Ctrl Pts',(-10.3452042073052,12.2,-1.33488889724864));
#263942=CARTESIAN_POINT('Ctrl Pts',(-10.3425423128151,12.2,-1.33490051274876));
#263943=CARTESIAN_POINT('Ctrl Pts',(-10.3398804180833,12.2,-1.33491212824994));
#263944=CARTESIAN_POINT('Ctrl Pts',(-10.3372694660563,12.2,-1.33491581842531));
#263945=CARTESIAN_POINT('Ctrl Pts',(-10.3347102518357,12.2,-1.33491213900813));
#263946=CARTESIAN_POINT('Ctrl Pts',(-10.3321510378476,12.2,-1.33490845959128));
#263947=CARTESIAN_POINT('Ctrl Pts',(-10.3296435620565,12.2,-1.33489741024112));
#263948=CARTESIAN_POINT('Ctrl Pts',(-10.3271886359678,12.2,-1.3348795649917));
#263949=CARTESIAN_POINT('Ctrl Pts',(-10.3243245553822,12.2,-1.33485874553297));
#263950=CARTESIAN_POINT('Ctrl Pts',(-10.3215320018072,12.2,-1.33482867661023));
#263951=CARTESIAN_POINT('Ctrl Pts',(-10.3188123009065,12.2,-1.33479029774821));
#263952=CARTESIAN_POINT('Ctrl Pts',(-10.3160926002175,12.2,-1.33475191888917));
#263953=CARTESIAN_POINT('Ctrl Pts',(-10.3134457526233,12.2,-1.33470523165128));
#263954=CARTESIAN_POINT('Ctrl Pts',(-10.3108731234737,12.2,-1.33465121353007));
#263955=CARTESIAN_POINT('Ctrl Pts',(-10.3086680125165,12.2,-1.33460491227792));
#263956=CARTESIAN_POINT('Ctrl Pts',(-10.3065174318478,12.2,-1.33455322546687));
#263957=CARTESIAN_POINT('Ctrl Pts',(-10.3044222659027,12.2,-1.3344967904636));
#263958=CARTESIAN_POINT('Ctrl Pts',(-10.3023271001479,12.2,-1.33444035546544));
#263959=CARTESIAN_POINT('Ctrl Pts',(-10.3002873493213,12.2,-1.33437917274797));
#263960=CARTESIAN_POINT('Ctrl Pts',(-10.2983039235509,12.2,-1.33431390075005));
#263961=CARTESIAN_POINT('Ctrl Pts',(-10.2950077328095,12.2,-1.33420542734085));
#263962=CARTESIAN_POINT('Ctrl Pts',(-10.2918670873981,12.2,-1.33408564009489));
#263963=CARTESIAN_POINT('Ctrl Pts',(-10.2888863240001,12.2,-1.33395773200002));
#263964=CARTESIAN_POINT('Ctrl Pts',(-10.2888863240001,15.2,-1.33395773200002));
#263965=CARTESIAN_POINT('Ctrl Pts',(-10.2906713387415,15.2,-1.33403432910097));
#263966=CARTESIAN_POINT('Ctrl Pts',(-10.2925136934523,15.2,-1.33410802241805));
#263967=CARTESIAN_POINT('Ctrl Pts',(-10.2944124475503,15.2,-1.33417810627568));
#263968=CARTESIAN_POINT('Ctrl Pts',(-10.2963203584004,15.2,-1.3342485281131));
#263969=CARTESIAN_POINT('Ctrl Pts',(-10.2982852153479,15.2,-1.33431531312478));
#263970=CARTESIAN_POINT('Ctrl Pts',(-10.3003060912289,15.2,-1.33437778604772));
#263971=CARTESIAN_POINT('Ctrl Pts',(-10.3026637794814,15.2,-1.33445067111597));
#263972=CARTESIAN_POINT('Ctrl Pts',(-10.3050977134762,15.2,-1.33451768705885));
#263973=CARTESIAN_POINT('Ctrl Pts',(-10.3076064654823,15.2,-1.33457780198607));
#263974=CARTESIAN_POINT('Ctrl Pts',(-10.3097568245957,15.2,-1.33462932907256));
#263975=CARTESIAN_POINT('Ctrl Pts',(-10.3119621540712,15.2,-1.33467578925836));
#263976=CARTESIAN_POINT('Ctrl Pts',(-10.314221578227,15.2,-1.33471655051229));
#263977=CARTESIAN_POINT('Ctrl Pts',(-10.3168575727676,15.2,-1.33476410530298));
#263978=CARTESIAN_POINT('Ctrl Pts',(-10.319567196023,15.2,-1.33480390623188));
#263979=CARTESIAN_POINT('Ctrl Pts',(-10.3223490987067,15.2,-1.33483499002212));
#263980=CARTESIAN_POINT('Ctrl Pts',(-10.3247335869998,15.2,-1.334861633274));
#263981=CARTESIAN_POINT('Ctrl Pts',(-10.3271711798945,15.2,-1.33488187265031));
#263982=CARTESIAN_POINT('Ctrl Pts',(-10.329661049491,15.2,-1.33489512398462));
#263983=CARTESIAN_POINT('Ctrl Pts',(-10.3321509188613,15.2,-1.33490837531773));
#263984=CARTESIAN_POINT('Ctrl Pts',(-10.3346930649442,15.2,-1.33491463737498));
#263985=CARTESIAN_POINT('Ctrl Pts',(-10.3372866821833,15.2,-1.33491334179169));
#263986=CARTESIAN_POINT('Ctrl Pts',(-10.3398802994224,15.2,-1.33491204620841));
#263987=CARTESIAN_POINT('Ctrl Pts',(-10.3425253879222,15.2,-1.33490319475141));
#263988=CARTESIAN_POINT('Ctrl Pts',(-10.3452211602893,15.2,-1.33488623525165));
#263989=CARTESIAN_POINT('Ctrl Pts',(-10.3479169329013,15.2,-1.33486927575035));
#263990=CARTESIAN_POINT('Ctrl Pts',(-10.3506633886323,15.2,-1.33484420971545));
#263991=CARTESIAN_POINT('Ctrl Pts',(-10.3534597592881,15.2,-1.33481050221302));
#263992=CARTESIAN_POINT('Ctrl Pts',(-10.3562561296899,15.2,-1.33477679471366));
#263993=CARTESIAN_POINT('Ctrl Pts',(-10.3591024159266,15.2,-1.33473444504839));
#263994=CARTESIAN_POINT('Ctrl Pts',(-10.3619978645013,15.2,-1.33468293571667));
#263995=CARTESIAN_POINT('Ctrl Pts',(-10.364893313076,15.2,-1.33463142638496));
#263996=CARTESIAN_POINT('Ctrl Pts',(-10.3678379272646,15.2,-1.33457075874251));
#263997=CARTESIAN_POINT('Ctrl Pts',(-10.3708309698204,15.2,-1.33450042649549));
#263998=CARTESIAN_POINT('Ctrl Pts',(-10.3738240126481,15.2,-1.33443009424208));
#263999=CARTESIAN_POINT('Ctrl Pts',(-10.3768654853318,15.2,-1.33435009930414));
#264000=CARTESIAN_POINT('Ctrl Pts',(-10.3799546683367,15.2,-1.3342599522152));
#264001=CARTESIAN_POINT('Ctrl Pts',(-10.383043851061,15.2,-1.33416980513445));
#264002=CARTESIAN_POINT('Ctrl Pts',(-10.3861807463457,15.2,-1.33406950702371));
#264003=CARTESIAN_POINT('Ctrl Pts',(-10.3893646491487,15.2,-1.33395858102728));
#264004=CARTESIAN_POINT('Ctrl Pts',(-10.3925485519517,15.2,-1.33384765503084));
#264005=CARTESIAN_POINT('Ctrl Pts',(-10.3957794643427,15.2,-1.33372610281025));
#264006=CARTESIAN_POINT('Ctrl Pts',(-10.3990566960549,15.2,-1.33359346256555));
#264007=CARTESIAN_POINT('Ctrl Pts',(-10.4023339280648,15.2,-1.3334608223088));
#264008=CARTESIAN_POINT('Ctrl Pts',(-10.4056574817472,15.2,-1.33331709156735));
#264009=CARTESIAN_POINT('Ctrl Pts',(-10.4090266809339,15.2,-1.33316182547477));
#264010=CARTESIAN_POINT('Ctrl Pts',(-10.4123958798146,15.2,-1.3330065593963));
#264011=CARTESIAN_POINT('Ctrl Pts',(-10.4158107252875,15.2,-1.3328397546176));
#264012=CARTESIAN_POINT('Ctrl Pts',(-10.4192705589137,15.2,-1.33266097845691));
#264013=CARTESIAN_POINT('Ctrl Pts',(-10.4233070316872,15.2,-1.33245240625861));
#264014=CARTESIAN_POINT('Ctrl Pts',(-10.4274047334869,15.2,-1.33222753370442));
#264015=CARTESIAN_POINT('Ctrl Pts',(-10.4315626413885,15.2,-1.33198569293577));
#264016=CARTESIAN_POINT('Ctrl Pts',(-10.435126562262,15.2,-1.33177840085911));
#264017=CARTESIAN_POINT('Ctrl Pts',(-10.4387347159883,15.2,-1.33155864115441));
#264018=CARTESIAN_POINT('Ctrl Pts',(-10.4423864699409,15.2,-1.33132600224564));
#264019=CARTESIAN_POINT('Ctrl Pts',(-10.4478641008697,15.2,-1.33097704388247));
#264020=CARTESIAN_POINT('Ctrl Pts',(-10.4534398288274,15.2,-1.33059910656405));
#264021=CARTESIAN_POINT('Ctrl Pts',(-10.459111570651,15.2,-1.33019084730967));
#264022=CARTESIAN_POINT('Ctrl Pts',(-10.4628927322101,15.2,-1.32991867444869));
#264023=CARTESIAN_POINT('Ctrl Pts',(-10.4667165679495,15.2,-1.32963302655132));
#264024=CARTESIAN_POINT('Ctrl Pts',(-10.470582473413,15.2,-1.32933351970072));
#264025=CARTESIAN_POINT('Ctrl Pts',(-10.4757370136799,15.2,-1.32893417726047));
#264026=CARTESIAN_POINT('Ctrl Pts',(-10.4809663449806,15.2,-1.32851019518761));
#264027=CARTESIAN_POINT('Ctrl Pts',(-10.4862690668431,15.2,-1.32806068772572));
#264028=CARTESIAN_POINT('Ctrl Pts',(-10.4902461081497,15.2,-1.32772355713696));
#264029=CARTESIAN_POINT('Ctrl Pts',(-10.4942644315975,15.2,-1.32737207171173));
#264030=CARTESIAN_POINT('Ctrl Pts',(-10.4983234597833,15.2,-1.32700586797504));
#264031=CARTESIAN_POINT('Ctrl Pts',(-10.5017059833944,15.2,-1.32670069818338));
#264032=CARTESIAN_POINT('Ctrl Pts',(-10.505116773614,15.2,-1.32638530727359));
#264033=CARTESIAN_POINT('Ctrl Pts',(-10.5085555014769,15.2,-1.32605949171653));
#264034=CARTESIAN_POINT('Ctrl Pts',(-10.5119942293398,15.2,-1.32573367615947));
#264035=CARTESIAN_POINT('Ctrl Pts',(-10.5154608943717,15.2,-1.32539743567784));
#264036=CARTESIAN_POINT('Ctrl Pts',(-10.5189551722203,15.2,-1.32505057026062));
#264037=CARTESIAN_POINT('Ctrl Pts',(-10.522449450069,15.2,-1.3247037048434));
#264038=CARTESIAN_POINT('Ctrl Pts',(-10.525971341803,15.2,-1.32434621568201));
#264039=CARTESIAN_POINT('Ctrl Pts',(-10.5295205239573,15.2,-1.32397790450089));
#264040=CARTESIAN_POINT('Ctrl Pts',(-10.5330697061115,15.2,-1.32360959331977));
#264041=CARTESIAN_POINT('Ctrl Pts',(-10.5366461820254,15.2,-1.32323046192497));
#264042=CARTESIAN_POINT('Ctrl Pts',(-10.5402496341517,15.2,-1.32284031898805));
#264043=CARTESIAN_POINT('Ctrl Pts',(-10.543853086278,15.2,-1.32245017605112));
#264044=CARTESIAN_POINT('Ctrl Pts',(-10.5474835150206,15.2,-1.32204901959146));
#264045=CARTESIAN_POINT('Ctrl Pts',(-10.551140607245,15.2,-1.32163666493777));
#264046=CARTESIAN_POINT('Ctrl Pts',(-10.5547976994694,15.2,-1.32122431028407));
#264047=CARTESIAN_POINT('Ctrl Pts',(-10.558481457722,15.2,-1.32080075384964));
#264048=CARTESIAN_POINT('Ctrl Pts',(-10.5621915732103,15.2,-1.32036581516815));
#264049=CARTESIAN_POINT('Ctrl Pts',(-10.5659016882941,15.2,-1.31993087653407));
#264050=CARTESIAN_POINT('Ctrl Pts',(-10.5696381619368,15.2,-1.31948455459797));
#264051=CARTESIAN_POINT('Ctrl Pts',(-10.5734006879829,15.2,-1.3190266693016));
#264052=CARTESIAN_POINT('Ctrl Pts',(-10.5771632144391,15.2,-1.31856878395532));
#264053=CARTESIAN_POINT('Ctrl Pts',(-10.5809517962087,15.2,-1.31809933588424));
#264054=CARTESIAN_POINT('Ctrl Pts',(-10.5847661325261,15.2,-1.31761814657965));
#264055=CARTESIAN_POINT('Ctrl Pts',(-10.5893433363564,15.2,-1.31704071938266));
#264056=CARTESIAN_POINT('Ctrl Pts',(-10.5939576252204,15.2,-1.31644638797239));
#264057=CARTESIAN_POINT('Ctrl Pts',(-10.5986084914583,15.2,-1.31583485440751));
#264058=CARTESIAN_POINT('Ctrl Pts',(-10.6024842131121,15.2,-1.31532524313121));
#264059=CARTESIAN_POINT('Ctrl Pts',(-10.6063853355615,15.2,-1.31480368478678));
#264060=CARTESIAN_POINT('Ctrl Pts',(-10.6103115670219,15.2,-1.31427001193857));
#264061=CARTESIAN_POINT('Ctrl Pts',(-10.6158082907241,15.2,-1.31352286999761));
#264062=CARTESIAN_POINT('Ctrl Pts',(-10.6213542277175,15.2,-1.31275198199561));
#264063=CARTESIAN_POINT('Ctrl Pts',(-10.6269485919773,15.2,-1.31195689832433));
#264064=CARTESIAN_POINT('Ctrl Pts',(-10.6309445666975,15.2,-1.31138898138089));
#264065=CARTESIAN_POINT('Ctrl Pts',(-10.6349652493134,15.2,-1.31080871873089));
#264066=CARTESIAN_POINT('Ctrl Pts',(-10.6390103568055,15.2,-1.31021595182715));
#264067=CARTESIAN_POINT('Ctrl Pts',(-10.6430554642976,15.2,-1.3096231849234));
#264068=CARTESIAN_POINT('Ctrl Pts',(-10.6471249966725,15.2,-1.30901791343972));
#264069=CARTESIAN_POINT('Ctrl Pts',(-10.6512186754907,15.2,-1.30839997906539));
#264070=CARTESIAN_POINT('Ctrl Pts',(-10.6553123543089,15.2,-1.30778204469104));
#264071=CARTESIAN_POINT('Ctrl Pts',(-10.6594301784139,15.2,-1.30715144689694));
#264072=CARTESIAN_POINT('Ctrl Pts',(-10.6635718732043,15.2,-1.30650803405038));
#264073=CARTESIAN_POINT('Ctrl Pts',(-10.6677135679947,15.2,-1.30586462120383));
#264074=CARTESIAN_POINT('Ctrl Pts',(-10.6718791328065,15.2,-1.30520839202564));
#264075=CARTESIAN_POINT('Ctrl Pts',(-10.6760682944227,15.2,-1.30453919521708));
#264076=CARTESIAN_POINT('Ctrl Pts',(-10.6802574560389,15.2,-1.30386999840852));
#264077=CARTESIAN_POINT('Ctrl Pts',(-10.6844702153,15.2,-1.30318783430561));
#264078=CARTESIAN_POINT('Ctrl Pts',(-10.6887063019667,15.2,-1.30249255500005));
#264079=CARTESIAN_POINT('Ctrl Pts',(-10.6920951714847,15.2,-1.30193633152529));
#264080=CARTESIAN_POINT('Ctrl Pts',(-10.6954989715822,15.2,-1.30137171455233));
#264081=CARTESIAN_POINT('Ctrl Pts',(-10.6989175643256,15.2,-1.30079862913134));
#264082=CARTESIAN_POINT('Ctrl Pts',(-10.7023361566032,15.2,-1.30022554378844));
#264083=CARTESIAN_POINT('Ctrl Pts',(-10.7057695414556,15.2,-1.29964398993542));
#264084=CARTESIAN_POINT('Ctrl Pts',(-10.7092175850227,15.2,-1.29905389525878));
#264085=CARTESIAN_POINT('Ctrl Pts',(-10.7143896506082,15.2,-1.29816875320362));
#264086=CARTESIAN_POINT('Ctrl Pts',(-10.7195946954383,15.2,-1.29726439269918));
#264087=CARTESIAN_POINT('Ctrl Pts',(-10.7248322682458,15.2,-1.29634057156741));
#264088=CARTESIAN_POINT('Ctrl Pts',(-10.7291969124106,15.2,-1.2955707205963));
#264089=CARTESIAN_POINT('Ctrl Pts',(-10.7335841449306,15.2,-1.2947873542425));
#264090=CARTESIAN_POINT('Ctrl Pts',(-10.7379937092465,15.2,-1.29399033809252));
#264091=CARTESIAN_POINT('Ctrl Pts',(-10.7415213608915,15.2,-1.29335272513779));
#264092=CARTESIAN_POINT('Ctrl Pts',(-10.7450633034961,15.2,-1.29270637431324));
#264093=CARTESIAN_POINT('Ctrl Pts',(-10.7486194070242,15.2,-1.29205121822141));
#264094=CARTESIAN_POINT('Ctrl Pts',(-10.7521755100677,15.2,-1.29139606221884));
#264095=CARTESIAN_POINT('Ctrl Pts',(-10.7557457737529,15.2,-1.29073209939859));
#264096=CARTESIAN_POINT('Ctrl Pts',(-10.7593300686806,15.2,-1.29005926334339));
#264097=CARTESIAN_POINT('Ctrl Pts',(-10.7629143640968,15.2,-1.28938642719651));
#264098=CARTESIAN_POINT('Ctrl Pts',(-10.7665126894836,15.2,-1.28870471745705));
#264099=CARTESIAN_POINT('Ctrl Pts',(-10.7701249182525,15.2,-1.28801406674958));
#264100=CARTESIAN_POINT('Ctrl Pts',(-10.7737371465292,15.2,-1.28732341613621));
#264101=CARTESIAN_POINT('Ctrl Pts',(-10.7773632748011,15.2,-1.28662382462094));
#264102=CARTESIAN_POINT('Ctrl Pts',(-10.7810031791132,15.2,-1.28591522662424));
#264103=CARTESIAN_POINT('Ctrl Pts',(-10.7855530598753,15.2,-1.28502947905594));
#264104=CARTESIAN_POINT('Ctrl Pts',(-10.7901244635677,15.2,-1.28412965881288));
#264105=CARTESIAN_POINT('Ctrl Pts',(-10.7947171418993,15.2,-1.2832156381196));
#264106=CARTESIAN_POINT('Ctrl Pts',(-10.7983912847648,15.2,-1.28248442152512));
#264107=CARTESIAN_POINT('Ctrl Pts',(-10.802079043534,15.2,-1.28174411832992));
#264108=CARTESIAN_POINT('Ctrl Pts',(-10.8057802937525,15.2,-1.28099466367454));
#264109=CARTESIAN_POINT('Ctrl Pts',(-10.8094815434668,15.2,-1.28024520912126));
#264110=CARTESIAN_POINT('Ctrl Pts',(-10.8131962844855,15.2,-1.27948660363966));
#264111=CARTESIAN_POINT('Ctrl Pts',(-10.8169243916238,15.2,-1.27871878492559));
#264112=CARTESIAN_POINT('Ctrl Pts',(-10.8215845259277,15.2,-1.27775901145454));
#264113=CARTESIAN_POINT('Ctrl Pts',(-10.8262655452923,15.2,-1.27678483963929));
#264114=CARTESIAN_POINT('Ctrl Pts',(-10.83096721036,15.2,-1.27579615290437));
#264115=CARTESIAN_POINT('Ctrl Pts',(-10.8347285426192,15.2,-1.27500520347332));
#264116=CARTESIAN_POINT('Ctrl Pts',(-10.8385030876956,15.2,-1.27420496198066));
#264117=CARTESIAN_POINT('Ctrl Pts',(-10.8422907232526,15.2,-1.27339537126616));
#264118=CARTESIAN_POINT('Ctrl Pts',(-10.8489190852193,15.2,-1.27197858757095));
#264119=CARTESIAN_POINT('Ctrl Pts',(-10.8555875370922,15.2,-1.27053316286473));
#264120=CARTESIAN_POINT('Ctrl Pts',(-10.8622954308934,15.2,-1.26905878560396));
#264121=CARTESIAN_POINT('Ctrl Pts',(-10.8661285126925,15.2,-1.26821628439409));
#264122=CARTESIAN_POINT('Ctrl Pts',(-10.8699744735899,15.2,-1.26736432863545));
#264123=CARTESIAN_POINT('Ctrl Pts',(-10.873833194718,15.2,-1.26650286009539));
#264124=CARTESIAN_POINT('Ctrl Pts',(-10.8786565965225,15.2,-1.26542602433228));
#264125=CARTESIAN_POINT('Ctrl Pts',(-10.8834999359364,15.2,-1.26433432554453));
#264126=CARTESIAN_POINT('Ctrl Pts',(-10.888362980264,15.2,-1.26322765227565));
#264127=CARTESIAN_POINT('Ctrl Pts',(-10.8922534159381,15.2,-1.2623423136123));
#264128=CARTESIAN_POINT('Ctrl Pts',(-10.8961564639672,15.2,-1.26144739104688));
#264129=CARTESIAN_POINT('Ctrl Pts',(-10.9000720063485,15.2,-1.26054282855215));
#264130=CARTESIAN_POINT('Ctrl Pts',(-10.9039875481964,15.2,-1.25963826618067));
#264131=CARTESIAN_POINT('Ctrl Pts',(-10.9079155838343,15.2,-1.25872406573544));
#264132=CARTESIAN_POINT('Ctrl Pts',(-10.911855998178,15.2,-1.25780016986716));
#264133=CARTESIAN_POINT('Ctrl Pts',(-10.9157964130586,15.2,-1.25687627387299));
#264134=CARTESIAN_POINT('Ctrl Pts',(-10.9197492047296,15.2,-1.255942682261));
#264135=CARTESIAN_POINT('Ctrl Pts',(-10.9237142590576,15.2,-1.25499934293117));
#264136=CARTESIAN_POINT('Ctrl Pts',(-10.9286705766975,15.2,-1.25382016883316));
#264137=CARTESIAN_POINT('Ctrl Pts',(-10.9336460544901,15.2,-1.2526257623933));
#264138=CARTESIAN_POINT('Ctrl Pts',(-10.9386404673799,15.2,-1.25141601760956));
#264139=CARTESIAN_POINT('Ctrl Pts',(-10.942635997365,15.2,-1.25044822186169));
#264140=CARTESIAN_POINT('Ctrl Pts',(-10.9466436456065,15.2,-1.24947061170765));
#264141=CARTESIAN_POINT('Ctrl Pts',(-10.9506632993882,15.2,-1.24848313328902));
#264142=CARTESIAN_POINT('Ctrl Pts',(-10.9556878670261,15.2,-1.24724878516483));
#264143=CARTESIAN_POINT('Ctrl Pts',(-10.9607311917589,15.2,-1.24599901938746));
#264144=CARTESIAN_POINT('Ctrl Pts',(-10.9657930537024,15.2,-1.24473373362438));
#264145=CARTESIAN_POINT('Ctrl Pts',(-10.9708549156459,15.2,-1.2434684478613));
#264146=CARTESIAN_POINT('Ctrl Pts',(-10.9759353155186,15.2,-1.2421876429066));
#264147=CARTESIAN_POINT('Ctrl Pts',(-10.9810340340139,15.2,-1.24089121977576));
#264148=CARTESIAN_POINT('Ctrl Pts',(-10.9851130090325,15.2,-1.23985408121456));
#264149=CARTESIAN_POINT('Ctrl Pts',(-10.9892037076405,15.2,-1.23880694764417));
#264150=CARTESIAN_POINT('Ctrl Pts',(-10.9933060194207,15.2,-1.23774976908553));
#264151=CARTESIAN_POINT('Ctrl Pts',(-10.9984339088666,15.2,-1.23642829595925));
#264152=CARTESIAN_POINT('Ctrl Pts',(-11.0035799444407,15.2,-1.23509112729103));
#264153=CARTESIAN_POINT('Ctrl Pts',(-11.0087439096505,15.2,-1.23373816833142));
#264154=CARTESIAN_POINT('Ctrl Pts',(-11.0128750814806,15.2,-1.23265580125221));
#264155=CARTESIAN_POINT('Ctrl Pts',(-11.0170177294263,15.2,-1.23156332727119));
#264156=CARTESIAN_POINT('Ctrl Pts',(-11.0211717432722,15.2,-1.23046070080081));
#264157=CARTESIAN_POINT('Ctrl Pts',(-11.027402764324,15.2,-1.22880676102011));
#264158=CARTESIAN_POINT('Ctrl Pts',(-11.0336593575536,15.2,-1.22712997358033));
#264159=CARTESIAN_POINT('Ctrl Pts',(-11.0399411605736,15.2,-1.22543018189366));
#264160=CARTESIAN_POINT('Ctrl Pts',(-11.044129029634,15.2,-1.22429698733295));
#264161=CARTESIAN_POINT('Ctrl Pts',(-11.0483281021154,15.2,-1.2231535688452));
#264162=CARTESIAN_POINT('Ctrl Pts',(-11.0525382712529,15.2,-1.22199987899927));
#264163=CARTESIAN_POINT('Ctrl Pts',(-11.0567484398168,15.2,-1.22084618931053));
#264164=CARTESIAN_POINT('Ctrl Pts',(-11.0609697047996,15.2,-1.21968222907277));
#264165=CARTESIAN_POINT('Ctrl Pts',(-11.0652019593414,15.2,-1.21850795339204));
#264166=CARTESIAN_POINT('Ctrl Pts',(-11.0694342144598,15.2,-1.21733367755132));
#264167=CARTESIAN_POINT('Ctrl Pts',(-11.073677459532,15.2,-1.21614908547629));
#264168=CARTESIAN_POINT('Ctrl Pts',(-11.0779315880417,15.2,-1.21495413296673));
#264169=CARTESIAN_POINT('Ctrl Pts',(-11.0821857165513,15.2,-1.21375918045716));
#264170=CARTESIAN_POINT('Ctrl Pts',(-11.0864507294622,15.2,-1.21255386732693));
#264171=CARTESIAN_POINT('Ctrl Pts',(-11.0907265199741,15.2,-1.21133815009294));
#264172=CARTESIAN_POINT('Ctrl Pts',(-11.0939333625668,15.2,-1.21042636225027));
#264173=CARTESIAN_POINT('Ctrl Pts',(-11.097146268145,15.2,-1.20950872135125));
#264174=CARTESIAN_POINT('Ctrl Pts',(-11.1003651928562,15.2,-1.20858520954632));
#264175=CARTESIAN_POINT('Ctrl Pts',(-11.1057300675698,15.2,-1.20704602314885));
#264176=CARTESIAN_POINT('Ctrl Pts',(-11.1111116610158,15.2,-1.20549052939023));
#264177=CARTESIAN_POINT('Ctrl Pts',(-11.1165097696978,15.2,-1.20391864306944));
#264178=CARTESIAN_POINT('Ctrl Pts',(-11.1197486347892,15.2,-1.20297551131124));
#264179=CARTESIAN_POINT('Ctrl Pts',(-11.122993445822,15.2,-1.20202647842835));
#264180=CARTESIAN_POINT('Ctrl Pts',(-11.1262441588711,15.2,-1.2010715276292));
#264181=CARTESIAN_POINT('Ctrl Pts',(-11.1305784427397,15.2,-1.19979825995483));
#264182=CARTESIAN_POINT('Ctrl Pts',(-11.1349232189575,15.2,-1.19851446950407));
#264183=CARTESIAN_POINT('Ctrl Pts',(-11.1392783851514,15.2,-1.19722011571282));
#264184=CARTESIAN_POINT('Ctrl Pts',(-11.1425447599452,15.2,-1.19624935032529));
#264185=CARTESIAN_POINT('Ctrl Pts',(-11.1458169791386,15.2,-1.19527264272776));
#264186=CARTESIAN_POINT('Ctrl Pts',(-11.1490949992687,15.2,-1.1942899759726));
#264187=CARTESIAN_POINT('Ctrl Pts',(-11.1523730199944,15.2,-1.19330730903893));
#264188=CARTESIAN_POINT('Ctrl Pts',(-11.155656842005,15.2,-1.19231868312859));
#264189=CARTESIAN_POINT('Ctrl Pts',(-11.1589464226921,15.2,-1.1913240797749));
#264190=CARTESIAN_POINT('Ctrl Pts',(-11.1622360027817,15.2,-1.19032947660189));
#264191=CARTESIAN_POINT('Ctrl Pts',(-11.1655313414627,15.2,-1.18932889818752));
#264192=CARTESIAN_POINT('Ctrl Pts',(-11.1688323950933,15.2,-1.18832232589024));
#264193=CARTESIAN_POINT('Ctrl Pts',(-11.1732337997341,15.2,-1.18698022955482));
#264194=CARTESIAN_POINT('Ctrl Pts',(-11.1776453663527,15.2,-1.18562747753135));
#264195=CARTESIAN_POINT('Ctrl Pts',(-11.1820669926001,15.2,-1.18426403246451));
#264196=CARTESIAN_POINT('Ctrl Pts',(-11.1853832124363,15.2,-1.18324144861794));
#264197=CARTESIAN_POINT('Ctrl Pts',(-11.1887050921963,15.2,-1.18221284900386));
#264198=CARTESIAN_POINT('Ctrl Pts',(-11.192032588283,15.2,-1.1811782177506));
#264199=CARTESIAN_POINT('Ctrl Pts',(-11.1953600849741,15.2,-1.18014358630939));
#264200=CARTESIAN_POINT('Ctrl Pts',(-11.1986931977752,15.2,-1.17910292269149));
#264201=CARTESIAN_POINT('Ctrl Pts',(-11.2020318859695,15.2,-1.1780562112052));
#264202=CARTESIAN_POINT('Ctrl Pts',(-11.2053705735573,15.2,-1.17700949990907));
#264203=CARTESIAN_POINT('Ctrl Pts',(-11.2087148357031,15.2,-1.1759567397466));
#264204=CARTESIAN_POINT('Ctrl Pts',(-11.2120646308319,15.2,-1.17489791636787));
#264205=CARTESIAN_POINT('Ctrl Pts',(-11.2176476229161,15.2,-1.17313321067255));
#264206=CARTESIAN_POINT('Ctrl Pts',(-11.2232459852591,15.2,-1.17135165884336));
#264207=CARTESIAN_POINT('Ctrl Pts',(-11.2288595241517,15.2,-1.16955319055789));
#264208=CARTESIAN_POINT('Ctrl Pts',(-11.2322276473649,15.2,-1.16847410962581));
#264209=CARTESIAN_POINT('Ctrl Pts',(-11.2356012328241,15.2,-1.16738893674188));
#264210=CARTESIAN_POINT('Ctrl Pts',(-11.2389802419101,15.2,-1.16629765936434));
#264211=CARTESIAN_POINT('Ctrl Pts',(-11.2423592509961,15.2,-1.16520638198679));
#264212=CARTESIAN_POINT('Ctrl Pts',(-11.2457436822565,15.2,-1.16410899759329));
#264213=CARTESIAN_POINT('Ctrl Pts',(-11.249133494425,15.2,-1.16300549275839));
#264214=CARTESIAN_POINT('Ctrl Pts',(-11.2547831815778,15.2,-1.16116631796673));
#264215=CARTESIAN_POINT('Ctrl Pts',(-11.2604478168889,15.2,-1.15931013866118));
#264216=CARTESIAN_POINT('Ctrl Pts',(-11.2661272105,15.2,-1.1574368865084));
#264217=CARTESIAN_POINT('Ctrl Pts',(-11.2718066041111,15.2,-1.15556363435561));
#264218=CARTESIAN_POINT('Ctrl Pts',(-11.2775007568383,15.2,-1.15367330726883));
#264219=CARTESIAN_POINT('Ctrl Pts',(-11.2832094782531,15.2,-1.15176583927402));
#264220=CARTESIAN_POINT('Ctrl Pts',(-11.2877764550117,15.2,-1.15023986500291));
#264221=CARTESIAN_POINT('Ctrl Pts',(-11.2923527583261,15.2,-1.14870291865603));
#264222=CARTESIAN_POINT('Ctrl Pts',(-11.2969382902836,15.2,-1.14715496772814));
#264223=CARTESIAN_POINT('Ctrl Pts',(-11.3026702056991,15.2,-1.1452200289101));
#264224=CARTESIAN_POINT('Ctrl Pts',(-11.3084165421699,15.2,-1.14326789436179));
#264225=CARTESIAN_POINT('Ctrl Pts',(-11.3141771134882,15.2,-1.14129849651598));
#264226=CARTESIAN_POINT('Ctrl Pts',(-11.3176334567815,15.2,-1.14011685763677));
#264227=CARTESIAN_POINT('Ctrl Pts',(-11.3210949255012,15.2,-1.13892900546413));
#264228=CARTESIAN_POINT('Ctrl Pts',(-11.3245614792557,15.2,-1.13773492449808));
#264229=CARTESIAN_POINT('Ctrl Pts',(-11.3291835498788,15.2,-1.13614281690487));
#264230=CARTESIAN_POINT('Ctrl Pts',(-11.3338146609246,15.2,-1.13453963629871));
#264231=CARTESIAN_POINT('Ctrl Pts',(-11.3384547169552,15.2,-1.13292534953449));
#264232=CARTESIAN_POINT('Ctrl Pts',(-11.3419347591362,15.2,-1.13171463440633));
#264233=CARTESIAN_POINT('Ctrl Pts',(-11.3454198337803,15.2,-1.13049767263829));
#264234=CARTESIAN_POINT('Ctrl Pts',(-11.348909900403,15.2,-1.12927445084995));
#264235=CARTESIAN_POINT('Ctrl Pts',(-11.3523999670258,15.2,-1.12805122906162));
#264236=CARTESIAN_POINT('Ctrl Pts',(-11.3558950257149,15.2,-1.12682174560703));
#264237=CARTESIAN_POINT('Ctrl Pts',(-11.3593950397537,15.2,-1.12558598931945));
#264238=CARTESIAN_POINT('Ctrl Pts',(-11.3628950544283,15.2,-1.12435023280738));
#264239=CARTESIAN_POINT('Ctrl Pts',(-11.3664000220544,15.2,-1.1231082022102));
#264240=CARTESIAN_POINT('Ctrl Pts',(-11.3699099047735,15.2,-1.12185988473625));
#264241=CARTESIAN_POINT('Ctrl Pts',(-11.373419786855,15.2,-1.12061156748908));
#264242=CARTESIAN_POINT('Ctrl Pts',(-11.3769345828659,15.2,-1.11935696200728));
#264243=CARTESIAN_POINT('Ctrl Pts',(-11.3804542531644,15.2,-1.11809605573937));
#264244=CARTESIAN_POINT('Ctrl Pts',(-11.3839739234629,15.2,-1.11683514947147));
#264245=CARTESIAN_POINT('Ctrl Pts',(-11.3874984671626,15.2,-1.11556794208208));
#264246=CARTESIAN_POINT('Ctrl Pts',(-11.3910278474098,15.2,-1.11429442183614));
#264247=CARTESIAN_POINT('Ctrl Pts',(-11.3957336875257,15.2,-1.11259639491866));
#264248=CARTESIAN_POINT('Ctrl Pts',(-11.4004481282759,15.2,-1.11088714409233));
#264249=CARTESIAN_POINT('Ctrl Pts',(-11.4051710834445,15.2,-1.10916664128969));
#264250=CARTESIAN_POINT('Ctrl Pts',(-11.4110747778878,15.2,-1.10701601261058));
#264251=CARTESIAN_POINT('Ctrl Pts',(-11.4169917723552,15.2,-1.10484780395616));
#264252=CARTESIAN_POINT('Ctrl Pts',(-11.4229218548033,15.2,-1.10266194023708));
#264253=CARTESIAN_POINT('Ctrl Pts',(-11.4264799041429,15.2,-1.10135042205328));
#264254=CARTESIAN_POINT('Ctrl Pts',(-11.4300426634359,15.2,-1.10003254938976));
#264255=CARTESIAN_POINT('Ctrl Pts',(-11.4336101084723,15.2,-1.09870831335541));
#264256=CARTESIAN_POINT('Ctrl Pts',(-11.4383667022862,15.2,-1.09694266514923));
#264257=CARTESIAN_POINT('Ctrl Pts',(-11.4431316236994,15.2,-1.09516570948731));
#264258=CARTESIAN_POINT('Ctrl Pts',(-11.4479048650001,15.2,-1.09337742900002));
#264259=CARTESIAN_POINT('Ctrl Pts',(-10.3708900240001,15.2,-0.292001929000012));
#264260=CARTESIAN_POINT('Ctrl Pts',(-10.3708900240001,11.6,-0.292001929000012));
#264261=CARTESIAN_POINT('Ctrl Pts',(-10.3710632460001,15.2,-0.292021795000017));
#264262=CARTESIAN_POINT('Ctrl Pts',(-10.3710632460001,11.6,-0.292021795000017));
#264263=CARTESIAN_POINT('Ctrl Pts',(-10.3714157310001,15.2,-0.292062310000016));
#264264=CARTESIAN_POINT('Ctrl Pts',(-10.3714157310001,11.6,-0.292062310000017));
#264265=CARTESIAN_POINT('Ctrl Pts',(-10.3719498000001,15.2,-0.292123961000015));
#264266=CARTESIAN_POINT('Ctrl Pts',(-10.3719498000001,11.6,-0.292123961000015));
#264267=CARTESIAN_POINT('Ctrl Pts',(-10.3726691760001,15.2,-0.292207548000012));
#264268=CARTESIAN_POINT('Ctrl Pts',(-10.3726691760001,11.6,-0.292207548000012));
#264269=CARTESIAN_POINT('Ctrl Pts',(-10.3735789750001,15.2,-0.292314181000015));
#264270=CARTESIAN_POINT('Ctrl Pts',(-10.3735789750001,11.6,-0.292314181000016));
#264271=CARTESIAN_POINT('Ctrl Pts',(-10.3745034120001,15.2,-0.292423469000016));
#264272=CARTESIAN_POINT('Ctrl Pts',(-10.3745034120001,11.6,-0.292423469000016));
#264273=CARTESIAN_POINT('Ctrl Pts',(-10.3754371840001,15.2,-0.292534812000014));
#264274=CARTESIAN_POINT('Ctrl Pts',(-10.3754371840001,11.6,-0.292534812000014));
#264275=CARTESIAN_POINT('Ctrl Pts',(-10.3763802670001,15.2,-0.292648223000014));
#264276=CARTESIAN_POINT('Ctrl Pts',(-10.3763802670001,11.6,-0.292648223000014));
#264277=CARTESIAN_POINT('Ctrl Pts',(-10.3773326270001,15.2,-0.292763718000018));
#264278=CARTESIAN_POINT('Ctrl Pts',(-10.3773326270001,11.6,-0.292763718000018));
#264279=CARTESIAN_POINT('Ctrl Pts',(-10.3782942400001,15.2,-0.292881310000013));
#264280=CARTESIAN_POINT('Ctrl Pts',(-10.3782942400001,11.6,-0.292881310000013));
#264281=CARTESIAN_POINT('Ctrl Pts',(-10.3792650740001,15.2,-0.293001015000014));
#264282=CARTESIAN_POINT('Ctrl Pts',(-10.3792650740001,11.6,-0.293001015000014));
#264283=CARTESIAN_POINT('Ctrl Pts',(-10.3802451030001,15.2,-0.293122847000014));
#264284=CARTESIAN_POINT('Ctrl Pts',(-10.3802451030001,11.6,-0.293122847000014));
#264285=CARTESIAN_POINT('Ctrl Pts',(-10.3812342970001,15.2,-0.293246820000017));
#264286=CARTESIAN_POINT('Ctrl Pts',(-10.3812342970001,11.6,-0.293246820000018));
#264287=CARTESIAN_POINT('Ctrl Pts',(-10.3822326280001,15.2,-0.293372950000013));
#264288=CARTESIAN_POINT('Ctrl Pts',(-10.3822326280001,11.6,-0.293372950000013));
#264289=CARTESIAN_POINT('Ctrl Pts',(-10.3832400690001,15.2,-0.293501248000014));
#264290=CARTESIAN_POINT('Ctrl Pts',(-10.3832400690001,11.6,-0.293501248000015));
#264291=CARTESIAN_POINT('Ctrl Pts',(-10.3842565920001,15.2,-0.293631732000015));
#264292=CARTESIAN_POINT('Ctrl Pts',(-10.3842565920001,11.6,-0.293631732000015));
#264293=CARTESIAN_POINT('Ctrl Pts',(-10.3852821680001,15.2,-0.293764413000015));
#264294=CARTESIAN_POINT('Ctrl Pts',(-10.3852821680001,11.6,-0.293764413000015));
#264295=CARTESIAN_POINT('Ctrl Pts',(-10.3863167710001,15.2,-0.293899307000016));
#264296=CARTESIAN_POINT('Ctrl Pts',(-10.3863167710001,11.6,-0.293899307000017));
#264297=CARTESIAN_POINT('Ctrl Pts',(-10.3873603720001,15.2,-0.294036427000015));
#264298=CARTESIAN_POINT('Ctrl Pts',(-10.3873603720001,11.6,-0.294036427000016));
#264299=CARTESIAN_POINT('Ctrl Pts',(-10.3884129450001,15.2,-0.294175788000013));
#264300=CARTESIAN_POINT('Ctrl Pts',(-10.3884129450001,11.6,-0.294175788000013));
#264301=CARTESIAN_POINT('Ctrl Pts',(-10.3894744620001,15.2,-0.294317401000015));
#264302=CARTESIAN_POINT('Ctrl Pts',(-10.3894744620001,11.6,-0.294317401000015));
#264303=CARTESIAN_POINT('Ctrl Pts',(-10.3905448950001,15.2,-0.294461282000014));
#264304=CARTESIAN_POINT('Ctrl Pts',(-10.3905448950001,11.6,-0.294461282000014));
#264305=CARTESIAN_POINT('Ctrl Pts',(-10.3916242180001,15.2,-0.294607444000015));
#264306=CARTESIAN_POINT('Ctrl Pts',(-10.3916242180001,11.6,-0.294607444000015));
#264307=CARTESIAN_POINT('Ctrl Pts',(-10.3927124050001,15.2,-0.294755901000014));
#264308=CARTESIAN_POINT('Ctrl Pts',(-10.3927124050001,11.6,-0.294755901000015));
#264309=CARTESIAN_POINT('Ctrl Pts',(-10.3938094280001,15.2,-0.294906666000014));
#264310=CARTESIAN_POINT('Ctrl Pts',(-10.3938094280001,11.6,-0.294906666000015));
#264311=CARTESIAN_POINT('Ctrl Pts',(-10.3949152600001,15.2,-0.295059752000015));
#264312=CARTESIAN_POINT('Ctrl Pts',(-10.3949152600001,11.6,-0.295059752000016));
#264313=CARTESIAN_POINT('Ctrl Pts',(-10.3960298750001,15.2,-0.295215173000014));
#264314=CARTESIAN_POINT('Ctrl Pts',(-10.3960298750001,11.6,-0.295215173000015));
#264315=CARTESIAN_POINT('Ctrl Pts',(-10.3971532480001,15.2,-0.295372943000016));
#264316=CARTESIAN_POINT('Ctrl Pts',(-10.3971532480001,11.6,-0.295372943000017));
#264317=CARTESIAN_POINT('Ctrl Pts',(-10.3982853500001,15.2,-0.295533072000014));
#264318=CARTESIAN_POINT('Ctrl Pts',(-10.3982853500001,11.6,-0.295533072000014));
#264319=CARTESIAN_POINT('Ctrl Pts',(-10.3994261560001,15.2,-0.295695576000017));
#264320=CARTESIAN_POINT('Ctrl Pts',(-10.3994261560001,11.6,-0.295695576000017));
#264321=CARTESIAN_POINT('Ctrl Pts',(-10.4005756420001,15.2,-0.295860468000013));
#264322=CARTESIAN_POINT('Ctrl Pts',(-10.4005756420001,11.6,-0.295860468000014));
#264323=CARTESIAN_POINT('Ctrl Pts',(-10.4017337790001,15.2,-0.296027759000013));
#264324=CARTESIAN_POINT('Ctrl Pts',(-10.4017337790001,11.6,-0.296027759000013));
#264325=CARTESIAN_POINT('Ctrl Pts',(-10.4029005420001,15.2,-0.296197463000016));
#264326=CARTESIAN_POINT('Ctrl Pts',(-10.4029005420001,11.6,-0.296197463000017));
#264327=CARTESIAN_POINT('Ctrl Pts',(-10.4040759070001,15.2,-0.296369593000012));
#264328=CARTESIAN_POINT('Ctrl Pts',(-10.4040759070001,11.6,-0.296369593000013));
#264329=CARTESIAN_POINT('Ctrl Pts',(-10.4052598460001,15.2,-0.296544162000014));
#264330=CARTESIAN_POINT('Ctrl Pts',(-10.4052598460001,11.6,-0.296544162000015));
#264331=CARTESIAN_POINT('Ctrl Pts',(-10.4064523340001,15.2,-0.296721181000015));
#264332=CARTESIAN_POINT('Ctrl Pts',(-10.4064523340001,11.6,-0.296721181000015));
#264333=CARTESIAN_POINT('Ctrl Pts',(-10.4076533470001,15.2,-0.296900665000015));
#264334=CARTESIAN_POINT('Ctrl Pts',(-10.4076533470001,11.6,-0.296900665000015));
#264335=CARTESIAN_POINT('Ctrl Pts',(-10.4088628590001,15.2,-0.297082624000016));
#264336=CARTESIAN_POINT('Ctrl Pts',(-10.4088628590001,11.6,-0.297082624000016));
#264337=CARTESIAN_POINT('Ctrl Pts',(-10.4100808450001,15.2,-0.297267072000014));
#264338=CARTESIAN_POINT('Ctrl Pts',(-10.4100808450001,11.6,-0.297267072000014));
#264339=CARTESIAN_POINT('Ctrl Pts',(-10.4113072790001,15.2,-0.297454022000014));
#264340=CARTESIAN_POINT('Ctrl Pts',(-10.4113072790001,11.6,-0.297454022000015));
#264341=CARTESIAN_POINT('Ctrl Pts',(-10.4125421370001,15.2,-0.297643484000014));
#264342=CARTESIAN_POINT('Ctrl Pts',(-10.4125421370001,11.6,-0.297643484000015));
#264343=CARTESIAN_POINT('Ctrl Pts',(-10.4137853940001,15.2,-0.297835472000014));
#264344=CARTESIAN_POINT('Ctrl Pts',(-10.4137853940001,11.6,-0.297835472000015));
#264345=CARTESIAN_POINT('Ctrl Pts',(-10.4150370250001,15.2,-0.298029998000011));
#264346=CARTESIAN_POINT('Ctrl Pts',(-10.4150370250001,11.6,-0.298029998000012));
#264347=CARTESIAN_POINT('Ctrl Pts',(-10.4162970050001,15.2,-0.298227073000015));
#264348=CARTESIAN_POINT('Ctrl Pts',(-10.4162970050001,11.6,-0.298227073000015));
#264349=CARTESIAN_POINT('Ctrl Pts',(-10.4175653100001,15.2,-0.298426711000013));
#264350=CARTESIAN_POINT('Ctrl Pts',(-10.4175653100001,11.6,-0.298426711000013));
#264351=CARTESIAN_POINT('Ctrl Pts',(-10.4188419160001,15.2,-0.298628922000015));
#264352=CARTESIAN_POINT('Ctrl Pts',(-10.4188419160001,11.6,-0.298628922000015));
#264353=CARTESIAN_POINT('Ctrl Pts',(-10.4201267970001,15.2,-0.298833719000013));
#264354=CARTESIAN_POINT('Ctrl Pts',(-10.4201267970001,11.6,-0.298833719000014));
#264355=CARTESIAN_POINT('Ctrl Pts',(-10.4214199300001,15.2,-0.299041114000014));
#264356=CARTESIAN_POINT('Ctrl Pts',(-10.4214199300001,11.6,-0.299041114000014));
#264357=CARTESIAN_POINT('Ctrl Pts',(-10.4227212920001,15.2,-0.299251118000012));
#264358=CARTESIAN_POINT('Ctrl Pts',(-10.4227212920001,11.6,-0.299251118000013));
#264359=CARTESIAN_POINT('Ctrl Pts',(-10.4240308570001,15.2,-0.299463743000015));
#264360=CARTESIAN_POINT('Ctrl Pts',(-10.4240308570001,11.6,-0.299463743000015));
#264361=CARTESIAN_POINT('Ctrl Pts',(-10.4253486020001,15.2,-0.299679001000013));
#264362=CARTESIAN_POINT('Ctrl Pts',(-10.4253486020001,11.6,-0.299679001000013));
#264363=CARTESIAN_POINT('Ctrl Pts',(-10.4266745030001,15.2,-0.299896903000012));
#264364=CARTESIAN_POINT('Ctrl Pts',(-10.4266745030001,11.6,-0.299896903000012));
#264365=CARTESIAN_POINT('Ctrl Pts',(-10.4280085350001,15.2,-0.300117461000013));
#264366=CARTESIAN_POINT('Ctrl Pts',(-10.4280085350001,11.6,-0.300117461000014));
#264367=CARTESIAN_POINT('Ctrl Pts',(-10.4293506770001,15.2,-0.300340686000014));
#264368=CARTESIAN_POINT('Ctrl Pts',(-10.4293506770001,11.6,-0.300340686000014));
#264369=CARTESIAN_POINT('Ctrl Pts',(-10.4307009030001,15.2,-0.300566590000013));
#264370=CARTESIAN_POINT('Ctrl Pts',(-10.4307009030001,11.6,-0.300566590000014));
#264371=CARTESIAN_POINT('Ctrl Pts',(-10.4320591910001,15.2,-0.300795184000013));
#264372=CARTESIAN_POINT('Ctrl Pts',(-10.4320591910001,11.6,-0.300795184000014));
#264373=CARTESIAN_POINT('Ctrl Pts',(-10.4334255170001,15.2,-0.301026479000015));
#264374=CARTESIAN_POINT('Ctrl Pts',(-10.4334255170001,11.6,-0.301026479000015));
#264375=CARTESIAN_POINT('Ctrl Pts',(-10.4347998580001,15.2,-0.301260488000015));
#264376=CARTESIAN_POINT('Ctrl Pts',(-10.4347998580001,11.6,-0.301260488000015));
#264377=CARTESIAN_POINT('Ctrl Pts',(-10.4361821910001,15.2,-0.301497219000013));
#264378=CARTESIAN_POINT('Ctrl Pts',(-10.4361821910001,11.6,-0.301497219000014));
#264379=CARTESIAN_POINT('Ctrl Pts',(-10.4375724920001,15.2,-0.301736686000016));
#264380=CARTESIAN_POINT('Ctrl Pts',(-10.4375724920001,11.6,-0.301736686000016));
#264381=CARTESIAN_POINT('Ctrl Pts',(-10.4389707380001,15.2,-0.301978898000015));
#264382=CARTESIAN_POINT('Ctrl Pts',(-10.4389707380001,11.6,-0.301978898000015));
#264383=CARTESIAN_POINT('Ctrl Pts',(-10.4403769080001,15.2,-0.302223867000015));
#264384=CARTESIAN_POINT('Ctrl Pts',(-10.4403769080001,11.6,-0.302223867000016));
#264385=CARTESIAN_POINT('Ctrl Pts',(-10.4417909780001,15.2,-0.302471605000014));
#264386=CARTESIAN_POINT('Ctrl Pts',(-10.4417909780001,11.6,-0.302471605000015));
#264387=CARTESIAN_POINT('Ctrl Pts',(-10.4432129240001,15.2,-0.302722121000016));
#264388=CARTESIAN_POINT('Ctrl Pts',(-10.4432129240001,11.6,-0.302722121000017));
#264389=CARTESIAN_POINT('Ctrl Pts',(-10.4446427250001,15.2,-0.302975426000014));
#264390=CARTESIAN_POINT('Ctrl Pts',(-10.4446427250001,11.6,-0.302975426000014));
#264391=CARTESIAN_POINT('Ctrl Pts',(-10.4460803580001,15.2,-0.303231532000012));
#264392=CARTESIAN_POINT('Ctrl Pts',(-10.4460803580001,11.6,-0.303231532000013));
#264393=CARTESIAN_POINT('Ctrl Pts',(-10.4475258000001,15.2,-0.303490448000012));
#264394=CARTESIAN_POINT('Ctrl Pts',(-10.4475258000001,11.6,-0.303490448000013));
#264395=CARTESIAN_POINT('Ctrl Pts',(-10.4489790300001,15.2,-0.303752186000015));
#264396=CARTESIAN_POINT('Ctrl Pts',(-10.4489790300001,11.6,-0.303752186000015));
#264397=CARTESIAN_POINT('Ctrl Pts',(-10.4504400240001,15.2,-0.304016756000016));
#264398=CARTESIAN_POINT('Ctrl Pts',(-10.4504400240001,11.6,-0.304016756000017));
#264399=CARTESIAN_POINT('Ctrl Pts',(-10.4519087610001,15.2,-0.304284170000013));
#264400=CARTESIAN_POINT('Ctrl Pts',(-10.4519087610001,11.6,-0.304284170000014));
#264401=CARTESIAN_POINT('Ctrl Pts',(-10.4533852190001,15.2,-0.304554436000015));
#264402=CARTESIAN_POINT('Ctrl Pts',(-10.4533852190001,11.6,-0.304554436000016));
#264403=CARTESIAN_POINT('Ctrl Pts',(-10.4548693740001,15.2,-0.304827566000014));
#264404=CARTESIAN_POINT('Ctrl Pts',(-10.4548693740001,11.6,-0.304827566000015));
#264405=CARTESIAN_POINT('Ctrl Pts',(-10.4563612070001,15.2,-0.305103570000016));
#264406=CARTESIAN_POINT('Ctrl Pts',(-10.4563612070001,11.6,-0.305103570000016));
#264407=CARTESIAN_POINT('Ctrl Pts',(-10.4578606950001,15.2,-0.305382458000012));
#264408=CARTESIAN_POINT('Ctrl Pts',(-10.4578606950001,11.6,-0.305382458000012));
#264409=CARTESIAN_POINT('Ctrl Pts',(-10.4593678150001,15.2,-0.305664241000017));
#264410=CARTESIAN_POINT('Ctrl Pts',(-10.4593678150001,11.6,-0.305664241000017));
#264411=CARTESIAN_POINT('Ctrl Pts',(-10.4608825450001,15.2,-0.305948928000017));
#264412=CARTESIAN_POINT('Ctrl Pts',(-10.4608825450001,11.6,-0.305948928000018));
#264413=CARTESIAN_POINT('Ctrl Pts',(-10.4624048670001,15.2,-0.306236531000015));
#264414=CARTESIAN_POINT('Ctrl Pts',(-10.4624048670001,11.6,-0.306236531000015));
#264415=CARTESIAN_POINT('Ctrl Pts',(-10.4639347550001,15.2,-0.306527058000015));
#264416=CARTESIAN_POINT('Ctrl Pts',(-10.4639347550001,11.6,-0.306527058000015));
#264417=CARTESIAN_POINT('Ctrl Pts',(-10.4654721910001,15.2,-0.306820521000013));
#264418=CARTESIAN_POINT('Ctrl Pts',(-10.4654721910001,11.6,-0.306820521000013));
#264419=CARTESIAN_POINT('Ctrl Pts',(-10.4670171510001,15.2,-0.307116929000015));
#264420=CARTESIAN_POINT('Ctrl Pts',(-10.4670171510001,11.6,-0.307116929000016));
#264421=CARTESIAN_POINT('Ctrl Pts',(-10.4685696160001,15.2,-0.307416292000013));
#264422=CARTESIAN_POINT('Ctrl Pts',(-10.4685696160001,11.6,-0.307416292000014));
#264423=CARTESIAN_POINT('Ctrl Pts',(-10.4701295620001,15.2,-0.307718619000017));
#264424=CARTESIAN_POINT('Ctrl Pts',(-10.4701295620001,11.6,-0.307718619000017));
#264425=CARTESIAN_POINT('Ctrl Pts',(-10.4716969700001,15.2,-0.308023923000014));
#264426=CARTESIAN_POINT('Ctrl Pts',(-10.4716969700001,11.6,-0.308023923000014));
#264427=CARTESIAN_POINT('Ctrl Pts',(-10.4732718190001,15.2,-0.308332210000017));
#264428=CARTESIAN_POINT('Ctrl Pts',(-10.4732718190001,11.6,-0.308332210000018));
#264429=CARTESIAN_POINT('Ctrl Pts',(-10.4748540860001,15.2,-0.308643492000016));
#264430=CARTESIAN_POINT('Ctrl Pts',(-10.4748540860001,11.6,-0.308643492000016));
#264431=CARTESIAN_POINT('Ctrl Pts',(-10.4764437530001,15.2,-0.308957777000014));
#264432=CARTESIAN_POINT('Ctrl Pts',(-10.4764437530001,11.6,-0.308957777000014));
#264433=CARTESIAN_POINT('Ctrl Pts',(-10.4780407970001,15.2,-0.309275076000013));
#264434=CARTESIAN_POINT('Ctrl Pts',(-10.4780407970001,11.6,-0.309275076000013));
#264435=CARTESIAN_POINT('Ctrl Pts',(-10.4796451980001,15.2,-0.309595399000013));
#264436=CARTESIAN_POINT('Ctrl Pts',(-10.4796451980001,11.6,-0.309595399000014));
#264437=CARTESIAN_POINT('Ctrl Pts',(-10.4812569350001,15.2,-0.309918754000016));
#264438=CARTESIAN_POINT('Ctrl Pts',(-10.4812569350001,11.6,-0.309918754000016));
#264439=CARTESIAN_POINT('Ctrl Pts',(-10.4828759870001,15.2,-0.310245152000017));
#264440=CARTESIAN_POINT('Ctrl Pts',(-10.4828759870001,11.6,-0.310245152000018));
#264441=CARTESIAN_POINT('Ctrl Pts',(-10.4845023350001,15.2,-0.310574602000013));
#264442=CARTESIAN_POINT('Ctrl Pts',(-10.4845023350001,11.6,-0.310574602000014));
#264443=CARTESIAN_POINT('Ctrl Pts',(-10.4861359570001,15.2,-0.310907114000014));
#264444=CARTESIAN_POINT('Ctrl Pts',(-10.4861359570001,11.6,-0.310907114000015));
#264445=CARTESIAN_POINT('Ctrl Pts',(-10.4877768330001,15.2,-0.311242696000011));
#264446=CARTESIAN_POINT('Ctrl Pts',(-10.4877768330001,11.6,-0.311242696000012));
#264447=CARTESIAN_POINT('Ctrl Pts',(-10.4894249420001,15.2,-0.311581357000015));
#264448=CARTESIAN_POINT('Ctrl Pts',(-10.4894249420001,11.6,-0.311581357000015));
#264449=CARTESIAN_POINT('Ctrl Pts',(-10.4910802660001,15.2,-0.311923107000016));
#264450=CARTESIAN_POINT('Ctrl Pts',(-10.4910802660001,11.6,-0.311923107000017));
#264451=CARTESIAN_POINT('Ctrl Pts',(-10.4927427830001,15.2,-0.312267956000016));
#264452=CARTESIAN_POINT('Ctrl Pts',(-10.4927427830001,11.6,-0.312267956000017));
#264453=CARTESIAN_POINT('Ctrl Pts',(-10.4944124730001,15.2,-0.312615913000016));
#264454=CARTESIAN_POINT('Ctrl Pts',(-10.4944124730001,11.6,-0.312615913000017));
#264455=CARTESIAN_POINT('Ctrl Pts',(-10.4960893160001,15.2,-0.312966987000016));
#264456=CARTESIAN_POINT('Ctrl Pts',(-10.4960893160001,11.6,-0.312966987000017));
#264457=CARTESIAN_POINT('Ctrl Pts',(-10.4977732930001,15.2,-0.313321185000017));
#264458=CARTESIAN_POINT('Ctrl Pts',(-10.4977732930001,11.6,-0.313321185000018));
#264459=CARTESIAN_POINT('Ctrl Pts',(-10.4994643820001,15.2,-0.313678519000016));
#264460=CARTESIAN_POINT('Ctrl Pts',(-10.4994643820001,11.6,-0.313678519000016));
#264461=CARTESIAN_POINT('Ctrl Pts',(-10.5011625650001,15.2,-0.314038997000012));
#264462=CARTESIAN_POINT('Ctrl Pts',(-10.5011625650001,11.6,-0.314038997000013));
#264463=CARTESIAN_POINT('Ctrl Pts',(-10.5028678220001,15.2,-0.314402627000017));
#264464=CARTESIAN_POINT('Ctrl Pts',(-10.5028678220001,11.6,-0.314402627000017));
#264465=CARTESIAN_POINT('Ctrl Pts',(-10.5045801340001,15.2,-0.314769419000012));
#264466=CARTESIAN_POINT('Ctrl Pts',(-10.5045801340001,11.6,-0.314769419000012));
#264467=CARTESIAN_POINT('Ctrl Pts',(-10.5062994780001,15.2,-0.315139382000016));
#264468=CARTESIAN_POINT('Ctrl Pts',(-10.5062994780001,11.6,-0.315139382000016));
#264469=CARTESIAN_POINT('Ctrl Pts',(-10.5080258380001,15.2,-0.315512524000017));
#264470=CARTESIAN_POINT('Ctrl Pts',(-10.5080258380001,11.6,-0.315512524000017));
#264471=CARTESIAN_POINT('Ctrl Pts',(-10.5097591940001,15.2,-0.315888854000015));
#264472=CARTESIAN_POINT('Ctrl Pts',(-10.5097591940001,11.6,-0.315888854000015));
#264473=CARTESIAN_POINT('Ctrl Pts',(-10.5114995250001,15.2,-0.316268381000011));
#264474=CARTESIAN_POINT('Ctrl Pts',(-10.5114995250001,11.6,-0.316268381000012));
#264475=CARTESIAN_POINT('Ctrl Pts',(-10.5132468120001,15.2,-0.316651113000015));
#264476=CARTESIAN_POINT('Ctrl Pts',(-10.5132468120001,11.6,-0.316651113000015));
#264477=CARTESIAN_POINT('Ctrl Pts',(-10.5150010370001,15.2,-0.317037060000014));
#264478=CARTESIAN_POINT('Ctrl Pts',(-10.5150010370001,11.6,-0.317037060000014));
#264479=CARTESIAN_POINT('Ctrl Pts',(-10.5167621800001,15.2,-0.317426229000013));
#264480=CARTESIAN_POINT('Ctrl Pts',(-10.5167621800001,11.6,-0.317426229000013));
#264481=CARTESIAN_POINT('Ctrl Pts',(-10.5185302210001,15.2,-0.317818628000013));
#264482=CARTESIAN_POINT('Ctrl Pts',(-10.5185302210001,11.6,-0.317818628000013));
#264483=CARTESIAN_POINT('Ctrl Pts',(-10.5203051430001,15.2,-0.318214269000014));
#264484=CARTESIAN_POINT('Ctrl Pts',(-10.5203051430001,11.6,-0.318214269000015));
#264485=CARTESIAN_POINT('Ctrl Pts',(-10.5220869250001,15.2,-0.318613157000014));
#264486=CARTESIAN_POINT('Ctrl Pts',(-10.5220869250001,11.6,-0.318613157000014));
#264487=CARTESIAN_POINT('Ctrl Pts',(-10.5238755480001,15.2,-0.319015302000012));
#264488=CARTESIAN_POINT('Ctrl Pts',(-10.5238755480001,11.6,-0.319015302000012));
#264489=CARTESIAN_POINT('Ctrl Pts',(-10.5256709940001,15.2,-0.319420713000014));
#264490=CARTESIAN_POINT('Ctrl Pts',(-10.5256709940001,11.6,-0.319420713000014));
#264491=CARTESIAN_POINT('Ctrl Pts',(-10.5274732440001,15.2,-0.319829396000015));
#264492=CARTESIAN_POINT('Ctrl Pts',(-10.5274732440001,11.6,-0.319829396000016));
#264493=CARTESIAN_POINT('Ctrl Pts',(-10.5292822790001,15.2,-0.320241361000013));
#264494=CARTESIAN_POINT('Ctrl Pts',(-10.5292822790001,11.6,-0.320241361000014));
#264495=CARTESIAN_POINT('Ctrl Pts',(-10.5310980810001,15.2,-0.320656616000012));
#264496=CARTESIAN_POINT('Ctrl Pts',(-10.5310980810001,11.6,-0.320656616000013));
#264497=CARTESIAN_POINT('Ctrl Pts',(-10.5329206290001,15.2,-0.321075169000018));
#264498=CARTESIAN_POINT('Ctrl Pts',(-10.5329206290001,11.6,-0.321075169000018));
#264499=CARTESIAN_POINT('Ctrl Pts',(-10.5347499080001,15.2,-0.321497029000017));
#264500=CARTESIAN_POINT('Ctrl Pts',(-10.5347499080001,11.6,-0.321497029000018));
#264501=CARTESIAN_POINT('Ctrl Pts',(-10.5365858960001,15.2,-0.321922203000016));
#264502=CARTESIAN_POINT('Ctrl Pts',(-10.5365858960001,11.6,-0.321922203000016));
#264503=CARTESIAN_POINT('Ctrl Pts',(-10.5384285770001,15.2,-0.322350700000014));
#264504=CARTESIAN_POINT('Ctrl Pts',(-10.5384285770001,11.6,-0.322350700000014));
#264505=CARTESIAN_POINT('Ctrl Pts',(-10.5402779310001,15.2,-0.322782527000012));
#264506=CARTESIAN_POINT('Ctrl Pts',(-10.5402779310001,11.6,-0.322782527000012));
#264507=CARTESIAN_POINT('Ctrl Pts',(-10.5421339400001,15.2,-0.323217694000015));
#264508=CARTESIAN_POINT('Ctrl Pts',(-10.5421339400001,11.6,-0.323217694000016));
#264509=CARTESIAN_POINT('Ctrl Pts',(-10.5439965860001,15.2,-0.323656207000016));
#264510=CARTESIAN_POINT('Ctrl Pts',(-10.5439965860001,11.6,-0.323656207000016));
#264511=CARTESIAN_POINT('Ctrl Pts',(-10.5458658520001,15.2,-0.324098074000014));
#264512=CARTESIAN_POINT('Ctrl Pts',(-10.5458658520001,11.6,-0.324098074000015));
#264513=CARTESIAN_POINT('Ctrl Pts',(-10.5477417170001,15.2,-0.324543305000016));
#264514=CARTESIAN_POINT('Ctrl Pts',(-10.5477417170001,11.6,-0.324543305000016));
#264515=CARTESIAN_POINT('Ctrl Pts',(-10.5496241650001,15.2,-0.324991905000012));
#264516=CARTESIAN_POINT('Ctrl Pts',(-10.5496241650001,11.6,-0.324991905000012));
#264517=CARTESIAN_POINT('Ctrl Pts',(-10.5515131770001,15.2,-0.325443883000016));
#264518=CARTESIAN_POINT('Ctrl Pts',(-10.5515131770001,11.6,-0.325443883000017));
#264519=CARTESIAN_POINT('Ctrl Pts',(-10.5534087350001,15.2,-0.325899248000017));
#264520=CARTESIAN_POINT('Ctrl Pts',(-10.5534087350001,11.6,-0.325899248000017));
#264521=CARTESIAN_POINT('Ctrl Pts',(-10.5553108210001,15.2,-0.326358007000014));
#264522=CARTESIAN_POINT('Ctrl Pts',(-10.5553108210001,11.6,-0.326358007000014));
#264523=CARTESIAN_POINT('Ctrl Pts',(-10.5572194180001,15.2,-0.326820167000013));
#264524=CARTESIAN_POINT('Ctrl Pts',(-10.5572194180001,11.6,-0.326820167000013));
#264525=CARTESIAN_POINT('Ctrl Pts',(-10.5591345070001,15.2,-0.327285736000014));
#264526=CARTESIAN_POINT('Ctrl Pts',(-10.5591345070001,11.6,-0.327285736000014));
#264527=CARTESIAN_POINT('Ctrl Pts',(-10.5610560710001,15.2,-0.327754722000013));
#264528=CARTESIAN_POINT('Ctrl Pts',(-10.5610560710001,11.6,-0.327754722000014));
#264529=CARTESIAN_POINT('Ctrl Pts',(-10.5629840910001,15.2,-0.328227133000016));
#264530=CARTESIAN_POINT('Ctrl Pts',(-10.5629840910001,11.6,-0.328227133000017));
#264531=CARTESIAN_POINT('Ctrl Pts',(-10.5649185510001,15.2,-0.328702975000015));
#264532=CARTESIAN_POINT('Ctrl Pts',(-10.5649185510001,11.6,-0.328702975000015));
#264533=CARTESIAN_POINT('Ctrl Pts',(-10.5668594320001,15.2,-0.329182256000013));
#264534=CARTESIAN_POINT('Ctrl Pts',(-10.5668594320001,11.6,-0.329182256000014));
#264535=CARTESIAN_POINT('Ctrl Pts',(-10.5688067180001,15.2,-0.329664985000013));
#264536=CARTESIAN_POINT('Ctrl Pts',(-10.5688067180001,11.6,-0.329664985000014));
#264537=CARTESIAN_POINT('Ctrl Pts',(-10.5707603900001,15.2,-0.330151169000015));
#264538=CARTESIAN_POINT('Ctrl Pts',(-10.5707603900001,11.6,-0.330151169000015));
#264539=CARTESIAN_POINT('Ctrl Pts',(-10.5727204310001,15.2,-0.330640814000014));
#264540=CARTESIAN_POINT('Ctrl Pts',(-10.5727204310001,11.6,-0.330640814000014));
#264541=CARTESIAN_POINT('Ctrl Pts',(-10.5746868240001,15.2,-0.331133928000016));
#264542=CARTESIAN_POINT('Ctrl Pts',(-10.5746868240001,11.6,-0.331133928000016));
#264543=CARTESIAN_POINT('Ctrl Pts',(-10.5766595510001,15.2,-0.331630519000012));
#264544=CARTESIAN_POINT('Ctrl Pts',(-10.5766595510001,11.6,-0.331630519000013));
#264545=CARTESIAN_POINT('Ctrl Pts',(-10.5786385950001,15.2,-0.332130595000013));
#264546=CARTESIAN_POINT('Ctrl Pts',(-10.5786385950001,11.6,-0.332130595000014));
#264547=CARTESIAN_POINT('Ctrl Pts',(-10.5806239380001,15.2,-0.332634161000014));
#264548=CARTESIAN_POINT('Ctrl Pts',(-10.5806239380001,11.6,-0.332634161000014));
#264549=CARTESIAN_POINT('Ctrl Pts',(-10.5826155640001,15.2,-0.333141226000016));
#264550=CARTESIAN_POINT('Ctrl Pts',(-10.5826155640001,11.6,-0.333141226000016));
#264551=CARTESIAN_POINT('Ctrl Pts',(-10.5846134550001,15.2,-0.333651796000014));
#264552=CARTESIAN_POINT('Ctrl Pts',(-10.5846134550001,11.6,-0.333651796000014));
#264553=CARTESIAN_POINT('Ctrl Pts',(-10.5866175950001,15.2,-0.334165879000015));
#264554=CARTESIAN_POINT('Ctrl Pts',(-10.5866175950001,11.6,-0.334165879000015));
#264555=CARTESIAN_POINT('Ctrl Pts',(-10.5886279650001,15.2,-0.334683483000013));
#264556=CARTESIAN_POINT('Ctrl Pts',(-10.5886279650001,11.6,-0.334683483000014));
#264557=CARTESIAN_POINT('Ctrl Pts',(-10.5906445490001,15.2,-0.335204613000015));
#264558=CARTESIAN_POINT('Ctrl Pts',(-10.5906445490001,11.6,-0.335204613000016));
#264559=CARTESIAN_POINT('Ctrl Pts',(-10.5926673320001,15.2,-0.335729278000017));
#264560=CARTESIAN_POINT('Ctrl Pts',(-10.5926673320001,11.6,-0.335729278000017));
#264561=CARTESIAN_POINT('Ctrl Pts',(-10.5946962940001,15.2,-0.336257483000013));
#264562=CARTESIAN_POINT('Ctrl Pts',(-10.5946962940001,11.6,-0.336257483000014));
#264563=CARTESIAN_POINT('Ctrl Pts',(-10.5967314190001,15.2,-0.336789237000015));
#264564=CARTESIAN_POINT('Ctrl Pts',(-10.5967314190001,11.6,-0.336789237000015));
#264565=CARTESIAN_POINT('Ctrl Pts',(-10.5987726910001,15.2,-0.337324546000013));
#264566=CARTESIAN_POINT('Ctrl Pts',(-10.5987726910001,11.6,-0.337324546000013));
#264567=CARTESIAN_POINT('Ctrl Pts',(-10.6008200940001,15.2,-0.337863418000013));
#264568=CARTESIAN_POINT('Ctrl Pts',(-10.6008200940001,11.6,-0.337863418000013));
#264569=CARTESIAN_POINT('Ctrl Pts',(-10.6028736090001,15.2,-0.338405859000015));
#264570=CARTESIAN_POINT('Ctrl Pts',(-10.6028736090001,11.6,-0.338405859000015));
#264571=CARTESIAN_POINT('Ctrl Pts',(-10.6049332210001,15.2,-0.338951874000015));
#264572=CARTESIAN_POINT('Ctrl Pts',(-10.6049332210001,11.6,-0.338951874000016));
#264573=CARTESIAN_POINT('Ctrl Pts',(-10.6069989120001,15.2,-0.339501473000015));
#264574=CARTESIAN_POINT('Ctrl Pts',(-10.6069989120001,11.6,-0.339501473000015));
#264575=CARTESIAN_POINT('Ctrl Pts',(-10.6090706680001,15.2,-0.340054662000018));
#264576=CARTESIAN_POINT('Ctrl Pts',(-10.6090706680001,11.6,-0.340054662000018));
#264577=CARTESIAN_POINT('Ctrl Pts',(-10.6111484700001,15.2,-0.340611447000012));
#264578=CARTESIAN_POINT('Ctrl Pts',(-10.6111484700001,11.6,-0.340611447000013));
#264579=CARTESIAN_POINT('Ctrl Pts',(-10.6132323020001,15.2,-0.341171835000011));
#264580=CARTESIAN_POINT('Ctrl Pts',(-10.6132323020001,11.6,-0.341171835000012));
#264581=CARTESIAN_POINT('Ctrl Pts',(-10.6153221490001,15.2,-0.341735833000012));
#264582=CARTESIAN_POINT('Ctrl Pts',(-10.6153221490001,11.6,-0.341735833000012));
#264583=CARTESIAN_POINT('Ctrl Pts',(-10.6174179920001,15.2,-0.342303448000014));
#264584=CARTESIAN_POINT('Ctrl Pts',(-10.6174179920001,11.6,-0.342303448000015));
#264585=CARTESIAN_POINT('Ctrl Pts',(-10.6195198180001,15.2,-0.342874685000014));
#264586=CARTESIAN_POINT('Ctrl Pts',(-10.6195198180001,11.6,-0.342874685000015));
#264587=CARTESIAN_POINT('Ctrl Pts',(-10.6216276080001,15.2,-0.343449552000017));
#264588=CARTESIAN_POINT('Ctrl Pts',(-10.6216276080001,11.6,-0.343449552000017));
#264589=CARTESIAN_POINT('Ctrl Pts',(-10.6237413470001,15.2,-0.344028056000014));
#264590=CARTESIAN_POINT('Ctrl Pts',(-10.6237413470001,11.6,-0.344028056000015));
#264591=CARTESIAN_POINT('Ctrl Pts',(-10.6258610180001,15.2,-0.344610202000015));
#264592=CARTESIAN_POINT('Ctrl Pts',(-10.6258610180001,11.6,-0.344610202000016));
#264593=CARTESIAN_POINT('Ctrl Pts',(-10.6279866070001,15.2,-0.345195998000012));
#264594=CARTESIAN_POINT('Ctrl Pts',(-10.6279866070001,11.6,-0.345195998000012));
#264595=CARTESIAN_POINT('Ctrl Pts',(-10.6301180950001,15.2,-0.345785450000013));
#264596=CARTESIAN_POINT('Ctrl Pts',(-10.6301180950001,11.6,-0.345785450000014));
#264597=CARTESIAN_POINT('Ctrl Pts',(-10.6322554680001,15.2,-0.346378564000016));
#264598=CARTESIAN_POINT('Ctrl Pts',(-10.6322554680001,11.6,-0.346378564000017));
#264599=CARTESIAN_POINT('Ctrl Pts',(-10.6343987090001,15.2,-0.346975347000011));
#264600=CARTESIAN_POINT('Ctrl Pts',(-10.6343987090001,11.6,-0.346975347000012));
#264601=CARTESIAN_POINT('Ctrl Pts',(-10.6365478020001,15.2,-0.347575805000013));
#264602=CARTESIAN_POINT('Ctrl Pts',(-10.6365478020001,11.6,-0.347575805000014));
#264603=CARTESIAN_POINT('Ctrl Pts',(-10.6387027320001,15.2,-0.348179945000013));
#264604=CARTESIAN_POINT('Ctrl Pts',(-10.6387027320001,11.6,-0.348179945000014));
#264605=CARTESIAN_POINT('Ctrl Pts',(-10.6408634830001,15.2,-0.348787773000012));
#264606=CARTESIAN_POINT('Ctrl Pts',(-10.6408634830001,11.6,-0.348787773000013));
#264607=CARTESIAN_POINT('Ctrl Pts',(-10.6430300390001,15.2,-0.349399295000015));
#264608=CARTESIAN_POINT('Ctrl Pts',(-10.6430300390001,11.6,-0.349399295000015));
#264609=CARTESIAN_POINT('Ctrl Pts',(-10.6452023830001,15.2,-0.350014516000012));
#264610=CARTESIAN_POINT('Ctrl Pts',(-10.6452023830001,11.6,-0.350014516000013));
#264611=CARTESIAN_POINT('Ctrl Pts',(-10.6473805010001,15.2,-0.350633446000015));
#264612=CARTESIAN_POINT('Ctrl Pts',(-10.6473805010001,11.6,-0.350633446000015));
#264613=CARTESIAN_POINT('Ctrl Pts',(-10.6495643770001,15.2,-0.351256088000014));
#264614=CARTESIAN_POINT('Ctrl Pts',(-10.6495643770001,11.6,-0.351256088000014));
#264615=CARTESIAN_POINT('Ctrl Pts',(-10.6517539940001,15.2,-0.351882449000014));
#264616=CARTESIAN_POINT('Ctrl Pts',(-10.6517539940001,11.6,-0.351882449000014));
#264617=CARTESIAN_POINT('Ctrl Pts',(-10.6539493380001,15.2,-0.352512536000016));
#264618=CARTESIAN_POINT('Ctrl Pts',(-10.6539493380001,11.6,-0.352512536000016));
#264619=CARTESIAN_POINT('Ctrl Pts',(-10.6561503920001,15.2,-0.353146354000016));
#264620=CARTESIAN_POINT('Ctrl Pts',(-10.6561503920001,11.6,-0.353146354000016));
#264621=CARTESIAN_POINT('Ctrl Pts',(-10.6583571410001,15.2,-0.353783910000014));
#264622=CARTESIAN_POINT('Ctrl Pts',(-10.6583571410001,11.6,-0.353783910000014));
#264623=CARTESIAN_POINT('Ctrl Pts',(-10.6605695710001,15.2,-0.354425210000016));
#264624=CARTESIAN_POINT('Ctrl Pts',(-10.6605695710001,11.6,-0.354425210000016));
#264625=CARTESIAN_POINT('Ctrl Pts',(-10.6627876650001,15.2,-0.355070259000012));
#264626=CARTESIAN_POINT('Ctrl Pts',(-10.6627876650001,11.6,-0.355070259000013));
#264627=CARTESIAN_POINT('Ctrl Pts',(-10.6650114070001,15.2,-0.355719063000013));
#264628=CARTESIAN_POINT('Ctrl Pts',(-10.6650114070001,11.6,-0.355719063000013));
#264629=CARTESIAN_POINT('Ctrl Pts',(-10.6672407830001,15.2,-0.356371629000014));
#264630=CARTESIAN_POINT('Ctrl Pts',(-10.6672407830001,11.6,-0.356371629000015));
#264631=CARTESIAN_POINT('Ctrl Pts',(-10.6694757780001,15.2,-0.357027964000016));
#264632=CARTESIAN_POINT('Ctrl Pts',(-10.6694757780001,11.6,-0.357027964000017));
#264633=CARTESIAN_POINT('Ctrl Pts',(-10.6717163760001,15.2,-0.357688071000015));
#264634=CARTESIAN_POINT('Ctrl Pts',(-10.6717163760001,11.6,-0.357688071000016));
#264635=CARTESIAN_POINT('Ctrl Pts',(-10.6739625620001,15.2,-0.358351959000016));
#264636=CARTESIAN_POINT('Ctrl Pts',(-10.6739625620001,11.6,-0.358351959000017));
#264637=CARTESIAN_POINT('Ctrl Pts',(-10.6762143200001,15.2,-0.359019631000015));
#264638=CARTESIAN_POINT('Ctrl Pts',(-10.6762143200001,11.6,-0.359019631000015));
#264639=CARTESIAN_POINT('Ctrl Pts',(-10.6784716350001,15.2,-0.359691096000017));
#264640=CARTESIAN_POINT('Ctrl Pts',(-10.6784716350001,11.6,-0.359691096000017));
#264641=CARTESIAN_POINT('Ctrl Pts',(-10.6807344940001,15.2,-0.360366356000017));
#264642=CARTESIAN_POINT('Ctrl Pts',(-10.6807344940001,11.6,-0.360366356000017));
#264643=CARTESIAN_POINT('Ctrl Pts',(-10.6830028780001,15.2,-0.361045420000017));
#264644=CARTESIAN_POINT('Ctrl Pts',(-10.6830028780001,11.6,-0.361045420000017));
#264645=CARTESIAN_POINT('Ctrl Pts',(-10.6852767760001,15.2,-0.361728293000017));
#264646=CARTESIAN_POINT('Ctrl Pts',(-10.6852767760001,11.6,-0.361728293000017));
#264647=CARTESIAN_POINT('Ctrl Pts',(-10.6875561710001,15.2,-0.362414981000012));
#264648=CARTESIAN_POINT('Ctrl Pts',(-10.6875561710001,11.6,-0.362414981000013));
#264649=CARTESIAN_POINT('Ctrl Pts',(-10.6898410480001,15.2,-0.363105487000013));
#264650=CARTESIAN_POINT('Ctrl Pts',(-10.6898410480001,11.6,-0.363105487000013));
#264651=CARTESIAN_POINT('Ctrl Pts',(-10.6921313930001,15.2,-0.363799821000015));
#264652=CARTESIAN_POINT('Ctrl Pts',(-10.6921313930001,11.6,-0.363799821000015));
#264653=CARTESIAN_POINT('Ctrl Pts',(-10.6944271900001,15.2,-0.364497985000014));
#264654=CARTESIAN_POINT('Ctrl Pts',(-10.6944271900001,11.6,-0.364497985000015));
#264655=CARTESIAN_POINT('Ctrl Pts',(-10.6967284250001,15.2,-0.365199987000011));
#264656=CARTESIAN_POINT('Ctrl Pts',(-10.6967284250001,11.6,-0.365199987000012));
#264657=CARTESIAN_POINT('Ctrl Pts',(-10.6990350820001,15.2,-0.365905831000015));
#264658=CARTESIAN_POINT('Ctrl Pts',(-10.6990350820001,11.6,-0.365905831000016));
#264659=CARTESIAN_POINT('Ctrl Pts',(-10.7013471480001,15.2,-0.366615523000018));
#264660=CARTESIAN_POINT('Ctrl Pts',(-10.7013471480001,11.6,-0.366615523000018));
#264661=CARTESIAN_POINT('Ctrl Pts',(-10.7036646080001,15.2,-0.367329069000015));
#264662=CARTESIAN_POINT('Ctrl Pts',(-10.7036646080001,11.6,-0.367329069000016));
#264663=CARTESIAN_POINT('Ctrl Pts',(-10.7059874460001,15.2,-0.368046475000017));
#264664=CARTESIAN_POINT('Ctrl Pts',(-10.7059874460001,11.6,-0.368046475000017));
#264665=CARTESIAN_POINT('Ctrl Pts',(-10.7083156480001,15.2,-0.368767746000014));
#264666=CARTESIAN_POINT('Ctrl Pts',(-10.7083156480001,11.6,-0.368767746000014));
#264667=CARTESIAN_POINT('Ctrl Pts',(-10.7106492000001,15.2,-0.369492887000016));
#264668=CARTESIAN_POINT('Ctrl Pts',(-10.7106492000001,11.6,-0.369492887000016));
#264669=CARTESIAN_POINT('Ctrl Pts',(-10.7129880860001,15.2,-0.370221904000014));
#264670=CARTESIAN_POINT('Ctrl Pts',(-10.7129880860001,11.6,-0.370221904000015));
#264671=CARTESIAN_POINT('Ctrl Pts',(-10.7153322940001,15.2,-0.370954801000014));
#264672=CARTESIAN_POINT('Ctrl Pts',(-10.7153322940001,11.6,-0.370954801000015));
#264673=CARTESIAN_POINT('Ctrl Pts',(-10.7176818070001,15.2,-0.371691587000011));
#264674=CARTESIAN_POINT('Ctrl Pts',(-10.7176818070001,11.6,-0.371691587000012));
#264675=CARTESIAN_POINT('Ctrl Pts',(-10.7200366120001,15.2,-0.372432264000011));
#264676=CARTESIAN_POINT('Ctrl Pts',(-10.7200366120001,11.6,-0.372432264000012));
#264677=CARTESIAN_POINT('Ctrl Pts',(-10.7223966940001,15.2,-0.373176838000013));
#264678=CARTESIAN_POINT('Ctrl Pts',(-10.7223966940001,11.6,-0.373176838000014));
#264679=CARTESIAN_POINT('Ctrl Pts',(-10.7247620380001,15.2,-0.373925315000014));
#264680=CARTESIAN_POINT('Ctrl Pts',(-10.7247620380001,11.6,-0.373925315000015));
#264681=CARTESIAN_POINT('Ctrl Pts',(-10.7271326310001,15.2,-0.374677700000015));
#264682=CARTESIAN_POINT('Ctrl Pts',(-10.7271326310001,11.6,-0.374677700000015));
#264683=CARTESIAN_POINT('Ctrl Pts',(-10.7295084580001,15.2,-0.375433998000014));
#264684=CARTESIAN_POINT('Ctrl Pts',(-10.7295084580001,11.6,-0.375433998000015));
#264685=CARTESIAN_POINT('Ctrl Pts',(-10.7318895040001,15.2,-0.376194215000014));
#264686=CARTESIAN_POINT('Ctrl Pts',(-10.7318895040001,11.6,-0.376194215000015));
#264687=CARTESIAN_POINT('Ctrl Pts',(-10.7342757570001,15.2,-0.376958356000014));
#264688=CARTESIAN_POINT('Ctrl Pts',(-10.7342757570001,11.6,-0.376958356000015));
#264689=CARTESIAN_POINT('Ctrl Pts',(-10.7366672000001,15.2,-0.377726425000016));
#264690=CARTESIAN_POINT('Ctrl Pts',(-10.7366672000001,11.6,-0.377726425000016));
#264691=CARTESIAN_POINT('Ctrl Pts',(-10.7390638200001,15.2,-0.378498429000014));
#264692=CARTESIAN_POINT('Ctrl Pts',(-10.7390638200001,11.6,-0.378498429000014));
#264693=CARTESIAN_POINT('Ctrl Pts',(-10.7414656040001,15.2,-0.379274372000014));
#264694=CARTESIAN_POINT('Ctrl Pts',(-10.7414656040001,11.6,-0.379274372000014));
#264695=CARTESIAN_POINT('Ctrl Pts',(-10.7438725370001,15.2,-0.380054260000016));
#264696=CARTESIAN_POINT('Ctrl Pts',(-10.7438725370001,11.6,-0.380054260000016));
#264697=CARTESIAN_POINT('Ctrl Pts',(-10.7462846040001,15.2,-0.380838098000016));
#264698=CARTESIAN_POINT('Ctrl Pts',(-10.7462846040001,11.6,-0.380838098000016));
#264699=CARTESIAN_POINT('Ctrl Pts',(-10.7487017930001,15.2,-0.381625889000015));
#264700=CARTESIAN_POINT('Ctrl Pts',(-10.7487017930001,11.6,-0.381625889000015));
#264701=CARTESIAN_POINT('Ctrl Pts',(-10.7511240870001,15.2,-0.382417641000017));
#264702=CARTESIAN_POINT('Ctrl Pts',(-10.7511240870001,11.6,-0.382417641000017));
#264703=CARTESIAN_POINT('Ctrl Pts',(-10.7535514750001,15.2,-0.383213358000014));
#264704=CARTESIAN_POINT('Ctrl Pts',(-10.7535514750001,11.6,-0.383213358000015));
#264705=CARTESIAN_POINT('Ctrl Pts',(-10.7559839420001,15.2,-0.384013044000016));
#264706=CARTESIAN_POINT('Ctrl Pts',(-10.7559839420001,11.6,-0.384013044000016));
#264707=CARTESIAN_POINT('Ctrl Pts',(-10.7584214740001,15.2,-0.384816705000013));
#264708=CARTESIAN_POINT('Ctrl Pts',(-10.7584214740001,11.6,-0.384816705000013));
#264709=CARTESIAN_POINT('Ctrl Pts',(-10.7608640580001,15.2,-0.385624345000015));
#264710=CARTESIAN_POINT('Ctrl Pts',(-10.7608640580001,11.6,-0.385624345000016));
#264711=CARTESIAN_POINT('Ctrl Pts',(-10.7633116780001,15.2,-0.386435971000014));
#264712=CARTESIAN_POINT('Ctrl Pts',(-10.7633116780001,11.6,-0.386435971000015));
#264713=CARTESIAN_POINT('Ctrl Pts',(-10.7657643230001,15.2,-0.387251586000015));
#264714=CARTESIAN_POINT('Ctrl Pts',(-10.7657643230001,11.6,-0.387251586000015));
#264715=CARTESIAN_POINT('Ctrl Pts',(-10.7682219760001,15.2,-0.388071196000013));
#264716=CARTESIAN_POINT('Ctrl Pts',(-10.7682219760001,11.6,-0.388071196000013));
#264717=CARTESIAN_POINT('Ctrl Pts',(-10.7706846260001,15.2,-0.388894805000017));
#264718=CARTESIAN_POINT('Ctrl Pts',(-10.7706846260001,11.6,-0.388894805000018));
#264719=CARTESIAN_POINT('Ctrl Pts',(-10.7731522590001,15.2,-0.389722418000016));
#264720=CARTESIAN_POINT('Ctrl Pts',(-10.7731522590001,11.6,-0.389722418000016));
#264721=CARTESIAN_POINT('Ctrl Pts',(-10.7756248610001,15.2,-0.390554041000013));
#264722=CARTESIAN_POINT('Ctrl Pts',(-10.7756248610001,11.6,-0.390554041000013));
#264723=CARTESIAN_POINT('Ctrl Pts',(-10.7781024170001,15.2,-0.391389677000014));
#264724=CARTESIAN_POINT('Ctrl Pts',(-10.7781024170001,11.6,-0.391389677000014));
#264725=CARTESIAN_POINT('Ctrl Pts',(-10.7805849160001,15.2,-0.392229332000014));
#264726=CARTESIAN_POINT('Ctrl Pts',(-10.7805849160001,11.6,-0.392229332000014));
#264727=CARTESIAN_POINT('Ctrl Pts',(-10.7830723410001,15.2,-0.393073009000013));
#264728=CARTESIAN_POINT('Ctrl Pts',(-10.7830723410001,11.6,-0.393073009000014));
#264729=CARTESIAN_POINT('Ctrl Pts',(-10.7855646820001,15.2,-0.393920716000018));
#264730=CARTESIAN_POINT('Ctrl Pts',(-10.7855646820001,11.6,-0.393920716000018));
#264731=CARTESIAN_POINT('Ctrl Pts',(-10.7880619230001,15.2,-0.394772456000014));
#264732=CARTESIAN_POINT('Ctrl Pts',(-10.7880619230001,11.6,-0.394772456000015));
#264733=CARTESIAN_POINT('Ctrl Pts',(-10.7905640520001,15.2,-0.395628232000016));
#264734=CARTESIAN_POINT('Ctrl Pts',(-10.7905640520001,11.6,-0.395628232000016));
#264735=CARTESIAN_POINT('Ctrl Pts',(-10.7930710550001,15.2,-0.396488052000015));
#264736=CARTESIAN_POINT('Ctrl Pts',(-10.7930710550001,11.6,-0.396488052000015));
#264737=CARTESIAN_POINT('Ctrl Pts',(-10.7955829180001,15.2,-0.397351917000015));
#264738=CARTESIAN_POINT('Ctrl Pts',(-10.7955829180001,11.6,-0.397351917000015));
#264739=CARTESIAN_POINT('Ctrl Pts',(-10.7980996290001,15.2,-0.398219835000013));
#264740=CARTESIAN_POINT('Ctrl Pts',(-10.7980996290001,11.6,-0.398219835000014));
#264741=CARTESIAN_POINT('Ctrl Pts',(-10.8006211740001,15.2,-0.399091809000014));
#264742=CARTESIAN_POINT('Ctrl Pts',(-10.8006211740001,11.6,-0.399091809000014));
#264743=CARTESIAN_POINT('Ctrl Pts',(-10.8031475400001,15.2,-0.399967843000013));
#264744=CARTESIAN_POINT('Ctrl Pts',(-10.8031475400001,11.6,-0.399967843000014));
#264745=CARTESIAN_POINT('Ctrl Pts',(-10.8056787130001,15.2,-0.400847944000016));
#264746=CARTESIAN_POINT('Ctrl Pts',(-10.8056787130001,11.6,-0.400847944000016));
#264747=CARTESIAN_POINT('Ctrl Pts',(-10.8082146790001,15.2,-0.401732113000013));
#264748=CARTESIAN_POINT('Ctrl Pts',(-10.8082146790001,11.6,-0.401732113000013));
#264749=CARTESIAN_POINT('Ctrl Pts',(-10.8107554270001,15.2,-0.402620357000014));
#264750=CARTESIAN_POINT('Ctrl Pts',(-10.8107554270001,11.6,-0.402620357000015));
#264751=CARTESIAN_POINT('Ctrl Pts',(-10.8133009430001,15.2,-0.403512679000015));
#264752=CARTESIAN_POINT('Ctrl Pts',(-10.8133009430001,11.6,-0.403512679000016));
#264753=CARTESIAN_POINT('Ctrl Pts',(-10.8158512130001,15.2,-0.404409086000013));
#264754=CARTESIAN_POINT('Ctrl Pts',(-10.8158512130001,11.6,-0.404409086000013));
#264755=CARTESIAN_POINT('Ctrl Pts',(-10.8184062250001,15.2,-0.405309580000015));
#264756=CARTESIAN_POINT('Ctrl Pts',(-10.8184062250001,11.6,-0.405309580000015));
#264757=CARTESIAN_POINT('Ctrl Pts',(-10.8209659650001,15.2,-0.406214166000014));
#264758=CARTESIAN_POINT('Ctrl Pts',(-10.8209659650001,11.6,-0.406214166000014));
#264759=CARTESIAN_POINT('Ctrl Pts',(-10.8235304190001,15.2,-0.407122849000014));
#264760=CARTESIAN_POINT('Ctrl Pts',(-10.8235304190001,11.6,-0.407122849000015));
#264761=CARTESIAN_POINT('Ctrl Pts',(-10.8260995770001,15.2,-0.408035633000012));
#264762=CARTESIAN_POINT('Ctrl Pts',(-10.8260995770001,11.6,-0.408035633000013));
#264763=CARTESIAN_POINT('Ctrl Pts',(-10.8286734240001,15.2,-0.408952523000017));
#264764=CARTESIAN_POINT('Ctrl Pts',(-10.8286734240001,11.6,-0.408952523000017));
#264765=CARTESIAN_POINT('Ctrl Pts',(-10.8312519470001,15.2,-0.409873522000015));
#264766=CARTESIAN_POINT('Ctrl Pts',(-10.8312519470001,11.6,-0.409873522000015));
#264767=CARTESIAN_POINT('Ctrl Pts',(-10.8338351330001,15.2,-0.410798635000016));
#264768=CARTESIAN_POINT('Ctrl Pts',(-10.8338351330001,11.6,-0.410798635000016));
#264769=CARTESIAN_POINT('Ctrl Pts',(-10.8364229690001,15.2,-0.411727867000016));
#264770=CARTESIAN_POINT('Ctrl Pts',(-10.8364229690001,11.6,-0.411727867000016));
#264771=CARTESIAN_POINT('Ctrl Pts',(-10.8390154430001,15.2,-0.412661222000015));
#264772=CARTESIAN_POINT('Ctrl Pts',(-10.8390154430001,11.6,-0.412661222000015));
#264773=CARTESIAN_POINT('Ctrl Pts',(-10.8416125420001,15.2,-0.413598703000013));
#264774=CARTESIAN_POINT('Ctrl Pts',(-10.8416125420001,11.6,-0.413598703000014));
#264775=CARTESIAN_POINT('Ctrl Pts',(-10.8442142530001,15.2,-0.414540317000016));
#264776=CARTESIAN_POINT('Ctrl Pts',(-10.8442142530001,11.6,-0.414540317000017));
#264777=CARTESIAN_POINT('Ctrl Pts',(-10.8468205630001,15.2,-0.415486065000015));
#264778=CARTESIAN_POINT('Ctrl Pts',(-10.8468205630001,11.6,-0.415486065000015));
#264779=CARTESIAN_POINT('Ctrl Pts',(-10.8494314580001,15.2,-0.416435953000014));
#264780=CARTESIAN_POINT('Ctrl Pts',(-10.8494314580001,11.6,-0.416435953000014));
#264781=CARTESIAN_POINT('Ctrl Pts',(-10.8520469280001,15.2,-0.417389985000014));
#264782=CARTESIAN_POINT('Ctrl Pts',(-10.8520469280001,11.6,-0.417389985000014));
#264783=CARTESIAN_POINT('Ctrl Pts',(-10.8546669570001,15.2,-0.418348165000015));
#264784=CARTESIAN_POINT('Ctrl Pts',(-10.8546669570001,11.6,-0.418348165000016));
#264785=CARTESIAN_POINT('Ctrl Pts',(-10.8572915350001,15.2,-0.419310498000014));
#264786=CARTESIAN_POINT('Ctrl Pts',(-10.8572915350001,11.6,-0.419310498000014));
#264787=CARTESIAN_POINT('Ctrl Pts',(-10.8599206490001,15.2,-0.420276987000014));
#264788=CARTESIAN_POINT('Ctrl Pts',(-10.8599206490001,11.6,-0.420276987000015));
#264789=CARTESIAN_POINT('Ctrl Pts',(-10.8625542860001,15.2,-0.421247636000013));
#264790=CARTESIAN_POINT('Ctrl Pts',(-10.8625542860001,11.6,-0.421247636000013));
#264791=CARTESIAN_POINT('Ctrl Pts',(-10.8651924320001,15.2,-0.422222450000014));
#264792=CARTESIAN_POINT('Ctrl Pts',(-10.8651924320001,11.6,-0.422222450000014));
#264793=CARTESIAN_POINT('Ctrl Pts',(-10.8678350770001,15.2,-0.423201432000013));
#264794=CARTESIAN_POINT('Ctrl Pts',(-10.8678350770001,11.6,-0.423201432000014));
#264795=CARTESIAN_POINT('Ctrl Pts',(-10.8704822050001,15.2,-0.424184588000016));
#264796=CARTESIAN_POINT('Ctrl Pts',(-10.8704822050001,11.6,-0.424184588000017));
#264797=CARTESIAN_POINT('Ctrl Pts',(-10.8731338070001,15.2,-0.425171920000014));
#264798=CARTESIAN_POINT('Ctrl Pts',(-10.8731338070001,11.6,-0.425171920000014));
#264799=CARTESIAN_POINT('Ctrl Pts',(-10.8757898690001,15.2,-0.426163433000015));
#264800=CARTESIAN_POINT('Ctrl Pts',(-10.8757898690001,11.6,-0.426163433000016));
#264801=CARTESIAN_POINT('Ctrl Pts',(-10.8784503780001,15.2,-0.427159131000017));
#264802=CARTESIAN_POINT('Ctrl Pts',(-10.8784503780001,11.6,-0.427159131000017));
#264803=CARTESIAN_POINT('Ctrl Pts',(-10.8811153220001,15.2,-0.428159018000014));
#264804=CARTESIAN_POINT('Ctrl Pts',(-10.8811153220001,11.6,-0.428159018000014));
#264805=CARTESIAN_POINT('Ctrl Pts',(-10.8837846900001,15.2,-0.429163097000016));
#264806=CARTESIAN_POINT('Ctrl Pts',(-10.8837846900001,11.6,-0.429163097000016));
#264807=CARTESIAN_POINT('Ctrl Pts',(-10.8864584680001,15.2,-0.430171373000015));
#264808=CARTESIAN_POINT('Ctrl Pts',(-10.8864584680001,11.6,-0.430171373000015));
#264809=CARTESIAN_POINT('Ctrl Pts',(-10.8891366430001,15.2,-0.431183850000014));
#264810=CARTESIAN_POINT('Ctrl Pts',(-10.8891366430001,11.6,-0.431183850000015));
#264811=CARTESIAN_POINT('Ctrl Pts',(-10.8918192040001,15.2,-0.432200531000015));
#264812=CARTESIAN_POINT('Ctrl Pts',(-10.8918192040001,11.6,-0.432200531000016));
#264813=CARTESIAN_POINT('Ctrl Pts',(-10.8945061380001,15.2,-0.433221421000014));
#264814=CARTESIAN_POINT('Ctrl Pts',(-10.8945061380001,11.6,-0.433221421000014));
#264815=CARTESIAN_POINT('Ctrl Pts',(-10.8971974330001,15.2,-0.434246522000015));
#264816=CARTESIAN_POINT('Ctrl Pts',(-10.8971974330001,11.6,-0.434246522000015));
#264817=CARTESIAN_POINT('Ctrl Pts',(-10.8998930780001,15.2,-0.435275840000013));
#264818=CARTESIAN_POINT('Ctrl Pts',(-10.8998930780001,11.6,-0.435275840000014));
#264819=CARTESIAN_POINT('Ctrl Pts',(-10.9025930590001,15.2,-0.436309378000015));
#264820=CARTESIAN_POINT('Ctrl Pts',(-10.9025930590001,11.6,-0.436309378000015));
#264821=CARTESIAN_POINT('Ctrl Pts',(-10.9052973640001,15.2,-0.437347141000015));
#264822=CARTESIAN_POINT('Ctrl Pts',(-10.9052973640001,11.6,-0.437347141000016));
#264823=CARTESIAN_POINT('Ctrl Pts',(-10.9080059810001,15.2,-0.438389130000014));
#264824=CARTESIAN_POINT('Ctrl Pts',(-10.9080059810001,11.6,-0.438389130000015));
#264825=CARTESIAN_POINT('Ctrl Pts',(-10.9107188990001,15.2,-0.439435350000017));
#264826=CARTESIAN_POINT('Ctrl Pts',(-10.9107188990001,11.6,-0.439435350000017));
#264827=CARTESIAN_POINT('Ctrl Pts',(-10.9134361040001,15.2,-0.440485807000015));
#264828=CARTESIAN_POINT('Ctrl Pts',(-10.9134361040001,11.6,-0.440485807000015));
#264829=CARTESIAN_POINT('Ctrl Pts',(-10.9161575860001,15.2,-0.441540501000013));
#264830=CARTESIAN_POINT('Ctrl Pts',(-10.9161575860001,11.6,-0.441540501000013));
#264831=CARTESIAN_POINT('Ctrl Pts',(-10.9188833300001,15.2,-0.442599438000015));
#264832=CARTESIAN_POINT('Ctrl Pts',(-10.9188833300001,11.6,-0.442599438000016));
#264833=CARTESIAN_POINT('Ctrl Pts',(-10.9216133270001,15.2,-0.443662622000014));
#264834=CARTESIAN_POINT('Ctrl Pts',(-10.9216133270001,11.6,-0.443662622000014));
#264835=CARTESIAN_POINT('Ctrl Pts',(-10.9243475630001,15.2,-0.444730056000013));
#264836=CARTESIAN_POINT('Ctrl Pts',(-10.9243475630001,11.6,-0.444730056000014));
#264837=CARTESIAN_POINT('Ctrl Pts',(-10.9270860270001,15.2,-0.445801743000014));
#264838=CARTESIAN_POINT('Ctrl Pts',(-10.9270860270001,11.6,-0.445801743000014));
#264839=CARTESIAN_POINT('Ctrl Pts',(-10.9298287070001,15.2,-0.446877689000011));
#264840=CARTESIAN_POINT('Ctrl Pts',(-10.9298287070001,11.6,-0.446877689000012));
#264841=CARTESIAN_POINT('Ctrl Pts',(-10.9325755900001,15.2,-0.447957894000015));
#264842=CARTESIAN_POINT('Ctrl Pts',(-10.9325755900001,11.6,-0.447957894000016));
#264843=CARTESIAN_POINT('Ctrl Pts',(-10.9353266640001,15.2,-0.449042364000016));
#264844=CARTESIAN_POINT('Ctrl Pts',(-10.9353266640001,11.6,-0.449042364000017));
#264845=CARTESIAN_POINT('Ctrl Pts',(-10.9380819200001,15.2,-0.450131103000011));
#264846=CARTESIAN_POINT('Ctrl Pts',(-10.9380819200001,11.6,-0.450131103000011));
#264847=CARTESIAN_POINT('Ctrl Pts',(-10.9408413420001,15.2,-0.451224112000013));
#264848=CARTESIAN_POINT('Ctrl Pts',(-10.9408413420001,11.6,-0.451224112000013));
#264849=CARTESIAN_POINT('Ctrl Pts',(-10.9436049220001,15.2,-0.452321397000013));
#264850=CARTESIAN_POINT('Ctrl Pts',(-10.9436049220001,11.6,-0.452321397000013));
#264851=CARTESIAN_POINT('Ctrl Pts',(-10.9463726460001,15.2,-0.453422962000012));
#264852=CARTESIAN_POINT('Ctrl Pts',(-10.9463726460001,11.6,-0.453422962000012));
#264853=CARTESIAN_POINT('Ctrl Pts',(-10.9491445020001,15.2,-0.454528810000014));
#264854=CARTESIAN_POINT('Ctrl Pts',(-10.9491445020001,11.6,-0.454528810000015));
#264855=CARTESIAN_POINT('Ctrl Pts',(-10.9519204780001,15.2,-0.455638942000016));
#264856=CARTESIAN_POINT('Ctrl Pts',(-10.9519204780001,11.6,-0.455638942000017));
#264857=CARTESIAN_POINT('Ctrl Pts',(-10.9547005640001,15.2,-0.456753364000013));
#264858=CARTESIAN_POINT('Ctrl Pts',(-10.9547005640001,11.6,-0.456753364000014));
#264859=CARTESIAN_POINT('Ctrl Pts',(-10.9574847480001,15.2,-0.457872080000015));
#264860=CARTESIAN_POINT('Ctrl Pts',(-10.9574847480001,11.6,-0.457872080000015));
#264861=CARTESIAN_POINT('Ctrl Pts',(-10.9602730170001,15.2,-0.458995091000016));
#264862=CARTESIAN_POINT('Ctrl Pts',(-10.9602730170001,11.6,-0.458995091000017));
#264863=CARTESIAN_POINT('Ctrl Pts',(-10.9630653590001,15.2,-0.460122402000014));
#264864=CARTESIAN_POINT('Ctrl Pts',(-10.9630653590001,11.6,-0.460122402000014));
#264865=CARTESIAN_POINT('Ctrl Pts',(-10.9658617640001,15.2,-0.461254017000012));
#264866=CARTESIAN_POINT('Ctrl Pts',(-10.9658617640001,11.6,-0.461254017000013));
#264867=CARTESIAN_POINT('Ctrl Pts',(-10.9686622200001,15.2,-0.462389938000012));
#264868=CARTESIAN_POINT('Ctrl Pts',(-10.9686622200001,11.6,-0.462389938000012));
#264869=CARTESIAN_POINT('Ctrl Pts',(-10.9714667150001,15.2,-0.463530170000013));
#264870=CARTESIAN_POINT('Ctrl Pts',(-10.9714667150001,11.6,-0.463530170000013));
#264871=CARTESIAN_POINT('Ctrl Pts',(-10.9742752370001,15.2,-0.464674714000015));
#264872=CARTESIAN_POINT('Ctrl Pts',(-10.9742752370001,11.6,-0.464674714000016));
#264873=CARTESIAN_POINT('Ctrl Pts',(-10.9770877740001,15.2,-0.465823575000015));
#264874=CARTESIAN_POINT('Ctrl Pts',(-10.9770877740001,11.6,-0.465823575000015));
#264875=CARTESIAN_POINT('Ctrl Pts',(-10.9799043170001,15.2,-0.466976757000013));
#264876=CARTESIAN_POINT('Ctrl Pts',(-10.9799043170001,11.6,-0.466976757000013));
#264877=CARTESIAN_POINT('Ctrl Pts',(-10.9827248520001,15.2,-0.468134263000017));
#264878=CARTESIAN_POINT('Ctrl Pts',(-10.9827248520001,11.6,-0.468134263000018));
#264879=CARTESIAN_POINT('Ctrl Pts',(-10.9855493680001,15.2,-0.469296094000011));
#264880=CARTESIAN_POINT('Ctrl Pts',(-10.9855493680001,11.6,-0.469296094000012));
#264881=CARTESIAN_POINT('Ctrl Pts',(-10.9883778540001,15.2,-0.470462257000013));
#264882=CARTESIAN_POINT('Ctrl Pts',(-10.9883778540001,11.6,-0.470462257000013));
#264883=CARTESIAN_POINT('Ctrl Pts',(-10.9912102990001,15.2,-0.471632753000013));
#264884=CARTESIAN_POINT('Ctrl Pts',(-10.9912102990001,11.6,-0.471632753000014));
#264885=CARTESIAN_POINT('Ctrl Pts',(-10.9940466900001,15.2,-0.472807585000012));
#264886=CARTESIAN_POINT('Ctrl Pts',(-10.9940466900001,11.6,-0.472807585000013));
#264887=CARTESIAN_POINT('Ctrl Pts',(-10.9968870170001,15.2,-0.473986757000016));
#264888=CARTESIAN_POINT('Ctrl Pts',(-10.9968870170001,11.6,-0.473986757000016));
#264889=CARTESIAN_POINT('Ctrl Pts',(-10.9997312680001,15.2,-0.475170273000014));
#264890=CARTESIAN_POINT('Ctrl Pts',(-10.9997312680001,11.6,-0.475170273000014));
#264891=CARTESIAN_POINT('Ctrl Pts',(-11.0025794320001,15.2,-0.476358134000012));
#264892=CARTESIAN_POINT('Ctrl Pts',(-11.0025794320001,11.6,-0.476358134000013));
#264893=CARTESIAN_POINT('Ctrl Pts',(-11.0054314970001,15.2,-0.477550346000015));
#264894=CARTESIAN_POINT('Ctrl Pts',(-11.0054314970001,11.6,-0.477550346000016));
#264895=CARTESIAN_POINT('Ctrl Pts',(-11.0082874530001,15.2,-0.478746910000014));
#264896=CARTESIAN_POINT('Ctrl Pts',(-11.0082874530001,11.6,-0.478746910000015));
#264897=CARTESIAN_POINT('Ctrl Pts',(-11.0111472870001,15.2,-0.479947831000014));
#264898=CARTESIAN_POINT('Ctrl Pts',(-11.0111472870001,11.6,-0.479947831000014));
#264899=CARTESIAN_POINT('Ctrl Pts',(-11.0140109890001,15.2,-0.481153110000014));
#264900=CARTESIAN_POINT('Ctrl Pts',(-11.0140109890001,11.6,-0.481153110000015));
#264901=CARTESIAN_POINT('Ctrl Pts',(-11.0168785470001,15.2,-0.482362752000016));
#264902=CARTESIAN_POINT('Ctrl Pts',(-11.0168785470001,11.6,-0.482362752000017));
#264903=CARTESIAN_POINT('Ctrl Pts',(-11.0197499510001,15.2,-0.483576758000015));
#264904=CARTESIAN_POINT('Ctrl Pts',(-11.0197499510001,11.6,-0.483576758000015));
#264905=CARTESIAN_POINT('Ctrl Pts',(-11.0226251880001,15.2,-0.484795134000016));
#264906=CARTESIAN_POINT('Ctrl Pts',(-11.0226251880001,11.6,-0.484795134000016));
#264907=CARTESIAN_POINT('Ctrl Pts',(-11.0255042470001,15.2,-0.486017881000014));
#264908=CARTESIAN_POINT('Ctrl Pts',(-11.0255042470001,11.6,-0.486017881000014));
#264909=CARTESIAN_POINT('Ctrl Pts',(-11.0283871190001,15.2,-0.487245003000014));
#264910=CARTESIAN_POINT('Ctrl Pts',(-11.0283871190001,11.6,-0.487245003000015));
#264911=CARTESIAN_POINT('Ctrl Pts',(-11.0312737910001,15.2,-0.488476502000013));
#264912=CARTESIAN_POINT('Ctrl Pts',(-11.0312737910001,11.6,-0.488476502000013));
#264913=CARTESIAN_POINT('Ctrl Pts',(-11.0341642530001,15.2,-0.489712383000014));
#264914=CARTESIAN_POINT('Ctrl Pts',(-11.0341642530001,11.6,-0.489712383000014));
#264915=CARTESIAN_POINT('Ctrl Pts',(-11.0370584920001,15.2,-0.490952646000018));
#264916=CARTESIAN_POINT('Ctrl Pts',(-11.0370584920001,11.6,-0.490952646000018));
#264917=CARTESIAN_POINT('Ctrl Pts',(-11.0399564980001,15.2,-0.492197297000012));
#264918=CARTESIAN_POINT('Ctrl Pts',(-11.0399564980001,11.6,-0.492197297000013));
#264919=CARTESIAN_POINT('Ctrl Pts',(-11.0428582610001,15.2,-0.493446338000014));
#264920=CARTESIAN_POINT('Ctrl Pts',(-11.0428582610001,11.6,-0.493446338000015));
#264921=CARTESIAN_POINT('Ctrl Pts',(-11.0457637680001,15.2,-0.494699772000011));
#264922=CARTESIAN_POINT('Ctrl Pts',(-11.0457637680001,11.6,-0.494699772000012));
#264923=CARTESIAN_POINT('Ctrl Pts',(-11.0486730100001,15.2,-0.495957601000012));
#264924=CARTESIAN_POINT('Ctrl Pts',(-11.0486730100001,11.6,-0.495957601000013));
#264925=CARTESIAN_POINT('Ctrl Pts',(-11.0515859750001,15.2,-0.497219830000013));
#264926=CARTESIAN_POINT('Ctrl Pts',(-11.0515859750001,11.6,-0.497219830000013));
#264927=CARTESIAN_POINT('Ctrl Pts',(-11.0545026510001,15.2,-0.498486460000014));
#264928=CARTESIAN_POINT('Ctrl Pts',(-11.0545026510001,11.6,-0.498486460000014));
#264929=CARTESIAN_POINT('Ctrl Pts',(-11.0574230290001,15.2,-0.499757494000015));
#264930=CARTESIAN_POINT('Ctrl Pts',(-11.0574230290001,11.6,-0.499757494000015));
#264931=CARTESIAN_POINT('Ctrl Pts',(-11.0603470970001,15.2,-0.501032937000012));
#264932=CARTESIAN_POINT('Ctrl Pts',(-11.0603470970001,11.6,-0.501032937000013));
#264933=CARTESIAN_POINT('Ctrl Pts',(-11.0632748440001,15.2,-0.502312789000015));
#264934=CARTESIAN_POINT('Ctrl Pts',(-11.0632748440001,11.6,-0.502312789000015));
#264935=CARTESIAN_POINT('Ctrl Pts',(-11.0662062590001,15.2,-0.503597056000018));
#264936=CARTESIAN_POINT('Ctrl Pts',(-11.0662062590001,11.6,-0.503597056000018));
#264937=CARTESIAN_POINT('Ctrl Pts',(-11.0691413320001,15.2,-0.504885738000014));
#264938=CARTESIAN_POINT('Ctrl Pts',(-11.0691413320001,11.6,-0.504885738000014));
#264939=CARTESIAN_POINT('Ctrl Pts',(-11.0720800520001,15.2,-0.506178839000011));
#264940=CARTESIAN_POINT('Ctrl Pts',(-11.0720800520001,11.6,-0.506178839000011));
#264941=CARTESIAN_POINT('Ctrl Pts',(-11.0750224080001,15.2,-0.507476362000014));
#264942=CARTESIAN_POINT('Ctrl Pts',(-11.0750224080001,11.6,-0.507476362000015));
#264943=CARTESIAN_POINT('Ctrl Pts',(-11.0779683880001,15.2,-0.508778311000011));
#264944=CARTESIAN_POINT('Ctrl Pts',(-11.0779683880001,11.6,-0.508778311000011));
#264945=CARTESIAN_POINT('Ctrl Pts',(-11.0809179820001,15.2,-0.510084687000014));
#264946=CARTESIAN_POINT('Ctrl Pts',(-11.0809179820001,11.6,-0.510084687000015));
#264947=CARTESIAN_POINT('Ctrl Pts',(-11.0838711810001,15.2,-0.511395492000015));
#264948=CARTESIAN_POINT('Ctrl Pts',(-11.0838711810001,11.6,-0.511395492000016));
#264949=CARTESIAN_POINT('Ctrl Pts',(-11.0868279720001,15.2,-0.512710732000015));
#264950=CARTESIAN_POINT('Ctrl Pts',(-11.0868279720001,11.6,-0.512710732000015));
#264951=CARTESIAN_POINT('Ctrl Pts',(-11.0897883450001,15.2,-0.514030406000017));
#264952=CARTESIAN_POINT('Ctrl Pts',(-11.0897883450001,11.6,-0.514030406000017));
#264953=CARTESIAN_POINT('Ctrl Pts',(-11.0927522890001,15.2,-0.515354521000013));
#264954=CARTESIAN_POINT('Ctrl Pts',(-11.0927522890001,11.6,-0.515354521000014));
#264955=CARTESIAN_POINT('Ctrl Pts',(-11.0957197940001,15.2,-0.516683076000017));
#264956=CARTESIAN_POINT('Ctrl Pts',(-11.0957197940001,11.6,-0.516683076000018));
#264957=CARTESIAN_POINT('Ctrl Pts',(-11.0986908480001,15.2,-0.518016075000016));
#264958=CARTESIAN_POINT('Ctrl Pts',(-11.0986908480001,11.6,-0.518016075000017));
#264959=CARTESIAN_POINT('Ctrl Pts',(-11.1016654420001,15.2,-0.519353522000015));
#264960=CARTESIAN_POINT('Ctrl Pts',(-11.1016654420001,11.6,-0.519353522000015));
#264961=CARTESIAN_POINT('Ctrl Pts',(-11.1046435640001,15.2,-0.520695418000017));
#264962=CARTESIAN_POINT('Ctrl Pts',(-11.1046435640001,11.6,-0.520695418000017));
#264963=CARTESIAN_POINT('Ctrl Pts',(-11.1076252050001,15.2,-0.522041766000014));
#264964=CARTESIAN_POINT('Ctrl Pts',(-11.1076252050001,11.6,-0.522041766000015));
#264965=CARTESIAN_POINT('Ctrl Pts',(-11.1106103520001,15.2,-0.523392569000016));
#264966=CARTESIAN_POINT('Ctrl Pts',(-11.1106103520001,11.6,-0.523392569000017));
#264967=CARTESIAN_POINT('Ctrl Pts',(-11.1135989970001,15.2,-0.524747830000014));
#264968=CARTESIAN_POINT('Ctrl Pts',(-11.1135989970001,11.6,-0.524747830000015));
#264969=CARTESIAN_POINT('Ctrl Pts',(-11.1165911290001,15.2,-0.526107550000017));
#264970=CARTESIAN_POINT('Ctrl Pts',(-11.1165911290001,11.6,-0.526107550000017));
#264971=CARTESIAN_POINT('Ctrl Pts',(-11.1195867360001,15.2,-0.527471735000016));
#264972=CARTESIAN_POINT('Ctrl Pts',(-11.1195867360001,11.6,-0.527471735000016));
#264973=CARTESIAN_POINT('Ctrl Pts',(-11.1225858080001,15.2,-0.528840384000016));
#264974=CARTESIAN_POINT('Ctrl Pts',(-11.1225858080001,11.6,-0.528840384000016));
#264975=CARTESIAN_POINT('Ctrl Pts',(-11.1255883350001,15.2,-0.530213501000016));
#264976=CARTESIAN_POINT('Ctrl Pts',(-11.1255883350001,11.6,-0.530213501000017));
#264977=CARTESIAN_POINT('Ctrl Pts',(-11.1285943060001,15.2,-0.531591090000014));
#264978=CARTESIAN_POINT('Ctrl Pts',(-11.1285943060001,11.6,-0.531591090000015));
#264979=CARTESIAN_POINT('Ctrl Pts',(-11.1316037120001,15.2,-0.532973151000018));
#264980=CARTESIAN_POINT('Ctrl Pts',(-11.1316037120001,11.6,-0.532973151000018));
#264981=CARTESIAN_POINT('Ctrl Pts',(-11.1346165400001,15.2,-0.534359689000015));
#264982=CARTESIAN_POINT('Ctrl Pts',(-11.1346165400001,11.6,-0.534359689000015));
#264983=CARTESIAN_POINT('Ctrl Pts',(-11.1376327810001,15.2,-0.535750705000013));
#264984=CARTESIAN_POINT('Ctrl Pts',(-11.1376327810001,11.6,-0.535750705000014));
#264985=CARTESIAN_POINT('Ctrl Pts',(-11.1406524250001,15.2,-0.537146200000014));
#264986=CARTESIAN_POINT('Ctrl Pts',(-11.1406524250001,11.6,-0.537146200000014));
#264987=CARTESIAN_POINT('Ctrl Pts',(-11.1436754620001,15.2,-0.538546181000013));
#264988=CARTESIAN_POINT('Ctrl Pts',(-11.1436754620001,11.6,-0.538546181000013));
#264989=CARTESIAN_POINT('Ctrl Pts',(-11.1467018790001,15.2,-0.539950647000014));
#264990=CARTESIAN_POINT('Ctrl Pts',(-11.1467018790001,11.6,-0.539950647000014));
#264991=CARTESIAN_POINT('Ctrl Pts',(-11.1497316690001,15.2,-0.541359602000018));
#264992=CARTESIAN_POINT('Ctrl Pts',(-11.1497316690001,11.6,-0.541359602000018));
#264993=CARTESIAN_POINT('Ctrl Pts',(-11.1527648200001,15.2,-0.542773047000011));
#264994=CARTESIAN_POINT('Ctrl Pts',(-11.1527648200001,11.6,-0.542773047000012));
#264995=CARTESIAN_POINT('Ctrl Pts',(-11.1558013220001,15.2,-0.544190986000017));
#264996=CARTESIAN_POINT('Ctrl Pts',(-11.1558013220001,11.6,-0.544190986000018));
#264997=CARTESIAN_POINT('Ctrl Pts',(-11.1588411640001,15.2,-0.545613421000013));
#264998=CARTESIAN_POINT('Ctrl Pts',(-11.1588411640001,11.6,-0.545613421000013));
#264999=CARTESIAN_POINT('Ctrl Pts',(-11.1618843360001,15.2,-0.547040354000017));
#265000=CARTESIAN_POINT('Ctrl Pts',(-11.1618843360001,11.6,-0.547040354000017));
#265001=CARTESIAN_POINT('Ctrl Pts',(-11.1649308290001,15.2,-0.548471788000011));
#265002=CARTESIAN_POINT('Ctrl Pts',(-11.1649308290001,11.6,-0.548471788000012));
#265003=CARTESIAN_POINT('Ctrl Pts',(-11.1679806310001,15.2,-0.549907725000014));
#265004=CARTESIAN_POINT('Ctrl Pts',(-11.1679806310001,11.6,-0.549907725000014));
#265005=CARTESIAN_POINT('Ctrl Pts',(-11.1710337330001,15.2,-0.551348168000012));
#265006=CARTESIAN_POINT('Ctrl Pts',(-11.1710337330001,11.6,-0.551348168000013));
#265007=CARTESIAN_POINT('Ctrl Pts',(-11.1740901240001,15.2,-0.552793118000015));
#265008=CARTESIAN_POINT('Ctrl Pts',(-11.1740901240001,11.6,-0.552793118000015));
#265009=CARTESIAN_POINT('Ctrl Pts',(-11.1771497950001,15.2,-0.554242580000013));
#265010=CARTESIAN_POINT('Ctrl Pts',(-11.1771497950001,11.6,-0.554242580000013));
#265011=CARTESIAN_POINT('Ctrl Pts',(-11.1802127340001,15.2,-0.555696554000011));
#265012=CARTESIAN_POINT('Ctrl Pts',(-11.1802127340001,11.6,-0.555696554000012));
#265013=CARTESIAN_POINT('Ctrl Pts',(-11.1832789320001,15.2,-0.557155042000015));
#265014=CARTESIAN_POINT('Ctrl Pts',(-11.1832789320001,11.6,-0.557155042000015));
#265015=CARTESIAN_POINT('Ctrl Pts',(-11.1863483800001,15.2,-0.558618049000015));
#265016=CARTESIAN_POINT('Ctrl Pts',(-11.1863483800001,11.6,-0.558618049000015));
#265017=CARTESIAN_POINT('Ctrl Pts',(-11.1894210660001,15.2,-0.560085575000016));
#265018=CARTESIAN_POINT('Ctrl Pts',(-11.1894210660001,11.6,-0.560085575000016));
#265019=CARTESIAN_POINT('Ctrl Pts',(-11.1924969800001,15.2,-0.561557623000013));
#265020=CARTESIAN_POINT('Ctrl Pts',(-11.1924969800001,11.6,-0.561557623000013));
#265021=CARTESIAN_POINT('Ctrl Pts',(-11.1955761130001,15.2,-0.563034196000016));
#265022=CARTESIAN_POINT('Ctrl Pts',(-11.1955761130001,11.6,-0.563034196000017));
#265023=CARTESIAN_POINT('Ctrl Pts',(-11.1986584540001,15.2,-0.564515295000017));
#265024=CARTESIAN_POINT('Ctrl Pts',(-11.1986584540001,11.6,-0.564515295000017));
#265025=CARTESIAN_POINT('Ctrl Pts',(-11.2017439940001,15.2,-0.566000924000014));
#265026=CARTESIAN_POINT('Ctrl Pts',(-11.2017439940001,11.6,-0.566000924000015));
#265027=CARTESIAN_POINT('Ctrl Pts',(-11.2048327210001,15.2,-0.567491084000018));
#265028=CARTESIAN_POINT('Ctrl Pts',(-11.2048327210001,11.6,-0.567491084000018));
#265029=CARTESIAN_POINT('Ctrl Pts',(-11.2079246280001,15.2,-0.568985776000015));
#265030=CARTESIAN_POINT('Ctrl Pts',(-11.2079246280001,11.6,-0.568985776000015));
#265031=CARTESIAN_POINT('Ctrl Pts',(-11.2110197020001,15.2,-0.570485006000014));
#265032=CARTESIAN_POINT('Ctrl Pts',(-11.2110197020001,11.6,-0.570485006000015));
#265033=CARTESIAN_POINT('Ctrl Pts',(-11.2141179350001,15.2,-0.571988772000012));
#265034=CARTESIAN_POINT('Ctrl Pts',(-11.2141179350001,11.6,-0.571988772000012));
#265035=CARTESIAN_POINT('Ctrl Pts',(-11.2172193170001,15.2,-0.573497079000016));
#265036=CARTESIAN_POINT('Ctrl Pts',(-11.2172193170001,11.6,-0.573497079000016));
#265037=CARTESIAN_POINT('Ctrl Pts',(-11.2203238380001,15.2,-0.575009928000014));
#265038=CARTESIAN_POINT('Ctrl Pts',(-11.2203238380001,11.6,-0.575009928000015));
#265039=CARTESIAN_POINT('Ctrl Pts',(-11.2234314850001,15.2,-0.576527323000011));
#265040=CARTESIAN_POINT('Ctrl Pts',(-11.2234314850001,11.6,-0.576527323000012));
#265041=CARTESIAN_POINT('Ctrl Pts',(-11.2265422530001,15.2,-0.578049263000011));
#265042=CARTESIAN_POINT('Ctrl Pts',(-11.2265422530001,11.6,-0.578049263000012));
#265043=CARTESIAN_POINT('Ctrl Pts',(-11.2296561290001,15.2,-0.579575753000015));
#265044=CARTESIAN_POINT('Ctrl Pts',(-11.2296561290001,11.6,-0.579575753000015));
#265045=CARTESIAN_POINT('Ctrl Pts',(-11.2327731030001,15.2,-0.581106794000017));
#265046=CARTESIAN_POINT('Ctrl Pts',(-11.2327731030001,11.6,-0.581106794000017));
#265047=CARTESIAN_POINT('Ctrl Pts',(-11.2358931670001,15.2,-0.582642387000014));
#265048=CARTESIAN_POINT('Ctrl Pts',(-11.2358931670001,11.6,-0.582642387000015));
#265049=CARTESIAN_POINT('Ctrl Pts',(-11.2390163100001,15.2,-0.584182538000011));
#265050=CARTESIAN_POINT('Ctrl Pts',(-11.2390163100001,11.6,-0.584182538000011));
#265051=CARTESIAN_POINT('Ctrl Pts',(-11.2421425230001,15.2,-0.585727245000012));
#265052=CARTESIAN_POINT('Ctrl Pts',(-11.2421425230001,11.6,-0.585727245000012));
#265053=CARTESIAN_POINT('Ctrl Pts',(-11.2452717950001,15.2,-0.587276511000017));
#265054=CARTESIAN_POINT('Ctrl Pts',(-11.2452717950001,11.6,-0.587276511000017));
#265055=CARTESIAN_POINT('Ctrl Pts',(-11.2484041180001,15.2,-0.588830340000013));
#265056=CARTESIAN_POINT('Ctrl Pts',(-11.2484041180001,11.6,-0.588830340000013));
#265057=CARTESIAN_POINT('Ctrl Pts',(-11.2515394790001,15.2,-0.590388732000013));
#265058=CARTESIAN_POINT('Ctrl Pts',(-11.2515394790001,11.6,-0.590388732000014));
#265059=CARTESIAN_POINT('Ctrl Pts',(-11.2546778710001,15.2,-0.591951690000014));
#265060=CARTESIAN_POINT('Ctrl Pts',(-11.2546778710001,11.6,-0.591951690000015));
#265061=CARTESIAN_POINT('Ctrl Pts',(-11.2578192840001,15.2,-0.593519216000011));
#265062=CARTESIAN_POINT('Ctrl Pts',(-11.2578192840001,11.6,-0.593519216000012));
#265063=CARTESIAN_POINT('Ctrl Pts',(-11.2609637080001,15.2,-0.595091312000013));
#265064=CARTESIAN_POINT('Ctrl Pts',(-11.2609637080001,11.6,-0.595091312000014));
#265065=CARTESIAN_POINT('Ctrl Pts',(-11.2641111320001,15.2,-0.596667981000016));
#265066=CARTESIAN_POINT('Ctrl Pts',(-11.2641111320001,11.6,-0.596667981000017));
#265067=CARTESIAN_POINT('Ctrl Pts',(-11.2672615480001,15.2,-0.598249222000016));
#265068=CARTESIAN_POINT('Ctrl Pts',(-11.2672615480001,11.6,-0.598249222000016));
#265069=CARTESIAN_POINT('Ctrl Pts',(-11.2704149460001,15.2,-0.599835041000016));
#265070=CARTESIAN_POINT('Ctrl Pts',(-11.2704149460001,11.6,-0.599835041000017));
#265071=CARTESIAN_POINT('Ctrl Pts',(-11.2735713160001,15.2,-0.601425437000014));
#265072=CARTESIAN_POINT('Ctrl Pts',(-11.2735713160001,11.6,-0.601425437000014));
#265073=CARTESIAN_POINT('Ctrl Pts',(-11.2767306480001,15.2,-0.603020414000017));
#265074=CARTESIAN_POINT('Ctrl Pts',(-11.2767306480001,11.6,-0.603020414000018));
#265075=CARTESIAN_POINT('Ctrl Pts',(-11.2798929340001,15.2,-0.604619973000013));
#265076=CARTESIAN_POINT('Ctrl Pts',(-11.2798929340001,11.6,-0.604619973000014));
#265077=CARTESIAN_POINT('Ctrl Pts',(-11.2830581620001,15.2,-0.606224115000016));
#265078=CARTESIAN_POINT('Ctrl Pts',(-11.2830581620001,11.6,-0.606224115000016));
#265079=CARTESIAN_POINT('Ctrl Pts',(-11.2862263240001,15.2,-0.607832843000011));
#265080=CARTESIAN_POINT('Ctrl Pts',(-11.2862263240001,11.6,-0.607832843000012));
#265081=CARTESIAN_POINT('Ctrl Pts',(-11.2893974100001,15.2,-0.609446160000013));
#265082=CARTESIAN_POINT('Ctrl Pts',(-11.2893974100001,11.6,-0.609446160000014));
#265083=CARTESIAN_POINT('Ctrl Pts',(-11.2925714100001,15.2,-0.611064067000013));
#265084=CARTESIAN_POINT('Ctrl Pts',(-11.2925714100001,11.6,-0.611064067000014));
#265085=CARTESIAN_POINT('Ctrl Pts',(-11.2957483150001,15.2,-0.612686565000011));
#265086=CARTESIAN_POINT('Ctrl Pts',(-11.2957483150001,11.6,-0.612686565000012));
#265087=CARTESIAN_POINT('Ctrl Pts',(-11.2989281170001,15.2,-0.614313657000016));
#265088=CARTESIAN_POINT('Ctrl Pts',(-11.2989281170001,11.6,-0.614313657000017));
#265089=CARTESIAN_POINT('Ctrl Pts',(-11.3021108030001,15.2,-0.615945345000015));
#265090=CARTESIAN_POINT('Ctrl Pts',(-11.3021108030001,11.6,-0.615945345000016));
#265091=CARTESIAN_POINT('Ctrl Pts',(-11.3052963650001,15.2,-0.617581630000017));
#265092=CARTESIAN_POINT('Ctrl Pts',(-11.3052963650001,11.6,-0.617581630000017));
#265093=CARTESIAN_POINT('Ctrl Pts',(-11.3084847960001,15.2,-0.619222515000013));
#265094=CARTESIAN_POINT('Ctrl Pts',(-11.3084847960001,11.6,-0.619222515000013));
#265095=CARTESIAN_POINT('Ctrl Pts',(-11.3116760820001,15.2,-0.620868001000012));
#265096=CARTESIAN_POINT('Ctrl Pts',(-11.3116760820001,11.6,-0.620868001000013));
#265097=CARTESIAN_POINT('Ctrl Pts',(-11.3148702170001,15.2,-0.622518091000015));
#265098=CARTESIAN_POINT('Ctrl Pts',(-11.3148702170001,11.6,-0.622518091000015));
#265099=CARTESIAN_POINT('Ctrl Pts',(-11.3180671910001,15.2,-0.624172784000017));
#265100=CARTESIAN_POINT('Ctrl Pts',(-11.3180671910001,11.6,-0.624172784000017));
#265101=CARTESIAN_POINT('Ctrl Pts',(-11.3212669940001,15.2,-0.625832085000013));
#265102=CARTESIAN_POINT('Ctrl Pts',(-11.3212669940001,11.6,-0.625832085000014));
#265103=CARTESIAN_POINT('Ctrl Pts',(-11.3244696160001,15.2,-0.627495996000014));
#265104=CARTESIAN_POINT('Ctrl Pts',(-11.3244696160001,11.6,-0.627495996000014));
#265105=CARTESIAN_POINT('Ctrl Pts',(-11.3276750490001,15.2,-0.629164515000014));
#265106=CARTESIAN_POINT('Ctrl Pts',(-11.3276750490001,11.6,-0.629164515000014));
#265107=CARTESIAN_POINT('Ctrl Pts',(-11.3308832820001,15.2,-0.630837648000018));
#265108=CARTESIAN_POINT('Ctrl Pts',(-11.3308832820001,11.6,-0.630837648000018));
#265109=CARTESIAN_POINT('Ctrl Pts',(-11.3340943080001,15.2,-0.632515395000013));
#265110=CARTESIAN_POINT('Ctrl Pts',(-11.3340943080001,11.6,-0.632515395000013));
#265111=CARTESIAN_POINT('Ctrl Pts',(-11.3373081150001,15.2,-0.634197758000017));
#265112=CARTESIAN_POINT('Ctrl Pts',(-11.3373081150001,11.6,-0.634197758000017));
#265113=CARTESIAN_POINT('Ctrl Pts',(-11.3405246950001,15.2,-0.635884737000012));
#265114=CARTESIAN_POINT('Ctrl Pts',(-11.3405246950001,11.6,-0.635884737000012));
#265115=CARTESIAN_POINT('Ctrl Pts',(-11.3437440390001,15.2,-0.637576336000016));
#265116=CARTESIAN_POINT('Ctrl Pts',(-11.3437440390001,11.6,-0.637576336000017));
#265117=CARTESIAN_POINT('Ctrl Pts',(-11.3469661360001,15.2,-0.639272557000012));
#265118=CARTESIAN_POINT('Ctrl Pts',(-11.3469661360001,11.6,-0.639272557000013));
#265119=CARTESIAN_POINT('Ctrl Pts',(-11.3501909790001,15.2,-0.640973401000018));
#265120=CARTESIAN_POINT('Ctrl Pts',(-11.3501909790001,11.6,-0.640973401000018));
#265121=CARTESIAN_POINT('Ctrl Pts',(-11.3534185570001,15.2,-0.642678869000015));
#265122=CARTESIAN_POINT('Ctrl Pts',(-11.3534185570001,11.6,-0.642678869000016));
#265123=CARTESIAN_POINT('Ctrl Pts',(-11.3566488620001,15.2,-0.644388964000013));
#265124=CARTESIAN_POINT('Ctrl Pts',(-11.3566488620001,11.6,-0.644388964000014));
#265125=CARTESIAN_POINT('Ctrl Pts',(-11.3598818840001,15.2,-0.646103687000017));
#265126=CARTESIAN_POINT('Ctrl Pts',(-11.3598818840001,11.6,-0.646103687000017));
#265127=CARTESIAN_POINT('Ctrl Pts',(-11.3631176140001,15.2,-0.647823039000013));
#265128=CARTESIAN_POINT('Ctrl Pts',(-11.3631176140001,11.6,-0.647823039000013));
#265129=CARTESIAN_POINT('Ctrl Pts',(-11.3663560430001,15.2,-0.649547023000014));
#265130=CARTESIAN_POINT('Ctrl Pts',(-11.3663560430001,11.6,-0.649547023000015));
#265131=CARTESIAN_POINT('Ctrl Pts',(-11.3695971620001,15.2,-0.651275639000013));
#265132=CARTESIAN_POINT('Ctrl Pts',(-11.3695971620001,11.6,-0.651275639000013));
#265133=CARTESIAN_POINT('Ctrl Pts',(-11.3728409600001,15.2,-0.653008892000013));
#265134=CARTESIAN_POINT('Ctrl Pts',(-11.3728409600001,11.6,-0.653008892000014));
#265135=CARTESIAN_POINT('Ctrl Pts',(-11.3760874300001,15.2,-0.654746780000015));
#265136=CARTESIAN_POINT('Ctrl Pts',(-11.3760874300001,11.6,-0.654746780000016));
#265137=CARTESIAN_POINT('Ctrl Pts',(-11.3793365610001,15.2,-0.656489306000014));
#265138=CARTESIAN_POINT('Ctrl Pts',(-11.3793365610001,11.6,-0.656489306000015));
#265139=CARTESIAN_POINT('Ctrl Pts',(-11.3825883450001,15.2,-0.658236472000016));
#265140=CARTESIAN_POINT('Ctrl Pts',(-11.3825883450001,11.6,-0.658236472000016));
#265141=CARTESIAN_POINT('Ctrl Pts',(-11.3858427730001,15.2,-0.659988280000015));
#265142=CARTESIAN_POINT('Ctrl Pts',(-11.3858427730001,11.6,-0.659988280000015));
#265143=CARTESIAN_POINT('Ctrl Pts',(-11.3890998350001,15.2,-0.661744730000016));
#265144=CARTESIAN_POINT('Ctrl Pts',(-11.3890998350001,11.6,-0.661744730000016));
#265145=CARTESIAN_POINT('Ctrl Pts',(-11.3923595230001,15.2,-0.663505825000015));
#265146=CARTESIAN_POINT('Ctrl Pts',(-11.3923595230001,11.6,-0.663505825000015));
#265147=CARTESIAN_POINT('Ctrl Pts',(-11.3956218280001,15.2,-0.665271566000012));
#265148=CARTESIAN_POINT('Ctrl Pts',(-11.3956218280001,11.6,-0.665271566000012));
#265149=CARTESIAN_POINT('Ctrl Pts',(-11.3988867400001,15.2,-0.667041955000016));
#265150=CARTESIAN_POINT('Ctrl Pts',(-11.3988867400001,11.6,-0.667041955000017));
#265151=CARTESIAN_POINT('Ctrl Pts',(-11.4021542520001,15.2,-0.668816993000014));
#265152=CARTESIAN_POINT('Ctrl Pts',(-11.4021542520001,11.6,-0.668816993000015));
#265153=CARTESIAN_POINT('Ctrl Pts',(-11.4054243520001,15.2,-0.670596683000015));
#265154=CARTESIAN_POINT('Ctrl Pts',(-11.4054243520001,11.6,-0.670596683000016));
#265155=CARTESIAN_POINT('Ctrl Pts',(-11.4086970320001,15.2,-0.672381023000015));
#265156=CARTESIAN_POINT('Ctrl Pts',(-11.4086970320001,11.6,-0.672381023000015));
#265157=CARTESIAN_POINT('Ctrl Pts',(-11.4119722840001,15.2,-0.674170019000013));
#265158=CARTESIAN_POINT('Ctrl Pts',(-11.4119722840001,11.6,-0.674170019000014));
#265159=CARTESIAN_POINT('Ctrl Pts',(-11.4152500960001,15.2,-0.675963670000015));
#265160=CARTESIAN_POINT('Ctrl Pts',(-11.4152500960001,11.6,-0.675963670000015));
#265161=CARTESIAN_POINT('Ctrl Pts',(-11.4185304610001,15.2,-0.677761979000016));
#265162=CARTESIAN_POINT('Ctrl Pts',(-11.4185304610001,11.6,-0.677761979000016));
#265163=CARTESIAN_POINT('Ctrl Pts',(-11.4218133690001,15.2,-0.679564946000015));
#265164=CARTESIAN_POINT('Ctrl Pts',(-11.4218133690001,11.6,-0.679564946000016));
#265165=CARTESIAN_POINT('Ctrl Pts',(-11.4250988120001,15.2,-0.681372573000014));
#265166=CARTESIAN_POINT('Ctrl Pts',(-11.4250988120001,11.6,-0.681372573000015));
#265167=CARTESIAN_POINT('Ctrl Pts',(-11.4283867810001,15.2,-0.683184862000012));
#265168=CARTESIAN_POINT('Ctrl Pts',(-11.4283867810001,11.6,-0.683184862000013));
#265169=CARTESIAN_POINT('Ctrl Pts',(-11.4316772700001,15.2,-0.685001814000015));
#265170=CARTESIAN_POINT('Ctrl Pts',(-11.4316772700001,11.6,-0.685001814000015));
#265171=CARTESIAN_POINT('Ctrl Pts',(-11.4349702680001,15.2,-0.686823430000012));
#265172=CARTESIAN_POINT('Ctrl Pts',(-11.4349702680001,11.6,-0.686823430000012));
#265173=CARTESIAN_POINT('Ctrl Pts',(-11.4382657700001,15.2,-0.688649711000018));
#265174=CARTESIAN_POINT('Ctrl Pts',(-11.4382657700001,11.6,-0.688649711000018));
#265175=CARTESIAN_POINT('Ctrl Pts',(-11.4415637630001,15.2,-0.690480659000015));
#265176=CARTESIAN_POINT('Ctrl Pts',(-11.4415637630001,11.6,-0.690480659000015));
#265177=CARTESIAN_POINT('Ctrl Pts',(-11.4448642400001,15.2,-0.692316276000016));
#265178=CARTESIAN_POINT('Ctrl Pts',(-11.4448642400001,11.6,-0.692316276000016));
#265179=CARTESIAN_POINT('Ctrl Pts',(-11.4481671870001,15.2,-0.694156565000017));
#265180=CARTESIAN_POINT('Ctrl Pts',(-11.4481671870001,11.6,-0.694156565000017));
#265181=CARTESIAN_POINT('Ctrl Pts',(-11.4514725950001,15.2,-0.696001525000014));
#265182=CARTESIAN_POINT('Ctrl Pts',(-11.4514725950001,11.6,-0.696001525000014));
#265183=CARTESIAN_POINT('Ctrl Pts',(-11.4547804530001,15.2,-0.697851159000016));
#265184=CARTESIAN_POINT('Ctrl Pts',(-11.4547804530001,11.6,-0.697851159000016));
#265185=CARTESIAN_POINT('Ctrl Pts',(-11.4580907510001,15.2,-0.699705470000014));
#265186=CARTESIAN_POINT('Ctrl Pts',(-11.4580907510001,11.6,-0.699705470000014));
#265187=CARTESIAN_POINT('Ctrl Pts',(-11.4614034810001,15.2,-0.701564457000017));
#265188=CARTESIAN_POINT('Ctrl Pts',(-11.4614034810001,11.6,-0.701564457000017));
#265189=CARTESIAN_POINT('Ctrl Pts',(-11.4647186380001,15.2,-0.703428121000016));
#265190=CARTESIAN_POINT('Ctrl Pts',(-11.4647186380001,11.6,-0.703428121000016));
#265191=CARTESIAN_POINT('Ctrl Pts',(-11.4680362160001,15.2,-0.705296464000016));
#265192=CARTESIAN_POINT('Ctrl Pts',(-11.4680362160001,11.6,-0.705296464000016));
#265193=CARTESIAN_POINT('Ctrl Pts',(-11.4713562160001,15.2,-0.707169486000012));
#265194=CARTESIAN_POINT('Ctrl Pts',(-11.4713562160001,11.6,-0.707169486000013));
#265195=CARTESIAN_POINT('Ctrl Pts',(-11.4740141490001,15.2,-0.708671646000014));
#265196=CARTESIAN_POINT('Ctrl Pts',(-11.4740141490001,11.6,-0.708671646000015));
#265197=CARTESIAN_POINT('Ctrl Pts',(-11.4760086880001,15.2,-0.709800372000018));
#265198=CARTESIAN_POINT('Ctrl Pts',(-11.4760086880001,11.6,-0.709800372000018));
#265199=CARTESIAN_POINT('Ctrl Pts',(-11.4773388640001,15.2,-0.710553791000015));
#265200=CARTESIAN_POINT('Ctrl Pts',(-11.4773388640001,11.6,-0.710553791000015));
#265201=CARTESIAN_POINT('Ctrl Pts',(-11.4780040730001,15.2,-0.710930734000015));
#265202=CARTESIAN_POINT('Ctrl Pts',(-11.4780040730001,11.6,-0.710930734000015));
#265203=CARTESIAN_POINT('Ctrl Pts',(-10.3708900240001,15.2,-0.292001929000012));
#265204=CARTESIAN_POINT('Ctrl Pts',(-10.3710632460001,15.2,-0.292021795000017));
#265205=CARTESIAN_POINT('Ctrl Pts',(-10.3714157310001,15.2,-0.292062310000016));
#265206=CARTESIAN_POINT('Ctrl Pts',(-10.3719498000001,15.2,-0.292123961000015));
#265207=CARTESIAN_POINT('Ctrl Pts',(-10.3726691760001,15.2,-0.292207548000012));
#265208=CARTESIAN_POINT('Ctrl Pts',(-10.3735789750001,15.2,-0.292314181000015));
#265209=CARTESIAN_POINT('Ctrl Pts',(-10.3745034120001,15.2,-0.292423469000016));
#265210=CARTESIAN_POINT('Ctrl Pts',(-10.3754371840001,15.2,-0.292534812000014));
#265211=CARTESIAN_POINT('Ctrl Pts',(-10.3763802670001,15.2,-0.292648223000014));
#265212=CARTESIAN_POINT('Ctrl Pts',(-10.3773326270001,15.2,-0.292763718000018));
#265213=CARTESIAN_POINT('Ctrl Pts',(-10.3782942400001,15.2,-0.292881310000013));
#265214=CARTESIAN_POINT('Ctrl Pts',(-10.3792650740001,15.2,-0.293001015000014));
#265215=CARTESIAN_POINT('Ctrl Pts',(-10.3802451030001,15.2,-0.293122847000014));
#265216=CARTESIAN_POINT('Ctrl Pts',(-10.3812342970001,15.2,-0.293246820000017));
#265217=CARTESIAN_POINT('Ctrl Pts',(-10.3822326280001,15.2,-0.293372950000013));
#265218=CARTESIAN_POINT('Ctrl Pts',(-10.3832400690001,15.2,-0.293501248000014));
#265219=CARTESIAN_POINT('Ctrl Pts',(-10.3842565920001,15.2,-0.293631732000015));
#265220=CARTESIAN_POINT('Ctrl Pts',(-10.3852821680001,15.2,-0.293764413000015));
#265221=CARTESIAN_POINT('Ctrl Pts',(-10.3863167710001,15.2,-0.293899307000016));
#265222=CARTESIAN_POINT('Ctrl Pts',(-10.3873603720001,15.2,-0.294036427000015));
#265223=CARTESIAN_POINT('Ctrl Pts',(-10.3884129450001,15.2,-0.294175788000013));
#265224=CARTESIAN_POINT('Ctrl Pts',(-10.3894744620001,15.2,-0.294317401000015));
#265225=CARTESIAN_POINT('Ctrl Pts',(-10.3905448950001,15.2,-0.294461282000014));
#265226=CARTESIAN_POINT('Ctrl Pts',(-10.3916242180001,15.2,-0.294607444000015));
#265227=CARTESIAN_POINT('Ctrl Pts',(-10.3927124050001,15.2,-0.294755901000014));
#265228=CARTESIAN_POINT('Ctrl Pts',(-10.3938094280001,15.2,-0.294906666000014));
#265229=CARTESIAN_POINT('Ctrl Pts',(-10.3949152600001,15.2,-0.295059752000015));
#265230=CARTESIAN_POINT('Ctrl Pts',(-10.3960298750001,15.2,-0.295215173000014));
#265231=CARTESIAN_POINT('Ctrl Pts',(-10.3971532480001,15.2,-0.295372943000016));
#265232=CARTESIAN_POINT('Ctrl Pts',(-10.3982853500001,15.2,-0.295533072000014));
#265233=CARTESIAN_POINT('Ctrl Pts',(-10.3994261560001,15.2,-0.295695576000017));
#265234=CARTESIAN_POINT('Ctrl Pts',(-10.4005756420001,15.2,-0.295860468000013));
#265235=CARTESIAN_POINT('Ctrl Pts',(-10.4017337790001,15.2,-0.296027759000013));
#265236=CARTESIAN_POINT('Ctrl Pts',(-10.4029005420001,15.2,-0.296197463000016));
#265237=CARTESIAN_POINT('Ctrl Pts',(-10.4040759070001,15.2,-0.296369593000012));
#265238=CARTESIAN_POINT('Ctrl Pts',(-10.4052598460001,15.2,-0.296544162000014));
#265239=CARTESIAN_POINT('Ctrl Pts',(-10.4064523340001,15.2,-0.296721181000015));
#265240=CARTESIAN_POINT('Ctrl Pts',(-10.4076533470001,15.2,-0.296900665000015));
#265241=CARTESIAN_POINT('Ctrl Pts',(-10.4088628590001,15.2,-0.297082624000016));
#265242=CARTESIAN_POINT('Ctrl Pts',(-10.4100808450001,15.2,-0.297267072000014));
#265243=CARTESIAN_POINT('Ctrl Pts',(-10.4113072790001,15.2,-0.297454022000014));
#265244=CARTESIAN_POINT('Ctrl Pts',(-10.4125421370001,15.2,-0.297643484000014));
#265245=CARTESIAN_POINT('Ctrl Pts',(-10.4137853940001,15.2,-0.297835472000014));
#265246=CARTESIAN_POINT('Ctrl Pts',(-10.4150370250001,15.2,-0.298029998000011));
#265247=CARTESIAN_POINT('Ctrl Pts',(-10.4162970050001,15.2,-0.298227073000015));
#265248=CARTESIAN_POINT('Ctrl Pts',(-10.4175653100001,15.2,-0.298426711000013));
#265249=CARTESIAN_POINT('Ctrl Pts',(-10.4188419160001,15.2,-0.298628922000015));
#265250=CARTESIAN_POINT('Ctrl Pts',(-10.4201267970001,15.2,-0.298833719000013));
#265251=CARTESIAN_POINT('Ctrl Pts',(-10.4214199300001,15.2,-0.299041114000014));
#265252=CARTESIAN_POINT('Ctrl Pts',(-10.4227212920001,15.2,-0.299251118000012));
#265253=CARTESIAN_POINT('Ctrl Pts',(-10.4240308570001,15.2,-0.299463743000015));
#265254=CARTESIAN_POINT('Ctrl Pts',(-10.4253486020001,15.2,-0.299679001000013));
#265255=CARTESIAN_POINT('Ctrl Pts',(-10.4266745030001,15.2,-0.299896903000012));
#265256=CARTESIAN_POINT('Ctrl Pts',(-10.4280085350001,15.2,-0.300117461000013));
#265257=CARTESIAN_POINT('Ctrl Pts',(-10.4293506770001,15.2,-0.300340686000014));
#265258=CARTESIAN_POINT('Ctrl Pts',(-10.4307009030001,15.2,-0.300566590000013));
#265259=CARTESIAN_POINT('Ctrl Pts',(-10.4320591910001,15.2,-0.300795184000013));
#265260=CARTESIAN_POINT('Ctrl Pts',(-10.4334255170001,15.2,-0.301026479000015));
#265261=CARTESIAN_POINT('Ctrl Pts',(-10.4347998580001,15.2,-0.301260488000015));
#265262=CARTESIAN_POINT('Ctrl Pts',(-10.4361821910001,15.2,-0.301497219000013));
#265263=CARTESIAN_POINT('Ctrl Pts',(-10.4375724920001,15.2,-0.301736686000016));
#265264=CARTESIAN_POINT('Ctrl Pts',(-10.4389707380001,15.2,-0.301978898000015));
#265265=CARTESIAN_POINT('Ctrl Pts',(-10.4403769080001,15.2,-0.302223867000015));
#265266=CARTESIAN_POINT('Ctrl Pts',(-10.4417909780001,15.2,-0.302471605000014));
#265267=CARTESIAN_POINT('Ctrl Pts',(-10.4432129240001,15.2,-0.302722121000016));
#265268=CARTESIAN_POINT('Ctrl Pts',(-10.4446427250001,15.2,-0.302975426000014));
#265269=CARTESIAN_POINT('Ctrl Pts',(-10.4460803580001,15.2,-0.303231532000012));
#265270=CARTESIAN_POINT('Ctrl Pts',(-10.4475258000001,15.2,-0.303490448000012));
#265271=CARTESIAN_POINT('Ctrl Pts',(-10.4489790300001,15.2,-0.303752186000015));
#265272=CARTESIAN_POINT('Ctrl Pts',(-10.4504400240001,15.2,-0.304016756000016));
#265273=CARTESIAN_POINT('Ctrl Pts',(-10.4519087610001,15.2,-0.304284170000013));
#265274=CARTESIAN_POINT('Ctrl Pts',(-10.4533852190001,15.2,-0.304554436000015));
#265275=CARTESIAN_POINT('Ctrl Pts',(-10.4548693740001,15.2,-0.304827566000014));
#265276=CARTESIAN_POINT('Ctrl Pts',(-10.4563612070001,15.2,-0.305103570000016));
#265277=CARTESIAN_POINT('Ctrl Pts',(-10.4578606950001,15.2,-0.305382458000012));
#265278=CARTESIAN_POINT('Ctrl Pts',(-10.4593678150001,15.2,-0.305664241000017));
#265279=CARTESIAN_POINT('Ctrl Pts',(-10.4608825450001,15.2,-0.305948928000017));
#265280=CARTESIAN_POINT('Ctrl Pts',(-10.4624048670001,15.2,-0.306236531000015));
#265281=CARTESIAN_POINT('Ctrl Pts',(-10.4639347550001,15.2,-0.306527058000015));
#265282=CARTESIAN_POINT('Ctrl Pts',(-10.4654721910001,15.2,-0.306820521000013));
#265283=CARTESIAN_POINT('Ctrl Pts',(-10.4670171510001,15.2,-0.307116929000015));
#265284=CARTESIAN_POINT('Ctrl Pts',(-10.4685696160001,15.2,-0.307416292000013));
#265285=CARTESIAN_POINT('Ctrl Pts',(-10.4701295620001,15.2,-0.307718619000017));
#265286=CARTESIAN_POINT('Ctrl Pts',(-10.4716969700001,15.2,-0.308023923000014));
#265287=CARTESIAN_POINT('Ctrl Pts',(-10.4732718190001,15.2,-0.308332210000017));
#265288=CARTESIAN_POINT('Ctrl Pts',(-10.4748540860001,15.2,-0.308643492000016));
#265289=CARTESIAN_POINT('Ctrl Pts',(-10.4764437530001,15.2,-0.308957777000014));
#265290=CARTESIAN_POINT('Ctrl Pts',(-10.4780407970001,15.2,-0.309275076000013));
#265291=CARTESIAN_POINT('Ctrl Pts',(-10.4796451980001,15.2,-0.309595399000013));
#265292=CARTESIAN_POINT('Ctrl Pts',(-10.4812569350001,15.2,-0.309918754000016));
#265293=CARTESIAN_POINT('Ctrl Pts',(-10.4828759870001,15.2,-0.310245152000017));
#265294=CARTESIAN_POINT('Ctrl Pts',(-10.4845023350001,15.2,-0.310574602000013));
#265295=CARTESIAN_POINT('Ctrl Pts',(-10.4861359570001,15.2,-0.310907114000014));
#265296=CARTESIAN_POINT('Ctrl Pts',(-10.4877768330001,15.2,-0.311242696000011));
#265297=CARTESIAN_POINT('Ctrl Pts',(-10.4894249420001,15.2,-0.311581357000015));
#265298=CARTESIAN_POINT('Ctrl Pts',(-10.4910802660001,15.2,-0.311923107000016));
#265299=CARTESIAN_POINT('Ctrl Pts',(-10.4927427830001,15.2,-0.312267956000016));
#265300=CARTESIAN_POINT('Ctrl Pts',(-10.4944124730001,15.2,-0.312615913000016));
#265301=CARTESIAN_POINT('Ctrl Pts',(-10.4960893160001,15.2,-0.312966987000016));
#265302=CARTESIAN_POINT('Ctrl Pts',(-10.4977732930001,15.2,-0.313321185000017));
#265303=CARTESIAN_POINT('Ctrl Pts',(-10.4994643820001,15.2,-0.313678519000016));
#265304=CARTESIAN_POINT('Ctrl Pts',(-10.5011625650001,15.2,-0.314038997000012));
#265305=CARTESIAN_POINT('Ctrl Pts',(-10.5028678220001,15.2,-0.314402627000017));
#265306=CARTESIAN_POINT('Ctrl Pts',(-10.5049225963254,15.2,-0.314842777384019));
#265307=CARTESIAN_POINT('Ctrl Pts',(-10.5069879188374,15.2,-0.315287684308014));
#265308=CARTESIAN_POINT('Ctrl Pts',(-10.5090637571627,15.2,-0.315737363692019));
#265309=CARTESIAN_POINT('Ctrl Pts',(-10.5111500674852,15.2,-0.316191834574724));
#265310=CARTESIAN_POINT('Ctrl Pts',(-10.5132468120001,15.2,-0.316651113000015));
#265311=CARTESIAN_POINT('Ctrl Pts',(-10.5150010370001,15.2,-0.317037060000014));
#265312=CARTESIAN_POINT('Ctrl Pts',(-10.5167621800001,15.2,-0.317426229000013));
#265313=CARTESIAN_POINT('Ctrl Pts',(-10.5185302210001,15.2,-0.317818628000013));
#265314=CARTESIAN_POINT('Ctrl Pts',(-10.5203051430001,15.2,-0.318214269000014));
#265315=CARTESIAN_POINT('Ctrl Pts',(-10.5220869250001,15.2,-0.318613157000014));
#265316=CARTESIAN_POINT('Ctrl Pts',(-10.5238755480001,15.2,-0.319015302000012));
#265317=CARTESIAN_POINT('Ctrl Pts',(-10.5256709940001,15.2,-0.319420713000014));
#265318=CARTESIAN_POINT('Ctrl Pts',(-10.5274732440001,15.2,-0.319829396000015));
#265319=CARTESIAN_POINT('Ctrl Pts',(-10.5292822790001,15.2,-0.320241361000013));
#265320=CARTESIAN_POINT('Ctrl Pts',(-10.5310980810001,15.2,-0.320656616000012));
#265321=CARTESIAN_POINT('Ctrl Pts',(-10.5329206290001,15.2,-0.321075169000018));
#265322=CARTESIAN_POINT('Ctrl Pts',(-10.5347499080001,15.2,-0.321497029000017));
#265323=CARTESIAN_POINT('Ctrl Pts',(-10.5365858960001,15.2,-0.321922203000016));
#265324=CARTESIAN_POINT('Ctrl Pts',(-10.5384285770001,15.2,-0.322350700000014));
#265325=CARTESIAN_POINT('Ctrl Pts',(-10.5402779310001,15.2,-0.322782527000012));
#265326=CARTESIAN_POINT('Ctrl Pts',(-10.5421339400001,15.2,-0.323217694000015));
#265327=CARTESIAN_POINT('Ctrl Pts',(-10.5439965860001,15.2,-0.323656207000016));
#265328=CARTESIAN_POINT('Ctrl Pts',(-10.5458658520001,15.2,-0.324098074000014));
#265329=CARTESIAN_POINT('Ctrl Pts',(-10.5477417170001,15.2,-0.324543305000016));
#265330=CARTESIAN_POINT('Ctrl Pts',(-10.5496241650001,15.2,-0.324991905000012));
#265331=CARTESIAN_POINT('Ctrl Pts',(-10.5515131770001,15.2,-0.325443883000016));
#265332=CARTESIAN_POINT('Ctrl Pts',(-10.5534087350001,15.2,-0.325899248000017));
#265333=CARTESIAN_POINT('Ctrl Pts',(-10.5553108210001,15.2,-0.326358007000014));
#265334=CARTESIAN_POINT('Ctrl Pts',(-10.5572194180001,15.2,-0.326820167000013));
#265335=CARTESIAN_POINT('Ctrl Pts',(-10.5591345070001,15.2,-0.327285736000014));
#265336=CARTESIAN_POINT('Ctrl Pts',(-10.5610560710001,15.2,-0.327754722000013));
#265337=CARTESIAN_POINT('Ctrl Pts',(-10.5629840910001,15.2,-0.328227133000016));
#265338=CARTESIAN_POINT('Ctrl Pts',(-10.5649185510001,15.2,-0.328702975000015));
#265339=CARTESIAN_POINT('Ctrl Pts',(-10.5668594320001,15.2,-0.329182256000013));
#265340=CARTESIAN_POINT('Ctrl Pts',(-10.5688067180001,15.2,-0.329664985000013));
#265341=CARTESIAN_POINT('Ctrl Pts',(-10.5707603900001,15.2,-0.330151169000015));
#265342=CARTESIAN_POINT('Ctrl Pts',(-10.5727204310001,15.2,-0.330640814000014));
#265343=CARTESIAN_POINT('Ctrl Pts',(-10.5746868240001,15.2,-0.331133928000016));
#265344=CARTESIAN_POINT('Ctrl Pts',(-10.5766595510001,15.2,-0.331630519000012));
#265345=CARTESIAN_POINT('Ctrl Pts',(-10.5786385950001,15.2,-0.332130595000013));
#265346=CARTESIAN_POINT('Ctrl Pts',(-10.5806239380001,15.2,-0.332634161000014));
#265347=CARTESIAN_POINT('Ctrl Pts',(-10.5826155640001,15.2,-0.333141226000016));
#265348=CARTESIAN_POINT('Ctrl Pts',(-10.5846134550001,15.2,-0.333651796000014));
#265349=CARTESIAN_POINT('Ctrl Pts',(-10.5866175950001,15.2,-0.334165879000015));
#265350=CARTESIAN_POINT('Ctrl Pts',(-10.5886279650001,15.2,-0.334683483000013));
#265351=CARTESIAN_POINT('Ctrl Pts',(-10.5906445490001,15.2,-0.335204613000015));
#265352=CARTESIAN_POINT('Ctrl Pts',(-10.5926673320001,15.2,-0.335729278000017));
#265353=CARTESIAN_POINT('Ctrl Pts',(-10.5946962940001,15.2,-0.336257483000013));
#265354=CARTESIAN_POINT('Ctrl Pts',(-10.5967314190001,15.2,-0.336789237000015));
#265355=CARTESIAN_POINT('Ctrl Pts',(-10.5987726910001,15.2,-0.337324546000013));
#265356=CARTESIAN_POINT('Ctrl Pts',(-10.6008200940001,15.2,-0.337863418000013));
#265357=CARTESIAN_POINT('Ctrl Pts',(-10.6028736090001,15.2,-0.338405859000015));
#265358=CARTESIAN_POINT('Ctrl Pts',(-10.6049332210001,15.2,-0.338951874000015));
#265359=CARTESIAN_POINT('Ctrl Pts',(-10.6069989120001,15.2,-0.339501473000015));
#265360=CARTESIAN_POINT('Ctrl Pts',(-10.6090706680001,15.2,-0.340054662000018));
#265361=CARTESIAN_POINT('Ctrl Pts',(-10.6111484700001,15.2,-0.340611447000012));
#265362=CARTESIAN_POINT('Ctrl Pts',(-10.6132323020001,15.2,-0.341171835000011));
#265363=CARTESIAN_POINT('Ctrl Pts',(-10.6153221490001,15.2,-0.341735833000012));
#265364=CARTESIAN_POINT('Ctrl Pts',(-10.6174179920001,15.2,-0.342303448000014));
#265365=CARTESIAN_POINT('Ctrl Pts',(-10.6195198180001,15.2,-0.342874685000014));
#265366=CARTESIAN_POINT('Ctrl Pts',(-10.6216276080001,15.2,-0.343449552000017));
#265367=CARTESIAN_POINT('Ctrl Pts',(-10.6237413470001,15.2,-0.344028056000014));
#265368=CARTESIAN_POINT('Ctrl Pts',(-10.6258610180001,15.2,-0.344610202000015));
#265369=CARTESIAN_POINT('Ctrl Pts',(-10.6279866070001,15.2,-0.345195998000012));
#265370=CARTESIAN_POINT('Ctrl Pts',(-10.6301180950001,15.2,-0.345785450000013));
#265371=CARTESIAN_POINT('Ctrl Pts',(-10.6322554680001,15.2,-0.346378564000016));
#265372=CARTESIAN_POINT('Ctrl Pts',(-10.6343987090001,15.2,-0.346975347000011));
#265373=CARTESIAN_POINT('Ctrl Pts',(-10.6365478020001,15.2,-0.347575805000013));
#265374=CARTESIAN_POINT('Ctrl Pts',(-10.6387027320001,15.2,-0.348179945000013));
#265375=CARTESIAN_POINT('Ctrl Pts',(-10.6408634830001,15.2,-0.348787773000012));
#265376=CARTESIAN_POINT('Ctrl Pts',(-10.6430300390001,15.2,-0.349399295000015));
#265377=CARTESIAN_POINT('Ctrl Pts',(-10.6452023830001,15.2,-0.350014516000012));
#265378=CARTESIAN_POINT('Ctrl Pts',(-10.6473805010001,15.2,-0.350633446000015));
#265379=CARTESIAN_POINT('Ctrl Pts',(-10.6495643770001,15.2,-0.351256088000014));
#265380=CARTESIAN_POINT('Ctrl Pts',(-10.6517539940001,15.2,-0.351882449000014));
#265381=CARTESIAN_POINT('Ctrl Pts',(-10.6539493380001,15.2,-0.352512536000016));
#265382=CARTESIAN_POINT('Ctrl Pts',(-10.6561503920001,15.2,-0.353146354000016));
#265383=CARTESIAN_POINT('Ctrl Pts',(-10.6583571410001,15.2,-0.353783910000014));
#265384=CARTESIAN_POINT('Ctrl Pts',(-10.6605695710001,15.2,-0.354425210000016));
#265385=CARTESIAN_POINT('Ctrl Pts',(-10.6627876650001,15.2,-0.355070259000012));
#265386=CARTESIAN_POINT('Ctrl Pts',(-10.6650114070001,15.2,-0.355719063000013));
#265387=CARTESIAN_POINT('Ctrl Pts',(-10.6672407830001,15.2,-0.356371629000014));
#265388=CARTESIAN_POINT('Ctrl Pts',(-10.6694757780001,15.2,-0.357027964000016));
#265389=CARTESIAN_POINT('Ctrl Pts',(-10.6717163760001,15.2,-0.357688071000015));
#265390=CARTESIAN_POINT('Ctrl Pts',(-10.6739625620001,15.2,-0.358351959000016));
#265391=CARTESIAN_POINT('Ctrl Pts',(-10.6762143200001,15.2,-0.359019631000015));
#265392=CARTESIAN_POINT('Ctrl Pts',(-10.6784716350001,15.2,-0.359691096000017));
#265393=CARTESIAN_POINT('Ctrl Pts',(-10.6807344940001,15.2,-0.360366356000017));
#265394=CARTESIAN_POINT('Ctrl Pts',(-10.6830028780001,15.2,-0.361045420000017));
#265395=CARTESIAN_POINT('Ctrl Pts',(-10.6852767760001,15.2,-0.361728293000017));
#265396=CARTESIAN_POINT('Ctrl Pts',(-10.6875561710001,15.2,-0.362414981000012));
#265397=CARTESIAN_POINT('Ctrl Pts',(-10.6898410480001,15.2,-0.363105487000013));
#265398=CARTESIAN_POINT('Ctrl Pts',(-10.6921313930001,15.2,-0.363799821000015));
#265399=CARTESIAN_POINT('Ctrl Pts',(-10.6944271900001,15.2,-0.364497985000014));
#265400=CARTESIAN_POINT('Ctrl Pts',(-10.6967284250001,15.2,-0.365199987000011));
#265401=CARTESIAN_POINT('Ctrl Pts',(-10.6990350820001,15.2,-0.365905831000015));
#265402=CARTESIAN_POINT('Ctrl Pts',(-10.7018095613513,15.2,-0.366757461446432));
#265403=CARTESIAN_POINT('Ctrl Pts',(-10.7045921314508,15.2,-0.367614872815749));
#265404=CARTESIAN_POINT('Ctrl Pts',(-10.7073827605493,15.2,-0.368478077184284));
#265405=CARTESIAN_POINT('Ctrl Pts',(-10.7101814229016,15.2,-0.369347083631473));
#265406=CARTESIAN_POINT('Ctrl Pts',(-10.7129880860001,15.2,-0.370221904000014));
#265407=CARTESIAN_POINT('Ctrl Pts',(-10.7153322940001,15.2,-0.370954801000014));
#265408=CARTESIAN_POINT('Ctrl Pts',(-10.7176818070001,15.2,-0.371691587000011));
#265409=CARTESIAN_POINT('Ctrl Pts',(-10.7200366120001,15.2,-0.372432264000011));
#265410=CARTESIAN_POINT('Ctrl Pts',(-10.7223966940001,15.2,-0.373176838000013));
#265411=CARTESIAN_POINT('Ctrl Pts',(-10.7247620380001,15.2,-0.373925315000014));
#265412=CARTESIAN_POINT('Ctrl Pts',(-10.7271326310001,15.2,-0.374677700000015));
#265413=CARTESIAN_POINT('Ctrl Pts',(-10.7295084580001,15.2,-0.375433998000014));
#265414=CARTESIAN_POINT('Ctrl Pts',(-10.7318895040001,15.2,-0.376194215000014));
#265415=CARTESIAN_POINT('Ctrl Pts',(-10.7342757570001,15.2,-0.376958356000014));
#265416=CARTESIAN_POINT('Ctrl Pts',(-10.7366672000001,15.2,-0.377726425000016));
#265417=CARTESIAN_POINT('Ctrl Pts',(-10.7390638200001,15.2,-0.378498429000014));
#265418=CARTESIAN_POINT('Ctrl Pts',(-10.7414656040001,15.2,-0.379274372000014));
#265419=CARTESIAN_POINT('Ctrl Pts',(-10.7438725370001,15.2,-0.380054260000016));
#265420=CARTESIAN_POINT('Ctrl Pts',(-10.7462846040001,15.2,-0.380838098000016));
#265421=CARTESIAN_POINT('Ctrl Pts',(-10.7487017930001,15.2,-0.381625889000015));
#265422=CARTESIAN_POINT('Ctrl Pts',(-10.7511240870001,15.2,-0.382417641000017));
#265423=CARTESIAN_POINT('Ctrl Pts',(-10.7535514750001,15.2,-0.383213358000014));
#265424=CARTESIAN_POINT('Ctrl Pts',(-10.7559839420001,15.2,-0.384013044000016));
#265425=CARTESIAN_POINT('Ctrl Pts',(-10.7584214740001,15.2,-0.384816705000013));
#265426=CARTESIAN_POINT('Ctrl Pts',(-10.7608640580001,15.2,-0.385624345000015));
#265427=CARTESIAN_POINT('Ctrl Pts',(-10.7633116780001,15.2,-0.386435971000014));
#265428=CARTESIAN_POINT('Ctrl Pts',(-10.7657643230001,15.2,-0.387251586000015));
#265429=CARTESIAN_POINT('Ctrl Pts',(-10.7682219760001,15.2,-0.388071196000013));
#265430=CARTESIAN_POINT('Ctrl Pts',(-10.7706846260001,15.2,-0.388894805000017));
#265431=CARTESIAN_POINT('Ctrl Pts',(-10.7731522590001,15.2,-0.389722418000016));
#265432=CARTESIAN_POINT('Ctrl Pts',(-10.7756248610001,15.2,-0.390554041000013));
#265433=CARTESIAN_POINT('Ctrl Pts',(-10.7781024170001,15.2,-0.391389677000014));
#265434=CARTESIAN_POINT('Ctrl Pts',(-10.7805849160001,15.2,-0.392229332000014));
#265435=CARTESIAN_POINT('Ctrl Pts',(-10.7830723410001,15.2,-0.393073009000013));
#265436=CARTESIAN_POINT('Ctrl Pts',(-10.7855646820001,15.2,-0.393920716000018));
#265437=CARTESIAN_POINT('Ctrl Pts',(-10.7880619230001,15.2,-0.394772456000014));
#265438=CARTESIAN_POINT('Ctrl Pts',(-10.7905640520001,15.2,-0.395628232000016));
#265439=CARTESIAN_POINT('Ctrl Pts',(-10.7930710550001,15.2,-0.396488052000015));
#265440=CARTESIAN_POINT('Ctrl Pts',(-10.7955829180001,15.2,-0.397351917000015));
#265441=CARTESIAN_POINT('Ctrl Pts',(-10.7980996290001,15.2,-0.398219835000013));
#265442=CARTESIAN_POINT('Ctrl Pts',(-10.8006211740001,15.2,-0.399091809000014));
#265443=CARTESIAN_POINT('Ctrl Pts',(-10.8031475400001,15.2,-0.399967843000013));
#265444=CARTESIAN_POINT('Ctrl Pts',(-10.8056787130001,15.2,-0.400847944000016));
#265445=CARTESIAN_POINT('Ctrl Pts',(-10.8082146790001,15.2,-0.401732113000013));
#265446=CARTESIAN_POINT('Ctrl Pts',(-10.8107554270001,15.2,-0.402620357000014));
#265447=CARTESIAN_POINT('Ctrl Pts',(-10.8133009430001,15.2,-0.403512679000015));
#265448=CARTESIAN_POINT('Ctrl Pts',(-10.8158512130001,15.2,-0.404409086000013));
#265449=CARTESIAN_POINT('Ctrl Pts',(-10.8184062250001,15.2,-0.405309580000015));
#265450=CARTESIAN_POINT('Ctrl Pts',(-10.8209659650001,15.2,-0.406214166000014));
#265451=CARTESIAN_POINT('Ctrl Pts',(-10.8235304190001,15.2,-0.407122849000014));
#265452=CARTESIAN_POINT('Ctrl Pts',(-10.8260995770001,15.2,-0.408035633000012));
#265453=CARTESIAN_POINT('Ctrl Pts',(-10.8286734240001,15.2,-0.408952523000017));
#265454=CARTESIAN_POINT('Ctrl Pts',(-10.8312519470001,15.2,-0.409873522000015));
#265455=CARTESIAN_POINT('Ctrl Pts',(-10.8338351330001,15.2,-0.410798635000016));
#265456=CARTESIAN_POINT('Ctrl Pts',(-10.8364229690001,15.2,-0.411727867000016));
#265457=CARTESIAN_POINT('Ctrl Pts',(-10.8390154430001,15.2,-0.412661222000015));
#265458=CARTESIAN_POINT('Ctrl Pts',(-10.8416125420001,15.2,-0.413598703000013));
#265459=CARTESIAN_POINT('Ctrl Pts',(-10.8442142530001,15.2,-0.414540317000016));
#265460=CARTESIAN_POINT('Ctrl Pts',(-10.8468205630001,15.2,-0.415486065000015));
#265461=CARTESIAN_POINT('Ctrl Pts',(-10.8494314580001,15.2,-0.416435953000014));
#265462=CARTESIAN_POINT('Ctrl Pts',(-10.8520469280001,15.2,-0.417389985000014));
#265463=CARTESIAN_POINT('Ctrl Pts',(-10.8546669570001,15.2,-0.418348165000015));
#265464=CARTESIAN_POINT('Ctrl Pts',(-10.8572915350001,15.2,-0.419310498000014));
#265465=CARTESIAN_POINT('Ctrl Pts',(-10.8599206490001,15.2,-0.420276987000014));
#265466=CARTESIAN_POINT('Ctrl Pts',(-10.8625542860001,15.2,-0.421247636000013));
#265467=CARTESIAN_POINT('Ctrl Pts',(-10.8651924320001,15.2,-0.422222450000014));
#265468=CARTESIAN_POINT('Ctrl Pts',(-10.8678350770001,15.2,-0.423201432000013));
#265469=CARTESIAN_POINT('Ctrl Pts',(-10.8704822050001,15.2,-0.424184588000016));
#265470=CARTESIAN_POINT('Ctrl Pts',(-10.8731338070001,15.2,-0.425171920000014));
#265471=CARTESIAN_POINT('Ctrl Pts',(-10.8757898690001,15.2,-0.426163433000015));
#265472=CARTESIAN_POINT('Ctrl Pts',(-10.8784503780001,15.2,-0.427159131000017));
#265473=CARTESIAN_POINT('Ctrl Pts',(-10.8811153220001,15.2,-0.428159018000014));
#265474=CARTESIAN_POINT('Ctrl Pts',(-10.8837846900001,15.2,-0.429163097000016));
#265475=CARTESIAN_POINT('Ctrl Pts',(-10.8864584680001,15.2,-0.430171373000015));
#265476=CARTESIAN_POINT('Ctrl Pts',(-10.8891366430001,15.2,-0.431183850000014));
#265477=CARTESIAN_POINT('Ctrl Pts',(-10.8918192040001,15.2,-0.432200531000015));
#265478=CARTESIAN_POINT('Ctrl Pts',(-10.8945061380001,15.2,-0.433221421000014));
#265479=CARTESIAN_POINT('Ctrl Pts',(-10.8971974330001,15.2,-0.434246522000015));
#265480=CARTESIAN_POINT('Ctrl Pts',(-10.8998930780001,15.2,-0.435275840000013));
#265481=CARTESIAN_POINT('Ctrl Pts',(-10.9025930590001,15.2,-0.436309378000015));
#265482=CARTESIAN_POINT('Ctrl Pts',(-10.9052973640001,15.2,-0.437347141000015));
#265483=CARTESIAN_POINT('Ctrl Pts',(-10.9080059810001,15.2,-0.438389130000014));
#265484=CARTESIAN_POINT('Ctrl Pts',(-10.9107188990001,15.2,-0.439435350000017));
#265485=CARTESIAN_POINT('Ctrl Pts',(-10.9134361040001,15.2,-0.440485807000015));
#265486=CARTESIAN_POINT('Ctrl Pts',(-10.9161575860001,15.2,-0.441540501000013));
#265487=CARTESIAN_POINT('Ctrl Pts',(-10.9188833300001,15.2,-0.442599438000015));
#265488=CARTESIAN_POINT('Ctrl Pts',(-10.9216133270001,15.2,-0.443662622000014));
#265489=CARTESIAN_POINT('Ctrl Pts',(-10.9243475630001,15.2,-0.444730056000013));
#265490=CARTESIAN_POINT('Ctrl Pts',(-10.9270860270001,15.2,-0.445801743000014));
#265491=CARTESIAN_POINT('Ctrl Pts',(-10.9298287070001,15.2,-0.446877689000011));
#265492=CARTESIAN_POINT('Ctrl Pts',(-10.9325755900001,15.2,-0.447957894000015));
#265493=CARTESIAN_POINT('Ctrl Pts',(-10.9353266640001,15.2,-0.449042364000016));
#265494=CARTESIAN_POINT('Ctrl Pts',(-10.9380819200001,15.2,-0.450131103000011));
#265495=CARTESIAN_POINT('Ctrl Pts',(-10.9408413420001,15.2,-0.451224112000013));
#265496=CARTESIAN_POINT('Ctrl Pts',(-10.9436049220001,15.2,-0.452321397000013));
#265497=CARTESIAN_POINT('Ctrl Pts',(-10.9463726460001,15.2,-0.453422962000012));
#265498=CARTESIAN_POINT('Ctrl Pts',(-10.9491445020001,15.2,-0.454528810000014));
#265499=CARTESIAN_POINT('Ctrl Pts',(-10.9519204780001,15.2,-0.455638942000016));
#265500=CARTESIAN_POINT('Ctrl Pts',(-10.9547005640001,15.2,-0.456753364000013));
#265501=CARTESIAN_POINT('Ctrl Pts',(-10.9574847480001,15.2,-0.457872080000015));
#265502=CARTESIAN_POINT('Ctrl Pts',(-10.9602730170001,15.2,-0.458995091000016));
#265503=CARTESIAN_POINT('Ctrl Pts',(-10.9630653590001,15.2,-0.460122402000014));
#265504=CARTESIAN_POINT('Ctrl Pts',(-10.9658617640001,15.2,-0.461254017000012));
#265505=CARTESIAN_POINT('Ctrl Pts',(-10.9686622200001,15.2,-0.462389938000012));
#265506=CARTESIAN_POINT('Ctrl Pts',(-10.9714667150001,15.2,-0.463530170000013));
#265507=CARTESIAN_POINT('Ctrl Pts',(-10.9742752370001,15.2,-0.464674714000015));
#265508=CARTESIAN_POINT('Ctrl Pts',(-10.9770877740001,15.2,-0.465823575000015));
#265509=CARTESIAN_POINT('Ctrl Pts',(-10.9799043170001,15.2,-0.466976757000013));
#265510=CARTESIAN_POINT('Ctrl Pts',(-10.9827248520001,15.2,-0.468134263000017));
#265511=CARTESIAN_POINT('Ctrl Pts',(-10.9855493680001,15.2,-0.469296094000011));
#265512=CARTESIAN_POINT('Ctrl Pts',(-10.9883778540001,15.2,-0.470462257000013));
#265513=CARTESIAN_POINT('Ctrl Pts',(-10.9912102990001,15.2,-0.471632753000013));
#265514=CARTESIAN_POINT('Ctrl Pts',(-10.9940466900001,15.2,-0.472807585000012));
#265515=CARTESIAN_POINT('Ctrl Pts',(-10.9968870170001,15.2,-0.473986757000016));
#265516=CARTESIAN_POINT('Ctrl Pts',(-10.9997312680001,15.2,-0.475170273000014));
#265517=CARTESIAN_POINT('Ctrl Pts',(-11.0025794320001,15.2,-0.476358134000012));
#265518=CARTESIAN_POINT('Ctrl Pts',(-11.0054314970001,15.2,-0.477550346000015));
#265519=CARTESIAN_POINT('Ctrl Pts',(-11.0082874530001,15.2,-0.478746910000014));
#265520=CARTESIAN_POINT('Ctrl Pts',(-11.0111472870001,15.2,-0.479947831000014));
#265521=CARTESIAN_POINT('Ctrl Pts',(-11.0140109890001,15.2,-0.481153110000014));
#265522=CARTESIAN_POINT('Ctrl Pts',(-11.0168785470001,15.2,-0.482362752000016));
#265523=CARTESIAN_POINT('Ctrl Pts',(-11.0197499510001,15.2,-0.483576758000015));
#265524=CARTESIAN_POINT('Ctrl Pts',(-11.0226251880001,15.2,-0.484795134000016));
#265525=CARTESIAN_POINT('Ctrl Pts',(-11.0255042470001,15.2,-0.486017881000014));
#265526=CARTESIAN_POINT('Ctrl Pts',(-11.0283871190001,15.2,-0.487245003000014));
#265527=CARTESIAN_POINT('Ctrl Pts',(-11.0312737910001,15.2,-0.488476502000013));
#265528=CARTESIAN_POINT('Ctrl Pts',(-11.0341642530001,15.2,-0.489712383000014));
#265529=CARTESIAN_POINT('Ctrl Pts',(-11.0370584920001,15.2,-0.490952646000018));
#265530=CARTESIAN_POINT('Ctrl Pts',(-11.0399564980001,15.2,-0.492197297000012));
#265531=CARTESIAN_POINT('Ctrl Pts',(-11.0428582610001,15.2,-0.493446338000014));
#265532=CARTESIAN_POINT('Ctrl Pts',(-11.0457637680001,15.2,-0.494699772000011));
#265533=CARTESIAN_POINT('Ctrl Pts',(-11.0486730100001,15.2,-0.495957601000012));
#265534=CARTESIAN_POINT('Ctrl Pts',(-11.0515859750001,15.2,-0.497219830000013));
#265535=CARTESIAN_POINT('Ctrl Pts',(-11.0545026510001,15.2,-0.498486460000014));
#265536=CARTESIAN_POINT('Ctrl Pts',(-11.0574230290001,15.2,-0.499757494000015));
#265537=CARTESIAN_POINT('Ctrl Pts',(-11.0603470970001,15.2,-0.501032937000012));
#265538=CARTESIAN_POINT('Ctrl Pts',(-11.0632748440001,15.2,-0.502312789000015));
#265539=CARTESIAN_POINT('Ctrl Pts',(-11.0662062590001,15.2,-0.503597056000018));
#265540=CARTESIAN_POINT('Ctrl Pts',(-11.0691413320001,15.2,-0.504885738000014));
#265541=CARTESIAN_POINT('Ctrl Pts',(-11.0720800520001,15.2,-0.506178839000011));
#265542=CARTESIAN_POINT('Ctrl Pts',(-11.0750224080001,15.2,-0.507476362000014));
#265543=CARTESIAN_POINT('Ctrl Pts',(-11.0779683880001,15.2,-0.508778311000011));
#265544=CARTESIAN_POINT('Ctrl Pts',(-11.0809179820001,15.2,-0.510084687000014));
#265545=CARTESIAN_POINT('Ctrl Pts',(-11.0838711810001,15.2,-0.511395492000015));
#265546=CARTESIAN_POINT('Ctrl Pts',(-11.0868279720001,15.2,-0.512710732000015));
#265547=CARTESIAN_POINT('Ctrl Pts',(-11.0897883450001,15.2,-0.514030406000017));
#265548=CARTESIAN_POINT('Ctrl Pts',(-11.0927522890001,15.2,-0.515354521000013));
#265549=CARTESIAN_POINT('Ctrl Pts',(-11.0957197940001,15.2,-0.516683076000017));
#265550=CARTESIAN_POINT('Ctrl Pts',(-11.0986908480001,15.2,-0.518016075000016));
#265551=CARTESIAN_POINT('Ctrl Pts',(-11.1016654420001,15.2,-0.519353522000015));
#265552=CARTESIAN_POINT('Ctrl Pts',(-11.1046435640001,15.2,-0.520695418000017));
#265553=CARTESIAN_POINT('Ctrl Pts',(-11.1076252050001,15.2,-0.522041766000014));
#265554=CARTESIAN_POINT('Ctrl Pts',(-11.1106103520001,15.2,-0.523392569000016));
#265555=CARTESIAN_POINT('Ctrl Pts',(-11.1135989970001,15.2,-0.524747830000014));
#265556=CARTESIAN_POINT('Ctrl Pts',(-11.1165911290001,15.2,-0.526107550000017));
#265557=CARTESIAN_POINT('Ctrl Pts',(-11.1195867360001,15.2,-0.527471735000016));
#265558=CARTESIAN_POINT('Ctrl Pts',(-11.1225858080001,15.2,-0.528840384000016));
#265559=CARTESIAN_POINT('Ctrl Pts',(-11.1255883350001,15.2,-0.530213501000016));
#265560=CARTESIAN_POINT('Ctrl Pts',(-11.1285943060001,15.2,-0.531591090000014));
#265561=CARTESIAN_POINT('Ctrl Pts',(-11.1316037120001,15.2,-0.532973151000018));
#265562=CARTESIAN_POINT('Ctrl Pts',(-11.1346165400001,15.2,-0.534359689000015));
#265563=CARTESIAN_POINT('Ctrl Pts',(-11.1376327810001,15.2,-0.535750705000013));
#265564=CARTESIAN_POINT('Ctrl Pts',(-11.1406524250001,15.2,-0.537146200000014));
#265565=CARTESIAN_POINT('Ctrl Pts',(-11.1436754620001,15.2,-0.538546181000013));
#265566=CARTESIAN_POINT('Ctrl Pts',(-11.1467018790001,15.2,-0.539950647000014));
#265567=CARTESIAN_POINT('Ctrl Pts',(-11.1497316690001,15.2,-0.541359602000018));
#265568=CARTESIAN_POINT('Ctrl Pts',(-11.1527648200001,15.2,-0.542773047000011));
#265569=CARTESIAN_POINT('Ctrl Pts',(-11.1558013220001,15.2,-0.544190986000017));
#265570=CARTESIAN_POINT('Ctrl Pts',(-11.1588411640001,15.2,-0.545613421000013));
#265571=CARTESIAN_POINT('Ctrl Pts',(-11.1618843360001,15.2,-0.547040354000017));
#265572=CARTESIAN_POINT('Ctrl Pts',(-11.1649308290001,15.2,-0.548471788000011));
#265573=CARTESIAN_POINT('Ctrl Pts',(-11.1679806310001,15.2,-0.549907725000014));
#265574=CARTESIAN_POINT('Ctrl Pts',(-11.1710337330001,15.2,-0.551348168000012));
#265575=CARTESIAN_POINT('Ctrl Pts',(-11.1740901240001,15.2,-0.552793118000015));
#265576=CARTESIAN_POINT('Ctrl Pts',(-11.1771497950001,15.2,-0.554242580000013));
#265577=CARTESIAN_POINT('Ctrl Pts',(-11.1802127340001,15.2,-0.555696554000011));
#265578=CARTESIAN_POINT('Ctrl Pts',(-11.1832789320001,15.2,-0.557155042000015));
#265579=CARTESIAN_POINT('Ctrl Pts',(-11.1863483800001,15.2,-0.558618049000015));
#265580=CARTESIAN_POINT('Ctrl Pts',(-11.1894210660001,15.2,-0.560085575000016));
#265581=CARTESIAN_POINT('Ctrl Pts',(-11.1924969800001,15.2,-0.561557623000013));
#265582=CARTESIAN_POINT('Ctrl Pts',(-11.1955761130001,15.2,-0.563034196000016));
#265583=CARTESIAN_POINT('Ctrl Pts',(-11.1986584540001,15.2,-0.564515295000017));
#265584=CARTESIAN_POINT('Ctrl Pts',(-11.2017439940001,15.2,-0.566000924000014));
#265585=CARTESIAN_POINT('Ctrl Pts',(-11.2048327210001,15.2,-0.567491084000018));
#265586=CARTESIAN_POINT('Ctrl Pts',(-11.2079246280001,15.2,-0.568985776000015));
#265587=CARTESIAN_POINT('Ctrl Pts',(-11.2110197020001,15.2,-0.570485006000014));
#265588=CARTESIAN_POINT('Ctrl Pts',(-11.2141179350001,15.2,-0.571988772000012));
#265589=CARTESIAN_POINT('Ctrl Pts',(-11.2172193170001,15.2,-0.573497079000016));
#265590=CARTESIAN_POINT('Ctrl Pts',(-11.2203238380001,15.2,-0.575009928000014));
#265591=CARTESIAN_POINT('Ctrl Pts',(-11.2234314850001,15.2,-0.576527323000011));
#265592=CARTESIAN_POINT('Ctrl Pts',(-11.2265422530001,15.2,-0.578049263000011));
#265593=CARTESIAN_POINT('Ctrl Pts',(-11.2296561290001,15.2,-0.579575753000015));
#265594=CARTESIAN_POINT('Ctrl Pts',(-11.2327731030001,15.2,-0.581106794000017));
#265595=CARTESIAN_POINT('Ctrl Pts',(-11.2358931670001,15.2,-0.582642387000014));
#265596=CARTESIAN_POINT('Ctrl Pts',(-11.2390163100001,15.2,-0.584182538000011));
#265597=CARTESIAN_POINT('Ctrl Pts',(-11.2421425230001,15.2,-0.585727245000012));
#265598=CARTESIAN_POINT('Ctrl Pts',(-11.2452717950001,15.2,-0.587276511000017));
#265599=CARTESIAN_POINT('Ctrl Pts',(-11.2484041180001,15.2,-0.588830340000013));
#265600=CARTESIAN_POINT('Ctrl Pts',(-11.2515394790001,15.2,-0.590388732000013));
#265601=CARTESIAN_POINT('Ctrl Pts',(-11.2546778710001,15.2,-0.591951690000014));
#265602=CARTESIAN_POINT('Ctrl Pts',(-11.2578192840001,15.2,-0.593519216000011));
#265603=CARTESIAN_POINT('Ctrl Pts',(-11.2609637080001,15.2,-0.595091312000013));
#265604=CARTESIAN_POINT('Ctrl Pts',(-11.2641111320001,15.2,-0.596667981000016));
#265605=CARTESIAN_POINT('Ctrl Pts',(-11.2672615480001,15.2,-0.598249222000016));
#265606=CARTESIAN_POINT('Ctrl Pts',(-11.2704149460001,15.2,-0.599835041000016));
#265607=CARTESIAN_POINT('Ctrl Pts',(-11.2735713160001,15.2,-0.601425437000014));
#265608=CARTESIAN_POINT('Ctrl Pts',(-11.2767306480001,15.2,-0.603020414000017));
#265609=CARTESIAN_POINT('Ctrl Pts',(-11.2798929340001,15.2,-0.604619973000013));
#265610=CARTESIAN_POINT('Ctrl Pts',(-11.2830581620001,15.2,-0.606224115000016));
#265611=CARTESIAN_POINT('Ctrl Pts',(-11.2862263240001,15.2,-0.607832843000011));
#265612=CARTESIAN_POINT('Ctrl Pts',(-11.2893974100001,15.2,-0.609446160000013));
#265613=CARTESIAN_POINT('Ctrl Pts',(-11.2925714100001,15.2,-0.611064067000013));
#265614=CARTESIAN_POINT('Ctrl Pts',(-11.2957483150001,15.2,-0.612686565000011));
#265615=CARTESIAN_POINT('Ctrl Pts',(-11.2989281170001,15.2,-0.614313657000016));
#265616=CARTESIAN_POINT('Ctrl Pts',(-11.3021108030001,15.2,-0.615945345000015));
#265617=CARTESIAN_POINT('Ctrl Pts',(-11.3052963650001,15.2,-0.617581630000017));
#265618=CARTESIAN_POINT('Ctrl Pts',(-11.3084847960001,15.2,-0.619222515000013));
#265619=CARTESIAN_POINT('Ctrl Pts',(-11.3116760820001,15.2,-0.620868001000012));
#265620=CARTESIAN_POINT('Ctrl Pts',(-11.3148702170001,15.2,-0.622518091000015));
#265621=CARTESIAN_POINT('Ctrl Pts',(-11.3180671910001,15.2,-0.624172784000017));
#265622=CARTESIAN_POINT('Ctrl Pts',(-11.3212669940001,15.2,-0.625832085000013));
#265623=CARTESIAN_POINT('Ctrl Pts',(-11.3244696160001,15.2,-0.627495996000014));
#265624=CARTESIAN_POINT('Ctrl Pts',(-11.3276750490001,15.2,-0.629164515000014));
#265625=CARTESIAN_POINT('Ctrl Pts',(-11.3308832820001,15.2,-0.630837648000018));
#265626=CARTESIAN_POINT('Ctrl Pts',(-11.3340943080001,15.2,-0.632515395000013));
#265627=CARTESIAN_POINT('Ctrl Pts',(-11.3373081150001,15.2,-0.634197758000017));
#265628=CARTESIAN_POINT('Ctrl Pts',(-11.3405246950001,15.2,-0.635884737000012));
#265629=CARTESIAN_POINT('Ctrl Pts',(-11.3437440390001,15.2,-0.637576336000016));
#265630=CARTESIAN_POINT('Ctrl Pts',(-11.3469661360001,15.2,-0.639272557000012));
#265631=CARTESIAN_POINT('Ctrl Pts',(-11.3501909790001,15.2,-0.640973401000018));
#265632=CARTESIAN_POINT('Ctrl Pts',(-11.3534185570001,15.2,-0.642678869000015));
#265633=CARTESIAN_POINT('Ctrl Pts',(-11.3566488620001,15.2,-0.644388964000013));
#265634=CARTESIAN_POINT('Ctrl Pts',(-11.3598818840001,15.2,-0.646103687000017));
#265635=CARTESIAN_POINT('Ctrl Pts',(-11.3631176140001,15.2,-0.647823039000013));
#265636=CARTESIAN_POINT('Ctrl Pts',(-11.3663560430001,15.2,-0.649547023000014));
#265637=CARTESIAN_POINT('Ctrl Pts',(-11.3695971620001,15.2,-0.651275639000013));
#265638=CARTESIAN_POINT('Ctrl Pts',(-11.3728409600001,15.2,-0.653008892000013));
#265639=CARTESIAN_POINT('Ctrl Pts',(-11.3760874300001,15.2,-0.654746780000015));
#265640=CARTESIAN_POINT('Ctrl Pts',(-11.3793365610001,15.2,-0.656489306000014));
#265641=CARTESIAN_POINT('Ctrl Pts',(-11.3825883450001,15.2,-0.658236472000016));
#265642=CARTESIAN_POINT('Ctrl Pts',(-11.3858427730001,15.2,-0.659988280000015));
#265643=CARTESIAN_POINT('Ctrl Pts',(-11.3890998350001,15.2,-0.661744730000016));
#265644=CARTESIAN_POINT('Ctrl Pts',(-11.3923595230001,15.2,-0.663505825000015));
#265645=CARTESIAN_POINT('Ctrl Pts',(-11.3956218280001,15.2,-0.665271566000012));
#265646=CARTESIAN_POINT('Ctrl Pts',(-11.3988867400001,15.2,-0.667041955000016));
#265647=CARTESIAN_POINT('Ctrl Pts',(-11.4021542520001,15.2,-0.668816993000014));
#265648=CARTESIAN_POINT('Ctrl Pts',(-11.4054243520001,15.2,-0.670596683000015));
#265649=CARTESIAN_POINT('Ctrl Pts',(-11.4086970320001,15.2,-0.672381023000015));
#265650=CARTESIAN_POINT('Ctrl Pts',(-11.4119722840001,15.2,-0.674170019000013));
#265651=CARTESIAN_POINT('Ctrl Pts',(-11.4152500960001,15.2,-0.675963670000015));
#265652=CARTESIAN_POINT('Ctrl Pts',(-11.4185304610001,15.2,-0.677761979000016));
#265653=CARTESIAN_POINT('Ctrl Pts',(-11.4218133690001,15.2,-0.679564946000015));
#265654=CARTESIAN_POINT('Ctrl Pts',(-11.4250988120001,15.2,-0.681372573000014));
#265655=CARTESIAN_POINT('Ctrl Pts',(-11.4283867810001,15.2,-0.683184862000012));
#265656=CARTESIAN_POINT('Ctrl Pts',(-11.4316772700001,15.2,-0.685001814000015));
#265657=CARTESIAN_POINT('Ctrl Pts',(-11.4349702680001,15.2,-0.686823430000012));
#265658=CARTESIAN_POINT('Ctrl Pts',(-11.4382657700001,15.2,-0.688649711000018));
#265659=CARTESIAN_POINT('Ctrl Pts',(-11.4415637630001,15.2,-0.690480659000015));
#265660=CARTESIAN_POINT('Ctrl Pts',(-11.4448642400001,15.2,-0.692316276000016));
#265661=CARTESIAN_POINT('Ctrl Pts',(-11.4481671870001,15.2,-0.694156565000017));
#265662=CARTESIAN_POINT('Ctrl Pts',(-11.4514725950001,15.2,-0.696001525000014));
#265663=CARTESIAN_POINT('Ctrl Pts',(-11.4547804530001,15.2,-0.697851159000016));
#265664=CARTESIAN_POINT('Ctrl Pts',(-11.4580907510001,15.2,-0.699705470000014));
#265665=CARTESIAN_POINT('Ctrl Pts',(-11.4614034810001,15.2,-0.701564457000017));
#265666=CARTESIAN_POINT('Ctrl Pts',(-11.4647186380001,15.2,-0.703428121000016));
#265667=CARTESIAN_POINT('Ctrl Pts',(-11.4680362160001,15.2,-0.705296464000016));
#265668=CARTESIAN_POINT('Ctrl Pts',(-11.4713562160001,15.2,-0.707169486000012));
#265669=CARTESIAN_POINT('Ctrl Pts',(-11.4740141490001,15.2,-0.708671646000014));
#265670=CARTESIAN_POINT('Ctrl Pts',(-11.4760086880001,15.2,-0.709800372000018));
#265671=CARTESIAN_POINT('Ctrl Pts',(-11.4773388640001,15.2,-0.710553791000015));
#265672=CARTESIAN_POINT('Ctrl Pts',(-11.4780040730001,15.2,-0.710930734000015));
#265673=CARTESIAN_POINT('Ctrl Pts',(-10.3708900240001,12.2,-0.292001929000012));
#265674=CARTESIAN_POINT('Ctrl Pts',(-10.3710632460001,12.2,-0.292021795000017));
#265675=CARTESIAN_POINT('Ctrl Pts',(-10.3714157310001,12.2,-0.292062310000016));
#265676=CARTESIAN_POINT('Ctrl Pts',(-10.3719498000001,12.2,-0.292123961000015));
#265677=CARTESIAN_POINT('Ctrl Pts',(-10.3726691760001,12.2,-0.292207548000012));
#265678=CARTESIAN_POINT('Ctrl Pts',(-10.3735789750001,12.2,-0.292314181000015));
#265679=CARTESIAN_POINT('Ctrl Pts',(-10.3745034120001,12.2,-0.292423469000016));
#265680=CARTESIAN_POINT('Ctrl Pts',(-10.3754371840001,12.2,-0.292534812000014));
#265681=CARTESIAN_POINT('Ctrl Pts',(-10.3763802670001,12.2,-0.292648223000014));
#265682=CARTESIAN_POINT('Ctrl Pts',(-10.3773326270001,12.2,-0.292763718000018));
#265683=CARTESIAN_POINT('Ctrl Pts',(-10.3782942400001,12.2,-0.292881310000013));
#265684=CARTESIAN_POINT('Ctrl Pts',(-10.3792650740001,12.2,-0.293001015000014));
#265685=CARTESIAN_POINT('Ctrl Pts',(-10.3802451030001,12.2,-0.293122847000014));
#265686=CARTESIAN_POINT('Ctrl Pts',(-10.3812342970001,12.2,-0.293246820000017));
#265687=CARTESIAN_POINT('Ctrl Pts',(-10.3822326280001,12.2,-0.293372950000013));
#265688=CARTESIAN_POINT('Ctrl Pts',(-10.3832400690001,12.2,-0.293501248000014));
#265689=CARTESIAN_POINT('Ctrl Pts',(-10.3842565920001,12.2,-0.293631732000015));
#265690=CARTESIAN_POINT('Ctrl Pts',(-10.3852821680001,12.2,-0.293764413000015));
#265691=CARTESIAN_POINT('Ctrl Pts',(-10.3863167710001,12.2,-0.293899307000016));
#265692=CARTESIAN_POINT('Ctrl Pts',(-10.3873603720001,12.2,-0.294036427000015));
#265693=CARTESIAN_POINT('Ctrl Pts',(-10.3884129450001,12.2,-0.294175788000013));
#265694=CARTESIAN_POINT('Ctrl Pts',(-10.3894744620001,12.2,-0.294317401000015));
#265695=CARTESIAN_POINT('Ctrl Pts',(-10.3905448950001,12.2,-0.294461282000014));
#265696=CARTESIAN_POINT('Ctrl Pts',(-10.3916242180001,12.2,-0.294607444000015));
#265697=CARTESIAN_POINT('Ctrl Pts',(-10.3927124050001,12.2,-0.294755901000014));
#265698=CARTESIAN_POINT('Ctrl Pts',(-10.3938094280001,12.2,-0.294906666000014));
#265699=CARTESIAN_POINT('Ctrl Pts',(-10.3949152600001,12.2,-0.295059752000015));
#265700=CARTESIAN_POINT('Ctrl Pts',(-10.3960298750001,12.2,-0.295215173000014));
#265701=CARTESIAN_POINT('Ctrl Pts',(-10.3971532480001,12.2,-0.295372943000016));
#265702=CARTESIAN_POINT('Ctrl Pts',(-10.3982853500001,12.2,-0.295533072000014));
#265703=CARTESIAN_POINT('Ctrl Pts',(-10.3994261560001,12.2,-0.295695576000017));
#265704=CARTESIAN_POINT('Ctrl Pts',(-10.4005756420001,12.2,-0.295860468000013));
#265705=CARTESIAN_POINT('Ctrl Pts',(-10.4017337790001,12.2,-0.296027759000013));
#265706=CARTESIAN_POINT('Ctrl Pts',(-10.4029005420001,12.2,-0.296197463000016));
#265707=CARTESIAN_POINT('Ctrl Pts',(-10.4040759070001,12.2,-0.296369593000012));
#265708=CARTESIAN_POINT('Ctrl Pts',(-10.4052598460001,12.2,-0.296544162000014));
#265709=CARTESIAN_POINT('Ctrl Pts',(-10.4064523340001,12.2,-0.296721181000015));
#265710=CARTESIAN_POINT('Ctrl Pts',(-10.4076533470001,12.2,-0.296900665000015));
#265711=CARTESIAN_POINT('Ctrl Pts',(-10.4088628590001,12.2,-0.297082624000016));
#265712=CARTESIAN_POINT('Ctrl Pts',(-10.4100808450001,12.2,-0.297267072000014));
#265713=CARTESIAN_POINT('Ctrl Pts',(-10.4113072790001,12.2,-0.297454022000014));
#265714=CARTESIAN_POINT('Ctrl Pts',(-10.4125421370001,12.2,-0.297643484000014));
#265715=CARTESIAN_POINT('Ctrl Pts',(-10.4137853940001,12.2,-0.297835472000014));
#265716=CARTESIAN_POINT('Ctrl Pts',(-10.4150370250001,12.2,-0.298029998000011));
#265717=CARTESIAN_POINT('Ctrl Pts',(-10.4162970050001,12.2,-0.298227073000015));
#265718=CARTESIAN_POINT('Ctrl Pts',(-10.4175653100001,12.2,-0.298426711000013));
#265719=CARTESIAN_POINT('Ctrl Pts',(-10.4188419160001,12.2,-0.298628922000015));
#265720=CARTESIAN_POINT('Ctrl Pts',(-10.4201267970001,12.2,-0.298833719000013));
#265721=CARTESIAN_POINT('Ctrl Pts',(-10.4214199300001,12.2,-0.299041114000014));
#265722=CARTESIAN_POINT('Ctrl Pts',(-10.4227212920001,12.2,-0.299251118000012));
#265723=CARTESIAN_POINT('Ctrl Pts',(-10.4240308570001,12.2,-0.299463743000015));
#265724=CARTESIAN_POINT('Ctrl Pts',(-10.4253486020001,12.2,-0.299679001000013));
#265725=CARTESIAN_POINT('Ctrl Pts',(-10.4266745030001,12.2,-0.299896903000012));
#265726=CARTESIAN_POINT('Ctrl Pts',(-10.4280085350001,12.2,-0.300117461000013));
#265727=CARTESIAN_POINT('Ctrl Pts',(-10.4293506770001,12.2,-0.300340686000014));
#265728=CARTESIAN_POINT('Ctrl Pts',(-10.4307009030001,12.2,-0.300566590000013));
#265729=CARTESIAN_POINT('Ctrl Pts',(-10.4320591910001,12.2,-0.300795184000013));
#265730=CARTESIAN_POINT('Ctrl Pts',(-10.4334255170001,12.2,-0.301026479000015));
#265731=CARTESIAN_POINT('Ctrl Pts',(-10.4347998580001,12.2,-0.301260488000015));
#265732=CARTESIAN_POINT('Ctrl Pts',(-10.4361821910001,12.2,-0.301497219000013));
#265733=CARTESIAN_POINT('Ctrl Pts',(-10.4375724920001,12.2,-0.301736686000016));
#265734=CARTESIAN_POINT('Ctrl Pts',(-10.4389707380001,12.2,-0.301978898000015));
#265735=CARTESIAN_POINT('Ctrl Pts',(-10.4403769080001,12.2,-0.302223867000015));
#265736=CARTESIAN_POINT('Ctrl Pts',(-10.4417909780001,12.2,-0.302471605000014));
#265737=CARTESIAN_POINT('Ctrl Pts',(-10.4432129240001,12.2,-0.302722121000016));
#265738=CARTESIAN_POINT('Ctrl Pts',(-10.4446427250001,12.2,-0.302975426000014));
#265739=CARTESIAN_POINT('Ctrl Pts',(-10.4460803580001,12.2,-0.303231532000012));
#265740=CARTESIAN_POINT('Ctrl Pts',(-10.4475258000001,12.2,-0.303490448000012));
#265741=CARTESIAN_POINT('Ctrl Pts',(-10.4489790300001,12.2,-0.303752186000015));
#265742=CARTESIAN_POINT('Ctrl Pts',(-10.4504400240001,12.2,-0.304016756000016));
#265743=CARTESIAN_POINT('Ctrl Pts',(-10.4519087610001,12.2,-0.304284170000013));
#265744=CARTESIAN_POINT('Ctrl Pts',(-10.4533852190001,12.2,-0.304554436000015));
#265745=CARTESIAN_POINT('Ctrl Pts',(-10.4548693740001,12.2,-0.304827566000014));
#265746=CARTESIAN_POINT('Ctrl Pts',(-10.4563612070001,12.2,-0.305103570000016));
#265747=CARTESIAN_POINT('Ctrl Pts',(-10.4578606950001,12.2,-0.305382458000012));
#265748=CARTESIAN_POINT('Ctrl Pts',(-10.4593678150001,12.2,-0.305664241000017));
#265749=CARTESIAN_POINT('Ctrl Pts',(-10.4608825450001,12.2,-0.305948928000017));
#265750=CARTESIAN_POINT('Ctrl Pts',(-10.4624048670001,12.2,-0.306236531000015));
#265751=CARTESIAN_POINT('Ctrl Pts',(-10.4639347550001,12.2,-0.306527058000015));
#265752=CARTESIAN_POINT('Ctrl Pts',(-10.4654721910001,12.2,-0.306820521000013));
#265753=CARTESIAN_POINT('Ctrl Pts',(-10.4670171510001,12.2,-0.307116929000015));
#265754=CARTESIAN_POINT('Ctrl Pts',(-10.4685696160001,12.2,-0.307416292000013));
#265755=CARTESIAN_POINT('Ctrl Pts',(-10.4701295620001,12.2,-0.307718619000017));
#265756=CARTESIAN_POINT('Ctrl Pts',(-10.4716969700001,12.2,-0.308023923000014));
#265757=CARTESIAN_POINT('Ctrl Pts',(-10.4732718190001,12.2,-0.308332210000017));
#265758=CARTESIAN_POINT('Ctrl Pts',(-10.4748540860001,12.2,-0.308643492000016));
#265759=CARTESIAN_POINT('Ctrl Pts',(-10.4764437530001,12.2,-0.308957777000014));
#265760=CARTESIAN_POINT('Ctrl Pts',(-10.4780407970001,12.2,-0.309275076000013));
#265761=CARTESIAN_POINT('Ctrl Pts',(-10.4796451980001,12.2,-0.309595399000013));
#265762=CARTESIAN_POINT('Ctrl Pts',(-10.4812569350001,12.2,-0.309918754000016));
#265763=CARTESIAN_POINT('Ctrl Pts',(-10.4828759870001,12.2,-0.310245152000017));
#265764=CARTESIAN_POINT('Ctrl Pts',(-10.4845023350001,12.2,-0.310574602000013));
#265765=CARTESIAN_POINT('Ctrl Pts',(-10.4861359570001,12.2,-0.310907114000014));
#265766=CARTESIAN_POINT('Ctrl Pts',(-10.4877768330001,12.2,-0.311242696000011));
#265767=CARTESIAN_POINT('Ctrl Pts',(-10.4894249420001,12.2,-0.311581357000015));
#265768=CARTESIAN_POINT('Ctrl Pts',(-10.4910802660001,12.2,-0.311923107000016));
#265769=CARTESIAN_POINT('Ctrl Pts',(-10.4927427830001,12.2,-0.312267956000016));
#265770=CARTESIAN_POINT('Ctrl Pts',(-10.4944124730001,12.2,-0.312615913000016));
#265771=CARTESIAN_POINT('Ctrl Pts',(-10.4960893160001,12.2,-0.312966987000016));
#265772=CARTESIAN_POINT('Ctrl Pts',(-10.4977732930001,12.2,-0.313321185000017));
#265773=CARTESIAN_POINT('Ctrl Pts',(-10.4994643820001,12.2,-0.313678519000016));
#265774=CARTESIAN_POINT('Ctrl Pts',(-10.5011625650001,12.2,-0.314038997000012));
#265775=CARTESIAN_POINT('Ctrl Pts',(-10.5028678220001,12.2,-0.314402627000017));
#265776=CARTESIAN_POINT('Ctrl Pts',(-10.5049225963254,12.2,-0.314842777384019));
#265777=CARTESIAN_POINT('Ctrl Pts',(-10.5069879188374,12.2,-0.315287684308014));
#265778=CARTESIAN_POINT('Ctrl Pts',(-10.5090637571627,12.2,-0.315737363692019));
#265779=CARTESIAN_POINT('Ctrl Pts',(-10.5111500674852,12.2,-0.316191834574724));
#265780=CARTESIAN_POINT('Ctrl Pts',(-10.5132468120001,12.2,-0.316651113000015));
#265781=CARTESIAN_POINT('Ctrl Pts',(-10.5150010370001,12.2,-0.317037060000014));
#265782=CARTESIAN_POINT('Ctrl Pts',(-10.5167621800001,12.2,-0.317426229000013));
#265783=CARTESIAN_POINT('Ctrl Pts',(-10.5185302210001,12.2,-0.317818628000013));
#265784=CARTESIAN_POINT('Ctrl Pts',(-10.5203051430001,12.2,-0.318214269000014));
#265785=CARTESIAN_POINT('Ctrl Pts',(-10.5220869250001,12.2,-0.318613157000014));
#265786=CARTESIAN_POINT('Ctrl Pts',(-10.5238755480001,12.2,-0.319015302000012));
#265787=CARTESIAN_POINT('Ctrl Pts',(-10.5256709940001,12.2,-0.319420713000014));
#265788=CARTESIAN_POINT('Ctrl Pts',(-10.5274732440001,12.2,-0.319829396000015));
#265789=CARTESIAN_POINT('Ctrl Pts',(-10.5292822790001,12.2,-0.320241361000013));
#265790=CARTESIAN_POINT('Ctrl Pts',(-10.5310980810001,12.2,-0.320656616000012));
#265791=CARTESIAN_POINT('Ctrl Pts',(-10.5329206290001,12.2,-0.321075169000018));
#265792=CARTESIAN_POINT('Ctrl Pts',(-10.5347499080001,12.2,-0.321497029000017));
#265793=CARTESIAN_POINT('Ctrl Pts',(-10.5365858960001,12.2,-0.321922203000016));
#265794=CARTESIAN_POINT('Ctrl Pts',(-10.5384285770001,12.2,-0.322350700000014));
#265795=CARTESIAN_POINT('Ctrl Pts',(-10.5402779310001,12.2,-0.322782527000012));
#265796=CARTESIAN_POINT('Ctrl Pts',(-10.5421339400001,12.2,-0.323217694000015));
#265797=CARTESIAN_POINT('Ctrl Pts',(-10.5439965860001,12.2,-0.323656207000016));
#265798=CARTESIAN_POINT('Ctrl Pts',(-10.5458658520001,12.2,-0.324098074000014));
#265799=CARTESIAN_POINT('Ctrl Pts',(-10.5477417170001,12.2,-0.324543305000016));
#265800=CARTESIAN_POINT('Ctrl Pts',(-10.5496241650001,12.2,-0.324991905000012));
#265801=CARTESIAN_POINT('Ctrl Pts',(-10.5515131770001,12.2,-0.325443883000016));
#265802=CARTESIAN_POINT('Ctrl Pts',(-10.5534087350001,12.2,-0.325899248000017));
#265803=CARTESIAN_POINT('Ctrl Pts',(-10.5553108210001,12.2,-0.326358007000014));
#265804=CARTESIAN_POINT('Ctrl Pts',(-10.5572194180001,12.2,-0.326820167000013));
#265805=CARTESIAN_POINT('Ctrl Pts',(-10.5591345070001,12.2,-0.327285736000014));
#265806=CARTESIAN_POINT('Ctrl Pts',(-10.5610560710001,12.2,-0.327754722000013));
#265807=CARTESIAN_POINT('Ctrl Pts',(-10.5629840910001,12.2,-0.328227133000016));
#265808=CARTESIAN_POINT('Ctrl Pts',(-10.5649185510001,12.2,-0.328702975000015));
#265809=CARTESIAN_POINT('Ctrl Pts',(-10.5668594320001,12.2,-0.329182256000013));
#265810=CARTESIAN_POINT('Ctrl Pts',(-10.5688067180001,12.2,-0.329664985000013));
#265811=CARTESIAN_POINT('Ctrl Pts',(-10.5707603900001,12.2,-0.330151169000015));
#265812=CARTESIAN_POINT('Ctrl Pts',(-10.5727204310001,12.2,-0.330640814000014));
#265813=CARTESIAN_POINT('Ctrl Pts',(-10.5746868240001,12.2,-0.331133928000016));
#265814=CARTESIAN_POINT('Ctrl Pts',(-10.5766595510001,12.2,-0.331630519000012));
#265815=CARTESIAN_POINT('Ctrl Pts',(-10.5786385950001,12.2,-0.332130595000013));
#265816=CARTESIAN_POINT('Ctrl Pts',(-10.5806239380001,12.2,-0.332634161000014));
#265817=CARTESIAN_POINT('Ctrl Pts',(-10.5826155640001,12.2,-0.333141226000016));
#265818=CARTESIAN_POINT('Ctrl Pts',(-10.5846134550001,12.2,-0.333651796000014));
#265819=CARTESIAN_POINT('Ctrl Pts',(-10.5866175950001,12.2,-0.334165879000015));
#265820=CARTESIAN_POINT('Ctrl Pts',(-10.5886279650001,12.2,-0.334683483000013));
#265821=CARTESIAN_POINT('Ctrl Pts',(-10.5906445490001,12.2,-0.335204613000015));
#265822=CARTESIAN_POINT('Ctrl Pts',(-10.5926673320001,12.2,-0.335729278000017));
#265823=CARTESIAN_POINT('Ctrl Pts',(-10.5946962940001,12.2,-0.336257483000013));
#265824=CARTESIAN_POINT('Ctrl Pts',(-10.5967314190001,12.2,-0.336789237000015));
#265825=CARTESIAN_POINT('Ctrl Pts',(-10.5987726910001,12.2,-0.337324546000013));
#265826=CARTESIAN_POINT('Ctrl Pts',(-10.6008200940001,12.2,-0.337863418000013));
#265827=CARTESIAN_POINT('Ctrl Pts',(-10.6028736090001,12.2,-0.338405859000015));
#265828=CARTESIAN_POINT('Ctrl Pts',(-10.6049332210001,12.2,-0.338951874000015));
#265829=CARTESIAN_POINT('Ctrl Pts',(-10.6069989120001,12.2,-0.339501473000015));
#265830=CARTESIAN_POINT('Ctrl Pts',(-10.6090706680001,12.2,-0.340054662000018));
#265831=CARTESIAN_POINT('Ctrl Pts',(-10.6111484700001,12.2,-0.340611447000012));
#265832=CARTESIAN_POINT('Ctrl Pts',(-10.6132323020001,12.2,-0.341171835000011));
#265833=CARTESIAN_POINT('Ctrl Pts',(-10.6153221490001,12.2,-0.341735833000012));
#265834=CARTESIAN_POINT('Ctrl Pts',(-10.6174179920001,12.2,-0.342303448000014));
#265835=CARTESIAN_POINT('Ctrl Pts',(-10.6195198180001,12.2,-0.342874685000014));
#265836=CARTESIAN_POINT('Ctrl Pts',(-10.6216276080001,12.2,-0.343449552000017));
#265837=CARTESIAN_POINT('Ctrl Pts',(-10.6237413470001,12.2,-0.344028056000014));
#265838=CARTESIAN_POINT('Ctrl Pts',(-10.6258610180001,12.2,-0.344610202000015));
#265839=CARTESIAN_POINT('Ctrl Pts',(-10.6279866070001,12.2,-0.345195998000012));
#265840=CARTESIAN_POINT('Ctrl Pts',(-10.6301180950001,12.2,-0.345785450000013));
#265841=CARTESIAN_POINT('Ctrl Pts',(-10.6322554680001,12.2,-0.346378564000016));
#265842=CARTESIAN_POINT('Ctrl Pts',(-10.6343987090001,12.2,-0.346975347000011));
#265843=CARTESIAN_POINT('Ctrl Pts',(-10.6365478020001,12.2,-0.347575805000013));
#265844=CARTESIAN_POINT('Ctrl Pts',(-10.6387027320001,12.2,-0.348179945000013));
#265845=CARTESIAN_POINT('Ctrl Pts',(-10.6408634830001,12.2,-0.348787773000012));
#265846=CARTESIAN_POINT('Ctrl Pts',(-10.6430300390001,12.2,-0.349399295000015));
#265847=CARTESIAN_POINT('Ctrl Pts',(-10.6452023830001,12.2,-0.350014516000012));
#265848=CARTESIAN_POINT('Ctrl Pts',(-10.6473805010001,12.2,-0.350633446000015));
#265849=CARTESIAN_POINT('Ctrl Pts',(-10.6495643770001,12.2,-0.351256088000014));
#265850=CARTESIAN_POINT('Ctrl Pts',(-10.6517539940001,12.2,-0.351882449000014));
#265851=CARTESIAN_POINT('Ctrl Pts',(-10.6539493380001,12.2,-0.352512536000016));
#265852=CARTESIAN_POINT('Ctrl Pts',(-10.6561503920001,12.2,-0.353146354000016));
#265853=CARTESIAN_POINT('Ctrl Pts',(-10.6583571410001,12.2,-0.353783910000014));
#265854=CARTESIAN_POINT('Ctrl Pts',(-10.6605695710001,12.2,-0.354425210000016));
#265855=CARTESIAN_POINT('Ctrl Pts',(-10.6627876650001,12.2,-0.355070259000012));
#265856=CARTESIAN_POINT('Ctrl Pts',(-10.6650114070001,12.2,-0.355719063000013));
#265857=CARTESIAN_POINT('Ctrl Pts',(-10.6672407830001,12.2,-0.356371629000014));
#265858=CARTESIAN_POINT('Ctrl Pts',(-10.6694757780001,12.2,-0.357027964000016));
#265859=CARTESIAN_POINT('Ctrl Pts',(-10.6717163760001,12.2,-0.357688071000015));
#265860=CARTESIAN_POINT('Ctrl Pts',(-10.6739625620001,12.2,-0.358351959000016));
#265861=CARTESIAN_POINT('Ctrl Pts',(-10.6762143200001,12.2,-0.359019631000015));
#265862=CARTESIAN_POINT('Ctrl Pts',(-10.6784716350001,12.2,-0.359691096000017));
#265863=CARTESIAN_POINT('Ctrl Pts',(-10.6807344940001,12.2,-0.360366356000017));
#265864=CARTESIAN_POINT('Ctrl Pts',(-10.6830028780001,12.2,-0.361045420000017));
#265865=CARTESIAN_POINT('Ctrl Pts',(-10.6852767760001,12.2,-0.361728293000017));
#265866=CARTESIAN_POINT('Ctrl Pts',(-10.6875561710001,12.2,-0.362414981000012));
#265867=CARTESIAN_POINT('Ctrl Pts',(-10.6898410480001,12.2,-0.363105487000013));
#265868=CARTESIAN_POINT('Ctrl Pts',(-10.6921313930001,12.2,-0.363799821000015));
#265869=CARTESIAN_POINT('Ctrl Pts',(-10.6944271900001,12.2,-0.364497985000014));
#265870=CARTESIAN_POINT('Ctrl Pts',(-10.6967284250001,12.2,-0.365199987000011));
#265871=CARTESIAN_POINT('Ctrl Pts',(-10.6990350820001,12.2,-0.365905831000015));
#265872=CARTESIAN_POINT('Ctrl Pts',(-10.7018095613513,12.2,-0.366757461446432));
#265873=CARTESIAN_POINT('Ctrl Pts',(-10.7045921314508,12.2,-0.367614872815749));
#265874=CARTESIAN_POINT('Ctrl Pts',(-10.7073827605493,12.2,-0.368478077184284));
#265875=CARTESIAN_POINT('Ctrl Pts',(-10.7101814229016,12.2,-0.369347083631473));
#265876=CARTESIAN_POINT('Ctrl Pts',(-10.7129880860001,12.2,-0.370221904000014));
#265877=CARTESIAN_POINT('Ctrl Pts',(-10.7153322940001,12.2,-0.370954801000014));
#265878=CARTESIAN_POINT('Ctrl Pts',(-10.7176818070001,12.2,-0.371691587000011));
#265879=CARTESIAN_POINT('Ctrl Pts',(-10.7200366120001,12.2,-0.372432264000011));
#265880=CARTESIAN_POINT('Ctrl Pts',(-10.7223966940001,12.2,-0.373176838000013));
#265881=CARTESIAN_POINT('Ctrl Pts',(-10.7247620380001,12.2,-0.373925315000014));
#265882=CARTESIAN_POINT('Ctrl Pts',(-10.7271326310001,12.2,-0.374677700000015));
#265883=CARTESIAN_POINT('Ctrl Pts',(-10.7295084580001,12.2,-0.375433998000014));
#265884=CARTESIAN_POINT('Ctrl Pts',(-10.7318895040001,12.2,-0.376194215000014));
#265885=CARTESIAN_POINT('Ctrl Pts',(-10.7342757570001,12.2,-0.376958356000014));
#265886=CARTESIAN_POINT('Ctrl Pts',(-10.7366672000001,12.2,-0.377726425000016));
#265887=CARTESIAN_POINT('Ctrl Pts',(-10.7390638200001,12.2,-0.378498429000014));
#265888=CARTESIAN_POINT('Ctrl Pts',(-10.7414656040001,12.2,-0.379274372000014));
#265889=CARTESIAN_POINT('Ctrl Pts',(-10.7438725370001,12.2,-0.380054260000016));
#265890=CARTESIAN_POINT('Ctrl Pts',(-10.7462846040001,12.2,-0.380838098000016));
#265891=CARTESIAN_POINT('Ctrl Pts',(-10.7487017930001,12.2,-0.381625889000015));
#265892=CARTESIAN_POINT('Ctrl Pts',(-10.7511240870001,12.2,-0.382417641000017));
#265893=CARTESIAN_POINT('Ctrl Pts',(-10.7535514750001,12.2,-0.383213358000014));
#265894=CARTESIAN_POINT('Ctrl Pts',(-10.7559839420001,12.2,-0.384013044000016));
#265895=CARTESIAN_POINT('Ctrl Pts',(-10.7584214740001,12.2,-0.384816705000013));
#265896=CARTESIAN_POINT('Ctrl Pts',(-10.7608640580001,12.2,-0.385624345000015));
#265897=CARTESIAN_POINT('Ctrl Pts',(-10.7633116780001,12.2,-0.386435971000014));
#265898=CARTESIAN_POINT('Ctrl Pts',(-10.7657643230001,12.2,-0.387251586000015));
#265899=CARTESIAN_POINT('Ctrl Pts',(-10.7682219760001,12.2,-0.388071196000013));
#265900=CARTESIAN_POINT('Ctrl Pts',(-10.7706846260001,12.2,-0.388894805000017));
#265901=CARTESIAN_POINT('Ctrl Pts',(-10.7731522590001,12.2,-0.389722418000016));
#265902=CARTESIAN_POINT('Ctrl Pts',(-10.7756248610001,12.2,-0.390554041000013));
#265903=CARTESIAN_POINT('Ctrl Pts',(-10.7781024170001,12.2,-0.391389677000014));
#265904=CARTESIAN_POINT('Ctrl Pts',(-10.7805849160001,12.2,-0.392229332000014));
#265905=CARTESIAN_POINT('Ctrl Pts',(-10.7830723410001,12.2,-0.393073009000013));
#265906=CARTESIAN_POINT('Ctrl Pts',(-10.7855646820001,12.2,-0.393920716000018));
#265907=CARTESIAN_POINT('Ctrl Pts',(-10.7880619230001,12.2,-0.394772456000014));
#265908=CARTESIAN_POINT('Ctrl Pts',(-10.7905640520001,12.2,-0.395628232000016));
#265909=CARTESIAN_POINT('Ctrl Pts',(-10.7930710550001,12.2,-0.396488052000015));
#265910=CARTESIAN_POINT('Ctrl Pts',(-10.7955829180001,12.2,-0.397351917000015));
#265911=CARTESIAN_POINT('Ctrl Pts',(-10.7980996290001,12.2,-0.398219835000013));
#265912=CARTESIAN_POINT('Ctrl Pts',(-10.8006211740001,12.2,-0.399091809000014));
#265913=CARTESIAN_POINT('Ctrl Pts',(-10.8031475400001,12.2,-0.399967843000013));
#265914=CARTESIAN_POINT('Ctrl Pts',(-10.8056787130001,12.2,-0.400847944000016));
#265915=CARTESIAN_POINT('Ctrl Pts',(-10.8082146790001,12.2,-0.401732113000013));
#265916=CARTESIAN_POINT('Ctrl Pts',(-10.8107554270001,12.2,-0.402620357000014));
#265917=CARTESIAN_POINT('Ctrl Pts',(-10.8133009430001,12.2,-0.403512679000015));
#265918=CARTESIAN_POINT('Ctrl Pts',(-10.8158512130001,12.2,-0.404409086000013));
#265919=CARTESIAN_POINT('Ctrl Pts',(-10.8184062250001,12.2,-0.405309580000015));
#265920=CARTESIAN_POINT('Ctrl Pts',(-10.8209659650001,12.2,-0.406214166000014));
#265921=CARTESIAN_POINT('Ctrl Pts',(-10.8235304190001,12.2,-0.407122849000014));
#265922=CARTESIAN_POINT('Ctrl Pts',(-10.8260995770001,12.2,-0.408035633000012));
#265923=CARTESIAN_POINT('Ctrl Pts',(-10.8286734240001,12.2,-0.408952523000017));
#265924=CARTESIAN_POINT('Ctrl Pts',(-10.8312519470001,12.2,-0.409873522000015));
#265925=CARTESIAN_POINT('Ctrl Pts',(-10.8338351330001,12.2,-0.410798635000016));
#265926=CARTESIAN_POINT('Ctrl Pts',(-10.8364229690001,12.2,-0.411727867000016));
#265927=CARTESIAN_POINT('Ctrl Pts',(-10.8390154430001,12.2,-0.412661222000015));
#265928=CARTESIAN_POINT('Ctrl Pts',(-10.8416125420001,12.2,-0.413598703000013));
#265929=CARTESIAN_POINT('Ctrl Pts',(-10.8442142530001,12.2,-0.414540317000016));
#265930=CARTESIAN_POINT('Ctrl Pts',(-10.8468205630001,12.2,-0.415486065000015));
#265931=CARTESIAN_POINT('Ctrl Pts',(-10.8494314580001,12.2,-0.416435953000014));
#265932=CARTESIAN_POINT('Ctrl Pts',(-10.8520469280001,12.2,-0.417389985000014));
#265933=CARTESIAN_POINT('Ctrl Pts',(-10.8546669570001,12.2,-0.418348165000015));
#265934=CARTESIAN_POINT('Ctrl Pts',(-10.8572915350001,12.2,-0.419310498000014));
#265935=CARTESIAN_POINT('Ctrl Pts',(-10.8599206490001,12.2,-0.420276987000014));
#265936=CARTESIAN_POINT('Ctrl Pts',(-10.8625542860001,12.2,-0.421247636000013));
#265937=CARTESIAN_POINT('Ctrl Pts',(-10.8651924320001,12.2,-0.422222450000014));
#265938=CARTESIAN_POINT('Ctrl Pts',(-10.8678350770001,12.2,-0.423201432000013));
#265939=CARTESIAN_POINT('Ctrl Pts',(-10.8704822050001,12.2,-0.424184588000016));
#265940=CARTESIAN_POINT('Ctrl Pts',(-10.8731338070001,12.2,-0.425171920000014));
#265941=CARTESIAN_POINT('Ctrl Pts',(-10.8757898690001,12.2,-0.426163433000015));
#265942=CARTESIAN_POINT('Ctrl Pts',(-10.8784503780001,12.2,-0.427159131000017));
#265943=CARTESIAN_POINT('Ctrl Pts',(-10.8811153220001,12.2,-0.428159018000014));
#265944=CARTESIAN_POINT('Ctrl Pts',(-10.8837846900001,12.2,-0.429163097000016));
#265945=CARTESIAN_POINT('Ctrl Pts',(-10.8864584680001,12.2,-0.430171373000015));
#265946=CARTESIAN_POINT('Ctrl Pts',(-10.8891366430001,12.2,-0.431183850000014));
#265947=CARTESIAN_POINT('Ctrl Pts',(-10.8918192040001,12.2,-0.432200531000015));
#265948=CARTESIAN_POINT('Ctrl Pts',(-10.8945061380001,12.2,-0.433221421000014));
#265949=CARTESIAN_POINT('Ctrl Pts',(-10.8971974330001,12.2,-0.434246522000015));
#265950=CARTESIAN_POINT('Ctrl Pts',(-10.8998930780001,12.2,-0.435275840000013));
#265951=CARTESIAN_POINT('Ctrl Pts',(-10.9025930590001,12.2,-0.436309378000015));
#265952=CARTESIAN_POINT('Ctrl Pts',(-10.9052973640001,12.2,-0.437347141000015));
#265953=CARTESIAN_POINT('Ctrl Pts',(-10.9080059810001,12.2,-0.438389130000014));
#265954=CARTESIAN_POINT('Ctrl Pts',(-10.9107188990001,12.2,-0.439435350000017));
#265955=CARTESIAN_POINT('Ctrl Pts',(-10.9134361040001,12.2,-0.440485807000015));
#265956=CARTESIAN_POINT('Ctrl Pts',(-10.9161575860001,12.2,-0.441540501000013));
#265957=CARTESIAN_POINT('Ctrl Pts',(-10.9188833300001,12.2,-0.442599438000015));
#265958=CARTESIAN_POINT('Ctrl Pts',(-10.9216133270001,12.2,-0.443662622000014));
#265959=CARTESIAN_POINT('Ctrl Pts',(-10.9243475630001,12.2,-0.444730056000013));
#265960=CARTESIAN_POINT('Ctrl Pts',(-10.9270860270001,12.2,-0.445801743000014));
#265961=CARTESIAN_POINT('Ctrl Pts',(-10.9298287070001,12.2,-0.446877689000011));
#265962=CARTESIAN_POINT('Ctrl Pts',(-10.9325755900001,12.2,-0.447957894000015));
#265963=CARTESIAN_POINT('Ctrl Pts',(-10.9353266640001,12.2,-0.449042364000016));
#265964=CARTESIAN_POINT('Ctrl Pts',(-10.9380819200001,12.2,-0.450131103000011));
#265965=CARTESIAN_POINT('Ctrl Pts',(-10.9408413420001,12.2,-0.451224112000013));
#265966=CARTESIAN_POINT('Ctrl Pts',(-10.9436049220001,12.2,-0.452321397000013));
#265967=CARTESIAN_POINT('Ctrl Pts',(-10.9463726460001,12.2,-0.453422962000012));
#265968=CARTESIAN_POINT('Ctrl Pts',(-10.9491445020001,12.2,-0.454528810000014));
#265969=CARTESIAN_POINT('Ctrl Pts',(-10.9519204780001,12.2,-0.455638942000016));
#265970=CARTESIAN_POINT('Ctrl Pts',(-10.9547005640001,12.2,-0.456753364000013));
#265971=CARTESIAN_POINT('Ctrl Pts',(-10.9574847480001,12.2,-0.457872080000015));
#265972=CARTESIAN_POINT('Ctrl Pts',(-10.9602730170001,12.2,-0.458995091000016));
#265973=CARTESIAN_POINT('Ctrl Pts',(-10.9630653590001,12.2,-0.460122402000014));
#265974=CARTESIAN_POINT('Ctrl Pts',(-10.9658617640001,12.2,-0.461254017000012));
#265975=CARTESIAN_POINT('Ctrl Pts',(-10.9686622200001,12.2,-0.462389938000012));
#265976=CARTESIAN_POINT('Ctrl Pts',(-10.9714667150001,12.2,-0.463530170000013));
#265977=CARTESIAN_POINT('Ctrl Pts',(-10.9742752370001,12.2,-0.464674714000015));
#265978=CARTESIAN_POINT('Ctrl Pts',(-10.9770877740001,12.2,-0.465823575000015));
#265979=CARTESIAN_POINT('Ctrl Pts',(-10.9799043170001,12.2,-0.466976757000013));
#265980=CARTESIAN_POINT('Ctrl Pts',(-10.9827248520001,12.2,-0.468134263000017));
#265981=CARTESIAN_POINT('Ctrl Pts',(-10.9855493680001,12.2,-0.469296094000011));
#265982=CARTESIAN_POINT('Ctrl Pts',(-10.9883778540001,12.2,-0.470462257000013));
#265983=CARTESIAN_POINT('Ctrl Pts',(-10.9912102990001,12.2,-0.471632753000013));
#265984=CARTESIAN_POINT('Ctrl Pts',(-10.9940466900001,12.2,-0.472807585000012));
#265985=CARTESIAN_POINT('Ctrl Pts',(-10.9968870170001,12.2,-0.473986757000016));
#265986=CARTESIAN_POINT('Ctrl Pts',(-10.9997312680001,12.2,-0.475170273000014));
#265987=CARTESIAN_POINT('Ctrl Pts',(-11.0025794320001,12.2,-0.476358134000012));
#265988=CARTESIAN_POINT('Ctrl Pts',(-11.0054314970001,12.2,-0.477550346000015));
#265989=CARTESIAN_POINT('Ctrl Pts',(-11.0082874530001,12.2,-0.478746910000014));
#265990=CARTESIAN_POINT('Ctrl Pts',(-11.0111472870001,12.2,-0.479947831000014));
#265991=CARTESIAN_POINT('Ctrl Pts',(-11.0140109890001,12.2,-0.481153110000014));
#265992=CARTESIAN_POINT('Ctrl Pts',(-11.0168785470001,12.2,-0.482362752000016));
#265993=CARTESIAN_POINT('Ctrl Pts',(-11.0197499510001,12.2,-0.483576758000015));
#265994=CARTESIAN_POINT('Ctrl Pts',(-11.0226251880001,12.2,-0.484795134000016));
#265995=CARTESIAN_POINT('Ctrl Pts',(-11.0255042470001,12.2,-0.486017881000014));
#265996=CARTESIAN_POINT('Ctrl Pts',(-11.0283871190001,12.2,-0.487245003000014));
#265997=CARTESIAN_POINT('Ctrl Pts',(-11.0312737910001,12.2,-0.488476502000013));
#265998=CARTESIAN_POINT('Ctrl Pts',(-11.0341642530001,12.2,-0.489712383000014));
#265999=CARTESIAN_POINT('Ctrl Pts',(-11.0370584920001,12.2,-0.490952646000018));
#266000=CARTESIAN_POINT('Ctrl Pts',(-11.0399564980001,12.2,-0.492197297000012));
#266001=CARTESIAN_POINT('Ctrl Pts',(-11.0428582610001,12.2,-0.493446338000014));
#266002=CARTESIAN_POINT('Ctrl Pts',(-11.0457637680001,12.2,-0.494699772000011));
#266003=CARTESIAN_POINT('Ctrl Pts',(-11.0486730100001,12.2,-0.495957601000012));
#266004=CARTESIAN_POINT('Ctrl Pts',(-11.0515859750001,12.2,-0.497219830000013));
#266005=CARTESIAN_POINT('Ctrl Pts',(-11.0545026510001,12.2,-0.498486460000014));
#266006=CARTESIAN_POINT('Ctrl Pts',(-11.0574230290001,12.2,-0.499757494000015));
#266007=CARTESIAN_POINT('Ctrl Pts',(-11.0603470970001,12.2,-0.501032937000012));
#266008=CARTESIAN_POINT('Ctrl Pts',(-11.0632748440001,12.2,-0.502312789000015));
#266009=CARTESIAN_POINT('Ctrl Pts',(-11.0662062590001,12.2,-0.503597056000018));
#266010=CARTESIAN_POINT('Ctrl Pts',(-11.0691413320001,12.2,-0.504885738000014));
#266011=CARTESIAN_POINT('Ctrl Pts',(-11.0720800520001,12.2,-0.506178839000011));
#266012=CARTESIAN_POINT('Ctrl Pts',(-11.0750224080001,12.2,-0.507476362000014));
#266013=CARTESIAN_POINT('Ctrl Pts',(-11.0779683880001,12.2,-0.508778311000011));
#266014=CARTESIAN_POINT('Ctrl Pts',(-11.0809179820001,12.2,-0.510084687000014));
#266015=CARTESIAN_POINT('Ctrl Pts',(-11.0838711810001,12.2,-0.511395492000015));
#266016=CARTESIAN_POINT('Ctrl Pts',(-11.0868279720001,12.2,-0.512710732000015));
#266017=CARTESIAN_POINT('Ctrl Pts',(-11.0897883450001,12.2,-0.514030406000017));
#266018=CARTESIAN_POINT('Ctrl Pts',(-11.0927522890001,12.2,-0.515354521000013));
#266019=CARTESIAN_POINT('Ctrl Pts',(-11.0957197940001,12.2,-0.516683076000017));
#266020=CARTESIAN_POINT('Ctrl Pts',(-11.0986908480001,12.2,-0.518016075000016));
#266021=CARTESIAN_POINT('Ctrl Pts',(-11.1016654420001,12.2,-0.519353522000015));
#266022=CARTESIAN_POINT('Ctrl Pts',(-11.1046435640001,12.2,-0.520695418000017));
#266023=CARTESIAN_POINT('Ctrl Pts',(-11.1076252050001,12.2,-0.522041766000014));
#266024=CARTESIAN_POINT('Ctrl Pts',(-11.1106103520001,12.2,-0.523392569000016));
#266025=CARTESIAN_POINT('Ctrl Pts',(-11.1135989970001,12.2,-0.524747830000014));
#266026=CARTESIAN_POINT('Ctrl Pts',(-11.1165911290001,12.2,-0.526107550000017));
#266027=CARTESIAN_POINT('Ctrl Pts',(-11.1195867360001,12.2,-0.527471735000016));
#266028=CARTESIAN_POINT('Ctrl Pts',(-11.1225858080001,12.2,-0.528840384000016));
#266029=CARTESIAN_POINT('Ctrl Pts',(-11.1255883350001,12.2,-0.530213501000016));
#266030=CARTESIAN_POINT('Ctrl Pts',(-11.1285943060001,12.2,-0.531591090000014));
#266031=CARTESIAN_POINT('Ctrl Pts',(-11.1316037120001,12.2,-0.532973151000018));
#266032=CARTESIAN_POINT('Ctrl Pts',(-11.1346165400001,12.2,-0.534359689000015));
#266033=CARTESIAN_POINT('Ctrl Pts',(-11.1376327810001,12.2,-0.535750705000013));
#266034=CARTESIAN_POINT('Ctrl Pts',(-11.1406524250001,12.2,-0.537146200000014));
#266035=CARTESIAN_POINT('Ctrl Pts',(-11.1436754620001,12.2,-0.538546181000013));
#266036=CARTESIAN_POINT('Ctrl Pts',(-11.1467018790001,12.2,-0.539950647000014));
#266037=CARTESIAN_POINT('Ctrl Pts',(-11.1497316690001,12.2,-0.541359602000018));
#266038=CARTESIAN_POINT('Ctrl Pts',(-11.1527648200001,12.2,-0.542773047000011));
#266039=CARTESIAN_POINT('Ctrl Pts',(-11.1558013220001,12.2,-0.544190986000017));
#266040=CARTESIAN_POINT('Ctrl Pts',(-11.1588411640001,12.2,-0.545613421000013));
#266041=CARTESIAN_POINT('Ctrl Pts',(-11.1618843360001,12.2,-0.547040354000017));
#266042=CARTESIAN_POINT('Ctrl Pts',(-11.1649308290001,12.2,-0.548471788000011));
#266043=CARTESIAN_POINT('Ctrl Pts',(-11.1679806310001,12.2,-0.549907725000014));
#266044=CARTESIAN_POINT('Ctrl Pts',(-11.1710337330001,12.2,-0.551348168000012));
#266045=CARTESIAN_POINT('Ctrl Pts',(-11.1740901240001,12.2,-0.552793118000015));
#266046=CARTESIAN_POINT('Ctrl Pts',(-11.1771497950001,12.2,-0.554242580000013));
#266047=CARTESIAN_POINT('Ctrl Pts',(-11.1802127340001,12.2,-0.555696554000011));
#266048=CARTESIAN_POINT('Ctrl Pts',(-11.1832789320001,12.2,-0.557155042000015));
#266049=CARTESIAN_POINT('Ctrl Pts',(-11.1863483800001,12.2,-0.558618049000015));
#266050=CARTESIAN_POINT('Ctrl Pts',(-11.1894210660001,12.2,-0.560085575000016));
#266051=CARTESIAN_POINT('Ctrl Pts',(-11.1924969800001,12.2,-0.561557623000013));
#266052=CARTESIAN_POINT('Ctrl Pts',(-11.1955761130001,12.2,-0.563034196000016));
#266053=CARTESIAN_POINT('Ctrl Pts',(-11.1986584540001,12.2,-0.564515295000017));
#266054=CARTESIAN_POINT('Ctrl Pts',(-11.2017439940001,12.2,-0.566000924000014));
#266055=CARTESIAN_POINT('Ctrl Pts',(-11.2048327210001,12.2,-0.567491084000018));
#266056=CARTESIAN_POINT('Ctrl Pts',(-11.2079246280001,12.2,-0.568985776000015));
#266057=CARTESIAN_POINT('Ctrl Pts',(-11.2110197020001,12.2,-0.570485006000014));
#266058=CARTESIAN_POINT('Ctrl Pts',(-11.2141179350001,12.2,-0.571988772000012));
#266059=CARTESIAN_POINT('Ctrl Pts',(-11.2172193170001,12.2,-0.573497079000016));
#266060=CARTESIAN_POINT('Ctrl Pts',(-11.2203238380001,12.2,-0.575009928000014));
#266061=CARTESIAN_POINT('Ctrl Pts',(-11.2234314850001,12.2,-0.576527323000011));
#266062=CARTESIAN_POINT('Ctrl Pts',(-11.2265422530001,12.2,-0.578049263000011));
#266063=CARTESIAN_POINT('Ctrl Pts',(-11.2296561290001,12.2,-0.579575753000015));
#266064=CARTESIAN_POINT('Ctrl Pts',(-11.2327731030001,12.2,-0.581106794000017));
#266065=CARTESIAN_POINT('Ctrl Pts',(-11.2358931670001,12.2,-0.582642387000014));
#266066=CARTESIAN_POINT('Ctrl Pts',(-11.2390163100001,12.2,-0.584182538000011));
#266067=CARTESIAN_POINT('Ctrl Pts',(-11.2421425230001,12.2,-0.585727245000012));
#266068=CARTESIAN_POINT('Ctrl Pts',(-11.2452717950001,12.2,-0.587276511000017));
#266069=CARTESIAN_POINT('Ctrl Pts',(-11.2484041180001,12.2,-0.588830340000013));
#266070=CARTESIAN_POINT('Ctrl Pts',(-11.2515394790001,12.2,-0.590388732000013));
#266071=CARTESIAN_POINT('Ctrl Pts',(-11.2546778710001,12.2,-0.591951690000014));
#266072=CARTESIAN_POINT('Ctrl Pts',(-11.2578192840001,12.2,-0.593519216000011));
#266073=CARTESIAN_POINT('Ctrl Pts',(-11.2609637080001,12.2,-0.595091312000013));
#266074=CARTESIAN_POINT('Ctrl Pts',(-11.2641111320001,12.2,-0.596667981000016));
#266075=CARTESIAN_POINT('Ctrl Pts',(-11.2672615480001,12.2,-0.598249222000016));
#266076=CARTESIAN_POINT('Ctrl Pts',(-11.2704149460001,12.2,-0.599835041000016));
#266077=CARTESIAN_POINT('Ctrl Pts',(-11.2735713160001,12.2,-0.601425437000014));
#266078=CARTESIAN_POINT('Ctrl Pts',(-11.2767306480001,12.2,-0.603020414000017));
#266079=CARTESIAN_POINT('Ctrl Pts',(-11.2798929340001,12.2,-0.604619973000013));
#266080=CARTESIAN_POINT('Ctrl Pts',(-11.2830581620001,12.2,-0.606224115000016));
#266081=CARTESIAN_POINT('Ctrl Pts',(-11.2862263240001,12.2,-0.607832843000011));
#266082=CARTESIAN_POINT('Ctrl Pts',(-11.2893974100001,12.2,-0.609446160000013));
#266083=CARTESIAN_POINT('Ctrl Pts',(-11.2925714100001,12.2,-0.611064067000013));
#266084=CARTESIAN_POINT('Ctrl Pts',(-11.2957483150001,12.2,-0.612686565000011));
#266085=CARTESIAN_POINT('Ctrl Pts',(-11.2989281170001,12.2,-0.614313657000016));
#266086=CARTESIAN_POINT('Ctrl Pts',(-11.3021108030001,12.2,-0.615945345000015));
#266087=CARTESIAN_POINT('Ctrl Pts',(-11.3052963650001,12.2,-0.617581630000017));
#266088=CARTESIAN_POINT('Ctrl Pts',(-11.3084847960001,12.2,-0.619222515000013));
#266089=CARTESIAN_POINT('Ctrl Pts',(-11.3116760820001,12.2,-0.620868001000012));
#266090=CARTESIAN_POINT('Ctrl Pts',(-11.3148702170001,12.2,-0.622518091000015));
#266091=CARTESIAN_POINT('Ctrl Pts',(-11.3180671910001,12.2,-0.624172784000017));
#266092=CARTESIAN_POINT('Ctrl Pts',(-11.3212669940001,12.2,-0.625832085000013));
#266093=CARTESIAN_POINT('Ctrl Pts',(-11.3244696160001,12.2,-0.627495996000014));
#266094=CARTESIAN_POINT('Ctrl Pts',(-11.3276750490001,12.2,-0.629164515000014));
#266095=CARTESIAN_POINT('Ctrl Pts',(-11.3308832820001,12.2,-0.630837648000018));
#266096=CARTESIAN_POINT('Ctrl Pts',(-11.3340943080001,12.2,-0.632515395000013));
#266097=CARTESIAN_POINT('Ctrl Pts',(-11.3373081150001,12.2,-0.634197758000017));
#266098=CARTESIAN_POINT('Ctrl Pts',(-11.3405246950001,12.2,-0.635884737000012));
#266099=CARTESIAN_POINT('Ctrl Pts',(-11.3437440390001,12.2,-0.637576336000016));
#266100=CARTESIAN_POINT('Ctrl Pts',(-11.3469661360001,12.2,-0.639272557000012));
#266101=CARTESIAN_POINT('Ctrl Pts',(-11.3501909790001,12.2,-0.640973401000018));
#266102=CARTESIAN_POINT('Ctrl Pts',(-11.3534185570001,12.2,-0.642678869000015));
#266103=CARTESIAN_POINT('Ctrl Pts',(-11.3566488620001,12.2,-0.644388964000013));
#266104=CARTESIAN_POINT('Ctrl Pts',(-11.3598818840001,12.2,-0.646103687000017));
#266105=CARTESIAN_POINT('Ctrl Pts',(-11.3631176140001,12.2,-0.647823039000013));
#266106=CARTESIAN_POINT('Ctrl Pts',(-11.3663560430001,12.2,-0.649547023000014));
#266107=CARTESIAN_POINT('Ctrl Pts',(-11.3695971620001,12.2,-0.651275639000013));
#266108=CARTESIAN_POINT('Ctrl Pts',(-11.3728409600001,12.2,-0.653008892000013));
#266109=CARTESIAN_POINT('Ctrl Pts',(-11.3760874300001,12.2,-0.654746780000015));
#266110=CARTESIAN_POINT('Ctrl Pts',(-11.3793365610001,12.2,-0.656489306000014));
#266111=CARTESIAN_POINT('Ctrl Pts',(-11.3825883450001,12.2,-0.658236472000016));
#266112=CARTESIAN_POINT('Ctrl Pts',(-11.3858427730001,12.2,-0.659988280000015));
#266113=CARTESIAN_POINT('Ctrl Pts',(-11.3890998350001,12.2,-0.661744730000016));
#266114=CARTESIAN_POINT('Ctrl Pts',(-11.3923595230001,12.2,-0.663505825000015));
#266115=CARTESIAN_POINT('Ctrl Pts',(-11.3956218280001,12.2,-0.665271566000012));
#266116=CARTESIAN_POINT('Ctrl Pts',(-11.3988867400001,12.2,-0.667041955000016));
#266117=CARTESIAN_POINT('Ctrl Pts',(-11.4021542520001,12.2,-0.668816993000014));
#266118=CARTESIAN_POINT('Ctrl Pts',(-11.4054243520001,12.2,-0.670596683000015));
#266119=CARTESIAN_POINT('Ctrl Pts',(-11.4086970320001,12.2,-0.672381023000015));
#266120=CARTESIAN_POINT('Ctrl Pts',(-11.4119722840001,12.2,-0.674170019000013));
#266121=CARTESIAN_POINT('Ctrl Pts',(-11.4152500960001,12.2,-0.675963670000015));
#266122=CARTESIAN_POINT('Ctrl Pts',(-11.4185304610001,12.2,-0.677761979000016));
#266123=CARTESIAN_POINT('Ctrl Pts',(-11.4218133690001,12.2,-0.679564946000015));
#266124=CARTESIAN_POINT('Ctrl Pts',(-11.4250988120001,12.2,-0.681372573000014));
#266125=CARTESIAN_POINT('Ctrl Pts',(-11.4283867810001,12.2,-0.683184862000012));
#266126=CARTESIAN_POINT('Ctrl Pts',(-11.4316772700001,12.2,-0.685001814000015));
#266127=CARTESIAN_POINT('Ctrl Pts',(-11.4349702680001,12.2,-0.686823430000012));
#266128=CARTESIAN_POINT('Ctrl Pts',(-11.4382657700001,12.2,-0.688649711000018));
#266129=CARTESIAN_POINT('Ctrl Pts',(-11.4415637630001,12.2,-0.690480659000015));
#266130=CARTESIAN_POINT('Ctrl Pts',(-11.4448642400001,12.2,-0.692316276000016));
#266131=CARTESIAN_POINT('Ctrl Pts',(-11.4481671870001,12.2,-0.694156565000017));
#266132=CARTESIAN_POINT('Ctrl Pts',(-11.4514725950001,12.2,-0.696001525000014));
#266133=CARTESIAN_POINT('Ctrl Pts',(-11.4547804530001,12.2,-0.697851159000016));
#266134=CARTESIAN_POINT('Ctrl Pts',(-11.4580907510001,12.2,-0.699705470000014));
#266135=CARTESIAN_POINT('Ctrl Pts',(-11.4614034810001,12.2,-0.701564457000017));
#266136=CARTESIAN_POINT('Ctrl Pts',(-11.4647186380001,12.2,-0.703428121000016));
#266137=CARTESIAN_POINT('Ctrl Pts',(-11.4680362160001,12.2,-0.705296464000016));
#266138=CARTESIAN_POINT('Ctrl Pts',(-11.4713562160001,12.2,-0.707169486000012));
#266139=CARTESIAN_POINT('Ctrl Pts',(-11.4740141490001,12.2,-0.708671646000014));
#266140=CARTESIAN_POINT('Ctrl Pts',(-11.4760086880001,12.2,-0.709800372000018));
#266141=CARTESIAN_POINT('Ctrl Pts',(-11.4773388640001,12.2,-0.710553791000015));
#266142=CARTESIAN_POINT('Ctrl Pts',(-11.4780040730001,12.2,-0.710930734000015));
#266143=CARTESIAN_POINT('Origin',(-5.66257110645729E-14,15.2,-1.77635683940025E-14));
#266144=CARTESIAN_POINT('',(-10.2237731093969,15.2,-1.76496130634431));
#266145=CARTESIAN_POINT('',(-10.2237731093969,12.2,-1.76496130634431));
#266146=CARTESIAN_POINT('',(-10.2237731090001,15.2,-1.76496130600002));
#266147=CARTESIAN_POINT('Origin',(-5.66257110645729E-14,12.2,-1.77635683940025E-14));
#266148=CARTESIAN_POINT('Origin',(-5.66257110645729E-14,15.2,-1.77635683940025E-14));
#266149=CARTESIAN_POINT('Origin',(-5.66257110645729E-14,15.2,-1.77635683940025E-14));
#266150=CARTESIAN_POINT('',(-11.2599985490001,15.2,-2.33718477800001));
#266151=CARTESIAN_POINT('',(-11.1757778680001,15.2,-2.71145515300002));
#266152=CARTESIAN_POINT('Origin',(-5.66257110645729E-14,15.2,-1.77635683940025E-14));
#266153=CARTESIAN_POINT('',(-11.1757778680001,12.2,-2.71145515300002));
#266154=CARTESIAN_POINT('',(-11.1757778680001,15.2,-2.71145515300002));
#266155=CARTESIAN_POINT('',(-11.2599985490001,12.2,-2.33718477800001));
#266156=CARTESIAN_POINT('Origin',(-5.66257110645729E-14,12.2,-1.77635683940025E-14));
#266157=CARTESIAN_POINT('',(-11.2599985490001,15.2,-2.33718477800001));
#266158=CARTESIAN_POINT('Ctrl Pts',(-10.2237731100001,15.2,-1.76496130700002));
#266159=CARTESIAN_POINT('Ctrl Pts',(-10.2237731100001,11.6,-1.76496130700002));
#266160=CARTESIAN_POINT('Ctrl Pts',(-10.2239417410001,15.2,-1.76500562400001));
#266161=CARTESIAN_POINT('Ctrl Pts',(-10.2239417410001,11.6,-1.76500562400001));
#266162=CARTESIAN_POINT('Ctrl Pts',(-10.2242848730001,15.2,-1.76509588800001));
#266163=CARTESIAN_POINT('Ctrl Pts',(-10.2242848730001,11.6,-1.76509588800001));
#266164=CARTESIAN_POINT('Ctrl Pts',(-10.2248047310001,15.2,-1.76523291900001));
#266165=CARTESIAN_POINT('Ctrl Pts',(-10.2248047310001,11.6,-1.76523291900002));
#266166=CARTESIAN_POINT('Ctrl Pts',(-10.2255048910001,15.2,-1.76541803300001));
#266167=CARTESIAN_POINT('Ctrl Pts',(-10.2255048910001,11.6,-1.76541803300002));
#266168=CARTESIAN_POINT('Ctrl Pts',(-10.2263902540001,15.2,-1.76565305800001));
#266169=CARTESIAN_POINT('Ctrl Pts',(-10.2263902540001,11.6,-1.76565305800001));
#266170=CARTESIAN_POINT('Ctrl Pts',(-10.2272897270001,15.2,-1.76589279500002));
#266171=CARTESIAN_POINT('Ctrl Pts',(-10.2272897270001,11.6,-1.76589279500002));
#266172=CARTESIAN_POINT('Ctrl Pts',(-10.2281981500001,15.2,-1.76613589400001));
#266173=CARTESIAN_POINT('Ctrl Pts',(-10.2281981500001,11.6,-1.76613589400001));
#266174=CARTESIAN_POINT('Ctrl Pts',(-10.2291154920001,15.2,-1.76638236500001));
#266175=CARTESIAN_POINT('Ctrl Pts',(-10.2291154920001,11.6,-1.76638236500001));
#266176=CARTESIAN_POINT('Ctrl Pts',(-10.2300417240001,15.2,-1.76663221900001));
#266177=CARTESIAN_POINT('Ctrl Pts',(-10.2300417240001,11.6,-1.76663221900002));
#266178=CARTESIAN_POINT('Ctrl Pts',(-10.2309768130001,15.2,-1.76688546700001));
#266179=CARTESIAN_POINT('Ctrl Pts',(-10.2309768130001,11.6,-1.76688546700001));
#266180=CARTESIAN_POINT('Ctrl Pts',(-10.2319207290001,15.2,-1.76714211800002));
#266181=CARTESIAN_POINT('Ctrl Pts',(-10.2319207290001,11.6,-1.76714211800002));
#266182=CARTESIAN_POINT('Ctrl Pts',(-10.2328734440001,15.2,-1.76740218200001));
#266183=CARTESIAN_POINT('Ctrl Pts',(-10.2328734440001,11.6,-1.76740218200001));
#266184=CARTESIAN_POINT('Ctrl Pts',(-10.2338349260001,15.2,-1.76766567100001));
#266185=CARTESIAN_POINT('Ctrl Pts',(-10.2338349260001,11.6,-1.76766567100001));
#266186=CARTESIAN_POINT('Ctrl Pts',(-10.2348051460001,15.2,-1.76793259300001));
#266187=CARTESIAN_POINT('Ctrl Pts',(-10.2348051460001,11.6,-1.76793259300001));
#266188=CARTESIAN_POINT('Ctrl Pts',(-10.2357840740001,15.2,-1.76820296000002));
#266189=CARTESIAN_POINT('Ctrl Pts',(-10.2357840740001,11.6,-1.76820296000002));
#266190=CARTESIAN_POINT('Ctrl Pts',(-10.2367716800001,15.2,-1.76847678200001));
#266191=CARTESIAN_POINT('Ctrl Pts',(-10.2367716800001,11.6,-1.76847678200002));
#266192=CARTESIAN_POINT('Ctrl Pts',(-10.2377679360001,15.2,-1.76875406700002));
#266193=CARTESIAN_POINT('Ctrl Pts',(-10.2377679360001,11.6,-1.76875406700002));
#266194=CARTESIAN_POINT('Ctrl Pts',(-10.2387728090001,15.2,-1.76903482700002));
#266195=CARTESIAN_POINT('Ctrl Pts',(-10.2387728090001,11.6,-1.76903482700002));
#266196=CARTESIAN_POINT('Ctrl Pts',(-10.2397862740001,15.2,-1.76931907200002));
#266197=CARTESIAN_POINT('Ctrl Pts',(-10.2397862740001,11.6,-1.76931907200002));
#266198=CARTESIAN_POINT('Ctrl Pts',(-10.2408083000001,15.2,-1.76960681000002));
#266199=CARTESIAN_POINT('Ctrl Pts',(-10.2408083000001,11.6,-1.76960681000002));
#266200=CARTESIAN_POINT('Ctrl Pts',(-10.2418388590001,15.2,-1.76989805200002));
#266201=CARTESIAN_POINT('Ctrl Pts',(-10.2418388590001,11.6,-1.76989805200002));
#266202=CARTESIAN_POINT('Ctrl Pts',(-10.2428779210001,15.2,-1.77019280700002));
#266203=CARTESIAN_POINT('Ctrl Pts',(-10.2428779210001,11.6,-1.77019280700002));
#266204=CARTESIAN_POINT('Ctrl Pts',(-10.2439254560001,15.2,-1.77049108600002));
#266205=CARTESIAN_POINT('Ctrl Pts',(-10.2439254560001,11.6,-1.77049108600002));
#266206=CARTESIAN_POINT('Ctrl Pts',(-10.2449814390001,15.2,-1.77079289700002));
#266207=CARTESIAN_POINT('Ctrl Pts',(-10.2449814390001,11.6,-1.77079289700002));
#266208=CARTESIAN_POINT('Ctrl Pts',(-10.2460458400001,15.2,-1.77109824900001));
#266209=CARTESIAN_POINT('Ctrl Pts',(-10.2460458400001,11.6,-1.77109824900001));
#266210=CARTESIAN_POINT('Ctrl Pts',(-10.2471186300001,15.2,-1.77140715300002));
#266211=CARTESIAN_POINT('Ctrl Pts',(-10.2471186300001,11.6,-1.77140715300002));
#266212=CARTESIAN_POINT('Ctrl Pts',(-10.2481997820001,15.2,-1.77171961900001));
#266213=CARTESIAN_POINT('Ctrl Pts',(-10.2481997820001,11.6,-1.77171961900001));
#266214=CARTESIAN_POINT('Ctrl Pts',(-10.2492892660001,15.2,-1.77203565400001));
#266215=CARTESIAN_POINT('Ctrl Pts',(-10.2492892660001,11.6,-1.77203565400002));
#266216=CARTESIAN_POINT('Ctrl Pts',(-10.2503870570001,15.2,-1.77235526900001));
#266217=CARTESIAN_POINT('Ctrl Pts',(-10.2503870570001,11.6,-1.77235526900001));
#266218=CARTESIAN_POINT('Ctrl Pts',(-10.2514931250001,15.2,-1.77267847300001));
#266219=CARTESIAN_POINT('Ctrl Pts',(-10.2514931250001,11.6,-1.77267847300001));
#266220=CARTESIAN_POINT('Ctrl Pts',(-10.2526074440001,15.2,-1.77300527500002));
#266221=CARTESIAN_POINT('Ctrl Pts',(-10.2526074440001,11.6,-1.77300527500002));
#266222=CARTESIAN_POINT('Ctrl Pts',(-10.2537299850001,15.2,-1.77333568400002));
#266223=CARTESIAN_POINT('Ctrl Pts',(-10.2537299850001,11.6,-1.77333568400002));
#266224=CARTESIAN_POINT('Ctrl Pts',(-10.2548607200001,15.2,-1.77366970900001));
#266225=CARTESIAN_POINT('Ctrl Pts',(-10.2548607200001,11.6,-1.77366970900001));
#266226=CARTESIAN_POINT('Ctrl Pts',(-10.2559996250001,15.2,-1.77400735800001));
#266227=CARTESIAN_POINT('Ctrl Pts',(-10.2559996250001,11.6,-1.77400735800001));
#266228=CARTESIAN_POINT('Ctrl Pts',(-10.2571466690001,15.2,-1.77434864200002));
#266229=CARTESIAN_POINT('Ctrl Pts',(-10.2571466690001,11.6,-1.77434864200002));
#266230=CARTESIAN_POINT('Ctrl Pts',(-10.2583018280001,15.2,-1.77469356900001));
#266231=CARTESIAN_POINT('Ctrl Pts',(-10.2583018280001,11.6,-1.77469356900001));
#266232=CARTESIAN_POINT('Ctrl Pts',(-10.2594650730001,15.2,-1.77504214700001));
#266233=CARTESIAN_POINT('Ctrl Pts',(-10.2594650730001,11.6,-1.77504214700001));
#266234=CARTESIAN_POINT('Ctrl Pts',(-10.2606363780001,15.2,-1.77539438600002));
#266235=CARTESIAN_POINT('Ctrl Pts',(-10.2606363780001,11.6,-1.77539438600002));
#266236=CARTESIAN_POINT('Ctrl Pts',(-10.2618157170001,15.2,-1.77575029400002));
#266237=CARTESIAN_POINT('Ctrl Pts',(-10.2618157170001,11.6,-1.77575029400002));
#266238=CARTESIAN_POINT('Ctrl Pts',(-10.2630030620001,15.2,-1.77610988000001));
#266239=CARTESIAN_POINT('Ctrl Pts',(-10.2630030620001,11.6,-1.77610988000001));
#266240=CARTESIAN_POINT('Ctrl Pts',(-10.2641983870001,15.2,-1.77647315300002));
#266241=CARTESIAN_POINT('Ctrl Pts',(-10.2641983870001,11.6,-1.77647315300002));
#266242=CARTESIAN_POINT('Ctrl Pts',(-10.2654016660001,15.2,-1.77684012100002));
#266243=CARTESIAN_POINT('Ctrl Pts',(-10.2654016660001,11.6,-1.77684012100002));
#266244=CARTESIAN_POINT('Ctrl Pts',(-10.2666128740001,15.2,-1.77721079200001));
#266245=CARTESIAN_POINT('Ctrl Pts',(-10.2666128740001,11.6,-1.77721079200001));
#266246=CARTESIAN_POINT('Ctrl Pts',(-10.2678319830001,15.2,-1.77758517500001));
#266247=CARTESIAN_POINT('Ctrl Pts',(-10.2678319830001,11.6,-1.77758517500001));
#266248=CARTESIAN_POINT('Ctrl Pts',(-10.2690589670001,15.2,-1.77796328000001));
#266249=CARTESIAN_POINT('Ctrl Pts',(-10.2690589670001,11.6,-1.77796328000001));
#266250=CARTESIAN_POINT('Ctrl Pts',(-10.2702938010001,15.2,-1.77834511200002));
#266251=CARTESIAN_POINT('Ctrl Pts',(-10.2702938010001,11.6,-1.77834511200002));
#266252=CARTESIAN_POINT('Ctrl Pts',(-10.2715364580001,15.2,-1.77873068300002));
#266253=CARTESIAN_POINT('Ctrl Pts',(-10.2715364580001,11.6,-1.77873068300002));
#266254=CARTESIAN_POINT('Ctrl Pts',(-10.2727869140001,15.2,-1.77911999900001));
#266255=CARTESIAN_POINT('Ctrl Pts',(-10.2727869140001,11.6,-1.77911999900001));
#266256=CARTESIAN_POINT('Ctrl Pts',(-10.2740451430001,15.2,-1.77951306800002));
#266257=CARTESIAN_POINT('Ctrl Pts',(-10.2740451430001,11.6,-1.77951306800002));
#266258=CARTESIAN_POINT('Ctrl Pts',(-10.2753111180001,15.2,-1.77990989900001));
#266259=CARTESIAN_POINT('Ctrl Pts',(-10.2753111180001,11.6,-1.77990989900001));
#266260=CARTESIAN_POINT('Ctrl Pts',(-10.2765848160001,15.2,-1.78031050100001));
#266261=CARTESIAN_POINT('Ctrl Pts',(-10.2765848160001,11.6,-1.78031050100001));
#266262=CARTESIAN_POINT('Ctrl Pts',(-10.2778662100001,15.2,-1.78071488100001));
#266263=CARTESIAN_POINT('Ctrl Pts',(-10.2778662100001,11.6,-1.78071488100001));
#266264=CARTESIAN_POINT('Ctrl Pts',(-10.2791552770001,15.2,-1.78112304700001));
#266265=CARTESIAN_POINT('Ctrl Pts',(-10.2791552770001,11.6,-1.78112304700001));
#266266=CARTESIAN_POINT('Ctrl Pts',(-10.2804519880001,15.2,-1.78153500600001));
#266267=CARTESIAN_POINT('Ctrl Pts',(-10.2804519880001,11.6,-1.78153500600002));
#266268=CARTESIAN_POINT('Ctrl Pts',(-10.2817563210001,15.2,-1.78195076800002));
#266269=CARTESIAN_POINT('Ctrl Pts',(-10.2817563210001,11.6,-1.78195076800002));
#266270=CARTESIAN_POINT('Ctrl Pts',(-10.2830682520001,15.2,-1.78237034000002));
#266271=CARTESIAN_POINT('Ctrl Pts',(-10.2830682520001,11.6,-1.78237034000002));
#266272=CARTESIAN_POINT('Ctrl Pts',(-10.2843877540001,15.2,-1.78279372900001));
#266273=CARTESIAN_POINT('Ctrl Pts',(-10.2843877540001,11.6,-1.78279372900001));
#266274=CARTESIAN_POINT('Ctrl Pts',(-10.2857148030001,15.2,-1.78322094400002));
#266275=CARTESIAN_POINT('Ctrl Pts',(-10.2857148030001,11.6,-1.78322094400002));
#266276=CARTESIAN_POINT('Ctrl Pts',(-10.2870493750001,15.2,-1.78365199300002));
#266277=CARTESIAN_POINT('Ctrl Pts',(-10.2870493750001,11.6,-1.78365199300002));
#266278=CARTESIAN_POINT('Ctrl Pts',(-10.2883914450001,15.2,-1.78408688200001));
#266279=CARTESIAN_POINT('Ctrl Pts',(-10.2883914450001,11.6,-1.78408688200001));
#266280=CARTESIAN_POINT('Ctrl Pts',(-10.2897409890001,15.2,-1.78452562100002));
#266281=CARTESIAN_POINT('Ctrl Pts',(-10.2897409890001,11.6,-1.78452562100002));
#266282=CARTESIAN_POINT('Ctrl Pts',(-10.2910979840001,15.2,-1.78496821600001));
#266283=CARTESIAN_POINT('Ctrl Pts',(-10.2910979840001,11.6,-1.78496821600001));
#266284=CARTESIAN_POINT('Ctrl Pts',(-10.2924624030001,15.2,-1.78541467500001));
#266285=CARTESIAN_POINT('Ctrl Pts',(-10.2924624030001,11.6,-1.78541467500001));
#266286=CARTESIAN_POINT('Ctrl Pts',(-10.2938342240001,15.2,-1.78586500400002));
#266287=CARTESIAN_POINT('Ctrl Pts',(-10.2938342240001,11.6,-1.78586500400002));
#266288=CARTESIAN_POINT('Ctrl Pts',(-10.2952134230001,15.2,-1.78631921300001));
#266289=CARTESIAN_POINT('Ctrl Pts',(-10.2952134230001,11.6,-1.78631921300001));
#266290=CARTESIAN_POINT('Ctrl Pts',(-10.2965999750001,15.2,-1.78677730900001));
#266291=CARTESIAN_POINT('Ctrl Pts',(-10.2965999750001,11.6,-1.78677730900001));
#266292=CARTESIAN_POINT('Ctrl Pts',(-10.2979938570001,15.2,-1.78723929800002));
#266293=CARTESIAN_POINT('Ctrl Pts',(-10.2979938570001,11.6,-1.78723929800002));
#266294=CARTESIAN_POINT('Ctrl Pts',(-10.2993950460001,15.2,-1.78770518800001));
#266295=CARTESIAN_POINT('Ctrl Pts',(-10.2993950460001,11.6,-1.78770518800001));
#266296=CARTESIAN_POINT('Ctrl Pts',(-10.3008035180001,15.2,-1.78817498600001));
#266297=CARTESIAN_POINT('Ctrl Pts',(-10.3008035180001,11.6,-1.78817498600001));
#266298=CARTESIAN_POINT('Ctrl Pts',(-10.3022192480001,15.2,-1.78864870100002));
#266299=CARTESIAN_POINT('Ctrl Pts',(-10.3022192480001,11.6,-1.78864870100002));
#266300=CARTESIAN_POINT('Ctrl Pts',(-10.3036422150001,15.2,-1.78912633800001));
#266301=CARTESIAN_POINT('Ctrl Pts',(-10.3036422150001,11.6,-1.78912633800001));
#266302=CARTESIAN_POINT('Ctrl Pts',(-10.3050723940001,15.2,-1.78960790500001));
#266303=CARTESIAN_POINT('Ctrl Pts',(-10.3050723940001,11.6,-1.78960790500002));
#266304=CARTESIAN_POINT('Ctrl Pts',(-10.3065097620001,15.2,-1.79009341000001));
#266305=CARTESIAN_POINT('Ctrl Pts',(-10.3065097620001,11.6,-1.79009341000001));
#266306=CARTESIAN_POINT('Ctrl Pts',(-10.3079542970001,15.2,-1.79058285800001));
#266307=CARTESIAN_POINT('Ctrl Pts',(-10.3079542970001,11.6,-1.79058285800001));
#266308=CARTESIAN_POINT('Ctrl Pts',(-10.3094059740001,15.2,-1.79107625800001));
#266309=CARTESIAN_POINT('Ctrl Pts',(-10.3094059740001,11.6,-1.79107625800001));
#266310=CARTESIAN_POINT('Ctrl Pts',(-10.3108647730001,15.2,-1.79157361600002));
#266311=CARTESIAN_POINT('Ctrl Pts',(-10.3108647730001,11.6,-1.79157361600002));
#266312=CARTESIAN_POINT('Ctrl Pts',(-10.3123306680001,15.2,-1.79207494100002));
#266313=CARTESIAN_POINT('Ctrl Pts',(-10.3123306680001,11.6,-1.79207494100002));
#266314=CARTESIAN_POINT('Ctrl Pts',(-10.3138036390001,15.2,-1.79258023700001));
#266315=CARTESIAN_POINT('Ctrl Pts',(-10.3138036390001,11.6,-1.79258023700001));
#266316=CARTESIAN_POINT('Ctrl Pts',(-10.3152836600001,15.2,-1.79308951300001));
#266317=CARTESIAN_POINT('Ctrl Pts',(-10.3152836600001,11.6,-1.79308951300001));
#266318=CARTESIAN_POINT('Ctrl Pts',(-10.3167707130001,15.2,-1.79360277400002));
#266319=CARTESIAN_POINT('Ctrl Pts',(-10.3167707130001,11.6,-1.79360277400002));
#266320=CARTESIAN_POINT('Ctrl Pts',(-10.3182647710001,15.2,-1.79412002800001));
#266321=CARTESIAN_POINT('Ctrl Pts',(-10.3182647710001,11.6,-1.79412002800001));
#266322=CARTESIAN_POINT('Ctrl Pts',(-10.3197658140001,15.2,-1.79464128300001));
#266323=CARTESIAN_POINT('Ctrl Pts',(-10.3197658140001,11.6,-1.79464128300001));
#266324=CARTESIAN_POINT('Ctrl Pts',(-10.3212738190001,15.2,-1.79516654400001));
#266325=CARTESIAN_POINT('Ctrl Pts',(-10.3212738190001,11.6,-1.79516654400001));
#266326=CARTESIAN_POINT('Ctrl Pts',(-10.3227887640001,15.2,-1.79569581700001));
#266327=CARTESIAN_POINT('Ctrl Pts',(-10.3227887640001,11.6,-1.79569581700001));
#266328=CARTESIAN_POINT('Ctrl Pts',(-10.3243106270001,15.2,-1.79622911100001));
#266329=CARTESIAN_POINT('Ctrl Pts',(-10.3243106270001,11.6,-1.79622911100001));
#266330=CARTESIAN_POINT('Ctrl Pts',(-10.3258393850001,15.2,-1.79676643100001));
#266331=CARTESIAN_POINT('Ctrl Pts',(-10.3258393850001,11.6,-1.79676643100001));
#266332=CARTESIAN_POINT('Ctrl Pts',(-10.3273750170001,15.2,-1.79730778300002));
#266333=CARTESIAN_POINT('Ctrl Pts',(-10.3273750170001,11.6,-1.79730778300002));
#266334=CARTESIAN_POINT('Ctrl Pts',(-10.3289175010001,15.2,-1.79785317600002));
#266335=CARTESIAN_POINT('Ctrl Pts',(-10.3289175010001,11.6,-1.79785317600002));
#266336=CARTESIAN_POINT('Ctrl Pts',(-10.3304668150001,15.2,-1.79840261500001));
#266337=CARTESIAN_POINT('Ctrl Pts',(-10.3304668150001,11.6,-1.79840261500001));
#266338=CARTESIAN_POINT('Ctrl Pts',(-10.3320229360001,15.2,-1.79895610500001));
#266339=CARTESIAN_POINT('Ctrl Pts',(-10.3320229360001,11.6,-1.79895610500001));
#266340=CARTESIAN_POINT('Ctrl Pts',(-10.3335858440001,15.2,-1.79951365400001));
#266341=CARTESIAN_POINT('Ctrl Pts',(-10.3335858440001,11.6,-1.79951365400001));
#266342=CARTESIAN_POINT('Ctrl Pts',(-10.3351555170001,15.2,-1.80007527000001));
#266343=CARTESIAN_POINT('Ctrl Pts',(-10.3351555170001,11.6,-1.80007527000001));
#266344=CARTESIAN_POINT('Ctrl Pts',(-10.3367319330001,15.2,-1.80064095700001));
#266345=CARTESIAN_POINT('Ctrl Pts',(-10.3367319330001,11.6,-1.80064095700002));
#266346=CARTESIAN_POINT('Ctrl Pts',(-10.3383150710001,15.2,-1.80121072200001));
#266347=CARTESIAN_POINT('Ctrl Pts',(-10.3383150710001,11.6,-1.80121072200001));
#266348=CARTESIAN_POINT('Ctrl Pts',(-10.3399049090001,15.2,-1.80178457100002));
#266349=CARTESIAN_POINT('Ctrl Pts',(-10.3399049090001,11.6,-1.80178457100002));
#266350=CARTESIAN_POINT('Ctrl Pts',(-10.3415014270001,15.2,-1.80236251100002));
#266351=CARTESIAN_POINT('Ctrl Pts',(-10.3415014270001,11.6,-1.80236251100002));
#266352=CARTESIAN_POINT('Ctrl Pts',(-10.3431046030001,15.2,-1.80294454800002));
#266353=CARTESIAN_POINT('Ctrl Pts',(-10.3431046030001,11.6,-1.80294454800002));
#266354=CARTESIAN_POINT('Ctrl Pts',(-10.3447144150001,15.2,-1.80353068700001));
#266355=CARTESIAN_POINT('Ctrl Pts',(-10.3447144150001,11.6,-1.80353068700001));
#266356=CARTESIAN_POINT('Ctrl Pts',(-10.3463308440001,15.2,-1.80412093600001));
#266357=CARTESIAN_POINT('Ctrl Pts',(-10.3463308440001,11.6,-1.80412093600001));
#266358=CARTESIAN_POINT('Ctrl Pts',(-10.3479538660001,15.2,-1.80471530000001));
#266359=CARTESIAN_POINT('Ctrl Pts',(-10.3479538660001,11.6,-1.80471530000002));
#266360=CARTESIAN_POINT('Ctrl Pts',(-10.3495834630001,15.2,-1.80531378500001));
#266361=CARTESIAN_POINT('Ctrl Pts',(-10.3495834630001,11.6,-1.80531378500001));
#266362=CARTESIAN_POINT('Ctrl Pts',(-10.3512196130001,15.2,-1.80591639700001));
#266363=CARTESIAN_POINT('Ctrl Pts',(-10.3512196130001,11.6,-1.80591639700001));
#266364=CARTESIAN_POINT('Ctrl Pts',(-10.3528622950001,15.2,-1.80652314400001));
#266365=CARTESIAN_POINT('Ctrl Pts',(-10.3528622950001,11.6,-1.80652314400001));
#266366=CARTESIAN_POINT('Ctrl Pts',(-10.3545114890001,15.2,-1.80713402800002));
#266367=CARTESIAN_POINT('Ctrl Pts',(-10.3545114890001,11.6,-1.80713402800002));
#266368=CARTESIAN_POINT('Ctrl Pts',(-10.3561671730001,15.2,-1.80774905900002));
#266369=CARTESIAN_POINT('Ctrl Pts',(-10.3561671730001,11.6,-1.80774905900002));
#266370=CARTESIAN_POINT('Ctrl Pts',(-10.3578293270001,15.2,-1.80836824100002));
#266371=CARTESIAN_POINT('Ctrl Pts',(-10.3578293270001,11.6,-1.80836824100002));
#266372=CARTESIAN_POINT('Ctrl Pts',(-10.3594979320001,15.2,-1.80899157900001));
#266373=CARTESIAN_POINT('Ctrl Pts',(-10.3594979320001,11.6,-1.80899157900001));
#266374=CARTESIAN_POINT('Ctrl Pts',(-10.3611729670001,15.2,-1.80961908100001));
#266375=CARTESIAN_POINT('Ctrl Pts',(-10.3611729670001,11.6,-1.80961908100001));
#266376=CARTESIAN_POINT('Ctrl Pts',(-10.3628544100001,15.2,-1.81025075100001));
#266377=CARTESIAN_POINT('Ctrl Pts',(-10.3628544100001,11.6,-1.81025075100001));
#266378=CARTESIAN_POINT('Ctrl Pts',(-10.3645422430001,15.2,-1.81088659500002));
#266379=CARTESIAN_POINT('Ctrl Pts',(-10.3645422430001,11.6,-1.81088659500002));
#266380=CARTESIAN_POINT('Ctrl Pts',(-10.3662364440001,15.2,-1.81152662100001));
#266381=CARTESIAN_POINT('Ctrl Pts',(-10.3662364440001,11.6,-1.81152662100002));
#266382=CARTESIAN_POINT('Ctrl Pts',(-10.3679369930001,15.2,-1.81217083200002));
#266383=CARTESIAN_POINT('Ctrl Pts',(-10.3679369930001,11.6,-1.81217083200002));
#266384=CARTESIAN_POINT('Ctrl Pts',(-10.3696438710001,15.2,-1.81281923400002));
#266385=CARTESIAN_POINT('Ctrl Pts',(-10.3696438710001,11.6,-1.81281923400002));
#266386=CARTESIAN_POINT('Ctrl Pts',(-10.3713570580001,15.2,-1.81347183300002));
#266387=CARTESIAN_POINT('Ctrl Pts',(-10.3713570580001,11.6,-1.81347183300002));
#266388=CARTESIAN_POINT('Ctrl Pts',(-10.3730765340001,15.2,-1.81412863500002));
#266389=CARTESIAN_POINT('Ctrl Pts',(-10.3730765340001,11.6,-1.81412863500002));
#266390=CARTESIAN_POINT('Ctrl Pts',(-10.3748022770001,15.2,-1.81478964500001));
#266391=CARTESIAN_POINT('Ctrl Pts',(-10.3748022770001,11.6,-1.81478964500001));
#266392=CARTESIAN_POINT('Ctrl Pts',(-10.3765342700001,15.2,-1.81545487000002));
#266393=CARTESIAN_POINT('Ctrl Pts',(-10.3765342700001,11.6,-1.81545487000002));
#266394=CARTESIAN_POINT('Ctrl Pts',(-10.3782724920001,15.2,-1.81612431500001));
#266395=CARTESIAN_POINT('Ctrl Pts',(-10.3782724920001,11.6,-1.81612431500001));
#266396=CARTESIAN_POINT('Ctrl Pts',(-10.3800169250001,15.2,-1.81679798300001));
#266397=CARTESIAN_POINT('Ctrl Pts',(-10.3800169250001,11.6,-1.81679798300001));
#266398=CARTESIAN_POINT('Ctrl Pts',(-10.3817675460001,15.2,-1.81747588200002));
#266399=CARTESIAN_POINT('Ctrl Pts',(-10.3817675460001,11.6,-1.81747588200002));
#266400=CARTESIAN_POINT('Ctrl Pts',(-10.3835243380001,15.2,-1.81815801700001));
#266401=CARTESIAN_POINT('Ctrl Pts',(-10.3835243380001,11.6,-1.81815801700001));
#266402=CARTESIAN_POINT('Ctrl Pts',(-10.3852872810001,15.2,-1.81884439400001));
#266403=CARTESIAN_POINT('Ctrl Pts',(-10.3852872810001,11.6,-1.81884439400001));
#266404=CARTESIAN_POINT('Ctrl Pts',(-10.3870563570001,15.2,-1.81953501600002));
#266405=CARTESIAN_POINT('Ctrl Pts',(-10.3870563570001,11.6,-1.81953501600002));
#266406=CARTESIAN_POINT('Ctrl Pts',(-10.3888315440001,15.2,-1.82022989000002));
#266407=CARTESIAN_POINT('Ctrl Pts',(-10.3888315440001,11.6,-1.82022989000002));
#266408=CARTESIAN_POINT('Ctrl Pts',(-10.3906128240001,15.2,-1.82092902200001));
#266409=CARTESIAN_POINT('Ctrl Pts',(-10.3906128240001,11.6,-1.82092902200001));
#266410=CARTESIAN_POINT('Ctrl Pts',(-10.3924001790001,15.2,-1.82163241600001));
#266411=CARTESIAN_POINT('Ctrl Pts',(-10.3924001790001,11.6,-1.82163241600001));
#266412=CARTESIAN_POINT('Ctrl Pts',(-10.3941935880001,15.2,-1.82234007800002));
#266413=CARTESIAN_POINT('Ctrl Pts',(-10.3941935880001,11.6,-1.82234007800002));
#266414=CARTESIAN_POINT('Ctrl Pts',(-10.3959930320001,15.2,-1.82305201200001));
#266415=CARTESIAN_POINT('Ctrl Pts',(-10.3959930320001,11.6,-1.82305201200002));
#266416=CARTESIAN_POINT('Ctrl Pts',(-10.3977984930001,15.2,-1.82376822500002));
#266417=CARTESIAN_POINT('Ctrl Pts',(-10.3977984930001,11.6,-1.82376822500002));
#266418=CARTESIAN_POINT('Ctrl Pts',(-10.3996099520001,15.2,-1.82448872100001));
#266419=CARTESIAN_POINT('Ctrl Pts',(-10.3996099520001,11.6,-1.82448872100002));
#266420=CARTESIAN_POINT('Ctrl Pts',(-10.4014273890001,15.2,-1.82521350500001));
#266421=CARTESIAN_POINT('Ctrl Pts',(-10.4014273890001,11.6,-1.82521350500001));
#266422=CARTESIAN_POINT('Ctrl Pts',(-10.4032507880001,15.2,-1.82594258300002));
#266423=CARTESIAN_POINT('Ctrl Pts',(-10.4032507880001,11.6,-1.82594258300002));
#266424=CARTESIAN_POINT('Ctrl Pts',(-10.4050801260001,15.2,-1.82667595800002));
#266425=CARTESIAN_POINT('Ctrl Pts',(-10.4050801260001,11.6,-1.82667595800002));
#266426=CARTESIAN_POINT('Ctrl Pts',(-10.4069153870001,15.2,-1.82741363800002));
#266427=CARTESIAN_POINT('Ctrl Pts',(-10.4069153870001,11.6,-1.82741363800002));
#266428=CARTESIAN_POINT('Ctrl Pts',(-10.4087565520001,15.2,-1.82815562600001));
#266429=CARTESIAN_POINT('Ctrl Pts',(-10.4087565520001,11.6,-1.82815562600001));
#266430=CARTESIAN_POINT('Ctrl Pts',(-10.4106036030001,15.2,-1.82890192700001));
#266431=CARTESIAN_POINT('Ctrl Pts',(-10.4106036030001,11.6,-1.82890192700001));
#266432=CARTESIAN_POINT('Ctrl Pts',(-10.4124565210001,15.2,-1.82965254700001));
#266433=CARTESIAN_POINT('Ctrl Pts',(-10.4124565210001,11.6,-1.82965254700001));
#266434=CARTESIAN_POINT('Ctrl Pts',(-10.4143152860001,15.2,-1.83040749000002));
#266435=CARTESIAN_POINT('Ctrl Pts',(-10.4143152860001,11.6,-1.83040749000002));
#266436=CARTESIAN_POINT('Ctrl Pts',(-10.4161798810001,15.2,-1.83116676100001));
#266437=CARTESIAN_POINT('Ctrl Pts',(-10.4161798810001,11.6,-1.83116676100001));
#266438=CARTESIAN_POINT('Ctrl Pts',(-10.4180502880001,15.2,-1.83193036600001));
#266439=CARTESIAN_POINT('Ctrl Pts',(-10.4180502880001,11.6,-1.83193036600001));
#266440=CARTESIAN_POINT('Ctrl Pts',(-10.4199264880001,15.2,-1.83269830700001));
#266441=CARTESIAN_POINT('Ctrl Pts',(-10.4199264880001,11.6,-1.83269830700001));
#266442=CARTESIAN_POINT('Ctrl Pts',(-10.4218084630001,15.2,-1.83347059200001));
#266443=CARTESIAN_POINT('Ctrl Pts',(-10.4218084630001,11.6,-1.83347059200001));
#266444=CARTESIAN_POINT('Ctrl Pts',(-10.4236961950001,15.2,-1.83424722500002));
#266445=CARTESIAN_POINT('Ctrl Pts',(-10.4236961950001,11.6,-1.83424722500002));
#266446=CARTESIAN_POINT('Ctrl Pts',(-10.4255896650001,15.2,-1.83502820900001));
#266447=CARTESIAN_POINT('Ctrl Pts',(-10.4255896650001,11.6,-1.83502820900001));
#266448=CARTESIAN_POINT('Ctrl Pts',(-10.4274888570001,15.2,-1.83581355100001));
#266449=CARTESIAN_POINT('Ctrl Pts',(-10.4274888570001,11.6,-1.83581355100001));
#266450=CARTESIAN_POINT('Ctrl Pts',(-10.4293937510001,15.2,-1.83660325400002));
#266451=CARTESIAN_POINT('Ctrl Pts',(-10.4293937510001,11.6,-1.83660325400002));
#266452=CARTESIAN_POINT('Ctrl Pts',(-10.4313043290001,15.2,-1.83739732300001));
#266453=CARTESIAN_POINT('Ctrl Pts',(-10.4313043290001,11.6,-1.83739732300001));
#266454=CARTESIAN_POINT('Ctrl Pts',(-10.4332205740001,15.2,-1.83819576400001));
#266455=CARTESIAN_POINT('Ctrl Pts',(-10.4332205740001,11.6,-1.83819576400001));
#266456=CARTESIAN_POINT('Ctrl Pts',(-10.4351424680001,15.2,-1.83899858000002));
#266457=CARTESIAN_POINT('Ctrl Pts',(-10.4351424680001,11.6,-1.83899858000002));
#266458=CARTESIAN_POINT('Ctrl Pts',(-10.4370699940001,15.2,-1.83980577500002));
#266459=CARTESIAN_POINT('Ctrl Pts',(-10.4370699940001,11.6,-1.83980577500002));
#266460=CARTESIAN_POINT('Ctrl Pts',(-10.4390031330001,15.2,-1.84061735600002));
#266461=CARTESIAN_POINT('Ctrl Pts',(-10.4390031330001,11.6,-1.84061735600002));
#266462=CARTESIAN_POINT('Ctrl Pts',(-10.4409418670001,15.2,-1.84143332600001));
#266463=CARTESIAN_POINT('Ctrl Pts',(-10.4409418670001,11.6,-1.84143332600002));
#266464=CARTESIAN_POINT('Ctrl Pts',(-10.4428861800001,15.2,-1.84225369000002));
#266465=CARTESIAN_POINT('Ctrl Pts',(-10.4428861800001,11.6,-1.84225369000002));
#266466=CARTESIAN_POINT('Ctrl Pts',(-10.4448360520001,15.2,-1.84307845200001));
#266467=CARTESIAN_POINT('Ctrl Pts',(-10.4448360520001,11.6,-1.84307845200001));
#266468=CARTESIAN_POINT('Ctrl Pts',(-10.4467914690001,15.2,-1.84390761700001));
#266469=CARTESIAN_POINT('Ctrl Pts',(-10.4467914690001,11.6,-1.84390761700001));
#266470=CARTESIAN_POINT('Ctrl Pts',(-10.4487524110001,15.2,-1.84474118900001));
#266471=CARTESIAN_POINT('Ctrl Pts',(-10.4487524110001,11.6,-1.84474118900001));
#266472=CARTESIAN_POINT('Ctrl Pts',(-10.4507188600001,15.2,-1.84557917300001));
#266473=CARTESIAN_POINT('Ctrl Pts',(-10.4507188600001,11.6,-1.84557917300001));
#266474=CARTESIAN_POINT('Ctrl Pts',(-10.4526908010001,15.2,-1.84642157200001));
#266475=CARTESIAN_POINT('Ctrl Pts',(-10.4526908010001,11.6,-1.84642157200001));
#266476=CARTESIAN_POINT('Ctrl Pts',(-10.4546682150001,15.2,-1.84726839200001));
#266477=CARTESIAN_POINT('Ctrl Pts',(-10.4546682150001,11.6,-1.84726839200001));
#266478=CARTESIAN_POINT('Ctrl Pts',(-10.4566510860001,15.2,-1.84811963600001));
#266479=CARTESIAN_POINT('Ctrl Pts',(-10.4566510860001,11.6,-1.84811963600001));
#266480=CARTESIAN_POINT('Ctrl Pts',(-10.4586393950001,15.2,-1.84897530900002));
#266481=CARTESIAN_POINT('Ctrl Pts',(-10.4586393950001,11.6,-1.84897530900002));
#266482=CARTESIAN_POINT('Ctrl Pts',(-10.4606331260001,15.2,-1.84983541700001));
#266483=CARTESIAN_POINT('Ctrl Pts',(-10.4606331260001,11.6,-1.84983541700001));
#266484=CARTESIAN_POINT('Ctrl Pts',(-10.4626322630001,15.2,-1.85069996000002));
#266485=CARTESIAN_POINT('Ctrl Pts',(-10.4626322630001,11.6,-1.85069996000002));
#266486=CARTESIAN_POINT('Ctrl Pts',(-10.4646367870001,15.2,-1.85156894600001));
#266487=CARTESIAN_POINT('Ctrl Pts',(-10.4646367870001,11.6,-1.85156894600001));
#266488=CARTESIAN_POINT('Ctrl Pts',(-10.4666466810001,15.2,-1.85244237700001));
#266489=CARTESIAN_POINT('Ctrl Pts',(-10.4666466810001,11.6,-1.85244237700001));
#266490=CARTESIAN_POINT('Ctrl Pts',(-10.4686619290001,15.2,-1.85332026000002));
#266491=CARTESIAN_POINT('Ctrl Pts',(-10.4686619290001,11.6,-1.85332026000002));
#266492=CARTESIAN_POINT('Ctrl Pts',(-10.4706825140001,15.2,-1.85420259600001));
#266493=CARTESIAN_POINT('Ctrl Pts',(-10.4706825140001,11.6,-1.85420259600001));
#266494=CARTESIAN_POINT('Ctrl Pts',(-10.4727084200001,15.2,-1.85508939100002));
#266495=CARTESIAN_POINT('Ctrl Pts',(-10.4727084200001,11.6,-1.85508939100002));
#266496=CARTESIAN_POINT('Ctrl Pts',(-10.4747396280001,15.2,-1.85598064700002));
#266497=CARTESIAN_POINT('Ctrl Pts',(-10.4747396280001,11.6,-1.85598064700002));
#266498=CARTESIAN_POINT('Ctrl Pts',(-10.4767761230001,15.2,-1.85687637000001));
#266499=CARTESIAN_POINT('Ctrl Pts',(-10.4767761230001,11.6,-1.85687637000001));
#266500=CARTESIAN_POINT('Ctrl Pts',(-10.4788178880001,15.2,-1.85777656500001));
#266501=CARTESIAN_POINT('Ctrl Pts',(-10.4788178880001,11.6,-1.85777656500001));
#266502=CARTESIAN_POINT('Ctrl Pts',(-10.4808649060001,15.2,-1.85868123400001));
#266503=CARTESIAN_POINT('Ctrl Pts',(-10.4808649060001,11.6,-1.85868123400002));
#266504=CARTESIAN_POINT('Ctrl Pts',(-10.4829171610001,15.2,-1.85959038200001));
#266505=CARTESIAN_POINT('Ctrl Pts',(-10.4829171610001,11.6,-1.85959038200001));
#266506=CARTESIAN_POINT('Ctrl Pts',(-10.4849746350001,15.2,-1.86050401200001));
#266507=CARTESIAN_POINT('Ctrl Pts',(-10.4849746350001,11.6,-1.86050401200002));
#266508=CARTESIAN_POINT('Ctrl Pts',(-10.4870373130001,15.2,-1.86142212900001));
#266509=CARTESIAN_POINT('Ctrl Pts',(-10.4870373130001,11.6,-1.86142212900001));
#266510=CARTESIAN_POINT('Ctrl Pts',(-10.4891051780001,15.2,-1.86234473700001));
#266511=CARTESIAN_POINT('Ctrl Pts',(-10.4891051780001,11.6,-1.86234473700001));
#266512=CARTESIAN_POINT('Ctrl Pts',(-10.4911782130001,15.2,-1.86327184000001));
#266513=CARTESIAN_POINT('Ctrl Pts',(-10.4911782130001,11.6,-1.86327184000001));
#266514=CARTESIAN_POINT('Ctrl Pts',(-10.4932564020001,15.2,-1.86420344000001));
#266515=CARTESIAN_POINT('Ctrl Pts',(-10.4932564020001,11.6,-1.86420344000001));
#266516=CARTESIAN_POINT('Ctrl Pts',(-10.4953397300001,15.2,-1.86513954400001));
#266517=CARTESIAN_POINT('Ctrl Pts',(-10.4953397300001,11.6,-1.86513954400001));
#266518=CARTESIAN_POINT('Ctrl Pts',(-10.4974281790001,15.2,-1.86608015400001));
#266519=CARTESIAN_POINT('Ctrl Pts',(-10.4974281790001,11.6,-1.86608015400001));
#266520=CARTESIAN_POINT('Ctrl Pts',(-10.4995217330001,15.2,-1.86702527300001));
#266521=CARTESIAN_POINT('Ctrl Pts',(-10.4995217330001,11.6,-1.86702527300001));
#266522=CARTESIAN_POINT('Ctrl Pts',(-10.5016203770001,15.2,-1.86797490600001));
#266523=CARTESIAN_POINT('Ctrl Pts',(-10.5016203770001,11.6,-1.86797490600001));
#266524=CARTESIAN_POINT('Ctrl Pts',(-10.5037240940001,15.2,-1.86892905700001));
#266525=CARTESIAN_POINT('Ctrl Pts',(-10.5037240940001,11.6,-1.86892905700002));
#266526=CARTESIAN_POINT('Ctrl Pts',(-10.5058328690001,15.2,-1.86988772900001));
#266527=CARTESIAN_POINT('Ctrl Pts',(-10.5058328690001,11.6,-1.86988772900001));
#266528=CARTESIAN_POINT('Ctrl Pts',(-10.5079466830001,15.2,-1.87085092700002));
#266529=CARTESIAN_POINT('Ctrl Pts',(-10.5079466830001,11.6,-1.87085092700002));
#266530=CARTESIAN_POINT('Ctrl Pts',(-10.5100655220001,15.2,-1.87181865400001));
#266531=CARTESIAN_POINT('Ctrl Pts',(-10.5100655220001,11.6,-1.87181865400001));
#266532=CARTESIAN_POINT('Ctrl Pts',(-10.5121893710001,15.2,-1.87279091200002));
#266533=CARTESIAN_POINT('Ctrl Pts',(-10.5121893710001,11.6,-1.87279091200002));
#266534=CARTESIAN_POINT('Ctrl Pts',(-10.5143182130001,15.2,-1.87376770800002));
#266535=CARTESIAN_POINT('Ctrl Pts',(-10.5143182130001,11.6,-1.87376770800002));
#266536=CARTESIAN_POINT('Ctrl Pts',(-10.5164520310001,15.2,-1.87474904400001));
#266537=CARTESIAN_POINT('Ctrl Pts',(-10.5164520310001,11.6,-1.87474904400002));
#266538=CARTESIAN_POINT('Ctrl Pts',(-10.5185908110001,15.2,-1.87573492300002));
#266539=CARTESIAN_POINT('Ctrl Pts',(-10.5185908110001,11.6,-1.87573492300002));
#266540=CARTESIAN_POINT('Ctrl Pts',(-10.5207345370001,15.2,-1.87672534900001));
#266541=CARTESIAN_POINT('Ctrl Pts',(-10.5207345370001,11.6,-1.87672534900001));
#266542=CARTESIAN_POINT('Ctrl Pts',(-10.5228831920001,15.2,-1.87772032600002));
#266543=CARTESIAN_POINT('Ctrl Pts',(-10.5228831920001,11.6,-1.87772032600002));
#266544=CARTESIAN_POINT('Ctrl Pts',(-10.5250367610001,15.2,-1.87871985700002));
#266545=CARTESIAN_POINT('Ctrl Pts',(-10.5250367610001,11.6,-1.87871985700002));
#266546=CARTESIAN_POINT('Ctrl Pts',(-10.5271952300001,15.2,-1.87972394700001));
#266547=CARTESIAN_POINT('Ctrl Pts',(-10.5271952300001,11.6,-1.87972394700001));
#266548=CARTESIAN_POINT('Ctrl Pts',(-10.5293585800001,15.2,-1.88073259700001));
#266549=CARTESIAN_POINT('Ctrl Pts',(-10.5293585800001,11.6,-1.88073259700001));
#266550=CARTESIAN_POINT('Ctrl Pts',(-10.5315267990001,15.2,-1.88174581200002));
#266551=CARTESIAN_POINT('Ctrl Pts',(-10.5315267990001,11.6,-1.88174581200002));
#266552=CARTESIAN_POINT('Ctrl Pts',(-10.5336998690001,15.2,-1.88276359700001));
#266553=CARTESIAN_POINT('Ctrl Pts',(-10.5336998690001,11.6,-1.88276359700001));
#266554=CARTESIAN_POINT('Ctrl Pts',(-10.5358777760001,15.2,-1.88378595200001));
#266555=CARTESIAN_POINT('Ctrl Pts',(-10.5358777760001,11.6,-1.88378595200001));
#266556=CARTESIAN_POINT('Ctrl Pts',(-10.5380605030001,15.2,-1.88481288500002));
#266557=CARTESIAN_POINT('Ctrl Pts',(-10.5380605030001,11.6,-1.88481288500002));
#266558=CARTESIAN_POINT('Ctrl Pts',(-10.5402480350001,15.2,-1.88584439400001));
#266559=CARTESIAN_POINT('Ctrl Pts',(-10.5402480350001,11.6,-1.88584439400001));
#266560=CARTESIAN_POINT('Ctrl Pts',(-10.5424403580001,15.2,-1.88688048700001));
#266561=CARTESIAN_POINT('Ctrl Pts',(-10.5424403580001,11.6,-1.88688048700001));
#266562=CARTESIAN_POINT('Ctrl Pts',(-10.5446374560001,15.2,-1.88792116400001));
#266563=CARTESIAN_POINT('Ctrl Pts',(-10.5446374560001,11.6,-1.88792116400002));
#266564=CARTESIAN_POINT('Ctrl Pts',(-10.5468393120001,15.2,-1.88896643200001));
#266565=CARTESIAN_POINT('Ctrl Pts',(-10.5468393120001,11.6,-1.88896643200001));
#266566=CARTESIAN_POINT('Ctrl Pts',(-10.5490459140001,15.2,-1.89001629000002));
#266567=CARTESIAN_POINT('Ctrl Pts',(-10.5490459140001,11.6,-1.89001629000002));
#266568=CARTESIAN_POINT('Ctrl Pts',(-10.5512572450001,15.2,-1.89107074500001));
#266569=CARTESIAN_POINT('Ctrl Pts',(-10.5512572450001,11.6,-1.89107074500001));
#266570=CARTESIAN_POINT('Ctrl Pts',(-10.5534732880001,15.2,-1.89212980000002));
#266571=CARTESIAN_POINT('Ctrl Pts',(-10.5534732880001,11.6,-1.89212980000002));
#266572=CARTESIAN_POINT('Ctrl Pts',(-10.5556940320001,15.2,-1.89319345500001));
#266573=CARTESIAN_POINT('Ctrl Pts',(-10.5556940320001,11.6,-1.89319345500001));
#266574=CARTESIAN_POINT('Ctrl Pts',(-10.5579194590001,15.2,-1.89426171700001));
#266575=CARTESIAN_POINT('Ctrl Pts',(-10.5579194590001,11.6,-1.89426171700001));
#266576=CARTESIAN_POINT('Ctrl Pts',(-10.5601495550001,15.2,-1.89533458700001));
#266577=CARTESIAN_POINT('Ctrl Pts',(-10.5601495550001,11.6,-1.89533458700002));
#266578=CARTESIAN_POINT('Ctrl Pts',(-10.5623843040001,15.2,-1.89641206900002));
#266579=CARTESIAN_POINT('Ctrl Pts',(-10.5623843040001,11.6,-1.89641206900002));
#266580=CARTESIAN_POINT('Ctrl Pts',(-10.5646236920001,15.2,-1.89749416600002));
#266581=CARTESIAN_POINT('Ctrl Pts',(-10.5646236920001,11.6,-1.89749416600002));
#266582=CARTESIAN_POINT('Ctrl Pts',(-10.5668677030001,15.2,-1.89858088200001));
#266583=CARTESIAN_POINT('Ctrl Pts',(-10.5668677030001,11.6,-1.89858088200001));
#266584=CARTESIAN_POINT('Ctrl Pts',(-10.5691163240001,15.2,-1.89967222000002));
#266585=CARTESIAN_POINT('Ctrl Pts',(-10.5691163240001,11.6,-1.89967222000002));
#266586=CARTESIAN_POINT('Ctrl Pts',(-10.5713695390001,15.2,-1.90076818100001));
#266587=CARTESIAN_POINT('Ctrl Pts',(-10.5713695390001,11.6,-1.90076818100001));
#266588=CARTESIAN_POINT('Ctrl Pts',(-10.5736273340001,15.2,-1.90186877100002));
#266589=CARTESIAN_POINT('Ctrl Pts',(-10.5736273340001,11.6,-1.90186877100002));
#266590=CARTESIAN_POINT('Ctrl Pts',(-10.5758896930001,15.2,-1.90297399200002));
#266591=CARTESIAN_POINT('Ctrl Pts',(-10.5758896930001,11.6,-1.90297399200002));
#266592=CARTESIAN_POINT('Ctrl Pts',(-10.5781566020001,15.2,-1.90408384600001));
#266593=CARTESIAN_POINT('Ctrl Pts',(-10.5781566020001,11.6,-1.90408384600001));
#266594=CARTESIAN_POINT('Ctrl Pts',(-10.5804280450001,15.2,-1.90519833800002));
#266595=CARTESIAN_POINT('Ctrl Pts',(-10.5804280450001,11.6,-1.90519833800002));
#266596=CARTESIAN_POINT('Ctrl Pts',(-10.5827040090001,15.2,-1.90631747000001));
#266597=CARTESIAN_POINT('Ctrl Pts',(-10.5827040090001,11.6,-1.90631747000001));
#266598=CARTESIAN_POINT('Ctrl Pts',(-10.5849844800001,15.2,-1.90744124500001));
#266599=CARTESIAN_POINT('Ctrl Pts',(-10.5849844800001,11.6,-1.90744124500001));
#266600=CARTESIAN_POINT('Ctrl Pts',(-10.5872694410001,15.2,-1.90856966700002));
#266601=CARTESIAN_POINT('Ctrl Pts',(-10.5872694410001,11.6,-1.90856966700002));
#266602=CARTESIAN_POINT('Ctrl Pts',(-10.5895588790001,15.2,-1.90970273700001));
#266603=CARTESIAN_POINT('Ctrl Pts',(-10.5895588790001,11.6,-1.90970273700001));
#266604=CARTESIAN_POINT('Ctrl Pts',(-10.5918527800001,15.2,-1.91084046000002));
#266605=CARTESIAN_POINT('Ctrl Pts',(-10.5918527800001,11.6,-1.91084046000002));
#266606=CARTESIAN_POINT('Ctrl Pts',(-10.5941511290001,15.2,-1.91198283800002));
#266607=CARTESIAN_POINT('Ctrl Pts',(-10.5941511290001,11.6,-1.91198283800002));
#266608=CARTESIAN_POINT('Ctrl Pts',(-10.5964539110001,15.2,-1.91312987400002));
#266609=CARTESIAN_POINT('Ctrl Pts',(-10.5964539110001,11.6,-1.91312987400002));
#266610=CARTESIAN_POINT('Ctrl Pts',(-10.5987611120001,15.2,-1.91428157100002));
#266611=CARTESIAN_POINT('Ctrl Pts',(-10.5987611120001,11.6,-1.91428157100002));
#266612=CARTESIAN_POINT('Ctrl Pts',(-10.6010727180001,15.2,-1.91543793200001));
#266613=CARTESIAN_POINT('Ctrl Pts',(-10.6010727180001,11.6,-1.91543793200002));
#266614=CARTESIAN_POINT('Ctrl Pts',(-10.6033887130001,15.2,-1.91659895900001));
#266615=CARTESIAN_POINT('Ctrl Pts',(-10.6033887130001,11.6,-1.91659895900001));
#266616=CARTESIAN_POINT('Ctrl Pts',(-10.6057090860001,15.2,-1.91776465800002));
#266617=CARTESIAN_POINT('Ctrl Pts',(-10.6057090860001,11.6,-1.91776465800002));
#266618=CARTESIAN_POINT('Ctrl Pts',(-10.6080338200001,15.2,-1.91893502800002));
#266619=CARTESIAN_POINT('Ctrl Pts',(-10.6080338200001,11.6,-1.91893502800002));
#266620=CARTESIAN_POINT('Ctrl Pts',(-10.6103629020001,15.2,-1.92011007300001));
#266621=CARTESIAN_POINT('Ctrl Pts',(-10.6103629020001,11.6,-1.92011007300001));
#266622=CARTESIAN_POINT('Ctrl Pts',(-10.6126963170001,15.2,-1.92128979600001));
#266623=CARTESIAN_POINT('Ctrl Pts',(-10.6126963170001,11.6,-1.92128979600001));
#266624=CARTESIAN_POINT('Ctrl Pts',(-10.6150340510001,15.2,-1.92247420100002));
#266625=CARTESIAN_POINT('Ctrl Pts',(-10.6150340510001,11.6,-1.92247420100002));
#266626=CARTESIAN_POINT('Ctrl Pts',(-10.6173760910001,15.2,-1.92366329000001));
#266627=CARTESIAN_POINT('Ctrl Pts',(-10.6173760910001,11.6,-1.92366329000001));
#266628=CARTESIAN_POINT('Ctrl Pts',(-10.6197224210001,15.2,-1.92485706400001));
#266629=CARTESIAN_POINT('Ctrl Pts',(-10.6197224210001,11.6,-1.92485706400001));
#266630=CARTESIAN_POINT('Ctrl Pts',(-10.6220730290001,15.2,-1.92605552900002));
#266631=CARTESIAN_POINT('Ctrl Pts',(-10.6220730290001,11.6,-1.92605552900002));
#266632=CARTESIAN_POINT('Ctrl Pts',(-10.6244279010001,15.2,-1.92725868500002));
#266633=CARTESIAN_POINT('Ctrl Pts',(-10.6244279010001,11.6,-1.92725868500002));
#266634=CARTESIAN_POINT('Ctrl Pts',(-10.6267870210001,15.2,-1.92846653600002));
#266635=CARTESIAN_POINT('Ctrl Pts',(-10.6267870210001,11.6,-1.92846653600002));
#266636=CARTESIAN_POINT('Ctrl Pts',(-10.6291503760001,15.2,-1.92967908500002));
#266637=CARTESIAN_POINT('Ctrl Pts',(-10.6291503760001,11.6,-1.92967908500002));
#266638=CARTESIAN_POINT('Ctrl Pts',(-10.6315179530001,15.2,-1.93089633400001));
#266639=CARTESIAN_POINT('Ctrl Pts',(-10.6315179530001,11.6,-1.93089633400001));
#266640=CARTESIAN_POINT('Ctrl Pts',(-10.6338897380001,15.2,-1.93211828500001));
#266641=CARTESIAN_POINT('Ctrl Pts',(-10.6338897380001,11.6,-1.93211828500001));
#266642=CARTESIAN_POINT('Ctrl Pts',(-10.6362657160001,15.2,-1.93334494300001));
#266643=CARTESIAN_POINT('Ctrl Pts',(-10.6362657160001,11.6,-1.93334494300002));
#266644=CARTESIAN_POINT('Ctrl Pts',(-10.6386458730001,15.2,-1.93457630700001));
#266645=CARTESIAN_POINT('Ctrl Pts',(-10.6386458730001,11.6,-1.93457630700001));
#266646=CARTESIAN_POINT('Ctrl Pts',(-10.6410301980001,15.2,-1.93581238300002));
#266647=CARTESIAN_POINT('Ctrl Pts',(-10.6410301980001,11.6,-1.93581238300002));
#266648=CARTESIAN_POINT('Ctrl Pts',(-10.6434186740001,15.2,-1.93705317200001));
#266649=CARTESIAN_POINT('Ctrl Pts',(-10.6434186740001,11.6,-1.93705317200001));
#266650=CARTESIAN_POINT('Ctrl Pts',(-10.6458112890001,15.2,-1.93829867700002));
#266651=CARTESIAN_POINT('Ctrl Pts',(-10.6458112890001,11.6,-1.93829867700002));
#266652=CARTESIAN_POINT('Ctrl Pts',(-10.6482080300001,15.2,-1.93954890100001));
#266653=CARTESIAN_POINT('Ctrl Pts',(-10.6482080300001,11.6,-1.93954890100001));
#266654=CARTESIAN_POINT('Ctrl Pts',(-10.6506088810001,15.2,-1.94080384500001));
#266655=CARTESIAN_POINT('Ctrl Pts',(-10.6506088810001,11.6,-1.94080384500001));
#266656=CARTESIAN_POINT('Ctrl Pts',(-10.6530138300001,15.2,-1.94206351200001));
#266657=CARTESIAN_POINT('Ctrl Pts',(-10.6530138300001,11.6,-1.94206351200001));
#266658=CARTESIAN_POINT('Ctrl Pts',(-10.6554228640001,15.2,-1.94332790700001));
#266659=CARTESIAN_POINT('Ctrl Pts',(-10.6554228640001,11.6,-1.94332790700001));
#266660=CARTESIAN_POINT('Ctrl Pts',(-10.6578359690001,15.2,-1.94459703000001));
#266661=CARTESIAN_POINT('Ctrl Pts',(-10.6578359690001,11.6,-1.94459703000002));
#266662=CARTESIAN_POINT('Ctrl Pts',(-10.6602531300001,15.2,-1.94587088200001));
#266663=CARTESIAN_POINT('Ctrl Pts',(-10.6602531300001,11.6,-1.94587088200001));
#266664=CARTESIAN_POINT('Ctrl Pts',(-10.6626743350001,15.2,-1.94714946900001));
#266665=CARTESIAN_POINT('Ctrl Pts',(-10.6626743350001,11.6,-1.94714946900001));
#266666=CARTESIAN_POINT('Ctrl Pts',(-10.6650995710001,15.2,-1.94843279300001));
#266667=CARTESIAN_POINT('Ctrl Pts',(-10.6650995710001,11.6,-1.94843279300001));
#266668=CARTESIAN_POINT('Ctrl Pts',(-10.6675288230001,15.2,-1.94972085400002));
#266669=CARTESIAN_POINT('Ctrl Pts',(-10.6675288230001,11.6,-1.94972085400002));
#266670=CARTESIAN_POINT('Ctrl Pts',(-10.6699620800001,15.2,-1.95101365600001));
#266671=CARTESIAN_POINT('Ctrl Pts',(-10.6699620800001,11.6,-1.95101365600001));
#266672=CARTESIAN_POINT('Ctrl Pts',(-10.6723993270001,15.2,-1.95231120100001));
#266673=CARTESIAN_POINT('Ctrl Pts',(-10.6723993270001,11.6,-1.95231120100001));
#266674=CARTESIAN_POINT('Ctrl Pts',(-10.6748405500001,15.2,-1.95361349100001));
#266675=CARTESIAN_POINT('Ctrl Pts',(-10.6748405500001,11.6,-1.95361349100002));
#266676=CARTESIAN_POINT('Ctrl Pts',(-10.6772857370001,15.2,-1.95492053000001));
#266677=CARTESIAN_POINT('Ctrl Pts',(-10.6772857370001,11.6,-1.95492053000002));
#266678=CARTESIAN_POINT('Ctrl Pts',(-10.6797348740001,15.2,-1.95623231900001));
#266679=CARTESIAN_POINT('Ctrl Pts',(-10.6797348740001,11.6,-1.95623231900001));
#266680=CARTESIAN_POINT('Ctrl Pts',(-10.6821879490001,15.2,-1.95754886000001));
#266681=CARTESIAN_POINT('Ctrl Pts',(-10.6821879490001,11.6,-1.95754886000001));
#266682=CARTESIAN_POINT('Ctrl Pts',(-10.6846449480001,15.2,-1.95887015700002));
#266683=CARTESIAN_POINT('Ctrl Pts',(-10.6846449480001,11.6,-1.95887015700002));
#266684=CARTESIAN_POINT('Ctrl Pts',(-10.6871058570001,15.2,-1.96019621100001));
#266685=CARTESIAN_POINT('Ctrl Pts',(-10.6871058570001,11.6,-1.96019621100001));
#266686=CARTESIAN_POINT('Ctrl Pts',(-10.6895706640001,15.2,-1.96152702300001));
#266687=CARTESIAN_POINT('Ctrl Pts',(-10.6895706640001,11.6,-1.96152702300001));
#266688=CARTESIAN_POINT('Ctrl Pts',(-10.6920393560001,15.2,-1.96286259900001));
#266689=CARTESIAN_POINT('Ctrl Pts',(-10.6920393560001,11.6,-1.96286259900001));
#266690=CARTESIAN_POINT('Ctrl Pts',(-10.6945119200001,15.2,-1.96420293800001));
#266691=CARTESIAN_POINT('Ctrl Pts',(-10.6945119200001,11.6,-1.96420293800002));
#266692=CARTESIAN_POINT('Ctrl Pts',(-10.6969883420001,15.2,-1.96554804400002));
#266693=CARTESIAN_POINT('Ctrl Pts',(-10.6969883420001,11.6,-1.96554804400002));
#266694=CARTESIAN_POINT('Ctrl Pts',(-10.6994686090001,15.2,-1.96689791700001));
#266695=CARTESIAN_POINT('Ctrl Pts',(-10.6994686090001,11.6,-1.96689791700001));
#266696=CARTESIAN_POINT('Ctrl Pts',(-10.7019527100001,15.2,-1.96825256300002));
#266697=CARTESIAN_POINT('Ctrl Pts',(-10.7019527100001,11.6,-1.96825256300002));
#266698=CARTESIAN_POINT('Ctrl Pts',(-10.7044406300001,15.2,-1.96961198000002));
#266699=CARTESIAN_POINT('Ctrl Pts',(-10.7044406300001,11.6,-1.96961198000002));
#266700=CARTESIAN_POINT('Ctrl Pts',(-10.7069323560001,15.2,-1.97097617300001));
#266701=CARTESIAN_POINT('Ctrl Pts',(-10.7069323560001,11.6,-1.97097617300001));
#266702=CARTESIAN_POINT('Ctrl Pts',(-10.7094278770001,15.2,-1.97234514300002));
#266703=CARTESIAN_POINT('Ctrl Pts',(-10.7094278770001,11.6,-1.97234514300002));
#266704=CARTESIAN_POINT('Ctrl Pts',(-10.7119271780001,15.2,-1.97371889300001));
#266705=CARTESIAN_POINT('Ctrl Pts',(-10.7119271780001,11.6,-1.97371889300001));
#266706=CARTESIAN_POINT('Ctrl Pts',(-10.7144302480001,15.2,-1.97509742500001));
#266707=CARTESIAN_POINT('Ctrl Pts',(-10.7144302480001,11.6,-1.97509742500001));
#266708=CARTESIAN_POINT('Ctrl Pts',(-10.7169370730001,15.2,-1.97648074000002));
#266709=CARTESIAN_POINT('Ctrl Pts',(-10.7169370730001,11.6,-1.97648074000002));
#266710=CARTESIAN_POINT('Ctrl Pts',(-10.7194476400001,15.2,-1.97786884100001));
#266711=CARTESIAN_POINT('Ctrl Pts',(-10.7194476400001,11.6,-1.97786884100001));
#266712=CARTESIAN_POINT('Ctrl Pts',(-10.7219619380001,15.2,-1.97926173000001));
#266713=CARTESIAN_POINT('Ctrl Pts',(-10.7219619380001,11.6,-1.97926173000001));
#266714=CARTESIAN_POINT('Ctrl Pts',(-10.7244799520001,15.2,-1.98065940900001));
#266715=CARTESIAN_POINT('Ctrl Pts',(-10.7244799520001,11.6,-1.98065940900001));
#266716=CARTESIAN_POINT('Ctrl Pts',(-10.7270016720001,15.2,-1.98206188000002));
#266717=CARTESIAN_POINT('Ctrl Pts',(-10.7270016720001,11.6,-1.98206188000002));
#266718=CARTESIAN_POINT('Ctrl Pts',(-10.7295270830001,15.2,-1.98346914600001));
#266719=CARTESIAN_POINT('Ctrl Pts',(-10.7295270830001,11.6,-1.98346914600001));
#266720=CARTESIAN_POINT('Ctrl Pts',(-10.7320561730001,15.2,-1.98488120800001));
#266721=CARTESIAN_POINT('Ctrl Pts',(-10.7320561730001,11.6,-1.98488120800001));
#266722=CARTESIAN_POINT('Ctrl Pts',(-10.7345889310001,15.2,-1.98629806800001));
#266723=CARTESIAN_POINT('Ctrl Pts',(-10.7345889310001,11.6,-1.98629806800001));
#266724=CARTESIAN_POINT('Ctrl Pts',(-10.7371253410001,15.2,-1.98771972800001));
#266725=CARTESIAN_POINT('Ctrl Pts',(-10.7371253410001,11.6,-1.98771972800001));
#266726=CARTESIAN_POINT('Ctrl Pts',(-10.7396653940001,15.2,-1.98914619100002));
#266727=CARTESIAN_POINT('Ctrl Pts',(-10.7396653940001,11.6,-1.98914619100002));
#266728=CARTESIAN_POINT('Ctrl Pts',(-10.7422090760001,15.2,-1.99057745700001));
#266729=CARTESIAN_POINT('Ctrl Pts',(-10.7422090760001,11.6,-1.99057745700001));
#266730=CARTESIAN_POINT('Ctrl Pts',(-10.7447563740001,15.2,-1.99201353000001));
#266731=CARTESIAN_POINT('Ctrl Pts',(-10.7447563740001,11.6,-1.99201353000001));
#266732=CARTESIAN_POINT('Ctrl Pts',(-10.7473072760001,15.2,-1.99345441100002));
#266733=CARTESIAN_POINT('Ctrl Pts',(-10.7473072760001,11.6,-1.99345441100002));
#266734=CARTESIAN_POINT('Ctrl Pts',(-10.7498617710001,15.2,-1.99490010200002));
#266735=CARTESIAN_POINT('Ctrl Pts',(-10.7498617710001,11.6,-1.99490010200002));
#266736=CARTESIAN_POINT('Ctrl Pts',(-10.7524198440001,15.2,-1.99635060600002));
#266737=CARTESIAN_POINT('Ctrl Pts',(-10.7524198440001,11.6,-1.99635060600002));
#266738=CARTESIAN_POINT('Ctrl Pts',(-10.7549814840001,15.2,-1.99780592200002));
#266739=CARTESIAN_POINT('Ctrl Pts',(-10.7549814840001,11.6,-1.99780592200002));
#266740=CARTESIAN_POINT('Ctrl Pts',(-10.7575466780001,15.2,-1.99926605500002));
#266741=CARTESIAN_POINT('Ctrl Pts',(-10.7575466780001,11.6,-1.99926605500002));
#266742=CARTESIAN_POINT('Ctrl Pts',(-10.7601154160001,15.2,-2.00073100600001));
#266743=CARTESIAN_POINT('Ctrl Pts',(-10.7601154160001,11.6,-2.00073100600001));
#266744=CARTESIAN_POINT('Ctrl Pts',(-10.7626876820001,15.2,-2.00220077700001));
#266745=CARTESIAN_POINT('Ctrl Pts',(-10.7626876820001,11.6,-2.00220077700001));
#266746=CARTESIAN_POINT('Ctrl Pts',(-10.7652634670001,15.2,-2.00367536800002));
#266747=CARTESIAN_POINT('Ctrl Pts',(-10.7652634670001,11.6,-2.00367536800002));
#266748=CARTESIAN_POINT('Ctrl Pts',(-10.7678427560001,15.2,-2.00515478300002));
#266749=CARTESIAN_POINT('Ctrl Pts',(-10.7678427560001,11.6,-2.00515478300002));
#266750=CARTESIAN_POINT('Ctrl Pts',(-10.7704255400001,15.2,-2.00663902300001));
#266751=CARTESIAN_POINT('Ctrl Pts',(-10.7704255400001,11.6,-2.00663902300001));
#266752=CARTESIAN_POINT('Ctrl Pts',(-10.7730118040001,15.2,-2.00812809000002));
#266753=CARTESIAN_POINT('Ctrl Pts',(-10.7730118040001,11.6,-2.00812809000002));
#266754=CARTESIAN_POINT('Ctrl Pts',(-10.7756015380001,15.2,-2.00962198600001));
#266755=CARTESIAN_POINT('Ctrl Pts',(-10.7756015380001,11.6,-2.00962198600001));
#266756=CARTESIAN_POINT('Ctrl Pts',(-10.7781947270001,15.2,-2.01112071200001));
#266757=CARTESIAN_POINT('Ctrl Pts',(-10.7781947270001,11.6,-2.01112071200001));
#266758=CARTESIAN_POINT('Ctrl Pts',(-10.7807913610001,15.2,-2.01262427100001));
#266759=CARTESIAN_POINT('Ctrl Pts',(-10.7807913610001,11.6,-2.01262427100001));
#266760=CARTESIAN_POINT('Ctrl Pts',(-10.7833914290001,15.2,-2.01413266400001));
#266761=CARTESIAN_POINT('Ctrl Pts',(-10.7833914290001,11.6,-2.01413266400001));
#266762=CARTESIAN_POINT('Ctrl Pts',(-10.7859949160001,15.2,-2.01564589300002));
#266763=CARTESIAN_POINT('Ctrl Pts',(-10.7859949160001,11.6,-2.01564589300002));
#266764=CARTESIAN_POINT('Ctrl Pts',(-10.7886018120001,15.2,-2.01716395900001));
#266765=CARTESIAN_POINT('Ctrl Pts',(-10.7886018120001,11.6,-2.01716395900001));
#266766=CARTESIAN_POINT('Ctrl Pts',(-10.7912121050001,15.2,-2.01868686500001));
#266767=CARTESIAN_POINT('Ctrl Pts',(-10.7912121050001,11.6,-2.01868686500001));
#266768=CARTESIAN_POINT('Ctrl Pts',(-10.7938257820001,15.2,-2.02021461100002));
#266769=CARTESIAN_POINT('Ctrl Pts',(-10.7938257820001,11.6,-2.02021461100002));
#266770=CARTESIAN_POINT('Ctrl Pts',(-10.7964428320001,15.2,-2.02174720000002));
#266771=CARTESIAN_POINT('Ctrl Pts',(-10.7964428320001,11.6,-2.02174720000002));
#266772=CARTESIAN_POINT('Ctrl Pts',(-10.7990632420001,15.2,-2.02328463400002));
#266773=CARTESIAN_POINT('Ctrl Pts',(-10.7990632420001,11.6,-2.02328463400002));
#266774=CARTESIAN_POINT('Ctrl Pts',(-10.8016870010001,15.2,-2.02482691400002));
#266775=CARTESIAN_POINT('Ctrl Pts',(-10.8016870010001,11.6,-2.02482691400002));
#266776=CARTESIAN_POINT('Ctrl Pts',(-10.8043140960001,15.2,-2.02637404200001));
#266777=CARTESIAN_POINT('Ctrl Pts',(-10.8043140960001,11.6,-2.02637404200001));
#266778=CARTESIAN_POINT('Ctrl Pts',(-10.8069445180001,15.2,-2.02792601900001));
#266779=CARTESIAN_POINT('Ctrl Pts',(-10.8069445180001,11.6,-2.02792601900002));
#266780=CARTESIAN_POINT('Ctrl Pts',(-10.8095782520001,15.2,-2.02948284700001));
#266781=CARTESIAN_POINT('Ctrl Pts',(-10.8095782520001,11.6,-2.02948284700002));
#266782=CARTESIAN_POINT('Ctrl Pts',(-10.8122152870001,15.2,-2.03104452700002));
#266783=CARTESIAN_POINT('Ctrl Pts',(-10.8122152870001,11.6,-2.03104452700002));
#266784=CARTESIAN_POINT('Ctrl Pts',(-10.8148556120001,15.2,-2.03261106200001));
#266785=CARTESIAN_POINT('Ctrl Pts',(-10.8148556120001,11.6,-2.03261106200001));
#266786=CARTESIAN_POINT('Ctrl Pts',(-10.8174992140001,15.2,-2.03418245300002));
#266787=CARTESIAN_POINT('Ctrl Pts',(-10.8174992140001,11.6,-2.03418245300002));
#266788=CARTESIAN_POINT('Ctrl Pts',(-10.8201460830001,15.2,-2.03575870100002));
#266789=CARTESIAN_POINT('Ctrl Pts',(-10.8201460830001,11.6,-2.03575870100002));
#266790=CARTESIAN_POINT('Ctrl Pts',(-10.8227962070001,15.2,-2.03733980800001));
#266791=CARTESIAN_POINT('Ctrl Pts',(-10.8227962070001,11.6,-2.03733980800001));
#266792=CARTESIAN_POINT('Ctrl Pts',(-10.8254495730001,15.2,-2.03892577600001));
#266793=CARTESIAN_POINT('Ctrl Pts',(-10.8254495730001,11.6,-2.03892577600001));
#266794=CARTESIAN_POINT('Ctrl Pts',(-10.8281061700001,15.2,-2.04051660600001));
#266795=CARTESIAN_POINT('Ctrl Pts',(-10.8281061700001,11.6,-2.04051660600001));
#266796=CARTESIAN_POINT('Ctrl Pts',(-10.8307659860001,15.2,-2.04211229900002));
#266797=CARTESIAN_POINT('Ctrl Pts',(-10.8307659860001,11.6,-2.04211229900002));
#266798=CARTESIAN_POINT('Ctrl Pts',(-10.8334290110001,15.2,-2.04371285800002));
#266799=CARTESIAN_POINT('Ctrl Pts',(-10.8334290110001,11.6,-2.04371285800002));
#266800=CARTESIAN_POINT('Ctrl Pts',(-10.8360952310001,15.2,-2.04531828300002));
#266801=CARTESIAN_POINT('Ctrl Pts',(-10.8360952310001,11.6,-2.04531828300002));
#266802=CARTESIAN_POINT('Ctrl Pts',(-10.8387646370001,15.2,-2.04692857600001));
#266803=CARTESIAN_POINT('Ctrl Pts',(-10.8387646370001,11.6,-2.04692857600001));
#266804=CARTESIAN_POINT('Ctrl Pts',(-10.8414372150001,15.2,-2.04854373900002));
#266805=CARTESIAN_POINT('Ctrl Pts',(-10.8414372150001,11.6,-2.04854373900002));
#266806=CARTESIAN_POINT('Ctrl Pts',(-10.8441129560001,15.2,-2.05016377300002));
#266807=CARTESIAN_POINT('Ctrl Pts',(-10.8441129560001,11.6,-2.05016377300002));
#266808=CARTESIAN_POINT('Ctrl Pts',(-10.8467918470001,15.2,-2.05178868100001));
#266809=CARTESIAN_POINT('Ctrl Pts',(-10.8467918470001,11.6,-2.05178868100001));
#266810=CARTESIAN_POINT('Ctrl Pts',(-10.8494738750001,15.2,-2.05341846100001));
#266811=CARTESIAN_POINT('Ctrl Pts',(-10.8494738750001,11.6,-2.05341846100001));
#266812=CARTESIAN_POINT('Ctrl Pts',(-10.8521590310001,15.2,-2.05505311700001));
#266813=CARTESIAN_POINT('Ctrl Pts',(-10.8521590310001,11.6,-2.05505311700001));
#266814=CARTESIAN_POINT('Ctrl Pts',(-10.8548473040001,15.2,-2.05669265100001));
#266815=CARTESIAN_POINT('Ctrl Pts',(-10.8548473040001,11.6,-2.05669265100001));
#266816=CARTESIAN_POINT('Ctrl Pts',(-10.8575386810001,15.2,-2.05833706200002));
#266817=CARTESIAN_POINT('Ctrl Pts',(-10.8575386810001,11.6,-2.05833706200002));
#266818=CARTESIAN_POINT('Ctrl Pts',(-10.8602331500001,15.2,-2.05998635300002));
#266819=CARTESIAN_POINT('Ctrl Pts',(-10.8602331500001,11.6,-2.05998635300002));
#266820=CARTESIAN_POINT('Ctrl Pts',(-10.8629307020001,15.2,-2.06164052600001));
#266821=CARTESIAN_POINT('Ctrl Pts',(-10.8629307020001,11.6,-2.06164052600002));
#266822=CARTESIAN_POINT('Ctrl Pts',(-10.8656313230001,15.2,-2.06329958000001));
#266823=CARTESIAN_POINT('Ctrl Pts',(-10.8656313230001,11.6,-2.06329958000001));
#266824=CARTESIAN_POINT('Ctrl Pts',(-10.8683350050001,15.2,-2.06496352000002));
#266825=CARTESIAN_POINT('Ctrl Pts',(-10.8683350050001,11.6,-2.06496352000002));
#266826=CARTESIAN_POINT('Ctrl Pts',(-10.8710417330001,15.2,-2.06663234400001));
#266827=CARTESIAN_POINT('Ctrl Pts',(-10.8710417330001,11.6,-2.06663234400001));
#266828=CARTESIAN_POINT('Ctrl Pts',(-10.8737514990001,15.2,-2.06830605400001));
#266829=CARTESIAN_POINT('Ctrl Pts',(-10.8737514990001,11.6,-2.06830605400001));
#266830=CARTESIAN_POINT('Ctrl Pts',(-10.8764642900001,15.2,-2.06998465200002));
#266831=CARTESIAN_POINT('Ctrl Pts',(-10.8764642900001,11.6,-2.06998465200002));
#266832=CARTESIAN_POINT('Ctrl Pts',(-10.8791800940001,15.2,-2.07166814000002));
#266833=CARTESIAN_POINT('Ctrl Pts',(-10.8791800940001,11.6,-2.07166814000002));
#266834=CARTESIAN_POINT('Ctrl Pts',(-10.8818989020001,15.2,-2.07335651800001));
#266835=CARTESIAN_POINT('Ctrl Pts',(-10.8818989020001,11.6,-2.07335651800001));
#266836=CARTESIAN_POINT('Ctrl Pts',(-10.8846207020001,15.2,-2.07504978700001));
#266837=CARTESIAN_POINT('Ctrl Pts',(-10.8846207020001,11.6,-2.07504978700001));
#266838=CARTESIAN_POINT('Ctrl Pts',(-10.8873454820001,15.2,-2.07674795000001));
#266839=CARTESIAN_POINT('Ctrl Pts',(-10.8873454820001,11.6,-2.07674795000001));
#266840=CARTESIAN_POINT('Ctrl Pts',(-10.8900732320001,15.2,-2.07845100700002));
#266841=CARTESIAN_POINT('Ctrl Pts',(-10.8900732320001,11.6,-2.07845100700002));
#266842=CARTESIAN_POINT('Ctrl Pts',(-10.8928039400001,15.2,-2.08015896100001));
#266843=CARTESIAN_POINT('Ctrl Pts',(-10.8928039400001,11.6,-2.08015896100001));
#266844=CARTESIAN_POINT('Ctrl Pts',(-10.8955375960001,15.2,-2.08187181000001));
#266845=CARTESIAN_POINT('Ctrl Pts',(-10.8955375960001,11.6,-2.08187181000001));
#266846=CARTESIAN_POINT('Ctrl Pts',(-10.8982741870001,15.2,-2.08358955900001));
#266847=CARTESIAN_POINT('Ctrl Pts',(-10.8982741870001,11.6,-2.08358955900001));
#266848=CARTESIAN_POINT('Ctrl Pts',(-10.9010137040001,15.2,-2.08531220500001));
#266849=CARTESIAN_POINT('Ctrl Pts',(-10.9010137040001,11.6,-2.08531220500001));
#266850=CARTESIAN_POINT('Ctrl Pts',(-10.9037561350001,15.2,-2.08703975300002));
#266851=CARTESIAN_POINT('Ctrl Pts',(-10.9037561350001,11.6,-2.08703975300002));
#266852=CARTESIAN_POINT('Ctrl Pts',(-10.9065014700001,15.2,-2.08877220300002));
#266853=CARTESIAN_POINT('Ctrl Pts',(-10.9065014700001,11.6,-2.08877220300002));
#266854=CARTESIAN_POINT('Ctrl Pts',(-10.9092496960001,15.2,-2.09050955500001));
#266855=CARTESIAN_POINT('Ctrl Pts',(-10.9092496960001,11.6,-2.09050955500001));
#266856=CARTESIAN_POINT('Ctrl Pts',(-10.9120008040001,15.2,-2.09225181200001));
#266857=CARTESIAN_POINT('Ctrl Pts',(-10.9120008040001,11.6,-2.09225181200001));
#266858=CARTESIAN_POINT('Ctrl Pts',(-10.9147547830001,15.2,-2.09399897400001));
#266859=CARTESIAN_POINT('Ctrl Pts',(-10.9147547830001,11.6,-2.09399897400001));
#266860=CARTESIAN_POINT('Ctrl Pts',(-10.9175116210001,15.2,-2.09575104200002));
#266861=CARTESIAN_POINT('Ctrl Pts',(-10.9175116210001,11.6,-2.09575104200002));
#266862=CARTESIAN_POINT('Ctrl Pts',(-10.9202713070001,15.2,-2.09750801800002));
#266863=CARTESIAN_POINT('Ctrl Pts',(-10.9202713070001,11.6,-2.09750801800002));
#266864=CARTESIAN_POINT('Ctrl Pts',(-10.9230338300001,15.2,-2.09926990300001));
#266865=CARTESIAN_POINT('Ctrl Pts',(-10.9230338300001,11.6,-2.09926990300001));
#266866=CARTESIAN_POINT('Ctrl Pts',(-10.9257991820001,15.2,-2.10103669800001));
#266867=CARTESIAN_POINT('Ctrl Pts',(-10.9257991820001,11.6,-2.10103669800001));
#266868=CARTESIAN_POINT('Ctrl Pts',(-10.9285673490001,15.2,-2.10280840300001));
#266869=CARTESIAN_POINT('Ctrl Pts',(-10.9285673490001,11.6,-2.10280840300001));
#266870=CARTESIAN_POINT('Ctrl Pts',(-10.9313383210001,15.2,-2.10458502100002));
#266871=CARTESIAN_POINT('Ctrl Pts',(-10.9313383210001,11.6,-2.10458502100002));
#266872=CARTESIAN_POINT('Ctrl Pts',(-10.9341120880001,15.2,-2.10636655200001));
#266873=CARTESIAN_POINT('Ctrl Pts',(-10.9341120880001,11.6,-2.10636655200001));
#266874=CARTESIAN_POINT('Ctrl Pts',(-10.9368886390001,15.2,-2.10815299600001));
#266875=CARTESIAN_POINT('Ctrl Pts',(-10.9368886390001,11.6,-2.10815299600001));
#266876=CARTESIAN_POINT('Ctrl Pts',(-10.9396679630001,15.2,-2.10994435800002));
#266877=CARTESIAN_POINT('Ctrl Pts',(-10.9396679630001,11.6,-2.10994435800002));
#266878=CARTESIAN_POINT('Ctrl Pts',(-10.9424500480001,15.2,-2.11174063500001));
#266879=CARTESIAN_POINT('Ctrl Pts',(-10.9424500480001,11.6,-2.11174063500001));
#266880=CARTESIAN_POINT('Ctrl Pts',(-10.9452348850001,15.2,-2.11354182900001));
#266881=CARTESIAN_POINT('Ctrl Pts',(-10.9452348850001,11.6,-2.11354182900001));
#266882=CARTESIAN_POINT('Ctrl Pts',(-10.9480224640001,15.2,-2.11534794200002));
#266883=CARTESIAN_POINT('Ctrl Pts',(-10.9480224640001,11.6,-2.11534794200002));
#266884=CARTESIAN_POINT('Ctrl Pts',(-10.9508127730001,15.2,-2.11715897500001));
#266885=CARTESIAN_POINT('Ctrl Pts',(-10.9508127730001,11.6,-2.11715897500001));
#266886=CARTESIAN_POINT('Ctrl Pts',(-10.9536058010001,15.2,-2.11897492800002));
#266887=CARTESIAN_POINT('Ctrl Pts',(-10.9536058010001,11.6,-2.11897492800002));
#266888=CARTESIAN_POINT('Ctrl Pts',(-10.9564015380001,15.2,-2.12079580400002));
#266889=CARTESIAN_POINT('Ctrl Pts',(-10.9564015380001,11.6,-2.12079580400002));
#266890=CARTESIAN_POINT('Ctrl Pts',(-10.9591999740001,15.2,-2.12262160100002));
#266891=CARTESIAN_POINT('Ctrl Pts',(-10.9591999740001,11.6,-2.12262160100002));
#266892=CARTESIAN_POINT('Ctrl Pts',(-10.9620010970001,15.2,-2.12445232200002));
#266893=CARTESIAN_POINT('Ctrl Pts',(-10.9620010970001,11.6,-2.12445232200002));
#266894=CARTESIAN_POINT('Ctrl Pts',(-10.9648048980001,15.2,-2.12628796700002));
#266895=CARTESIAN_POINT('Ctrl Pts',(-10.9648048980001,11.6,-2.12628796700002));
#266896=CARTESIAN_POINT('Ctrl Pts',(-10.9676113650001,15.2,-2.12812853800001));
#266897=CARTESIAN_POINT('Ctrl Pts',(-10.9676113650001,11.6,-2.12812853800001));
#266898=CARTESIAN_POINT('Ctrl Pts',(-10.9704204880001,15.2,-2.12997403600002));
#266899=CARTESIAN_POINT('Ctrl Pts',(-10.9704204880001,11.6,-2.12997403600002));
#266900=CARTESIAN_POINT('Ctrl Pts',(-10.9732322570001,15.2,-2.13182446100001));
#266901=CARTESIAN_POINT('Ctrl Pts',(-10.9732322570001,11.6,-2.13182446100001));
#266902=CARTESIAN_POINT('Ctrl Pts',(-10.9760466620001,15.2,-2.13367981500001));
#266903=CARTESIAN_POINT('Ctrl Pts',(-10.9760466620001,11.6,-2.13367981500001));
#266904=CARTESIAN_POINT('Ctrl Pts',(-10.9788636920001,15.2,-2.13554009700001));
#266905=CARTESIAN_POINT('Ctrl Pts',(-10.9788636920001,11.6,-2.13554009700002));
#266906=CARTESIAN_POINT('Ctrl Pts',(-10.9816833350001,15.2,-2.13740531000001));
#266907=CARTESIAN_POINT('Ctrl Pts',(-10.9816833350001,11.6,-2.13740531000001));
#266908=CARTESIAN_POINT('Ctrl Pts',(-10.9845055830001,15.2,-2.13927545500002));
#266909=CARTESIAN_POINT('Ctrl Pts',(-10.9845055830001,11.6,-2.13927545500002));
#266910=CARTESIAN_POINT('Ctrl Pts',(-10.9873304240001,15.2,-2.14115053100001));
#266911=CARTESIAN_POINT('Ctrl Pts',(-10.9873304240001,11.6,-2.14115053100001));
#266912=CARTESIAN_POINT('Ctrl Pts',(-10.9901578480001,15.2,-2.14303054100001));
#266913=CARTESIAN_POINT('Ctrl Pts',(-10.9901578480001,11.6,-2.14303054100002));
#266914=CARTESIAN_POINT('Ctrl Pts',(-10.9929878450001,15.2,-2.14491548300002));
#266915=CARTESIAN_POINT('Ctrl Pts',(-10.9929878450001,11.6,-2.14491548300002));
#266916=CARTESIAN_POINT('Ctrl Pts',(-10.9958204050001,15.2,-2.14680536000001));
#266917=CARTESIAN_POINT('Ctrl Pts',(-10.9958204050001,11.6,-2.14680536000001));
#266918=CARTESIAN_POINT('Ctrl Pts',(-10.9986555170001,15.2,-2.14870017400001));
#266919=CARTESIAN_POINT('Ctrl Pts',(-10.9986555170001,11.6,-2.14870017400001));
#266920=CARTESIAN_POINT('Ctrl Pts',(-11.0014931700001,15.2,-2.15059992300001));
#266921=CARTESIAN_POINT('Ctrl Pts',(-11.0014931700001,11.6,-2.15059992300001));
#266922=CARTESIAN_POINT('Ctrl Pts',(-11.0043333550001,15.2,-2.15250461100001));
#266923=CARTESIAN_POINT('Ctrl Pts',(-11.0043333550001,11.6,-2.15250461100002));
#266924=CARTESIAN_POINT('Ctrl Pts',(-11.0071760610001,15.2,-2.15441423500002));
#266925=CARTESIAN_POINT('Ctrl Pts',(-11.0071760610001,11.6,-2.15441423500002));
#266926=CARTESIAN_POINT('Ctrl Pts',(-11.0100212790001,15.2,-2.15632879900001));
#266927=CARTESIAN_POINT('Ctrl Pts',(-11.0100212790001,11.6,-2.15632879900001));
#266928=CARTESIAN_POINT('Ctrl Pts',(-11.0128689970001,15.2,-2.15824830200001));
#266929=CARTESIAN_POINT('Ctrl Pts',(-11.0128689970001,11.6,-2.15824830200001));
#266930=CARTESIAN_POINT('Ctrl Pts',(-11.0157192050001,15.2,-2.16017274600001));
#266931=CARTESIAN_POINT('Ctrl Pts',(-11.0157192050001,11.6,-2.16017274600001));
#266932=CARTESIAN_POINT('Ctrl Pts',(-11.0185718950001,15.2,-2.16210213100001));
#266933=CARTESIAN_POINT('Ctrl Pts',(-11.0185718950001,11.6,-2.16210213100001));
#266934=CARTESIAN_POINT('Ctrl Pts',(-11.0214270540001,15.2,-2.16403645900002));
#266935=CARTESIAN_POINT('Ctrl Pts',(-11.0214270540001,11.6,-2.16403645900002));
#266936=CARTESIAN_POINT('Ctrl Pts',(-11.0242846730001,15.2,-2.16597572800001));
#266937=CARTESIAN_POINT('Ctrl Pts',(-11.0242846730001,11.6,-2.16597572800001));
#266938=CARTESIAN_POINT('Ctrl Pts',(-11.0271447430001,15.2,-2.16791994200001));
#266939=CARTESIAN_POINT('Ctrl Pts',(-11.0271447430001,11.6,-2.16791994200001));
#266940=CARTESIAN_POINT('Ctrl Pts',(-11.0300072520001,15.2,-2.16986910100001));
#266941=CARTESIAN_POINT('Ctrl Pts',(-11.0300072520001,11.6,-2.16986910100002));
#266942=CARTESIAN_POINT('Ctrl Pts',(-11.0328721920001,15.2,-2.17182320300001));
#266943=CARTESIAN_POINT('Ctrl Pts',(-11.0328721920001,11.6,-2.17182320300001));
#266944=CARTESIAN_POINT('Ctrl Pts',(-11.0357395510001,15.2,-2.17378225200001));
#266945=CARTESIAN_POINT('Ctrl Pts',(-11.0357395510001,11.6,-2.17378225200001));
#266946=CARTESIAN_POINT('Ctrl Pts',(-11.0386093190001,15.2,-2.17574624800001));
#266947=CARTESIAN_POINT('Ctrl Pts',(-11.0386093190001,11.6,-2.17574624800001));
#266948=CARTESIAN_POINT('Ctrl Pts',(-11.0414814870001,15.2,-2.17771519000001));
#266949=CARTESIAN_POINT('Ctrl Pts',(-11.0414814870001,11.6,-2.17771519000001));
#266950=CARTESIAN_POINT('Ctrl Pts',(-11.0443560440001,15.2,-2.17968908100001));
#266951=CARTESIAN_POINT('Ctrl Pts',(-11.0443560440001,11.6,-2.17968908100001));
#266952=CARTESIAN_POINT('Ctrl Pts',(-11.0472329810001,15.2,-2.18166792000002));
#266953=CARTESIAN_POINT('Ctrl Pts',(-11.0472329810001,11.6,-2.18166792000002));
#266954=CARTESIAN_POINT('Ctrl Pts',(-11.0501122880001,15.2,-2.18365170900002));
#266955=CARTESIAN_POINT('Ctrl Pts',(-11.0501122880001,11.6,-2.18365170900002));
#266956=CARTESIAN_POINT('Ctrl Pts',(-11.0529939540001,15.2,-2.18564044700001));
#266957=CARTESIAN_POINT('Ctrl Pts',(-11.0529939540001,11.6,-2.18564044700001));
#266958=CARTESIAN_POINT('Ctrl Pts',(-11.0558779690001,15.2,-2.18763413700001));
#266959=CARTESIAN_POINT('Ctrl Pts',(-11.0558779690001,11.6,-2.18763413700001));
#266960=CARTESIAN_POINT('Ctrl Pts',(-11.0587643250001,15.2,-2.18963277700002));
#266961=CARTESIAN_POINT('Ctrl Pts',(-11.0587643250001,11.6,-2.18963277700002));
#266962=CARTESIAN_POINT('Ctrl Pts',(-11.0616530110001,15.2,-2.19163636900001));
#266963=CARTESIAN_POINT('Ctrl Pts',(-11.0616530110001,11.6,-2.19163636900001));
#266964=CARTESIAN_POINT('Ctrl Pts',(-11.0645440160001,15.2,-2.19364491400002));
#266965=CARTESIAN_POINT('Ctrl Pts',(-11.0645440160001,11.6,-2.19364491400002));
#266966=CARTESIAN_POINT('Ctrl Pts',(-11.0674373310001,15.2,-2.19565841300001));
#266967=CARTESIAN_POINT('Ctrl Pts',(-11.0674373310001,11.6,-2.19565841300001));
#266968=CARTESIAN_POINT('Ctrl Pts',(-11.0703329460001,15.2,-2.19767686500001));
#266969=CARTESIAN_POINT('Ctrl Pts',(-11.0703329460001,11.6,-2.19767686500001));
#266970=CARTESIAN_POINT('Ctrl Pts',(-11.0732308520001,15.2,-2.19970027200001));
#266971=CARTESIAN_POINT('Ctrl Pts',(-11.0732308520001,11.6,-2.19970027200001));
#266972=CARTESIAN_POINT('Ctrl Pts',(-11.0761310380001,15.2,-2.20172863400002));
#266973=CARTESIAN_POINT('Ctrl Pts',(-11.0761310380001,11.6,-2.20172863400002));
#266974=CARTESIAN_POINT('Ctrl Pts',(-11.0790334940001,15.2,-2.20376195100001));
#266975=CARTESIAN_POINT('Ctrl Pts',(-11.0790334940001,11.6,-2.20376195100001));
#266976=CARTESIAN_POINT('Ctrl Pts',(-11.0819382120001,15.2,-2.20580022500001));
#266977=CARTESIAN_POINT('Ctrl Pts',(-11.0819382120001,11.6,-2.20580022500001));
#266978=CARTESIAN_POINT('Ctrl Pts',(-11.0848451810001,15.2,-2.20784345600002));
#266979=CARTESIAN_POINT('Ctrl Pts',(-11.0848451810001,11.6,-2.20784345600002));
#266980=CARTESIAN_POINT('Ctrl Pts',(-11.0877543900001,15.2,-2.20989164400001));
#266981=CARTESIAN_POINT('Ctrl Pts',(-11.0877543900001,11.6,-2.20989164400002));
#266982=CARTESIAN_POINT('Ctrl Pts',(-11.0906658320001,15.2,-2.21194478900001));
#266983=CARTESIAN_POINT('Ctrl Pts',(-11.0906658320001,11.6,-2.21194478900001));
#266984=CARTESIAN_POINT('Ctrl Pts',(-11.0935794960001,15.2,-2.21400289400002));
#266985=CARTESIAN_POINT('Ctrl Pts',(-11.0935794960001,11.6,-2.21400289400002));
#266986=CARTESIAN_POINT('Ctrl Pts',(-11.0964953710001,15.2,-2.21606595800001));
#266987=CARTESIAN_POINT('Ctrl Pts',(-11.0964953710001,11.6,-2.21606595800001));
#266988=CARTESIAN_POINT('Ctrl Pts',(-11.0994134490001,15.2,-2.21813398000001));
#266989=CARTESIAN_POINT('Ctrl Pts',(-11.0994134490001,11.6,-2.21813398000001));
#266990=CARTESIAN_POINT('Ctrl Pts',(-11.1023337200001,15.2,-2.22020696400001));
#266991=CARTESIAN_POINT('Ctrl Pts',(-11.1023337200001,11.6,-2.22020696400001));
#266992=CARTESIAN_POINT('Ctrl Pts',(-11.1052561740001,15.2,-2.22228490700001));
#266993=CARTESIAN_POINT('Ctrl Pts',(-11.1052561740001,11.6,-2.22228490700001));
#266994=CARTESIAN_POINT('Ctrl Pts',(-11.1081808010001,15.2,-2.22436781200001));
#266995=CARTESIAN_POINT('Ctrl Pts',(-11.1081808010001,11.6,-2.22436781200001));
#266996=CARTESIAN_POINT('Ctrl Pts',(-11.1111075920001,15.2,-2.22645567900001));
#266997=CARTESIAN_POINT('Ctrl Pts',(-11.1111075920001,11.6,-2.22645567900001));
#266998=CARTESIAN_POINT('Ctrl Pts',(-11.1140365370001,15.2,-2.22854850700001));
#266999=CARTESIAN_POINT('Ctrl Pts',(-11.1140365370001,11.6,-2.22854850700001));
#267000=CARTESIAN_POINT('Ctrl Pts',(-11.1169676280001,15.2,-2.23064629800001));
#267001=CARTESIAN_POINT('Ctrl Pts',(-11.1169676280001,11.6,-2.23064629800001));
#267002=CARTESIAN_POINT('Ctrl Pts',(-11.1199008530001,15.2,-2.23274905300002));
#267003=CARTESIAN_POINT('Ctrl Pts',(-11.1199008530001,11.6,-2.23274905300002));
#267004=CARTESIAN_POINT('Ctrl Pts',(-11.1228362040001,15.2,-2.23485677100001));
#267005=CARTESIAN_POINT('Ctrl Pts',(-11.1228362040001,11.6,-2.23485677100001));
#267006=CARTESIAN_POINT('Ctrl Pts',(-11.1257736700001,15.2,-2.23696945200002));
#267007=CARTESIAN_POINT('Ctrl Pts',(-11.1257736700001,11.6,-2.23696945200002));
#267008=CARTESIAN_POINT('Ctrl Pts',(-11.1287132440001,15.2,-2.23908709800002));
#267009=CARTESIAN_POINT('Ctrl Pts',(-11.1287132440001,11.6,-2.23908709800002));
#267010=CARTESIAN_POINT('Ctrl Pts',(-11.1316549140001,15.2,-2.24120971000001));
#267011=CARTESIAN_POINT('Ctrl Pts',(-11.1316549140001,11.6,-2.24120971000001));
#267012=CARTESIAN_POINT('Ctrl Pts',(-11.1345986720001,15.2,-2.24333728500001));
#267013=CARTESIAN_POINT('Ctrl Pts',(-11.1345986720001,11.6,-2.24333728500001));
#267014=CARTESIAN_POINT('Ctrl Pts',(-11.1375445070001,15.2,-2.24546982700002));
#267015=CARTESIAN_POINT('Ctrl Pts',(-11.1375445070001,11.6,-2.24546982700002));
#267016=CARTESIAN_POINT('Ctrl Pts',(-11.1404924120001,15.2,-2.24760733500001));
#267017=CARTESIAN_POINT('Ctrl Pts',(-11.1404924120001,11.6,-2.24760733500002));
#267018=CARTESIAN_POINT('Ctrl Pts',(-11.1434423750001,15.2,-2.24974981000001));
#267019=CARTESIAN_POINT('Ctrl Pts',(-11.1434423750001,11.6,-2.24974981000001));
#267020=CARTESIAN_POINT('Ctrl Pts',(-11.1463943880001,15.2,-2.25189725100002));
#267021=CARTESIAN_POINT('Ctrl Pts',(-11.1463943880001,11.6,-2.25189725100002));
#267022=CARTESIAN_POINT('Ctrl Pts',(-11.1493484410001,15.2,-2.25404966000001));
#267023=CARTESIAN_POINT('Ctrl Pts',(-11.1493484410001,11.6,-2.25404966000002));
#267024=CARTESIAN_POINT('Ctrl Pts',(-11.1523045240001,15.2,-2.25620703600002));
#267025=CARTESIAN_POINT('Ctrl Pts',(-11.1523045240001,11.6,-2.25620703600002));
#267026=CARTESIAN_POINT('Ctrl Pts',(-11.1552626310001,15.2,-2.25836938000001));
#267027=CARTESIAN_POINT('Ctrl Pts',(-11.1552626310001,11.6,-2.25836938000001));
#267028=CARTESIAN_POINT('Ctrl Pts',(-11.1582227480001,15.2,-2.26053669300001));
#267029=CARTESIAN_POINT('Ctrl Pts',(-11.1582227480001,11.6,-2.26053669300002));
#267030=CARTESIAN_POINT('Ctrl Pts',(-11.1611848690001,15.2,-2.26270897400001));
#267031=CARTESIAN_POINT('Ctrl Pts',(-11.1611848690001,11.6,-2.26270897400001));
#267032=CARTESIAN_POINT('Ctrl Pts',(-11.1641489820001,15.2,-2.26488622400002));
#267033=CARTESIAN_POINT('Ctrl Pts',(-11.1641489820001,11.6,-2.26488622400002));
#267034=CARTESIAN_POINT('Ctrl Pts',(-11.1671150810001,15.2,-2.26706844400002));
#267035=CARTESIAN_POINT('Ctrl Pts',(-11.1671150810001,11.6,-2.26706844400002));
#267036=CARTESIAN_POINT('Ctrl Pts',(-11.1700831540001,15.2,-2.26925563400002));
#267037=CARTESIAN_POINT('Ctrl Pts',(-11.1700831540001,11.6,-2.26925563400002));
#267038=CARTESIAN_POINT('Ctrl Pts',(-11.1730531910001,15.2,-2.27144779400001));
#267039=CARTESIAN_POINT('Ctrl Pts',(-11.1730531910001,11.6,-2.27144779400001));
#267040=CARTESIAN_POINT('Ctrl Pts',(-11.1760251850001,15.2,-2.27364492400001));
#267041=CARTESIAN_POINT('Ctrl Pts',(-11.1760251850001,11.6,-2.27364492400001));
#267042=CARTESIAN_POINT('Ctrl Pts',(-11.1789991260001,15.2,-2.27584702400002));
#267043=CARTESIAN_POINT('Ctrl Pts',(-11.1789991260001,11.6,-2.27584702400002));
#267044=CARTESIAN_POINT('Ctrl Pts',(-11.1819750050001,15.2,-2.27805409600002));
#267045=CARTESIAN_POINT('Ctrl Pts',(-11.1819750050001,11.6,-2.27805409600002));
#267046=CARTESIAN_POINT('Ctrl Pts',(-11.1849528130001,15.2,-2.28026613900001));
#267047=CARTESIAN_POINT('Ctrl Pts',(-11.1849528130001,11.6,-2.28026613900001));
#267048=CARTESIAN_POINT('Ctrl Pts',(-11.1879325400001,15.2,-2.28248315300001));
#267049=CARTESIAN_POINT('Ctrl Pts',(-11.1879325400001,11.6,-2.28248315300001));
#267050=CARTESIAN_POINT('Ctrl Pts',(-11.1909141790001,15.2,-2.28470513900001));
#267051=CARTESIAN_POINT('Ctrl Pts',(-11.1909141790001,11.6,-2.28470513900001));
#267052=CARTESIAN_POINT('Ctrl Pts',(-11.1938977190001,15.2,-2.28693209700001));
#267053=CARTESIAN_POINT('Ctrl Pts',(-11.1938977190001,11.6,-2.28693209700001));
#267054=CARTESIAN_POINT('Ctrl Pts',(-11.1968831490001,15.2,-2.28916402700001));
#267055=CARTESIAN_POINT('Ctrl Pts',(-11.1968831490001,11.6,-2.28916402700001));
#267056=CARTESIAN_POINT('Ctrl Pts',(-11.1998704640001,15.2,-2.29140093100002));
#267057=CARTESIAN_POINT('Ctrl Pts',(-11.1998704640001,11.6,-2.29140093100002));
#267058=CARTESIAN_POINT('Ctrl Pts',(-11.2028596490001,15.2,-2.29364280600001));
#267059=CARTESIAN_POINT('Ctrl Pts',(-11.2028596490001,11.6,-2.29364280600001));
#267060=CARTESIAN_POINT('Ctrl Pts',(-11.2058506990001,15.2,-2.29588965500001));
#267061=CARTESIAN_POINT('Ctrl Pts',(-11.2058506990001,11.6,-2.29588965500001));
#267062=CARTESIAN_POINT('Ctrl Pts',(-11.2088436030001,15.2,-2.29814147700001));
#267063=CARTESIAN_POINT('Ctrl Pts',(-11.2088436030001,11.6,-2.29814147700001));
#267064=CARTESIAN_POINT('Ctrl Pts',(-11.2118383520001,15.2,-2.30039827300001));
#267065=CARTESIAN_POINT('Ctrl Pts',(-11.2118383520001,11.6,-2.30039827300002));
#267066=CARTESIAN_POINT('Ctrl Pts',(-11.2148349390001,15.2,-2.30266004200002));
#267067=CARTESIAN_POINT('Ctrl Pts',(-11.2148349390001,11.6,-2.30266004200002));
#267068=CARTESIAN_POINT('Ctrl Pts',(-11.2178333560001,15.2,-2.30492678400001));
#267069=CARTESIAN_POINT('Ctrl Pts',(-11.2178333560001,11.6,-2.30492678400001));
#267070=CARTESIAN_POINT('Ctrl Pts',(-11.2208335940001,15.2,-2.30719850100002));
#267071=CARTESIAN_POINT('Ctrl Pts',(-11.2208335940001,11.6,-2.30719850100002));
#267072=CARTESIAN_POINT('Ctrl Pts',(-11.2238356440001,15.2,-2.30947519200001));
#267073=CARTESIAN_POINT('Ctrl Pts',(-11.2238356440001,11.6,-2.30947519200001));
#267074=CARTESIAN_POINT('Ctrl Pts',(-11.2268394980001,15.2,-2.31175685800002));
#267075=CARTESIAN_POINT('Ctrl Pts',(-11.2268394980001,11.6,-2.31175685800002));
#267076=CARTESIAN_POINT('Ctrl Pts',(-11.2298451450001,15.2,-2.31404349800002));
#267077=CARTESIAN_POINT('Ctrl Pts',(-11.2298451450001,11.6,-2.31404349800002));
#267078=CARTESIAN_POINT('Ctrl Pts',(-11.2328525720001,15.2,-2.31633511300001));
#267079=CARTESIAN_POINT('Ctrl Pts',(-11.2328525720001,11.6,-2.31633511300001));
#267080=CARTESIAN_POINT('Ctrl Pts',(-11.2358617710001,15.2,-2.31863170300001));
#267081=CARTESIAN_POINT('Ctrl Pts',(-11.2358617710001,11.6,-2.31863170300001));
#267082=CARTESIAN_POINT('Ctrl Pts',(-11.2388727300001,15.2,-2.32093326800001));
#267083=CARTESIAN_POINT('Ctrl Pts',(-11.2388727300001,11.6,-2.32093326800001));
#267084=CARTESIAN_POINT('Ctrl Pts',(-11.2418854380001,15.2,-2.32323980800002));
#267085=CARTESIAN_POINT('Ctrl Pts',(-11.2418854380001,11.6,-2.32323980800002));
#267086=CARTESIAN_POINT('Ctrl Pts',(-11.2448998880001,15.2,-2.32555132400002));
#267087=CARTESIAN_POINT('Ctrl Pts',(-11.2448998880001,11.6,-2.32555132400002));
#267088=CARTESIAN_POINT('Ctrl Pts',(-11.2479160730001,15.2,-2.32786781500002));
#267089=CARTESIAN_POINT('Ctrl Pts',(-11.2479160730001,11.6,-2.32786781500002));
#267090=CARTESIAN_POINT('Ctrl Pts',(-11.2509339910001,15.2,-2.33018928300002));
#267091=CARTESIAN_POINT('Ctrl Pts',(-11.2509339910001,11.6,-2.33018928300002));
#267092=CARTESIAN_POINT('Ctrl Pts',(-11.2539536380001,15.2,-2.33251572400002));
#267093=CARTESIAN_POINT('Ctrl Pts',(-11.2539536380001,11.6,-2.33251572400002));
#267094=CARTESIAN_POINT('Ctrl Pts',(-11.2563707390001,15.2,-2.33438085900001));
#267095=CARTESIAN_POINT('Ctrl Pts',(-11.2563707390001,11.6,-2.33438085900001));
#267096=CARTESIAN_POINT('Ctrl Pts',(-11.2581843410001,15.2,-2.33578194700002));
#267097=CARTESIAN_POINT('Ctrl Pts',(-11.2581843410001,11.6,-2.33578194700002));
#267098=CARTESIAN_POINT('Ctrl Pts',(-11.2593937550001,15.2,-2.33671700200001));
#267099=CARTESIAN_POINT('Ctrl Pts',(-11.2593937550001,11.6,-2.33671700200001));
#267100=CARTESIAN_POINT('Ctrl Pts',(-11.2599985490001,15.2,-2.33718477800001));
#267101=CARTESIAN_POINT('Ctrl Pts',(-11.2599985490001,11.6,-2.33718477800001));
#267102=CARTESIAN_POINT('Ctrl Pts',(-10.2237731100001,15.2,-1.76496130700002));
#267103=CARTESIAN_POINT('Ctrl Pts',(-10.2255010902461,15.2,-1.76541542813168));
#267104=CARTESIAN_POINT('Ctrl Pts',(-10.2272829932875,15.2,-1.76588926588842));
#267105=CARTESIAN_POINT('Ctrl Pts',(-10.2291177142657,15.2,-1.76638321069588));
#267106=CARTESIAN_POINT('Ctrl Pts',(-10.2309612831959,15.2,-1.76687953755489));
#267107=CARTESIAN_POINT('Ctrl Pts',(-10.232858179982,15.2,-1.76739616339468));
#267108=CARTESIAN_POINT('Ctrl Pts',(-10.2348073231887,15.2,-1.76793345428534));
#267109=CARTESIAN_POINT('Ctrl Pts',(-10.2367564662182,15.2,-1.76847074512719));
#267110=CARTESIAN_POINT('Ctrl Pts',(-10.2387578531412,15.2,-1.76902870433768));
#267111=CARTESIAN_POINT('Ctrl Pts',(-10.2408104332333,15.2,-1.76960768598331));
#267112=CARTESIAN_POINT('Ctrl Pts',(-10.2428630133254,15.2,-1.77018666762894));
#267113=CARTESIAN_POINT('Ctrl Pts',(-10.2449667829903,15.2,-1.77078667199102));
#267114=CARTESIAN_POINT('Ctrl Pts',(-10.2471207202667,15.2,-1.77140804341492));
#267115=CARTESIAN_POINT('Ctrl Pts',(-10.2492746577388,15.2,-1.77202941489526));
#267116=CARTESIAN_POINT('Ctrl Pts',(-10.2514787619861,15.2,-1.77267215260972));
#267117=CARTESIAN_POINT('Ctrl Pts',(-10.2537320337789,15.2,-1.77333658806407));
#267118=CARTESIAN_POINT('Ctrl Pts',(-10.2559853053671,15.2,-1.77400102345808));
#267119=CARTESIAN_POINT('Ctrl Pts',(-10.258287747059,15.2,-1.77468715486442));
#267120=CARTESIAN_POINT('Ctrl Pts',(-10.2606383864844,15.2,-1.77539530325863));
#267121=CARTESIAN_POINT('Ctrl Pts',(-10.2633807992897,15.2,-1.77622147642809));
#267122=CARTESIAN_POINT('Ctrl Pts',(-10.2661888137587,15.2,-1.77707761705611));
#267123=CARTESIAN_POINT('Ctrl Pts',(-10.2690609297517,15.2,-1.77796421189115));
#267124=CARTESIAN_POINT('Ctrl Pts',(-10.2715227433321,15.2,-1.77872415028173));
#267125=CARTESIAN_POINT('Ctrl Pts',(-10.2740316522823,15.2,-1.77950646228422));
#267126=CARTESIAN_POINT('Ctrl Pts',(-10.2765867400345,15.2,-1.78031144550867));
#267127=CARTESIAN_POINT('Ctrl Pts',(-10.2791418277867,15.2,-1.78111642873313));
#267128=CARTESIAN_POINT('Ctrl Pts',(-10.2817430937041,15.2,-1.78194408006062));
#267129=CARTESIAN_POINT('Ctrl Pts',(-10.2843896406059,15.2,-1.78279468544538));
#267130=CARTESIAN_POINT('Ctrl Pts',(-10.2870361877482,15.2,-1.78364529090741));
#267131=CARTESIAN_POINT('Ctrl Pts',(-10.2897280174628,15.2,-1.78451885324728));
#267132=CARTESIAN_POINT('Ctrl Pts',(-10.2924642537816,15.2,-1.78541564263106));
#267133=CARTESIAN_POINT('Ctrl Pts',(-10.2952004898518,15.2,-1.78631243193339));
#267134=CARTESIAN_POINT('Ctrl Pts',(-10.2979811346214,15.2,-1.78723245113474));
#267135=CARTESIAN_POINT('Ctrl Pts',(-10.3008053326874,15.2,-1.78817596526816));
#267136=CARTESIAN_POINT('Ctrl Pts',(-10.3036295307534,15.2,-1.78911947940158));
#267137=CARTESIAN_POINT('Ctrl Pts',(-10.3064972822325,15.2,-1.79008648825811));
#267138=CARTESIAN_POINT('Ctrl Pts',(-10.3094077542915,15.2,-1.79107724747108));
#267139=CARTESIAN_POINT('Ctrl Pts',(-10.3123182263506,15.2,-1.79206800668404));
#267140=CARTESIAN_POINT('Ctrl Pts',(-10.3152714195936,15.2,-1.79308251806783));
#267141=CARTESIAN_POINT('Ctrl Pts',(-10.3182665168985,15.2,-1.79412102811178));
#267142=CARTESIAN_POINT('Ctrl Pts',(-10.3212616144756,15.2,-1.79515953825006));
#267143=CARTESIAN_POINT('Ctrl Pts',(-10.324298617665,15.2,-1.79622204704902));
#267144=CARTESIAN_POINT('Ctrl Pts',(-10.3273767301679,15.2,-1.79730879327597));
#267145=CARTESIAN_POINT('Ctrl Pts',(-10.3304548423912,15.2,-1.79839553940421));
#267146=CARTESIAN_POINT('Ctrl Pts',(-10.3335740630195,15.2,-1.79950652338884));
#267147=CARTESIAN_POINT('Ctrl Pts',(-10.3367336133196,15.2,-1.80064197642986));
#267148=CARTESIAN_POINT('Ctrl Pts',(-10.3404197555278,15.2,-1.80196667171315));
#267149=CARTESIAN_POINT('Ctrl Pts',(-10.3441607915552,15.2,-1.80332467195882));
#267150=CARTESIAN_POINT('Ctrl Pts',(-10.3479555098941,15.2,-1.80471633031509));
#267151=CARTESIAN_POINT('Ctrl Pts',(-10.3512081254443,15.2,-1.80590918027283));
#267152=CARTESIAN_POINT('Ctrl Pts',(-10.354500184008,15.2,-1.80712675892025));
#267153=CARTESIAN_POINT('Ctrl Pts',(-10.357830939552,15.2,-1.80836927995736));
#267154=CARTESIAN_POINT('Ctrl Pts',(-10.3611616950959,15.2,-1.80961180099447));
#267155=CARTESIAN_POINT('Ctrl Pts',(-10.3645311512467,15.2,-1.81087926565776));
#267156=CARTESIAN_POINT('Ctrl Pts',(-10.3679385748703,15.2,-1.81217187960908));
#267157=CARTESIAN_POINT('Ctrl Pts',(-10.3713459988033,15.2,-1.81346449367781));
#267158=CARTESIAN_POINT('Ctrl Pts',(-10.3747913931235,15.2,-1.81478225687398));
#267159=CARTESIAN_POINT('Ctrl Pts',(-10.3782740448983,15.2,-1.81612537086494));
#267160=CARTESIAN_POINT('Ctrl Pts',(-10.382337138161,15.2,-1.81769233700473));
#267161=CARTESIAN_POINT('Ctrl Pts',(-10.3864509388899,15.2,-1.81929380616216));
#267162=CARTESIAN_POINT('Ctrl Pts',(-10.390614342336,15.2,-1.82093008736377));
#267163=CARTESIAN_POINT('Ctrl Pts',(-10.394182974278,15.2,-1.8223326142718));
#267164=CARTESIAN_POINT('Ctrl Pts',(-10.3977880466902,15.2,-1.82376071572395));
#267165=CARTESIAN_POINT('Ctrl Pts',(-10.4014288796402,15.2,-1.82521457855431));
#267166=CARTESIAN_POINT('Ctrl Pts',(-10.4050697122595,15.2,-1.82666844125262));
#267167=CARTESIAN_POINT('Ctrl Pts',(-10.4087463029747,15.2,-1.82814806405555));
#267168=CARTESIAN_POINT('Ctrl Pts',(-10.4124579827733,15.2,-1.82965362775762));
#267169=CARTESIAN_POINT('Ctrl Pts',(-10.4155510493845,15.2,-1.8309082642216));
#267170=CARTESIAN_POINT('Ctrl Pts',(-10.4186684823111,15.2,-1.83218091350552));
#267171=CARTESIAN_POINT('Ctrl Pts',(-10.4218099022417,15.2,-1.83347167899163));
#267172=CARTESIAN_POINT('Ctrl Pts',(-10.4249513221722,15.2,-1.83476244447774));
#267173=CARTESIAN_POINT('Ctrl Pts',(-10.4281167289928,15.2,-1.83607132367796));
#267174=CARTESIAN_POINT('Ctrl Pts',(-10.4313057457434,15.2,-1.83739841597569));
#267175=CARTESIAN_POINT('Ctrl Pts',(-10.4344947624941,15.2,-1.83872550827343));
#267176=CARTESIAN_POINT('Ctrl Pts',(-10.4377073919272,15.2,-1.84007081228831));
#267177=CARTESIAN_POINT('Ctrl Pts',(-10.4409432619284,15.2,-1.84143442458093));
#267178=CARTESIAN_POINT('Ctrl Pts',(-10.4448263057888,15.2,-1.84307075927262));
#267179=CARTESIAN_POINT('Ctrl Pts',(-10.4487428171215,15.2,-1.84473345744554));
#267180=CARTESIAN_POINT('Ctrl Pts',(-10.4526921690599,15.2,-1.84642267713301));
#267181=CARTESIAN_POINT('Ctrl Pts',(-10.4559832957948,15.2,-1.84783036025705));
#267182=CARTESIAN_POINT('Ctrl Pts',(-10.4592972280831,15.2,-1.84925646249822));
#267183=CARTESIAN_POINT('Ctrl Pts',(-10.4626336097649,15.2,-1.85070107069918));
#267184=CARTESIAN_POINT('Ctrl Pts',(-10.4659699914466,15.2,-1.85214567890014));
#267185=CARTESIAN_POINT('Ctrl Pts',(-10.4693288195611,15.2,-1.85360879656108));
#267186=CARTESIAN_POINT('Ctrl Pts',(-10.4727097455333,15.2,-1.8550905062833));
#267187=CARTESIAN_POINT('Ctrl Pts',(-10.4767668565526,15.2,-1.85686855788536));
#267188=CARTESIAN_POINT('Ctrl Pts',(-10.4808557861972,15.2,-1.8586733857911));
#267189=CARTESIAN_POINT('Ctrl Pts',(-10.4849759355848,15.2,-1.8605051335645));
#267190=CARTESIAN_POINT('Ctrl Pts',(-10.4884093935326,15.2,-1.8620315900978));
#267191=CARTESIAN_POINT('Ctrl Pts',(-10.4918645315683,15.2,-1.86357674172655));
#267192=CARTESIAN_POINT('Ctrl Pts',(-10.4953410100394,15.2,-1.86514067040613));
#267193=CARTESIAN_POINT('Ctrl Pts',(-10.4995127844322,15.2,-1.86701738492392));
#267194=CARTESIAN_POINT('Ctrl Pts',(-10.503715288887,15.2,-1.86892113392835));
#267195=CARTESIAN_POINT('Ctrl Pts',(-10.507947939703,15.2,-1.87085205945211));
#267196=CARTESIAN_POINT('Ctrl Pts',(-10.5114751481398,15.2,-1.87246116379216));
#267197=CARTESIAN_POINT('Ctrl Pts',(-10.5150232947072,15.2,-1.87408913832673));
#267198=CARTESIAN_POINT('Ctrl Pts',(-10.5185920470249,15.2,-1.87573605953456));
#267199=CARTESIAN_POINT('Ctrl Pts',(-10.5221607997315,15.2,-1.87738298092189));
#267200=CARTESIAN_POINT('Ctrl Pts',(-10.5257501579795,15.2,-1.87904884983669));
#267201=CARTESIAN_POINT('Ctrl Pts',(-10.5293597967279,15.2,-1.88073373802959));
#267202=CARTESIAN_POINT('Ctrl Pts',(-10.5329694354762,15.2,-1.88241862622248));
#267203=CARTESIAN_POINT('Ctrl Pts',(-10.5365993551742,15.2,-1.88412253748728));
#267204=CARTESIAN_POINT('Ctrl Pts',(-10.5402492322559,15.2,-1.88584553970794));
#267205=CARTESIAN_POINT('Ctrl Pts',(-10.5446290849927,15.2,-1.8879131424854));
#267206=CARTESIAN_POINT('Ctrl Pts',(-10.5490376785725,15.2,-1.89000823945703));
#267207=CARTESIAN_POINT('Ctrl Pts',(-10.5534744636209,15.2,-1.89213095026371));
#267208=CARTESIAN_POINT('Ctrl Pts',(-10.5571717842932,15.2,-1.89389987583955));
#267209=CARTESIAN_POINT('Ctrl Pts',(-10.5608886844427,15.2,-1.89568797632368));
#267210=CARTESIAN_POINT('Ctrl Pts',(-10.5646248482637,15.2,-1.89749532097804));
#267211=CARTESIAN_POINT('Ctrl Pts',(-10.5683610120847,15.2,-1.8993026656324));
#267212=CARTESIAN_POINT('Ctrl Pts',(-10.5721164430588,15.2,-1.90112925419539));
#267213=CARTESIAN_POINT('Ctrl Pts',(-10.575890830977,15.2,-1.90297515051642));
#267214=CARTESIAN_POINT('Ctrl Pts',(-10.5796652184838,15.2,-1.90482104663624));
#267215=CARTESIAN_POINT('Ctrl Pts',(-10.5834585628684,15.2,-1.90668625191048));
#267216=CARTESIAN_POINT('Ctrl Pts',(-10.5872705597431,15.2,-1.9085708287868));
#267217=CARTESIAN_POINT('Ctrl Pts',(-10.5903201577414,15.2,-1.91007849053437));
#267218=CARTESIAN_POINT('Ctrl Pts',(-10.5933816951381,15.2,-1.91159855016644));
#267219=CARTESIAN_POINT('Ctrl Pts',(-10.59645501575,15.2,-1.91313103924996));
#267220=CARTESIAN_POINT('Ctrl Pts',(-10.5995283363619,15.2,-1.91466352833349));
#267221=CARTESIAN_POINT('Ctrl Pts',(-10.6026134402864,15.2,-1.91620844646012));
#267222=CARTESIAN_POINT('Ctrl Pts',(-10.6057101767897,15.2,-1.91776582604627));
#267223=CARTESIAN_POINT('Ctrl Pts',(-10.608806912871,15.2,-1.91932320542022));
#267224=CARTESIAN_POINT('Ctrl Pts',(-10.6119152799916,15.2,-1.92089304261277));
#267225=CARTESIAN_POINT('Ctrl Pts',(-10.6150351274729,15.2,-1.92247537199056));
#267226=CARTESIAN_POINT('Ctrl Pts',(-10.6181549753793,15.2,-1.92405770158394));
#267227=CARTESIAN_POINT('Ctrl Pts',(-10.6212863036442,15.2,-1.92565252052667));
#267228=CARTESIAN_POINT('Ctrl Pts',(-10.6244289635388,15.2,-1.92725985900444));
#267229=CARTESIAN_POINT('Ctrl Pts',(-10.6275716230053,15.2,-1.92886719726321));
#267230=CARTESIAN_POINT('Ctrl Pts',(-10.630725612537,15.2,-1.93048705547868));
#267231=CARTESIAN_POINT('Ctrl Pts',(-10.6338907859997,15.2,-1.93211946156664));
#267232=CARTESIAN_POINT('Ctrl Pts',(-10.6370559598937,15.2,-1.93375186787701));
#267233=CARTESIAN_POINT('Ctrl Pts',(-10.6402323162592,15.2,-1.93539682139965));
#267234=CARTESIAN_POINT('Ctrl Pts',(-10.6434197092043,15.2,-1.93705435124055));
#267235=CARTESIAN_POINT('Ctrl Pts',(-10.646607101715,15.2,-1.93871188085561));
#267236=CARTESIAN_POINT('Ctrl Pts',(-10.6498055307425,15.2,-1.94038198568146));
#267237=CARTESIAN_POINT('Ctrl Pts',(-10.6530148509794,15.2,-1.94206469382086));
#267238=CARTESIAN_POINT('Ctrl Pts',(-10.6562241716536,15.2,-1.94374740218952));
#267239=CARTESIAN_POINT('Ctrl Pts',(-10.6594443837097,15.2,-1.94544271250135));
#267240=CARTESIAN_POINT('Ctrl Pts',(-10.6626753429976,15.2,-1.94715065337304));
#267241=CARTESIAN_POINT('Ctrl Pts',(-10.6659063018453,15.2,-1.94885859401202));
#267242=CARTESIAN_POINT('Ctrl Pts',(-10.6691480087602,15.2,-1.95057916340473));
#267243=CARTESIAN_POINT('Ctrl Pts',(-10.6724003205448,15.2,-1.9523123870152));
#267244=CARTESIAN_POINT('Ctrl Pts',(-10.6756526327725,15.2,-1.95404561086182));
#267245=CARTESIAN_POINT('Ctrl Pts',(-10.6789155489775,15.2,-1.95579149007773));
#267246=CARTESIAN_POINT('Ctrl Pts',(-10.6821889302677,15.2,-1.95755004911885));
#267247=CARTESIAN_POINT('Ctrl Pts',(-10.6862806566575,15.2,-1.95974824780045));
#267248=CARTESIAN_POINT('Ctrl Pts',(-10.6903887316523,15.2,-1.96196625875095));
#267249=CARTESIAN_POINT('Ctrl Pts',(-10.6945128847782,15.2,-1.96420412986311));
#267250=CARTESIAN_POINT('Ctrl Pts',(-10.6978122070091,15.2,-1.96599442660647));
#267251=CARTESIAN_POINT('Ctrl Pts',(-10.7011218184748,15.2,-1.96779743342872));
#267252=CARTESIAN_POINT('Ctrl Pts',(-10.704441581035,15.2,-1.96961317370323));
#267253=CARTESIAN_POINT('Ctrl Pts',(-10.7077613440476,15.2,-1.97142891422513));
#267254=CARTESIAN_POINT('Ctrl Pts',(-10.7110912583488,15.2,-1.97325738926053));
#267255=CARTESIAN_POINT('Ctrl Pts',(-10.7144311870315,15.2,-1.97509862091727));
#267256=CARTESIAN_POINT('Ctrl Pts',(-10.7177711152591,15.2,-1.97693985232314));
#267257=CARTESIAN_POINT('Ctrl Pts',(-10.7211210569069,15.2,-1.97879383991255));
#267258=CARTESIAN_POINT('Ctrl Pts',(-10.724480877909,15.2,-1.98066060670309));
#267259=CARTESIAN_POINT('Ctrl Pts',(-10.728680654505,15.2,-1.98299406538202));
#267260=CARTESIAN_POINT('Ctrl Pts',(-10.7328958667709,15.2,-1.98534749229066));
#267261=CARTESIAN_POINT('Ctrl Pts',(-10.7371262512173,15.2,-1.98772092844951));
#267262=CARTESIAN_POINT('Ctrl Pts',(-10.7405105589589,15.2,-1.98961967748008));
#267263=CARTESIAN_POINT('Ctrl Pts',(-10.7439045777533,15.2,-1.99153123194891));
#267264=CARTESIAN_POINT('Ctrl Pts',(-10.747308174495,15.2,-1.99345561366574));
#267265=CARTESIAN_POINT('Ctrl Pts',(-10.7515626701902,15.2,-1.99586109068067));
#267266=CARTESIAN_POINT('Ctrl Pts',(-10.755832130074,15.2,-1.99828660933676));
#267267=CARTESIAN_POINT('Ctrl Pts',(-10.7601162983386,15.2,-2.00073221114336));
#267268=CARTESIAN_POINT('Ctrl Pts',(-10.7644004666033,15.2,-2.00317781294997));
#267269=CARTESIAN_POINT('Ctrl Pts',(-10.768699341812,15.2,-2.00564349469633));
#267270=CARTESIAN_POINT('Ctrl Pts',(-10.7730126719591,15.2,-2.00812929753027));
#267271=CARTESIAN_POINT('Ctrl Pts',(-10.7773260021062,15.2,-2.01061510036421));
#267272=CARTESIAN_POINT('Ctrl Pts',(-10.7816537844946,15.2,-2.01312102315096));
#267273=CARTESIAN_POINT('Ctrl Pts',(-10.7859957688013,15.2,-2.01564710259705));
#267274=CARTESIAN_POINT('Ctrl Pts',(-10.7894693559627,15.2,-2.01766796598872));
#267275=CARTESIAN_POINT('Ctrl Pts',(-10.7929520333507,15.2,-2.01970172907593));
#267276=CARTESIAN_POINT('Ctrl Pts',(-10.7964436717313,15.2,-2.02174841107444));
#267277=CARTESIAN_POINT('Ctrl Pts',(-10.8016811300159,15.2,-2.02481843449049));
#267278=CARTESIAN_POINT('Ctrl Pts',(-10.8069387517696,15.2,-2.02791752556847));
#267279=CARTESIAN_POINT('Ctrl Pts',(-10.8122161100586,15.2,-2.03104574107428));
#267280=CARTESIAN_POINT('Ctrl Pts',(-10.8157343484386,15.2,-2.03313121779401));
#267281=CARTESIAN_POINT('Ctrl Pts',(-10.8192613591206,15.2,-2.03522963990326));
#267282=CARTESIAN_POINT('Ctrl Pts',(-10.8227970175143,15.2,-2.0373410232402));
#267283=CARTESIAN_POINT('Ctrl Pts',(-10.8263326763897,15.2,-2.03945240686481));
#267284=CARTESIAN_POINT('Ctrl Pts',(-10.8298769814559,15.2,-2.0415767519705));
#267285=CARTESIAN_POINT('Ctrl Pts',(-10.8334298103726,15.2,-2.04371407486609));
#267286=CARTESIAN_POINT('Ctrl Pts',(-10.8378708462765,15.2,-2.04638572833997));
#267287=CARTESIAN_POINT('Ctrl Pts',(-10.8423252008944,15.2,-2.04907765926418));
#267288=CARTESIAN_POINT('Ctrl Pts',(-10.8467926318677,15.2,-2.05178989940473));
#267289=CARTESIAN_POINT('Ctrl Pts',(-10.8503665763542,15.2,-2.05395969133979));
#267290=CARTESIAN_POINT('Ctrl Pts',(-10.8539488914665,15.2,-2.0561424805486));
#267291=CARTESIAN_POINT('Ctrl Pts',(-10.8575394540226,15.2,-2.05833828199014));
#267292=CARTESIAN_POINT('Ctrl Pts',(-10.8611300170679,15.2,-2.06053408373086));
#267293=CARTESIAN_POINT('Ctrl Pts',(-10.8647288282285,15.2,-2.06274289860748));
#267294=CARTESIAN_POINT('Ctrl Pts',(-10.8683357671481,15.2,-2.06496474139658));
#267295=CARTESIAN_POINT('Ctrl Pts',(-10.8728444405519,15.2,-2.06774204473157));
#267296=CARTESIAN_POINT('Ctrl Pts',(-10.8773658122587,15.2,-2.07053970168913));
#267297=CARTESIAN_POINT('Ctrl Pts',(-10.8818996505931,15.2,-2.07335774113523));
#267298=CARTESIAN_POINT('Ctrl Pts',(-10.885526720964,15.2,-2.07561217250782));
#267299=CARTESIAN_POINT('Ctrl Pts',(-10.8891617691983,15.2,-2.07787964948287));
#267300=CARTESIAN_POINT('Ctrl Pts',(-10.8928046769725,15.2,-2.08016018480675));
#267301=CARTESIAN_POINT('Ctrl Pts',(-10.8964475852431,15.2,-2.08244072044135));
#267302=CARTESIAN_POINT('Ctrl Pts',(-10.9000983519841,15.2,-2.08473431341673));
#267303=CARTESIAN_POINT('Ctrl Pts',(-10.9037568615732,15.2,-2.08704097887711));
#267304=CARTESIAN_POINT('Ctrl Pts',(-10.9074153706638,15.2,-2.0893476440232));
#267305=CARTESIAN_POINT('Ctrl Pts',(-10.9110816210367,15.2,-2.0916673803426));
#267306=CARTESIAN_POINT('Ctrl Pts',(-10.9147554974581,15.2,-2.09400020031771));
#267307=CARTESIAN_POINT('Ctrl Pts',(-10.91842937438,15.2,-2.09633302061067));
#267308=CARTESIAN_POINT('Ctrl Pts',(-10.9221108745994,15.2,-2.09867892545313));
#267309=CARTESIAN_POINT('Ctrl Pts',(-10.9257998863187,15.2,-2.10103792586734));
#267310=CARTESIAN_POINT('Ctrl Pts',(-10.9304111507165,15.2,-2.1039866762244));
#267311=CARTESIAN_POINT('Ctrl Pts',(-10.9350341478386,15.2,-2.10695588808379));
#267312=CARTESIAN_POINT('Ctrl Pts',(-10.9396686538812,15.2,-2.10994558718269));
#267313=CARTESIAN_POINT('Ctrl Pts',(-10.9443031599238,15.2,-2.11293528628159));
#267314=CARTESIAN_POINT('Ctrl Pts',(-10.9489491760805,15.2,-2.11594546820026));
#267315=CARTESIAN_POINT('Ctrl Pts',(-10.9536064788592,15.2,-2.11897615910472));
#267316=CARTESIAN_POINT('Ctrl Pts',(-10.9564008604249,15.2,-2.12079457358132));
#267317=CARTESIAN_POINT('Ctrl Pts',(-10.9591993058536,15.2,-2.12262037026221));
#267318=CARTESIAN_POINT('Ctrl Pts',(-10.9620017670173,15.2,-2.12445355337138));
#267319=CARTESIAN_POINT('Ctrl Pts',(-10.9648042281809,15.2,-2.12628673648055));
#267320=CARTESIAN_POINT('Ctrl Pts',(-10.9676107047415,15.2,-2.12812730645135));
#267321=CARTESIAN_POINT('Ctrl Pts',(-10.9704211498064,15.2,-2.12997526796818));
#267322=CARTESIAN_POINT('Ctrl Pts',(-10.9732315948713,15.2,-2.13182322948502));
#267323=CARTESIAN_POINT('Ctrl Pts',(-10.9760460097191,15.2,-2.13367858213431));
#267324=CARTESIAN_POINT('Ctrl Pts',(-10.9788643452834,15.2,-2.13554132973329));
#267325=CARTESIAN_POINT('Ctrl Pts',(-10.9816826808476,15.2,-2.13740407733227));
#267326=CARTESIAN_POINT('Ctrl Pts',(-10.9845049378784,15.2,-2.13927422128096));
#267327=CARTESIAN_POINT('Ctrl Pts',(-10.987331069442,15.2,-2.14115176425377));
#267328=CARTESIAN_POINT('Ctrl Pts',(-10.9901572010057,15.2,-2.14302930722657));
#267329=CARTESIAN_POINT('Ctrl Pts',(-10.9929872073303,15.2,-2.14491424832566));
#267330=CARTESIAN_POINT('Ctrl Pts',(-10.9958210424518,15.2,-2.14680659385058));
#267331=CARTESIAN_POINT('Ctrl Pts',(-10.9986548775733,15.2,-2.1486989393755));
#267332=CARTESIAN_POINT('Ctrl Pts',(-11.0014925400843,15.2,-2.15059868867118));
#267333=CARTESIAN_POINT('Ctrl Pts',(-11.0043339846473,15.2,-2.15250584464254));
#267334=CARTESIAN_POINT('Ctrl Pts',(-11.0071754297264,15.2,-2.15441300096038));
#267335=CARTESIAN_POINT('Ctrl Pts',(-11.0100206574732,15.2,-2.15632756378862));
#267336=CARTESIAN_POINT('Ctrl Pts',(-11.0128696201378,15.2,-2.15824953765229));
#267337=CARTESIAN_POINT('Ctrl Pts',(-11.0157185822848,15.2,-2.1601715111668));
#267338=CARTESIAN_POINT('Ctrl Pts',(-11.0185712811649,15.2,-2.1621008959976));
#267339=CARTESIAN_POINT('Ctrl Pts',(-11.0214276693114,15.2,-2.1640376945112));
#267340=CARTESIAN_POINT('Ctrl Pts',(-11.0242840574579,15.2,-2.16597449302479));
#267341=CARTESIAN_POINT('Ctrl Pts',(-11.0271441361437,15.2,-2.16791870628042));
#267342=CARTESIAN_POINT('Ctrl Pts',(-11.0300078597193,15.2,-2.16987033680174));
#267343=CARTESIAN_POINT('Ctrl Pts',(-11.0328715832949,15.2,-2.17182196732306));
#267344=CARTESIAN_POINT('Ctrl Pts',(-11.0357389519054,15.2,-2.17378101551073));
#267345=CARTESIAN_POINT('Ctrl Pts',(-11.0386099189808,15.2,-2.17574748453151));
#267346=CARTESIAN_POINT('Ctrl Pts',(-11.042437875429,15.2,-2.17836944346405));
#267347=CARTESIAN_POINT('Ctrl Pts',(-11.0462722306763,15.2,-2.18100459512617));
#267348=CARTESIAN_POINT('Ctrl Pts',(-11.0501128783863,15.2,-2.18365294671631));
#267349=CARTESIAN_POINT('Ctrl Pts',(-11.0529933639072,15.2,-2.1856392102285));
#267350=CARTESIAN_POINT('Ctrl Pts',(-11.0558773878361,15.2,-2.18763289915694));
#267351=CARTESIAN_POINT('Ctrl Pts',(-11.0587649078148,15.2,-2.18963401520988));
#267352=CARTESIAN_POINT('Ctrl Pts',(-11.0616524277935,15.2,-2.19163513126281));
#267353=CARTESIAN_POINT('Ctrl Pts',(-11.0645434418947,15.2,-2.19364367579918));
#267354=CARTESIAN_POINT('Ctrl Pts',(-11.067437906011,15.2,-2.1956596512768));
#267355=CARTESIAN_POINT('Ctrl Pts',(-11.0703323701273,15.2,-2.19767562675442));
#267356=CARTESIAN_POINT('Ctrl Pts',(-11.0732302853563,15.2,-2.19969903324606));
#267357=CARTESIAN_POINT('Ctrl Pts',(-11.0761316055141,15.2,-2.20172987276479));
#267358=CARTESIAN_POINT('Ctrl Pts',(-11.0790329256718,15.2,-2.20376071228352));
#267359=CARTESIAN_POINT('Ctrl Pts',(-11.0819376525724,15.2,-2.20579898560209));
#267360=CARTESIAN_POINT('Ctrl Pts',(-11.0848457407164,15.2,-2.20784469502711));
#267361=CARTESIAN_POINT('Ctrl Pts',(-11.0877538288605,15.2,-2.20989040445212));
#267362=CARTESIAN_POINT('Ctrl Pts',(-11.0906652795376,15.2,-2.21194354895998));
#267363=CARTESIAN_POINT('Ctrl Pts',(-11.0935800481396,15.2,-2.21400413330076));
#267364=CARTESIAN_POINT('Ctrl Pts',(-11.0964948172711,15.2,-2.21606471801588));
#267365=CARTESIAN_POINT('Ctrl Pts',(-11.0994129042952,15.2,-2.21813274044978));
#267366=CARTESIAN_POINT('Ctrl Pts',(-11.1023342663869,15.2,-2.22020820425242));
#267367=CARTESIAN_POINT('Ctrl Pts',(-11.1052556279479,15.2,-2.22228366767801));
#267368=CARTESIAN_POINT('Ctrl Pts',(-11.108180263692,15.2,-2.22436657203656));
#267369=CARTESIAN_POINT('Ctrl Pts',(-11.1111081308359,15.2,-2.22645691950293));
#267370=CARTESIAN_POINT('Ctrl Pts',(-11.1140359979798,15.2,-2.22854726696931));
#267371=CARTESIAN_POINT('Ctrl Pts',(-11.1169670973626,15.2,-2.23064505736877));
#267372=CARTESIAN_POINT('Ctrl Pts',(-11.1199013844777,15.2,-2.23275029376021));
#267373=CARTESIAN_POINT('Ctrl Pts',(-11.1228356715928,15.2,-2.23485553015164));
#267374=CARTESIAN_POINT('Ctrl Pts',(-11.1257731469575,15.2,-2.23696821061548));
#267375=CARTESIAN_POINT('Ctrl Pts',(-11.1287137680307,15.2,-2.23908833946471));
#267376=CARTESIAN_POINT('Ctrl Pts',(-11.1326345964844,15.2,-2.24191517818711));
#267377=CARTESIAN_POINT('Ctrl Pts',(-11.1365610160725,15.2,-2.24475525504296));
#267378=CARTESIAN_POINT('Ctrl Pts',(-11.1404929271762,15.2,-2.24760857719982));
#267379=CARTESIAN_POINT('Ctrl Pts',(-11.1434418602362,15.2,-2.24974856862308));
#267380=CARTESIAN_POINT('Ctrl Pts',(-11.1463938816293,15.2,-2.25189600957929));
#267381=CARTESIAN_POINT('Ctrl Pts',(-11.1493489488555,15.2,-2.25405090200164));
#267382=CARTESIAN_POINT('Ctrl Pts',(-11.1523040160817,15.2,-2.25620579442399));
#267383=CARTESIAN_POINT('Ctrl Pts',(-11.1552621307969,15.2,-2.25836813808755));
#267384=CARTESIAN_POINT('Ctrl Pts',(-11.1582232489527,15.2,-2.2605379350186));
#267385=CARTESIAN_POINT('Ctrl Pts',(-11.1611843671086,15.2,-2.26270773194965));
#267386=CARTESIAN_POINT('Ctrl Pts',(-11.164148489525,15.2,-2.26488498156748));
#267387=CARTESIAN_POINT('Ctrl Pts',(-11.167115574514,15.2,-2.26706968649798));
#267388=CARTESIAN_POINT('Ctrl Pts',(-11.170082659503,15.2,-2.26925439142848));
#267389=CARTESIAN_POINT('Ctrl Pts',(-11.1730527048343,15.2,-2.27144655127422));
#267390=CARTESIAN_POINT('Ctrl Pts',(-11.1760256714344,15.2,-2.273646166277));
#267391=CARTESIAN_POINT('Ctrl Pts',(-11.1789986380344,15.2,-2.27584578127977));
#267392=CARTESIAN_POINT('Ctrl Pts',(-11.1819745254426,15.2,-2.27805285281535));
#267393=CARTESIAN_POINT('Ctrl Pts',(-11.1849532921257,15.2,-2.28026738127553));
#267394=CARTESIAN_POINT('Ctrl Pts',(-11.1899179034445,15.2,-2.28395826217661));
#267395=CARTESIAN_POINT('Ctrl Pts',(-11.1948905154792,15.2,-2.2876698573484));
#267396=CARTESIAN_POINT('Ctrl Pts',(-11.1998709310052,15.2,-2.29140217336677));
#267397=CARTESIAN_POINT('Ctrl Pts',(-11.2028591802123,15.2,-2.29364156289643));
#267398=CARTESIAN_POINT('Ctrl Pts',(-11.2058502378899,15.2,-2.29588841107478));
#267399=CARTESIAN_POINT('Ctrl Pts',(-11.2088440636141,15.2,-2.29814271999186));
#267400=CARTESIAN_POINT('Ctrl Pts',(-11.2128358316089,15.2,-2.30114846548766));
#267401=CARTESIAN_POINT('Ctrl Pts',(-11.2168325224014,15.2,-2.30416747235136));
#267402=CARTESIAN_POINT('Ctrl Pts',(-11.2208340470084,15.2,-2.30719974451662));
#267403=CARTESIAN_POINT('Ctrl Pts',(-11.2248355716153,15.2,-2.31023201668189));
#267404=CARTESIAN_POINT('Ctrl Pts',(-11.2288419325145,15.2,-2.31327755374869));
#267405=CARTESIAN_POINT('Ctrl Pts',(-11.2328530156225,15.2,-2.31633635725008));
#267406=CARTESIAN_POINT('Ctrl Pts',(-11.2358613276802,15.2,-2.31863045966774));
#267407=CARTESIAN_POINT('Ctrl Pts',(-11.2388722956251,15.2,-2.32093202439778));
#267408=CARTESIAN_POINT('Ctrl Pts',(-11.2418858740831,15.2,-2.32324105243011));
#267409=CARTESIAN_POINT('Ctrl Pts',(-11.2448994525412,15.2,-2.32555008046245));
#267410=CARTESIAN_POINT('Ctrl Pts',(-11.2479156413857,15.2,-2.32786657213309));
#267411=CARTESIAN_POINT('Ctrl Pts',(-11.2509344236132,15.2,-2.33019052657526));
#267412=CARTESIAN_POINT('Ctrl Pts',(-11.2539532058406,15.2,-2.33251448101743));
#267413=CARTESIAN_POINT('Ctrl Pts',(-11.2569745784507,15.2,-2.33484589757511));
#267414=CARTESIAN_POINT('Ctrl Pts',(-11.2599985490001,15.2,-2.33718477800001));
#267415=CARTESIAN_POINT('Ctrl Pts',(-10.2237731100001,12.2,-1.76496130700002));
#267416=CARTESIAN_POINT('Ctrl Pts',(-10.2255010902461,12.2,-1.76541542813168));
#267417=CARTESIAN_POINT('Ctrl Pts',(-10.2272829932875,12.2,-1.76588926588842));
#267418=CARTESIAN_POINT('Ctrl Pts',(-10.2291177142657,12.2,-1.76638321069588));
#267419=CARTESIAN_POINT('Ctrl Pts',(-10.2309612831959,12.2,-1.76687953755489));
#267420=CARTESIAN_POINT('Ctrl Pts',(-10.232858179982,12.2,-1.76739616339468));
#267421=CARTESIAN_POINT('Ctrl Pts',(-10.2348073231887,12.2,-1.76793345428534));
#267422=CARTESIAN_POINT('Ctrl Pts',(-10.2367564662182,12.2,-1.7684707451272));
#267423=CARTESIAN_POINT('Ctrl Pts',(-10.2387578531412,12.2,-1.76902870433768));
#267424=CARTESIAN_POINT('Ctrl Pts',(-10.2408104332333,12.2,-1.76960768598331));
#267425=CARTESIAN_POINT('Ctrl Pts',(-10.2428630133254,12.2,-1.77018666762894));
#267426=CARTESIAN_POINT('Ctrl Pts',(-10.2449667829903,12.2,-1.77078667199102));
#267427=CARTESIAN_POINT('Ctrl Pts',(-10.2471207202667,12.2,-1.77140804341492));
#267428=CARTESIAN_POINT('Ctrl Pts',(-10.2492746577388,12.2,-1.77202941489526));
#267429=CARTESIAN_POINT('Ctrl Pts',(-10.2514787619861,12.2,-1.77267215260972));
#267430=CARTESIAN_POINT('Ctrl Pts',(-10.2537320337789,12.2,-1.77333658806407));
#267431=CARTESIAN_POINT('Ctrl Pts',(-10.2559853053671,12.2,-1.77400102345808));
#267432=CARTESIAN_POINT('Ctrl Pts',(-10.258287747059,12.2,-1.77468715486442));
#267433=CARTESIAN_POINT('Ctrl Pts',(-10.2606383864844,12.2,-1.77539530325863));
#267434=CARTESIAN_POINT('Ctrl Pts',(-10.2629890259098,12.2,-1.77610345165284));
#267435=CARTESIAN_POINT('Ctrl Pts',(-10.2653878629661,12.2,-1.7768336161957));
#267436=CARTESIAN_POINT('Ctrl Pts',(-10.2678339516252,12.2,-1.77758610541739));
#267437=CARTESIAN_POINT('Ctrl Pts',(-10.2702800405064,12.2,-1.77833859470743));
#267438=CARTESIAN_POINT('Ctrl Pts',(-10.2727733800186,12.2,-1.77911340744191));
#267439=CARTESIAN_POINT('Ctrl Pts',(-10.2753130489935,12.2,-1.77991084182023));
#267440=CARTESIAN_POINT('Ctrl Pts',(-10.2778527177377,12.2,-1.78070827612613));
#267441=CARTESIAN_POINT('Ctrl Pts',(-10.2804387162622,12.2,-1.78152833200897));
#267442=CARTESIAN_POINT('Ctrl Pts',(-10.2830701449186,12.2,-1.78237129431268));
#267443=CARTESIAN_POINT('Ctrl Pts',(-10.285701573575,12.2,-1.78321425661639));
#267444=CARTESIAN_POINT('Ctrl Pts',(-10.2883784300777,12.2,-1.7840801268016));
#267445=CARTESIAN_POINT('Ctrl Pts',(-10.2910998398935,12.2,-1.78496918193495));
#267446=CARTESIAN_POINT('Ctrl Pts',(-10.2942748181768,12.2,-1.78600641297769));
#267447=CARTESIAN_POINT('Ctrl Pts',(-10.2975104347728,12.2,-1.78707519872204));
#267448=CARTESIAN_POINT('Ctrl Pts',(-10.3008053326874,12.2,-1.78817596526816));
#267449=CARTESIAN_POINT('Ctrl Pts',(-10.3036295307534,12.2,-1.78911947940158));
#267450=CARTESIAN_POINT('Ctrl Pts',(-10.3064972822325,12.2,-1.79008648825811));
#267451=CARTESIAN_POINT('Ctrl Pts',(-10.3094077542915,12.2,-1.79107724747108));
#267452=CARTESIAN_POINT('Ctrl Pts',(-10.3123182263506,12.2,-1.79206800668404));
#267453=CARTESIAN_POINT('Ctrl Pts',(-10.3152714195936,12.2,-1.79308251806783));
#267454=CARTESIAN_POINT('Ctrl Pts',(-10.3182665168985,12.2,-1.79412102811178));
#267455=CARTESIAN_POINT('Ctrl Pts',(-10.3212616144756,12.2,-1.79515953825006));
#267456=CARTESIAN_POINT('Ctrl Pts',(-10.324298617665,12.2,-1.79622204704902));
#267457=CARTESIAN_POINT('Ctrl Pts',(-10.3273767301679,12.2,-1.79730879327597));
#267458=CARTESIAN_POINT('Ctrl Pts',(-10.3304548423912,12.2,-1.79839553940421));
#267459=CARTESIAN_POINT('Ctrl Pts',(-10.3335740630195,12.2,-1.79950652338883));
#267460=CARTESIAN_POINT('Ctrl Pts',(-10.3367336133196,12.2,-1.80064197642986));
#267461=CARTESIAN_POINT('Ctrl Pts',(-10.3398931636198,12.2,-1.80177742947088));
#267462=CARTESIAN_POINT('Ctrl Pts',(-10.3430930445673,12.2,-1.80293735075724));
#267463=CARTESIAN_POINT('Ctrl Pts',(-10.3463324919469,12.2,-1.80412196462919));
#267464=CARTESIAN_POINT('Ctrl Pts',(-10.3495719396208,12.2,-1.80530657860875));
#267465=CARTESIAN_POINT('Ctrl Pts',(-10.3528509557568,12.2,-1.80651588300733));
#267466=CARTESIAN_POINT('Ctrl Pts',(-10.3561687906893,12.2,-1.80775009682568));
#267467=CARTESIAN_POINT('Ctrl Pts',(-10.3594866253204,12.2,-1.80898431053191));
#267468=CARTESIAN_POINT('Ctrl Pts',(-10.3628432843648,12.2,-1.81024342956528));
#267469=CARTESIAN_POINT('Ctrl Pts',(-10.3662380310068,12.2,-1.81152766727439));
#267470=CARTESIAN_POINT('Ctrl Pts',(-10.3701985689613,12.2,-1.81302594467945));
#267471=CARTESIAN_POINT('Ctrl Pts',(-10.3742109513193,12.2,-1.81455840460315));
#267472=CARTESIAN_POINT('Ctrl Pts',(-10.3782740448983,12.2,-1.81612537086494));
#267473=CARTESIAN_POINT('Ctrl Pts',(-10.3817566963567,12.2,-1.81746848473391));
#267474=CARTESIAN_POINT('Ctrl Pts',(-10.3852766033615,12.2,-1.81883694769372));
#267475=CARTESIAN_POINT('Ctrl Pts',(-10.3888330672484,12.2,-1.82023095448267));
#267476=CARTESIAN_POINT('Ctrl Pts',(-10.3923895311352,12.2,-1.82162496127163));
#267477=CARTESIAN_POINT('Ctrl Pts',(-10.3959825532721,12.2,-1.82304451198837));
#267478=CARTESIAN_POINT('Ctrl Pts',(-10.3996114461378,12.2,-1.82448979285078));
#267479=CARTESIAN_POINT('Ctrl Pts',(-10.4032403393331,12.2,-1.82593507384445));
#267480=CARTESIAN_POINT('Ctrl Pts',(-10.4069051039612,12.2,-1.82740608488698));
#267481=CARTESIAN_POINT('Ctrl Pts',(-10.4106050700997,12.2,-1.82890300687817));
#267482=CARTESIAN_POINT('Ctrl Pts',(-10.413688375047,12.2,-1.83015044180285));
#267483=CARTESIAN_POINT('Ctrl Pts',(-10.4167961221577,12.2,-1.83141587063305));
#267484=CARTESIAN_POINT('Ctrl Pts',(-10.4199279321596,12.2,-1.83269939313452));
#267485=CARTESIAN_POINT('Ctrl Pts',(-10.4230597421616,12.2,-1.833982915636));
#267486=CARTESIAN_POINT('Ctrl Pts',(-10.4262156148528,12.2,-1.83528453491556));
#267487=CARTESIAN_POINT('Ctrl Pts',(-10.4293951724242,12.2,-1.83660434568094));
#267488=CARTESIAN_POINT('Ctrl Pts',(-10.432574729649,12.2,-1.83792415630246));
#267489=CARTESIAN_POINT('Ctrl Pts',(-10.435777973226,12.2,-1.83926216018301));
#267490=CARTESIAN_POINT('Ctrl Pts',(-10.4390045313446,12.2,-1.84061845308924));
#267491=CARTESIAN_POINT('Ctrl Pts',(-10.442231089815,12.2,-1.8419747461433));
#267492=CARTESIAN_POINT('Ctrl Pts',(-10.4454809638072,12.2,-1.84334932791373));
#267493=CARTESIAN_POINT('Ctrl Pts',(-10.4487537873469,12.2,-1.84474229180111));
#267494=CARTESIAN_POINT('Ctrl Pts',(-10.4520266108867,12.2,-1.84613525568848));
#267495=CARTESIAN_POINT('Ctrl Pts',(-10.4553223855062,12.2,-1.84754659954724));
#267496=CARTESIAN_POINT('Ctrl Pts',(-10.4586407501149,12.2,-1.84897641753405));
#267497=CARTESIAN_POINT('Ctrl Pts',(-10.4619591147235,12.2,-1.85040623552086));
#267498=CARTESIAN_POINT('Ctrl Pts',(-10.4653000711647,12.2,-1.85185452354401));
#267499=CARTESIAN_POINT('Ctrl Pts',(-10.4686632630385,12.2,-1.85332137319582));
#267500=CARTESIAN_POINT('Ctrl Pts',(-10.4720264549123,12.2,-1.85478822284762));
#267501=CARTESIAN_POINT('Ctrl Pts',(-10.4754118841618,12.2,-1.85627362960824));
#267502=CARTESIAN_POINT('Ctrl Pts',(-10.4788192010356,12.2,-1.85777768342671));
#267503=CARTESIAN_POINT('Ctrl Pts',(-10.4822265179095,12.2,-1.85928173724519));
#267504=CARTESIAN_POINT('Ctrl Pts',(-10.4856557227825,12.2,-1.86080443447551));
#267505=CARTESIAN_POINT('Ctrl Pts',(-10.4891064705065,12.2,-1.86234586073246));
#267506=CARTESIAN_POINT('Ctrl Pts',(-10.4925572182304,12.2,-1.86388728698941));
#267507=CARTESIAN_POINT('Ctrl Pts',(-10.4960295093722,12.2,-1.86544744086663));
#267508=CARTESIAN_POINT('Ctrl Pts',(-10.4995230054833,12.2,-1.86702640149163));
#267509=CARTESIAN_POINT('Ctrl Pts',(-10.5030165015945,12.2,-1.86860536211663));
#267510=CARTESIAN_POINT('Ctrl Pts',(-10.506531203358,12.2,-1.87020313199346));
#267511=CARTESIAN_POINT('Ctrl Pts',(-10.5100667744853,12.2,-1.87181978679252));
#267512=CARTESIAN_POINT('Ctrl Pts',(-10.5136023456125,12.2,-1.87343644159158));
#267513=CARTESIAN_POINT('Ctrl Pts',(-10.5171587875552,12.2,-1.87507198386286));
#267514=CARTESIAN_POINT('Ctrl Pts',(-10.5207357695007,12.2,-1.87672648684995));
#267515=CARTESIAN_POINT('Ctrl Pts',(-10.5243127514462,12.2,-1.87838098983705));
#267516=CARTESIAN_POINT('Ctrl Pts',(-10.5279102734079,12.2,-1.8800544542209));
#267517=CARTESIAN_POINT('Ctrl Pts',(-10.5315280120201,12.2,-1.88174695456911));
#267518=CARTESIAN_POINT('Ctrl Pts',(-10.5351457506322,12.2,-1.88343945491733));
#267519=CARTESIAN_POINT('Ctrl Pts',(-10.5387837034383,12.2,-1.88515099101782));
#267520=CARTESIAN_POINT('Ctrl Pts',(-10.542441551981,12.2,-1.8868816331716));
#267521=CARTESIAN_POINT('Ctrl Pts',(-10.5460994005237,12.2,-1.88861227532538));
#267522=CARTESIAN_POINT('Ctrl Pts',(-10.5497771429487,12.2,-1.89036202468788));
#267523=CARTESIAN_POINT('Ctrl Pts',(-10.5534744636209,12.2,-1.89213095026371));
#267524=CARTESIAN_POINT('Ctrl Pts',(-10.5571717842932,12.2,-1.89389987583954));
#267525=CARTESIAN_POINT('Ctrl Pts',(-10.5608886844426,12.2,-1.89568797632368));
#267526=CARTESIAN_POINT('Ctrl Pts',(-10.5646248482637,12.2,-1.89749532097804));
#267527=CARTESIAN_POINT('Ctrl Pts',(-10.5676137790762,12.2,-1.89894119658332));
#267528=CARTESIAN_POINT('Ctrl Pts',(-10.5706150406843,12.2,-1.900399387862));
#267529=CARTESIAN_POINT('Ctrl Pts',(-10.5736284747704,12.2,-1.90186992862987));
#267530=CARTESIAN_POINT('Ctrl Pts',(-10.5766419092672,12.2,-1.9033404695981));
#267531=CARTESIAN_POINT('Ctrl Pts',(-10.5796675142364,12.2,-1.90482335909585));
#267532=CARTESIAN_POINT('Ctrl Pts',(-10.5827051361659,12.2,-1.90631863097534));
#267533=CARTESIAN_POINT('Ctrl Pts',(-10.5857427576814,12.2,-1.9078139026511));
#267534=CARTESIAN_POINT('Ctrl Pts',(-10.5887923936676,12.2,-1.90932155614812));
#267535=CARTESIAN_POINT('Ctrl Pts',(-10.5918538917498,12.2,-1.91084162363415));
#267536=CARTESIAN_POINT('Ctrl Pts',(-10.5949153902492,12.2,-1.9123616913273));
#267537=CARTESIAN_POINT('Ctrl Pts',(-10.5979887495418,12.2,-1.91389417279693));
#267538=CARTESIAN_POINT('Ctrl Pts',(-10.601073815544,12.2,-1.91543909865971));
#267539=CARTESIAN_POINT('Ctrl Pts',(-10.6041588811259,12.2,-1.916984024312));
#267540=CARTESIAN_POINT('Ctrl Pts',(-10.607255655185,12.2,-1.91854139660934));
#267541=CARTESIAN_POINT('Ctrl Pts',(-10.6103639848074,12.2,-1.92011124228058));
#267542=CARTESIAN_POINT('Ctrl Pts',(-10.6134723148533,12.2,-1.9216810881657));
#267543=CARTESIAN_POINT('Ctrl Pts',(-10.6165922000125,12.2,-1.92326341040938));
#267544=CARTESIAN_POINT('Ctrl Pts',(-10.6197234907394,12.2,-1.92485823683046));
#267545=CARTESIAN_POINT('Ctrl Pts',(-10.6236376039348,12.2,-1.92685176974816));
#267546=CARTESIAN_POINT('Ctrl Pts',(-10.6275695389298,12.2,-1.92886484250423));
#267547=CARTESIAN_POINT('Ctrl Pts',(-10.6315190052501,12.2,-1.93089750965803));
#267548=CARTESIAN_POINT('Ctrl Pts',(-10.6346785780481,12.2,-1.93252364324812));
#267549=CARTESIAN_POINT('Ctrl Pts',(-10.6378493697099,12.2,-1.93416231752513));
#267550=CARTESIAN_POINT('Ctrl Pts',(-10.64103123533,12.2,-1.9358135610271));
#267551=CARTESIAN_POINT('Ctrl Pts',(-10.6442131013837,12.2,-1.93746480475404));
#267552=CARTESIAN_POINT('Ctrl Pts',(-10.6474060403006,12.2,-1.93912861803384));
#267553=CARTESIAN_POINT('Ctrl Pts',(-10.6506099057537,12.2,-1.94080502590379));
#267554=CARTESIAN_POINT('Ctrl Pts',(-10.6538137707703,12.2,-1.94248143354534));
#267555=CARTESIAN_POINT('Ctrl Pts',(-10.6570285647847,12.2,-1.94417043913438));
#267556=CARTESIAN_POINT('Ctrl Pts',(-10.6602541404643,12.2,-1.94587206543842));
#267557=CARTESIAN_POINT('Ctrl Pts',(-10.6634797165834,12.2,-1.94757369197431));
#267558=CARTESIAN_POINT('Ctrl Pts',(-10.6667160762633,12.2,-1.94928794342693));
#267559=CARTESIAN_POINT('Ctrl Pts',(-10.6699630775106,12.2,-1.95101484175114));
#267560=CARTESIAN_POINT('Ctrl Pts',(-10.6732100783154,12.2,-1.95274173984006));
#267561=CARTESIAN_POINT('Ctrl Pts',(-10.6764677183284,12.2,-1.95448128654135));
#267562=CARTESIAN_POINT('Ctrl Pts',(-10.679735857949,12.2,-1.95623350673015));
#267563=CARTESIAN_POINT('Ctrl Pts',(-10.6830039980149,12.2,-1.95798572715768));
#267564=CARTESIAN_POINT('Ctrl Pts',(-10.6862826371819,12.2,-1.95975062156697));
#267565=CARTESIAN_POINT('Ctrl Pts',(-10.68957163525,12.2,-1.96152821394163));
#267566=CARTESIAN_POINT('Ctrl Pts',(-10.6928606333181,12.2,-1.96330580631628));
#267567=CARTESIAN_POINT('Ctrl Pts',(-10.6961599906042,12.2,-1.96509609748965));
#267568=CARTESIAN_POINT('Ctrl Pts',(-10.6994695680078,12.2,-1.9668991104781));
#267569=CARTESIAN_POINT('Ctrl Pts',(-10.7027791449605,12.2,-1.96870212322088));
#267570=CARTESIAN_POINT('Ctrl Pts',(-10.7060989423993,12.2,-1.97051785785383));
#267571=CARTESIAN_POINT('Ctrl Pts',(-10.7094288220311,12.2,-1.97234633799039));
#267572=CARTESIAN_POINT('Ctrl Pts',(-10.7127587021165,12.2,-1.97417481837608));
#267573=CARTESIAN_POINT('Ctrl Pts',(-10.7160986645253,12.2,-1.97601604464519));
#267574=CARTESIAN_POINT('Ctrl Pts',(-10.7194485732644,12.2,-1.9778700383031));
#267575=CARTESIAN_POINT('Ctrl Pts',(-10.7227984815471,12.2,-1.9797240317084));
#267576=CARTESIAN_POINT('Ctrl Pts',(-10.7261583367035,12.2,-1.98159079284259));
#267577=CARTESIAN_POINT('Ctrl Pts',(-10.729528002483,12.2,-1.98347034485477));
#267578=CARTESIAN_POINT('Ctrl Pts',(-10.7328976687215,12.2,-1.98534989712303));
#267579=CARTESIAN_POINT('Ctrl Pts',(-10.7362771462287,12.2,-1.98724223897082));
#267580=CARTESIAN_POINT('Ctrl Pts',(-10.7396663017502,12.2,-1.98914739205982));
#267581=CARTESIAN_POINT('Ctrl Pts',(-10.7430554568099,12.2,-1.99105254488924));
#267582=CARTESIAN_POINT('Ctrl Pts',(-10.7464542883118,12.2,-1.99297050843982));
#267583=CARTESIAN_POINT('Ctrl Pts',(-10.7498626652548,12.2,-1.99490130505891));
#267584=CARTESIAN_POINT('Ctrl Pts',(-10.7532710426621,12.2,-1.99683210194107));
#267585=CARTESIAN_POINT('Ctrl Pts',(-10.7566889635401,12.2,-1.99877572959145));
#267586=CARTESIAN_POINT('Ctrl Pts',(-10.7601162983386,12.2,-2.00073221114336));
#267587=CARTESIAN_POINT('Ctrl Pts',(-10.7635436326702,12.2,-2.0026886924287));
#267588=CARTESIAN_POINT('Ctrl Pts',(-10.7669803790409,12.2,-2.00465802463765));
#267589=CARTESIAN_POINT('Ctrl Pts',(-10.7704264095417,12.2,-2.00664022946241));
#267590=CARTESIAN_POINT('Ctrl Pts',(-10.773872440512,12.2,-2.00862243455724));
#267591=CARTESIAN_POINT('Ctrl Pts',(-10.777327753005,12.2,-2.01061751139563));
#267592=CARTESIAN_POINT('Ctrl Pts',(-10.78079221975,12.2,-2.01262547967257));
#267593=CARTESIAN_POINT('Ctrl Pts',(-10.7842566860229,12.2,-2.01463344767593));
#267594=CARTESIAN_POINT('Ctrl Pts',(-10.7877303053996,12.2,-2.01665430669337));
#267595=CARTESIAN_POINT('Ctrl Pts',(-10.7912129504473,12.2,-2.01868807469245));
#267596=CARTESIAN_POINT('Ctrl Pts',(-10.7946955959695,12.2,-2.02072184296864));
#267597=CARTESIAN_POINT('Ctrl Pts',(-10.7981872667314,12.2,-2.02276852037937));
#267598=CARTESIAN_POINT('Ctrl Pts',(-10.8016878350333,12.2,-2.02482812599162));
#267599=CARTESIAN_POINT('Ctrl Pts',(-10.8051884033352,12.2,-2.02688773160387));
#267600=CARTESIAN_POINT('Ctrl Pts',(-10.8086978711993,12.2,-2.02896026407041));
#267601=CARTESIAN_POINT('Ctrl Pts',(-10.8122161100586,12.2,-2.03104574107428));
#267602=CARTESIAN_POINT('Ctrl Pts',(-10.8157343484386,12.2,-2.03313121779401));
#267603=CARTESIAN_POINT('Ctrl Pts',(-10.8192613591206,12.2,-2.03522963990326));
#267604=CARTESIAN_POINT('Ctrl Pts',(-10.8227970175143,12.2,-2.03734102324019));
#267605=CARTESIAN_POINT('Ctrl Pts',(-10.8263326763897,12.2,-2.03945240686481));
#267606=CARTESIAN_POINT('Ctrl Pts',(-10.8298769814559,12.2,-2.0415767519705));
#267607=CARTESIAN_POINT('Ctrl Pts',(-10.8334298103726,12.2,-2.04371407486609));
#267608=CARTESIAN_POINT('Ctrl Pts',(-10.8369826388052,12.2,-2.04585139747047));
#267609=CARTESIAN_POINT('Ctrl Pts',(-10.8405439902784,12.2,-2.04800169673705));
#267610=CARTESIAN_POINT('Ctrl Pts',(-10.8441137432083,12.2,-2.05016499128157));
#267611=CARTESIAN_POINT('Ctrl Pts',(-10.8485759347354,12.2,-2.05286910968329));
#267612=CARTESIAN_POINT('Ctrl Pts',(-10.8530512504606,12.2,-2.05559352996384));
#267613=CARTESIAN_POINT('Ctrl Pts',(-10.8575394540226,12.2,-2.05833828199014));
#267614=CARTESIAN_POINT('Ctrl Pts',(-10.8611300170679,12.2,-2.06053408373086));
#267615=CARTESIAN_POINT('Ctrl Pts',(-10.8647288282285,12.2,-2.06274289860748));
#267616=CARTESIAN_POINT('Ctrl Pts',(-10.8683357671481,12.2,-2.06496474139658));
#267617=CARTESIAN_POINT('Ctrl Pts',(-10.8719427055763,12.2,-2.06718658388294));
#267618=CARTESIAN_POINT('Ctrl Pts',(-10.8755577714756,12.2,-2.06942145178704));
#267619=CARTESIAN_POINT('Ctrl Pts',(-10.8791808446789,12.2,-2.07166936232466));
#267620=CARTESIAN_POINT('Ctrl Pts',(-10.8828039183759,12.2,-2.07391727316855));
#267621=CARTESIAN_POINT('Ctrl Pts',(-10.8864350008862,12.2,-2.07617822391079));
#267622=CARTESIAN_POINT('Ctrl Pts',(-10.8900739720448,12.2,-2.07845223153834));
#267623=CARTESIAN_POINT('Ctrl Pts',(-10.8937129427075,12.2,-2.08072623885605));
#267624=CARTESIAN_POINT('Ctrl Pts',(-10.8973598017395,12.2,-2.08301330084816));
#267625=CARTESIAN_POINT('Ctrl Pts',(-10.901014432218,12.2,-2.08531343027038));
#267626=CARTESIAN_POINT('Ctrl Pts',(-10.9046690631944,12.2,-2.087613560006));
#267627=CARTESIAN_POINT('Ctrl Pts',(-10.9083314651191,12.2,-2.08992675893207));
#267628=CARTESIAN_POINT('Ctrl Pts',(-10.9120015220418,12.2,-2.09225303844859));
#267629=CARTESIAN_POINT('Ctrl Pts',(-10.9156715784645,12.2,-2.09457931764816));
#267630=CARTESIAN_POINT('Ctrl Pts',(-10.9193492880053,12.2,-2.09691867683739));
#267631=CARTESIAN_POINT('Ctrl Pts',(-10.9230345366653,12.2,-2.09927113015035));
#267632=CARTESIAN_POINT('Ctrl Pts',(-10.9267197858274,12.2,-2.10162358378383));
#267633=CARTESIAN_POINT('Ctrl Pts',(-10.9304125733227,12.2,-2.10398913007794));
#267634=CARTESIAN_POINT('Ctrl Pts',(-10.9341127843026,12.2,-2.10636778048621));
#267635=CARTESIAN_POINT('Ctrl Pts',(-10.9378129947784,12.2,-2.10874643057038));
#267636=CARTESIAN_POINT('Ctrl Pts',(-10.9415206274026,12.2,-2.11113818704638));
#267637=CARTESIAN_POINT('Ctrl Pts',(-10.945235569876,12.2,-2.11354305834844));
#267638=CARTESIAN_POINT('Ctrl Pts',(-10.9489505128555,12.2,-2.11594792997817));
#267639=CARTESIAN_POINT('Ctrl Pts',(-10.9526727650712,12.2,-2.11836591876081));
#267640=CARTESIAN_POINT('Ctrl Pts',(-10.9564022127359,12.2,-2.12079703429329));
#267641=CARTESIAN_POINT('Ctrl Pts',(-10.9591992982303,12.2,-2.12262037077703));
#267642=CARTESIAN_POINT('Ctrl Pts',(-10.96200043152,12.2,-2.12445109042344));
#267643=CARTESIAN_POINT('Ctrl Pts',(-10.9648055645141,12.2,-2.12628919848996));
#267644=CARTESIAN_POINT('Ctrl Pts',(-10.9676106975083,12.2,-2.12812730655649));
#267645=CARTESIAN_POINT('Ctrl Pts',(-10.9704198296627,12.2,-2.12997280354942));
#267646=CARTESIAN_POINT('Ctrl Pts',(-10.9732329156851,12.2,-2.13182569302312));
#267647=CARTESIAN_POINT('Ctrl Pts',(-10.9760460017076,12.2,-2.13367858249682));
#267648=CARTESIAN_POINT('Ctrl Pts',(-10.9788630410381,12.2,-2.13553886364502));
#267649=CARTESIAN_POINT('Ctrl Pts',(-10.9816839856017,12.2,-2.13740654257615));
#267650=CARTESIAN_POINT('Ctrl Pts',(-10.9845049306779,12.2,-2.13927422184658));
#267651=CARTESIAN_POINT('Ctrl Pts',(-10.9873297817884,12.2,-2.14114929813576));
#267652=CARTESIAN_POINT('Ctrl Pts',(-10.9901584918667,12.2,-2.14303177445202));
#267653=CARTESIAN_POINT('Ctrl Pts',(-10.9929872014311,12.2,-2.14491425042629));
#267654=CARTESIAN_POINT('Ctrl Pts',(-10.9958197711097,12.2,-2.14680412655707));
#267655=CARTESIAN_POINT('Ctrl Pts',(-10.9986561528155,12.2,-2.14870140816711));
#267656=CARTESIAN_POINT('Ctrl Pts',(-11.0014925345213,12.2,-2.15059868977715));
#267657=CARTESIAN_POINT('Ctrl Pts',(-11.0043327282631,12.2,-2.15250337611066));
#267658=CARTESIAN_POINT('Ctrl Pts',(-11.0071766892851,12.2,-2.15441547016684));
#267659=CARTESIAN_POINT('Ctrl Pts',(-11.0109686371422,12.2,-2.15696492879262));
#267660=CARTESIAN_POINT('Ctrl Pts',(-11.0147672805285,12.2,-2.15952755784075));
#267661=CARTESIAN_POINT('Ctrl Pts',(-11.0185725116612,12.2,-2.16210336629549));
#267662=CARTESIAN_POINT('Ctrl Pts',(-11.0214264356588,12.2,-2.16403522307523));
#267663=CARTESIAN_POINT('Ctrl Pts',(-11.0242840643241,12.2,-2.16597449195708));
#267664=CARTESIAN_POINT('Ctrl Pts',(-11.0271453534071,12.2,-2.16792117865768));
#267665=CARTESIAN_POINT('Ctrl Pts',(-11.0300066419703,12.2,-2.16986786500463));
#267666=CARTESIAN_POINT('Ctrl Pts',(-11.0328715910656,12.2,-2.17182196663529));
#267667=CARTESIAN_POINT('Ctrl Pts',(-11.0357401538134,12.2,-2.17378348912121));
#267668=CARTESIAN_POINT('Ctrl Pts',(-11.0386087165612,12.2,-2.17574501160713));
#267669=CARTESIAN_POINT('Ctrl Pts',(-11.041480893201,12.2,-2.17771395327));
#267670=CARTESIAN_POINT('Ctrl Pts',(-11.0443566393052,12.2,-2.17969031824051));
#267671=CARTESIAN_POINT('Ctrl Pts',(-11.0472323854094,12.2,-2.18166668321103));
#267672=CARTESIAN_POINT('Ctrl Pts',(-11.0501117016214,12.2,-2.18365047098897));
#267673=CARTESIAN_POINT('Ctrl Pts',(-11.0529945412667,12.2,-2.18564168495829));
#267674=CARTESIAN_POINT('Ctrl Pts',(-11.055877380912,12.2,-2.18763289892761));
#267675=CARTESIAN_POINT('Ctrl Pts',(-11.0587637458904,12.2,-2.18963153852162));
#267676=CARTESIAN_POINT('Ctrl Pts',(-11.0616535904518,12.2,-2.19163760703143));
#267677=CARTESIAN_POINT('Ctrl Pts',(-11.0645434350131,12.2,-2.19364367554123));
#267678=CARTESIAN_POINT('Ctrl Pts',(-11.0674367584672,12.2,-2.19565717373235));
#267679=CARTESIAN_POINT('Ctrl Pts',(-11.070333518173,12.2,-2.19767810334237));
#267680=CARTESIAN_POINT('Ctrl Pts',(-11.0732302778787,12.2,-2.19969903295239));
#267681=CARTESIAN_POINT('Ctrl Pts',(-11.0761304727397,12.2,-2.20172739428115));
#267682=CARTESIAN_POINT('Ctrl Pts',(-11.0790340588421,12.2,-2.2037631897895));
#267683=CARTESIAN_POINT('Ctrl Pts',(-11.0819376454719,12.2,-2.20579898566768));
#267684=CARTESIAN_POINT('Ctrl Pts',(-11.0848446236777,12.2,-2.20784221679796));
#267685=CARTESIAN_POINT('Ctrl Pts',(-11.0877549488512,12.2,-2.20989288372202));
#267686=CARTESIAN_POINT('Ctrl Pts',(-11.0906652734959,12.2,-2.21194355027354));
#267687=CARTESIAN_POINT('Ctrl Pts',(-11.0935789464071,12.2,-2.2140016547163));
#267688=CARTESIAN_POINT('Ctrl Pts',(-11.0964959220514,12.2,-2.2160671977669));
#267689=CARTESIAN_POINT('Ctrl Pts',(-11.0994128976957,12.2,-2.2181327408175));
#267690=CARTESIAN_POINT('Ctrl Pts',(-11.1023331776563,12.2,-2.22020572342555));
#267691=CARTESIAN_POINT('Ctrl Pts',(-11.1052567172584,12.2,-2.22228614747496));
#267692=CARTESIAN_POINT('Ctrl Pts',(-11.1081802568605,12.2,-2.22436657152438));
#267693=CARTESIAN_POINT('Ctrl Pts',(-11.1111070560874,12.2,-2.22645443796513));
#267694=CARTESIAN_POINT('Ctrl Pts',(-11.1140370731474,12.2,-2.22854974751337));
#267695=CARTESIAN_POINT('Ctrl Pts',(-11.1169670902073,12.2,-2.2306450570616));
#267696=CARTESIAN_POINT('Ctrl Pts',(-11.1199003244256,12.2,-2.23274781174721));
#267697=CARTESIAN_POINT('Ctrl Pts',(-11.1228367322153,12.2,-2.23485801135843));
#267698=CARTESIAN_POINT('Ctrl Pts',(-11.1257731400049,12.2,-2.23696821096966));
#267699=CARTESIAN_POINT('Ctrl Pts',(-11.1287127222325,12.2,-2.2390858568816));
#267700=CARTESIAN_POINT('Ctrl Pts',(-11.1316554353335,12.2,-2.24121095034504));
#267701=CARTESIAN_POINT('Ctrl Pts',(-11.1345981489691,12.2,-2.24333604419453));
#267702=CARTESIAN_POINT('Ctrl Pts',(-11.1375439935806,12.2,-2.24546858538778));
#267703=CARTESIAN_POINT('Ctrl Pts',(-11.1404929271762,12.2,-2.24760857719981));
#267704=CARTESIAN_POINT('Ctrl Pts',(-11.1434418602362,12.2,-2.24974856862307));
#267705=CARTESIAN_POINT('Ctrl Pts',(-11.1463938816293,12.2,-2.25189600957929));
#267706=CARTESIAN_POINT('Ctrl Pts',(-11.1493489488555,12.2,-2.25405090200164));
#267707=CARTESIAN_POINT('Ctrl Pts',(-11.1523040160817,12.2,-2.25620579442399));
#267708=CARTESIAN_POINT('Ctrl Pts',(-11.1552621307969,12.2,-2.25836813808755));
#267709=CARTESIAN_POINT('Ctrl Pts',(-11.1582232489527,12.2,-2.2605379350186));
#267710=CARTESIAN_POINT('Ctrl Pts',(-11.1611843671086,12.2,-2.26270773194965));
#267711=CARTESIAN_POINT('Ctrl Pts',(-11.164148489525,12.2,-2.26488498156748));
#267712=CARTESIAN_POINT('Ctrl Pts',(-11.167115574514,12.2,-2.26706968649798));
#267713=CARTESIAN_POINT('Ctrl Pts',(-11.170082659503,12.2,-2.26925439142848));
#267714=CARTESIAN_POINT('Ctrl Pts',(-11.1730527048343,12.2,-2.27144655127423));
#267715=CARTESIAN_POINT('Ctrl Pts',(-11.1760256714344,12.2,-2.273646166277));
#267716=CARTESIAN_POINT('Ctrl Pts',(-11.1789986380344,12.2,-2.27584578127977));
#267717=CARTESIAN_POINT('Ctrl Pts',(-11.1819745254426,12.2,-2.27805285281535));
#267718=CARTESIAN_POINT('Ctrl Pts',(-11.1849532921257,12.2,-2.28026738127554));
#267719=CARTESIAN_POINT('Ctrl Pts',(-11.1879320593499,12.2,-2.28248191013803));
#267720=CARTESIAN_POINT('Ctrl Pts',(-11.1909137074332,12.2,-2.28470389609429));
#267721=CARTESIAN_POINT('Ctrl Pts',(-11.1938981922006,12.2,-2.28693334050264));
#267722=CARTESIAN_POINT('Ctrl Pts',(-11.1968826764259,12.2,-2.28916278450598));
#267723=CARTESIAN_POINT('Ctrl Pts',(-11.1998699989042,12.2,-2.29139968778616));
#267724=CARTESIAN_POINT('Ctrl Pts',(-11.2028601157786,12.2,-2.29364404990093));
#267725=CARTESIAN_POINT('Ctrl Pts',(-11.2068469380967,12.2,-2.29663653258472));
#267726=CARTESIAN_POINT('Ctrl Pts',(-11.2108387281032,12.2,-2.29964227782317));
#267727=CARTESIAN_POINT('Ctrl Pts',(-11.214835396165,12.2,-2.30266128501995));
#267728=CARTESIAN_POINT('Ctrl Pts',(-11.2178328973476,12.2,-2.30492554052038));
#267729=CARTESIAN_POINT('Ctrl Pts',(-11.2208331432215,12.2,-2.30719725682027));
#267730=CARTESIAN_POINT('Ctrl Pts',(-11.2238360943204,12.2,-2.30947643523644));
#267731=CARTESIAN_POINT('Ctrl Pts',(-11.2268390459648,12.2,-2.31175561406666));
#267732=CARTESIAN_POINT('Ctrl Pts',(-11.2298447030183,12.2,-2.31404225441566));
#267733=CARTESIAN_POINT('Ctrl Pts',(-11.2328530156225,12.2,-2.31633635725008));
#267734=CARTESIAN_POINT('Ctrl Pts',(-11.2358613276802,12.2,-2.31863045966774));
#267735=CARTESIAN_POINT('Ctrl Pts',(-11.2388722956251,12.2,-2.32093202439778));
#267736=CARTESIAN_POINT('Ctrl Pts',(-11.2418858740831,12.2,-2.32324105243011));
#267737=CARTESIAN_POINT('Ctrl Pts',(-11.2448994525412,12.2,-2.32555008046245));
#267738=CARTESIAN_POINT('Ctrl Pts',(-11.2479156413857,12.2,-2.32786657213309));
#267739=CARTESIAN_POINT('Ctrl Pts',(-11.2509344236132,12.2,-2.33019052657526));
#267740=CARTESIAN_POINT('Ctrl Pts',(-11.2539532058406,12.2,-2.33251448101743));
#267741=CARTESIAN_POINT('Ctrl Pts',(-11.2569745784507,12.2,-2.33484589757511));
#267742=CARTESIAN_POINT('Ctrl Pts',(-11.2599985490001,12.2,-2.33718477800001));
#267743=CARTESIAN_POINT('Ctrl Pts',(-11.1757778680001,15.2,-2.71145515300002));
#267744=CARTESIAN_POINT('Ctrl Pts',(-11.1757778680001,11.6,-2.71145515300002));
#267745=CARTESIAN_POINT('Ctrl Pts',(-11.1750309950001,15.2,-2.71161876900001));
#267746=CARTESIAN_POINT('Ctrl Pts',(-11.1750309950001,11.6,-2.71161876900001));
#267747=CARTESIAN_POINT('Ctrl Pts',(-11.1735376180001,15.2,-2.71194562400002));
#267748=CARTESIAN_POINT('Ctrl Pts',(-11.1735376180001,11.6,-2.71194562400002));
#267749=CARTESIAN_POINT('Ctrl Pts',(-11.1712986600001,15.2,-2.71243478000001));
#267750=CARTESIAN_POINT('Ctrl Pts',(-11.1712986600001,11.6,-2.71243478000002));
#267751=CARTESIAN_POINT('Ctrl Pts',(-11.1683155990001,15.2,-2.71308473500001));
#267752=CARTESIAN_POINT('Ctrl Pts',(-11.1683155990001,11.6,-2.71308473500001));
#267753=CARTESIAN_POINT('Ctrl Pts',(-11.1645904650001,15.2,-2.71389342400001));
#267754=CARTESIAN_POINT('Ctrl Pts',(-11.1645904650001,11.6,-2.71389342400001));
#267755=CARTESIAN_POINT('Ctrl Pts',(-11.1608690250001,15.2,-2.71469835800001));
#267756=CARTESIAN_POINT('Ctrl Pts',(-11.1608690250001,11.6,-2.71469835800001));
#267757=CARTESIAN_POINT('Ctrl Pts',(-11.1571512810001,15.2,-2.71549953800001));
#267758=CARTESIAN_POINT('Ctrl Pts',(-11.1571512810001,11.6,-2.71549953800002));
#267759=CARTESIAN_POINT('Ctrl Pts',(-11.1534372360001,15.2,-2.71629696600002));
#267760=CARTESIAN_POINT('Ctrl Pts',(-11.1534372360001,11.6,-2.71629696600002));
#267761=CARTESIAN_POINT('Ctrl Pts',(-11.1497268980001,15.2,-2.71709064400001));
#267762=CARTESIAN_POINT('Ctrl Pts',(-11.1497268980001,11.6,-2.71709064400001));
#267763=CARTESIAN_POINT('Ctrl Pts',(-11.1460202710001,15.2,-2.71788057600002));
#267764=CARTESIAN_POINT('Ctrl Pts',(-11.1460202710001,11.6,-2.71788057600002));
#267765=CARTESIAN_POINT('Ctrl Pts',(-11.1423173660001,15.2,-2.71866676600002));
#267766=CARTESIAN_POINT('Ctrl Pts',(-11.1423173660001,11.6,-2.71866676600002));
#267767=CARTESIAN_POINT('Ctrl Pts',(-11.1386181920001,15.2,-2.71944921800001));
#267768=CARTESIAN_POINT('Ctrl Pts',(-11.1386181920001,11.6,-2.71944921800001));
#267769=CARTESIAN_POINT('Ctrl Pts',(-11.1349227590001,15.2,-2.72022793900002));
#267770=CARTESIAN_POINT('Ctrl Pts',(-11.1349227590001,11.6,-2.72022793900002));
#267771=CARTESIAN_POINT('Ctrl Pts',(-11.1312310760001,15.2,-2.72100293300001));
#267772=CARTESIAN_POINT('Ctrl Pts',(-11.1312310760001,11.6,-2.72100293300001));
#267773=CARTESIAN_POINT('Ctrl Pts',(-11.1275431540001,15.2,-2.72177420400002));
#267774=CARTESIAN_POINT('Ctrl Pts',(-11.1275431540001,11.6,-2.72177420400002));
#267775=CARTESIAN_POINT('Ctrl Pts',(-11.1238590000001,15.2,-2.72254175700001));
#267776=CARTESIAN_POINT('Ctrl Pts',(-11.1238590000001,11.6,-2.72254175700001));
#267777=CARTESIAN_POINT('Ctrl Pts',(-11.1201786230001,15.2,-2.72330559600002));
#267778=CARTESIAN_POINT('Ctrl Pts',(-11.1201786230001,11.6,-2.72330559600002));
#267779=CARTESIAN_POINT('Ctrl Pts',(-11.1165020290001,15.2,-2.72406572300001));
#267780=CARTESIAN_POINT('Ctrl Pts',(-11.1165020290001,11.6,-2.72406572300001));
#267781=CARTESIAN_POINT('Ctrl Pts',(-11.1128292270001,15.2,-2.72482214500001));
#267782=CARTESIAN_POINT('Ctrl Pts',(-11.1128292270001,11.6,-2.72482214500001));
#267783=CARTESIAN_POINT('Ctrl Pts',(-11.1091602230001,15.2,-2.72557486300002));
#267784=CARTESIAN_POINT('Ctrl Pts',(-11.1091602230001,11.6,-2.72557486300002));
#267785=CARTESIAN_POINT('Ctrl Pts',(-11.1054950240001,15.2,-2.72632388100002));
#267786=CARTESIAN_POINT('Ctrl Pts',(-11.1054950240001,11.6,-2.72632388100002));
#267787=CARTESIAN_POINT('Ctrl Pts',(-11.1018336410001,15.2,-2.72706920300001));
#267788=CARTESIAN_POINT('Ctrl Pts',(-11.1018336410001,11.6,-2.72706920300001));
#267789=CARTESIAN_POINT('Ctrl Pts',(-11.0981760790001,15.2,-2.72781083400002));
#267790=CARTESIAN_POINT('Ctrl Pts',(-11.0981760790001,11.6,-2.72781083400002));
#267791=CARTESIAN_POINT('Ctrl Pts',(-11.0945223470001,15.2,-2.72854877900001));
#267792=CARTESIAN_POINT('Ctrl Pts',(-11.0945223470001,11.6,-2.72854877900001));
#267793=CARTESIAN_POINT('Ctrl Pts',(-11.0908724560001,15.2,-2.72928304000001));
#267794=CARTESIAN_POINT('Ctrl Pts',(-11.0908724560001,11.6,-2.72928304000001));
#267795=CARTESIAN_POINT('Ctrl Pts',(-11.0872264110001,15.2,-2.73001362300001));
#267796=CARTESIAN_POINT('Ctrl Pts',(-11.0872264110001,11.6,-2.73001362300001));
#267797=CARTESIAN_POINT('Ctrl Pts',(-11.0835842240001,15.2,-2.73074053200002));
#267798=CARTESIAN_POINT('Ctrl Pts',(-11.0835842240001,11.6,-2.73074053200002));
#267799=CARTESIAN_POINT('Ctrl Pts',(-11.0799458990001,15.2,-2.73146377200002));
#267800=CARTESIAN_POINT('Ctrl Pts',(-11.0799458990001,11.6,-2.73146377200002));
#267801=CARTESIAN_POINT('Ctrl Pts',(-11.0763114490001,15.2,-2.73218334500001));
#267802=CARTESIAN_POINT('Ctrl Pts',(-11.0763114490001,11.6,-2.73218334500001));
#267803=CARTESIAN_POINT('Ctrl Pts',(-11.0726808780001,15.2,-2.73289925600002));
#267804=CARTESIAN_POINT('Ctrl Pts',(-11.0726808780001,11.6,-2.73289925600002));
#267805=CARTESIAN_POINT('Ctrl Pts',(-11.0690541960001,15.2,-2.73361151100001));
#267806=CARTESIAN_POINT('Ctrl Pts',(-11.0690541960001,11.6,-2.73361151100001));
#267807=CARTESIAN_POINT('Ctrl Pts',(-11.0654314110001,15.2,-2.73432011200001));
#267808=CARTESIAN_POINT('Ctrl Pts',(-11.0654314110001,11.6,-2.73432011200002));
#267809=CARTESIAN_POINT('Ctrl Pts',(-11.0618125300001,15.2,-2.73502506300002));
#267810=CARTESIAN_POINT('Ctrl Pts',(-11.0618125300001,11.6,-2.73502506300002));
#267811=CARTESIAN_POINT('Ctrl Pts',(-11.0581975630001,15.2,-2.73572637000001));
#267812=CARTESIAN_POINT('Ctrl Pts',(-11.0581975630001,11.6,-2.73572637000001));
#267813=CARTESIAN_POINT('Ctrl Pts',(-11.0545865170001,15.2,-2.73642403700002));
#267814=CARTESIAN_POINT('Ctrl Pts',(-11.0545865170001,11.6,-2.73642403700002));
#267815=CARTESIAN_POINT('Ctrl Pts',(-11.0509794010001,15.2,-2.73711806700002));
#267816=CARTESIAN_POINT('Ctrl Pts',(-11.0509794010001,11.6,-2.73711806700002));
#267817=CARTESIAN_POINT('Ctrl Pts',(-11.0473762230001,15.2,-2.73780846600001));
#267818=CARTESIAN_POINT('Ctrl Pts',(-11.0473762230001,11.6,-2.73780846600001));
#267819=CARTESIAN_POINT('Ctrl Pts',(-11.0437769920001,15.2,-2.73849523700001));
#267820=CARTESIAN_POINT('Ctrl Pts',(-11.0437769920001,11.6,-2.73849523700001));
#267821=CARTESIAN_POINT('Ctrl Pts',(-11.0401817150001,15.2,-2.73917838500001));
#267822=CARTESIAN_POINT('Ctrl Pts',(-11.0401817150001,11.6,-2.73917838500001));
#267823=CARTESIAN_POINT('Ctrl Pts',(-11.0365904010001,15.2,-2.73985791400001));
#267824=CARTESIAN_POINT('Ctrl Pts',(-11.0365904010001,11.6,-2.73985791400001));
#267825=CARTESIAN_POINT('Ctrl Pts',(-11.0330030590001,15.2,-2.74053382800002));
#267826=CARTESIAN_POINT('Ctrl Pts',(-11.0330030590001,11.6,-2.74053382800002));
#267827=CARTESIAN_POINT('Ctrl Pts',(-11.0294196970001,15.2,-2.74120613200001));
#267828=CARTESIAN_POINT('Ctrl Pts',(-11.0294196970001,11.6,-2.74120613200001));
#267829=CARTESIAN_POINT('Ctrl Pts',(-11.0258403220001,15.2,-2.74187483000001));
#267830=CARTESIAN_POINT('Ctrl Pts',(-11.0258403220001,11.6,-2.74187483000001));
#267831=CARTESIAN_POINT('Ctrl Pts',(-11.0222649450001,15.2,-2.74253992800002));
#267832=CARTESIAN_POINT('Ctrl Pts',(-11.0222649450001,11.6,-2.74253992800002));
#267833=CARTESIAN_POINT('Ctrl Pts',(-11.0186935710001,15.2,-2.74320142800001));
#267834=CARTESIAN_POINT('Ctrl Pts',(-11.0186935710001,11.6,-2.74320142800002));
#267835=CARTESIAN_POINT('Ctrl Pts',(-11.0151262110001,15.2,-2.74385933600001));
#267836=CARTESIAN_POINT('Ctrl Pts',(-11.0151262110001,11.6,-2.74385933600001));
#267837=CARTESIAN_POINT('Ctrl Pts',(-11.0115628720001,15.2,-2.74451365600001));
#267838=CARTESIAN_POINT('Ctrl Pts',(-11.0115628720001,11.6,-2.74451365600001));
#267839=CARTESIAN_POINT('Ctrl Pts',(-11.0080035640001,15.2,-2.74516439200001));
#267840=CARTESIAN_POINT('Ctrl Pts',(-11.0080035640001,11.6,-2.74516439200002));
#267841=CARTESIAN_POINT('Ctrl Pts',(-11.0044482940001,15.2,-2.74581155000002));
#267842=CARTESIAN_POINT('Ctrl Pts',(-11.0044482940001,11.6,-2.74581155000002));
#267843=CARTESIAN_POINT('Ctrl Pts',(-11.0008970700001,15.2,-2.74645513200001));
#267844=CARTESIAN_POINT('Ctrl Pts',(-11.0008970700001,11.6,-2.74645513200001));
#267845=CARTESIAN_POINT('Ctrl Pts',(-10.9973499030001,15.2,-2.74709514500001));
#267846=CARTESIAN_POINT('Ctrl Pts',(-10.9973499030001,11.6,-2.74709514500001));
#267847=CARTESIAN_POINT('Ctrl Pts',(-10.9938067980001,15.2,-2.74773159100001));
#267848=CARTESIAN_POINT('Ctrl Pts',(-10.9938067980001,11.6,-2.74773159100001));
#267849=CARTESIAN_POINT('Ctrl Pts',(-10.9902677660001,15.2,-2.74836447800002));
#267850=CARTESIAN_POINT('Ctrl Pts',(-10.9902677660001,11.6,-2.74836447800002));
#267851=CARTESIAN_POINT('Ctrl Pts',(-10.9867328140001,15.2,-2.74899380700001));
#267852=CARTESIAN_POINT('Ctrl Pts',(-10.9867328140001,11.6,-2.74899380700001));
#267853=CARTESIAN_POINT('Ctrl Pts',(-10.9832019520001,15.2,-2.74961958600001));
#267854=CARTESIAN_POINT('Ctrl Pts',(-10.9832019520001,11.6,-2.74961958600001));
#267855=CARTESIAN_POINT('Ctrl Pts',(-10.9796751870001,15.2,-2.75024181600001));
#267856=CARTESIAN_POINT('Ctrl Pts',(-10.9796751870001,11.6,-2.75024181600001));
#267857=CARTESIAN_POINT('Ctrl Pts',(-10.9761525290001,15.2,-2.75086050400001));
#267858=CARTESIAN_POINT('Ctrl Pts',(-10.9761525290001,11.6,-2.75086050400001));
#267859=CARTESIAN_POINT('Ctrl Pts',(-10.9726339840001,15.2,-2.75147565300002));
#267860=CARTESIAN_POINT('Ctrl Pts',(-10.9726339840001,11.6,-2.75147565300002));
#267861=CARTESIAN_POINT('Ctrl Pts',(-10.9691195640001,15.2,-2.75208727000001));
#267862=CARTESIAN_POINT('Ctrl Pts',(-10.9691195640001,11.6,-2.75208727000001));
#267863=CARTESIAN_POINT('Ctrl Pts',(-10.9656092750001,15.2,-2.75269535800001));
#267864=CARTESIAN_POINT('Ctrl Pts',(-10.9656092750001,11.6,-2.75269535800002));
#267865=CARTESIAN_POINT('Ctrl Pts',(-10.9621031260001,15.2,-2.75329992100001));
#267866=CARTESIAN_POINT('Ctrl Pts',(-10.9621031260001,11.6,-2.75329992100001));
#267867=CARTESIAN_POINT('Ctrl Pts',(-10.9586011260001,15.2,-2.75390096500002));
#267868=CARTESIAN_POINT('Ctrl Pts',(-10.9586011260001,11.6,-2.75390096500002));
#267869=CARTESIAN_POINT('Ctrl Pts',(-10.9551032830001,15.2,-2.75449849500002));
#267870=CARTESIAN_POINT('Ctrl Pts',(-10.9551032830001,11.6,-2.75449849500002));
#267871=CARTESIAN_POINT('Ctrl Pts',(-10.9516096070001,15.2,-2.75509251400001));
#267872=CARTESIAN_POINT('Ctrl Pts',(-10.9516096070001,11.6,-2.75509251400001));
#267873=CARTESIAN_POINT('Ctrl Pts',(-10.9481201050001,15.2,-2.75568302700002));
#267874=CARTESIAN_POINT('Ctrl Pts',(-10.9481201050001,11.6,-2.75568302700002));
#267875=CARTESIAN_POINT('Ctrl Pts',(-10.9446347860001,15.2,-2.75627004100001));
#267876=CARTESIAN_POINT('Ctrl Pts',(-10.9446347860001,11.6,-2.75627004100001));
#267877=CARTESIAN_POINT('Ctrl Pts',(-10.9411536590001,15.2,-2.75685355800002));
#267878=CARTESIAN_POINT('Ctrl Pts',(-10.9411536590001,11.6,-2.75685355800002));
#267879=CARTESIAN_POINT('Ctrl Pts',(-10.9376767320001,15.2,-2.75743358500002));
#267880=CARTESIAN_POINT('Ctrl Pts',(-10.9376767320001,11.6,-2.75743358500002));
#267881=CARTESIAN_POINT('Ctrl Pts',(-10.9342040160001,15.2,-2.75801012600001));
#267882=CARTESIAN_POINT('Ctrl Pts',(-10.9342040160001,11.6,-2.75801012600001));
#267883=CARTESIAN_POINT('Ctrl Pts',(-10.9307355160001,15.2,-2.75858318400001));
#267884=CARTESIAN_POINT('Ctrl Pts',(-10.9307355160001,11.6,-2.75858318400001));
#267885=CARTESIAN_POINT('Ctrl Pts',(-10.9272712420001,15.2,-2.75915276600001));
#267886=CARTESIAN_POINT('Ctrl Pts',(-10.9272712420001,11.6,-2.75915276600002));
#267887=CARTESIAN_POINT('Ctrl Pts',(-10.9238112040001,15.2,-2.75971887600001));
#267888=CARTESIAN_POINT('Ctrl Pts',(-10.9238112040001,11.6,-2.75971887600001));
#267889=CARTESIAN_POINT('Ctrl Pts',(-10.9203554100001,15.2,-2.76028151900002));
#267890=CARTESIAN_POINT('Ctrl Pts',(-10.9203554100001,11.6,-2.76028151900002));
#267891=CARTESIAN_POINT('Ctrl Pts',(-10.9169038680001,15.2,-2.76084070000001));
#267892=CARTESIAN_POINT('Ctrl Pts',(-10.9169038680001,11.6,-2.76084070000001));
#267893=CARTESIAN_POINT('Ctrl Pts',(-10.9134565880001,15.2,-2.76139642400001));
#267894=CARTESIAN_POINT('Ctrl Pts',(-10.9134565880001,11.6,-2.76139642400001));
#267895=CARTESIAN_POINT('Ctrl Pts',(-10.9100135780001,15.2,-2.76194869600001));
#267896=CARTESIAN_POINT('Ctrl Pts',(-10.9100135780001,11.6,-2.76194869600001));
#267897=CARTESIAN_POINT('Ctrl Pts',(-10.9065748460001,15.2,-2.76249752000002));
#267898=CARTESIAN_POINT('Ctrl Pts',(-10.9065748460001,11.6,-2.76249752000002));
#267899=CARTESIAN_POINT('Ctrl Pts',(-10.9031404020001,15.2,-2.76304290100001));
#267900=CARTESIAN_POINT('Ctrl Pts',(-10.9031404020001,11.6,-2.76304290100002));
#267901=CARTESIAN_POINT('Ctrl Pts',(-10.8997102540001,15.2,-2.76358484600001));
#267902=CARTESIAN_POINT('Ctrl Pts',(-10.8997102540001,11.6,-2.76358484600001));
#267903=CARTESIAN_POINT('Ctrl Pts',(-10.8962844110001,15.2,-2.76412335800002));
#267904=CARTESIAN_POINT('Ctrl Pts',(-10.8962844110001,11.6,-2.76412335800002));
#267905=CARTESIAN_POINT('Ctrl Pts',(-10.8928628820001,15.2,-2.76465844200001));
#267906=CARTESIAN_POINT('Ctrl Pts',(-10.8928628820001,11.6,-2.76465844200001));
#267907=CARTESIAN_POINT('Ctrl Pts',(-10.8894456750001,15.2,-2.76519010300001));
#267908=CARTESIAN_POINT('Ctrl Pts',(-10.8894456750001,11.6,-2.76519010300001));
#267909=CARTESIAN_POINT('Ctrl Pts',(-10.8860328000001,15.2,-2.76571834600002));
#267910=CARTESIAN_POINT('Ctrl Pts',(-10.8860328000001,11.6,-2.76571834600002));
#267911=CARTESIAN_POINT('Ctrl Pts',(-10.8826242650001,15.2,-2.76624317800001));
#267912=CARTESIAN_POINT('Ctrl Pts',(-10.8826242650001,11.6,-2.76624317800001));
#267913=CARTESIAN_POINT('Ctrl Pts',(-10.8792200800001,15.2,-2.76676460200001));
#267914=CARTESIAN_POINT('Ctrl Pts',(-10.8792200800001,11.6,-2.76676460200001));
#267915=CARTESIAN_POINT('Ctrl Pts',(-10.8758202520001,15.2,-2.76728262200002));
#267916=CARTESIAN_POINT('Ctrl Pts',(-10.8758202520001,11.6,-2.76728262200002));
#267917=CARTESIAN_POINT('Ctrl Pts',(-10.8724247920001,15.2,-2.76779724700001));
#267918=CARTESIAN_POINT('Ctrl Pts',(-10.8724247920001,11.6,-2.76779724700001));
#267919=CARTESIAN_POINT('Ctrl Pts',(-10.8690337060001,15.2,-2.76830847900001));
#267920=CARTESIAN_POINT('Ctrl Pts',(-10.8690337060001,11.6,-2.76830847900001));
#267921=CARTESIAN_POINT('Ctrl Pts',(-10.8656470060001,15.2,-2.76881632300002));
#267922=CARTESIAN_POINT('Ctrl Pts',(-10.8656470060001,11.6,-2.76881632300002));
#267923=CARTESIAN_POINT('Ctrl Pts',(-10.8622646980001,15.2,-2.76932078500002));
#267924=CARTESIAN_POINT('Ctrl Pts',(-10.8622646980001,11.6,-2.76932078500002));
#267925=CARTESIAN_POINT('Ctrl Pts',(-10.8588867940001,15.2,-2.76982187100002));
#267926=CARTESIAN_POINT('Ctrl Pts',(-10.8588867940001,11.6,-2.76982187100002));
#267927=CARTESIAN_POINT('Ctrl Pts',(-10.8555133010001,15.2,-2.77031958400002));
#267928=CARTESIAN_POINT('Ctrl Pts',(-10.8555133010001,11.6,-2.77031958400002));
#267929=CARTESIAN_POINT('Ctrl Pts',(-10.8521442280001,15.2,-2.77081393100001));
#267930=CARTESIAN_POINT('Ctrl Pts',(-10.8521442280001,11.6,-2.77081393100001));
#267931=CARTESIAN_POINT('Ctrl Pts',(-10.8487795840001,15.2,-2.77130491700001));
#267932=CARTESIAN_POINT('Ctrl Pts',(-10.8487795840001,11.6,-2.77130491700001));
#267933=CARTESIAN_POINT('Ctrl Pts',(-10.8454193790001,15.2,-2.77179254700001));
#267934=CARTESIAN_POINT('Ctrl Pts',(-10.8454193790001,11.6,-2.77179254700001));
#267935=CARTESIAN_POINT('Ctrl Pts',(-10.8420636210001,15.2,-2.77227682600001));
#267936=CARTESIAN_POINT('Ctrl Pts',(-10.8420636210001,11.6,-2.77227682600001));
#267937=CARTESIAN_POINT('Ctrl Pts',(-10.8387123200001,15.2,-2.77275775900002));
#267938=CARTESIAN_POINT('Ctrl Pts',(-10.8387123200001,11.6,-2.77275775900002));
#267939=CARTESIAN_POINT('Ctrl Pts',(-10.8353654830001,15.2,-2.77323535200001));
#267940=CARTESIAN_POINT('Ctrl Pts',(-10.8353654830001,11.6,-2.77323535200001));
#267941=CARTESIAN_POINT('Ctrl Pts',(-10.8320231210001,15.2,-2.77370961000001));
#267942=CARTESIAN_POINT('Ctrl Pts',(-10.8320231210001,11.6,-2.77370961000001));
#267943=CARTESIAN_POINT('Ctrl Pts',(-10.8286852410001,15.2,-2.77418053700002));
#267944=CARTESIAN_POINT('Ctrl Pts',(-10.8286852410001,11.6,-2.77418053700002));
#267945=CARTESIAN_POINT('Ctrl Pts',(-10.8253518550001,15.2,-2.77464814100002));
#267946=CARTESIAN_POINT('Ctrl Pts',(-10.8253518550001,11.6,-2.77464814100002));
#267947=CARTESIAN_POINT('Ctrl Pts',(-10.8220229700001,15.2,-2.77511242500001));
#267948=CARTESIAN_POINT('Ctrl Pts',(-10.8220229700001,11.6,-2.77511242500002));
#267949=CARTESIAN_POINT('Ctrl Pts',(-10.8186985940001,15.2,-2.77557339600001));
#267950=CARTESIAN_POINT('Ctrl Pts',(-10.8186985940001,11.6,-2.77557339600001));
#267951=CARTESIAN_POINT('Ctrl Pts',(-10.8153787400001,15.2,-2.77603105800001));
#267952=CARTESIAN_POINT('Ctrl Pts',(-10.8153787400001,11.6,-2.77603105800001));
#267953=CARTESIAN_POINT('Ctrl Pts',(-10.8120634130001,15.2,-2.77648541700001));
#267954=CARTESIAN_POINT('Ctrl Pts',(-10.8120634130001,11.6,-2.77648541700001));
#267955=CARTESIAN_POINT('Ctrl Pts',(-10.8087526240001,15.2,-2.77693647800001));
#267956=CARTESIAN_POINT('Ctrl Pts',(-10.8087526240001,11.6,-2.77693647800001));
#267957=CARTESIAN_POINT('Ctrl Pts',(-10.8054463820001,15.2,-2.77738424700001));
#267958=CARTESIAN_POINT('Ctrl Pts',(-10.8054463820001,11.6,-2.77738424700001));
#267959=CARTESIAN_POINT('Ctrl Pts',(-10.8021446960001,15.2,-2.77782872900001));
#267960=CARTESIAN_POINT('Ctrl Pts',(-10.8021446960001,11.6,-2.77782872900001));
#267961=CARTESIAN_POINT('Ctrl Pts',(-10.7988475760001,15.2,-2.77826993000001));
#267962=CARTESIAN_POINT('Ctrl Pts',(-10.7988475760001,11.6,-2.77826993000002));
#267963=CARTESIAN_POINT('Ctrl Pts',(-10.7955550300001,15.2,-2.77870785600001));
#267964=CARTESIAN_POINT('Ctrl Pts',(-10.7955550300001,11.6,-2.77870785600001));
#267965=CARTESIAN_POINT('Ctrl Pts',(-10.7922670680001,15.2,-2.77914251000002));
#267966=CARTESIAN_POINT('Ctrl Pts',(-10.7922670680001,11.6,-2.77914251000002));
#267967=CARTESIAN_POINT('Ctrl Pts',(-10.7889836990001,15.2,-2.77957390000001));
#267968=CARTESIAN_POINT('Ctrl Pts',(-10.7889836990001,11.6,-2.77957390000001));
#267969=CARTESIAN_POINT('Ctrl Pts',(-10.7857049310001,15.2,-2.78000203100001));
#267970=CARTESIAN_POINT('Ctrl Pts',(-10.7857049310001,11.6,-2.78000203100001));
#267971=CARTESIAN_POINT('Ctrl Pts',(-10.7824307750001,15.2,-2.78042690900001));
#267972=CARTESIAN_POINT('Ctrl Pts',(-10.7824307750001,11.6,-2.78042690900001));
#267973=CARTESIAN_POINT('Ctrl Pts',(-10.7791612390001,15.2,-2.78084853700001));
#267974=CARTESIAN_POINT('Ctrl Pts',(-10.7791612390001,11.6,-2.78084853700001));
#267975=CARTESIAN_POINT('Ctrl Pts',(-10.7758963330001,15.2,-2.78126692300001));
#267976=CARTESIAN_POINT('Ctrl Pts',(-10.7758963330001,11.6,-2.78126692300001));
#267977=CARTESIAN_POINT('Ctrl Pts',(-10.7726360660001,15.2,-2.78168207300002));
#267978=CARTESIAN_POINT('Ctrl Pts',(-10.7726360660001,11.6,-2.78168207300002));
#267979=CARTESIAN_POINT('Ctrl Pts',(-10.7693804470001,15.2,-2.78209399100001));
#267980=CARTESIAN_POINT('Ctrl Pts',(-10.7693804470001,11.6,-2.78209399100001));
#267981=CARTESIAN_POINT('Ctrl Pts',(-10.7661294860001,15.2,-2.78250268300001));
#267982=CARTESIAN_POINT('Ctrl Pts',(-10.7661294860001,11.6,-2.78250268300001));
#267983=CARTESIAN_POINT('Ctrl Pts',(-10.7628831920001,15.2,-2.78290815600001));
#267984=CARTESIAN_POINT('Ctrl Pts',(-10.7628831920001,11.6,-2.78290815600002));
#267985=CARTESIAN_POINT('Ctrl Pts',(-10.7596415740001,15.2,-2.78331041300001));
#267986=CARTESIAN_POINT('Ctrl Pts',(-10.7596415740001,11.6,-2.78331041300001));
#267987=CARTESIAN_POINT('Ctrl Pts',(-10.7564046420001,15.2,-2.78370946300001));
#267988=CARTESIAN_POINT('Ctrl Pts',(-10.7564046420001,11.6,-2.78370946300001));
#267989=CARTESIAN_POINT('Ctrl Pts',(-10.7531724040001,15.2,-2.78410530900001));
#267990=CARTESIAN_POINT('Ctrl Pts',(-10.7531724040001,11.6,-2.78410530900001));
#267991=CARTESIAN_POINT('Ctrl Pts',(-10.7499448710001,15.2,-2.78449795800002));
#267992=CARTESIAN_POINT('Ctrl Pts',(-10.7499448710001,11.6,-2.78449795800002));
#267993=CARTESIAN_POINT('Ctrl Pts',(-10.7467220520001,15.2,-2.78488741600002));
#267994=CARTESIAN_POINT('Ctrl Pts',(-10.7467220520001,11.6,-2.78488741600002));
#267995=CARTESIAN_POINT('Ctrl Pts',(-10.7435039560001,15.2,-2.78527368900002));
#267996=CARTESIAN_POINT('Ctrl Pts',(-10.7435039560001,11.6,-2.78527368900002));
#267997=CARTESIAN_POINT('Ctrl Pts',(-10.7402905920001,15.2,-2.78565678100001));
#267998=CARTESIAN_POINT('Ctrl Pts',(-10.7402905920001,11.6,-2.78565678100001));
#267999=CARTESIAN_POINT('Ctrl Pts',(-10.7370819700001,15.2,-2.78603669900002));
#268000=CARTESIAN_POINT('Ctrl Pts',(-10.7370819700001,11.6,-2.78603669900002));
#268001=CARTESIAN_POINT('Ctrl Pts',(-10.7338780990001,15.2,-2.78641345000001));
#268002=CARTESIAN_POINT('Ctrl Pts',(-10.7338780990001,11.6,-2.78641345000001));
#268003=CARTESIAN_POINT('Ctrl Pts',(-10.7306789900001,15.2,-2.78678703700002));
#268004=CARTESIAN_POINT('Ctrl Pts',(-10.7306789900001,11.6,-2.78678703700002));
#268005=CARTESIAN_POINT('Ctrl Pts',(-10.7274846510001,15.2,-2.78715746900001));
#268006=CARTESIAN_POINT('Ctrl Pts',(-10.7274846510001,11.6,-2.78715746900001));
#268007=CARTESIAN_POINT('Ctrl Pts',(-10.7242950910001,15.2,-2.78752475000001));
#268008=CARTESIAN_POINT('Ctrl Pts',(-10.7242950910001,11.6,-2.78752475000001));
#268009=CARTESIAN_POINT('Ctrl Pts',(-10.7211103210001,15.2,-2.78788888700001));
#268010=CARTESIAN_POINT('Ctrl Pts',(-10.7211103210001,11.6,-2.78788888700001));
#268011=CARTESIAN_POINT('Ctrl Pts',(-10.7179303500001,15.2,-2.78824988400002));
#268012=CARTESIAN_POINT('Ctrl Pts',(-10.7179303500001,11.6,-2.78824988400002));
#268013=CARTESIAN_POINT('Ctrl Pts',(-10.7147551880001,15.2,-2.78860774800001));
#268014=CARTESIAN_POINT('Ctrl Pts',(-10.7147551880001,11.6,-2.78860774800001));
#268015=CARTESIAN_POINT('Ctrl Pts',(-10.7115848430001,15.2,-2.78896248700002));
#268016=CARTESIAN_POINT('Ctrl Pts',(-10.7115848430001,11.6,-2.78896248700002));
#268017=CARTESIAN_POINT('Ctrl Pts',(-10.7084193250001,15.2,-2.78931410400002));
#268018=CARTESIAN_POINT('Ctrl Pts',(-10.7084193250001,11.6,-2.78931410400002));
#268019=CARTESIAN_POINT('Ctrl Pts',(-10.7052586450001,15.2,-2.78966260600002));
#268020=CARTESIAN_POINT('Ctrl Pts',(-10.7052586450001,11.6,-2.78966260600002));
#268021=CARTESIAN_POINT('Ctrl Pts',(-10.7021028110001,15.2,-2.79000800100001));
#268022=CARTESIAN_POINT('Ctrl Pts',(-10.7021028110001,11.6,-2.79000800100001));
#268023=CARTESIAN_POINT('Ctrl Pts',(-10.6989518340001,15.2,-2.79035029100001));
#268024=CARTESIAN_POINT('Ctrl Pts',(-10.6989518340001,11.6,-2.79035029100001));
#268025=CARTESIAN_POINT('Ctrl Pts',(-10.6958057220001,15.2,-2.79068948600001));
#268026=CARTESIAN_POINT('Ctrl Pts',(-10.6958057220001,11.6,-2.79068948600001));
#268027=CARTESIAN_POINT('Ctrl Pts',(-10.6926644870001,15.2,-2.79102559000002));
#268028=CARTESIAN_POINT('Ctrl Pts',(-10.6926644870001,11.6,-2.79102559000002));
#268029=CARTESIAN_POINT('Ctrl Pts',(-10.6895281350001,15.2,-2.79135861000002));
#268030=CARTESIAN_POINT('Ctrl Pts',(-10.6895281350001,11.6,-2.79135861000002));
#268031=CARTESIAN_POINT('Ctrl Pts',(-10.6863966800001,15.2,-2.79168855100002));
#268032=CARTESIAN_POINT('Ctrl Pts',(-10.6863966800001,11.6,-2.79168855100002));
#268033=CARTESIAN_POINT('Ctrl Pts',(-10.6832701290001,15.2,-2.79201542000001));
#268034=CARTESIAN_POINT('Ctrl Pts',(-10.6832701290001,11.6,-2.79201542000001));
#268035=CARTESIAN_POINT('Ctrl Pts',(-10.6801484920001,15.2,-2.79233922300001));
#268036=CARTESIAN_POINT('Ctrl Pts',(-10.6801484920001,11.6,-2.79233922300001));
#268037=CARTESIAN_POINT('Ctrl Pts',(-10.6770317790001,15.2,-2.79265996700001));
#268038=CARTESIAN_POINT('Ctrl Pts',(-10.6770317790001,11.6,-2.79265996700001));
#268039=CARTESIAN_POINT('Ctrl Pts',(-10.6739200000001,15.2,-2.79297765700001));
#268040=CARTESIAN_POINT('Ctrl Pts',(-10.6739200000001,11.6,-2.79297765700001));
#268041=CARTESIAN_POINT('Ctrl Pts',(-10.6708131640001,15.2,-2.79329230000001));
#268042=CARTESIAN_POINT('Ctrl Pts',(-10.6708131640001,11.6,-2.79329230000001));
#268043=CARTESIAN_POINT('Ctrl Pts',(-10.6677112820001,15.2,-2.79360390200001));
#268044=CARTESIAN_POINT('Ctrl Pts',(-10.6677112820001,11.6,-2.79360390200001));
#268045=CARTESIAN_POINT('Ctrl Pts',(-10.6646143620001,15.2,-2.79391246900001));
#268046=CARTESIAN_POINT('Ctrl Pts',(-10.6646143620001,11.6,-2.79391246900001));
#268047=CARTESIAN_POINT('Ctrl Pts',(-10.6615224160001,15.2,-2.79421800700002));
#268048=CARTESIAN_POINT('Ctrl Pts',(-10.6615224160001,11.6,-2.79421800700002));
#268049=CARTESIAN_POINT('Ctrl Pts',(-10.6584354520001,15.2,-2.79452052500002));
#268050=CARTESIAN_POINT('Ctrl Pts',(-10.6584354520001,11.6,-2.79452052500002));
#268051=CARTESIAN_POINT('Ctrl Pts',(-10.6553534800001,15.2,-2.79482002500002));
#268052=CARTESIAN_POINT('Ctrl Pts',(-10.6553534800001,11.6,-2.79482002500002));
#268053=CARTESIAN_POINT('Ctrl Pts',(-10.6522765120001,15.2,-2.79511651600002));
#268054=CARTESIAN_POINT('Ctrl Pts',(-10.6522765120001,11.6,-2.79511651600002));
#268055=CARTESIAN_POINT('Ctrl Pts',(-10.6492045550001,15.2,-2.79541000500001));
#268056=CARTESIAN_POINT('Ctrl Pts',(-10.6492045550001,11.6,-2.79541000500001));
#268057=CARTESIAN_POINT('Ctrl Pts',(-10.6461376210001,15.2,-2.79570049800002));
#268058=CARTESIAN_POINT('Ctrl Pts',(-10.6461376210001,11.6,-2.79570049800002));
#268059=CARTESIAN_POINT('Ctrl Pts',(-10.6430757180001,15.2,-2.79598800000001));
#268060=CARTESIAN_POINT('Ctrl Pts',(-10.6430757180001,11.6,-2.79598800000001));
#268061=CARTESIAN_POINT('Ctrl Pts',(-10.6400188580001,15.2,-2.79627251700001));
#268062=CARTESIAN_POINT('Ctrl Pts',(-10.6400188580001,11.6,-2.79627251700001));
#268063=CARTESIAN_POINT('Ctrl Pts',(-10.6369670490001,15.2,-2.79655405800002));
#268064=CARTESIAN_POINT('Ctrl Pts',(-10.6369670490001,11.6,-2.79655405800002));
#268065=CARTESIAN_POINT('Ctrl Pts',(-10.6339203020001,15.2,-2.79683262800001));
#268066=CARTESIAN_POINT('Ctrl Pts',(-10.6339203020001,11.6,-2.79683262800001));
#268067=CARTESIAN_POINT('Ctrl Pts',(-10.6308786260001,15.2,-2.79710823500002));
#268068=CARTESIAN_POINT('Ctrl Pts',(-10.6308786260001,11.6,-2.79710823500002));
#268069=CARTESIAN_POINT('Ctrl Pts',(-10.6278420330001,15.2,-2.79738088400002));
#268070=CARTESIAN_POINT('Ctrl Pts',(-10.6278420330001,11.6,-2.79738088400002));
#268071=CARTESIAN_POINT('Ctrl Pts',(-10.6248105320001,15.2,-2.79765058100002));
#268072=CARTESIAN_POINT('Ctrl Pts',(-10.6248105320001,11.6,-2.79765058100002));
#268073=CARTESIAN_POINT('Ctrl Pts',(-10.6217841320001,15.2,-2.79791733300002));
#268074=CARTESIAN_POINT('Ctrl Pts',(-10.6217841320001,11.6,-2.79791733300002));
#268075=CARTESIAN_POINT('Ctrl Pts',(-10.6187628440001,15.2,-2.79818114900001));
#268076=CARTESIAN_POINT('Ctrl Pts',(-10.6187628440001,11.6,-2.79818114900001));
#268077=CARTESIAN_POINT('Ctrl Pts',(-10.6157466780001,15.2,-2.79844203300001));
#268078=CARTESIAN_POINT('Ctrl Pts',(-10.6157466780001,11.6,-2.79844203300002));
#268079=CARTESIAN_POINT('Ctrl Pts',(-10.6127356450001,15.2,-2.79869999200002));
#268080=CARTESIAN_POINT('Ctrl Pts',(-10.6127356450001,11.6,-2.79869999200002));
#268081=CARTESIAN_POINT('Ctrl Pts',(-10.6097297520001,15.2,-2.79895503300001));
#268082=CARTESIAN_POINT('Ctrl Pts',(-10.6097297520001,11.6,-2.79895503300002));
#268083=CARTESIAN_POINT('Ctrl Pts',(-10.6067290130001,15.2,-2.79920716400001));
#268084=CARTESIAN_POINT('Ctrl Pts',(-10.6067290130001,11.6,-2.79920716400001));
#268085=CARTESIAN_POINT('Ctrl Pts',(-10.6037334350001,15.2,-2.79945638900001));
#268086=CARTESIAN_POINT('Ctrl Pts',(-10.6037334350001,11.6,-2.79945638900002));
#268087=CARTESIAN_POINT('Ctrl Pts',(-10.6007430310001,15.2,-2.79970271700002));
#268088=CARTESIAN_POINT('Ctrl Pts',(-10.6007430310001,11.6,-2.79970271700002));
#268089=CARTESIAN_POINT('Ctrl Pts',(-10.5977578070001,15.2,-2.79994615300001));
#268090=CARTESIAN_POINT('Ctrl Pts',(-10.5977578070001,11.6,-2.79994615300002));
#268091=CARTESIAN_POINT('Ctrl Pts',(-10.5947777780001,15.2,-2.80018670600001));
#268092=CARTESIAN_POINT('Ctrl Pts',(-10.5947777780001,11.6,-2.80018670600001));
#268093=CARTESIAN_POINT('Ctrl Pts',(-10.5918029510001,15.2,-2.80042438200002));
#268094=CARTESIAN_POINT('Ctrl Pts',(-10.5918029510001,11.6,-2.80042438200002));
#268095=CARTESIAN_POINT('Ctrl Pts',(-10.5888333380001,15.2,-2.80065918700001));
#268096=CARTESIAN_POINT('Ctrl Pts',(-10.5888333380001,11.6,-2.80065918700001));
#268097=CARTESIAN_POINT('Ctrl Pts',(-10.5858689480001,15.2,-2.80089112800002));
#268098=CARTESIAN_POINT('Ctrl Pts',(-10.5858689480001,11.6,-2.80089112800002));
#268099=CARTESIAN_POINT('Ctrl Pts',(-10.5829097920001,15.2,-2.80112021200001));
#268100=CARTESIAN_POINT('Ctrl Pts',(-10.5829097920001,11.6,-2.80112021200001));
#268101=CARTESIAN_POINT('Ctrl Pts',(-10.5799558780001,15.2,-2.80134644700002));
#268102=CARTESIAN_POINT('Ctrl Pts',(-10.5799558780001,11.6,-2.80134644700002));
#268103=CARTESIAN_POINT('Ctrl Pts',(-10.5770072200001,15.2,-2.80156983800001));
#268104=CARTESIAN_POINT('Ctrl Pts',(-10.5770072200001,11.6,-2.80156983800001));
#268105=CARTESIAN_POINT('Ctrl Pts',(-10.5740638260001,15.2,-2.80179039400001));
#268106=CARTESIAN_POINT('Ctrl Pts',(-10.5740638260001,11.6,-2.80179039400001));
#268107=CARTESIAN_POINT('Ctrl Pts',(-10.5711257080001,15.2,-2.80200812100002));
#268108=CARTESIAN_POINT('Ctrl Pts',(-10.5711257080001,11.6,-2.80200812100002));
#268109=CARTESIAN_POINT('Ctrl Pts',(-10.5681928730001,15.2,-2.80222302500002));
#268110=CARTESIAN_POINT('Ctrl Pts',(-10.5681928730001,11.6,-2.80222302500002));
#268111=CARTESIAN_POINT('Ctrl Pts',(-10.5652653350001,15.2,-2.80243511500001));
#268112=CARTESIAN_POINT('Ctrl Pts',(-10.5652653350001,11.6,-2.80243511500002));
#268113=CARTESIAN_POINT('Ctrl Pts',(-10.5623431030001,15.2,-2.80264439700002));
#268114=CARTESIAN_POINT('Ctrl Pts',(-10.5623431030001,11.6,-2.80264439700002));
#268115=CARTESIAN_POINT('Ctrl Pts',(-10.5594261870001,15.2,-2.80285087700001));
#268116=CARTESIAN_POINT('Ctrl Pts',(-10.5594261870001,11.6,-2.80285087700001));
#268117=CARTESIAN_POINT('Ctrl Pts',(-10.5565145980001,15.2,-2.80305456500002));
#268118=CARTESIAN_POINT('Ctrl Pts',(-10.5565145980001,11.6,-2.80305456500002));
#268119=CARTESIAN_POINT('Ctrl Pts',(-10.5536083460001,15.2,-2.80325546500002));
#268120=CARTESIAN_POINT('Ctrl Pts',(-10.5536083460001,11.6,-2.80325546500002));
#268121=CARTESIAN_POINT('Ctrl Pts',(-10.5507074410001,15.2,-2.80345358600002));
#268122=CARTESIAN_POINT('Ctrl Pts',(-10.5507074410001,11.6,-2.80345358600002));
#268123=CARTESIAN_POINT('Ctrl Pts',(-10.5478118940001,15.2,-2.80364893500002));
#268124=CARTESIAN_POINT('Ctrl Pts',(-10.5478118940001,11.6,-2.80364893500002));
#268125=CARTESIAN_POINT('Ctrl Pts',(-10.5449217170001,15.2,-2.80384151900002));
#268126=CARTESIAN_POINT('Ctrl Pts',(-10.5449217170001,11.6,-2.80384151900002));
#268127=CARTESIAN_POINT('Ctrl Pts',(-10.5420369180001,15.2,-2.80403134500002));
#268128=CARTESIAN_POINT('Ctrl Pts',(-10.5420369180001,11.6,-2.80403134500002));
#268129=CARTESIAN_POINT('Ctrl Pts',(-10.5391575100001,15.2,-2.80421842000001));
#268130=CARTESIAN_POINT('Ctrl Pts',(-10.5391575100001,11.6,-2.80421842000001));
#268131=CARTESIAN_POINT('Ctrl Pts',(-10.5362835010001,15.2,-2.80440275200001));
#268132=CARTESIAN_POINT('Ctrl Pts',(-10.5362835010001,11.6,-2.80440275200002));
#268133=CARTESIAN_POINT('Ctrl Pts',(-10.5334149020001,15.2,-2.80458434800002));
#268134=CARTESIAN_POINT('Ctrl Pts',(-10.5334149020001,11.6,-2.80458434800002));
#268135=CARTESIAN_POINT('Ctrl Pts',(-10.5305517260001,15.2,-2.80476321500001));
#268136=CARTESIAN_POINT('Ctrl Pts',(-10.5305517260001,11.6,-2.80476321500002));
#268137=CARTESIAN_POINT('Ctrl Pts',(-10.5276939810001,15.2,-2.80493936100001));
#268138=CARTESIAN_POINT('Ctrl Pts',(-10.5276939810001,11.6,-2.80493936100001));
#268139=CARTESIAN_POINT('Ctrl Pts',(-10.5248416780001,15.2,-2.80511279300002));
#268140=CARTESIAN_POINT('Ctrl Pts',(-10.5248416780001,11.6,-2.80511279300002));
#268141=CARTESIAN_POINT('Ctrl Pts',(-10.5219948290001,15.2,-2.80528351800001));
#268142=CARTESIAN_POINT('Ctrl Pts',(-10.5219948290001,11.6,-2.80528351800002));
#268143=CARTESIAN_POINT('Ctrl Pts',(-10.5191534450001,15.2,-2.80545154400002));
#268144=CARTESIAN_POINT('Ctrl Pts',(-10.5191534450001,11.6,-2.80545154400002));
#268145=CARTESIAN_POINT('Ctrl Pts',(-10.5163175340001,15.2,-2.80561687900001));
#268146=CARTESIAN_POINT('Ctrl Pts',(-10.5163175340001,11.6,-2.80561687900002));
#268147=CARTESIAN_POINT('Ctrl Pts',(-10.5134871080001,15.2,-2.80577952900002));
#268148=CARTESIAN_POINT('Ctrl Pts',(-10.5134871080001,11.6,-2.80577952900002));
#268149=CARTESIAN_POINT('Ctrl Pts',(-10.5106621790001,15.2,-2.80593950300001));
#268150=CARTESIAN_POINT('Ctrl Pts',(-10.5106621790001,11.6,-2.80593950300001));
#268151=CARTESIAN_POINT('Ctrl Pts',(-10.5078427570001,15.2,-2.80609680700001));
#268152=CARTESIAN_POINT('Ctrl Pts',(-10.5078427570001,11.6,-2.80609680700001));
#268153=CARTESIAN_POINT('Ctrl Pts',(-10.5050288510001,15.2,-2.80625145000001));
#268154=CARTESIAN_POINT('Ctrl Pts',(-10.5050288510001,11.6,-2.80625145000002));
#268155=CARTESIAN_POINT('Ctrl Pts',(-10.5022204750001,15.2,-2.80640343900001));
#268156=CARTESIAN_POINT('Ctrl Pts',(-10.5022204750001,11.6,-2.80640343900001));
#268157=CARTESIAN_POINT('Ctrl Pts',(-10.4994176380001,15.2,-2.80655278100001));
#268158=CARTESIAN_POINT('Ctrl Pts',(-10.4994176380001,11.6,-2.80655278100001));
#268159=CARTESIAN_POINT('Ctrl Pts',(-10.4966203510001,15.2,-2.80669948500002));
#268160=CARTESIAN_POINT('Ctrl Pts',(-10.4966203510001,11.6,-2.80669948500002));
#268161=CARTESIAN_POINT('Ctrl Pts',(-10.4938286240001,15.2,-2.80684355700001));
#268162=CARTESIAN_POINT('Ctrl Pts',(-10.4938286240001,11.6,-2.80684355700001));
#268163=CARTESIAN_POINT('Ctrl Pts',(-10.4910424700001,15.2,-2.80698500600002));
#268164=CARTESIAN_POINT('Ctrl Pts',(-10.4910424700001,11.6,-2.80698500600002));
#268165=CARTESIAN_POINT('Ctrl Pts',(-10.4882618970001,15.2,-2.80712384000001));
#268166=CARTESIAN_POINT('Ctrl Pts',(-10.4882618970001,11.6,-2.80712384000001));
#268167=CARTESIAN_POINT('Ctrl Pts',(-10.4854869180001,15.2,-2.80726006400001));
#268168=CARTESIAN_POINT('Ctrl Pts',(-10.4854869180001,11.6,-2.80726006400001));
#268169=CARTESIAN_POINT('Ctrl Pts',(-10.4827175440001,15.2,-2.80739369000001));
#268170=CARTESIAN_POINT('Ctrl Pts',(-10.4827175440001,11.6,-2.80739369000001));
#268171=CARTESIAN_POINT('Ctrl Pts',(-10.4799537850001,15.2,-2.80752472200001));
#268172=CARTESIAN_POINT('Ctrl Pts',(-10.4799537850001,11.6,-2.80752472200001));
#268173=CARTESIAN_POINT('Ctrl Pts',(-10.4771956530001,15.2,-2.80765317100002));
#268174=CARTESIAN_POINT('Ctrl Pts',(-10.4771956530001,11.6,-2.80765317100002));
#268175=CARTESIAN_POINT('Ctrl Pts',(-10.4744431570001,15.2,-2.80777904200002));
#268176=CARTESIAN_POINT('Ctrl Pts',(-10.4744431570001,11.6,-2.80777904200002));
#268177=CARTESIAN_POINT('Ctrl Pts',(-10.4716963110001,15.2,-2.80790234500001));
#268178=CARTESIAN_POINT('Ctrl Pts',(-10.4716963110001,11.6,-2.80790234500001));
#268179=CARTESIAN_POINT('Ctrl Pts',(-10.4689551240001,15.2,-2.80802308700002));
#268180=CARTESIAN_POINT('Ctrl Pts',(-10.4689551240001,11.6,-2.80802308700002));
#268181=CARTESIAN_POINT('Ctrl Pts',(-10.4662196070001,15.2,-2.80814127600001));
#268182=CARTESIAN_POINT('Ctrl Pts',(-10.4662196070001,11.6,-2.80814127600001));
#268183=CARTESIAN_POINT('Ctrl Pts',(-10.4634897720001,15.2,-2.80825691900001));
#268184=CARTESIAN_POINT('Ctrl Pts',(-10.4634897720001,11.6,-2.80825691900001));
#268185=CARTESIAN_POINT('Ctrl Pts',(-10.4607656300001,15.2,-2.80837002600002));
#268186=CARTESIAN_POINT('Ctrl Pts',(-10.4607656300001,11.6,-2.80837002600002));
#268187=CARTESIAN_POINT('Ctrl Pts',(-10.4580471910001,15.2,-2.80848060400002));
#268188=CARTESIAN_POINT('Ctrl Pts',(-10.4580471910001,11.6,-2.80848060400002));
#268189=CARTESIAN_POINT('Ctrl Pts',(-10.4553344680001,15.2,-2.80858866000001));
#268190=CARTESIAN_POINT('Ctrl Pts',(-10.4553344680001,11.6,-2.80858866000001));
#268191=CARTESIAN_POINT('Ctrl Pts',(-10.4526274700001,15.2,-2.80869420500002));
#268192=CARTESIAN_POINT('Ctrl Pts',(-10.4526274700001,11.6,-2.80869420500002));
#268193=CARTESIAN_POINT('Ctrl Pts',(-10.4499262110001,15.2,-2.80879724300001));
#268194=CARTESIAN_POINT('Ctrl Pts',(-10.4499262110001,11.6,-2.80879724300001));
#268195=CARTESIAN_POINT('Ctrl Pts',(-10.4472306990001,15.2,-2.80889778700002));
#268196=CARTESIAN_POINT('Ctrl Pts',(-10.4472306990001,11.6,-2.80889778700002));
#268197=CARTESIAN_POINT('Ctrl Pts',(-10.4445409480001,15.2,-2.80899584100001));
#268198=CARTESIAN_POINT('Ctrl Pts',(-10.4445409480001,11.6,-2.80899584100002));
#268199=CARTESIAN_POINT('Ctrl Pts',(-10.4418569680001,15.2,-2.80909141400001));
#268200=CARTESIAN_POINT('Ctrl Pts',(-10.4418569680001,11.6,-2.80909141400001));
#268201=CARTESIAN_POINT('Ctrl Pts',(-10.4391787700001,15.2,-2.80918451700002));
#268202=CARTESIAN_POINT('Ctrl Pts',(-10.4391787700001,11.6,-2.80918451700002));
#268203=CARTESIAN_POINT('Ctrl Pts',(-10.4365063660001,15.2,-2.80927515500002));
#268204=CARTESIAN_POINT('Ctrl Pts',(-10.4365063660001,11.6,-2.80927515500002));
#268205=CARTESIAN_POINT('Ctrl Pts',(-10.4338397670001,15.2,-2.80936333700001));
#268206=CARTESIAN_POINT('Ctrl Pts',(-10.4338397670001,11.6,-2.80936333700002));
#268207=CARTESIAN_POINT('Ctrl Pts',(-10.4311789840001,15.2,-2.80944907300002));
#268208=CARTESIAN_POINT('Ctrl Pts',(-10.4311789840001,11.6,-2.80944907300002));
#268209=CARTESIAN_POINT('Ctrl Pts',(-10.4285240300001,15.2,-2.80953237000002));
#268210=CARTESIAN_POINT('Ctrl Pts',(-10.4285240300001,11.6,-2.80953237000002));
#268211=CARTESIAN_POINT('Ctrl Pts',(-10.4258749130001,15.2,-2.80961323700001));
#268212=CARTESIAN_POINT('Ctrl Pts',(-10.4258749130001,11.6,-2.80961323700002));
#268213=CARTESIAN_POINT('Ctrl Pts',(-10.4232316480001,15.2,-2.80969168100001));
#268214=CARTESIAN_POINT('Ctrl Pts',(-10.4232316480001,11.6,-2.80969168100001));
#268215=CARTESIAN_POINT('Ctrl Pts',(-10.4205942460001,15.2,-2.80976771100002));
#268216=CARTESIAN_POINT('Ctrl Pts',(-10.4205942460001,11.6,-2.80976771100002));
#268217=CARTESIAN_POINT('Ctrl Pts',(-10.4179627160001,15.2,-2.80984133700001));
#268218=CARTESIAN_POINT('Ctrl Pts',(-10.4179627160001,11.6,-2.80984133700001));
#268219=CARTESIAN_POINT('Ctrl Pts',(-10.4153370720001,15.2,-2.80991256500001));
#268220=CARTESIAN_POINT('Ctrl Pts',(-10.4153370720001,11.6,-2.80991256500001));
#268221=CARTESIAN_POINT('Ctrl Pts',(-10.4127173250001,15.2,-2.80998140700001));
#268222=CARTESIAN_POINT('Ctrl Pts',(-10.4127173250001,11.6,-2.80998140700001));
#268223=CARTESIAN_POINT('Ctrl Pts',(-10.4101034850001,15.2,-2.81004786800001));
#268224=CARTESIAN_POINT('Ctrl Pts',(-10.4101034850001,11.6,-2.81004786800001));
#268225=CARTESIAN_POINT('Ctrl Pts',(-10.4074955650001,15.2,-2.81011195800001));
#268226=CARTESIAN_POINT('Ctrl Pts',(-10.4074955650001,11.6,-2.81011195800001));
#268227=CARTESIAN_POINT('Ctrl Pts',(-10.4048935770001,15.2,-2.81017368600001));
#268228=CARTESIAN_POINT('Ctrl Pts',(-10.4048935770001,11.6,-2.81017368600002));
#268229=CARTESIAN_POINT('Ctrl Pts',(-10.4022975320001,15.2,-2.81023306000002));
#268230=CARTESIAN_POINT('Ctrl Pts',(-10.4022975320001,11.6,-2.81023306000002));
#268231=CARTESIAN_POINT('Ctrl Pts',(-10.3997074400001,15.2,-2.81029008900001));
#268232=CARTESIAN_POINT('Ctrl Pts',(-10.3997074400001,11.6,-2.81029008900001));
#268233=CARTESIAN_POINT('Ctrl Pts',(-10.3971233170001,15.2,-2.81034478200001));
#268234=CARTESIAN_POINT('Ctrl Pts',(-10.3971233170001,11.6,-2.81034478200001));
#268235=CARTESIAN_POINT('Ctrl Pts',(-10.3945451690001,15.2,-2.81039714800002));
#268236=CARTESIAN_POINT('Ctrl Pts',(-10.3945451690001,11.6,-2.81039714800002));
#268237=CARTESIAN_POINT('Ctrl Pts',(-10.3919730120001,15.2,-2.81044719300001));
#268238=CARTESIAN_POINT('Ctrl Pts',(-10.3919730120001,11.6,-2.81044719300001));
#268239=CARTESIAN_POINT('Ctrl Pts',(-10.3894068560001,15.2,-2.81049493000001));
#268240=CARTESIAN_POINT('Ctrl Pts',(-10.3894068560001,11.6,-2.81049493000001));
#268241=CARTESIAN_POINT('Ctrl Pts',(-10.3868467140001,15.2,-2.81054036500001));
#268242=CARTESIAN_POINT('Ctrl Pts',(-10.3868467140001,11.6,-2.81054036500001));
#268243=CARTESIAN_POINT('Ctrl Pts',(-10.3842925970001,15.2,-2.81058350800001));
#268244=CARTESIAN_POINT('Ctrl Pts',(-10.3842925970001,11.6,-2.81058350800001));
#268245=CARTESIAN_POINT('Ctrl Pts',(-10.3817445160001,15.2,-2.81062436900001));
#268246=CARTESIAN_POINT('Ctrl Pts',(-10.3817445160001,11.6,-2.81062436900001));
#268247=CARTESIAN_POINT('Ctrl Pts',(-10.3792024840001,15.2,-2.81066295300001));
#268248=CARTESIAN_POINT('Ctrl Pts',(-10.3792024840001,11.6,-2.81066295300001));
#268249=CARTESIAN_POINT('Ctrl Pts',(-10.3766665130001,15.2,-2.81069927400001));
#268250=CARTESIAN_POINT('Ctrl Pts',(-10.3766665130001,11.6,-2.81069927400001));
#268251=CARTESIAN_POINT('Ctrl Pts',(-10.3741366140001,15.2,-2.81073333600002));
#268252=CARTESIAN_POINT('Ctrl Pts',(-10.3741366140001,11.6,-2.81073333600002));
#268253=CARTESIAN_POINT('Ctrl Pts',(-10.3716127990001,15.2,-2.81076515200001));
#268254=CARTESIAN_POINT('Ctrl Pts',(-10.3716127990001,11.6,-2.81076515200001));
#268255=CARTESIAN_POINT('Ctrl Pts',(-10.3690950810001,15.2,-2.81079473000001));
#268256=CARTESIAN_POINT('Ctrl Pts',(-10.3690950810001,11.6,-2.81079473000002));
#268257=CARTESIAN_POINT('Ctrl Pts',(-10.3665834700001,15.2,-2.81082207900001));
#268258=CARTESIAN_POINT('Ctrl Pts',(-10.3665834700001,11.6,-2.81082207900001));
#268259=CARTESIAN_POINT('Ctrl Pts',(-10.3640779820001,15.2,-2.81084720700001));
#268260=CARTESIAN_POINT('Ctrl Pts',(-10.3640779820001,11.6,-2.81084720700001));
#268261=CARTESIAN_POINT('Ctrl Pts',(-10.3615786240001,15.2,-2.81087012400001));
#268262=CARTESIAN_POINT('Ctrl Pts',(-10.3615786240001,11.6,-2.81087012400001));
#268263=CARTESIAN_POINT('Ctrl Pts',(-10.3590854110001,15.2,-2.81089083900001));
#268264=CARTESIAN_POINT('Ctrl Pts',(-10.3590854110001,11.6,-2.81089083900001));
#268265=CARTESIAN_POINT('Ctrl Pts',(-10.3565983540001,15.2,-2.81090936300001));
#268266=CARTESIAN_POINT('Ctrl Pts',(-10.3565983540001,11.6,-2.81090936300001));
#268267=CARTESIAN_POINT('Ctrl Pts',(-10.3541174660001,15.2,-2.81092570300002));
#268268=CARTESIAN_POINT('Ctrl Pts',(-10.3541174660001,11.6,-2.81092570300002));
#268269=CARTESIAN_POINT('Ctrl Pts',(-10.3516427590001,15.2,-2.81093986800002));
#268270=CARTESIAN_POINT('Ctrl Pts',(-10.3516427590001,11.6,-2.81093986800002));
#268271=CARTESIAN_POINT('Ctrl Pts',(-10.3491742450001,15.2,-2.81095186900002));
#268272=CARTESIAN_POINT('Ctrl Pts',(-10.3491742450001,11.6,-2.81095186900002));
#268273=CARTESIAN_POINT('Ctrl Pts',(-10.3467119360001,15.2,-2.81096171500002));
#268274=CARTESIAN_POINT('Ctrl Pts',(-10.3467119360001,11.6,-2.81096171500002));
#268275=CARTESIAN_POINT('Ctrl Pts',(-10.3442558440001,15.2,-2.81096941500001));
#268276=CARTESIAN_POINT('Ctrl Pts',(-10.3442558440001,11.6,-2.81096941500001));
#268277=CARTESIAN_POINT('Ctrl Pts',(-10.3418059810001,15.2,-2.81097497900001));
#268278=CARTESIAN_POINT('Ctrl Pts',(-10.3418059810001,11.6,-2.81097497900001));
#268279=CARTESIAN_POINT('Ctrl Pts',(-10.3393623600001,15.2,-2.81097841600001));
#268280=CARTESIAN_POINT('Ctrl Pts',(-10.3393623600001,11.6,-2.81097841600001));
#268281=CARTESIAN_POINT('Ctrl Pts',(-10.3369249940001,15.2,-2.81097973500001));
#268282=CARTESIAN_POINT('Ctrl Pts',(-10.3369249940001,11.6,-2.81097973500001));
#268283=CARTESIAN_POINT('Ctrl Pts',(-10.3344938940001,15.2,-2.81097894800002));
#268284=CARTESIAN_POINT('Ctrl Pts',(-10.3344938940001,11.6,-2.81097894800002));
#268285=CARTESIAN_POINT('Ctrl Pts',(-10.3320690720001,15.2,-2.81097606100001));
#268286=CARTESIAN_POINT('Ctrl Pts',(-10.3320690720001,11.6,-2.81097606100001));
#268287=CARTESIAN_POINT('Ctrl Pts',(-10.3296505420001,15.2,-2.81097108600001));
#268288=CARTESIAN_POINT('Ctrl Pts',(-10.3296505420001,11.6,-2.81097108600001));
#268289=CARTESIAN_POINT('Ctrl Pts',(-10.3272383160001,15.2,-2.81096403100001));
#268290=CARTESIAN_POINT('Ctrl Pts',(-10.3272383160001,11.6,-2.81096403100001));
#268291=CARTESIAN_POINT('Ctrl Pts',(-10.3248324060001,15.2,-2.81095490800002));
#268292=CARTESIAN_POINT('Ctrl Pts',(-10.3248324060001,11.6,-2.81095490800002));
#268293=CARTESIAN_POINT('Ctrl Pts',(-10.3224328240001,15.2,-2.81094372600001));
#268294=CARTESIAN_POINT('Ctrl Pts',(-10.3224328240001,11.6,-2.81094372600002));
#268295=CARTESIAN_POINT('Ctrl Pts',(-10.3200395830001,15.2,-2.81093049300001));
#268296=CARTESIAN_POINT('Ctrl Pts',(-10.3200395830001,11.6,-2.81093049300001));
#268297=CARTESIAN_POINT('Ctrl Pts',(-10.3176526950001,15.2,-2.81091522000001));
#268298=CARTESIAN_POINT('Ctrl Pts',(-10.3176526950001,11.6,-2.81091522000001));
#268299=CARTESIAN_POINT('Ctrl Pts',(-10.3152721750001,15.2,-2.81089791800001));
#268300=CARTESIAN_POINT('Ctrl Pts',(-10.3152721750001,11.6,-2.81089791800001));
#268301=CARTESIAN_POINT('Ctrl Pts',(-10.3128980330001,15.2,-2.81087859400001));
#268302=CARTESIAN_POINT('Ctrl Pts',(-10.3128980330001,11.6,-2.81087859400001));
#268303=CARTESIAN_POINT('Ctrl Pts',(-10.3105302810001,15.2,-2.81085726100001));
#268304=CARTESIAN_POINT('Ctrl Pts',(-10.3105302810001,11.6,-2.81085726100002));
#268305=CARTESIAN_POINT('Ctrl Pts',(-10.3081689340001,15.2,-2.81083392700001));
#268306=CARTESIAN_POINT('Ctrl Pts',(-10.3081689340001,11.6,-2.81083392700001));
#268307=CARTESIAN_POINT('Ctrl Pts',(-10.3058140040001,15.2,-2.81080860400001));
#268308=CARTESIAN_POINT('Ctrl Pts',(-10.3058140040001,11.6,-2.81080860400001));
#268309=CARTESIAN_POINT('Ctrl Pts',(-10.3034655040001,15.2,-2.81078129900001));
#268310=CARTESIAN_POINT('Ctrl Pts',(-10.3034655040001,11.6,-2.81078129900001));
#268311=CARTESIAN_POINT('Ctrl Pts',(-10.3011234450001,15.2,-2.81075202400002));
#268312=CARTESIAN_POINT('Ctrl Pts',(-10.3011234450001,11.6,-2.81075202400002));
#268313=CARTESIAN_POINT('Ctrl Pts',(-10.2987878420001,15.2,-2.81072079000001));
#268314=CARTESIAN_POINT('Ctrl Pts',(-10.2987878420001,11.6,-2.81072079000001));
#268315=CARTESIAN_POINT('Ctrl Pts',(-10.2964587060001,15.2,-2.81068760400002));
#268316=CARTESIAN_POINT('Ctrl Pts',(-10.2964587060001,11.6,-2.81068760400002));
#268317=CARTESIAN_POINT('Ctrl Pts',(-10.2941360500001,15.2,-2.81065248000001));
#268318=CARTESIAN_POINT('Ctrl Pts',(-10.2941360500001,11.6,-2.81065248000001));
#268319=CARTESIAN_POINT('Ctrl Pts',(-10.2918198870001,15.2,-2.81061542500002));
#268320=CARTESIAN_POINT('Ctrl Pts',(-10.2918198870001,11.6,-2.81061542500002));
#268321=CARTESIAN_POINT('Ctrl Pts',(-10.2895102320001,15.2,-2.81057645100002));
#268322=CARTESIAN_POINT('Ctrl Pts',(-10.2895102320001,11.6,-2.81057645100002));
#268323=CARTESIAN_POINT('Ctrl Pts',(-10.2872070960001,15.2,-2.81053556800002));
#268324=CARTESIAN_POINT('Ctrl Pts',(-10.2872070960001,11.6,-2.81053556800002));
#268325=CARTESIAN_POINT('Ctrl Pts',(-10.2849104920001,15.2,-2.81049278600001));
#268326=CARTESIAN_POINT('Ctrl Pts',(-10.2849104920001,11.6,-2.81049278600001));
#268327=CARTESIAN_POINT('Ctrl Pts',(-10.2826204320001,15.2,-2.81044811600001));
#268328=CARTESIAN_POINT('Ctrl Pts',(-10.2826204320001,11.6,-2.81044811600002));
#268329=CARTESIAN_POINT('Ctrl Pts',(-10.2803369320001,15.2,-2.81040156800001));
#268330=CARTESIAN_POINT('Ctrl Pts',(-10.2803369320001,11.6,-2.81040156800001));
#268331=CARTESIAN_POINT('Ctrl Pts',(-10.2780600020001,15.2,-2.81035315300001));
#268332=CARTESIAN_POINT('Ctrl Pts',(-10.2780600020001,11.6,-2.81035315300001));
#268333=CARTESIAN_POINT('Ctrl Pts',(-10.2757896570001,15.2,-2.81030288000002));
#268334=CARTESIAN_POINT('Ctrl Pts',(-10.2757896570001,11.6,-2.81030288000002));
#268335=CARTESIAN_POINT('Ctrl Pts',(-10.2735259090001,15.2,-2.81025076200002));
#268336=CARTESIAN_POINT('Ctrl Pts',(-10.2735259090001,11.6,-2.81025076200002));
#268337=CARTESIAN_POINT('Ctrl Pts',(-10.2712687710001,15.2,-2.81019680600001));
#268338=CARTESIAN_POINT('Ctrl Pts',(-10.2712687710001,11.6,-2.81019680600001));
#268339=CARTESIAN_POINT('Ctrl Pts',(-10.2690182590001,15.2,-2.81014102700002));
#268340=CARTESIAN_POINT('Ctrl Pts',(-10.2690182590001,11.6,-2.81014102700002));
#268341=CARTESIAN_POINT('Ctrl Pts',(-10.2667743820001,15.2,-2.81008343100002));
#268342=CARTESIAN_POINT('Ctrl Pts',(-10.2667743820001,11.6,-2.81008343100002));
#268343=CARTESIAN_POINT('Ctrl Pts',(-10.2645371560001,15.2,-2.81002403300001));
#268344=CARTESIAN_POINT('Ctrl Pts',(-10.2645371560001,11.6,-2.81002403300001));
#268345=CARTESIAN_POINT('Ctrl Pts',(-10.2623065940001,15.2,-2.80996284100001));
#268346=CARTESIAN_POINT('Ctrl Pts',(-10.2623065940001,11.6,-2.80996284100001));
#268347=CARTESIAN_POINT('Ctrl Pts',(-10.2600827090001,15.2,-2.80989986700002));
#268348=CARTESIAN_POINT('Ctrl Pts',(-10.2600827090001,11.6,-2.80989986700002));
#268349=CARTESIAN_POINT('Ctrl Pts',(-10.2578655120001,15.2,-2.80983512200002));
#268350=CARTESIAN_POINT('Ctrl Pts',(-10.2578655120001,11.6,-2.80983512200002));
#268351=CARTESIAN_POINT('Ctrl Pts',(-10.2556550210001,15.2,-2.80976861500001));
#268352=CARTESIAN_POINT('Ctrl Pts',(-10.2556550210001,11.6,-2.80976861500001));
#268353=CARTESIAN_POINT('Ctrl Pts',(-10.2534512460001,15.2,-2.80970035900001));
#268354=CARTESIAN_POINT('Ctrl Pts',(-10.2534512460001,11.6,-2.80970035900001));
#268355=CARTESIAN_POINT('Ctrl Pts',(-10.2512542030001,15.2,-2.80963036400002));
#268356=CARTESIAN_POINT('Ctrl Pts',(-10.2512542030001,11.6,-2.80963036400002));
#268357=CARTESIAN_POINT('Ctrl Pts',(-10.2490639020001,15.2,-2.80955864200001));
#268358=CARTESIAN_POINT('Ctrl Pts',(-10.2490639020001,11.6,-2.80955864200001));
#268359=CARTESIAN_POINT('Ctrl Pts',(-10.2468803590001,15.2,-2.80948520200001));
#268360=CARTESIAN_POINT('Ctrl Pts',(-10.2468803590001,11.6,-2.80948520200001));
#268361=CARTESIAN_POINT('Ctrl Pts',(-10.2447035880001,15.2,-2.80941005800001));
#268362=CARTESIAN_POINT('Ctrl Pts',(-10.2447035880001,11.6,-2.80941005800001));
#268363=CARTESIAN_POINT('Ctrl Pts',(-10.2425336010001,15.2,-2.80933321800001));
#268364=CARTESIAN_POINT('Ctrl Pts',(-10.2425336010001,11.6,-2.80933321800001));
#268365=CARTESIAN_POINT('Ctrl Pts',(-10.2403704120001,15.2,-2.80925469500001));
#268366=CARTESIAN_POINT('Ctrl Pts',(-10.2403704120001,11.6,-2.80925469500001));
#268367=CARTESIAN_POINT('Ctrl Pts',(-10.2382140350001,15.2,-2.80917450000001));
#268368=CARTESIAN_POINT('Ctrl Pts',(-10.2382140350001,11.6,-2.80917450000001));
#268369=CARTESIAN_POINT('Ctrl Pts',(-10.2360644840001,15.2,-2.80909264400002));
#268370=CARTESIAN_POINT('Ctrl Pts',(-10.2360644840001,11.6,-2.80909264400002));
#268371=CARTESIAN_POINT('Ctrl Pts',(-10.2339217720001,15.2,-2.80900913800001));
#268372=CARTESIAN_POINT('Ctrl Pts',(-10.2339217720001,11.6,-2.80900913800001));
#268373=CARTESIAN_POINT('Ctrl Pts',(-10.2317859140001,15.2,-2.80892399500001));
#268374=CARTESIAN_POINT('Ctrl Pts',(-10.2317859140001,11.6,-2.80892399500001));
#268375=CARTESIAN_POINT('Ctrl Pts',(-10.2296569220001,15.2,-2.80883722400001));
#268376=CARTESIAN_POINT('Ctrl Pts',(-10.2296569220001,11.6,-2.80883722400001));
#268377=CARTESIAN_POINT('Ctrl Pts',(-10.2275348110001,15.2,-2.80874883800001));
#268378=CARTESIAN_POINT('Ctrl Pts',(-10.2275348110001,11.6,-2.80874883800002));
#268379=CARTESIAN_POINT('Ctrl Pts',(-10.2254195960001,15.2,-2.80865884700002));
#268380=CARTESIAN_POINT('Ctrl Pts',(-10.2254195960001,11.6,-2.80865884700002));
#268381=CARTESIAN_POINT('Ctrl Pts',(-10.2233112870001,15.2,-2.80856726500001));
#268382=CARTESIAN_POINT('Ctrl Pts',(-10.2233112870001,11.6,-2.80856726500002));
#268383=CARTESIAN_POINT('Ctrl Pts',(-10.2212099030001,15.2,-2.80847410200002));
#268384=CARTESIAN_POINT('Ctrl Pts',(-10.2212099030001,11.6,-2.80847410200002));
#268385=CARTESIAN_POINT('Ctrl Pts',(-10.2191154540001,15.2,-2.80837937100001));
#268386=CARTESIAN_POINT('Ctrl Pts',(-10.2191154540001,11.6,-2.80837937100001));
#268387=CARTESIAN_POINT('Ctrl Pts',(-10.2170279560001,15.2,-2.80828308000002));
#268388=CARTESIAN_POINT('Ctrl Pts',(-10.2170279560001,11.6,-2.80828308000002));
#268389=CARTESIAN_POINT('Ctrl Pts',(-10.2149474230001,15.2,-2.80818524500001));
#268390=CARTESIAN_POINT('Ctrl Pts',(-10.2149474230001,11.6,-2.80818524500001));
#268391=CARTESIAN_POINT('Ctrl Pts',(-10.2128738680001,15.2,-2.80808587500001));
#268392=CARTESIAN_POINT('Ctrl Pts',(-10.2128738680001,11.6,-2.80808587500002));
#268393=CARTESIAN_POINT('Ctrl Pts',(-10.2108073070001,15.2,-2.80798498300001));
#268394=CARTESIAN_POINT('Ctrl Pts',(-10.2108073070001,11.6,-2.80798498300001));
#268395=CARTESIAN_POINT('Ctrl Pts',(-10.2087477520001,15.2,-2.80788258200001));
#268396=CARTESIAN_POINT('Ctrl Pts',(-10.2087477520001,11.6,-2.80788258200001));
#268397=CARTESIAN_POINT('Ctrl Pts',(-10.2066952180001,15.2,-2.80777868100001));
#268398=CARTESIAN_POINT('Ctrl Pts',(-10.2066952180001,11.6,-2.80777868100001));
#268399=CARTESIAN_POINT('Ctrl Pts',(-10.2046497210001,15.2,-2.80767329400001));
#268400=CARTESIAN_POINT('Ctrl Pts',(-10.2046497210001,11.6,-2.80767329400002));
#268401=CARTESIAN_POINT('Ctrl Pts',(-10.2026112720001,15.2,-2.80756643300001));
#268402=CARTESIAN_POINT('Ctrl Pts',(-10.2026112720001,11.6,-2.80756643300002));
#268403=CARTESIAN_POINT('Ctrl Pts',(-10.2005798890001,15.2,-2.80745810900001));
#268404=CARTESIAN_POINT('Ctrl Pts',(-10.2005798890001,11.6,-2.80745810900001));
#268405=CARTESIAN_POINT('Ctrl Pts',(-10.1985555830001,15.2,-2.80734833400002));
#268406=CARTESIAN_POINT('Ctrl Pts',(-10.1985555830001,11.6,-2.80734833400002));
#268407=CARTESIAN_POINT('Ctrl Pts',(-10.1965383710001,15.2,-2.80723712200002));
#268408=CARTESIAN_POINT('Ctrl Pts',(-10.1965383710001,11.6,-2.80723712200002));
#268409=CARTESIAN_POINT('Ctrl Pts',(-10.1945282670001,15.2,-2.80712448400001));
#268410=CARTESIAN_POINT('Ctrl Pts',(-10.1945282670001,11.6,-2.80712448400001));
#268411=CARTESIAN_POINT('Ctrl Pts',(-10.1925252840001,15.2,-2.80701043200001));
#268412=CARTESIAN_POINT('Ctrl Pts',(-10.1925252840001,11.6,-2.80701043200001));
#268413=CARTESIAN_POINT('Ctrl Pts',(-10.1905294380001,15.2,-2.80689497800001));
#268414=CARTESIAN_POINT('Ctrl Pts',(-10.1905294380001,11.6,-2.80689497800001));
#268415=CARTESIAN_POINT('Ctrl Pts',(-10.1885407420001,15.2,-2.80677813600001));
#268416=CARTESIAN_POINT('Ctrl Pts',(-10.1885407420001,11.6,-2.80677813600001));
#268417=CARTESIAN_POINT('Ctrl Pts',(-10.1865592120001,15.2,-2.80665991700001));
#268418=CARTESIAN_POINT('Ctrl Pts',(-10.1865592120001,11.6,-2.80665991700001));
#268419=CARTESIAN_POINT('Ctrl Pts',(-10.1845848630001,15.2,-2.80654033300001));
#268420=CARTESIAN_POINT('Ctrl Pts',(-10.1845848630001,11.6,-2.80654033300001));
#268421=CARTESIAN_POINT('Ctrl Pts',(-10.1826177100001,15.2,-2.80641939900002));
#268422=CARTESIAN_POINT('Ctrl Pts',(-10.1826177100001,11.6,-2.80641939900002));
#268423=CARTESIAN_POINT('Ctrl Pts',(-10.1806577650001,15.2,-2.80629712500001));
#268424=CARTESIAN_POINT('Ctrl Pts',(-10.1806577650001,11.6,-2.80629712500002));
#268425=CARTESIAN_POINT('Ctrl Pts',(-10.1787050450001,15.2,-2.80617352500002));
#268426=CARTESIAN_POINT('Ctrl Pts',(-10.1787050450001,11.6,-2.80617352500002));
#268427=CARTESIAN_POINT('Ctrl Pts',(-10.1767595650001,15.2,-2.80604861000001));
#268428=CARTESIAN_POINT('Ctrl Pts',(-10.1767595650001,11.6,-2.80604861000001));
#268429=CARTESIAN_POINT('Ctrl Pts',(-10.1748213380001,15.2,-2.80592239500002));
#268430=CARTESIAN_POINT('Ctrl Pts',(-10.1748213380001,11.6,-2.80592239500002));
#268431=CARTESIAN_POINT('Ctrl Pts',(-10.1728903810001,15.2,-2.80579489000001));
#268432=CARTESIAN_POINT('Ctrl Pts',(-10.1728903810001,11.6,-2.80579489000001));
#268433=CARTESIAN_POINT('Ctrl Pts',(-10.1709667090001,15.2,-2.80566611100001));
#268434=CARTESIAN_POINT('Ctrl Pts',(-10.1709667090001,11.6,-2.80566611100001));
#268435=CARTESIAN_POINT('Ctrl Pts',(-10.1690503350001,15.2,-2.80553606900002));
#268436=CARTESIAN_POINT('Ctrl Pts',(-10.1690503350001,11.6,-2.80553606900002));
#268437=CARTESIAN_POINT('Ctrl Pts',(-10.1671412760001,15.2,-2.80540477800002));
#268438=CARTESIAN_POINT('Ctrl Pts',(-10.1671412760001,11.6,-2.80540477800002));
#268439=CARTESIAN_POINT('Ctrl Pts',(-10.1652395470001,15.2,-2.80527224900001));
#268440=CARTESIAN_POINT('Ctrl Pts',(-10.1652395470001,11.6,-2.80527224900002));
#268441=CARTESIAN_POINT('Ctrl Pts',(-10.1633451610001,15.2,-2.80513849600001));
#268442=CARTESIAN_POINT('Ctrl Pts',(-10.1633451610001,11.6,-2.80513849600002));
#268443=CARTESIAN_POINT('Ctrl Pts',(-10.1614581350001,15.2,-2.80500353400001));
#268444=CARTESIAN_POINT('Ctrl Pts',(-10.1614581350001,11.6,-2.80500353400001));
#268445=CARTESIAN_POINT('Ctrl Pts',(-10.1595784840001,15.2,-2.80486737300001));
#268446=CARTESIAN_POINT('Ctrl Pts',(-10.1595784840001,11.6,-2.80486737300001));
#268447=CARTESIAN_POINT('Ctrl Pts',(-10.1577062240001,15.2,-2.80473002900001));
#268448=CARTESIAN_POINT('Ctrl Pts',(-10.1577062240001,11.6,-2.80473002900001));
#268449=CARTESIAN_POINT('Ctrl Pts',(-10.1558413680001,15.2,-2.80459151300001));
#268450=CARTESIAN_POINT('Ctrl Pts',(-10.1558413680001,11.6,-2.80459151300001));
#268451=CARTESIAN_POINT('Ctrl Pts',(-10.1539839340001,15.2,-2.80445183900001));
#268452=CARTESIAN_POINT('Ctrl Pts',(-10.1539839340001,11.6,-2.80445183900001));
#268453=CARTESIAN_POINT('Ctrl Pts',(-10.1521339360001,15.2,-2.80431102100001));
#268454=CARTESIAN_POINT('Ctrl Pts',(-10.1521339360001,11.6,-2.80431102100001));
#268455=CARTESIAN_POINT('Ctrl Pts',(-10.1502913890001,15.2,-2.80416907300001));
#268456=CARTESIAN_POINT('Ctrl Pts',(-10.1502913890001,11.6,-2.80416907300001));
#268457=CARTESIAN_POINT('Ctrl Pts',(-10.1484563090001,15.2,-2.80402600700001));
#268458=CARTESIAN_POINT('Ctrl Pts',(-10.1484563090001,11.6,-2.80402600700001));
#268459=CARTESIAN_POINT('Ctrl Pts',(-10.1466287130001,15.2,-2.80388183700001));
#268460=CARTESIAN_POINT('Ctrl Pts',(-10.1466287130001,11.6,-2.80388183700001));
#268461=CARTESIAN_POINT('Ctrl Pts',(-10.1448086140001,15.2,-2.80373657700002));
#268462=CARTESIAN_POINT('Ctrl Pts',(-10.1448086140001,11.6,-2.80373657700002));
#268463=CARTESIAN_POINT('Ctrl Pts',(-10.1429960300001,15.2,-2.80359024000001));
#268464=CARTESIAN_POINT('Ctrl Pts',(-10.1429960300001,11.6,-2.80359024000001));
#268465=CARTESIAN_POINT('Ctrl Pts',(-10.1411909760001,15.2,-2.80344284000002));
#268466=CARTESIAN_POINT('Ctrl Pts',(-10.1411909760001,11.6,-2.80344284000002));
#268467=CARTESIAN_POINT('Ctrl Pts',(-10.1393934660001,15.2,-2.80329439100001));
#268468=CARTESIAN_POINT('Ctrl Pts',(-10.1393934660001,11.6,-2.80329439100001));
#268469=CARTESIAN_POINT('Ctrl Pts',(-10.1376035180001,15.2,-2.80314490700002));
#268470=CARTESIAN_POINT('Ctrl Pts',(-10.1376035180001,11.6,-2.80314490700002));
#268471=CARTESIAN_POINT('Ctrl Pts',(-10.1358211480001,15.2,-2.80299440200002));
#268472=CARTESIAN_POINT('Ctrl Pts',(-10.1358211480001,11.6,-2.80299440200002));
#268473=CARTESIAN_POINT('Ctrl Pts',(-10.1340463700001,15.2,-2.80284288800001));
#268474=CARTESIAN_POINT('Ctrl Pts',(-10.1340463700001,11.6,-2.80284288800001));
#268475=CARTESIAN_POINT('Ctrl Pts',(-10.1322792010001,15.2,-2.80269038200001));
#268476=CARTESIAN_POINT('Ctrl Pts',(-10.1322792010001,11.6,-2.80269038200002));
#268477=CARTESIAN_POINT('Ctrl Pts',(-10.1305196570001,15.2,-2.80253689600002));
#268478=CARTESIAN_POINT('Ctrl Pts',(-10.1305196570001,11.6,-2.80253689600002));
#268479=CARTESIAN_POINT('Ctrl Pts',(-10.1287677530001,15.2,-2.80238244500001));
#268480=CARTESIAN_POINT('Ctrl Pts',(-10.1287677530001,11.6,-2.80238244500001));
#268481=CARTESIAN_POINT('Ctrl Pts',(-10.1270235070001,15.2,-2.80222704300002));
#268482=CARTESIAN_POINT('Ctrl Pts',(-10.1270235070001,11.6,-2.80222704300002));
#268483=CARTESIAN_POINT('Ctrl Pts',(-10.1252869340001,15.2,-2.80207070400001));
#268484=CARTESIAN_POINT('Ctrl Pts',(-10.1252869340001,11.6,-2.80207070400001));
#268485=CARTESIAN_POINT('Ctrl Pts',(-10.1235580500001,15.2,-2.80191344300002));
#268486=CARTESIAN_POINT('Ctrl Pts',(-10.1235580500001,11.6,-2.80191344300002));
#268487=CARTESIAN_POINT('Ctrl Pts',(-10.1218368710001,15.2,-2.80175527400001));
#268488=CARTESIAN_POINT('Ctrl Pts',(-10.1218368710001,11.6,-2.80175527400001));
#268489=CARTESIAN_POINT('Ctrl Pts',(-10.1201234150001,15.2,-2.80159621100001));
#268490=CARTESIAN_POINT('Ctrl Pts',(-10.1201234150001,11.6,-2.80159621100002));
#268491=CARTESIAN_POINT('Ctrl Pts',(-10.1184176970001,15.2,-2.80143626900001));
#268492=CARTESIAN_POINT('Ctrl Pts',(-10.1184176970001,11.6,-2.80143626900002));
#268493=CARTESIAN_POINT('Ctrl Pts',(-10.1167197340001,15.2,-2.80127546300001));
#268494=CARTESIAN_POINT('Ctrl Pts',(-10.1167197340001,11.6,-2.80127546300002));
#268495=CARTESIAN_POINT('Ctrl Pts',(-10.1150295420001,15.2,-2.80111380600002));
#268496=CARTESIAN_POINT('Ctrl Pts',(-10.1150295420001,11.6,-2.80111380600002));
#268497=CARTESIAN_POINT('Ctrl Pts',(-10.1133471370001,15.2,-2.80095131400001));
#268498=CARTESIAN_POINT('Ctrl Pts',(-10.1133471370001,11.6,-2.80095131400001));
#268499=CARTESIAN_POINT('Ctrl Pts',(-10.1116725360001,15.2,-2.80078800200001));
#268500=CARTESIAN_POINT('Ctrl Pts',(-10.1116725360001,11.6,-2.80078800200001));
#268501=CARTESIAN_POINT('Ctrl Pts',(-10.1100057560001,15.2,-2.80062388500002));
#268502=CARTESIAN_POINT('Ctrl Pts',(-10.1100057560001,11.6,-2.80062388500002));
#268503=CARTESIAN_POINT('Ctrl Pts',(-10.1083468140001,15.2,-2.80045897600001));
#268504=CARTESIAN_POINT('Ctrl Pts',(-10.1083468140001,11.6,-2.80045897600001));
#268505=CARTESIAN_POINT('Ctrl Pts',(-10.1066957250001,15.2,-2.80029329300001));
#268506=CARTESIAN_POINT('Ctrl Pts',(-10.1066957250001,11.6,-2.80029329300001));
#268507=CARTESIAN_POINT('Ctrl Pts',(-10.1050525090001,15.2,-2.80012684900001));
#268508=CARTESIAN_POINT('Ctrl Pts',(-10.1050525090001,11.6,-2.80012684900001));
#268509=CARTESIAN_POINT('Ctrl Pts',(-10.1034171790001,15.2,-2.79995965800001));
#268510=CARTESIAN_POINT('Ctrl Pts',(-10.1034171790001,11.6,-2.79995965800001));
#268511=CARTESIAN_POINT('Ctrl Pts',(-10.1017897540001,15.2,-2.79979173800001));
#268512=CARTESIAN_POINT('Ctrl Pts',(-10.1017897540001,11.6,-2.79979173800002));
#268513=CARTESIAN_POINT('Ctrl Pts',(-10.1001702510001,15.2,-2.79962310200002));
#268514=CARTESIAN_POINT('Ctrl Pts',(-10.1001702510001,11.6,-2.79962310200002));
#268515=CARTESIAN_POINT('Ctrl Pts',(-10.0985586870001,15.2,-2.79945376700002));
#268516=CARTESIAN_POINT('Ctrl Pts',(-10.0985586870001,11.6,-2.79945376700002));
#268517=CARTESIAN_POINT('Ctrl Pts',(-10.0969550780001,15.2,-2.79928374700001));
#268518=CARTESIAN_POINT('Ctrl Pts',(-10.0969550780001,11.6,-2.79928374700001));
#268519=CARTESIAN_POINT('Ctrl Pts',(-10.0953594420001,15.2,-2.79911305800002));
#268520=CARTESIAN_POINT('Ctrl Pts',(-10.0953594420001,11.6,-2.79911305800002));
#268521=CARTESIAN_POINT('Ctrl Pts',(-10.0937717960001,15.2,-2.79894171500001));
#268522=CARTESIAN_POINT('Ctrl Pts',(-10.0937717960001,11.6,-2.79894171500001));
#268523=CARTESIAN_POINT('Ctrl Pts',(-10.0921921570001,15.2,-2.79876973500001));
#268524=CARTESIAN_POINT('Ctrl Pts',(-10.0921921570001,11.6,-2.79876973500001));
#268525=CARTESIAN_POINT('Ctrl Pts',(-10.0906205420001,15.2,-2.79859713200001));
#268526=CARTESIAN_POINT('Ctrl Pts',(-10.0906205420001,11.6,-2.79859713200001));
#268527=CARTESIAN_POINT('Ctrl Pts',(-10.0890569700001,15.2,-2.79842392300001));
#268528=CARTESIAN_POINT('Ctrl Pts',(-10.0890569700001,11.6,-2.79842392300001));
#268529=CARTESIAN_POINT('Ctrl Pts',(-10.0875014570001,15.2,-2.79825012400002));
#268530=CARTESIAN_POINT('Ctrl Pts',(-10.0875014570001,11.6,-2.79825012400002));
#268531=CARTESIAN_POINT('Ctrl Pts',(-10.0859540200001,15.2,-2.79807574900001));
#268532=CARTESIAN_POINT('Ctrl Pts',(-10.0859540200001,11.6,-2.79807574900001));
#268533=CARTESIAN_POINT('Ctrl Pts',(-10.0844146780001,15.2,-2.79790081600002));
#268534=CARTESIAN_POINT('Ctrl Pts',(-10.0844146780001,11.6,-2.79790081600002));
#268535=CARTESIAN_POINT('Ctrl Pts',(-10.0828834480001,15.2,-2.79772534000001));
#268536=CARTESIAN_POINT('Ctrl Pts',(-10.0828834480001,11.6,-2.79772534000002));
#268537=CARTESIAN_POINT('Ctrl Pts',(-10.0813603480001,15.2,-2.79754933600001));
#268538=CARTESIAN_POINT('Ctrl Pts',(-10.0813603480001,11.6,-2.79754933600001));
#268539=CARTESIAN_POINT('Ctrl Pts',(-10.0798453950001,15.2,-2.79737282200001));
#268540=CARTESIAN_POINT('Ctrl Pts',(-10.0798453950001,11.6,-2.79737282200002));
#268541=CARTESIAN_POINT('Ctrl Pts',(-10.0783386060001,15.2,-2.79719581400002));
#268542=CARTESIAN_POINT('Ctrl Pts',(-10.0783386060001,11.6,-2.79719581400002));
#268543=CARTESIAN_POINT('Ctrl Pts',(-10.0768400010001,15.2,-2.79701832800002));
#268544=CARTESIAN_POINT('Ctrl Pts',(-10.0768400010001,11.6,-2.79701832800002));
#268545=CARTESIAN_POINT('Ctrl Pts',(-10.0753495960001,15.2,-2.79684038000001));
#268546=CARTESIAN_POINT('Ctrl Pts',(-10.0753495960001,11.6,-2.79684038000001));
#268547=CARTESIAN_POINT('Ctrl Pts',(-10.0738674120001,15.2,-2.79666198700002));
#268548=CARTESIAN_POINT('Ctrl Pts',(-10.0738674120001,11.6,-2.79666198700002));
#268549=CARTESIAN_POINT('Ctrl Pts',(-10.0723934620001,15.2,-2.79648316500001));
#268550=CARTESIAN_POINT('Ctrl Pts',(-10.0723934620001,11.6,-2.79648316500001));
#268551=CARTESIAN_POINT('Ctrl Pts',(-10.0709277690001,15.2,-2.79630393100001));
#268552=CARTESIAN_POINT('Ctrl Pts',(-10.0709277690001,11.6,-2.79630393100002));
#268553=CARTESIAN_POINT('Ctrl Pts',(-10.0694703480001,15.2,-2.79612430200002));
#268554=CARTESIAN_POINT('Ctrl Pts',(-10.0694703480001,11.6,-2.79612430200002));
#268555=CARTESIAN_POINT('Ctrl Pts',(-10.0680212180001,15.2,-2.79594429400001));
#268556=CARTESIAN_POINT('Ctrl Pts',(-10.0680212180001,11.6,-2.79594429400001));
#268557=CARTESIAN_POINT('Ctrl Pts',(-10.0665803990001,15.2,-2.79576392500001));
#268558=CARTESIAN_POINT('Ctrl Pts',(-10.0665803990001,11.6,-2.79576392500001));
#268559=CARTESIAN_POINT('Ctrl Pts',(-10.0651479080001,15.2,-2.79558321000001));
#268560=CARTESIAN_POINT('Ctrl Pts',(-10.0651479080001,11.6,-2.79558321000001));
#268561=CARTESIAN_POINT('Ctrl Pts',(-10.0637237620001,15.2,-2.79540216900001));
#268562=CARTESIAN_POINT('Ctrl Pts',(-10.0637237620001,11.6,-2.79540216900001));
#268563=CARTESIAN_POINT('Ctrl Pts',(-10.0623079820001,15.2,-2.79522081700001));
#268564=CARTESIAN_POINT('Ctrl Pts',(-10.0623079820001,11.6,-2.79522081700002));
#268565=CARTESIAN_POINT('Ctrl Pts',(-10.0609005850001,15.2,-2.79503917100001));
#268566=CARTESIAN_POINT('Ctrl Pts',(-10.0609005850001,11.6,-2.79503917100001));
#268567=CARTESIAN_POINT('Ctrl Pts',(-10.0595015910001,15.2,-2.79485724800002));
#268568=CARTESIAN_POINT('Ctrl Pts',(-10.0595015910001,11.6,-2.79485724800002));
#268569=CARTESIAN_POINT('Ctrl Pts',(-10.0581110160001,15.2,-2.79467506700001));
#268570=CARTESIAN_POINT('Ctrl Pts',(-10.0581110160001,11.6,-2.79467506700001));
#268571=CARTESIAN_POINT('Ctrl Pts',(-10.0567288820001,15.2,-2.79449264500002));
#268572=CARTESIAN_POINT('Ctrl Pts',(-10.0567288820001,11.6,-2.79449264500002));
#268573=CARTESIAN_POINT('Ctrl Pts',(-10.0553552060001,15.2,-2.79430999900002));
#268574=CARTESIAN_POINT('Ctrl Pts',(-10.0553552060001,11.6,-2.79430999900002));
#268575=CARTESIAN_POINT('Ctrl Pts',(-10.0539900080001,15.2,-2.79412714600001));
#268576=CARTESIAN_POINT('Ctrl Pts',(-10.0539900080001,11.6,-2.79412714600001));
#268577=CARTESIAN_POINT('Ctrl Pts',(-10.0526333070001,15.2,-2.79394410600001));
#268578=CARTESIAN_POINT('Ctrl Pts',(-10.0526333070001,11.6,-2.79394410600002));
#268579=CARTESIAN_POINT('Ctrl Pts',(-10.0512851200001,15.2,-2.79376089400001));
#268580=CARTESIAN_POINT('Ctrl Pts',(-10.0512851200001,11.6,-2.79376089400001));
#268581=CARTESIAN_POINT('Ctrl Pts',(-10.0499454690001,15.2,-2.79357752900002));
#268582=CARTESIAN_POINT('Ctrl Pts',(-10.0499454690001,11.6,-2.79357752900002));
#268583=CARTESIAN_POINT('Ctrl Pts',(-10.0486143700001,15.2,-2.79339402900002));
#268584=CARTESIAN_POINT('Ctrl Pts',(-10.0486143700001,11.6,-2.79339402900002));
#268585=CARTESIAN_POINT('Ctrl Pts',(-10.0472918460001,15.2,-2.79321041100001));
#268586=CARTESIAN_POINT('Ctrl Pts',(-10.0472918460001,11.6,-2.79321041100001));
#268587=CARTESIAN_POINT('Ctrl Pts',(-10.0459779130001,15.2,-2.79302669500002));
#268588=CARTESIAN_POINT('Ctrl Pts',(-10.0459779130001,11.6,-2.79302669500002));
#268589=CARTESIAN_POINT('Ctrl Pts',(-10.0446725930001,15.2,-2.79284289900001));
#268590=CARTESIAN_POINT('Ctrl Pts',(-10.0446725930001,11.6,-2.79284289900001));
#268591=CARTESIAN_POINT('Ctrl Pts',(-10.0433759040001,15.2,-2.79265904000002));
#268592=CARTESIAN_POINT('Ctrl Pts',(-10.0433759040001,11.6,-2.79265904000002));
#268593=CARTESIAN_POINT('Ctrl Pts',(-10.0420878650001,15.2,-2.79247513800001));
#268594=CARTESIAN_POINT('Ctrl Pts',(-10.0420878650001,11.6,-2.79247513800002));
#268595=CARTESIAN_POINT('Ctrl Pts',(-10.0408084970001,15.2,-2.79229120900002));
#268596=CARTESIAN_POINT('Ctrl Pts',(-10.0408084970001,11.6,-2.79229120900002));
#268597=CARTESIAN_POINT('Ctrl Pts',(-10.0395378210001,15.2,-2.79210727300002));
#268598=CARTESIAN_POINT('Ctrl Pts',(-10.0395378210001,11.6,-2.79210727300002));
#268599=CARTESIAN_POINT('Ctrl Pts',(-10.0382758530001,15.2,-2.79192335000001));
#268600=CARTESIAN_POINT('Ctrl Pts',(-10.0382758530001,11.6,-2.79192335000001));
#268601=CARTESIAN_POINT('Ctrl Pts',(-10.0370226160001,15.2,-2.79173945600002));
#268602=CARTESIAN_POINT('Ctrl Pts',(-10.0370226160001,11.6,-2.79173945600002));
#268603=CARTESIAN_POINT('Ctrl Pts',(-10.0357781300001,15.2,-2.79155561300001));
#268604=CARTESIAN_POINT('Ctrl Pts',(-10.0357781300001,11.6,-2.79155561300001));
#268605=CARTESIAN_POINT('Ctrl Pts',(-10.0345424120001,15.2,-2.79137183600001));
#268606=CARTESIAN_POINT('Ctrl Pts',(-10.0345424120001,11.6,-2.79137183600001));
#268607=CARTESIAN_POINT('Ctrl Pts',(-10.0333154850001,15.2,-2.79118814800002));
#268608=CARTESIAN_POINT('Ctrl Pts',(-10.0333154850001,11.6,-2.79118814800002));
#268609=CARTESIAN_POINT('Ctrl Pts',(-10.0320973690001,15.2,-2.79100456500001));
#268610=CARTESIAN_POINT('Ctrl Pts',(-10.0320973690001,11.6,-2.79100456500002));
#268611=CARTESIAN_POINT('Ctrl Pts',(-10.0308880840001,15.2,-2.79082110900001));
#268612=CARTESIAN_POINT('Ctrl Pts',(-10.0308880840001,11.6,-2.79082110900002));
#268613=CARTESIAN_POINT('Ctrl Pts',(-10.0296876490001,15.2,-2.79063779700001));
#268614=CARTESIAN_POINT('Ctrl Pts',(-10.0296876490001,11.6,-2.79063779700001));
#268615=CARTESIAN_POINT('Ctrl Pts',(-10.0284960860001,15.2,-2.79045465000001));
#268616=CARTESIAN_POINT('Ctrl Pts',(-10.0284960860001,11.6,-2.79045465000001));
#268617=CARTESIAN_POINT('Ctrl Pts',(-10.0273134150001,15.2,-2.79027168600001));
#268618=CARTESIAN_POINT('Ctrl Pts',(-10.0273134150001,11.6,-2.79027168600001));
#268619=CARTESIAN_POINT('Ctrl Pts',(-10.0261396570001,15.2,-2.79008892600002));
#268620=CARTESIAN_POINT('Ctrl Pts',(-10.0261396570001,11.6,-2.79008892600002));
#268621=CARTESIAN_POINT('Ctrl Pts',(-10.0249748320001,15.2,-2.78990638900002));
#268622=CARTESIAN_POINT('Ctrl Pts',(-10.0249748320001,11.6,-2.78990638900002));
#268623=CARTESIAN_POINT('Ctrl Pts',(-10.0238189610001,15.2,-2.78972409500001));
#268624=CARTESIAN_POINT('Ctrl Pts',(-10.0238189610001,11.6,-2.78972409500002));
#268625=CARTESIAN_POINT('Ctrl Pts',(-10.0226720660001,15.2,-2.78954206400002));
#268626=CARTESIAN_POINT('Ctrl Pts',(-10.0226720660001,11.6,-2.78954206400002));
#268627=CARTESIAN_POINT('Ctrl Pts',(-10.0215341660001,15.2,-2.78936031700002));
#268628=CARTESIAN_POINT('Ctrl Pts',(-10.0215341660001,11.6,-2.78936031700002));
#268629=CARTESIAN_POINT('Ctrl Pts',(-10.0204052840001,15.2,-2.78917887200001));
#268630=CARTESIAN_POINT('Ctrl Pts',(-10.0204052840001,11.6,-2.78917887200001));
#268631=CARTESIAN_POINT('Ctrl Pts',(-10.0192854400001,15.2,-2.78899774900002));
#268632=CARTESIAN_POINT('Ctrl Pts',(-10.0192854400001,11.6,-2.78899774900002));
#268633=CARTESIAN_POINT('Ctrl Pts',(-10.0181746550001,15.2,-2.78881697100001));
#268634=CARTESIAN_POINT('Ctrl Pts',(-10.0181746550001,11.6,-2.78881697100001));
#268635=CARTESIAN_POINT('Ctrl Pts',(-10.0170729510001,15.2,-2.78863655800001));
#268636=CARTESIAN_POINT('Ctrl Pts',(-10.0170729510001,11.6,-2.78863655800001));
#268637=CARTESIAN_POINT('Ctrl Pts',(-10.0159803500001,15.2,-2.78845652900001));
#268638=CARTESIAN_POINT('Ctrl Pts',(-10.0159803500001,11.6,-2.78845652900001));
#268639=CARTESIAN_POINT('Ctrl Pts',(-10.0148968710001,15.2,-2.78827690400002));
#268640=CARTESIAN_POINT('Ctrl Pts',(-10.0148968710001,11.6,-2.78827690400002));
#268641=CARTESIAN_POINT('Ctrl Pts',(-10.0138225390001,15.2,-2.78809770600001));
#268642=CARTESIAN_POINT('Ctrl Pts',(-10.0138225390001,11.6,-2.78809770600001));
#268643=CARTESIAN_POINT('Ctrl Pts',(-10.0127573730001,15.2,-2.78791895500001));
#268644=CARTESIAN_POINT('Ctrl Pts',(-10.0127573730001,11.6,-2.78791895500001));
#268645=CARTESIAN_POINT('Ctrl Pts',(-10.0117013970001,15.2,-2.78774067200001));
#268646=CARTESIAN_POINT('Ctrl Pts',(-10.0117013970001,11.6,-2.78774067200001));
#268647=CARTESIAN_POINT('Ctrl Pts',(-10.0106546300001,15.2,-2.78756287700002));
#268648=CARTESIAN_POINT('Ctrl Pts',(-10.0106546300001,11.6,-2.78756287700002));
#268649=CARTESIAN_POINT('Ctrl Pts',(-10.0096170970001,15.2,-2.78738559300002));
#268650=CARTESIAN_POINT('Ctrl Pts',(-10.0096170970001,11.6,-2.78738559300002));
#268651=CARTESIAN_POINT('Ctrl Pts',(-10.0085888180001,15.2,-2.78720884000002));
#268652=CARTESIAN_POINT('Ctrl Pts',(-10.0085888180001,11.6,-2.78720884000002));
#268653=CARTESIAN_POINT('Ctrl Pts',(-10.0075698160001,15.2,-2.78703264000002));
#268654=CARTESIAN_POINT('Ctrl Pts',(-10.0075698160001,11.6,-2.78703264000002));
#268655=CARTESIAN_POINT('Ctrl Pts',(-10.0065601130001,15.2,-2.78685701400001));
#268656=CARTESIAN_POINT('Ctrl Pts',(-10.0065601130001,11.6,-2.78685701400002));
#268657=CARTESIAN_POINT('Ctrl Pts',(-10.0055597320001,15.2,-2.78668198500001));
#268658=CARTESIAN_POINT('Ctrl Pts',(-10.0055597320001,11.6,-2.78668198500002));
#268659=CARTESIAN_POINT('Ctrl Pts',(-10.0045686950001,15.2,-2.78650757300001));
#268660=CARTESIAN_POINT('Ctrl Pts',(-10.0045686950001,11.6,-2.78650757300001));
#268661=CARTESIAN_POINT('Ctrl Pts',(-10.0035870240001,15.2,-2.78633380100001));
#268662=CARTESIAN_POINT('Ctrl Pts',(-10.0035870240001,11.6,-2.78633380100001));
#268663=CARTESIAN_POINT('Ctrl Pts',(-10.0026147430001,15.2,-2.78616069100002));
#268664=CARTESIAN_POINT('Ctrl Pts',(-10.0026147430001,11.6,-2.78616069100002));
#268665=CARTESIAN_POINT('Ctrl Pts',(-10.0016518730001,15.2,-2.78598826400001));
#268666=CARTESIAN_POINT('Ctrl Pts',(-10.0016518730001,11.6,-2.78598826400001));
#268667=CARTESIAN_POINT('Ctrl Pts',(-10.0006984370001,15.2,-2.78581654400002));
#268668=CARTESIAN_POINT('Ctrl Pts',(-10.0006984370001,11.6,-2.78581654400002));
#268669=CARTESIAN_POINT('Ctrl Pts',(-9.99975446000006,15.2,-2.78564555200001));
#268670=CARTESIAN_POINT('Ctrl Pts',(-9.99975446000006,11.6,-2.78564555200001));
#268671=CARTESIAN_POINT('Ctrl Pts',(-9.99881996400006,15.2,-2.78547531100001));
#268672=CARTESIAN_POINT('Ctrl Pts',(-9.99881996400006,11.6,-2.78547531100001));
#268673=CARTESIAN_POINT('Ctrl Pts',(-9.99789497300006,15.2,-2.78530584400002));
#268674=CARTESIAN_POINT('Ctrl Pts',(-9.99789497300006,11.6,-2.78530584400002));
#268675=CARTESIAN_POINT('Ctrl Pts',(-9.99697950700006,15.2,-2.78513717200001));
#268676=CARTESIAN_POINT('Ctrl Pts',(-9.99697950700006,11.6,-2.78513717200001));
#268677=CARTESIAN_POINT('Ctrl Pts',(-9.99607881100006,15.2,-2.78497028600002));
#268678=CARTESIAN_POINT('Ctrl Pts',(-9.99607881100006,11.6,-2.78497028600002));
#268679=CARTESIAN_POINT('Ctrl Pts',(-9.99536684700006,15.2,-2.78483763500001));
#268680=CARTESIAN_POINT('Ctrl Pts',(-9.99536684700006,11.6,-2.78483763500002));
#268681=CARTESIAN_POINT('Ctrl Pts',(-9.99483840000006,15.2,-2.78473877000001));
#268682=CARTESIAN_POINT('Ctrl Pts',(-9.99483840000006,11.6,-2.78473877000002));
#268683=CARTESIAN_POINT('Ctrl Pts',(-9.99448967800006,15.2,-2.78467334900002));
#268684=CARTESIAN_POINT('Ctrl Pts',(-9.99448967800006,11.6,-2.78467334900002));
#268685=CARTESIAN_POINT('Ctrl Pts',(-9.99431831700005,15.2,-2.78464115900002));
#268686=CARTESIAN_POINT('Ctrl Pts',(-9.99431831700005,11.6,-2.78464115900002));
#268687=CARTESIAN_POINT('',(-9.99431831700005,12.2,-2.78464115900002));
#268688=CARTESIAN_POINT('',(-9.99431831700005,15.2,-2.78464115900002));
#268689=CARTESIAN_POINT('',(-9.99431831700005,12.2,-2.78464115900002));
#268690=CARTESIAN_POINT('Ctrl Pts',(-11.1757778680001,12.2,-2.71145515300002));
#268691=CARTESIAN_POINT('Ctrl Pts',(-11.1750309950001,12.2,-2.71161876900001));
#268692=CARTESIAN_POINT('Ctrl Pts',(-11.1735376180001,12.2,-2.71194562400002));
#268693=CARTESIAN_POINT('Ctrl Pts',(-11.1712986600001,12.2,-2.71243478000001));
#268694=CARTESIAN_POINT('Ctrl Pts',(-11.1683155990001,12.2,-2.71308473500001));
#268695=CARTESIAN_POINT('Ctrl Pts',(-11.1645904650001,12.2,-2.71389342400001));
#268696=CARTESIAN_POINT('Ctrl Pts',(-11.1608690250001,12.2,-2.71469835800001));
#268697=CARTESIAN_POINT('Ctrl Pts',(-11.1571512810001,12.2,-2.71549953800001));
#268698=CARTESIAN_POINT('Ctrl Pts',(-11.1534372360001,12.2,-2.71629696600002));
#268699=CARTESIAN_POINT('Ctrl Pts',(-11.1497268980001,12.2,-2.71709064400001));
#268700=CARTESIAN_POINT('Ctrl Pts',(-11.1460202710001,12.2,-2.71788057600002));
#268701=CARTESIAN_POINT('Ctrl Pts',(-11.1423173660001,12.2,-2.71866676600002));
#268702=CARTESIAN_POINT('Ctrl Pts',(-11.1386181920001,12.2,-2.71944921800001));
#268703=CARTESIAN_POINT('Ctrl Pts',(-11.1349227590001,12.2,-2.72022793900002));
#268704=CARTESIAN_POINT('Ctrl Pts',(-11.1312310760001,12.2,-2.72100293300001));
#268705=CARTESIAN_POINT('Ctrl Pts',(-11.1275431540001,12.2,-2.72177420400002));
#268706=CARTESIAN_POINT('Ctrl Pts',(-11.1238590000001,12.2,-2.72254175700001));
#268707=CARTESIAN_POINT('Ctrl Pts',(-11.1201786230001,12.2,-2.72330559600002));
#268708=CARTESIAN_POINT('Ctrl Pts',(-11.1165020290001,12.2,-2.72406572300001));
#268709=CARTESIAN_POINT('Ctrl Pts',(-11.1128292270001,12.2,-2.72482214500001));
#268710=CARTESIAN_POINT('Ctrl Pts',(-11.1091602230001,12.2,-2.72557486300002));
#268711=CARTESIAN_POINT('Ctrl Pts',(-11.1054950240001,12.2,-2.72632388100002));
#268712=CARTESIAN_POINT('Ctrl Pts',(-11.1018336410001,12.2,-2.72706920300001));
#268713=CARTESIAN_POINT('Ctrl Pts',(-11.0981760790001,12.2,-2.72781083400002));
#268714=CARTESIAN_POINT('Ctrl Pts',(-11.0945223470001,12.2,-2.72854877900001));
#268715=CARTESIAN_POINT('Ctrl Pts',(-11.0908724560001,12.2,-2.72928304000001));
#268716=CARTESIAN_POINT('Ctrl Pts',(-11.0872264110001,12.2,-2.73001362300001));
#268717=CARTESIAN_POINT('Ctrl Pts',(-11.0835842240001,12.2,-2.73074053200002));
#268718=CARTESIAN_POINT('Ctrl Pts',(-11.0799458990001,12.2,-2.73146377200002));
#268719=CARTESIAN_POINT('Ctrl Pts',(-11.0763114490001,12.2,-2.73218334500001));
#268720=CARTESIAN_POINT('Ctrl Pts',(-11.0726808780001,12.2,-2.73289925600002));
#268721=CARTESIAN_POINT('Ctrl Pts',(-11.0690541960001,12.2,-2.73361151100001));
#268722=CARTESIAN_POINT('Ctrl Pts',(-11.0654314110001,12.2,-2.73432011200001));
#268723=CARTESIAN_POINT('Ctrl Pts',(-11.0618125300001,12.2,-2.73502506300002));
#268724=CARTESIAN_POINT('Ctrl Pts',(-11.0581975630001,12.2,-2.73572637000001));
#268725=CARTESIAN_POINT('Ctrl Pts',(-11.0545865170001,12.2,-2.73642403700002));
#268726=CARTESIAN_POINT('Ctrl Pts',(-11.0509794010001,12.2,-2.73711806700002));
#268727=CARTESIAN_POINT('Ctrl Pts',(-11.0473762230001,12.2,-2.73780846600001));
#268728=CARTESIAN_POINT('Ctrl Pts',(-11.0437769920001,12.2,-2.73849523700001));
#268729=CARTESIAN_POINT('Ctrl Pts',(-11.0401817150001,12.2,-2.73917838500001));
#268730=CARTESIAN_POINT('Ctrl Pts',(-11.0365904010001,12.2,-2.73985791400001));
#268731=CARTESIAN_POINT('Ctrl Pts',(-11.0330030590001,12.2,-2.74053382800002));
#268732=CARTESIAN_POINT('Ctrl Pts',(-11.0294196970001,12.2,-2.74120613200001));
#268733=CARTESIAN_POINT('Ctrl Pts',(-11.0258403220001,12.2,-2.74187483000001));
#268734=CARTESIAN_POINT('Ctrl Pts',(-11.0222649450001,12.2,-2.74253992800002));
#268735=CARTESIAN_POINT('Ctrl Pts',(-11.0186935710001,12.2,-2.74320142800001));
#268736=CARTESIAN_POINT('Ctrl Pts',(-11.0151262110001,12.2,-2.74385933600001));
#268737=CARTESIAN_POINT('Ctrl Pts',(-11.0115628720001,12.2,-2.74451365600001));
#268738=CARTESIAN_POINT('Ctrl Pts',(-11.0080035640001,12.2,-2.74516439200001));
#268739=CARTESIAN_POINT('Ctrl Pts',(-11.0044482940001,12.2,-2.74581155000002));
#268740=CARTESIAN_POINT('Ctrl Pts',(-11.0008970700001,12.2,-2.74645513200001));
#268741=CARTESIAN_POINT('Ctrl Pts',(-10.9973499030001,12.2,-2.74709514500001));
#268742=CARTESIAN_POINT('Ctrl Pts',(-10.9938067980001,12.2,-2.74773159100001));
#268743=CARTESIAN_POINT('Ctrl Pts',(-10.9902677660001,12.2,-2.74836447800002));
#268744=CARTESIAN_POINT('Ctrl Pts',(-10.9867328140001,12.2,-2.74899380700001));
#268745=CARTESIAN_POINT('Ctrl Pts',(-10.9832019520001,12.2,-2.74961958600001));
#268746=CARTESIAN_POINT('Ctrl Pts',(-10.9796751870001,12.2,-2.75024181600001));
#268747=CARTESIAN_POINT('Ctrl Pts',(-10.9761525290001,12.2,-2.75086050400001));
#268748=CARTESIAN_POINT('Ctrl Pts',(-10.9726339840001,12.2,-2.75147565300002));
#268749=CARTESIAN_POINT('Ctrl Pts',(-10.9691195640001,12.2,-2.75208727000001));
#268750=CARTESIAN_POINT('Ctrl Pts',(-10.9656092750001,12.2,-2.75269535800001));
#268751=CARTESIAN_POINT('Ctrl Pts',(-10.9621031260001,12.2,-2.75329992100001));
#268752=CARTESIAN_POINT('Ctrl Pts',(-10.9586011260001,12.2,-2.75390096500002));
#268753=CARTESIAN_POINT('Ctrl Pts',(-10.9551032830001,12.2,-2.75449849500002));
#268754=CARTESIAN_POINT('Ctrl Pts',(-10.9516096070001,12.2,-2.75509251400001));
#268755=CARTESIAN_POINT('Ctrl Pts',(-10.9481201050001,12.2,-2.75568302700002));
#268756=CARTESIAN_POINT('Ctrl Pts',(-10.9446347860001,12.2,-2.75627004100001));
#268757=CARTESIAN_POINT('Ctrl Pts',(-10.9411536590001,12.2,-2.75685355800002));
#268758=CARTESIAN_POINT('Ctrl Pts',(-10.9376767320001,12.2,-2.75743358500002));
#268759=CARTESIAN_POINT('Ctrl Pts',(-10.9342040160001,12.2,-2.75801012600001));
#268760=CARTESIAN_POINT('Ctrl Pts',(-10.9307355160001,12.2,-2.75858318400001));
#268761=CARTESIAN_POINT('Ctrl Pts',(-10.9272712420001,12.2,-2.75915276600001));
#268762=CARTESIAN_POINT('Ctrl Pts',(-10.9238112040001,12.2,-2.75971887600001));
#268763=CARTESIAN_POINT('Ctrl Pts',(-10.9203554100001,12.2,-2.76028151900002));
#268764=CARTESIAN_POINT('Ctrl Pts',(-10.9169038680001,12.2,-2.76084070000001));
#268765=CARTESIAN_POINT('Ctrl Pts',(-10.9134565880001,12.2,-2.76139642400001));
#268766=CARTESIAN_POINT('Ctrl Pts',(-10.9100135780001,12.2,-2.76194869600001));
#268767=CARTESIAN_POINT('Ctrl Pts',(-10.9065748460001,12.2,-2.76249752000002));
#268768=CARTESIAN_POINT('Ctrl Pts',(-10.9031404020001,12.2,-2.76304290100001));
#268769=CARTESIAN_POINT('Ctrl Pts',(-10.8997102540001,12.2,-2.76358484600001));
#268770=CARTESIAN_POINT('Ctrl Pts',(-10.8962844110001,12.2,-2.76412335800002));
#268771=CARTESIAN_POINT('Ctrl Pts',(-10.8928628820001,12.2,-2.76465844200001));
#268772=CARTESIAN_POINT('Ctrl Pts',(-10.8894456750001,12.2,-2.76519010300001));
#268773=CARTESIAN_POINT('Ctrl Pts',(-10.8860328000001,12.2,-2.76571834600002));
#268774=CARTESIAN_POINT('Ctrl Pts',(-10.8826242650001,12.2,-2.76624317800001));
#268775=CARTESIAN_POINT('Ctrl Pts',(-10.8792200800001,12.2,-2.76676460200001));
#268776=CARTESIAN_POINT('Ctrl Pts',(-10.8758202520001,12.2,-2.76728262200002));
#268777=CARTESIAN_POINT('Ctrl Pts',(-10.8724247920001,12.2,-2.76779724700001));
#268778=CARTESIAN_POINT('Ctrl Pts',(-10.8690337060001,12.2,-2.76830847900001));
#268779=CARTESIAN_POINT('Ctrl Pts',(-10.8656470060001,12.2,-2.76881632300002));
#268780=CARTESIAN_POINT('Ctrl Pts',(-10.8622646980001,12.2,-2.76932078500002));
#268781=CARTESIAN_POINT('Ctrl Pts',(-10.8588867940001,12.2,-2.76982187100002));
#268782=CARTESIAN_POINT('Ctrl Pts',(-10.8555133010001,12.2,-2.77031958400002));
#268783=CARTESIAN_POINT('Ctrl Pts',(-10.8521442280001,12.2,-2.77081393100001));
#268784=CARTESIAN_POINT('Ctrl Pts',(-10.8487795840001,12.2,-2.77130491700001));
#268785=CARTESIAN_POINT('Ctrl Pts',(-10.8454193790001,12.2,-2.77179254700001));
#268786=CARTESIAN_POINT('Ctrl Pts',(-10.8420636210001,12.2,-2.77227682600001));
#268787=CARTESIAN_POINT('Ctrl Pts',(-10.8387123200001,12.2,-2.77275775900002));
#268788=CARTESIAN_POINT('Ctrl Pts',(-10.8353654830001,12.2,-2.77323535200001));
#268789=CARTESIAN_POINT('Ctrl Pts',(-10.8320231210001,12.2,-2.77370961000001));
#268790=CARTESIAN_POINT('Ctrl Pts',(-10.8286852410001,12.2,-2.77418053700002));
#268791=CARTESIAN_POINT('Ctrl Pts',(-10.8253518550001,12.2,-2.77464814100002));
#268792=CARTESIAN_POINT('Ctrl Pts',(-10.8220229700001,12.2,-2.77511242500001));
#268793=CARTESIAN_POINT('Ctrl Pts',(-10.8186985940001,12.2,-2.77557339600001));
#268794=CARTESIAN_POINT('Ctrl Pts',(-10.8153787400001,12.2,-2.77603105800001));
#268795=CARTESIAN_POINT('Ctrl Pts',(-10.8120634130001,12.2,-2.77648541700001));
#268796=CARTESIAN_POINT('Ctrl Pts',(-10.8087526240001,12.2,-2.77693647800001));
#268797=CARTESIAN_POINT('Ctrl Pts',(-10.8054463820001,12.2,-2.77738424700001));
#268798=CARTESIAN_POINT('Ctrl Pts',(-10.8021446960001,12.2,-2.77782872900001));
#268799=CARTESIAN_POINT('Ctrl Pts',(-10.7988475760001,12.2,-2.77826993000001));
#268800=CARTESIAN_POINT('Ctrl Pts',(-10.7955550300001,12.2,-2.77870785600001));
#268801=CARTESIAN_POINT('Ctrl Pts',(-10.7922670680001,12.2,-2.77914251000002));
#268802=CARTESIAN_POINT('Ctrl Pts',(-10.7889836990001,12.2,-2.77957390000001));
#268803=CARTESIAN_POINT('Ctrl Pts',(-10.7857049310001,12.2,-2.78000203100001));
#268804=CARTESIAN_POINT('Ctrl Pts',(-10.7824307750001,12.2,-2.78042690900001));
#268805=CARTESIAN_POINT('Ctrl Pts',(-10.7791612390001,12.2,-2.78084853700001));
#268806=CARTESIAN_POINT('Ctrl Pts',(-10.7758963330001,12.2,-2.78126692300001));
#268807=CARTESIAN_POINT('Ctrl Pts',(-10.7726360660001,12.2,-2.78168207300002));
#268808=CARTESIAN_POINT('Ctrl Pts',(-10.7693804470001,12.2,-2.78209399100001));
#268809=CARTESIAN_POINT('Ctrl Pts',(-10.7661294860001,12.2,-2.78250268300001));
#268810=CARTESIAN_POINT('Ctrl Pts',(-10.7628831920001,12.2,-2.78290815600001));
#268811=CARTESIAN_POINT('Ctrl Pts',(-10.7596415740001,12.2,-2.78331041300001));
#268812=CARTESIAN_POINT('Ctrl Pts',(-10.7564046420001,12.2,-2.78370946300001));
#268813=CARTESIAN_POINT('Ctrl Pts',(-10.7531724040001,12.2,-2.78410530900001));
#268814=CARTESIAN_POINT('Ctrl Pts',(-10.7499448710001,12.2,-2.78449795800002));
#268815=CARTESIAN_POINT('Ctrl Pts',(-10.7467220520001,12.2,-2.78488741600002));
#268816=CARTESIAN_POINT('Ctrl Pts',(-10.7435039560001,12.2,-2.78527368900002));
#268817=CARTESIAN_POINT('Ctrl Pts',(-10.7402905920001,12.2,-2.78565678100001));
#268818=CARTESIAN_POINT('Ctrl Pts',(-10.7370819700001,12.2,-2.78603669900002));
#268819=CARTESIAN_POINT('Ctrl Pts',(-10.7338780990001,12.2,-2.78641345000001));
#268820=CARTESIAN_POINT('Ctrl Pts',(-10.7306789900001,12.2,-2.78678703700002));
#268821=CARTESIAN_POINT('Ctrl Pts',(-10.7274846510001,12.2,-2.78715746900001));
#268822=CARTESIAN_POINT('Ctrl Pts',(-10.7242950910001,12.2,-2.78752475000001));
#268823=CARTESIAN_POINT('Ctrl Pts',(-10.7211103210001,12.2,-2.78788888700001));
#268824=CARTESIAN_POINT('Ctrl Pts',(-10.7179303500001,12.2,-2.78824988400002));
#268825=CARTESIAN_POINT('Ctrl Pts',(-10.7147551880001,12.2,-2.78860774800001));
#268826=CARTESIAN_POINT('Ctrl Pts',(-10.7115848430001,12.2,-2.78896248700002));
#268827=CARTESIAN_POINT('Ctrl Pts',(-10.7084193250001,12.2,-2.78931410400002));
#268828=CARTESIAN_POINT('Ctrl Pts',(-10.7052586450001,12.2,-2.78966260600002));
#268829=CARTESIAN_POINT('Ctrl Pts',(-10.7021028110001,12.2,-2.79000800100001));
#268830=CARTESIAN_POINT('Ctrl Pts',(-10.6989518340001,12.2,-2.79035029100001));
#268831=CARTESIAN_POINT('Ctrl Pts',(-10.6958057220001,12.2,-2.79068948600001));
#268832=CARTESIAN_POINT('Ctrl Pts',(-10.6926644870001,12.2,-2.79102559000002));
#268833=CARTESIAN_POINT('Ctrl Pts',(-10.6895281350001,12.2,-2.79135861000002));
#268834=CARTESIAN_POINT('Ctrl Pts',(-10.6863966800001,12.2,-2.79168855100002));
#268835=CARTESIAN_POINT('Ctrl Pts',(-10.6832701290001,12.2,-2.79201542000001));
#268836=CARTESIAN_POINT('Ctrl Pts',(-10.6801484920001,12.2,-2.79233922300001));
#268837=CARTESIAN_POINT('Ctrl Pts',(-10.6770317790001,12.2,-2.79265996700001));
#268838=CARTESIAN_POINT('Ctrl Pts',(-10.6739200000001,12.2,-2.79297765700001));
#268839=CARTESIAN_POINT('Ctrl Pts',(-10.6708131640001,12.2,-2.79329230000001));
#268840=CARTESIAN_POINT('Ctrl Pts',(-10.6677112820001,12.2,-2.79360390200001));
#268841=CARTESIAN_POINT('Ctrl Pts',(-10.6646143620001,12.2,-2.79391246900001));
#268842=CARTESIAN_POINT('Ctrl Pts',(-10.6615224160001,12.2,-2.79421800700002));
#268843=CARTESIAN_POINT('Ctrl Pts',(-10.6584354520001,12.2,-2.79452052500002));
#268844=CARTESIAN_POINT('Ctrl Pts',(-10.6553534800001,12.2,-2.79482002500002));
#268845=CARTESIAN_POINT('Ctrl Pts',(-10.6522765120001,12.2,-2.79511651600002));
#268846=CARTESIAN_POINT('Ctrl Pts',(-10.6492045550001,12.2,-2.79541000500001));
#268847=CARTESIAN_POINT('Ctrl Pts',(-10.6461376210001,12.2,-2.79570049800002));
#268848=CARTESIAN_POINT('Ctrl Pts',(-10.6430757180001,12.2,-2.79598800000001));
#268849=CARTESIAN_POINT('Ctrl Pts',(-10.6400188580001,12.2,-2.79627251700001));
#268850=CARTESIAN_POINT('Ctrl Pts',(-10.6369670490001,12.2,-2.79655405800002));
#268851=CARTESIAN_POINT('Ctrl Pts',(-10.6339203020001,12.2,-2.79683262800001));
#268852=CARTESIAN_POINT('Ctrl Pts',(-10.6308786260001,12.2,-2.79710823500002));
#268853=CARTESIAN_POINT('Ctrl Pts',(-10.6278420330001,12.2,-2.79738088400002));
#268854=CARTESIAN_POINT('Ctrl Pts',(-10.6248105320001,12.2,-2.79765058100002));
#268855=CARTESIAN_POINT('Ctrl Pts',(-10.6217841320001,12.2,-2.79791733300002));
#268856=CARTESIAN_POINT('Ctrl Pts',(-10.6187628440001,12.2,-2.79818114900001));
#268857=CARTESIAN_POINT('Ctrl Pts',(-10.6157466780001,12.2,-2.79844203300001));
#268858=CARTESIAN_POINT('Ctrl Pts',(-10.6127356450001,12.2,-2.79869999200002));
#268859=CARTESIAN_POINT('Ctrl Pts',(-10.6097297520001,12.2,-2.79895503300001));
#268860=CARTESIAN_POINT('Ctrl Pts',(-10.6067290130001,12.2,-2.79920716400001));
#268861=CARTESIAN_POINT('Ctrl Pts',(-10.6037334350001,12.2,-2.79945638900001));
#268862=CARTESIAN_POINT('Ctrl Pts',(-10.6007430310001,12.2,-2.79970271700002));
#268863=CARTESIAN_POINT('Ctrl Pts',(-10.5977578070001,12.2,-2.79994615300001));
#268864=CARTESIAN_POINT('Ctrl Pts',(-10.5947777780001,12.2,-2.80018670600001));
#268865=CARTESIAN_POINT('Ctrl Pts',(-10.5918029510001,12.2,-2.80042438200002));
#268866=CARTESIAN_POINT('Ctrl Pts',(-10.5888333380001,12.2,-2.80065918700001));
#268867=CARTESIAN_POINT('Ctrl Pts',(-10.5858689480001,12.2,-2.80089112800002));
#268868=CARTESIAN_POINT('Ctrl Pts',(-10.5829097920001,12.2,-2.80112021200001));
#268869=CARTESIAN_POINT('Ctrl Pts',(-10.5799558780001,12.2,-2.80134644700002));
#268870=CARTESIAN_POINT('Ctrl Pts',(-10.5770072200001,12.2,-2.80156983800001));
#268871=CARTESIAN_POINT('Ctrl Pts',(-10.5740638260001,12.2,-2.80179039400001));
#268872=CARTESIAN_POINT('Ctrl Pts',(-10.5711257080001,12.2,-2.80200812100002));
#268873=CARTESIAN_POINT('Ctrl Pts',(-10.5681928730001,12.2,-2.80222302500002));
#268874=CARTESIAN_POINT('Ctrl Pts',(-10.5652653350001,12.2,-2.80243511500001));
#268875=CARTESIAN_POINT('Ctrl Pts',(-10.5623431030001,12.2,-2.80264439700002));
#268876=CARTESIAN_POINT('Ctrl Pts',(-10.5594261870001,12.2,-2.80285087700001));
#268877=CARTESIAN_POINT('Ctrl Pts',(-10.5565145980001,12.2,-2.80305456500002));
#268878=CARTESIAN_POINT('Ctrl Pts',(-10.5536083460001,12.2,-2.80325546500002));
#268879=CARTESIAN_POINT('Ctrl Pts',(-10.5507074410001,12.2,-2.80345358600002));
#268880=CARTESIAN_POINT('Ctrl Pts',(-10.5478118940001,12.2,-2.80364893500002));
#268881=CARTESIAN_POINT('Ctrl Pts',(-10.5449217170001,12.2,-2.80384151900002));
#268882=CARTESIAN_POINT('Ctrl Pts',(-10.5420369180001,12.2,-2.80403134500002));
#268883=CARTESIAN_POINT('Ctrl Pts',(-10.5391575100001,12.2,-2.80421842000001));
#268884=CARTESIAN_POINT('Ctrl Pts',(-10.5362835010001,12.2,-2.80440275200001));
#268885=CARTESIAN_POINT('Ctrl Pts',(-10.5328411820124,12.2,-2.80462066721189));
#268886=CARTESIAN_POINT('Ctrl Pts',(-10.5294069978379,12.2,-2.80483448890378));
#268887=CARTESIAN_POINT('Ctrl Pts',(-10.5259809641622,12.2,-2.80504423309624));
#268888=CARTESIAN_POINT('Ctrl Pts',(-10.5225631056757,12.2,-2.80524991280756));
#268889=CARTESIAN_POINT('Ctrl Pts',(-10.5191534450001,12.2,-2.80545154400002));
#268890=CARTESIAN_POINT('Ctrl Pts',(-10.5163175340001,12.2,-2.80561687900001));
#268891=CARTESIAN_POINT('Ctrl Pts',(-10.5134871080001,12.2,-2.80577952900002));
#268892=CARTESIAN_POINT('Ctrl Pts',(-10.5106621790001,12.2,-2.80593950300001));
#268893=CARTESIAN_POINT('Ctrl Pts',(-10.5078427570001,12.2,-2.80609680700001));
#268894=CARTESIAN_POINT('Ctrl Pts',(-10.5050288510001,12.2,-2.80625145000001));
#268895=CARTESIAN_POINT('Ctrl Pts',(-10.5022204750001,12.2,-2.80640343900001));
#268896=CARTESIAN_POINT('Ctrl Pts',(-10.4994176380001,12.2,-2.80655278100001));
#268897=CARTESIAN_POINT('Ctrl Pts',(-10.4966203510001,12.2,-2.80669948500002));
#268898=CARTESIAN_POINT('Ctrl Pts',(-10.4938286240001,12.2,-2.80684355700001));
#268899=CARTESIAN_POINT('Ctrl Pts',(-10.4910424700001,12.2,-2.80698500600002));
#268900=CARTESIAN_POINT('Ctrl Pts',(-10.4882618970001,12.2,-2.80712384000001));
#268901=CARTESIAN_POINT('Ctrl Pts',(-10.4854869180001,12.2,-2.80726006400001));
#268902=CARTESIAN_POINT('Ctrl Pts',(-10.4827175440001,12.2,-2.80739369000001));
#268903=CARTESIAN_POINT('Ctrl Pts',(-10.4799537850001,12.2,-2.80752472200001));
#268904=CARTESIAN_POINT('Ctrl Pts',(-10.4771956530001,12.2,-2.80765317100002));
#268905=CARTESIAN_POINT('Ctrl Pts',(-10.4744431570001,12.2,-2.80777904200002));
#268906=CARTESIAN_POINT('Ctrl Pts',(-10.4716963110001,12.2,-2.80790234500001));
#268907=CARTESIAN_POINT('Ctrl Pts',(-10.4689551240001,12.2,-2.80802308700002));
#268908=CARTESIAN_POINT('Ctrl Pts',(-10.4662196070001,12.2,-2.80814127600001));
#268909=CARTESIAN_POINT('Ctrl Pts',(-10.4634897720001,12.2,-2.80825691900001));
#268910=CARTESIAN_POINT('Ctrl Pts',(-10.4607656300001,12.2,-2.80837002600002));
#268911=CARTESIAN_POINT('Ctrl Pts',(-10.4580471910001,12.2,-2.80848060400002));
#268912=CARTESIAN_POINT('Ctrl Pts',(-10.4553344680001,12.2,-2.80858866000001));
#268913=CARTESIAN_POINT('Ctrl Pts',(-10.4526274700001,12.2,-2.80869420500002));
#268914=CARTESIAN_POINT('Ctrl Pts',(-10.4499262110001,12.2,-2.80879724300001));
#268915=CARTESIAN_POINT('Ctrl Pts',(-10.4472306990001,12.2,-2.80889778700002));
#268916=CARTESIAN_POINT('Ctrl Pts',(-10.4445409480001,12.2,-2.80899584100001));
#268917=CARTESIAN_POINT('Ctrl Pts',(-10.4418569680001,12.2,-2.80909141400001));
#268918=CARTESIAN_POINT('Ctrl Pts',(-10.4391787700001,12.2,-2.80918451700002));
#268919=CARTESIAN_POINT('Ctrl Pts',(-10.4365063660001,12.2,-2.80927515500002));
#268920=CARTESIAN_POINT('Ctrl Pts',(-10.4338397670001,12.2,-2.80936333700001));
#268921=CARTESIAN_POINT('Ctrl Pts',(-10.4311789840001,12.2,-2.80944907300002));
#268922=CARTESIAN_POINT('Ctrl Pts',(-10.4285240300001,12.2,-2.80953237000002));
#268923=CARTESIAN_POINT('Ctrl Pts',(-10.4258749130001,12.2,-2.80961323700001));
#268924=CARTESIAN_POINT('Ctrl Pts',(-10.4232316480001,12.2,-2.80969168100001));
#268925=CARTESIAN_POINT('Ctrl Pts',(-10.4205942460001,12.2,-2.80976771100002));
#268926=CARTESIAN_POINT('Ctrl Pts',(-10.4179627160001,12.2,-2.80984133700001));
#268927=CARTESIAN_POINT('Ctrl Pts',(-10.4153370720001,12.2,-2.80991256500001));
#268928=CARTESIAN_POINT('Ctrl Pts',(-10.4127173250001,12.2,-2.80998140700001));
#268929=CARTESIAN_POINT('Ctrl Pts',(-10.4101034850001,12.2,-2.81004786800001));
#268930=CARTESIAN_POINT('Ctrl Pts',(-10.4074955650001,12.2,-2.81011195800001));
#268931=CARTESIAN_POINT('Ctrl Pts',(-10.4048935770001,12.2,-2.81017368600001));
#268932=CARTESIAN_POINT('Ctrl Pts',(-10.4022975320001,12.2,-2.81023306000002));
#268933=CARTESIAN_POINT('Ctrl Pts',(-10.3997074400001,12.2,-2.81029008900001));
#268934=CARTESIAN_POINT('Ctrl Pts',(-10.3971233170001,12.2,-2.81034478200001));
#268935=CARTESIAN_POINT('Ctrl Pts',(-10.3945451690001,12.2,-2.81039714800002));
#268936=CARTESIAN_POINT('Ctrl Pts',(-10.3919730120001,12.2,-2.81044719300001));
#268937=CARTESIAN_POINT('Ctrl Pts',(-10.3894068560001,12.2,-2.81049493000001));
#268938=CARTESIAN_POINT('Ctrl Pts',(-10.3868467140001,12.2,-2.81054036500001));
#268939=CARTESIAN_POINT('Ctrl Pts',(-10.3842925970001,12.2,-2.81058350800001));
#268940=CARTESIAN_POINT('Ctrl Pts',(-10.3817445160001,12.2,-2.81062436900001));
#268941=CARTESIAN_POINT('Ctrl Pts',(-10.3792024840001,12.2,-2.81066295300001));
#268942=CARTESIAN_POINT('Ctrl Pts',(-10.3766665130001,12.2,-2.81069927400001));
#268943=CARTESIAN_POINT('Ctrl Pts',(-10.3741366140001,12.2,-2.81073333600002));
#268944=CARTESIAN_POINT('Ctrl Pts',(-10.3716127990001,12.2,-2.81076515200001));
#268945=CARTESIAN_POINT('Ctrl Pts',(-10.3690950810001,12.2,-2.81079473000001));
#268946=CARTESIAN_POINT('Ctrl Pts',(-10.3665834700001,12.2,-2.81082207900001));
#268947=CARTESIAN_POINT('Ctrl Pts',(-10.3640779820001,12.2,-2.81084720700001));
#268948=CARTESIAN_POINT('Ctrl Pts',(-10.3615786240001,12.2,-2.81087012400001));
#268949=CARTESIAN_POINT('Ctrl Pts',(-10.3590854110001,12.2,-2.81089083900001));
#268950=CARTESIAN_POINT('Ctrl Pts',(-10.3565983540001,12.2,-2.81090936300001));
#268951=CARTESIAN_POINT('Ctrl Pts',(-10.3541174660001,12.2,-2.81092570300002));
#268952=CARTESIAN_POINT('Ctrl Pts',(-10.3516427590001,12.2,-2.81093986800002));
#268953=CARTESIAN_POINT('Ctrl Pts',(-10.3491742450001,12.2,-2.81095186900002));
#268954=CARTESIAN_POINT('Ctrl Pts',(-10.3467119360001,12.2,-2.81096171500002));
#268955=CARTESIAN_POINT('Ctrl Pts',(-10.3442558440001,12.2,-2.81096941500001));
#268956=CARTESIAN_POINT('Ctrl Pts',(-10.3418059810001,12.2,-2.81097497900001));
#268957=CARTESIAN_POINT('Ctrl Pts',(-10.3393623600001,12.2,-2.81097841600001));
#268958=CARTESIAN_POINT('Ctrl Pts',(-10.3369249940001,12.2,-2.81097973500001));
#268959=CARTESIAN_POINT('Ctrl Pts',(-10.3344938940001,12.2,-2.81097894800002));
#268960=CARTESIAN_POINT('Ctrl Pts',(-10.3320690720001,12.2,-2.81097606100001));
#268961=CARTESIAN_POINT('Ctrl Pts',(-10.3296505420001,12.2,-2.81097108600001));
#268962=CARTESIAN_POINT('Ctrl Pts',(-10.3272383160001,12.2,-2.81096403100001));
#268963=CARTESIAN_POINT('Ctrl Pts',(-10.3248324060001,12.2,-2.81095490800002));
#268964=CARTESIAN_POINT('Ctrl Pts',(-10.3224328240001,12.2,-2.81094372600001));
#268965=CARTESIAN_POINT('Ctrl Pts',(-10.3200395830001,12.2,-2.81093049300001));
#268966=CARTESIAN_POINT('Ctrl Pts',(-10.3176526950001,12.2,-2.81091522000001));
#268967=CARTESIAN_POINT('Ctrl Pts',(-10.3152721750001,12.2,-2.81089791800001));
#268968=CARTESIAN_POINT('Ctrl Pts',(-10.3128980330001,12.2,-2.81087859400001));
#268969=CARTESIAN_POINT('Ctrl Pts',(-10.3105302810001,12.2,-2.81085726100001));
#268970=CARTESIAN_POINT('Ctrl Pts',(-10.3081689340001,12.2,-2.81083392700001));
#268971=CARTESIAN_POINT('Ctrl Pts',(-10.3058140040001,12.2,-2.81080860400001));
#268972=CARTESIAN_POINT('Ctrl Pts',(-10.3034655040001,12.2,-2.81078129900001));
#268973=CARTESIAN_POINT('Ctrl Pts',(-10.3011234450001,12.2,-2.81075202400002));
#268974=CARTESIAN_POINT('Ctrl Pts',(-10.2987878420001,12.2,-2.81072079000001));
#268975=CARTESIAN_POINT('Ctrl Pts',(-10.2964587060001,12.2,-2.81068760400002));
#268976=CARTESIAN_POINT('Ctrl Pts',(-10.2941360500001,12.2,-2.81065248000001));
#268977=CARTESIAN_POINT('Ctrl Pts',(-10.2918198870001,12.2,-2.81061542500002));
#268978=CARTESIAN_POINT('Ctrl Pts',(-10.2895102320001,12.2,-2.81057645100002));
#268979=CARTESIAN_POINT('Ctrl Pts',(-10.2872070960001,12.2,-2.81053556800002));
#268980=CARTESIAN_POINT('Ctrl Pts',(-10.2849104920001,12.2,-2.81049278600001));
#268981=CARTESIAN_POINT('Ctrl Pts',(-10.2826204320001,12.2,-2.81044811600001));
#268982=CARTESIAN_POINT('Ctrl Pts',(-10.2803369320001,12.2,-2.81040156800001));
#268983=CARTESIAN_POINT('Ctrl Pts',(-10.2780600020001,12.2,-2.81035315300001));
#268984=CARTESIAN_POINT('Ctrl Pts',(-10.2757896570001,12.2,-2.81030288000002));
#268985=CARTESIAN_POINT('Ctrl Pts',(-10.2735259090001,12.2,-2.81025076200002));
#268986=CARTESIAN_POINT('Ctrl Pts',(-10.2712687710001,12.2,-2.81019680600001));
#268987=CARTESIAN_POINT('Ctrl Pts',(-10.2690182590001,12.2,-2.81014102700002));
#268988=CARTESIAN_POINT('Ctrl Pts',(-10.2667743820001,12.2,-2.81008343100002));
#268989=CARTESIAN_POINT('Ctrl Pts',(-10.2645371560001,12.2,-2.81002403300001));
#268990=CARTESIAN_POINT('Ctrl Pts',(-10.2623065940001,12.2,-2.80996284100001));
#268991=CARTESIAN_POINT('Ctrl Pts',(-10.2600827090001,12.2,-2.80989986700002));
#268992=CARTESIAN_POINT('Ctrl Pts',(-10.2578655120001,12.2,-2.80983512200002));
#268993=CARTESIAN_POINT('Ctrl Pts',(-10.2556550210001,12.2,-2.80976861500001));
#268994=CARTESIAN_POINT('Ctrl Pts',(-10.2534512460001,12.2,-2.80970035900001));
#268995=CARTESIAN_POINT('Ctrl Pts',(-10.2512542030001,12.2,-2.80963036400002));
#268996=CARTESIAN_POINT('Ctrl Pts',(-10.2490639020001,12.2,-2.80955864200001));
#268997=CARTESIAN_POINT('Ctrl Pts',(-10.2468803590001,12.2,-2.80948520200001));
#268998=CARTESIAN_POINT('Ctrl Pts',(-10.2447035880001,12.2,-2.80941005800001));
#268999=CARTESIAN_POINT('Ctrl Pts',(-10.2425336010001,12.2,-2.80933321800001));
#269000=CARTESIAN_POINT('Ctrl Pts',(-10.2403704120001,12.2,-2.80925469500001));
#269001=CARTESIAN_POINT('Ctrl Pts',(-10.2382140350001,12.2,-2.80917450000001));
#269002=CARTESIAN_POINT('Ctrl Pts',(-10.2360644840001,12.2,-2.80909264400002));
#269003=CARTESIAN_POINT('Ctrl Pts',(-10.2339217720001,12.2,-2.80900913800001));
#269004=CARTESIAN_POINT('Ctrl Pts',(-10.2317859140001,12.2,-2.80892399500001));
#269005=CARTESIAN_POINT('Ctrl Pts',(-10.2296569220001,12.2,-2.80883722400001));
#269006=CARTESIAN_POINT('Ctrl Pts',(-10.2275348110001,12.2,-2.80874883800001));
#269007=CARTESIAN_POINT('Ctrl Pts',(-10.2254195960001,12.2,-2.80865884700002));
#269008=CARTESIAN_POINT('Ctrl Pts',(-10.2233112870001,12.2,-2.80856726500001));
#269009=CARTESIAN_POINT('Ctrl Pts',(-10.2212099030001,12.2,-2.80847410200002));
#269010=CARTESIAN_POINT('Ctrl Pts',(-10.2191154540001,12.2,-2.80837937100001));
#269011=CARTESIAN_POINT('Ctrl Pts',(-10.2170279560001,12.2,-2.80828308000002));
#269012=CARTESIAN_POINT('Ctrl Pts',(-10.2149474230001,12.2,-2.80818524500001));
#269013=CARTESIAN_POINT('Ctrl Pts',(-10.2128738680001,12.2,-2.80808587500001));
#269014=CARTESIAN_POINT('Ctrl Pts',(-10.2108073070001,12.2,-2.80798498300001));
#269015=CARTESIAN_POINT('Ctrl Pts',(-10.2087477520001,12.2,-2.80788258200001));
#269016=CARTESIAN_POINT('Ctrl Pts',(-10.2066952180001,12.2,-2.80777868100001));
#269017=CARTESIAN_POINT('Ctrl Pts',(-10.2046497210001,12.2,-2.80767329400001));
#269018=CARTESIAN_POINT('Ctrl Pts',(-10.2026112720001,12.2,-2.80756643300001));
#269019=CARTESIAN_POINT('Ctrl Pts',(-10.2005798890001,12.2,-2.80745810900001));
#269020=CARTESIAN_POINT('Ctrl Pts',(-10.1985555830001,12.2,-2.80734833400002));
#269021=CARTESIAN_POINT('Ctrl Pts',(-10.1965383710001,12.2,-2.80723712200002));
#269022=CARTESIAN_POINT('Ctrl Pts',(-10.1945282670001,12.2,-2.80712448400001));
#269023=CARTESIAN_POINT('Ctrl Pts',(-10.1925252840001,12.2,-2.80701043200001));
#269024=CARTESIAN_POINT('Ctrl Pts',(-10.1905294380001,12.2,-2.80689497800001));
#269025=CARTESIAN_POINT('Ctrl Pts',(-10.1885407420001,12.2,-2.80677813600001));
#269026=CARTESIAN_POINT('Ctrl Pts',(-10.1865592120001,12.2,-2.80665991700001));
#269027=CARTESIAN_POINT('Ctrl Pts',(-10.1845848630001,12.2,-2.80654033300001));
#269028=CARTESIAN_POINT('Ctrl Pts',(-10.1826177100001,12.2,-2.80641939900002));
#269029=CARTESIAN_POINT('Ctrl Pts',(-10.1806577650001,12.2,-2.80629712500001));
#269030=CARTESIAN_POINT('Ctrl Pts',(-10.1787050450001,12.2,-2.80617352500002));
#269031=CARTESIAN_POINT('Ctrl Pts',(-10.1767595650001,12.2,-2.80604861000001));
#269032=CARTESIAN_POINT('Ctrl Pts',(-10.1748213380001,12.2,-2.80592239500002));
#269033=CARTESIAN_POINT('Ctrl Pts',(-10.1728903810001,12.2,-2.80579489000001));
#269034=CARTESIAN_POINT('Ctrl Pts',(-10.1709667090001,12.2,-2.80566611100001));
#269035=CARTESIAN_POINT('Ctrl Pts',(-10.1690503350001,12.2,-2.80553606900002));
#269036=CARTESIAN_POINT('Ctrl Pts',(-10.1671412760001,12.2,-2.80540477800002));
#269037=CARTESIAN_POINT('Ctrl Pts',(-10.1652395470001,12.2,-2.80527224900001));
#269038=CARTESIAN_POINT('Ctrl Pts',(-10.1633451610001,12.2,-2.80513849600001));
#269039=CARTESIAN_POINT('Ctrl Pts',(-10.1614581350001,12.2,-2.80500353400001));
#269040=CARTESIAN_POINT('Ctrl Pts',(-10.1595784840001,12.2,-2.80486737300001));
#269041=CARTESIAN_POINT('Ctrl Pts',(-10.1577062240001,12.2,-2.80473002900001));
#269042=CARTESIAN_POINT('Ctrl Pts',(-10.1558413680001,12.2,-2.80459151300001));
#269043=CARTESIAN_POINT('Ctrl Pts',(-10.1539839340001,12.2,-2.80445183900001));
#269044=CARTESIAN_POINT('Ctrl Pts',(-10.1521339360001,12.2,-2.80431102100001));
#269045=CARTESIAN_POINT('Ctrl Pts',(-10.1502913890001,12.2,-2.80416907300001));
#269046=CARTESIAN_POINT('Ctrl Pts',(-10.1484563090001,12.2,-2.80402600700001));
#269047=CARTESIAN_POINT('Ctrl Pts',(-10.1466287130001,12.2,-2.80388183700001));
#269048=CARTESIAN_POINT('Ctrl Pts',(-10.1448086140001,12.2,-2.80373657700002));
#269049=CARTESIAN_POINT('Ctrl Pts',(-10.1429960300001,12.2,-2.80359024000001));
#269050=CARTESIAN_POINT('Ctrl Pts',(-10.1411909760001,12.2,-2.80344284000002));
#269051=CARTESIAN_POINT('Ctrl Pts',(-10.1393934660001,12.2,-2.80329439100001));
#269052=CARTESIAN_POINT('Ctrl Pts',(-10.1376035180001,12.2,-2.80314490700002));
#269053=CARTESIAN_POINT('Ctrl Pts',(-10.1358211480001,12.2,-2.80299440200002));
#269054=CARTESIAN_POINT('Ctrl Pts',(-10.1340463700001,12.2,-2.80284288800001));
#269055=CARTESIAN_POINT('Ctrl Pts',(-10.1322792010001,12.2,-2.80269038200001));
#269056=CARTESIAN_POINT('Ctrl Pts',(-10.1305196570001,12.2,-2.80253689600002));
#269057=CARTESIAN_POINT('Ctrl Pts',(-10.1287677530001,12.2,-2.80238244500001));
#269058=CARTESIAN_POINT('Ctrl Pts',(-10.1270235070001,12.2,-2.80222704300002));
#269059=CARTESIAN_POINT('Ctrl Pts',(-10.1252869340001,12.2,-2.80207070400001));
#269060=CARTESIAN_POINT('Ctrl Pts',(-10.1235580500001,12.2,-2.80191344300002));
#269061=CARTESIAN_POINT('Ctrl Pts',(-10.1218368710001,12.2,-2.80175527400001));
#269062=CARTESIAN_POINT('Ctrl Pts',(-10.1201234150001,12.2,-2.80159621100001));
#269063=CARTESIAN_POINT('Ctrl Pts',(-10.1184176970001,12.2,-2.80143626900001));
#269064=CARTESIAN_POINT('Ctrl Pts',(-10.1167197340001,12.2,-2.80127546300001));
#269065=CARTESIAN_POINT('Ctrl Pts',(-10.1150295420001,12.2,-2.80111380600002));
#269066=CARTESIAN_POINT('Ctrl Pts',(-10.1133471370001,12.2,-2.80095131400001));
#269067=CARTESIAN_POINT('Ctrl Pts',(-10.1116725360001,12.2,-2.80078800200001));
#269068=CARTESIAN_POINT('Ctrl Pts',(-10.1100057560001,12.2,-2.80062388500002));
#269069=CARTESIAN_POINT('Ctrl Pts',(-10.1083468140001,12.2,-2.80045897600001));
#269070=CARTESIAN_POINT('Ctrl Pts',(-10.1066957250001,12.2,-2.80029329300001));
#269071=CARTESIAN_POINT('Ctrl Pts',(-10.1050525090001,12.2,-2.80012684900001));
#269072=CARTESIAN_POINT('Ctrl Pts',(-10.1034171790001,12.2,-2.79995965800001));
#269073=CARTESIAN_POINT('Ctrl Pts',(-10.1017897540001,12.2,-2.79979173800001));
#269074=CARTESIAN_POINT('Ctrl Pts',(-10.1001702510001,12.2,-2.79962310200002));
#269075=CARTESIAN_POINT('Ctrl Pts',(-10.0985586870001,12.2,-2.79945376700002));
#269076=CARTESIAN_POINT('Ctrl Pts',(-10.0969550780001,12.2,-2.79928374700001));
#269077=CARTESIAN_POINT('Ctrl Pts',(-10.0953594420001,12.2,-2.79911305800002));
#269078=CARTESIAN_POINT('Ctrl Pts',(-10.0937717960001,12.2,-2.79894171500001));
#269079=CARTESIAN_POINT('Ctrl Pts',(-10.0921921570001,12.2,-2.79876973500001));
#269080=CARTESIAN_POINT('Ctrl Pts',(-10.0906205420001,12.2,-2.79859713200001));
#269081=CARTESIAN_POINT('Ctrl Pts',(-10.0890569700001,12.2,-2.79842392300001));
#269082=CARTESIAN_POINT('Ctrl Pts',(-10.0875014570001,12.2,-2.79825012400002));
#269083=CARTESIAN_POINT('Ctrl Pts',(-10.0859540200001,12.2,-2.79807574900001));
#269084=CARTESIAN_POINT('Ctrl Pts',(-10.0844146780001,12.2,-2.79790081600002));
#269085=CARTESIAN_POINT('Ctrl Pts',(-10.0828834480001,12.2,-2.79772534000001));
#269086=CARTESIAN_POINT('Ctrl Pts',(-10.0813603480001,12.2,-2.79754933600001));
#269087=CARTESIAN_POINT('Ctrl Pts',(-10.0798453950001,12.2,-2.79737282200001));
#269088=CARTESIAN_POINT('Ctrl Pts',(-10.0783386060001,12.2,-2.79719581400002));
#269089=CARTESIAN_POINT('Ctrl Pts',(-10.0768400010001,12.2,-2.79701832800002));
#269090=CARTESIAN_POINT('Ctrl Pts',(-10.0753495960001,12.2,-2.79684038000001));
#269091=CARTESIAN_POINT('Ctrl Pts',(-10.0738674120001,12.2,-2.79666198700002));
#269092=CARTESIAN_POINT('Ctrl Pts',(-10.0723934620001,12.2,-2.79648316500001));
#269093=CARTESIAN_POINT('Ctrl Pts',(-10.0709277690001,12.2,-2.79630393100001));
#269094=CARTESIAN_POINT('Ctrl Pts',(-10.0694703480001,12.2,-2.79612430200002));
#269095=CARTESIAN_POINT('Ctrl Pts',(-10.0680212180001,12.2,-2.79594429400001));
#269096=CARTESIAN_POINT('Ctrl Pts',(-10.0665803990001,12.2,-2.79576392500001));
#269097=CARTESIAN_POINT('Ctrl Pts',(-10.0651479080001,12.2,-2.79558321000001));
#269098=CARTESIAN_POINT('Ctrl Pts',(-10.0637237620001,12.2,-2.79540216900001));
#269099=CARTESIAN_POINT('Ctrl Pts',(-10.0623079820001,12.2,-2.79522081700001));
#269100=CARTESIAN_POINT('Ctrl Pts',(-10.0609005850001,12.2,-2.79503917100001));
#269101=CARTESIAN_POINT('Ctrl Pts',(-10.0595015910001,12.2,-2.79485724800002));
#269102=CARTESIAN_POINT('Ctrl Pts',(-10.0581110160001,12.2,-2.79467506700001));
#269103=CARTESIAN_POINT('Ctrl Pts',(-10.0567288820001,12.2,-2.79449264500002));
#269104=CARTESIAN_POINT('Ctrl Pts',(-10.0553552060001,12.2,-2.79430999900002));
#269105=CARTESIAN_POINT('Ctrl Pts',(-10.0539900080001,12.2,-2.79412714600001));
#269106=CARTESIAN_POINT('Ctrl Pts',(-10.0526333070001,12.2,-2.79394410600001));
#269107=CARTESIAN_POINT('Ctrl Pts',(-10.0512851200001,12.2,-2.79376089400001));
#269108=CARTESIAN_POINT('Ctrl Pts',(-10.0499454690001,12.2,-2.79357752900002));
#269109=CARTESIAN_POINT('Ctrl Pts',(-10.0486143700001,12.2,-2.79339402900002));
#269110=CARTESIAN_POINT('Ctrl Pts',(-10.0472918460001,12.2,-2.79321041100001));
#269111=CARTESIAN_POINT('Ctrl Pts',(-10.0459779130001,12.2,-2.79302669500002));
#269112=CARTESIAN_POINT('Ctrl Pts',(-10.0446725930001,12.2,-2.79284289900001));
#269113=CARTESIAN_POINT('Ctrl Pts',(-10.0433759040001,12.2,-2.79265904000002));
#269114=CARTESIAN_POINT('Ctrl Pts',(-10.0420878650001,12.2,-2.79247513800001));
#269115=CARTESIAN_POINT('Ctrl Pts',(-10.0408084970001,12.2,-2.79229120900002));
#269116=CARTESIAN_POINT('Ctrl Pts',(-10.0395378210001,12.2,-2.79210727300002));
#269117=CARTESIAN_POINT('Ctrl Pts',(-10.0382758530001,12.2,-2.79192335000001));
#269118=CARTESIAN_POINT('Ctrl Pts',(-10.0370226160001,12.2,-2.79173945600002));
#269119=CARTESIAN_POINT('Ctrl Pts',(-10.0357781300001,12.2,-2.79155561300001));
#269120=CARTESIAN_POINT('Ctrl Pts',(-10.0345424120001,12.2,-2.79137183600001));
#269121=CARTESIAN_POINT('Ctrl Pts',(-10.0333154850001,12.2,-2.79118814800002));
#269122=CARTESIAN_POINT('Ctrl Pts',(-10.0320973690001,12.2,-2.79100456500001));
#269123=CARTESIAN_POINT('Ctrl Pts',(-10.0308880840001,12.2,-2.79082110900001));
#269124=CARTESIAN_POINT('Ctrl Pts',(-10.0296876490001,12.2,-2.79063779700001));
#269125=CARTESIAN_POINT('Ctrl Pts',(-10.0284960860001,12.2,-2.79045465000001));
#269126=CARTESIAN_POINT('Ctrl Pts',(-10.0273134150001,12.2,-2.79027168600001));
#269127=CARTESIAN_POINT('Ctrl Pts',(-10.0261396570001,12.2,-2.79008892600002));
#269128=CARTESIAN_POINT('Ctrl Pts',(-10.0249748320001,12.2,-2.78990638900002));
#269129=CARTESIAN_POINT('Ctrl Pts',(-10.0238189610001,12.2,-2.78972409500001));
#269130=CARTESIAN_POINT('Ctrl Pts',(-10.0226720660001,12.2,-2.78954206400002));
#269131=CARTESIAN_POINT('Ctrl Pts',(-10.0215341660001,12.2,-2.78936031700002));
#269132=CARTESIAN_POINT('Ctrl Pts',(-10.0204052840001,12.2,-2.78917887200001));
#269133=CARTESIAN_POINT('Ctrl Pts',(-10.0192854400001,12.2,-2.78899774900002));
#269134=CARTESIAN_POINT('Ctrl Pts',(-10.0181746550001,12.2,-2.78881697100001));
#269135=CARTESIAN_POINT('Ctrl Pts',(-10.0170729510001,12.2,-2.78863655800001));
#269136=CARTESIAN_POINT('Ctrl Pts',(-10.0159803500001,12.2,-2.78845652900001));
#269137=CARTESIAN_POINT('Ctrl Pts',(-10.0148968710001,12.2,-2.78827690400002));
#269138=CARTESIAN_POINT('Ctrl Pts',(-10.0138225390001,12.2,-2.78809770600001));
#269139=CARTESIAN_POINT('Ctrl Pts',(-10.0127573730001,12.2,-2.78791895500001));
#269140=CARTESIAN_POINT('Ctrl Pts',(-10.0117013970001,12.2,-2.78774067200001));
#269141=CARTESIAN_POINT('Ctrl Pts',(-10.0106546300001,12.2,-2.78756287700002));
#269142=CARTESIAN_POINT('Ctrl Pts',(-10.0096170970001,12.2,-2.78738559300002));
#269143=CARTESIAN_POINT('Ctrl Pts',(-10.0085888180001,12.2,-2.78720884000002));
#269144=CARTESIAN_POINT('Ctrl Pts',(-10.0075698160001,12.2,-2.78703264000002));
#269145=CARTESIAN_POINT('Ctrl Pts',(-10.0065601130001,12.2,-2.78685701400001));
#269146=CARTESIAN_POINT('Ctrl Pts',(-10.0055597320001,12.2,-2.78668198500001));
#269147=CARTESIAN_POINT('Ctrl Pts',(-10.0045686950001,12.2,-2.78650757300001));
#269148=CARTESIAN_POINT('Ctrl Pts',(-10.0035870240001,12.2,-2.78633380100001));
#269149=CARTESIAN_POINT('Ctrl Pts',(-10.0026147430001,12.2,-2.78616069100002));
#269150=CARTESIAN_POINT('Ctrl Pts',(-10.0016518730001,12.2,-2.78598826400001));
#269151=CARTESIAN_POINT('Ctrl Pts',(-10.0006984370001,12.2,-2.78581654400002));
#269152=CARTESIAN_POINT('Ctrl Pts',(-9.99975446000006,12.2,-2.78564555200001));
#269153=CARTESIAN_POINT('Ctrl Pts',(-9.99881996400006,12.2,-2.78547531100001));
#269154=CARTESIAN_POINT('Ctrl Pts',(-9.99789497300006,12.2,-2.78530584400002));
#269155=CARTESIAN_POINT('Ctrl Pts',(-9.99697950700006,12.2,-2.78513717200001));
#269156=CARTESIAN_POINT('Ctrl Pts',(-9.99607881100006,12.2,-2.78497028600002));
#269157=CARTESIAN_POINT('Ctrl Pts',(-9.99536684700006,12.2,-2.78483763500001));
#269158=CARTESIAN_POINT('Ctrl Pts',(-9.99483840000006,12.2,-2.78473877000001));
#269159=CARTESIAN_POINT('Ctrl Pts',(-9.99448967700006,12.2,-2.78467334900002));
#269160=CARTESIAN_POINT('Ctrl Pts',(-9.99431831700005,12.2,-2.78464115900002));
#269161=CARTESIAN_POINT('Ctrl Pts',(-9.99431831700005,15.2,-2.78464115900002));
#269162=CARTESIAN_POINT('Ctrl Pts',(-9.99448967700006,15.2,-2.78467334900002));
#269163=CARTESIAN_POINT('Ctrl Pts',(-9.99483840000006,15.2,-2.78473877000001));
#269164=CARTESIAN_POINT('Ctrl Pts',(-9.99536684700006,15.2,-2.78483763500001));
#269165=CARTESIAN_POINT('Ctrl Pts',(-9.99607881100006,15.2,-2.78497028600002));
#269166=CARTESIAN_POINT('Ctrl Pts',(-9.99697950700006,15.2,-2.78513717200001));
#269167=CARTESIAN_POINT('Ctrl Pts',(-9.99789497300006,15.2,-2.78530584400002));
#269168=CARTESIAN_POINT('Ctrl Pts',(-9.99881996400006,15.2,-2.78547531100001));
#269169=CARTESIAN_POINT('Ctrl Pts',(-9.99975446000006,15.2,-2.78564555200001));
#269170=CARTESIAN_POINT('Ctrl Pts',(-10.0006984370001,15.2,-2.78581654400002));
#269171=CARTESIAN_POINT('Ctrl Pts',(-10.0016518730001,15.2,-2.78598826400001));
#269172=CARTESIAN_POINT('Ctrl Pts',(-10.0026147430001,15.2,-2.78616069100002));
#269173=CARTESIAN_POINT('Ctrl Pts',(-10.0035870240001,15.2,-2.78633380100001));
#269174=CARTESIAN_POINT('Ctrl Pts',(-10.0045686950001,15.2,-2.78650757300001));
#269175=CARTESIAN_POINT('Ctrl Pts',(-10.0055597320001,15.2,-2.78668198500001));
#269176=CARTESIAN_POINT('Ctrl Pts',(-10.0065601130001,15.2,-2.78685701400001));
#269177=CARTESIAN_POINT('Ctrl Pts',(-10.0075698160001,15.2,-2.78703264000002));
#269178=CARTESIAN_POINT('Ctrl Pts',(-10.0085888180001,15.2,-2.78720884000002));
#269179=CARTESIAN_POINT('Ctrl Pts',(-10.0096170970001,15.2,-2.78738559300002));
#269180=CARTESIAN_POINT('Ctrl Pts',(-10.0106546300001,15.2,-2.78756287700002));
#269181=CARTESIAN_POINT('Ctrl Pts',(-10.0117013970001,15.2,-2.78774067200001));
#269182=CARTESIAN_POINT('Ctrl Pts',(-10.0127573730001,15.2,-2.78791895500001));
#269183=CARTESIAN_POINT('Ctrl Pts',(-10.0138225390001,15.2,-2.78809770600001));
#269184=CARTESIAN_POINT('Ctrl Pts',(-10.0148968710001,15.2,-2.78827690400002));
#269185=CARTESIAN_POINT('Ctrl Pts',(-10.0159803500001,15.2,-2.78845652900001));
#269186=CARTESIAN_POINT('Ctrl Pts',(-10.0170729510001,15.2,-2.78863655800001));
#269187=CARTESIAN_POINT('Ctrl Pts',(-10.0181746550001,15.2,-2.78881697100001));
#269188=CARTESIAN_POINT('Ctrl Pts',(-10.0192854400001,15.2,-2.78899774900002));
#269189=CARTESIAN_POINT('Ctrl Pts',(-10.0204052840001,15.2,-2.78917887200001));
#269190=CARTESIAN_POINT('Ctrl Pts',(-10.0215341660001,15.2,-2.78936031700002));
#269191=CARTESIAN_POINT('Ctrl Pts',(-10.0226720660001,15.2,-2.78954206400002));
#269192=CARTESIAN_POINT('Ctrl Pts',(-10.0238189610001,15.2,-2.78972409500001));
#269193=CARTESIAN_POINT('Ctrl Pts',(-10.0249748320001,15.2,-2.78990638900002));
#269194=CARTESIAN_POINT('Ctrl Pts',(-10.0261396570001,15.2,-2.79008892600002));
#269195=CARTESIAN_POINT('Ctrl Pts',(-10.0273134150001,15.2,-2.79027168600001));
#269196=CARTESIAN_POINT('Ctrl Pts',(-10.0284960860001,15.2,-2.79045465000001));
#269197=CARTESIAN_POINT('Ctrl Pts',(-10.0296876490001,15.2,-2.79063779700001));
#269198=CARTESIAN_POINT('Ctrl Pts',(-10.0308880840001,15.2,-2.79082110900001));
#269199=CARTESIAN_POINT('Ctrl Pts',(-10.0320973690001,15.2,-2.79100456500001));
#269200=CARTESIAN_POINT('Ctrl Pts',(-10.0333154850001,15.2,-2.79118814800002));
#269201=CARTESIAN_POINT('Ctrl Pts',(-10.0345424120001,15.2,-2.79137183600001));
#269202=CARTESIAN_POINT('Ctrl Pts',(-10.0357781300001,15.2,-2.79155561300001));
#269203=CARTESIAN_POINT('Ctrl Pts',(-10.0370226160001,15.2,-2.79173945600002));
#269204=CARTESIAN_POINT('Ctrl Pts',(-10.0382758530001,15.2,-2.79192335000001));
#269205=CARTESIAN_POINT('Ctrl Pts',(-10.0395378210001,15.2,-2.79210727300002));
#269206=CARTESIAN_POINT('Ctrl Pts',(-10.0408084970001,15.2,-2.79229120900002));
#269207=CARTESIAN_POINT('Ctrl Pts',(-10.0420878650001,15.2,-2.79247513800001));
#269208=CARTESIAN_POINT('Ctrl Pts',(-10.0433759040001,15.2,-2.79265904000002));
#269209=CARTESIAN_POINT('Ctrl Pts',(-10.0446725930001,15.2,-2.79284289900001));
#269210=CARTESIAN_POINT('Ctrl Pts',(-10.0459779130001,15.2,-2.79302669500002));
#269211=CARTESIAN_POINT('Ctrl Pts',(-10.0472918460001,15.2,-2.79321041100001));
#269212=CARTESIAN_POINT('Ctrl Pts',(-10.0486143700001,15.2,-2.79339402900002));
#269213=CARTESIAN_POINT('Ctrl Pts',(-10.0499454690001,15.2,-2.79357752900002));
#269214=CARTESIAN_POINT('Ctrl Pts',(-10.0512851200001,15.2,-2.79376089400001));
#269215=CARTESIAN_POINT('Ctrl Pts',(-10.0526333070001,15.2,-2.79394410600001));
#269216=CARTESIAN_POINT('Ctrl Pts',(-10.0539900080001,15.2,-2.79412714600001));
#269217=CARTESIAN_POINT('Ctrl Pts',(-10.0553552060001,15.2,-2.79430999900002));
#269218=CARTESIAN_POINT('Ctrl Pts',(-10.0567288820001,15.2,-2.79449264500002));
#269219=CARTESIAN_POINT('Ctrl Pts',(-10.0581110160001,15.2,-2.79467506700001));
#269220=CARTESIAN_POINT('Ctrl Pts',(-10.0595015910001,15.2,-2.79485724800002));
#269221=CARTESIAN_POINT('Ctrl Pts',(-10.0609005850001,15.2,-2.79503917100001));
#269222=CARTESIAN_POINT('Ctrl Pts',(-10.0623079820001,15.2,-2.79522081700001));
#269223=CARTESIAN_POINT('Ctrl Pts',(-10.0637237620001,15.2,-2.79540216900001));
#269224=CARTESIAN_POINT('Ctrl Pts',(-10.0651479080001,15.2,-2.79558321000001));
#269225=CARTESIAN_POINT('Ctrl Pts',(-10.0665803990001,15.2,-2.79576392500001));
#269226=CARTESIAN_POINT('Ctrl Pts',(-10.0680212180001,15.2,-2.79594429400001));
#269227=CARTESIAN_POINT('Ctrl Pts',(-10.0694703480001,15.2,-2.79612430200002));
#269228=CARTESIAN_POINT('Ctrl Pts',(-10.0709277690001,15.2,-2.79630393100001));
#269229=CARTESIAN_POINT('Ctrl Pts',(-10.0723934620001,15.2,-2.79648316500001));
#269230=CARTESIAN_POINT('Ctrl Pts',(-10.0738674120001,15.2,-2.79666198700002));
#269231=CARTESIAN_POINT('Ctrl Pts',(-10.0753495960001,15.2,-2.79684038000001));
#269232=CARTESIAN_POINT('Ctrl Pts',(-10.0768400010001,15.2,-2.79701832800002));
#269233=CARTESIAN_POINT('Ctrl Pts',(-10.0783386060001,15.2,-2.79719581400002));
#269234=CARTESIAN_POINT('Ctrl Pts',(-10.0798453950001,15.2,-2.79737282200001));
#269235=CARTESIAN_POINT('Ctrl Pts',(-10.0813603480001,15.2,-2.79754933600001));
#269236=CARTESIAN_POINT('Ctrl Pts',(-10.0828834480001,15.2,-2.79772534000001));
#269237=CARTESIAN_POINT('Ctrl Pts',(-10.0844146780001,15.2,-2.79790081600002));
#269238=CARTESIAN_POINT('Ctrl Pts',(-10.0859540200001,15.2,-2.79807574900001));
#269239=CARTESIAN_POINT('Ctrl Pts',(-10.0875014570001,15.2,-2.79825012400002));
#269240=CARTESIAN_POINT('Ctrl Pts',(-10.0890569700001,15.2,-2.79842392300001));
#269241=CARTESIAN_POINT('Ctrl Pts',(-10.0906205420001,15.2,-2.79859713200001));
#269242=CARTESIAN_POINT('Ctrl Pts',(-10.0921921570001,15.2,-2.79876973500001));
#269243=CARTESIAN_POINT('Ctrl Pts',(-10.0937717960001,15.2,-2.79894171500001));
#269244=CARTESIAN_POINT('Ctrl Pts',(-10.0953594420001,15.2,-2.79911305800002));
#269245=CARTESIAN_POINT('Ctrl Pts',(-10.0969550780001,15.2,-2.79928374700001));
#269246=CARTESIAN_POINT('Ctrl Pts',(-10.0985586870001,15.2,-2.79945376700002));
#269247=CARTESIAN_POINT('Ctrl Pts',(-10.1001702510001,15.2,-2.79962310200002));
#269248=CARTESIAN_POINT('Ctrl Pts',(-10.1017897540001,15.2,-2.79979173800001));
#269249=CARTESIAN_POINT('Ctrl Pts',(-10.1034171790001,15.2,-2.79995965800001));
#269250=CARTESIAN_POINT('Ctrl Pts',(-10.1050525090001,15.2,-2.80012684900001));
#269251=CARTESIAN_POINT('Ctrl Pts',(-10.1066957250001,15.2,-2.80029329300001));
#269252=CARTESIAN_POINT('Ctrl Pts',(-10.1083468140001,15.2,-2.80045897600001));
#269253=CARTESIAN_POINT('Ctrl Pts',(-10.1100057560001,15.2,-2.80062388500002));
#269254=CARTESIAN_POINT('Ctrl Pts',(-10.1116725360001,15.2,-2.80078800200001));
#269255=CARTESIAN_POINT('Ctrl Pts',(-10.1133471370001,15.2,-2.80095131400001));
#269256=CARTESIAN_POINT('Ctrl Pts',(-10.1150295420001,15.2,-2.80111380600002));
#269257=CARTESIAN_POINT('Ctrl Pts',(-10.1167197340001,15.2,-2.80127546300001));
#269258=CARTESIAN_POINT('Ctrl Pts',(-10.1184176970001,15.2,-2.80143626900001));
#269259=CARTESIAN_POINT('Ctrl Pts',(-10.1201234150001,15.2,-2.80159621100001));
#269260=CARTESIAN_POINT('Ctrl Pts',(-10.1218368710001,15.2,-2.80175527400001));
#269261=CARTESIAN_POINT('Ctrl Pts',(-10.1235580500001,15.2,-2.80191344300002));
#269262=CARTESIAN_POINT('Ctrl Pts',(-10.1252869340001,15.2,-2.80207070400001));
#269263=CARTESIAN_POINT('Ctrl Pts',(-10.1270235070001,15.2,-2.80222704300002));
#269264=CARTESIAN_POINT('Ctrl Pts',(-10.1287677530001,15.2,-2.80238244500001));
#269265=CARTESIAN_POINT('Ctrl Pts',(-10.1305196570001,15.2,-2.80253689600002));
#269266=CARTESIAN_POINT('Ctrl Pts',(-10.1322792010001,15.2,-2.80269038200001));
#269267=CARTESIAN_POINT('Ctrl Pts',(-10.1340463700001,15.2,-2.80284288800001));
#269268=CARTESIAN_POINT('Ctrl Pts',(-10.1358211480001,15.2,-2.80299440200002));
#269269=CARTESIAN_POINT('Ctrl Pts',(-10.1376035180001,15.2,-2.80314490700002));
#269270=CARTESIAN_POINT('Ctrl Pts',(-10.1393934660001,15.2,-2.80329439100001));
#269271=CARTESIAN_POINT('Ctrl Pts',(-10.1411909760001,15.2,-2.80344284000002));
#269272=CARTESIAN_POINT('Ctrl Pts',(-10.1429960300001,15.2,-2.80359024000001));
#269273=CARTESIAN_POINT('Ctrl Pts',(-10.1448086140001,15.2,-2.80373657700002));
#269274=CARTESIAN_POINT('Ctrl Pts',(-10.1466287130001,15.2,-2.80388183700001));
#269275=CARTESIAN_POINT('Ctrl Pts',(-10.1484563090001,15.2,-2.80402600700001));
#269276=CARTESIAN_POINT('Ctrl Pts',(-10.1502913890001,15.2,-2.80416907300001));
#269277=CARTESIAN_POINT('Ctrl Pts',(-10.1521339360001,15.2,-2.80431102100001));
#269278=CARTESIAN_POINT('Ctrl Pts',(-10.1539839340001,15.2,-2.80445183900001));
#269279=CARTESIAN_POINT('Ctrl Pts',(-10.1558413680001,15.2,-2.80459151300001));
#269280=CARTESIAN_POINT('Ctrl Pts',(-10.1577062240001,15.2,-2.80473002900001));
#269281=CARTESIAN_POINT('Ctrl Pts',(-10.1595784840001,15.2,-2.80486737300001));
#269282=CARTESIAN_POINT('Ctrl Pts',(-10.1614581350001,15.2,-2.80500353400001));
#269283=CARTESIAN_POINT('Ctrl Pts',(-10.1633451610001,15.2,-2.80513849600001));
#269284=CARTESIAN_POINT('Ctrl Pts',(-10.1652395470001,15.2,-2.80527224900001));
#269285=CARTESIAN_POINT('Ctrl Pts',(-10.1671412760001,15.2,-2.80540477800002));
#269286=CARTESIAN_POINT('Ctrl Pts',(-10.1690503350001,15.2,-2.80553606900002));
#269287=CARTESIAN_POINT('Ctrl Pts',(-10.1709667090001,15.2,-2.80566611100001));
#269288=CARTESIAN_POINT('Ctrl Pts',(-10.1728903810001,15.2,-2.80579489000001));
#269289=CARTESIAN_POINT('Ctrl Pts',(-10.1748213380001,15.2,-2.80592239500002));
#269290=CARTESIAN_POINT('Ctrl Pts',(-10.1767595650001,15.2,-2.80604861000001));
#269291=CARTESIAN_POINT('Ctrl Pts',(-10.1787050450001,15.2,-2.80617352500002));
#269292=CARTESIAN_POINT('Ctrl Pts',(-10.1806577650001,15.2,-2.80629712500001));
#269293=CARTESIAN_POINT('Ctrl Pts',(-10.1826177100001,15.2,-2.80641939900002));
#269294=CARTESIAN_POINT('Ctrl Pts',(-10.1845848630001,15.2,-2.80654033300001));
#269295=CARTESIAN_POINT('Ctrl Pts',(-10.1865592120001,15.2,-2.80665991700001));
#269296=CARTESIAN_POINT('Ctrl Pts',(-10.1885407420001,15.2,-2.80677813600001));
#269297=CARTESIAN_POINT('Ctrl Pts',(-10.1905294380001,15.2,-2.80689497800001));
#269298=CARTESIAN_POINT('Ctrl Pts',(-10.1925252840001,15.2,-2.80701043200001));
#269299=CARTESIAN_POINT('Ctrl Pts',(-10.1945282670001,15.2,-2.80712448400001));
#269300=CARTESIAN_POINT('Ctrl Pts',(-10.1965383710001,15.2,-2.80723712200002));
#269301=CARTESIAN_POINT('Ctrl Pts',(-10.1985555830001,15.2,-2.80734833400002));
#269302=CARTESIAN_POINT('Ctrl Pts',(-10.2005798890001,15.2,-2.80745810900001));
#269303=CARTESIAN_POINT('Ctrl Pts',(-10.2026112720001,15.2,-2.80756643300001));
#269304=CARTESIAN_POINT('Ctrl Pts',(-10.2046497210001,15.2,-2.80767329400001));
#269305=CARTESIAN_POINT('Ctrl Pts',(-10.2066952180001,15.2,-2.80777868100001));
#269306=CARTESIAN_POINT('Ctrl Pts',(-10.2087477520001,15.2,-2.80788258200001));
#269307=CARTESIAN_POINT('Ctrl Pts',(-10.2108073070001,15.2,-2.80798498300001));
#269308=CARTESIAN_POINT('Ctrl Pts',(-10.2128738680001,15.2,-2.80808587500001));
#269309=CARTESIAN_POINT('Ctrl Pts',(-10.2149474230001,15.2,-2.80818524500001));
#269310=CARTESIAN_POINT('Ctrl Pts',(-10.2170279560001,15.2,-2.80828308000002));
#269311=CARTESIAN_POINT('Ctrl Pts',(-10.2191154540001,15.2,-2.80837937100001));
#269312=CARTESIAN_POINT('Ctrl Pts',(-10.2212099030001,15.2,-2.80847410200002));
#269313=CARTESIAN_POINT('Ctrl Pts',(-10.2233112870001,15.2,-2.80856726500001));
#269314=CARTESIAN_POINT('Ctrl Pts',(-10.2254195960001,15.2,-2.80865884700002));
#269315=CARTESIAN_POINT('Ctrl Pts',(-10.2275348110001,15.2,-2.80874883800001));
#269316=CARTESIAN_POINT('Ctrl Pts',(-10.2296569220001,15.2,-2.80883722400001));
#269317=CARTESIAN_POINT('Ctrl Pts',(-10.2317859140001,15.2,-2.80892399500001));
#269318=CARTESIAN_POINT('Ctrl Pts',(-10.2339217720001,15.2,-2.80900913800001));
#269319=CARTESIAN_POINT('Ctrl Pts',(-10.2360644840001,15.2,-2.80909264400002));
#269320=CARTESIAN_POINT('Ctrl Pts',(-10.2382140350001,15.2,-2.80917450000001));
#269321=CARTESIAN_POINT('Ctrl Pts',(-10.2403704120001,15.2,-2.80925469500001));
#269322=CARTESIAN_POINT('Ctrl Pts',(-10.2425336010001,15.2,-2.80933321800001));
#269323=CARTESIAN_POINT('Ctrl Pts',(-10.2447035880001,15.2,-2.80941005800001));
#269324=CARTESIAN_POINT('Ctrl Pts',(-10.2468803590001,15.2,-2.80948520200001));
#269325=CARTESIAN_POINT('Ctrl Pts',(-10.2490639020001,15.2,-2.80955864200001));
#269326=CARTESIAN_POINT('Ctrl Pts',(-10.2512542030001,15.2,-2.80963036400002));
#269327=CARTESIAN_POINT('Ctrl Pts',(-10.2534512460001,15.2,-2.80970035900001));
#269328=CARTESIAN_POINT('Ctrl Pts',(-10.2556550210001,15.2,-2.80976861500001));
#269329=CARTESIAN_POINT('Ctrl Pts',(-10.2578655120001,15.2,-2.80983512200002));
#269330=CARTESIAN_POINT('Ctrl Pts',(-10.2600827090001,15.2,-2.80989986700002));
#269331=CARTESIAN_POINT('Ctrl Pts',(-10.2623065940001,15.2,-2.80996284100001));
#269332=CARTESIAN_POINT('Ctrl Pts',(-10.2645371560001,15.2,-2.81002403300001));
#269333=CARTESIAN_POINT('Ctrl Pts',(-10.2667743820001,15.2,-2.81008343100002));
#269334=CARTESIAN_POINT('Ctrl Pts',(-10.2690182590001,15.2,-2.81014102700002));
#269335=CARTESIAN_POINT('Ctrl Pts',(-10.2712687710001,15.2,-2.81019680600001));
#269336=CARTESIAN_POINT('Ctrl Pts',(-10.2735259090001,15.2,-2.81025076200002));
#269337=CARTESIAN_POINT('Ctrl Pts',(-10.2757896570001,15.2,-2.81030288000002));
#269338=CARTESIAN_POINT('Ctrl Pts',(-10.2780600020001,15.2,-2.81035315300001));
#269339=CARTESIAN_POINT('Ctrl Pts',(-10.2803369320001,15.2,-2.81040156800001));
#269340=CARTESIAN_POINT('Ctrl Pts',(-10.2826204320001,15.2,-2.81044811600001));
#269341=CARTESIAN_POINT('Ctrl Pts',(-10.2849104920001,15.2,-2.81049278600001));
#269342=CARTESIAN_POINT('Ctrl Pts',(-10.2872070960001,15.2,-2.81053556800002));
#269343=CARTESIAN_POINT('Ctrl Pts',(-10.2895102320001,15.2,-2.81057645100002));
#269344=CARTESIAN_POINT('Ctrl Pts',(-10.2918198870001,15.2,-2.81061542500002));
#269345=CARTESIAN_POINT('Ctrl Pts',(-10.2941360500001,15.2,-2.81065248000001));
#269346=CARTESIAN_POINT('Ctrl Pts',(-10.2964587060001,15.2,-2.81068760400002));
#269347=CARTESIAN_POINT('Ctrl Pts',(-10.2987878420001,15.2,-2.81072079000001));
#269348=CARTESIAN_POINT('Ctrl Pts',(-10.3011234450001,15.2,-2.81075202400002));
#269349=CARTESIAN_POINT('Ctrl Pts',(-10.3034655040001,15.2,-2.81078129900001));
#269350=CARTESIAN_POINT('Ctrl Pts',(-10.3058140040001,15.2,-2.81080860400001));
#269351=CARTESIAN_POINT('Ctrl Pts',(-10.3081689340001,15.2,-2.81083392700001));
#269352=CARTESIAN_POINT('Ctrl Pts',(-10.3105302810001,15.2,-2.81085726100001));
#269353=CARTESIAN_POINT('Ctrl Pts',(-10.3128980330001,15.2,-2.81087859400001));
#269354=CARTESIAN_POINT('Ctrl Pts',(-10.3152721750001,15.2,-2.81089791800001));
#269355=CARTESIAN_POINT('Ctrl Pts',(-10.3176526950001,15.2,-2.81091522000001));
#269356=CARTESIAN_POINT('Ctrl Pts',(-10.3200395830001,15.2,-2.81093049300001));
#269357=CARTESIAN_POINT('Ctrl Pts',(-10.3224328240001,15.2,-2.81094372600001));
#269358=CARTESIAN_POINT('Ctrl Pts',(-10.3248324060001,15.2,-2.81095490800002));
#269359=CARTESIAN_POINT('Ctrl Pts',(-10.3272383160001,15.2,-2.81096403100001));
#269360=CARTESIAN_POINT('Ctrl Pts',(-10.3296505420001,15.2,-2.81097108600001));
#269361=CARTESIAN_POINT('Ctrl Pts',(-10.3320690720001,15.2,-2.81097606100001));
#269362=CARTESIAN_POINT('Ctrl Pts',(-10.3344938940001,15.2,-2.81097894800002));
#269363=CARTESIAN_POINT('Ctrl Pts',(-10.3369249940001,15.2,-2.81097973500001));
#269364=CARTESIAN_POINT('Ctrl Pts',(-10.3393623600001,15.2,-2.81097841600001));
#269365=CARTESIAN_POINT('Ctrl Pts',(-10.3418059810001,15.2,-2.81097497900001));
#269366=CARTESIAN_POINT('Ctrl Pts',(-10.3442558440001,15.2,-2.81096941500001));
#269367=CARTESIAN_POINT('Ctrl Pts',(-10.3467119360001,15.2,-2.81096171500002));
#269368=CARTESIAN_POINT('Ctrl Pts',(-10.3491742450001,15.2,-2.81095186900002));
#269369=CARTESIAN_POINT('Ctrl Pts',(-10.3516427590001,15.2,-2.81093986800002));
#269370=CARTESIAN_POINT('Ctrl Pts',(-10.3541174660001,15.2,-2.81092570300002));
#269371=CARTESIAN_POINT('Ctrl Pts',(-10.3565983540001,15.2,-2.81090936300001));
#269372=CARTESIAN_POINT('Ctrl Pts',(-10.3590854110001,15.2,-2.81089083900001));
#269373=CARTESIAN_POINT('Ctrl Pts',(-10.3615786240001,15.2,-2.81087012400001));
#269374=CARTESIAN_POINT('Ctrl Pts',(-10.3640779820001,15.2,-2.81084720700001));
#269375=CARTESIAN_POINT('Ctrl Pts',(-10.3665834700001,15.2,-2.81082207900001));
#269376=CARTESIAN_POINT('Ctrl Pts',(-10.3690950810001,15.2,-2.81079473000001));
#269377=CARTESIAN_POINT('Ctrl Pts',(-10.3716127990001,15.2,-2.81076515200001));
#269378=CARTESIAN_POINT('Ctrl Pts',(-10.3741366140001,15.2,-2.81073333600002));
#269379=CARTESIAN_POINT('Ctrl Pts',(-10.3766665130001,15.2,-2.81069927400001));
#269380=CARTESIAN_POINT('Ctrl Pts',(-10.3792024840001,15.2,-2.81066295300001));
#269381=CARTESIAN_POINT('Ctrl Pts',(-10.3817445160001,15.2,-2.81062436900001));
#269382=CARTESIAN_POINT('Ctrl Pts',(-10.3842925970001,15.2,-2.81058350800001));
#269383=CARTESIAN_POINT('Ctrl Pts',(-10.3868467140001,15.2,-2.81054036500001));
#269384=CARTESIAN_POINT('Ctrl Pts',(-10.3894068560001,15.2,-2.81049493000001));
#269385=CARTESIAN_POINT('Ctrl Pts',(-10.3919730120001,15.2,-2.81044719300001));
#269386=CARTESIAN_POINT('Ctrl Pts',(-10.3945451690001,15.2,-2.81039714800002));
#269387=CARTESIAN_POINT('Ctrl Pts',(-10.3971233170001,15.2,-2.81034478200001));
#269388=CARTESIAN_POINT('Ctrl Pts',(-10.3997074400001,15.2,-2.81029008900001));
#269389=CARTESIAN_POINT('Ctrl Pts',(-10.4022975320001,15.2,-2.81023306000002));
#269390=CARTESIAN_POINT('Ctrl Pts',(-10.4048935770001,15.2,-2.81017368600001));
#269391=CARTESIAN_POINT('Ctrl Pts',(-10.4074955650001,15.2,-2.81011195800001));
#269392=CARTESIAN_POINT('Ctrl Pts',(-10.4101034850001,15.2,-2.81004786800001));
#269393=CARTESIAN_POINT('Ctrl Pts',(-10.4127173250001,15.2,-2.80998140700001));
#269394=CARTESIAN_POINT('Ctrl Pts',(-10.4153370720001,15.2,-2.80991256500001));
#269395=CARTESIAN_POINT('Ctrl Pts',(-10.4179627160001,15.2,-2.80984133700001));
#269396=CARTESIAN_POINT('Ctrl Pts',(-10.4205942460001,15.2,-2.80976771100002));
#269397=CARTESIAN_POINT('Ctrl Pts',(-10.4232316480001,15.2,-2.80969168100001));
#269398=CARTESIAN_POINT('Ctrl Pts',(-10.4258749130001,15.2,-2.80961323700001));
#269399=CARTESIAN_POINT('Ctrl Pts',(-10.4285240300001,15.2,-2.80953237000002));
#269400=CARTESIAN_POINT('Ctrl Pts',(-10.4311789840001,15.2,-2.80944907300002));
#269401=CARTESIAN_POINT('Ctrl Pts',(-10.4338397670001,15.2,-2.80936333700001));
#269402=CARTESIAN_POINT('Ctrl Pts',(-10.4365063660001,15.2,-2.80927515500002));
#269403=CARTESIAN_POINT('Ctrl Pts',(-10.4391787700001,15.2,-2.80918451700002));
#269404=CARTESIAN_POINT('Ctrl Pts',(-10.4418569680001,15.2,-2.80909141400001));
#269405=CARTESIAN_POINT('Ctrl Pts',(-10.4445409480001,15.2,-2.80899584100001));
#269406=CARTESIAN_POINT('Ctrl Pts',(-10.4472306990001,15.2,-2.80889778700002));
#269407=CARTESIAN_POINT('Ctrl Pts',(-10.4499262110001,15.2,-2.80879724300001));
#269408=CARTESIAN_POINT('Ctrl Pts',(-10.4526274700001,15.2,-2.80869420500002));
#269409=CARTESIAN_POINT('Ctrl Pts',(-10.4553344680001,15.2,-2.80858866000001));
#269410=CARTESIAN_POINT('Ctrl Pts',(-10.4580471910001,15.2,-2.80848060400002));
#269411=CARTESIAN_POINT('Ctrl Pts',(-10.4607656300001,15.2,-2.80837002600002));
#269412=CARTESIAN_POINT('Ctrl Pts',(-10.4634897720001,15.2,-2.80825691900001));
#269413=CARTESIAN_POINT('Ctrl Pts',(-10.4662196070001,15.2,-2.80814127600001));
#269414=CARTESIAN_POINT('Ctrl Pts',(-10.4689551240001,15.2,-2.80802308700002));
#269415=CARTESIAN_POINT('Ctrl Pts',(-10.4716963110001,15.2,-2.80790234500001));
#269416=CARTESIAN_POINT('Ctrl Pts',(-10.4744431570001,15.2,-2.80777904200002));
#269417=CARTESIAN_POINT('Ctrl Pts',(-10.4771956530001,15.2,-2.80765317100002));
#269418=CARTESIAN_POINT('Ctrl Pts',(-10.4799537850001,15.2,-2.80752472200001));
#269419=CARTESIAN_POINT('Ctrl Pts',(-10.4827175440001,15.2,-2.80739369000001));
#269420=CARTESIAN_POINT('Ctrl Pts',(-10.4854869180001,15.2,-2.80726006400001));
#269421=CARTESIAN_POINT('Ctrl Pts',(-10.4882618970001,15.2,-2.80712384000001));
#269422=CARTESIAN_POINT('Ctrl Pts',(-10.4910424700001,15.2,-2.80698500600002));
#269423=CARTESIAN_POINT('Ctrl Pts',(-10.4938286240001,15.2,-2.80684355700001));
#269424=CARTESIAN_POINT('Ctrl Pts',(-10.4966203510001,15.2,-2.80669948500002));
#269425=CARTESIAN_POINT('Ctrl Pts',(-10.4994176380001,15.2,-2.80655278100001));
#269426=CARTESIAN_POINT('Ctrl Pts',(-10.5022204750001,15.2,-2.80640343900001));
#269427=CARTESIAN_POINT('Ctrl Pts',(-10.5050288510001,15.2,-2.80625145000001));
#269428=CARTESIAN_POINT('Ctrl Pts',(-10.5078427570001,15.2,-2.80609680700001));
#269429=CARTESIAN_POINT('Ctrl Pts',(-10.5106621790001,15.2,-2.80593950300001));
#269430=CARTESIAN_POINT('Ctrl Pts',(-10.5134871080001,15.2,-2.80577952900002));
#269431=CARTESIAN_POINT('Ctrl Pts',(-10.5163175340001,15.2,-2.80561687900001));
#269432=CARTESIAN_POINT('Ctrl Pts',(-10.5191534450001,15.2,-2.80545154400002));
#269433=CARTESIAN_POINT('Ctrl Pts',(-10.5225631056762,15.2,-2.80524991280734));
#269434=CARTESIAN_POINT('Ctrl Pts',(-10.525980964162,15.2,-2.80504423309635));
#269435=CARTESIAN_POINT('Ctrl Pts',(-10.5294069978381,15.2,-2.80483448890367));
#269436=CARTESIAN_POINT('Ctrl Pts',(-10.532841182012,15.2,-2.80462066721212));
#269437=CARTESIAN_POINT('Ctrl Pts',(-10.5362835010001,15.2,-2.80440275200001));
#269438=CARTESIAN_POINT('Ctrl Pts',(-10.5391575100001,15.2,-2.80421842000001));
#269439=CARTESIAN_POINT('Ctrl Pts',(-10.5420369180001,15.2,-2.80403134500002));
#269440=CARTESIAN_POINT('Ctrl Pts',(-10.5449217170001,15.2,-2.80384151900002));
#269441=CARTESIAN_POINT('Ctrl Pts',(-10.5478118940001,15.2,-2.80364893500002));
#269442=CARTESIAN_POINT('Ctrl Pts',(-10.5507074410001,15.2,-2.80345358600002));
#269443=CARTESIAN_POINT('Ctrl Pts',(-10.5536083460001,15.2,-2.80325546500002));
#269444=CARTESIAN_POINT('Ctrl Pts',(-10.5565145980001,15.2,-2.80305456500002));
#269445=CARTESIAN_POINT('Ctrl Pts',(-10.5594261870001,15.2,-2.80285087700001));
#269446=CARTESIAN_POINT('Ctrl Pts',(-10.5623431030001,15.2,-2.80264439700002));
#269447=CARTESIAN_POINT('Ctrl Pts',(-10.5652653350001,15.2,-2.80243511500001));
#269448=CARTESIAN_POINT('Ctrl Pts',(-10.5681928730001,15.2,-2.80222302500002));
#269449=CARTESIAN_POINT('Ctrl Pts',(-10.5711257080001,15.2,-2.80200812100002));
#269450=CARTESIAN_POINT('Ctrl Pts',(-10.5740638260001,15.2,-2.80179039400001));
#269451=CARTESIAN_POINT('Ctrl Pts',(-10.5770072200001,15.2,-2.80156983800001));
#269452=CARTESIAN_POINT('Ctrl Pts',(-10.5799558780001,15.2,-2.80134644700002));
#269453=CARTESIAN_POINT('Ctrl Pts',(-10.5829097920001,15.2,-2.80112021200001));
#269454=CARTESIAN_POINT('Ctrl Pts',(-10.5858689480001,15.2,-2.80089112800002));
#269455=CARTESIAN_POINT('Ctrl Pts',(-10.5888333380001,15.2,-2.80065918700001));
#269456=CARTESIAN_POINT('Ctrl Pts',(-10.5918029510001,15.2,-2.80042438200002));
#269457=CARTESIAN_POINT('Ctrl Pts',(-10.5947777780001,15.2,-2.80018670600001));
#269458=CARTESIAN_POINT('Ctrl Pts',(-10.5977578070001,15.2,-2.79994615300001));
#269459=CARTESIAN_POINT('Ctrl Pts',(-10.6007430310001,15.2,-2.79970271700002));
#269460=CARTESIAN_POINT('Ctrl Pts',(-10.6037334350001,15.2,-2.79945638900001));
#269461=CARTESIAN_POINT('Ctrl Pts',(-10.6067290130001,15.2,-2.79920716400001));
#269462=CARTESIAN_POINT('Ctrl Pts',(-10.6097297520001,15.2,-2.79895503300001));
#269463=CARTESIAN_POINT('Ctrl Pts',(-10.6127356450001,15.2,-2.79869999200002));
#269464=CARTESIAN_POINT('Ctrl Pts',(-10.6157466780001,15.2,-2.79844203300001));
#269465=CARTESIAN_POINT('Ctrl Pts',(-10.6187628440001,15.2,-2.79818114900001));
#269466=CARTESIAN_POINT('Ctrl Pts',(-10.6217841320001,15.2,-2.79791733300002));
#269467=CARTESIAN_POINT('Ctrl Pts',(-10.6248105320001,15.2,-2.79765058100002));
#269468=CARTESIAN_POINT('Ctrl Pts',(-10.6278420330001,15.2,-2.79738088400002));
#269469=CARTESIAN_POINT('Ctrl Pts',(-10.6308786260001,15.2,-2.79710823500002));
#269470=CARTESIAN_POINT('Ctrl Pts',(-10.6339203020001,15.2,-2.79683262800001));
#269471=CARTESIAN_POINT('Ctrl Pts',(-10.6369670490001,15.2,-2.79655405800002));
#269472=CARTESIAN_POINT('Ctrl Pts',(-10.6400188580001,15.2,-2.79627251700001));
#269473=CARTESIAN_POINT('Ctrl Pts',(-10.6430757180001,15.2,-2.79598800000001));
#269474=CARTESIAN_POINT('Ctrl Pts',(-10.6461376210001,15.2,-2.79570049800002));
#269475=CARTESIAN_POINT('Ctrl Pts',(-10.6492045550001,15.2,-2.79541000500001));
#269476=CARTESIAN_POINT('Ctrl Pts',(-10.6522765120001,15.2,-2.79511651600002));
#269477=CARTESIAN_POINT('Ctrl Pts',(-10.6553534800001,15.2,-2.79482002500002));
#269478=CARTESIAN_POINT('Ctrl Pts',(-10.6584354520001,15.2,-2.79452052500002));
#269479=CARTESIAN_POINT('Ctrl Pts',(-10.6615224160001,15.2,-2.79421800700002));
#269480=CARTESIAN_POINT('Ctrl Pts',(-10.6646143620001,15.2,-2.79391246900001));
#269481=CARTESIAN_POINT('Ctrl Pts',(-10.6677112820001,15.2,-2.79360390200001));
#269482=CARTESIAN_POINT('Ctrl Pts',(-10.6708131640001,15.2,-2.79329230000001));
#269483=CARTESIAN_POINT('Ctrl Pts',(-10.6739200000001,15.2,-2.79297765700001));
#269484=CARTESIAN_POINT('Ctrl Pts',(-10.6770317790001,15.2,-2.79265996700001));
#269485=CARTESIAN_POINT('Ctrl Pts',(-10.6801484920001,15.2,-2.79233922300001));
#269486=CARTESIAN_POINT('Ctrl Pts',(-10.6832701290001,15.2,-2.79201542000001));
#269487=CARTESIAN_POINT('Ctrl Pts',(-10.6863966800001,15.2,-2.79168855100002));
#269488=CARTESIAN_POINT('Ctrl Pts',(-10.6895281350001,15.2,-2.79135861000002));
#269489=CARTESIAN_POINT('Ctrl Pts',(-10.6926644870001,15.2,-2.79102559000002));
#269490=CARTESIAN_POINT('Ctrl Pts',(-10.6958057220001,15.2,-2.79068948600001));
#269491=CARTESIAN_POINT('Ctrl Pts',(-10.6989518340001,15.2,-2.79035029100001));
#269492=CARTESIAN_POINT('Ctrl Pts',(-10.7021028110001,15.2,-2.79000800100001));
#269493=CARTESIAN_POINT('Ctrl Pts',(-10.7052586450001,15.2,-2.78966260600002));
#269494=CARTESIAN_POINT('Ctrl Pts',(-10.7084193250001,15.2,-2.78931410400002));
#269495=CARTESIAN_POINT('Ctrl Pts',(-10.7115848430001,15.2,-2.78896248700002));
#269496=CARTESIAN_POINT('Ctrl Pts',(-10.7147551880001,15.2,-2.78860774800001));
#269497=CARTESIAN_POINT('Ctrl Pts',(-10.7179303500001,15.2,-2.78824988400002));
#269498=CARTESIAN_POINT('Ctrl Pts',(-10.7211103210001,15.2,-2.78788888700001));
#269499=CARTESIAN_POINT('Ctrl Pts',(-10.7242950910001,15.2,-2.78752475000001));
#269500=CARTESIAN_POINT('Ctrl Pts',(-10.7274846510001,15.2,-2.78715746900001));
#269501=CARTESIAN_POINT('Ctrl Pts',(-10.7306789900001,15.2,-2.78678703700002));
#269502=CARTESIAN_POINT('Ctrl Pts',(-10.7338780990001,15.2,-2.78641345000001));
#269503=CARTESIAN_POINT('Ctrl Pts',(-10.7370819700001,15.2,-2.78603669900002));
#269504=CARTESIAN_POINT('Ctrl Pts',(-10.7402905920001,15.2,-2.78565678100001));
#269505=CARTESIAN_POINT('Ctrl Pts',(-10.7435039560001,15.2,-2.78527368900002));
#269506=CARTESIAN_POINT('Ctrl Pts',(-10.7467220520001,15.2,-2.78488741600002));
#269507=CARTESIAN_POINT('Ctrl Pts',(-10.7499448710001,15.2,-2.78449795800002));
#269508=CARTESIAN_POINT('Ctrl Pts',(-10.7531724040001,15.2,-2.78410530900001));
#269509=CARTESIAN_POINT('Ctrl Pts',(-10.7564046420001,15.2,-2.78370946300001));
#269510=CARTESIAN_POINT('Ctrl Pts',(-10.7596415740001,15.2,-2.78331041300001));
#269511=CARTESIAN_POINT('Ctrl Pts',(-10.7628831920001,15.2,-2.78290815600001));
#269512=CARTESIAN_POINT('Ctrl Pts',(-10.7661294860001,15.2,-2.78250268300001));
#269513=CARTESIAN_POINT('Ctrl Pts',(-10.7693804470001,15.2,-2.78209399100001));
#269514=CARTESIAN_POINT('Ctrl Pts',(-10.7726360660001,15.2,-2.78168207300002));
#269515=CARTESIAN_POINT('Ctrl Pts',(-10.7758963330001,15.2,-2.78126692300001));
#269516=CARTESIAN_POINT('Ctrl Pts',(-10.7791612390001,15.2,-2.78084853700001));
#269517=CARTESIAN_POINT('Ctrl Pts',(-10.7824307750001,15.2,-2.78042690900001));
#269518=CARTESIAN_POINT('Ctrl Pts',(-10.7857049310001,15.2,-2.78000203100001));
#269519=CARTESIAN_POINT('Ctrl Pts',(-10.7889836990001,15.2,-2.77957390000001));
#269520=CARTESIAN_POINT('Ctrl Pts',(-10.7922670680001,15.2,-2.77914251000002));
#269521=CARTESIAN_POINT('Ctrl Pts',(-10.7955550300001,15.2,-2.77870785600001));
#269522=CARTESIAN_POINT('Ctrl Pts',(-10.7988475760001,15.2,-2.77826993000001));
#269523=CARTESIAN_POINT('Ctrl Pts',(-10.8021446960001,15.2,-2.77782872900001));
#269524=CARTESIAN_POINT('Ctrl Pts',(-10.8054463820001,15.2,-2.77738424700001));
#269525=CARTESIAN_POINT('Ctrl Pts',(-10.8087526240001,15.2,-2.77693647800001));
#269526=CARTESIAN_POINT('Ctrl Pts',(-10.8120634130001,15.2,-2.77648541700001));
#269527=CARTESIAN_POINT('Ctrl Pts',(-10.8153787400001,15.2,-2.77603105800001));
#269528=CARTESIAN_POINT('Ctrl Pts',(-10.8186985940001,15.2,-2.77557339600001));
#269529=CARTESIAN_POINT('Ctrl Pts',(-10.8220229700001,15.2,-2.77511242500001));
#269530=CARTESIAN_POINT('Ctrl Pts',(-10.8253518550001,15.2,-2.77464814100002));
#269531=CARTESIAN_POINT('Ctrl Pts',(-10.8286852410001,15.2,-2.77418053700002));
#269532=CARTESIAN_POINT('Ctrl Pts',(-10.8320231210001,15.2,-2.77370961000001));
#269533=CARTESIAN_POINT('Ctrl Pts',(-10.8353654830001,15.2,-2.77323535200001));
#269534=CARTESIAN_POINT('Ctrl Pts',(-10.8387123200001,15.2,-2.77275775900002));
#269535=CARTESIAN_POINT('Ctrl Pts',(-10.8420636210001,15.2,-2.77227682600001));
#269536=CARTESIAN_POINT('Ctrl Pts',(-10.8454193790001,15.2,-2.77179254700001));
#269537=CARTESIAN_POINT('Ctrl Pts',(-10.8487795840001,15.2,-2.77130491700001));
#269538=CARTESIAN_POINT('Ctrl Pts',(-10.8521442280001,15.2,-2.77081393100001));
#269539=CARTESIAN_POINT('Ctrl Pts',(-10.8555133010001,15.2,-2.77031958400002));
#269540=CARTESIAN_POINT('Ctrl Pts',(-10.8588867940001,15.2,-2.76982187100002));
#269541=CARTESIAN_POINT('Ctrl Pts',(-10.8622646980001,15.2,-2.76932078500002));
#269542=CARTESIAN_POINT('Ctrl Pts',(-10.8656470060001,15.2,-2.76881632300002));
#269543=CARTESIAN_POINT('Ctrl Pts',(-10.8690337060001,15.2,-2.76830847900001));
#269544=CARTESIAN_POINT('Ctrl Pts',(-10.8724247920001,15.2,-2.76779724700001));
#269545=CARTESIAN_POINT('Ctrl Pts',(-10.8758202520001,15.2,-2.76728262200002));
#269546=CARTESIAN_POINT('Ctrl Pts',(-10.8792200800001,15.2,-2.76676460200001));
#269547=CARTESIAN_POINT('Ctrl Pts',(-10.8826242650001,15.2,-2.76624317800001));
#269548=CARTESIAN_POINT('Ctrl Pts',(-10.8860328000001,15.2,-2.76571834600002));
#269549=CARTESIAN_POINT('Ctrl Pts',(-10.8894456750001,15.2,-2.76519010300001));
#269550=CARTESIAN_POINT('Ctrl Pts',(-10.8928628820001,15.2,-2.76465844200001));
#269551=CARTESIAN_POINT('Ctrl Pts',(-10.8962844110001,15.2,-2.76412335800002));
#269552=CARTESIAN_POINT('Ctrl Pts',(-10.8997102540001,15.2,-2.76358484600001));
#269553=CARTESIAN_POINT('Ctrl Pts',(-10.9031404020001,15.2,-2.76304290100001));
#269554=CARTESIAN_POINT('Ctrl Pts',(-10.9065748460001,15.2,-2.76249752000002));
#269555=CARTESIAN_POINT('Ctrl Pts',(-10.9100135780001,15.2,-2.76194869600001));
#269556=CARTESIAN_POINT('Ctrl Pts',(-10.9134565880001,15.2,-2.76139642400001));
#269557=CARTESIAN_POINT('Ctrl Pts',(-10.9169038680001,15.2,-2.76084070000001));
#269558=CARTESIAN_POINT('Ctrl Pts',(-10.9203554100001,15.2,-2.76028151900002));
#269559=CARTESIAN_POINT('Ctrl Pts',(-10.9238112040001,15.2,-2.75971887600001));
#269560=CARTESIAN_POINT('Ctrl Pts',(-10.9272712420001,15.2,-2.75915276600001));
#269561=CARTESIAN_POINT('Ctrl Pts',(-10.9307355160001,15.2,-2.75858318400001));
#269562=CARTESIAN_POINT('Ctrl Pts',(-10.9342040160001,15.2,-2.75801012600001));
#269563=CARTESIAN_POINT('Ctrl Pts',(-10.9376767320001,15.2,-2.75743358500002));
#269564=CARTESIAN_POINT('Ctrl Pts',(-10.9411536590001,15.2,-2.75685355800002));
#269565=CARTESIAN_POINT('Ctrl Pts',(-10.9446347860001,15.2,-2.75627004100001));
#269566=CARTESIAN_POINT('Ctrl Pts',(-10.9481201050001,15.2,-2.75568302700002));
#269567=CARTESIAN_POINT('Ctrl Pts',(-10.9516096070001,15.2,-2.75509251400001));
#269568=CARTESIAN_POINT('Ctrl Pts',(-10.9551032830001,15.2,-2.75449849500002));
#269569=CARTESIAN_POINT('Ctrl Pts',(-10.9586011260001,15.2,-2.75390096500002));
#269570=CARTESIAN_POINT('Ctrl Pts',(-10.9621031260001,15.2,-2.75329992100001));
#269571=CARTESIAN_POINT('Ctrl Pts',(-10.9656092750001,15.2,-2.75269535800001));
#269572=CARTESIAN_POINT('Ctrl Pts',(-10.9691195640001,15.2,-2.75208727000001));
#269573=CARTESIAN_POINT('Ctrl Pts',(-10.9726339840001,15.2,-2.75147565300002));
#269574=CARTESIAN_POINT('Ctrl Pts',(-10.9761525290001,15.2,-2.75086050400001));
#269575=CARTESIAN_POINT('Ctrl Pts',(-10.9796751870001,15.2,-2.75024181600001));
#269576=CARTESIAN_POINT('Ctrl Pts',(-10.9832019520001,15.2,-2.74961958600001));
#269577=CARTESIAN_POINT('Ctrl Pts',(-10.9867328140001,15.2,-2.74899380700001));
#269578=CARTESIAN_POINT('Ctrl Pts',(-10.9902677660001,15.2,-2.74836447800002));
#269579=CARTESIAN_POINT('Ctrl Pts',(-10.9938067980001,15.2,-2.74773159100001));
#269580=CARTESIAN_POINT('Ctrl Pts',(-10.9973499030001,15.2,-2.74709514500001));
#269581=CARTESIAN_POINT('Ctrl Pts',(-11.0008970700001,15.2,-2.74645513200001));
#269582=CARTESIAN_POINT('Ctrl Pts',(-11.0044482940001,15.2,-2.74581155000002));
#269583=CARTESIAN_POINT('Ctrl Pts',(-11.0080035640001,15.2,-2.74516439200001));
#269584=CARTESIAN_POINT('Ctrl Pts',(-11.0115628720001,15.2,-2.74451365600001));
#269585=CARTESIAN_POINT('Ctrl Pts',(-11.0151262110001,15.2,-2.74385933600001));
#269586=CARTESIAN_POINT('Ctrl Pts',(-11.0186935710001,15.2,-2.74320142800001));
#269587=CARTESIAN_POINT('Ctrl Pts',(-11.0222649450001,15.2,-2.74253992800002));
#269588=CARTESIAN_POINT('Ctrl Pts',(-11.0258403220001,15.2,-2.74187483000001));
#269589=CARTESIAN_POINT('Ctrl Pts',(-11.0294196970001,15.2,-2.74120613200001));
#269590=CARTESIAN_POINT('Ctrl Pts',(-11.0330030590001,15.2,-2.74053382800002));
#269591=CARTESIAN_POINT('Ctrl Pts',(-11.0365904010001,15.2,-2.73985791400001));
#269592=CARTESIAN_POINT('Ctrl Pts',(-11.0401817150001,15.2,-2.73917838500001));
#269593=CARTESIAN_POINT('Ctrl Pts',(-11.0437769920001,15.2,-2.73849523700001));
#269594=CARTESIAN_POINT('Ctrl Pts',(-11.0473762230001,15.2,-2.73780846600001));
#269595=CARTESIAN_POINT('Ctrl Pts',(-11.0509794010001,15.2,-2.73711806700002));
#269596=CARTESIAN_POINT('Ctrl Pts',(-11.0545865170001,15.2,-2.73642403700002));
#269597=CARTESIAN_POINT('Ctrl Pts',(-11.0581975630001,15.2,-2.73572637000001));
#269598=CARTESIAN_POINT('Ctrl Pts',(-11.0618125300001,15.2,-2.73502506300002));
#269599=CARTESIAN_POINT('Ctrl Pts',(-11.0654314110001,15.2,-2.73432011200001));
#269600=CARTESIAN_POINT('Ctrl Pts',(-11.0690541960001,15.2,-2.73361151100001));
#269601=CARTESIAN_POINT('Ctrl Pts',(-11.0726808780001,15.2,-2.73289925600002));
#269602=CARTESIAN_POINT('Ctrl Pts',(-11.0763114490001,15.2,-2.73218334500001));
#269603=CARTESIAN_POINT('Ctrl Pts',(-11.0799458990001,15.2,-2.73146377200002));
#269604=CARTESIAN_POINT('Ctrl Pts',(-11.0835842240001,15.2,-2.73074053200002));
#269605=CARTESIAN_POINT('Ctrl Pts',(-11.0872264110001,15.2,-2.73001362300001));
#269606=CARTESIAN_POINT('Ctrl Pts',(-11.0908724560001,15.2,-2.72928304000001));
#269607=CARTESIAN_POINT('Ctrl Pts',(-11.0945223470001,15.2,-2.72854877900001));
#269608=CARTESIAN_POINT('Ctrl Pts',(-11.0981760790001,15.2,-2.72781083400002));
#269609=CARTESIAN_POINT('Ctrl Pts',(-11.1018336410001,15.2,-2.72706920300001));
#269610=CARTESIAN_POINT('Ctrl Pts',(-11.1054950240001,15.2,-2.72632388100002));
#269611=CARTESIAN_POINT('Ctrl Pts',(-11.1091602230001,15.2,-2.72557486300002));
#269612=CARTESIAN_POINT('Ctrl Pts',(-11.1128292270001,15.2,-2.72482214500001));
#269613=CARTESIAN_POINT('Ctrl Pts',(-11.1165020290001,15.2,-2.72406572300001));
#269614=CARTESIAN_POINT('Ctrl Pts',(-11.1201786230001,15.2,-2.72330559600002));
#269615=CARTESIAN_POINT('Ctrl Pts',(-11.1238590000001,15.2,-2.72254175700001));
#269616=CARTESIAN_POINT('Ctrl Pts',(-11.1275431540001,15.2,-2.72177420400002));
#269617=CARTESIAN_POINT('Ctrl Pts',(-11.1312310760001,15.2,-2.72100293300001));
#269618=CARTESIAN_POINT('Ctrl Pts',(-11.1349227590001,15.2,-2.72022793900002));
#269619=CARTESIAN_POINT('Ctrl Pts',(-11.1386181920001,15.2,-2.71944921800001));
#269620=CARTESIAN_POINT('Ctrl Pts',(-11.1423173660001,15.2,-2.71866676600002));
#269621=CARTESIAN_POINT('Ctrl Pts',(-11.1460202710001,15.2,-2.71788057600002));
#269622=CARTESIAN_POINT('Ctrl Pts',(-11.1497268980001,15.2,-2.71709064400001));
#269623=CARTESIAN_POINT('Ctrl Pts',(-11.1534372360001,15.2,-2.71629696600002));
#269624=CARTESIAN_POINT('Ctrl Pts',(-11.1571512810001,15.2,-2.71549953800001));
#269625=CARTESIAN_POINT('Ctrl Pts',(-11.1608690250001,15.2,-2.71469835800001));
#269626=CARTESIAN_POINT('Ctrl Pts',(-11.1645904650001,15.2,-2.71389342400001));
#269627=CARTESIAN_POINT('Ctrl Pts',(-11.1683155990001,15.2,-2.71308473500001));
#269628=CARTESIAN_POINT('Ctrl Pts',(-11.1712986600001,15.2,-2.71243478000001));
#269629=CARTESIAN_POINT('Ctrl Pts',(-11.1735376180001,15.2,-2.71194562400002));
#269630=CARTESIAN_POINT('Ctrl Pts',(-11.1750309950001,15.2,-2.71161876900001));
#269631=CARTESIAN_POINT('Ctrl Pts',(-11.1757778680001,15.2,-2.71145515300002));
#269632=CARTESIAN_POINT('Origin',(-5.66257110645729E-14,15.2,-1.77635683940025E-14));
#269633=CARTESIAN_POINT('',(-9.86852965800006,15.2,-3.20199116200001));
#269634=CARTESIAN_POINT('',(-9.86852965800006,12.2,-3.20199116200001));
#269635=CARTESIAN_POINT('',(-9.86852965800006,15.2,-3.20199116200001));
#269636=CARTESIAN_POINT('Origin',(-5.66257110645729E-14,12.2,-1.77635683940025E-14));
#269637=CARTESIAN_POINT('Origin',(-5.66257110645729E-14,15.2,-1.77635683940025E-14));
#269638=CARTESIAN_POINT('Origin',(-5.66257110645729E-14,15.2,-1.77635683940025E-14));
#269639=CARTESIAN_POINT('',(-10.8127719254279,15.2,-3.91586047903425));
#269640=CARTESIAN_POINT('',(-10.6761442620001,15.2,-4.27433546900001));
#269641=CARTESIAN_POINT('Origin',(-5.66257110645729E-14,15.2,-1.77635683940025E-14));
#269642=CARTESIAN_POINT('',(-10.6761442620001,12.2,-4.27433546900001));
#269643=CARTESIAN_POINT('',(-10.6761442620001,15.2,-4.27433546900001));
#269644=CARTESIAN_POINT('',(-10.8127719250001,12.2,-3.91586047900002));
#269645=CARTESIAN_POINT('Origin',(-5.66257110645729E-14,12.2,-1.77635683940025E-14));
#269646=CARTESIAN_POINT('',(-10.8127719250001,15.2,-3.91586047900002));
#269647=CARTESIAN_POINT('Ctrl Pts',(-10.6761442620001,15.2,-4.27433546900001));
#269648=CARTESIAN_POINT('Ctrl Pts',(-10.6761442620001,11.6,-4.27433546900002));
#269649=CARTESIAN_POINT('Ctrl Pts',(-10.6753817060001,15.2,-4.27439112800001));
#269650=CARTESIAN_POINT('Ctrl Pts',(-10.6753817060001,11.6,-4.27439112800002));
#269651=CARTESIAN_POINT('Ctrl Pts',(-10.6738570140001,15.2,-4.27450212700001));
#269652=CARTESIAN_POINT('Ctrl Pts',(-10.6738570140001,11.6,-4.27450212700002));
#269653=CARTESIAN_POINT('Ctrl Pts',(-10.6715712310001,15.2,-4.27466766700002));
#269654=CARTESIAN_POINT('Ctrl Pts',(-10.6715712310001,11.6,-4.27466766700002));
#269655=CARTESIAN_POINT('Ctrl Pts',(-10.6685260340001,15.2,-4.27488647300001));
#269656=CARTESIAN_POINT('Ctrl Pts',(-10.6685260340001,11.6,-4.27488647300002));
#269657=CARTESIAN_POINT('Ctrl Pts',(-10.6647237270001,15.2,-4.27515678900001));
#269658=CARTESIAN_POINT('Ctrl Pts',(-10.6647237270001,11.6,-4.27515678900001));
#269659=CARTESIAN_POINT('Ctrl Pts',(-10.6609256130001,15.2,-4.27542391400001));
#269660=CARTESIAN_POINT('Ctrl Pts',(-10.6609256130001,11.6,-4.27542391400001));
#269661=CARTESIAN_POINT('Ctrl Pts',(-10.6571316910001,15.2,-4.27568784800001));
#269662=CARTESIAN_POINT('Ctrl Pts',(-10.6571316910001,11.6,-4.27568784800001));
#269663=CARTESIAN_POINT('Ctrl Pts',(-10.6533419640001,15.2,-4.27594859600001));
#269664=CARTESIAN_POINT('Ctrl Pts',(-10.6533419640001,11.6,-4.27594859600002));
#269665=CARTESIAN_POINT('Ctrl Pts',(-10.6495564390001,15.2,-4.27620616000001));
#269666=CARTESIAN_POINT('Ctrl Pts',(-10.6495564390001,11.6,-4.27620616000001));
#269667=CARTESIAN_POINT('Ctrl Pts',(-10.6457751210001,15.2,-4.27646054300002));
#269668=CARTESIAN_POINT('Ctrl Pts',(-10.6457751210001,11.6,-4.27646054300002));
#269669=CARTESIAN_POINT('Ctrl Pts',(-10.6419980200001,15.2,-4.27671175200001));
#269670=CARTESIAN_POINT('Ctrl Pts',(-10.6419980200001,11.6,-4.27671175200001));
#269671=CARTESIAN_POINT('Ctrl Pts',(-10.6382251440001,15.2,-4.27695979300001));
#269672=CARTESIAN_POINT('Ctrl Pts',(-10.6382251440001,11.6,-4.27695979300002));
#269673=CARTESIAN_POINT('Ctrl Pts',(-10.6344565010001,15.2,-4.27720467200002));
#269674=CARTESIAN_POINT('Ctrl Pts',(-10.6344565010001,11.6,-4.27720467200002));
#269675=CARTESIAN_POINT('Ctrl Pts',(-10.6306921010001,15.2,-4.27744639700002));
#269676=CARTESIAN_POINT('Ctrl Pts',(-10.6306921010001,11.6,-4.27744639700002));
#269677=CARTESIAN_POINT('Ctrl Pts',(-10.6269319530001,15.2,-4.27768497100002));
#269678=CARTESIAN_POINT('Ctrl Pts',(-10.6269319530001,11.6,-4.27768497100002));
#269679=CARTESIAN_POINT('Ctrl Pts',(-10.6231760650001,15.2,-4.27792040200002));
#269680=CARTESIAN_POINT('Ctrl Pts',(-10.6231760650001,11.6,-4.27792040200002));
#269681=CARTESIAN_POINT('Ctrl Pts',(-10.6194244440001,15.2,-4.27815269400002));
#269682=CARTESIAN_POINT('Ctrl Pts',(-10.6194244440001,11.6,-4.27815269400002));
#269683=CARTESIAN_POINT('Ctrl Pts',(-10.6156770940001,15.2,-4.27838185100001));
#269684=CARTESIAN_POINT('Ctrl Pts',(-10.6156770940001,11.6,-4.27838185100002));
#269685=CARTESIAN_POINT('Ctrl Pts',(-10.6119340260001,15.2,-4.27860787900002));
#269686=CARTESIAN_POINT('Ctrl Pts',(-10.6119340260001,11.6,-4.27860787900002));
#269687=CARTESIAN_POINT('Ctrl Pts',(-10.6081952440001,15.2,-4.27883078100002));
#269688=CARTESIAN_POINT('Ctrl Pts',(-10.6081952440001,11.6,-4.27883078100002));
#269689=CARTESIAN_POINT('Ctrl Pts',(-10.6044607560001,15.2,-4.27905056300002));
#269690=CARTESIAN_POINT('Ctrl Pts',(-10.6044607560001,11.6,-4.27905056300002));
#269691=CARTESIAN_POINT('Ctrl Pts',(-10.6007305690001,15.2,-4.27926723000001));
#269692=CARTESIAN_POINT('Ctrl Pts',(-10.6007305690001,11.6,-4.27926723000002));
#269693=CARTESIAN_POINT('Ctrl Pts',(-10.5970046900001,15.2,-4.27948078700001));
#269694=CARTESIAN_POINT('Ctrl Pts',(-10.5970046900001,11.6,-4.27948078700001));
#269695=CARTESIAN_POINT('Ctrl Pts',(-10.5932831290001,15.2,-4.27969124000001));
#269696=CARTESIAN_POINT('Ctrl Pts',(-10.5932831290001,11.6,-4.27969124000002));
#269697=CARTESIAN_POINT('Ctrl Pts',(-10.5895658910001,15.2,-4.27989859400002));
#269698=CARTESIAN_POINT('Ctrl Pts',(-10.5895658910001,11.6,-4.27989859400002));
#269699=CARTESIAN_POINT('Ctrl Pts',(-10.5858529860001,15.2,-4.28010285500001));
#269700=CARTESIAN_POINT('Ctrl Pts',(-10.5858529860001,11.6,-4.28010285500002));
#269701=CARTESIAN_POINT('Ctrl Pts',(-10.5821444200001,15.2,-4.28030402700001));
#269702=CARTESIAN_POINT('Ctrl Pts',(-10.5821444200001,11.6,-4.28030402700002));
#269703=CARTESIAN_POINT('Ctrl Pts',(-10.5784402020001,15.2,-4.28050211700001));
#269704=CARTESIAN_POINT('Ctrl Pts',(-10.5784402020001,11.6,-4.28050211700001));
#269705=CARTESIAN_POINT('Ctrl Pts',(-10.5747403380001,15.2,-4.28069713100002));
#269706=CARTESIAN_POINT('Ctrl Pts',(-10.5747403380001,11.6,-4.28069713100002));
#269707=CARTESIAN_POINT('Ctrl Pts',(-10.5710448370001,15.2,-4.28088907100001));
#269708=CARTESIAN_POINT('Ctrl Pts',(-10.5710448370001,11.6,-4.28088907100001));
#269709=CARTESIAN_POINT('Ctrl Pts',(-10.5673537050001,15.2,-4.28107794500002));
#269710=CARTESIAN_POINT('Ctrl Pts',(-10.5673537050001,11.6,-4.28107794500002));
#269711=CARTESIAN_POINT('Ctrl Pts',(-10.5636669500001,15.2,-4.28126375800002));
#269712=CARTESIAN_POINT('Ctrl Pts',(-10.5636669500001,11.6,-4.28126375800002));
#269713=CARTESIAN_POINT('Ctrl Pts',(-10.5599845790001,15.2,-4.28144651300002));
#269714=CARTESIAN_POINT('Ctrl Pts',(-10.5599845790001,11.6,-4.28144651300002));
#269715=CARTESIAN_POINT('Ctrl Pts',(-10.5563066010001,15.2,-4.28162621800002));
#269716=CARTESIAN_POINT('Ctrl Pts',(-10.5563066010001,11.6,-4.28162621800002));
#269717=CARTESIAN_POINT('Ctrl Pts',(-10.5526330210001,15.2,-4.28180287800001));
#269718=CARTESIAN_POINT('Ctrl Pts',(-10.5526330210001,11.6,-4.28180287800001));
#269719=CARTESIAN_POINT('Ctrl Pts',(-10.5489638500001,15.2,-4.28197649800001));
#269720=CARTESIAN_POINT('Ctrl Pts',(-10.5489638500001,11.6,-4.28197649800001));
#269721=CARTESIAN_POINT('Ctrl Pts',(-10.5452990930001,15.2,-4.28214708400001));
#269722=CARTESIAN_POINT('Ctrl Pts',(-10.5452990930001,11.6,-4.28214708400002));
#269723=CARTESIAN_POINT('Ctrl Pts',(-10.5416387590001,15.2,-4.28231464000001));
#269724=CARTESIAN_POINT('Ctrl Pts',(-10.5416387590001,11.6,-4.28231464000001));
#269725=CARTESIAN_POINT('Ctrl Pts',(-10.5379828550001,15.2,-4.28247917300002));
#269726=CARTESIAN_POINT('Ctrl Pts',(-10.5379828550001,11.6,-4.28247917300002));
#269727=CARTESIAN_POINT('Ctrl Pts',(-10.5343313890001,15.2,-4.28264068800001));
#269728=CARTESIAN_POINT('Ctrl Pts',(-10.5343313890001,11.6,-4.28264068800001));
#269729=CARTESIAN_POINT('Ctrl Pts',(-10.5306843670001,15.2,-4.28279919100001));
#269730=CARTESIAN_POINT('Ctrl Pts',(-10.5306843670001,11.6,-4.28279919100001));
#269731=CARTESIAN_POINT('Ctrl Pts',(-10.5270418000001,15.2,-4.28295468600002));
#269732=CARTESIAN_POINT('Ctrl Pts',(-10.5270418000001,11.6,-4.28295468600002));
#269733=CARTESIAN_POINT('Ctrl Pts',(-10.5234036920001,15.2,-4.28310718100001));
#269734=CARTESIAN_POINT('Ctrl Pts',(-10.5234036920001,11.6,-4.28310718100002));
#269735=CARTESIAN_POINT('Ctrl Pts',(-10.5197700540001,15.2,-4.28325667900001));
#269736=CARTESIAN_POINT('Ctrl Pts',(-10.5197700540001,11.6,-4.28325667900001));
#269737=CARTESIAN_POINT('Ctrl Pts',(-10.5161408910001,15.2,-4.28340318700001));
#269738=CARTESIAN_POINT('Ctrl Pts',(-10.5161408910001,11.6,-4.28340318700002));
#269739=CARTESIAN_POINT('Ctrl Pts',(-10.5125162110001,15.2,-4.28354671000001));
#269740=CARTESIAN_POINT('Ctrl Pts',(-10.5125162110001,11.6,-4.28354671000002));
#269741=CARTESIAN_POINT('Ctrl Pts',(-10.5088960220001,15.2,-4.28368725300002));
#269742=CARTESIAN_POINT('Ctrl Pts',(-10.5088960220001,11.6,-4.28368725300002));
#269743=CARTESIAN_POINT('Ctrl Pts',(-10.5052803340001,15.2,-4.28382482400002));
#269744=CARTESIAN_POINT('Ctrl Pts',(-10.5052803340001,11.6,-4.28382482400002));
#269745=CARTESIAN_POINT('Ctrl Pts',(-10.5016691510001,15.2,-4.28395942600002));
#269746=CARTESIAN_POINT('Ctrl Pts',(-10.5016691510001,11.6,-4.28395942600002));
#269747=CARTESIAN_POINT('Ctrl Pts',(-10.4980624830001,15.2,-4.28409106600002));
#269748=CARTESIAN_POINT('Ctrl Pts',(-10.4980624830001,11.6,-4.28409106600002));
#269749=CARTESIAN_POINT('Ctrl Pts',(-10.4944603360001,15.2,-4.28421975000001));
#269750=CARTESIAN_POINT('Ctrl Pts',(-10.4944603360001,11.6,-4.28421975000001));
#269751=CARTESIAN_POINT('Ctrl Pts',(-10.4908627200001,15.2,-4.28434548200002));
#269752=CARTESIAN_POINT('Ctrl Pts',(-10.4908627200001,11.6,-4.28434548200002));
#269753=CARTESIAN_POINT('Ctrl Pts',(-10.4872696400001,15.2,-4.28446827000001));
#269754=CARTESIAN_POINT('Ctrl Pts',(-10.4872696400001,11.6,-4.28446827000002));
#269755=CARTESIAN_POINT('Ctrl Pts',(-10.4836811070001,15.2,-4.28458811800001));
#269756=CARTESIAN_POINT('Ctrl Pts',(-10.4836811070001,11.6,-4.28458811800002));
#269757=CARTESIAN_POINT('Ctrl Pts',(-10.4800971270001,15.2,-4.28470503200002));
#269758=CARTESIAN_POINT('Ctrl Pts',(-10.4800971270001,11.6,-4.28470503200002));
#269759=CARTESIAN_POINT('Ctrl Pts',(-10.4765177060001,15.2,-4.28481901800001));
#269760=CARTESIAN_POINT('Ctrl Pts',(-10.4765177060001,11.6,-4.28481901800002));
#269761=CARTESIAN_POINT('Ctrl Pts',(-10.4729428540001,15.2,-4.28493008200002));
#269762=CARTESIAN_POINT('Ctrl Pts',(-10.4729428540001,11.6,-4.28493008200002));
#269763=CARTESIAN_POINT('Ctrl Pts',(-10.4693725790001,15.2,-4.28503823000002));
#269764=CARTESIAN_POINT('Ctrl Pts',(-10.4693725790001,11.6,-4.28503823000002));
#269765=CARTESIAN_POINT('Ctrl Pts',(-10.4658068880001,15.2,-4.28514346700001));
#269766=CARTESIAN_POINT('Ctrl Pts',(-10.4658068880001,11.6,-4.28514346700002));
#269767=CARTESIAN_POINT('Ctrl Pts',(-10.4622457890001,15.2,-4.28524579800001));
#269768=CARTESIAN_POINT('Ctrl Pts',(-10.4622457890001,11.6,-4.28524579800001));
#269769=CARTESIAN_POINT('Ctrl Pts',(-10.4586892890001,15.2,-4.28534523100002));
#269770=CARTESIAN_POINT('Ctrl Pts',(-10.4586892890001,11.6,-4.28534523100002));
#269771=CARTESIAN_POINT('Ctrl Pts',(-10.4551373970001,15.2,-4.28544177200001));
#269772=CARTESIAN_POINT('Ctrl Pts',(-10.4551373970001,11.6,-4.28544177200001));
#269773=CARTESIAN_POINT('Ctrl Pts',(-10.4515901200001,15.2,-4.28553542300001));
#269774=CARTESIAN_POINT('Ctrl Pts',(-10.4515901200001,11.6,-4.28553542300001));
#269775=CARTESIAN_POINT('Ctrl Pts',(-10.4480474660001,15.2,-4.28562619500001));
#269776=CARTESIAN_POINT('Ctrl Pts',(-10.4480474660001,11.6,-4.28562619500001));
#269777=CARTESIAN_POINT('Ctrl Pts',(-10.4445094430001,15.2,-4.28571409000002));
#269778=CARTESIAN_POINT('Ctrl Pts',(-10.4445094430001,11.6,-4.28571409000002));
#269779=CARTESIAN_POINT('Ctrl Pts',(-10.4409760600001,15.2,-4.28579911600002));
#269780=CARTESIAN_POINT('Ctrl Pts',(-10.4409760600001,11.6,-4.28579911600002));
#269781=CARTESIAN_POINT('Ctrl Pts',(-10.4374473230001,15.2,-4.28588127800001));
#269782=CARTESIAN_POINT('Ctrl Pts',(-10.4374473230001,11.6,-4.28588127800001));
#269783=CARTESIAN_POINT('Ctrl Pts',(-10.4339232400001,15.2,-4.28596058300001));
#269784=CARTESIAN_POINT('Ctrl Pts',(-10.4339232400001,11.6,-4.28596058300002));
#269785=CARTESIAN_POINT('Ctrl Pts',(-10.4304038200001,15.2,-4.28603703500002));
#269786=CARTESIAN_POINT('Ctrl Pts',(-10.4304038200001,11.6,-4.28603703500002));
#269787=CARTESIAN_POINT('Ctrl Pts',(-10.4268890690001,15.2,-4.28611064100001));
#269788=CARTESIAN_POINT('Ctrl Pts',(-10.4268890690001,11.6,-4.28611064100001));
#269789=CARTESIAN_POINT('Ctrl Pts',(-10.4233789970001,15.2,-4.28618140900001));
#269790=CARTESIAN_POINT('Ctrl Pts',(-10.4233789970001,11.6,-4.28618140900001));
#269791=CARTESIAN_POINT('Ctrl Pts',(-10.4198736120001,15.2,-4.28624934200001));
#269792=CARTESIAN_POINT('Ctrl Pts',(-10.4198736120001,11.6,-4.28624934200002));
#269793=CARTESIAN_POINT('Ctrl Pts',(-10.4163729200001,15.2,-4.28631444700001));
#269794=CARTESIAN_POINT('Ctrl Pts',(-10.4163729200001,11.6,-4.28631444700002));
#269795=CARTESIAN_POINT('Ctrl Pts',(-10.4128769310001,15.2,-4.28637673200001));
#269796=CARTESIAN_POINT('Ctrl Pts',(-10.4128769310001,11.6,-4.28637673200001));
#269797=CARTESIAN_POINT('Ctrl Pts',(-10.4093856500001,15.2,-4.28643620000001));
#269798=CARTESIAN_POINT('Ctrl Pts',(-10.4093856500001,11.6,-4.28643620000001));
#269799=CARTESIAN_POINT('Ctrl Pts',(-10.4058990890001,15.2,-4.28649285900002));
#269800=CARTESIAN_POINT('Ctrl Pts',(-10.4058990890001,11.6,-4.28649285900002));
#269801=CARTESIAN_POINT('Ctrl Pts',(-10.4024172520001,15.2,-4.28654671400002));
#269802=CARTESIAN_POINT('Ctrl Pts',(-10.4024172520001,11.6,-4.28654671400002));
#269803=CARTESIAN_POINT('Ctrl Pts',(-10.3989401500001,15.2,-4.28659777200001));
#269804=CARTESIAN_POINT('Ctrl Pts',(-10.3989401500001,11.6,-4.28659777200001));
#269805=CARTESIAN_POINT('Ctrl Pts',(-10.3954677890001,15.2,-4.28664603900001));
#269806=CARTESIAN_POINT('Ctrl Pts',(-10.3954677890001,11.6,-4.28664603900002));
#269807=CARTESIAN_POINT('Ctrl Pts',(-10.3920001780001,15.2,-4.28669152100001));
#269808=CARTESIAN_POINT('Ctrl Pts',(-10.3920001780001,11.6,-4.28669152100001));
#269809=CARTESIAN_POINT('Ctrl Pts',(-10.3885373250001,15.2,-4.28673422400002));
#269810=CARTESIAN_POINT('Ctrl Pts',(-10.3885373250001,11.6,-4.28673422400002));
#269811=CARTESIAN_POINT('Ctrl Pts',(-10.3850792370001,15.2,-4.28677415500001));
#269812=CARTESIAN_POINT('Ctrl Pts',(-10.3850792370001,11.6,-4.28677415500002));
#269813=CARTESIAN_POINT('Ctrl Pts',(-10.3816259240001,15.2,-4.28681132000001));
#269814=CARTESIAN_POINT('Ctrl Pts',(-10.3816259240001,11.6,-4.28681132000001));
#269815=CARTESIAN_POINT('Ctrl Pts',(-10.3781773920001,15.2,-4.28684572300002));
#269816=CARTESIAN_POINT('Ctrl Pts',(-10.3781773920001,11.6,-4.28684572300002));
#269817=CARTESIAN_POINT('Ctrl Pts',(-10.3747336490001,15.2,-4.28687737300002));
#269818=CARTESIAN_POINT('Ctrl Pts',(-10.3747336490001,11.6,-4.28687737300002));
#269819=CARTESIAN_POINT('Ctrl Pts',(-10.3712947050001,15.2,-4.28690627600002));
#269820=CARTESIAN_POINT('Ctrl Pts',(-10.3712947050001,11.6,-4.28690627600002));
#269821=CARTESIAN_POINT('Ctrl Pts',(-10.3678605660001,15.2,-4.28693243800002));
#269822=CARTESIAN_POINT('Ctrl Pts',(-10.3678605660001,11.6,-4.28693243800002));
#269823=CARTESIAN_POINT('Ctrl Pts',(-10.3644312410001,15.2,-4.28695586400002));
#269824=CARTESIAN_POINT('Ctrl Pts',(-10.3644312410001,11.6,-4.28695586400002));
#269825=CARTESIAN_POINT('Ctrl Pts',(-10.3610067390001,15.2,-4.28697656100002));
#269826=CARTESIAN_POINT('Ctrl Pts',(-10.3610067390001,11.6,-4.28697656100002));
#269827=CARTESIAN_POINT('Ctrl Pts',(-10.3575870660001,15.2,-4.28699453700002));
#269828=CARTESIAN_POINT('Ctrl Pts',(-10.3575870660001,11.6,-4.28699453700002));
#269829=CARTESIAN_POINT('Ctrl Pts',(-10.3541722320001,15.2,-4.28700979600002));
#269830=CARTESIAN_POINT('Ctrl Pts',(-10.3541722320001,11.6,-4.28700979600002));
#269831=CARTESIAN_POINT('Ctrl Pts',(-10.3507622440001,15.2,-4.28702234500001));
#269832=CARTESIAN_POINT('Ctrl Pts',(-10.3507622440001,11.6,-4.28702234500001));
#269833=CARTESIAN_POINT('Ctrl Pts',(-10.3473571110001,15.2,-4.28703219200001));
#269834=CARTESIAN_POINT('Ctrl Pts',(-10.3473571110001,11.6,-4.28703219200001));
#269835=CARTESIAN_POINT('Ctrl Pts',(-10.3439568400001,15.2,-4.28703934200001));
#269836=CARTESIAN_POINT('Ctrl Pts',(-10.3439568400001,11.6,-4.28703934200002));
#269837=CARTESIAN_POINT('Ctrl Pts',(-10.3405614400001,15.2,-4.28704380100001));
#269838=CARTESIAN_POINT('Ctrl Pts',(-10.3405614400001,11.6,-4.28704380100002));
#269839=CARTESIAN_POINT('Ctrl Pts',(-10.3371709180001,15.2,-4.28704557600001));
#269840=CARTESIAN_POINT('Ctrl Pts',(-10.3371709180001,11.6,-4.28704557600002));
#269841=CARTESIAN_POINT('Ctrl Pts',(-10.3337852840001,15.2,-4.28704467400001));
#269842=CARTESIAN_POINT('Ctrl Pts',(-10.3337852840001,11.6,-4.28704467400001));
#269843=CARTESIAN_POINT('Ctrl Pts',(-10.3304045450001,15.2,-4.28704110100002));
#269844=CARTESIAN_POINT('Ctrl Pts',(-10.3304045450001,11.6,-4.28704110100002));
#269845=CARTESIAN_POINT('Ctrl Pts',(-10.3270287090001,15.2,-4.28703486400002));
#269846=CARTESIAN_POINT('Ctrl Pts',(-10.3270287090001,11.6,-4.28703486400002));
#269847=CARTESIAN_POINT('Ctrl Pts',(-10.3236577850001,15.2,-4.28702596900001));
#269848=CARTESIAN_POINT('Ctrl Pts',(-10.3236577850001,11.6,-4.28702596900001));
#269849=CARTESIAN_POINT('Ctrl Pts',(-10.3202917800001,15.2,-4.28701442200001));
#269850=CARTESIAN_POINT('Ctrl Pts',(-10.3202917800001,11.6,-4.28701442200001));
#269851=CARTESIAN_POINT('Ctrl Pts',(-10.3169307040001,15.2,-4.28700023100001));
#269852=CARTESIAN_POINT('Ctrl Pts',(-10.3169307040001,11.6,-4.28700023100001));
#269853=CARTESIAN_POINT('Ctrl Pts',(-10.3135745630001,15.2,-4.28698340100001));
#269854=CARTESIAN_POINT('Ctrl Pts',(-10.3135745630001,11.6,-4.28698340100001));
#269855=CARTESIAN_POINT('Ctrl Pts',(-10.3102233670001,15.2,-4.28696394000001));
#269856=CARTESIAN_POINT('Ctrl Pts',(-10.3102233670001,11.6,-4.28696394000002));
#269857=CARTESIAN_POINT('Ctrl Pts',(-10.3068771240001,15.2,-4.28694185400001));
#269858=CARTESIAN_POINT('Ctrl Pts',(-10.3068771240001,11.6,-4.28694185400001));
#269859=CARTESIAN_POINT('Ctrl Pts',(-10.3035358420001,15.2,-4.28691715000001));
#269860=CARTESIAN_POINT('Ctrl Pts',(-10.3035358420001,11.6,-4.28691715000001));
#269861=CARTESIAN_POINT('Ctrl Pts',(-10.3001995280001,15.2,-4.28688983400002));
#269862=CARTESIAN_POINT('Ctrl Pts',(-10.3001995280001,11.6,-4.28688983400002));
#269863=CARTESIAN_POINT('Ctrl Pts',(-10.2968681930001,15.2,-4.28685991300001));
#269864=CARTESIAN_POINT('Ctrl Pts',(-10.2968681930001,11.6,-4.28685991300001));
#269865=CARTESIAN_POINT('Ctrl Pts',(-10.2935418440001,15.2,-4.28682739500001));
#269866=CARTESIAN_POINT('Ctrl Pts',(-10.2935418440001,11.6,-4.28682739500002));
#269867=CARTESIAN_POINT('Ctrl Pts',(-10.2902204880001,15.2,-4.28679228400001));
#269868=CARTESIAN_POINT('Ctrl Pts',(-10.2902204880001,11.6,-4.28679228400001));
#269869=CARTESIAN_POINT('Ctrl Pts',(-10.2869041340001,15.2,-4.28675458900001));
#269870=CARTESIAN_POINT('Ctrl Pts',(-10.2869041340001,11.6,-4.28675458900001));
#269871=CARTESIAN_POINT('Ctrl Pts',(-10.2835927920001,15.2,-4.28671431600002));
#269872=CARTESIAN_POINT('Ctrl Pts',(-10.2835927920001,11.6,-4.28671431600002));
#269873=CARTESIAN_POINT('Ctrl Pts',(-10.2802864670001,15.2,-4.28667147200001));
#269874=CARTESIAN_POINT('Ctrl Pts',(-10.2802864670001,11.6,-4.28667147200002));
#269875=CARTESIAN_POINT('Ctrl Pts',(-10.2769851700001,15.2,-4.28662606300001));
#269876=CARTESIAN_POINT('Ctrl Pts',(-10.2769851700001,11.6,-4.28662606300002));
#269877=CARTESIAN_POINT('Ctrl Pts',(-10.2736889100001,15.2,-4.28657809700002));
#269878=CARTESIAN_POINT('Ctrl Pts',(-10.2736889100001,11.6,-4.28657809700002));
#269879=CARTESIAN_POINT('Ctrl Pts',(-10.2703976930001,15.2,-4.28652758000001));
#269880=CARTESIAN_POINT('Ctrl Pts',(-10.2703976930001,11.6,-4.28652758000002));
#269881=CARTESIAN_POINT('Ctrl Pts',(-10.2671115300001,15.2,-4.28647452000002));
#269882=CARTESIAN_POINT('Ctrl Pts',(-10.2671115300001,11.6,-4.28647452000002));
#269883=CARTESIAN_POINT('Ctrl Pts',(-10.2638304270001,15.2,-4.28641892300002));
#269884=CARTESIAN_POINT('Ctrl Pts',(-10.2638304270001,11.6,-4.28641892300002));
#269885=CARTESIAN_POINT('Ctrl Pts',(-10.2605543930001,15.2,-4.28636079400002));
#269886=CARTESIAN_POINT('Ctrl Pts',(-10.2605543930001,11.6,-4.28636079400002));
#269887=CARTESIAN_POINT('Ctrl Pts',(-10.2572834360001,15.2,-4.28630014400001));
#269888=CARTESIAN_POINT('Ctrl Pts',(-10.2572834360001,11.6,-4.28630014400001));
#269889=CARTESIAN_POINT('Ctrl Pts',(-10.2540175660001,15.2,-4.28623697700001));
#269890=CARTESIAN_POINT('Ctrl Pts',(-10.2540175660001,11.6,-4.28623697700001));
#269891=CARTESIAN_POINT('Ctrl Pts',(-10.2507567900001,15.2,-4.28617130100001));
#269892=CARTESIAN_POINT('Ctrl Pts',(-10.2507567900001,11.6,-4.28617130100002));
#269893=CARTESIAN_POINT('Ctrl Pts',(-10.2475011180001,15.2,-4.28610312300002));
#269894=CARTESIAN_POINT('Ctrl Pts',(-10.2475011180001,11.6,-4.28610312300002));
#269895=CARTESIAN_POINT('Ctrl Pts',(-10.2442505560001,15.2,-4.28603245000001));
#269896=CARTESIAN_POINT('Ctrl Pts',(-10.2442505560001,11.6,-4.28603245000002));
#269897=CARTESIAN_POINT('Ctrl Pts',(-10.2410051150001,15.2,-4.28595928900001));
#269898=CARTESIAN_POINT('Ctrl Pts',(-10.2410051150001,11.6,-4.28595928900002));
#269899=CARTESIAN_POINT('Ctrl Pts',(-10.2377648020001,15.2,-4.28588364700001));
#269900=CARTESIAN_POINT('Ctrl Pts',(-10.2377648020001,11.6,-4.28588364700001));
#269901=CARTESIAN_POINT('Ctrl Pts',(-10.2345296260001,15.2,-4.28580553000002));
#269902=CARTESIAN_POINT('Ctrl Pts',(-10.2345296260001,11.6,-4.28580553000002));
#269903=CARTESIAN_POINT('Ctrl Pts',(-10.2312995950001,15.2,-4.28572494700001));
#269904=CARTESIAN_POINT('Ctrl Pts',(-10.2312995950001,11.6,-4.28572494700001));
#269905=CARTESIAN_POINT('Ctrl Pts',(-10.2280747180001,15.2,-4.28564190400001));
#269906=CARTESIAN_POINT('Ctrl Pts',(-10.2280747180001,11.6,-4.28564190400001));
#269907=CARTESIAN_POINT('Ctrl Pts',(-10.2248550040001,15.2,-4.28555640900001));
#269908=CARTESIAN_POINT('Ctrl Pts',(-10.2248550040001,11.6,-4.28555640900001));
#269909=CARTESIAN_POINT('Ctrl Pts',(-10.2216404610001,15.2,-4.28546846800002));
#269910=CARTESIAN_POINT('Ctrl Pts',(-10.2216404610001,11.6,-4.28546846800002));
#269911=CARTESIAN_POINT('Ctrl Pts',(-10.2184310970001,15.2,-4.28537808900002));
#269912=CARTESIAN_POINT('Ctrl Pts',(-10.2184310970001,11.6,-4.28537808900002));
#269913=CARTESIAN_POINT('Ctrl Pts',(-10.2152269210001,15.2,-4.28528527800002));
#269914=CARTESIAN_POINT('Ctrl Pts',(-10.2152269210001,11.6,-4.28528527800002));
#269915=CARTESIAN_POINT('Ctrl Pts',(-10.2120279420001,15.2,-4.28519004500002));
#269916=CARTESIAN_POINT('Ctrl Pts',(-10.2120279420001,11.6,-4.28519004500002));
#269917=CARTESIAN_POINT('Ctrl Pts',(-10.2088341690001,15.2,-4.28509239400002));
#269918=CARTESIAN_POINT('Ctrl Pts',(-10.2088341690001,11.6,-4.28509239400002));
#269919=CARTESIAN_POINT('Ctrl Pts',(-10.2056456080001,15.2,-4.28499233500002));
#269920=CARTESIAN_POINT('Ctrl Pts',(-10.2056456080001,11.6,-4.28499233500002));
#269921=CARTESIAN_POINT('Ctrl Pts',(-10.2024622710001,15.2,-4.28488987200002));
#269922=CARTESIAN_POINT('Ctrl Pts',(-10.2024622710001,11.6,-4.28488987200002));
#269923=CARTESIAN_POINT('Ctrl Pts',(-10.1992841650001,15.2,-4.28478501600001));
#269924=CARTESIAN_POINT('Ctrl Pts',(-10.1992841650001,11.6,-4.28478501600001));
#269925=CARTESIAN_POINT('Ctrl Pts',(-10.1961112980001,15.2,-4.28467777200002));
#269926=CARTESIAN_POINT('Ctrl Pts',(-10.1961112980001,11.6,-4.28467777200002));
#269927=CARTESIAN_POINT('Ctrl Pts',(-10.1929436800001,15.2,-4.28456814900001));
#269928=CARTESIAN_POINT('Ctrl Pts',(-10.1929436800001,11.6,-4.28456814900002));
#269929=CARTESIAN_POINT('Ctrl Pts',(-10.1897813190001,15.2,-4.28445615300001));
#269930=CARTESIAN_POINT('Ctrl Pts',(-10.1897813190001,11.6,-4.28445615300001));
#269931=CARTESIAN_POINT('Ctrl Pts',(-10.1866242240001,15.2,-4.28434179100002));
#269932=CARTESIAN_POINT('Ctrl Pts',(-10.1866242240001,11.6,-4.28434179100002));
#269933=CARTESIAN_POINT('Ctrl Pts',(-10.1834724030001,15.2,-4.28422507100001));
#269934=CARTESIAN_POINT('Ctrl Pts',(-10.1834724030001,11.6,-4.28422507100001));
#269935=CARTESIAN_POINT('Ctrl Pts',(-10.1803258660001,15.2,-4.28410600200001));
#269936=CARTESIAN_POINT('Ctrl Pts',(-10.1803258660001,11.6,-4.28410600200001));
#269937=CARTESIAN_POINT('Ctrl Pts',(-10.1771846200001,15.2,-4.28398458900002));
#269938=CARTESIAN_POINT('Ctrl Pts',(-10.1771846200001,11.6,-4.28398458900002));
#269939=CARTESIAN_POINT('Ctrl Pts',(-10.1740486750001,15.2,-4.28386084200001));
#269940=CARTESIAN_POINT('Ctrl Pts',(-10.1740486750001,11.6,-4.28386084200001));
#269941=CARTESIAN_POINT('Ctrl Pts',(-10.1709180390001,15.2,-4.28373476600001));
#269942=CARTESIAN_POINT('Ctrl Pts',(-10.1709180390001,11.6,-4.28373476600001));
#269943=CARTESIAN_POINT('Ctrl Pts',(-10.1677927210001,15.2,-4.28360637000001));
#269944=CARTESIAN_POINT('Ctrl Pts',(-10.1677927210001,11.6,-4.28360637000001));
#269945=CARTESIAN_POINT('Ctrl Pts',(-10.1646727300001,15.2,-4.28347566200001));
#269946=CARTESIAN_POINT('Ctrl Pts',(-10.1646727300001,11.6,-4.28347566200001));
#269947=CARTESIAN_POINT('Ctrl Pts',(-10.1615580750001,15.2,-4.28334264800001));
#269948=CARTESIAN_POINT('Ctrl Pts',(-10.1615580750001,11.6,-4.28334264800002));
#269949=CARTESIAN_POINT('Ctrl Pts',(-10.1584487640001,15.2,-4.28320733700001));
#269950=CARTESIAN_POINT('Ctrl Pts',(-10.1584487640001,11.6,-4.28320733700002));
#269951=CARTESIAN_POINT('Ctrl Pts',(-10.1553448070001,15.2,-4.28306973600002));
#269952=CARTESIAN_POINT('Ctrl Pts',(-10.1553448070001,11.6,-4.28306973600002));
#269953=CARTESIAN_POINT('Ctrl Pts',(-10.1522462110001,15.2,-4.28292985300001));
#269954=CARTESIAN_POINT('Ctrl Pts',(-10.1522462110001,11.6,-4.28292985300002));
#269955=CARTESIAN_POINT('Ctrl Pts',(-10.1491529860001,15.2,-4.28278769400002));
#269956=CARTESIAN_POINT('Ctrl Pts',(-10.1491529860001,11.6,-4.28278769400002));
#269957=CARTESIAN_POINT('Ctrl Pts',(-10.1460651410001,15.2,-4.28264327000001));
#269958=CARTESIAN_POINT('Ctrl Pts',(-10.1460651410001,11.6,-4.28264327000001));
#269959=CARTESIAN_POINT('Ctrl Pts',(-10.1429826850001,15.2,-4.28249658600001));
#269960=CARTESIAN_POINT('Ctrl Pts',(-10.1429826850001,11.6,-4.28249658600001));
#269961=CARTESIAN_POINT('Ctrl Pts',(-10.1399056260001,15.2,-4.28234765100001));
#269962=CARTESIAN_POINT('Ctrl Pts',(-10.1399056260001,11.6,-4.28234765100001));
#269963=CARTESIAN_POINT('Ctrl Pts',(-10.1368339730001,15.2,-4.28219647200001));
#269964=CARTESIAN_POINT('Ctrl Pts',(-10.1368339730001,11.6,-4.28219647200002));
#269965=CARTESIAN_POINT('Ctrl Pts',(-10.1337677360001,15.2,-4.28204305800001));
#269966=CARTESIAN_POINT('Ctrl Pts',(-10.1337677360001,11.6,-4.28204305800001));
#269967=CARTESIAN_POINT('Ctrl Pts',(-10.1307069230001,15.2,-4.28188741500001));
#269968=CARTESIAN_POINT('Ctrl Pts',(-10.1307069230001,11.6,-4.28188741500002));
#269969=CARTESIAN_POINT('Ctrl Pts',(-10.1276515430001,15.2,-4.28172955400001));
#269970=CARTESIAN_POINT('Ctrl Pts',(-10.1276515430001,11.6,-4.28172955400001));
#269971=CARTESIAN_POINT('Ctrl Pts',(-10.1246016050001,15.2,-4.28156947900002));
#269972=CARTESIAN_POINT('Ctrl Pts',(-10.1246016050001,11.6,-4.28156947900002));
#269973=CARTESIAN_POINT('Ctrl Pts',(-10.1215571180001,15.2,-4.28140719900002));
#269974=CARTESIAN_POINT('Ctrl Pts',(-10.1215571180001,11.6,-4.28140719900002));
#269975=CARTESIAN_POINT('Ctrl Pts',(-10.1185180900001,15.2,-4.28124272500002));
#269976=CARTESIAN_POINT('Ctrl Pts',(-10.1185180900001,11.6,-4.28124272500002));
#269977=CARTESIAN_POINT('Ctrl Pts',(-10.1154845320001,15.2,-4.28107606000002));
#269978=CARTESIAN_POINT('Ctrl Pts',(-10.1154845320001,11.6,-4.28107606000002));
#269979=CARTESIAN_POINT('Ctrl Pts',(-10.1124564520001,15.2,-4.28090721700002));
#269980=CARTESIAN_POINT('Ctrl Pts',(-10.1124564520001,11.6,-4.28090721700002));
#269981=CARTESIAN_POINT('Ctrl Pts',(-10.1094338590001,15.2,-4.28073619900001));
#269982=CARTESIAN_POINT('Ctrl Pts',(-10.1094338590001,11.6,-4.28073619900002));
#269983=CARTESIAN_POINT('Ctrl Pts',(-10.1064167610001,15.2,-4.28056301800002));
#269984=CARTESIAN_POINT('Ctrl Pts',(-10.1064167610001,11.6,-4.28056301800002));
#269985=CARTESIAN_POINT('Ctrl Pts',(-10.1034051690001,15.2,-4.28038768100001));
#269986=CARTESIAN_POINT('Ctrl Pts',(-10.1034051690001,11.6,-4.28038768100001));
#269987=CARTESIAN_POINT('Ctrl Pts',(-10.1003990900001,15.2,-4.28021019400001));
#269988=CARTESIAN_POINT('Ctrl Pts',(-10.1003990900001,11.6,-4.28021019400001));
#269989=CARTESIAN_POINT('Ctrl Pts',(-10.0973985350001,15.2,-4.28003056800002));
#269990=CARTESIAN_POINT('Ctrl Pts',(-10.0973985350001,11.6,-4.28003056800002));
#269991=CARTESIAN_POINT('Ctrl Pts',(-10.0944035120001,15.2,-4.27984881000001));
#269992=CARTESIAN_POINT('Ctrl Pts',(-10.0944035120001,11.6,-4.27984881000001));
#269993=CARTESIAN_POINT('Ctrl Pts',(-10.0914140300001,15.2,-4.27966492700001));
#269994=CARTESIAN_POINT('Ctrl Pts',(-10.0914140300001,11.6,-4.27966492700001));
#269995=CARTESIAN_POINT('Ctrl Pts',(-10.0884300980001,15.2,-4.27947892900002));
#269996=CARTESIAN_POINT('Ctrl Pts',(-10.0884300980001,11.6,-4.27947892900002));
#269997=CARTESIAN_POINT('Ctrl Pts',(-10.0854517260001,15.2,-4.27929082300002));
#269998=CARTESIAN_POINT('Ctrl Pts',(-10.0854517260001,11.6,-4.27929082300002));
#269999=CARTESIAN_POINT('Ctrl Pts',(-10.0824789230001,15.2,-4.27910061900001));
#270000=CARTESIAN_POINT('Ctrl Pts',(-10.0824789230001,11.6,-4.27910061900001));
#270001=CARTESIAN_POINT('Ctrl Pts',(-10.0795116980001,15.2,-4.27890832200001));
#270002=CARTESIAN_POINT('Ctrl Pts',(-10.0795116980001,11.6,-4.27890832200002));
#270003=CARTESIAN_POINT('Ctrl Pts',(-10.0765500590001,15.2,-4.27871394200002));
#270004=CARTESIAN_POINT('Ctrl Pts',(-10.0765500590001,11.6,-4.27871394200002));
#270005=CARTESIAN_POINT('Ctrl Pts',(-10.0735940170001,15.2,-4.27851748900002));
#270006=CARTESIAN_POINT('Ctrl Pts',(-10.0735940170001,11.6,-4.27851748900002));
#270007=CARTESIAN_POINT('Ctrl Pts',(-10.0706435790001,15.2,-4.27831896900001));
#270008=CARTESIAN_POINT('Ctrl Pts',(-10.0706435790001,11.6,-4.27831896900001));
#270009=CARTESIAN_POINT('Ctrl Pts',(-10.0676987560001,15.2,-4.27811839100002));
#270010=CARTESIAN_POINT('Ctrl Pts',(-10.0676987560001,11.6,-4.27811839100002));
#270011=CARTESIAN_POINT('Ctrl Pts',(-10.0647595580001,15.2,-4.27791576300002));
#270012=CARTESIAN_POINT('Ctrl Pts',(-10.0647595580001,11.6,-4.27791576300002));
#270013=CARTESIAN_POINT('Ctrl Pts',(-10.0618259920001,15.2,-4.27771109500001));
#270014=CARTESIAN_POINT('Ctrl Pts',(-10.0618259920001,11.6,-4.27771109500002));
#270015=CARTESIAN_POINT('Ctrl Pts',(-10.0588980670001,15.2,-4.27750439400001));
#270016=CARTESIAN_POINT('Ctrl Pts',(-10.0588980670001,11.6,-4.27750439400001));
#270017=CARTESIAN_POINT('Ctrl Pts',(-10.0559757960001,15.2,-4.27729566900001));
#270018=CARTESIAN_POINT('Ctrl Pts',(-10.0559757960001,11.6,-4.27729566900002));
#270019=CARTESIAN_POINT('Ctrl Pts',(-10.0530591850001,15.2,-4.27708492700001));
#270020=CARTESIAN_POINT('Ctrl Pts',(-10.0530591850001,11.6,-4.27708492700001));
#270021=CARTESIAN_POINT('Ctrl Pts',(-10.0501482430001,15.2,-4.27687217800001));
#270022=CARTESIAN_POINT('Ctrl Pts',(-10.0501482430001,11.6,-4.27687217800001));
#270023=CARTESIAN_POINT('Ctrl Pts',(-10.0472429820001,15.2,-4.27665743200001));
#270024=CARTESIAN_POINT('Ctrl Pts',(-10.0472429820001,11.6,-4.27665743200001));
#270025=CARTESIAN_POINT('Ctrl Pts',(-10.0443434090001,15.2,-4.27644069400001));
#270026=CARTESIAN_POINT('Ctrl Pts',(-10.0443434090001,11.6,-4.27644069400001));
#270027=CARTESIAN_POINT('Ctrl Pts',(-10.0414495340001,15.2,-4.27622197600002));
#270028=CARTESIAN_POINT('Ctrl Pts',(-10.0414495340001,11.6,-4.27622197600002));
#270029=CARTESIAN_POINT('Ctrl Pts',(-10.0385613660001,15.2,-4.27600128400002));
#270030=CARTESIAN_POINT('Ctrl Pts',(-10.0385613660001,11.6,-4.27600128400002));
#270031=CARTESIAN_POINT('Ctrl Pts',(-10.0356789150001,15.2,-4.27577862800002));
#270032=CARTESIAN_POINT('Ctrl Pts',(-10.0356789150001,11.6,-4.27577862800002));
#270033=CARTESIAN_POINT('Ctrl Pts',(-10.0328021910001,15.2,-4.27555401600001));
#270034=CARTESIAN_POINT('Ctrl Pts',(-10.0328021910001,11.6,-4.27555401600001));
#270035=CARTESIAN_POINT('Ctrl Pts',(-10.0299312030001,15.2,-4.27532745800002));
#270036=CARTESIAN_POINT('Ctrl Pts',(-10.0299312030001,11.6,-4.27532745800002));
#270037=CARTESIAN_POINT('Ctrl Pts',(-10.0270659590001,15.2,-4.27509896100001));
#270038=CARTESIAN_POINT('Ctrl Pts',(-10.0270659590001,11.6,-4.27509896100002));
#270039=CARTESIAN_POINT('Ctrl Pts',(-10.0242064700001,15.2,-4.27486853600001));
#270040=CARTESIAN_POINT('Ctrl Pts',(-10.0242064700001,11.6,-4.27486853600001));
#270041=CARTESIAN_POINT('Ctrl Pts',(-10.0213527440001,15.2,-4.27463618900001));
#270042=CARTESIAN_POINT('Ctrl Pts',(-10.0213527440001,11.6,-4.27463618900001));
#270043=CARTESIAN_POINT('Ctrl Pts',(-10.0185047920001,15.2,-4.27440193000002));
#270044=CARTESIAN_POINT('Ctrl Pts',(-10.0185047920001,11.6,-4.27440193000002));
#270045=CARTESIAN_POINT('Ctrl Pts',(-10.0156626230001,15.2,-4.27416576900002));
#270046=CARTESIAN_POINT('Ctrl Pts',(-10.0156626230001,11.6,-4.27416576900002));
#270047=CARTESIAN_POINT('Ctrl Pts',(-10.0128262460001,15.2,-4.27392771400001));
#270048=CARTESIAN_POINT('Ctrl Pts',(-10.0128262460001,11.6,-4.27392771400002));
#270049=CARTESIAN_POINT('Ctrl Pts',(-10.0099956720001,15.2,-4.27368777300002));
#270050=CARTESIAN_POINT('Ctrl Pts',(-10.0099956720001,11.6,-4.27368777300002));
#270051=CARTESIAN_POINT('Ctrl Pts',(-10.0071709090001,15.2,-4.27344595700001));
#270052=CARTESIAN_POINT('Ctrl Pts',(-10.0071709090001,11.6,-4.27344595700002));
#270053=CARTESIAN_POINT('Ctrl Pts',(-10.0043519670001,15.2,-4.27320227300001));
#270054=CARTESIAN_POINT('Ctrl Pts',(-10.0043519670001,11.6,-4.27320227300001));
#270055=CARTESIAN_POINT('Ctrl Pts',(-10.0015388550001,15.2,-4.27295673000001));
#270056=CARTESIAN_POINT('Ctrl Pts',(-10.0015388550001,11.6,-4.27295673000002));
#270057=CARTESIAN_POINT('Ctrl Pts',(-9.99873158400005,15.2,-4.27270933800001));
#270058=CARTESIAN_POINT('Ctrl Pts',(-9.99873158400005,11.6,-4.27270933800001));
#270059=CARTESIAN_POINT('Ctrl Pts',(-9.99593016200006,15.2,-4.27246010600001));
#270060=CARTESIAN_POINT('Ctrl Pts',(-9.99593016200006,11.6,-4.27246010600001));
#270061=CARTESIAN_POINT('Ctrl Pts',(-9.99313460000005,15.2,-4.27220904400002));
#270062=CARTESIAN_POINT('Ctrl Pts',(-9.99313460000005,11.6,-4.27220904400002));
#270063=CARTESIAN_POINT('Ctrl Pts',(-9.99034490700006,15.2,-4.27195615900001));
#270064=CARTESIAN_POINT('Ctrl Pts',(-9.99034490700006,11.6,-4.27195615900002));
#270065=CARTESIAN_POINT('Ctrl Pts',(-9.98756109300006,15.2,-4.27170146000002));
#270066=CARTESIAN_POINT('Ctrl Pts',(-9.98756109300006,11.6,-4.27170146000002));
#270067=CARTESIAN_POINT('Ctrl Pts',(-9.98478316600006,15.2,-4.27144495800002));
#270068=CARTESIAN_POINT('Ctrl Pts',(-9.98478316600006,11.6,-4.27144495800002));
#270069=CARTESIAN_POINT('Ctrl Pts',(-9.98201113900006,15.2,-4.27118666200001));
#270070=CARTESIAN_POINT('Ctrl Pts',(-9.98201113900006,11.6,-4.27118666200002));
#270071=CARTESIAN_POINT('Ctrl Pts',(-9.97924501800006,15.2,-4.27092658000001));
#270072=CARTESIAN_POINT('Ctrl Pts',(-9.97924501800006,11.6,-4.27092658000001));
#270073=CARTESIAN_POINT('Ctrl Pts',(-9.97648481500006,15.2,-4.27066472200002));
#270074=CARTESIAN_POINT('Ctrl Pts',(-9.97648481500006,11.6,-4.27066472200002));
#270075=CARTESIAN_POINT('Ctrl Pts',(-9.97373054000006,15.2,-4.27040109700001));
#270076=CARTESIAN_POINT('Ctrl Pts',(-9.97373054000006,11.6,-4.27040109700001));
#270077=CARTESIAN_POINT('Ctrl Pts',(-9.97098220100006,15.2,-4.27013571500002));
#270078=CARTESIAN_POINT('Ctrl Pts',(-9.97098220100006,11.6,-4.27013571500002));
#270079=CARTESIAN_POINT('Ctrl Pts',(-9.96823980900006,15.2,-4.26986858400001));
#270080=CARTESIAN_POINT('Ctrl Pts',(-9.96823980900006,11.6,-4.26986858400001));
#270081=CARTESIAN_POINT('Ctrl Pts',(-9.96550337400006,15.2,-4.26959971500001));
#270082=CARTESIAN_POINT('Ctrl Pts',(-9.96550337400006,11.6,-4.26959971500002));
#270083=CARTESIAN_POINT('Ctrl Pts',(-9.96277290400006,15.2,-4.26932911600002));
#270084=CARTESIAN_POINT('Ctrl Pts',(-9.96277290400006,11.6,-4.26932911600002));
#270085=CARTESIAN_POINT('Ctrl Pts',(-9.96004841100006,15.2,-4.26905679700001));
#270086=CARTESIAN_POINT('Ctrl Pts',(-9.96004841100006,11.6,-4.26905679700001));
#270087=CARTESIAN_POINT('Ctrl Pts',(-9.95732990400005,15.2,-4.26878276700001));
#270088=CARTESIAN_POINT('Ctrl Pts',(-9.95732990400005,11.6,-4.26878276700002));
#270089=CARTESIAN_POINT('Ctrl Pts',(-9.95461739200006,15.2,-4.26850703700001));
#270090=CARTESIAN_POINT('Ctrl Pts',(-9.95461739200006,11.6,-4.26850703700001));
#270091=CARTESIAN_POINT('Ctrl Pts',(-9.95191088700006,15.2,-4.26822961500001));
#270092=CARTESIAN_POINT('Ctrl Pts',(-9.95191088700006,11.6,-4.26822961500002));
#270093=CARTESIAN_POINT('Ctrl Pts',(-9.94921039800006,15.2,-4.26795051200001));
#270094=CARTESIAN_POINT('Ctrl Pts',(-9.94921039800006,11.6,-4.26795051200001));
#270095=CARTESIAN_POINT('Ctrl Pts',(-9.94651593300006,15.2,-4.26766973600001));
#270096=CARTESIAN_POINT('Ctrl Pts',(-9.94651593300006,11.6,-4.26766973600001));
#270097=CARTESIAN_POINT('Ctrl Pts',(-9.94382750400005,15.2,-4.26738729700002));
#270098=CARTESIAN_POINT('Ctrl Pts',(-9.94382750400005,11.6,-4.26738729700002));
#270099=CARTESIAN_POINT('Ctrl Pts',(-9.94114512000005,15.2,-4.26710320400002));
#270100=CARTESIAN_POINT('Ctrl Pts',(-9.94114512000005,11.6,-4.26710320400002));
#270101=CARTESIAN_POINT('Ctrl Pts',(-9.93846879200006,15.2,-4.26681746900002));
#270102=CARTESIAN_POINT('Ctrl Pts',(-9.93846879200006,11.6,-4.26681746900002));
#270103=CARTESIAN_POINT('Ctrl Pts',(-9.93579852900006,15.2,-4.26653010000001));
#270104=CARTESIAN_POINT('Ctrl Pts',(-9.93579852900006,11.6,-4.26653010000001));
#270105=CARTESIAN_POINT('Ctrl Pts',(-9.93313434200006,15.2,-4.26624110700002));
#270106=CARTESIAN_POINT('Ctrl Pts',(-9.93313434200006,11.6,-4.26624110700002));
#270107=CARTESIAN_POINT('Ctrl Pts',(-9.93047624000006,15.2,-4.26595050000001));
#270108=CARTESIAN_POINT('Ctrl Pts',(-9.93047624000006,11.6,-4.26595050000001));
#270109=CARTESIAN_POINT('Ctrl Pts',(-9.92782423400006,15.2,-4.26565828900001));
#270110=CARTESIAN_POINT('Ctrl Pts',(-9.92782423400006,11.6,-4.26565828900001));
#270111=CARTESIAN_POINT('Ctrl Pts',(-9.92517833200005,15.2,-4.26536448200002));
#270112=CARTESIAN_POINT('Ctrl Pts',(-9.92517833200005,11.6,-4.26536448200002));
#270113=CARTESIAN_POINT('Ctrl Pts',(-9.92253854700006,15.2,-4.26506909300001));
#270114=CARTESIAN_POINT('Ctrl Pts',(-9.92253854700006,11.6,-4.26506909300001));
#270115=CARTESIAN_POINT('Ctrl Pts',(-9.91990488700005,15.2,-4.26477212700001));
#270116=CARTESIAN_POINT('Ctrl Pts',(-9.91990488700005,11.6,-4.26477212700001));
#270117=CARTESIAN_POINT('Ctrl Pts',(-9.91727736300006,15.2,-4.26447359700001));
#270118=CARTESIAN_POINT('Ctrl Pts',(-9.91727736300006,11.6,-4.26447359700001));
#270119=CARTESIAN_POINT('Ctrl Pts',(-9.91465598400006,15.2,-4.26417351200001));
#270120=CARTESIAN_POINT('Ctrl Pts',(-9.91465598400006,11.6,-4.26417351200001));
#270121=CARTESIAN_POINT('Ctrl Pts',(-9.91204076300006,15.2,-4.26387188200001));
#270122=CARTESIAN_POINT('Ctrl Pts',(-9.91204076300006,11.6,-4.26387188200002));
#270123=CARTESIAN_POINT('Ctrl Pts',(-9.90943170700006,15.2,-4.26356871900001));
#270124=CARTESIAN_POINT('Ctrl Pts',(-9.90943170700006,11.6,-4.26356871900001));
#270125=CARTESIAN_POINT('Ctrl Pts',(-9.90682882700006,15.2,-4.26326402900001));
#270126=CARTESIAN_POINT('Ctrl Pts',(-9.90682882700006,11.6,-4.26326402900001));
#270127=CARTESIAN_POINT('Ctrl Pts',(-9.90423213500006,15.2,-4.26295782600001));
#270128=CARTESIAN_POINT('Ctrl Pts',(-9.90423213500006,11.6,-4.26295782600001));
#270129=CARTESIAN_POINT('Ctrl Pts',(-9.90164163800006,15.2,-4.26265011800002));
#270130=CARTESIAN_POINT('Ctrl Pts',(-9.90164163800006,11.6,-4.26265011800002));
#270131=CARTESIAN_POINT('Ctrl Pts',(-9.89905735000006,15.2,-4.26234091600001));
#270132=CARTESIAN_POINT('Ctrl Pts',(-9.89905735000006,11.6,-4.26234091600001));
#270133=CARTESIAN_POINT('Ctrl Pts',(-9.89647927900006,15.2,-4.26203023000001));
#270134=CARTESIAN_POINT('Ctrl Pts',(-9.89647927900006,11.6,-4.26203023000001));
#270135=CARTESIAN_POINT('Ctrl Pts',(-9.89390743400006,15.2,-4.26171807000001));
#270136=CARTESIAN_POINT('Ctrl Pts',(-9.89390743400006,11.6,-4.26171807000001));
#270137=CARTESIAN_POINT('Ctrl Pts',(-9.89134182900005,15.2,-4.26140444800001));
#270138=CARTESIAN_POINT('Ctrl Pts',(-9.89134182900005,11.6,-4.26140444800002));
#270139=CARTESIAN_POINT('Ctrl Pts',(-9.88878247200006,15.2,-4.26108937200001));
#270140=CARTESIAN_POINT('Ctrl Pts',(-9.88878247200006,11.6,-4.26108937200001));
#270141=CARTESIAN_POINT('Ctrl Pts',(-9.88622937300006,15.2,-4.26077285200002));
#270142=CARTESIAN_POINT('Ctrl Pts',(-9.88622937300006,11.6,-4.26077285200002));
#270143=CARTESIAN_POINT('Ctrl Pts',(-9.88368254300006,15.2,-4.26045490100002));
#270144=CARTESIAN_POINT('Ctrl Pts',(-9.88368254300006,11.6,-4.26045490100002));
#270145=CARTESIAN_POINT('Ctrl Pts',(-9.88114199400006,15.2,-4.26013552700002));
#270146=CARTESIAN_POINT('Ctrl Pts',(-9.88114199400006,11.6,-4.26013552700002));
#270147=CARTESIAN_POINT('Ctrl Pts',(-9.87860773400006,15.2,-4.25981474300002));
#270148=CARTESIAN_POINT('Ctrl Pts',(-9.87860773400006,11.6,-4.25981474300002));
#270149=CARTESIAN_POINT('Ctrl Pts',(-9.87607977400006,15.2,-4.25949255600001));
#270150=CARTESIAN_POINT('Ctrl Pts',(-9.87607977400006,11.6,-4.25949255600001));
#270151=CARTESIAN_POINT('Ctrl Pts',(-9.87355812500006,15.2,-4.25916898000001));
#270152=CARTESIAN_POINT('Ctrl Pts',(-9.87355812500006,11.6,-4.25916898000002));
#270153=CARTESIAN_POINT('Ctrl Pts',(-9.87104279700005,15.2,-4.25884402400001));
#270154=CARTESIAN_POINT('Ctrl Pts',(-9.87104279700005,11.6,-4.25884402400001));
#270155=CARTESIAN_POINT('Ctrl Pts',(-9.86853380100005,15.2,-4.25851769800001));
#270156=CARTESIAN_POINT('Ctrl Pts',(-9.86853380100005,11.6,-4.25851769800001));
#270157=CARTESIAN_POINT('Ctrl Pts',(-9.86603114800005,15.2,-4.25819001500002));
#270158=CARTESIAN_POINT('Ctrl Pts',(-9.86603114800005,11.6,-4.25819001500002));
#270159=CARTESIAN_POINT('Ctrl Pts',(-9.86353484600006,15.2,-4.25786098200001));
#270160=CARTESIAN_POINT('Ctrl Pts',(-9.86353484600006,11.6,-4.25786098200002));
#270161=CARTESIAN_POINT('Ctrl Pts',(-9.86104490900006,15.2,-4.25753061300002));
#270162=CARTESIAN_POINT('Ctrl Pts',(-9.86104490900006,11.6,-4.25753061300002));
#270163=CARTESIAN_POINT('Ctrl Pts',(-9.85856134500006,15.2,-4.25719891600002));
#270164=CARTESIAN_POINT('Ctrl Pts',(-9.85856134500006,11.6,-4.25719891600002));
#270165=CARTESIAN_POINT('Ctrl Pts',(-9.85608416600006,15.2,-4.25686590500002));
#270166=CARTESIAN_POINT('Ctrl Pts',(-9.85608416600006,11.6,-4.25686590500002));
#270167=CARTESIAN_POINT('Ctrl Pts',(-9.85361338300006,15.2,-4.25653158900001));
#270168=CARTESIAN_POINT('Ctrl Pts',(-9.85361338300006,11.6,-4.25653158900001));
#270169=CARTESIAN_POINT('Ctrl Pts',(-9.85114900400006,15.2,-4.25619597800001));
#270170=CARTESIAN_POINT('Ctrl Pts',(-9.85114900400006,11.6,-4.25619597800001));
#270171=CARTESIAN_POINT('Ctrl Pts',(-9.84869104300006,15.2,-4.25585908400001));
#270172=CARTESIAN_POINT('Ctrl Pts',(-9.84869104300006,11.6,-4.25585908400001));
#270173=CARTESIAN_POINT('Ctrl Pts',(-9.84623950900006,15.2,-4.25552091800002));
#270174=CARTESIAN_POINT('Ctrl Pts',(-9.84623950900006,11.6,-4.25552091800002));
#270175=CARTESIAN_POINT('Ctrl Pts',(-9.84379441200005,15.2,-4.25518149100002));
#270176=CARTESIAN_POINT('Ctrl Pts',(-9.84379441200005,11.6,-4.25518149100002));
#270177=CARTESIAN_POINT('Ctrl Pts',(-9.84135576400006,15.2,-4.25484081400001));
#270178=CARTESIAN_POINT('Ctrl Pts',(-9.84135576400006,11.6,-4.25484081400001));
#270179=CARTESIAN_POINT('Ctrl Pts',(-9.83892357600006,15.2,-4.25449889700001));
#270180=CARTESIAN_POINT('Ctrl Pts',(-9.83892357600006,11.6,-4.25449889700001));
#270181=CARTESIAN_POINT('Ctrl Pts',(-9.83649785800005,15.2,-4.25415575300002));
#270182=CARTESIAN_POINT('Ctrl Pts',(-9.83649785800005,11.6,-4.25415575300002));
#270183=CARTESIAN_POINT('Ctrl Pts',(-9.83407862100006,15.2,-4.25381139100002));
#270184=CARTESIAN_POINT('Ctrl Pts',(-9.83407862100006,11.6,-4.25381139100002));
#270185=CARTESIAN_POINT('Ctrl Pts',(-9.83166587600006,15.2,-4.25346582400001));
#270186=CARTESIAN_POINT('Ctrl Pts',(-9.83166587600006,11.6,-4.25346582400001));
#270187=CARTESIAN_POINT('Ctrl Pts',(-9.82925963200006,15.2,-4.25311906200001));
#270188=CARTESIAN_POINT('Ctrl Pts',(-9.82925963200006,11.6,-4.25311906200002));
#270189=CARTESIAN_POINT('Ctrl Pts',(-9.82685990300006,15.2,-4.25277111600002));
#270190=CARTESIAN_POINT('Ctrl Pts',(-9.82685990300006,11.6,-4.25277111600002));
#270191=CARTESIAN_POINT('Ctrl Pts',(-9.82446669800006,15.2,-4.25242200000001));
#270192=CARTESIAN_POINT('Ctrl Pts',(-9.82446669800006,11.6,-4.25242200000001));
#270193=CARTESIAN_POINT('Ctrl Pts',(-9.82208002800006,15.2,-4.25207172100002));
#270194=CARTESIAN_POINT('Ctrl Pts',(-9.82208002800006,11.6,-4.25207172100002));
#270195=CARTESIAN_POINT('Ctrl Pts',(-9.81969990500006,15.2,-4.25172029500001));
#270196=CARTESIAN_POINT('Ctrl Pts',(-9.81969990500006,11.6,-4.25172029500002));
#270197=CARTESIAN_POINT('Ctrl Pts',(-9.81732633900006,15.2,-4.25136772900002));
#270198=CARTESIAN_POINT('Ctrl Pts',(-9.81732633900006,11.6,-4.25136772900002));
#270199=CARTESIAN_POINT('Ctrl Pts',(-9.81495934200005,15.2,-4.25101403800001));
#270200=CARTESIAN_POINT('Ctrl Pts',(-9.81495934200005,11.6,-4.25101403800001));
#270201=CARTESIAN_POINT('Ctrl Pts',(-9.81259892300006,15.2,-4.25065923100002));
#270202=CARTESIAN_POINT('Ctrl Pts',(-9.81259892300006,11.6,-4.25065923100002));
#270203=CARTESIAN_POINT('Ctrl Pts',(-9.81024509500006,15.2,-4.25030332100001));
#270204=CARTESIAN_POINT('Ctrl Pts',(-9.81024509500006,11.6,-4.25030332100001));
#270205=CARTESIAN_POINT('Ctrl Pts',(-9.80789786800005,15.2,-4.24994631800002));
#270206=CARTESIAN_POINT('Ctrl Pts',(-9.80789786800005,11.6,-4.24994631800002));
#270207=CARTESIAN_POINT('Ctrl Pts',(-9.80555725300006,15.2,-4.24958823700001));
#270208=CARTESIAN_POINT('Ctrl Pts',(-9.80555725300006,11.6,-4.24958823700001));
#270209=CARTESIAN_POINT('Ctrl Pts',(-9.80322326200006,15.2,-4.24922908500001));
#270210=CARTESIAN_POINT('Ctrl Pts',(-9.80322326200006,11.6,-4.24922908500002));
#270211=CARTESIAN_POINT('Ctrl Pts',(-9.80089590600006,15.2,-4.24886887800001));
#270212=CARTESIAN_POINT('Ctrl Pts',(-9.80089590600006,11.6,-4.24886887800001));
#270213=CARTESIAN_POINT('Ctrl Pts',(-9.79857519500005,15.2,-4.24850762500002));
#270214=CARTESIAN_POINT('Ctrl Pts',(-9.79857519500005,11.6,-4.24850762500002));
#270215=CARTESIAN_POINT('Ctrl Pts',(-9.79626114100006,15.2,-4.24814533800001));
#270216=CARTESIAN_POINT('Ctrl Pts',(-9.79626114100006,11.6,-4.24814533800001));
#270217=CARTESIAN_POINT('Ctrl Pts',(-9.79395375600006,15.2,-4.24778203100002));
#270218=CARTESIAN_POINT('Ctrl Pts',(-9.79395375600006,11.6,-4.24778203100002));
#270219=CARTESIAN_POINT('Ctrl Pts',(-9.79165305000006,15.2,-4.24741771300001));
#270220=CARTESIAN_POINT('Ctrl Pts',(-9.79165305000006,11.6,-4.24741771300001));
#270221=CARTESIAN_POINT('Ctrl Pts',(-9.78935903500006,15.2,-4.24705239700002));
#270222=CARTESIAN_POINT('Ctrl Pts',(-9.78935903500006,11.6,-4.24705239700002));
#270223=CARTESIAN_POINT('Ctrl Pts',(-9.78707172100006,15.2,-4.24668609500001));
#270224=CARTESIAN_POINT('Ctrl Pts',(-9.78707172100006,11.6,-4.24668609500001));
#270225=CARTESIAN_POINT('Ctrl Pts',(-9.78479112100005,15.2,-4.24631882000002));
#270226=CARTESIAN_POINT('Ctrl Pts',(-9.78479112100005,11.6,-4.24631882000002));
#270227=CARTESIAN_POINT('Ctrl Pts',(-9.78251724500005,15.2,-4.24595058300001));
#270228=CARTESIAN_POINT('Ctrl Pts',(-9.78251724500005,11.6,-4.24595058300001));
#270229=CARTESIAN_POINT('Ctrl Pts',(-9.78025010600006,15.2,-4.24558139600002));
#270230=CARTESIAN_POINT('Ctrl Pts',(-9.78025010600006,11.6,-4.24558139600002));
#270231=CARTESIAN_POINT('Ctrl Pts',(-9.77798971300006,15.2,-4.24521127100002));
#270232=CARTESIAN_POINT('Ctrl Pts',(-9.77798971300006,11.6,-4.24521127100002));
#270233=CARTESIAN_POINT('Ctrl Pts',(-9.77573607900006,15.2,-4.24484022000001));
#270234=CARTESIAN_POINT('Ctrl Pts',(-9.77573607900006,11.6,-4.24484022000002));
#270235=CARTESIAN_POINT('Ctrl Pts',(-9.77348921600005,15.2,-4.24446825700001));
#270236=CARTESIAN_POINT('Ctrl Pts',(-9.77348921600005,11.6,-4.24446825700001));
#270237=CARTESIAN_POINT('Ctrl Pts',(-9.77124913500005,15.2,-4.24409539200001));
#270238=CARTESIAN_POINT('Ctrl Pts',(-9.77124913500005,11.6,-4.24409539200001));
#270239=CARTESIAN_POINT('Ctrl Pts',(-9.76901584600006,15.2,-4.24372163900001));
#270240=CARTESIAN_POINT('Ctrl Pts',(-9.76901584600006,11.6,-4.24372163900001));
#270241=CARTESIAN_POINT('Ctrl Pts',(-9.76678936200006,15.2,-4.24334700900001));
#270242=CARTESIAN_POINT('Ctrl Pts',(-9.76678936200006,11.6,-4.24334700900001));
#270243=CARTESIAN_POINT('Ctrl Pts',(-9.76456969400006,15.2,-4.24297151500001));
#270244=CARTESIAN_POINT('Ctrl Pts',(-9.76456969400006,11.6,-4.24297151500001));
#270245=CARTESIAN_POINT('Ctrl Pts',(-9.76235685400006,15.2,-4.24259517000001));
#270246=CARTESIAN_POINT('Ctrl Pts',(-9.76235685400006,11.6,-4.24259517000001));
#270247=CARTESIAN_POINT('Ctrl Pts',(-9.76015085200006,15.2,-4.24221798600001));
#270248=CARTESIAN_POINT('Ctrl Pts',(-9.76015085200006,11.6,-4.24221798600002));
#270249=CARTESIAN_POINT('Ctrl Pts',(-9.75795170300006,15.2,-4.24183997400001));
#270250=CARTESIAN_POINT('Ctrl Pts',(-9.75795170300006,11.6,-4.24183997400002));
#270251=CARTESIAN_POINT('Ctrl Pts',(-9.75575941400006,15.2,-4.24146115000001));
#270252=CARTESIAN_POINT('Ctrl Pts',(-9.75575941400006,11.6,-4.24146115000002));
#270253=CARTESIAN_POINT('Ctrl Pts',(-9.75357400200006,15.2,-4.24108152300001));
#270254=CARTESIAN_POINT('Ctrl Pts',(-9.75357400200006,11.6,-4.24108152300002));
#270255=CARTESIAN_POINT('Ctrl Pts',(-9.75139547400006,15.2,-4.24070110800002));
#270256=CARTESIAN_POINT('Ctrl Pts',(-9.75139547400006,11.6,-4.24070110800002));
#270257=CARTESIAN_POINT('Ctrl Pts',(-9.74922384500006,15.2,-4.24031991600001));
#270258=CARTESIAN_POINT('Ctrl Pts',(-9.74922384500006,11.6,-4.24031991600002));
#270259=CARTESIAN_POINT('Ctrl Pts',(-9.74705912500006,15.2,-4.23993796200001));
#270260=CARTESIAN_POINT('Ctrl Pts',(-9.74705912500006,11.6,-4.23993796200001));
#270261=CARTESIAN_POINT('Ctrl Pts',(-9.74490132600006,15.2,-4.23955525700002));
#270262=CARTESIAN_POINT('Ctrl Pts',(-9.74490132600006,11.6,-4.23955525700002));
#270263=CARTESIAN_POINT('Ctrl Pts',(-9.74275046000006,15.2,-4.23917181500002));
#270264=CARTESIAN_POINT('Ctrl Pts',(-9.74275046000006,11.6,-4.23917181500002));
#270265=CARTESIAN_POINT('Ctrl Pts',(-9.74060653900005,15.2,-4.23878764800001));
#270266=CARTESIAN_POINT('Ctrl Pts',(-9.74060653900005,11.6,-4.23878764800001));
#270267=CARTESIAN_POINT('Ctrl Pts',(-9.73846957500006,15.2,-4.23840276900001));
#270268=CARTESIAN_POINT('Ctrl Pts',(-9.73846957500006,11.6,-4.23840276900001));
#270269=CARTESIAN_POINT('Ctrl Pts',(-9.73633957900006,15.2,-4.23801719200001));
#270270=CARTESIAN_POINT('Ctrl Pts',(-9.73633957900006,11.6,-4.23801719200002));
#270271=CARTESIAN_POINT('Ctrl Pts',(-9.73421656400006,15.2,-4.23763092800002));
#270272=CARTESIAN_POINT('Ctrl Pts',(-9.73421656400006,11.6,-4.23763092800002));
#270273=CARTESIAN_POINT('Ctrl Pts',(-9.73210054100005,15.2,-4.23724399300001));
#270274=CARTESIAN_POINT('Ctrl Pts',(-9.73210054100005,11.6,-4.23724399300002));
#270275=CARTESIAN_POINT('Ctrl Pts',(-9.72999152300006,15.2,-4.23685639700001));
#270276=CARTESIAN_POINT('Ctrl Pts',(-9.72999152300006,11.6,-4.23685639700001));
#270277=CARTESIAN_POINT('Ctrl Pts',(-9.72788952300006,15.2,-4.23646815600002));
#270278=CARTESIAN_POINT('Ctrl Pts',(-9.72788952300006,11.6,-4.23646815600002));
#270279=CARTESIAN_POINT('Ctrl Pts',(-9.72579454900006,15.2,-4.23607928100001));
#270280=CARTESIAN_POINT('Ctrl Pts',(-9.72579454900006,11.6,-4.23607928100001));
#270281=CARTESIAN_POINT('Ctrl Pts',(-9.72370661700005,15.2,-4.23568978700001));
#270282=CARTESIAN_POINT('Ctrl Pts',(-9.72370661700005,11.6,-4.23568978700002));
#270283=CARTESIAN_POINT('Ctrl Pts',(-9.72162573800006,15.2,-4.23529968600001));
#270284=CARTESIAN_POINT('Ctrl Pts',(-9.72162573800006,11.6,-4.23529968600001));
#270285=CARTESIAN_POINT('Ctrl Pts',(-9.71955192300006,15.2,-4.23490899300001));
#270286=CARTESIAN_POINT('Ctrl Pts',(-9.71955192300006,11.6,-4.23490899300001));
#270287=CARTESIAN_POINT('Ctrl Pts',(-9.71748518600006,15.2,-4.23451771900002));
#270288=CARTESIAN_POINT('Ctrl Pts',(-9.71748518600006,11.6,-4.23451771900002));
#270289=CARTESIAN_POINT('Ctrl Pts',(-9.71542553800005,15.2,-4.23412588100001));
#270290=CARTESIAN_POINT('Ctrl Pts',(-9.71542553800005,11.6,-4.23412588100002));
#270291=CARTESIAN_POINT('Ctrl Pts',(-9.71337299100006,15.2,-4.23373348900002));
#270292=CARTESIAN_POINT('Ctrl Pts',(-9.71337299100006,11.6,-4.23373348900002));
#270293=CARTESIAN_POINT('Ctrl Pts',(-9.71132755700006,15.2,-4.23334055800002));
#270294=CARTESIAN_POINT('Ctrl Pts',(-9.71132755700006,11.6,-4.23334055800002));
#270295=CARTESIAN_POINT('Ctrl Pts',(-9.70928925100005,15.2,-4.23294710300001));
#270296=CARTESIAN_POINT('Ctrl Pts',(-9.70928925100005,11.6,-4.23294710300001));
#270297=CARTESIAN_POINT('Ctrl Pts',(-9.70725808200006,15.2,-4.23255313500002));
#270298=CARTESIAN_POINT('Ctrl Pts',(-9.70725808200006,11.6,-4.23255313500002));
#270299=CARTESIAN_POINT('Ctrl Pts',(-9.70523406400006,15.2,-4.23215867100001));
#270300=CARTESIAN_POINT('Ctrl Pts',(-9.70523406400006,11.6,-4.23215867100002));
#270301=CARTESIAN_POINT('Ctrl Pts',(-9.70321720900006,15.2,-4.23176372200002));
#270302=CARTESIAN_POINT('Ctrl Pts',(-9.70321720900006,11.6,-4.23176372200002));
#270303=CARTESIAN_POINT('Ctrl Pts',(-9.70120753000005,15.2,-4.23136830300002));
#270304=CARTESIAN_POINT('Ctrl Pts',(-9.70120753000005,11.6,-4.23136830300002));
#270305=CARTESIAN_POINT('Ctrl Pts',(-9.69920503800006,15.2,-4.23097242800001));
#270306=CARTESIAN_POINT('Ctrl Pts',(-9.69920503800006,11.6,-4.23097242800001));
#270307=CARTESIAN_POINT('Ctrl Pts',(-9.69720974700006,15.2,-4.23057611000001));
#270308=CARTESIAN_POINT('Ctrl Pts',(-9.69720974700006,11.6,-4.23057611000001));
#270309=CARTESIAN_POINT('Ctrl Pts',(-9.69522166900006,15.2,-4.23017936500001));
#270310=CARTESIAN_POINT('Ctrl Pts',(-9.69522166900006,11.6,-4.23017936500001));
#270311=CARTESIAN_POINT('Ctrl Pts',(-9.69324081600006,15.2,-4.22978220500001));
#270312=CARTESIAN_POINT('Ctrl Pts',(-9.69324081600006,11.6,-4.22978220500002));
#270313=CARTESIAN_POINT('Ctrl Pts',(-9.69126720200006,15.2,-4.22938464600001));
#270314=CARTESIAN_POINT('Ctrl Pts',(-9.69126720200006,11.6,-4.22938464600001));
#270315=CARTESIAN_POINT('Ctrl Pts',(-9.68930083800006,15.2,-4.22898670000002));
#270316=CARTESIAN_POINT('Ctrl Pts',(-9.68930083800006,11.6,-4.22898670000002));
#270317=CARTESIAN_POINT('Ctrl Pts',(-9.68734173700006,15.2,-4.22858838400002));
#270318=CARTESIAN_POINT('Ctrl Pts',(-9.68734173700006,11.6,-4.22858838400002));
#270319=CARTESIAN_POINT('Ctrl Pts',(-9.68538991200005,15.2,-4.22818971000002));
#270320=CARTESIAN_POINT('Ctrl Pts',(-9.68538991200005,11.6,-4.22818971000002));
#270321=CARTESIAN_POINT('Ctrl Pts',(-9.68344537600006,15.2,-4.22779069300002));
#270322=CARTESIAN_POINT('Ctrl Pts',(-9.68344537600006,11.6,-4.22779069300002));
#270323=CARTESIAN_POINT('Ctrl Pts',(-9.68150814100006,15.2,-4.22739134800001));
#270324=CARTESIAN_POINT('Ctrl Pts',(-9.68150814100006,11.6,-4.22739134800001));
#270325=CARTESIAN_POINT('Ctrl Pts',(-9.67957822000006,15.2,-4.22699168800001));
#270326=CARTESIAN_POINT('Ctrl Pts',(-9.67957822000006,11.6,-4.22699168800001));
#270327=CARTESIAN_POINT('Ctrl Pts',(-9.67765562600006,15.2,-4.22659173000001));
#270328=CARTESIAN_POINT('Ctrl Pts',(-9.67765562600006,11.6,-4.22659173000001));
#270329=CARTESIAN_POINT('Ctrl Pts',(-9.67574037300006,15.2,-4.22619148600001));
#270330=CARTESIAN_POINT('Ctrl Pts',(-9.67574037300006,11.6,-4.22619148600001));
#270331=CARTESIAN_POINT('Ctrl Pts',(-9.67383247200006,15.2,-4.22579097300002));
#270332=CARTESIAN_POINT('Ctrl Pts',(-9.67383247200006,11.6,-4.22579097300002));
#270333=CARTESIAN_POINT('Ctrl Pts',(-9.67193193600006,15.2,-4.22539020400002));
#270334=CARTESIAN_POINT('Ctrl Pts',(-9.67193193600006,11.6,-4.22539020400002));
#270335=CARTESIAN_POINT('Ctrl Pts',(-9.67003878000006,15.2,-4.22498919400002));
#270336=CARTESIAN_POINT('Ctrl Pts',(-9.67003878000006,11.6,-4.22498919400002));
#270337=CARTESIAN_POINT('Ctrl Pts',(-9.66815301400005,15.2,-4.22458795800001));
#270338=CARTESIAN_POINT('Ctrl Pts',(-9.66815301400005,11.6,-4.22458795800001));
#270339=CARTESIAN_POINT('Ctrl Pts',(-9.66627465400006,15.2,-4.22418651100001));
#270340=CARTESIAN_POINT('Ctrl Pts',(-9.66627465400006,11.6,-4.22418651100002));
#270341=CARTESIAN_POINT('Ctrl Pts',(-9.66440371000006,15.2,-4.22378486900001));
#270342=CARTESIAN_POINT('Ctrl Pts',(-9.66440371000006,11.6,-4.22378486900001));
#270343=CARTESIAN_POINT('Ctrl Pts',(-9.66254019900006,15.2,-4.22338304400002));
#270344=CARTESIAN_POINT('Ctrl Pts',(-9.66254019900006,11.6,-4.22338304400002));
#270345=CARTESIAN_POINT('Ctrl Pts',(-9.66068413000006,15.2,-4.22298105400001));
#270346=CARTESIAN_POINT('Ctrl Pts',(-9.66068413000006,11.6,-4.22298105400001));
#270347=CARTESIAN_POINT('Ctrl Pts',(-9.65883551800006,15.2,-4.22257891400001));
#270348=CARTESIAN_POINT('Ctrl Pts',(-9.65883551800006,11.6,-4.22257891400002));
#270349=CARTESIAN_POINT('Ctrl Pts',(-9.65699437800006,15.2,-4.22217663600001));
#270350=CARTESIAN_POINT('Ctrl Pts',(-9.65699437800006,11.6,-4.22217663600002));
#270351=CARTESIAN_POINT('Ctrl Pts',(-9.65516071900005,15.2,-4.22177424000001));
#270352=CARTESIAN_POINT('Ctrl Pts',(-9.65516071900005,11.6,-4.22177424000001));
#270353=CARTESIAN_POINT('Ctrl Pts',(-9.65333455800006,15.2,-4.22137173700001));
#270354=CARTESIAN_POINT('Ctrl Pts',(-9.65333455800006,11.6,-4.22137173700001));
#270355=CARTESIAN_POINT('Ctrl Pts',(-9.65151590800006,15.2,-4.22096914500001));
#270356=CARTESIAN_POINT('Ctrl Pts',(-9.65151590800006,11.6,-4.22096914500001));
#270357=CARTESIAN_POINT('Ctrl Pts',(-9.64970478100006,15.2,-4.22056647800002));
#270358=CARTESIAN_POINT('Ctrl Pts',(-9.64970478100006,11.6,-4.22056647800002));
#270359=CARTESIAN_POINT('Ctrl Pts',(-9.64790118900006,15.2,-4.22016375300001));
#270360=CARTESIAN_POINT('Ctrl Pts',(-9.64790118900006,11.6,-4.22016375300002));
#270361=CARTESIAN_POINT('Ctrl Pts',(-9.64610514900006,15.2,-4.21976098400001));
#270362=CARTESIAN_POINT('Ctrl Pts',(-9.64610514900006,11.6,-4.21976098400001));
#270363=CARTESIAN_POINT('Ctrl Pts',(-9.64431667200006,15.2,-4.21935818700002));
#270364=CARTESIAN_POINT('Ctrl Pts',(-9.64431667200006,11.6,-4.21935818700002));
#270365=CARTESIAN_POINT('Ctrl Pts',(-9.64253577200006,15.2,-4.21895537800001));
#270366=CARTESIAN_POINT('Ctrl Pts',(-9.64253577200006,11.6,-4.21895537800001));
#270367=CARTESIAN_POINT('Ctrl Pts',(-9.64076246400005,15.2,-4.21855257300002));
#270368=CARTESIAN_POINT('Ctrl Pts',(-9.64076246400005,11.6,-4.21855257300002));
#270369=CARTESIAN_POINT('Ctrl Pts',(-9.63899675900005,15.2,-4.21814978700001));
#270370=CARTESIAN_POINT('Ctrl Pts',(-9.63899675900005,11.6,-4.21814978700001));
#270371=CARTESIAN_POINT('Ctrl Pts',(-9.63723867300006,15.2,-4.21774703800001));
#270372=CARTESIAN_POINT('Ctrl Pts',(-9.63723867300006,11.6,-4.21774703800002));
#270373=CARTESIAN_POINT('Ctrl Pts',(-9.63548821800006,15.2,-4.21734433900002));
#270374=CARTESIAN_POINT('Ctrl Pts',(-9.63548821800006,11.6,-4.21734433900002));
#270375=CARTESIAN_POINT('Ctrl Pts',(-9.63374540700006,15.2,-4.21694170700002));
#270376=CARTESIAN_POINT('Ctrl Pts',(-9.63374540700006,11.6,-4.21694170700002));
#270377=CARTESIAN_POINT('Ctrl Pts',(-9.63201025800006,15.2,-4.21653915900002));
#270378=CARTESIAN_POINT('Ctrl Pts',(-9.63201025800006,11.6,-4.21653915900002));
#270379=CARTESIAN_POINT('Ctrl Pts',(-9.63028278000005,15.2,-4.21613671100001));
#270380=CARTESIAN_POINT('Ctrl Pts',(-9.63028278000005,11.6,-4.21613671100001));
#270381=CARTESIAN_POINT('Ctrl Pts',(-9.62856298800006,15.2,-4.21573437800001));
#270382=CARTESIAN_POINT('Ctrl Pts',(-9.62856298800006,11.6,-4.21573437800001));
#270383=CARTESIAN_POINT('Ctrl Pts',(-9.62685089700006,15.2,-4.21533217700001));
#270384=CARTESIAN_POINT('Ctrl Pts',(-9.62685089700006,11.6,-4.21533217700001));
#270385=CARTESIAN_POINT('Ctrl Pts',(-9.62514652100005,15.2,-4.21493012500001));
#270386=CARTESIAN_POINT('Ctrl Pts',(-9.62514652100005,11.6,-4.21493012500001));
#270387=CARTESIAN_POINT('Ctrl Pts',(-9.62344987300006,15.2,-4.21452823700001));
#270388=CARTESIAN_POINT('Ctrl Pts',(-9.62344987300006,11.6,-4.21452823700002));
#270389=CARTESIAN_POINT('Ctrl Pts',(-9.62176096800006,15.2,-4.21412653000001));
#270390=CARTESIAN_POINT('Ctrl Pts',(-9.62176096800006,11.6,-4.21412653000001));
#270391=CARTESIAN_POINT('Ctrl Pts',(-9.62007981900006,15.2,-4.21372502300001));
#270392=CARTESIAN_POINT('Ctrl Pts',(-9.62007981900006,11.6,-4.21372502300002));
#270393=CARTESIAN_POINT('Ctrl Pts',(-9.61840643900005,15.2,-4.21332372800002));
#270394=CARTESIAN_POINT('Ctrl Pts',(-9.61840643900005,11.6,-4.21332372800002));
#270395=CARTESIAN_POINT('Ctrl Pts',(-9.61674084500006,15.2,-4.21292266500001));
#270396=CARTESIAN_POINT('Ctrl Pts',(-9.61674084500006,11.6,-4.21292266500001));
#270397=CARTESIAN_POINT('Ctrl Pts',(-9.61508305000006,15.2,-4.21252185000002));
#270398=CARTESIAN_POINT('Ctrl Pts',(-9.61508305000006,11.6,-4.21252185000002));
#270399=CARTESIAN_POINT('Ctrl Pts',(-9.61343306700006,15.2,-4.21212129900002));
#270400=CARTESIAN_POINT('Ctrl Pts',(-9.61343306700006,11.6,-4.21212129900002));
#270401=CARTESIAN_POINT('Ctrl Pts',(-9.61179091200006,15.2,-4.21172103000002));
#270402=CARTESIAN_POINT('Ctrl Pts',(-9.61179091200006,11.6,-4.21172103000002));
#270403=CARTESIAN_POINT('Ctrl Pts',(-9.61015659800006,15.2,-4.21132106100002));
#270404=CARTESIAN_POINT('Ctrl Pts',(-9.61015659800006,11.6,-4.21132106100002));
#270405=CARTESIAN_POINT('Ctrl Pts',(-9.60853014000006,15.2,-4.21092140600001));
#270406=CARTESIAN_POINT('Ctrl Pts',(-9.60853014000006,11.6,-4.21092140600001));
#270407=CARTESIAN_POINT('Ctrl Pts',(-9.60691155200006,15.2,-4.21052208500001));
#270408=CARTESIAN_POINT('Ctrl Pts',(-9.60691155200006,11.6,-4.21052208500001));
#270409=CARTESIAN_POINT('Ctrl Pts',(-9.60530084800006,15.2,-4.21012311200001));
#270410=CARTESIAN_POINT('Ctrl Pts',(-9.60530084800006,11.6,-4.21012311200002));
#270411=CARTESIAN_POINT('Ctrl Pts',(-9.60369804400005,15.2,-4.20972450700001));
#270412=CARTESIAN_POINT('Ctrl Pts',(-9.60369804400005,11.6,-4.20972450700001));
#270413=CARTESIAN_POINT('Ctrl Pts',(-9.60210315400005,15.2,-4.20932628800001));
#270414=CARTESIAN_POINT('Ctrl Pts',(-9.60210315400005,11.6,-4.20932628800002));
#270415=CARTESIAN_POINT('Ctrl Pts',(-9.60051619200006,15.2,-4.20892847000002));
#270416=CARTESIAN_POINT('Ctrl Pts',(-9.60051619200006,11.6,-4.20892847000002));
#270417=CARTESIAN_POINT('Ctrl Pts',(-9.59893717200006,15.2,-4.20853107100001));
#270418=CARTESIAN_POINT('Ctrl Pts',(-9.59893717200006,11.6,-4.20853107100002));
#270419=CARTESIAN_POINT('Ctrl Pts',(-9.59736611000006,15.2,-4.20813411000001));
#270420=CARTESIAN_POINT('Ctrl Pts',(-9.59736611000006,11.6,-4.20813411000002));
#270421=CARTESIAN_POINT('Ctrl Pts',(-9.59580302000006,15.2,-4.20773760300001));
#270422=CARTESIAN_POINT('Ctrl Pts',(-9.59580302000006,11.6,-4.20773760300001));
#270423=CARTESIAN_POINT('Ctrl Pts',(-9.59424791700006,15.2,-4.20734157000001));
#270424=CARTESIAN_POINT('Ctrl Pts',(-9.59424791700006,11.6,-4.20734157000001));
#270425=CARTESIAN_POINT('Ctrl Pts',(-9.59270081500006,15.2,-4.20694602600001));
#270426=CARTESIAN_POINT('Ctrl Pts',(-9.59270081500006,11.6,-4.20694602600001));
#270427=CARTESIAN_POINT('Ctrl Pts',(-9.59116173000006,15.2,-4.20655099000002));
#270428=CARTESIAN_POINT('Ctrl Pts',(-9.59116173000006,11.6,-4.20655099000002));
#270429=CARTESIAN_POINT('Ctrl Pts',(-9.58963067700006,15.2,-4.20615648000001));
#270430=CARTESIAN_POINT('Ctrl Pts',(-9.58963067700006,11.6,-4.20615648000001));
#270431=CARTESIAN_POINT('Ctrl Pts',(-9.58810767000006,15.2,-4.20576251400002));
#270432=CARTESIAN_POINT('Ctrl Pts',(-9.58810767000006,11.6,-4.20576251400002));
#270433=CARTESIAN_POINT('Ctrl Pts',(-9.58659272300006,15.2,-4.20536911000001));
#270434=CARTESIAN_POINT('Ctrl Pts',(-9.58659272300006,11.6,-4.20536911000002));
#270435=CARTESIAN_POINT('Ctrl Pts',(-9.58508585400006,15.2,-4.20497628800002));
#270436=CARTESIAN_POINT('Ctrl Pts',(-9.58508585400006,11.6,-4.20497628800002));
#270437=CARTESIAN_POINT('Ctrl Pts',(-9.58358707600006,15.2,-4.20458406300002));
#270438=CARTESIAN_POINT('Ctrl Pts',(-9.58358707600006,11.6,-4.20458406300002));
#270439=CARTESIAN_POINT('Ctrl Pts',(-9.58209640400005,15.2,-4.20419245700002));
#270440=CARTESIAN_POINT('Ctrl Pts',(-9.58209640400005,11.6,-4.20419245700002));
#270441=CARTESIAN_POINT('Ctrl Pts',(-9.58061385500006,15.2,-4.20380148500001));
#270442=CARTESIAN_POINT('Ctrl Pts',(-9.58061385500006,11.6,-4.20380148500001));
#270443=CARTESIAN_POINT('Ctrl Pts',(-9.57913944200006,15.2,-4.20341116800001));
#270444=CARTESIAN_POINT('Ctrl Pts',(-9.57913944200006,11.6,-4.20341116800001));
#270445=CARTESIAN_POINT('Ctrl Pts',(-9.57767318100006,15.2,-4.20302152200001));
#270446=CARTESIAN_POINT('Ctrl Pts',(-9.57767318100006,11.6,-4.20302152200002));
#270447=CARTESIAN_POINT('Ctrl Pts',(-9.57621508800005,15.2,-4.20263256900002));
#270448=CARTESIAN_POINT('Ctrl Pts',(-9.57621508800005,11.6,-4.20263256900002));
#270449=CARTESIAN_POINT('Ctrl Pts',(-9.57476517900006,15.2,-4.20224432500001));
#270450=CARTESIAN_POINT('Ctrl Pts',(-9.57476517900006,11.6,-4.20224432500001));
#270451=CARTESIAN_POINT('Ctrl Pts',(-9.57332346800005,15.2,-4.20185681100001));
#270452=CARTESIAN_POINT('Ctrl Pts',(-9.57332346800005,11.6,-4.20185681100001));
#270453=CARTESIAN_POINT('Ctrl Pts',(-9.57188997100006,15.2,-4.20147004400001));
#270454=CARTESIAN_POINT('Ctrl Pts',(-9.57188997100006,11.6,-4.20147004400001));
#270455=CARTESIAN_POINT('Ctrl Pts',(-9.57046470400006,15.2,-4.20108404600001));
#270456=CARTESIAN_POINT('Ctrl Pts',(-9.57046470400006,11.6,-4.20108404600002));
#270457=CARTESIAN_POINT('Ctrl Pts',(-9.56904768100006,15.2,-4.20069883200001));
#270458=CARTESIAN_POINT('Ctrl Pts',(-9.56904768100006,11.6,-4.20069883200001));
#270459=CARTESIAN_POINT('Ctrl Pts',(-9.56763891900006,15.2,-4.20031442400001));
#270460=CARTESIAN_POINT('Ctrl Pts',(-9.56763891900006,11.6,-4.20031442400001));
#270461=CARTESIAN_POINT('Ctrl Pts',(-9.56623843400006,15.2,-4.19993084100001));
#270462=CARTESIAN_POINT('Ctrl Pts',(-9.56623843400006,11.6,-4.19993084100002));
#270463=CARTESIAN_POINT('Ctrl Pts',(-9.56484624200005,15.2,-4.19954810100001));
#270464=CARTESIAN_POINT('Ctrl Pts',(-9.56484624200005,11.6,-4.19954810100002));
#270465=CARTESIAN_POINT('Ctrl Pts',(-9.56346235700006,15.2,-4.19916622400001));
#270466=CARTESIAN_POINT('Ctrl Pts',(-9.56346235700006,11.6,-4.19916622400002));
#270467=CARTESIAN_POINT('Ctrl Pts',(-9.56208679700006,15.2,-4.19878523200001));
#270468=CARTESIAN_POINT('Ctrl Pts',(-9.56208679700006,11.6,-4.19878523200001));
#270469=CARTESIAN_POINT('Ctrl Pts',(-9.56071957600006,15.2,-4.19840514100001));
#270470=CARTESIAN_POINT('Ctrl Pts',(-9.56071957600006,11.6,-4.19840514100002));
#270471=CARTESIAN_POINT('Ctrl Pts',(-9.55936071100006,15.2,-4.19802597300002));
#270472=CARTESIAN_POINT('Ctrl Pts',(-9.55936071100006,11.6,-4.19802597300002));
#270473=CARTESIAN_POINT('Ctrl Pts',(-9.55801021900006,15.2,-4.19764774700001));
#270474=CARTESIAN_POINT('Ctrl Pts',(-9.55801021900006,11.6,-4.19764774700001));
#270475=CARTESIAN_POINT('Ctrl Pts',(-9.55666811400006,15.2,-4.19727048300001));
#270476=CARTESIAN_POINT('Ctrl Pts',(-9.55666811400006,11.6,-4.19727048300001));
#270477=CARTESIAN_POINT('Ctrl Pts',(-9.55533441300006,15.2,-4.19689420200001));
#270478=CARTESIAN_POINT('Ctrl Pts',(-9.55533441300006,11.6,-4.19689420200002));
#270479=CARTESIAN_POINT('Ctrl Pts',(-9.55400913300006,15.2,-4.19651892300001));
#270480=CARTESIAN_POINT('Ctrl Pts',(-9.55400913300006,11.6,-4.19651892300002));
#270481=CARTESIAN_POINT('Ctrl Pts',(-9.55269229000006,15.2,-4.19614466600001));
#270482=CARTESIAN_POINT('Ctrl Pts',(-9.55269229000006,11.6,-4.19614466600002));
#270483=CARTESIAN_POINT('Ctrl Pts',(-9.55138390100006,15.2,-4.19577145200002));
#270484=CARTESIAN_POINT('Ctrl Pts',(-9.55138390100006,11.6,-4.19577145200002));
#270485=CARTESIAN_POINT('Ctrl Pts',(-9.55008398000006,15.2,-4.19539930100001));
#270486=CARTESIAN_POINT('Ctrl Pts',(-9.55008398000006,11.6,-4.19539930100001));
#270487=CARTESIAN_POINT('Ctrl Pts',(-9.54879254600005,15.2,-4.19502823400002));
#270488=CARTESIAN_POINT('Ctrl Pts',(-9.54879254600005,11.6,-4.19502823400002));
#270489=CARTESIAN_POINT('Ctrl Pts',(-9.54750961400006,15.2,-4.19465827100002));
#270490=CARTESIAN_POINT('Ctrl Pts',(-9.54750961400006,11.6,-4.19465827100002));
#270491=CARTESIAN_POINT('Ctrl Pts',(-9.54623520100006,15.2,-4.19428943400002));
#270492=CARTESIAN_POINT('Ctrl Pts',(-9.54623520100006,11.6,-4.19428943400002));
#270493=CARTESIAN_POINT('Ctrl Pts',(-9.54496932400006,15.2,-4.19392174100001));
#270494=CARTESIAN_POINT('Ctrl Pts',(-9.54496932400006,11.6,-4.19392174100001));
#270495=CARTESIAN_POINT('Ctrl Pts',(-9.54371199900006,15.2,-4.19355521600002));
#270496=CARTESIAN_POINT('Ctrl Pts',(-9.54371199900006,11.6,-4.19355521600002));
#270497=CARTESIAN_POINT('Ctrl Pts',(-9.54246324300006,15.2,-4.19318987800001));
#270498=CARTESIAN_POINT('Ctrl Pts',(-9.54246324300006,11.6,-4.19318987800002));
#270499=CARTESIAN_POINT('Ctrl Pts',(-9.54122307300005,15.2,-4.19282574800001));
#270500=CARTESIAN_POINT('Ctrl Pts',(-9.54122307300005,11.6,-4.19282574800001));
#270501=CARTESIAN_POINT('Ctrl Pts',(-9.53999150600006,15.2,-4.19246284900002));
#270502=CARTESIAN_POINT('Ctrl Pts',(-9.53999150600006,11.6,-4.19246284900002));
#270503=CARTESIAN_POINT('Ctrl Pts',(-9.53876855900005,15.2,-4.19210120000002));
#270504=CARTESIAN_POINT('Ctrl Pts',(-9.53876855900005,11.6,-4.19210120000002));
#270505=CARTESIAN_POINT('Ctrl Pts',(-9.53755424900006,15.2,-4.19174082400001));
#270506=CARTESIAN_POINT('Ctrl Pts',(-9.53755424900006,11.6,-4.19174082400002));
#270507=CARTESIAN_POINT('Ctrl Pts',(-9.53634859300006,15.2,-4.19138174200001));
#270508=CARTESIAN_POINT('Ctrl Pts',(-9.53634859300006,11.6,-4.19138174200001));
#270509=CARTESIAN_POINT('Ctrl Pts',(-9.53515160800006,15.2,-4.19102397600001));
#270510=CARTESIAN_POINT('Ctrl Pts',(-9.53515160800006,11.6,-4.19102397600002));
#270511=CARTESIAN_POINT('Ctrl Pts',(-9.53396331100006,15.2,-4.19066754700001));
#270512=CARTESIAN_POINT('Ctrl Pts',(-9.53396331100006,11.6,-4.19066754700001));
#270513=CARTESIAN_POINT('Ctrl Pts',(-9.53278371900005,15.2,-4.19031247800001));
#270514=CARTESIAN_POINT('Ctrl Pts',(-9.53278371900005,11.6,-4.19031247800001));
#270515=CARTESIAN_POINT('Ctrl Pts',(-9.53161285100006,15.2,-4.18995879000001));
#270516=CARTESIAN_POINT('Ctrl Pts',(-9.53161285100006,11.6,-4.18995879000002));
#270517=CARTESIAN_POINT('Ctrl Pts',(-9.53045072400006,15.2,-4.18960650400001));
#270518=CARTESIAN_POINT('Ctrl Pts',(-9.53045072400006,11.6,-4.18960650400001));
#270519=CARTESIAN_POINT('Ctrl Pts',(-9.52929735300006,15.2,-4.18925564400002));
#270520=CARTESIAN_POINT('Ctrl Pts',(-9.52929735300006,11.6,-4.18925564400002));
#270521=CARTESIAN_POINT('Ctrl Pts',(-9.52815275900005,15.2,-4.18890623000001));
#270522=CARTESIAN_POINT('Ctrl Pts',(-9.52815275900005,11.6,-4.18890623000001));
#270523=CARTESIAN_POINT('Ctrl Pts',(-9.52701695800006,15.2,-4.18855828800002));
#270524=CARTESIAN_POINT('Ctrl Pts',(-9.52701695800006,11.6,-4.18855828800002));
#270525=CARTESIAN_POINT('Ctrl Pts',(-9.52588996700005,15.2,-4.18821183700001));
#270526=CARTESIAN_POINT('Ctrl Pts',(-9.52588996700005,11.6,-4.18821183700001));
#270527=CARTESIAN_POINT('Ctrl Pts',(-9.52477180300006,15.2,-4.18786690100001));
#270528=CARTESIAN_POINT('Ctrl Pts',(-9.52477180300006,11.6,-4.18786690100002));
#270529=CARTESIAN_POINT('Ctrl Pts',(-9.52366248800006,15.2,-4.18752350200001));
#270530=CARTESIAN_POINT('Ctrl Pts',(-9.52366248800006,11.6,-4.18752350200002));
#270531=CARTESIAN_POINT('Ctrl Pts',(-9.52256203600006,15.2,-4.18718166400001));
#270532=CARTESIAN_POINT('Ctrl Pts',(-9.52256203600006,11.6,-4.18718166400002));
#270533=CARTESIAN_POINT('Ctrl Pts',(-9.52147046600006,15.2,-4.18684141000002));
#270534=CARTESIAN_POINT('Ctrl Pts',(-9.52147046600006,11.6,-4.18684141000002));
#270535=CARTESIAN_POINT('Ctrl Pts',(-9.52038779700005,15.2,-4.18650276100001));
#270536=CARTESIAN_POINT('Ctrl Pts',(-9.52038779700005,11.6,-4.18650276100002));
#270537=CARTESIAN_POINT('Ctrl Pts',(-9.51931404600005,15.2,-4.18616574200001));
#270538=CARTESIAN_POINT('Ctrl Pts',(-9.51931404600005,11.6,-4.18616574200002));
#270539=CARTESIAN_POINT('Ctrl Pts',(-9.51824923100006,15.2,-4.18583037500001));
#270540=CARTESIAN_POINT('Ctrl Pts',(-9.51824923100006,11.6,-4.18583037500001));
#270541=CARTESIAN_POINT('Ctrl Pts',(-9.51719337200006,15.2,-4.18549668500001));
#270542=CARTESIAN_POINT('Ctrl Pts',(-9.51719337200006,11.6,-4.18549668500001));
#270543=CARTESIAN_POINT('Ctrl Pts',(-9.51614648500006,15.2,-4.18516469500001));
#270544=CARTESIAN_POINT('Ctrl Pts',(-9.51614648500006,11.6,-4.18516469500002));
#270545=CARTESIAN_POINT('Ctrl Pts',(-9.51510859000006,15.2,-4.18483442700001));
#270546=CARTESIAN_POINT('Ctrl Pts',(-9.51510859000006,11.6,-4.18483442700001));
#270547=CARTESIAN_POINT('Ctrl Pts',(-9.51407970500006,15.2,-4.18450590600001));
#270548=CARTESIAN_POINT('Ctrl Pts',(-9.51407970500006,11.6,-4.18450590600001));
#270549=CARTESIAN_POINT('Ctrl Pts',(-9.51305984900005,15.2,-4.18417915700001));
#270550=CARTESIAN_POINT('Ctrl Pts',(-9.51305984900005,11.6,-4.18417915700002));
#270551=CARTESIAN_POINT('Ctrl Pts',(-9.51204904000006,15.2,-4.18385420100002));
#270552=CARTESIAN_POINT('Ctrl Pts',(-9.51204904000006,11.6,-4.18385420100002));
#270553=CARTESIAN_POINT('Ctrl Pts',(-9.51104729800005,15.2,-4.18353106500001));
#270554=CARTESIAN_POINT('Ctrl Pts',(-9.51104729800005,11.6,-4.18353106500002));
#270555=CARTESIAN_POINT('Ctrl Pts',(-9.51005464000006,15.2,-4.18320977200001));
#270556=CARTESIAN_POINT('Ctrl Pts',(-9.51005464000006,11.6,-4.18320977200001));
#270557=CARTESIAN_POINT('Ctrl Pts',(-9.50907108500006,15.2,-4.18289034600001));
#270558=CARTESIAN_POINT('Ctrl Pts',(-9.50907108500006,11.6,-4.18289034600001));
#270559=CARTESIAN_POINT('Ctrl Pts',(-9.50809665400006,15.2,-4.18257281300002));
#270560=CARTESIAN_POINT('Ctrl Pts',(-9.50809665400006,11.6,-4.18257281300002));
#270561=CARTESIAN_POINT('Ctrl Pts',(-9.50713136500006,15.2,-4.18225719500001));
#270562=CARTESIAN_POINT('Ctrl Pts',(-9.50713136500006,11.6,-4.18225719500002));
#270563=CARTESIAN_POINT('Ctrl Pts',(-9.50617523600006,15.2,-4.18194352000001));
#270564=CARTESIAN_POINT('Ctrl Pts',(-9.50617523600006,11.6,-4.18194352000001));
#270565=CARTESIAN_POINT('Ctrl Pts',(-9.50522828800005,15.2,-4.18163181000001));
#270566=CARTESIAN_POINT('Ctrl Pts',(-9.50522828800005,11.6,-4.18163181000002));
#270567=CARTESIAN_POINT('Ctrl Pts',(-9.50429053900006,15.2,-4.18132209200001));
#270568=CARTESIAN_POINT('Ctrl Pts',(-9.50429053900006,11.6,-4.18132209200001));
#270569=CARTESIAN_POINT('Ctrl Pts',(-9.50336200900006,15.2,-4.18101439000001));
#270570=CARTESIAN_POINT('Ctrl Pts',(-9.50336200900006,11.6,-4.18101439000001));
#270571=CARTESIAN_POINT('Ctrl Pts',(-9.50244271700006,15.2,-4.18070872900001));
#270572=CARTESIAN_POINT('Ctrl Pts',(-9.50244271700006,11.6,-4.18070872900001));
#270573=CARTESIAN_POINT('Ctrl Pts',(-9.50153268200006,15.2,-4.18040513500001));
#270574=CARTESIAN_POINT('Ctrl Pts',(-9.50153268200006,11.6,-4.18040513500001));
#270575=CARTESIAN_POINT('Ctrl Pts',(-9.50063192600006,15.2,-4.18010363500001));
#270576=CARTESIAN_POINT('Ctrl Pts',(-9.50063192600006,11.6,-4.18010363500002));
#270577=CARTESIAN_POINT('Ctrl Pts',(-9.49974046700006,15.2,-4.17980425200001));
#270578=CARTESIAN_POINT('Ctrl Pts',(-9.49974046700006,11.6,-4.17980425200002));
#270579=CARTESIAN_POINT('Ctrl Pts',(-9.49885832400006,15.2,-4.17950701300001));
#270580=CARTESIAN_POINT('Ctrl Pts',(-9.49885832400006,11.6,-4.17950701300002));
#270581=CARTESIAN_POINT('Ctrl Pts',(-9.49799054600006,15.2,-4.17921364400001));
#270582=CARTESIAN_POINT('Ctrl Pts',(-9.49799054600006,11.6,-4.17921364400002));
#270583=CARTESIAN_POINT('Ctrl Pts',(-9.49730470600005,15.2,-4.17898101900001));
#270584=CARTESIAN_POINT('Ctrl Pts',(-9.49730470600005,11.6,-4.17898101900002));
#270585=CARTESIAN_POINT('Ctrl Pts',(-9.49679571000006,15.2,-4.17880795400002));
#270586=CARTESIAN_POINT('Ctrl Pts',(-9.49679571000006,11.6,-4.17880795400002));
#270587=CARTESIAN_POINT('Ctrl Pts',(-9.49645984700006,15.2,-4.17869357200002));
#270588=CARTESIAN_POINT('Ctrl Pts',(-9.49645984700006,11.6,-4.17869357200002));
#270589=CARTESIAN_POINT('Ctrl Pts',(-9.49629481200006,15.2,-4.17863732200002));
#270590=CARTESIAN_POINT('Ctrl Pts',(-9.49629481200006,11.6,-4.17863732200002));
#270591=CARTESIAN_POINT('',(-9.49629481136457,12.2,-4.17863732134707));
#270592=CARTESIAN_POINT('',(-9.49629481136457,15.2,-4.17863732134707));
#270593=CARTESIAN_POINT('',(-9.49629481100006,12.2,-4.17863732100002));
#270594=CARTESIAN_POINT('Ctrl Pts',(-10.6761442620001,12.2,-4.27433546900002));
#270595=CARTESIAN_POINT('Ctrl Pts',(-10.6723314813074,12.2,-4.27461376405057));
#270596=CARTESIAN_POINT('Ctrl Pts',(-10.6685249858623,12.2,-4.27488727070577));
#270597=CARTESIAN_POINT('Ctrl Pts',(-10.664724775623,12.2,-4.27515599121663));
#270598=CARTESIAN_POINT('Ctrl Pts',(-10.6609245653838,12.2,-4.2754247117275));
#270599=CARTESIAN_POINT('Ctrl Pts',(-10.6571306407685,12.2,-4.27568864374578));
#270600=CARTESIAN_POINT('Ctrl Pts',(-10.6533430152162,12.2,-4.27594779995819));
#270601=CARTESIAN_POINT('Ctrl Pts',(-10.6495553896639,12.2,-4.27620695617061));
#270602=CARTESIAN_POINT('Ctrl Pts',(-10.64577406477,12.2,-4.27646133445405));
#270603=CARTESIAN_POINT('Ctrl Pts',(-10.641999077073,12.2,-4.27671095994562));
#270604=CARTESIAN_POINT('Ctrl Pts',(-10.6382240886901,12.2,-4.27696058548255));
#270605=CARTESIAN_POINT('Ctrl Pts',(-10.6344554370091,12.2,-4.27720545935147));
#270606=CARTESIAN_POINT('Ctrl Pts',(-10.6306931631715,12.2,-4.27744560934406));
#270607=CARTESIAN_POINT('Ctrl Pts',(-10.6269308900174,12.2,-4.27768575929303));
#270608=CARTESIAN_POINT('Ctrl Pts',(-10.623174996138,12.2,-4.27792118538392));
#270609=CARTESIAN_POINT('Ctrl Pts',(-10.6194255113997,12.2,-4.27815191029179));
#270610=CARTESIAN_POINT('Ctrl Pts',(-10.6156760266615,12.2,-4.27838263519966));
#270611=CARTESIAN_POINT('Ctrl Pts',(-10.6119329517445,12.2,-4.27860865854064));
#270612=CARTESIAN_POINT('Ctrl Pts',(-10.6081963174883,12.2,-4.27883000099191));
#270613=CARTESIAN_POINT('Ctrl Pts',(-10.6019685935017,12.2,-4.27919890509078));
#270614=CARTESIAN_POINT('Ctrl Pts',(-10.5957587585331,12.2,-4.27955480756196));
#270615=CARTESIAN_POINT('Ctrl Pts',(-10.5895669738118,12.2,-4.27989782075574));
#270616=CARTESIAN_POINT('Ctrl Pts',(-10.585851903114,12.2,-4.28010362866452));
#270617=CARTESIAN_POINT('Ctrl Pts',(-10.5821433307655,12.2,-4.28030479564053));
#270618=CARTESIAN_POINT('Ctrl Pts',(-10.578441290525,12.2,-4.28050134796672));
#270619=CARTESIAN_POINT('Ctrl Pts',(-10.5747392502845,12.2,-4.28069790029291));
#270620=CARTESIAN_POINT('Ctrl Pts',(-10.5710437423854,12.2,-4.28088983588595));
#270621=CARTESIAN_POINT('Ctrl Pts',(-10.5673547996439,12.2,-4.28107717971288));
#270622=CARTESIAN_POINT('Ctrl Pts',(-10.5636658569023,12.2,-4.28126452353981));
#270623=CARTESIAN_POINT('Ctrl Pts',(-10.5599834796454,12.2,-4.2814472737959));
#270624=CARTESIAN_POINT('Ctrl Pts',(-10.5563077012612,12.2,-4.28162545671553));
#270625=CARTESIAN_POINT('Ctrl Pts',(-10.5526319228771,12.2,-4.28180363963515));
#270626=CARTESIAN_POINT('Ctrl Pts',(-10.548962744233,12.2,-4.28197725503537));
#270627=CARTESIAN_POINT('Ctrl Pts',(-10.5453001995318,12.2,-4.28214632648818));
#270628=CARTESIAN_POINT('Ctrl Pts',(-10.5416376541652,12.2,-4.28231539797171));
#270629=CARTESIAN_POINT('Ctrl Pts',(-10.5379817430673,12.2,-4.28247992557895));
#270630=CARTESIAN_POINT('Ctrl Pts',(-10.5343324992462,12.2,-4.28263993501826));
#270631=CARTESIAN_POINT('Ctrl Pts',(-10.5294668419229,12.2,-4.28285328088888));
#270632=CARTESIAN_POINT('Ctrl Pts',(-10.524613039387,12.2,-4.28305859348278));
#270633=CARTESIAN_POINT('Ctrl Pts',(-10.5197711731709,12.2,-4.28325593146717));
#270634=CARTESIAN_POINT('Ctrl Pts',(-10.5161397733439,12.2,-4.28340393496218));
#270635=CARTESIAN_POINT('Ctrl Pts',(-10.5125150858668,12.2,-4.28354745247069));
#270636=CARTESIAN_POINT('Ctrl Pts',(-10.5088971479001,12.2,-4.28368650993143));
#270637=CARTESIAN_POINT('Ctrl Pts',(-10.5040732301729,12.2,-4.28387191989594));
#270638=CARTESIAN_POINT('Ctrl Pts',(-10.4992613097435,12.2,-4.28404940070511));
#270639=CARTESIAN_POINT('Ctrl Pts',(-10.4944614683161,12.2,-4.28421901204717));
#270640=CARTESIAN_POINT('Ctrl Pts',(-10.4908615875725,12.2,-4.28434622054216));
#270641=CARTESIAN_POINT('Ctrl Pts',(-10.4872685011197,12.2,-4.28446900300435));
#270642=CARTESIAN_POINT('Ctrl Pts',(-10.48368224525,12.2,-4.28458738450005));
#270643=CARTESIAN_POINT('Ctrl Pts',(-10.4800959893803,12.2,-4.28470576599575));
#270644=CARTESIAN_POINT('Ctrl Pts',(-10.476516561377,12.2,-4.28481974652496));
#270645=CARTESIAN_POINT('Ctrl Pts',(-10.4729439986312,12.2,-4.28492935297969));
#270646=CARTESIAN_POINT('Ctrl Pts',(-10.4693714358854,12.2,-4.28503895943442));
#270647=CARTESIAN_POINT('Ctrl Pts',(-10.4658057382475,12.2,-4.28514419088112));
#270648=CARTESIAN_POINT('Ctrl Pts',(-10.4622469395425,12.2,-4.28524507346138));
#270649=CARTESIAN_POINT('Ctrl Pts',(-10.458688140191,12.2,-4.28534595605997));
#270650=CARTESIAN_POINT('Ctrl Pts',(-10.4551362403248,12.2,-4.28544249114066));
#270651=CARTESIAN_POINT('Ctrl Pts',(-10.4515912749772,12.2,-4.28553470319514));
#270652=CARTESIAN_POINT('Ctrl Pts',(-10.4480463102736,12.2,-4.28562691523287));
#270653=CARTESIAN_POINT('Ctrl Pts',(-10.4445082802975,12.2,-4.28571480553221));
#270654=CARTESIAN_POINT('Ctrl Pts',(-10.4409772208336,12.2,-4.28579840003284));
#270655=CARTESIAN_POINT('Ctrl Pts',(-10.4374461613696,12.2,-4.28588199453348));
#270656=CARTESIAN_POINT('Ctrl Pts',(-10.433922071605,12.2,-4.28596129389458));
#270657=CARTESIAN_POINT('Ctrl Pts',(-10.4304049869001,12.2,-4.28603632351648));
#270658=CARTESIAN_POINT('Ctrl Pts',(-10.4268879021952,12.2,-4.28611135313839));
#270659=CARTESIAN_POINT('Ctrl Pts',(-10.4233778229894,12.2,-4.2861821153858));
#270660=CARTESIAN_POINT('Ctrl Pts',(-10.4198747852833,12.2,-4.28624863500838));
#270661=CARTESIAN_POINT('Ctrl Pts',(-10.4163717475773,12.2,-4.28631515463096));
#270662=CARTESIAN_POINT('Ctrl Pts',(-10.4128757505209,12.2,-4.28637743367872));
#270663=CARTESIAN_POINT('Ctrl Pts',(-10.4093868303138,12.2,-4.28643549771864));
#270664=CARTESIAN_POINT('Ctrl Pts',(-10.4058979101066,12.2,-4.28649356175857));
#270665=CARTESIAN_POINT('Ctrl Pts',(-10.4024160668705,12.2,-4.28654741123923));
#270666=CARTESIAN_POINT('Ctrl Pts',(-10.3989413359473,12.2,-4.28659707424039));
#270667=CARTESIAN_POINT('Ctrl Pts',(-10.3954666050242,12.2,-4.28664673724155));
#270668=CARTESIAN_POINT('Ctrl Pts',(-10.3919989866963,12.2,-4.28669221344197));
#270669=CARTESIAN_POINT('Ctrl Pts',(-10.3885385170294,12.2,-4.2867335309827));
#270670=CARTESIAN_POINT('Ctrl Pts',(-10.3850780467338,12.2,-4.28677484853094));
#270671=CARTESIAN_POINT('Ctrl Pts',(-10.3816247257653,12.2,-4.286812007603));
#270672=CARTESIAN_POINT('Ctrl Pts',(-10.3781785885154,12.2,-4.28684503473224));
#270673=CARTESIAN_POINT('Ctrl Pts',(-10.3747324518916,12.2,-4.28687806185548));
#270674=CARTESIAN_POINT('Ctrl Pts',(-10.3712935002508,12.2,-4.2869069595206));
#270675=CARTESIAN_POINT('Ctrl Pts',(-10.3678617691261,12.2,-4.28693175401935));
#270676=CARTESIAN_POINT('Ctrl Pts',(-10.3644300380014,12.2,-4.28695654851809));
#270677=CARTESIAN_POINT('Ctrl Pts',(-10.3610055284049,12.2,-4.28697723981727));
#270678=CARTESIAN_POINT('Ctrl Pts',(-10.3575882757219,12.2,-4.28699385777506));
#270679=CARTESIAN_POINT('Ctrl Pts',(-10.3541710230389,12.2,-4.28701047573284));
#270680=CARTESIAN_POINT('Ctrl Pts',(-10.3507610277449,12.2,-4.28702301880028));
#270681=CARTESIAN_POINT('Ctrl Pts',(-10.3473583265198,12.2,-4.28703151775837));
#270682=CARTESIAN_POINT('Ctrl Pts',(-10.3439556252946,12.2,-4.28704001671645));
#270683=CARTESIAN_POINT('Ctrl Pts',(-10.3405602175136,12.2,-4.28704446969959));
#270684=CARTESIAN_POINT('Ctrl Pts',(-10.3371721403444,12.2,-4.28704490674159));
#270685=CARTESIAN_POINT('Ctrl Pts',(-10.3337840631752,12.2,-4.28704534378359));
#270686=CARTESIAN_POINT('Ctrl Pts',(-10.3304033169305,12.2,-4.28704176500087));
#270687=CARTESIAN_POINT('Ctrl Pts',(-10.3270299377187,12.2,-4.28703419950169));
#270688=CARTESIAN_POINT('Ctrl Pts',(-10.3236565578941,12.2,-4.28702663400113));
#270689=CARTESIAN_POINT('Ctrl Pts',(-10.3202905453716,12.2,-4.28701508123278));
#270690=CARTESIAN_POINT('Ctrl Pts',(-10.3169319370512,12.2,-4.28699957127166));
#270691=CARTESIAN_POINT('Ctrl Pts',(-10.3135733293409,12.2,-4.28698406131335));
#270692=CARTESIAN_POINT('Ctrl Pts',(-10.3102221255145,12.2,-4.28696459394625));
#270693=CARTESIAN_POINT('Ctrl Pts',(-10.3068783635948,12.2,-4.28694119948714));
#270694=CARTESIAN_POINT('Ctrl Pts',(-10.302420014571,12.2,-4.28691000687642));
#270695=CARTESIAN_POINT('Ctrl Pts',(-10.2979748947121,12.2,-4.28687183206897));
#270696=CARTESIAN_POINT('Ctrl Pts',(-10.2935430926291,12.2,-4.28682674679533));
#270697=CARTESIAN_POINT('Ctrl Pts',(-10.2891112899422,12.2,-4.28678166151554));
#270698=CARTESIAN_POINT('Ctrl Pts',(-10.2846928040848,12.2,-4.28672966532104));
#270699=CARTESIAN_POINT('Ctrl Pts',(-10.2802877236233,12.2,-4.28667083076183));
#270700=CARTESIAN_POINT('Ctrl Pts',(-10.2758826437621,12.2,-4.28661199621064));
#270701=CARTESIAN_POINT('Ctrl Pts',(-10.2714909720224,12.2,-4.28654632313818));
#270702=CARTESIAN_POINT('Ctrl Pts',(-10.2671127956604,12.2,-4.28647388575218));
#270703=CARTESIAN_POINT('Ctrl Pts',(-10.2616400747605,12.2,-4.28638333901228));
#270704=CARTESIAN_POINT('Ctrl Pts',(-10.2561884385453,12.2,-4.2862822195345));
#270705=CARTESIAN_POINT('Ctrl Pts',(-10.2507580663219,12.2,-4.28617067550727));
#270706=CARTESIAN_POINT('Ctrl Pts',(-10.2464137683065,12.2,-4.28608144028063));
#270707=CARTESIAN_POINT('Ctrl Pts',(-10.2420830778455,12.2,-4.28598553343928));
#270708=CARTESIAN_POINT('Ctrl Pts',(-10.2377660858889,12.2,-4.2858830282666));
#270709=CARTESIAN_POINT('Ctrl Pts',(-10.2334490945205,12.2,-4.28578052310788));
#270710=CARTESIAN_POINT('Ctrl Pts',(-10.2291458010151,12.2,-4.28567142075143));
#270711=CARTESIAN_POINT('Ctrl Pts',(-10.2248562973725,12.2,-4.28555579753345));
#270712=CARTESIAN_POINT('Ctrl Pts',(-10.2205667931455,12.2,-4.28544017429972));
#270713=CARTESIAN_POINT('Ctrl Pts',(-10.2162910771914,12.2,-4.28531802910246));
#270714=CARTESIAN_POINT('Ctrl Pts',(-10.2120292431267,12.2,-4.28518944053947));
#270715=CARTESIAN_POINT('Ctrl Pts',(-10.2056364926104,12.2,-4.28499655771251));
#270716=CARTESIAN_POINT('Ctrl Pts',(-10.1992749719582,12.2,-4.28478917367839));
#270717=CARTESIAN_POINT('Ctrl Pts',(-10.1929449946034,12.2,-4.28456755577039));
#270718=CARTESIAN_POINT('Ctrl Pts',(-10.188725009317,12.2,-4.28441981048497));
#270719=CARTESIAN_POINT('Ctrl Pts',(-10.1845190429924,12.2,-4.2842657365357));
#270720=CARTESIAN_POINT('Ctrl Pts',(-10.1803271881668,12.2,-4.28410541601841));
#270721=CARTESIAN_POINT('Ctrl Pts',(-10.1761353339124,12.2,-4.28394509552296));
#270722=CARTESIAN_POINT('Ctrl Pts',(-10.1719575910844,12.2,-4.28377852720513));
#270723=CARTESIAN_POINT('Ctrl Pts',(-10.1677940530905,12.2,-4.28360579199743));
#270724=CARTESIAN_POINT('Ctrl Pts',(-10.1636305145293,12.2,-4.2834330567662));
#270725=CARTESIAN_POINT('Ctrl Pts',(-10.1594811815504,12.2,-4.28325415403423));
#270726=CARTESIAN_POINT('Ctrl Pts',(-10.1553461469371,12.2,-4.28306916546819));
#270727=CARTESIAN_POINT('Ctrl Pts',(-10.1512111128872,12.2,-4.28288417692736));
#270728=CARTESIAN_POINT('Ctrl Pts',(-10.1470903771138,12.2,-4.28269310169959));
#270729=CARTESIAN_POINT('Ctrl Pts',(-10.1429840348543,12.2,-4.28249602326193));
#270730=CARTESIAN_POINT('Ctrl Pts',(-10.1388776920352,12.2,-4.28229894479743));
#270731=CARTESIAN_POINT('Ctrl Pts',(-10.1347857421381,12.2,-4.28209586226968));
#270732=CARTESIAN_POINT('Ctrl Pts',(-10.1307082809168,12.2,-4.28188686042456));
#270733=CARTESIAN_POINT('Ctrl Pts',(-10.1266308202511,12.2,-4.28167785860793));
#270734=CARTESIAN_POINT('Ctrl Pts',(-10.1225678474186,12.2,-4.28146293579527));
#270735=CARTESIAN_POINT('Ctrl Pts',(-10.1185194581369,12.2,-4.28124217736946));
#270736=CARTESIAN_POINT('Ctrl Pts',(-10.1144710683037,12.2,-4.28102141891358));
#270737=CARTESIAN_POINT('Ctrl Pts',(-10.1104372633524,12.2,-4.28079482361548));
#270738=CARTESIAN_POINT('Ctrl Pts',(-10.1064181374667,12.2,-4.28056247899171));
#270739=CARTESIAN_POINT('Ctrl Pts',(-10.102399011581,12.2,-4.28033013436793));
#270740=CARTESIAN_POINT('Ctrl Pts',(-10.0983945658136,12.2,-4.28009203847127));
#270741=CARTESIAN_POINT('Ctrl Pts',(-10.0944048965977,12.2,-4.27984827873518));
#270742=CARTESIAN_POINT('Ctrl Pts',(-10.0894178108932,12.2,-4.27954357911489));
#270743=CARTESIAN_POINT('Ctrl Pts',(-10.0844538133152,12.2,-4.27923003070079));
#270744=CARTESIAN_POINT('Ctrl Pts',(-10.0795130951712,12.2,-4.27890780129218));
#270745=CARTESIAN_POINT('Ctrl Pts',(-10.0755605200098,12.2,-4.27865001772314));
#270746=CARTESIAN_POINT('Ctrl Pts',(-10.071622842161,12.2,-4.27838668153135));
#270747=CARTESIAN_POINT('Ctrl Pts',(-10.067700162225,12.2,-4.27811787851671));
#270748=CARTESIAN_POINT('Ctrl Pts',(-10.063777482289,12.2,-4.27784907550205));
#270749=CARTESIAN_POINT('Ctrl Pts',(-10.0598697977658,12.2,-4.27757480846732));
#270750=CARTESIAN_POINT('Ctrl Pts',(-10.0559772103886,12.2,-4.27729516472931));
#270751=CARTESIAN_POINT('Ctrl Pts',(-10.0520846235417,12.2,-4.2770155210294));
#270752=CARTESIAN_POINT('Ctrl Pts',(-10.0482071308073,12.2,-4.2767305019278));
#270753=CARTESIAN_POINT('Ctrl Pts',(-10.0443448334943,12.2,-4.27644019895023));
#270754=CARTESIAN_POINT('Ctrl Pts',(-10.0404825356551,12.2,-4.27614989593311));
#270755=CARTESIAN_POINT('Ctrl Pts',(-10.036635431628,12.2,-4.27585430849834));
#270756=CARTESIAN_POINT('Ctrl Pts',(-10.0328036243652,12.2,-4.27555352942585));
#270757=CARTESIAN_POINT('Ctrl Pts',(-10.0289718176244,12.2,-4.27525275039435));
#270758=CARTESIAN_POINT('Ctrl Pts',(-10.02515530504,12.2,-4.27494678055521));
#270759=CARTESIAN_POINT('Ctrl Pts',(-10.0213541877942,12.2,-4.27463571102542));
#270760=CARTESIAN_POINT('Ctrl Pts',(-10.0166027908485,12.2,-4.27424687408139));
#270761=CARTESIAN_POINT('Ctrl Pts',(-10.0118754504462,12.2,-4.27385007224096));
#270762=CARTESIAN_POINT('Ctrl Pts',(-10.0071723642442,12.2,-4.27344549001692));
#270763=CARTESIAN_POINT('Ctrl Pts',(-10.0034098950776,12.2,-4.27312182422005));
#270764=CARTESIAN_POINT('Ctrl Pts',(-9.99966294813059,12.2,-4.27279317682806));
#270765=CARTESIAN_POINT('Ctrl Pts',(-9.99593162637327,12.2,-4.2724596484205));
#270766=CARTESIAN_POINT('Ctrl Pts',(-9.99220030512434,12.2,-4.27212612005838));
#270767=CARTESIAN_POINT('Ctrl Pts',(-9.98848460922062,12.2,-4.27178770721357));
#270768=CARTESIAN_POINT('Ctrl Pts',(-9.98478464124428,12.2,-4.27144450951971));
#270769=CARTESIAN_POINT('Ctrl Pts',(-9.98108467276383,12.2,-4.2711013117791));
#270770=CARTESIAN_POINT('Ctrl Pts',(-9.97740043215235,12.2,-4.27075332805274));
#270771=CARTESIAN_POINT('Ctrl Pts',(-9.97373202349277,12.2,-4.27040065768217));
#270772=CARTESIAN_POINT('Ctrl Pts',(-9.97006361533301,12.2,-4.27004798735964));
#270773=CARTESIAN_POINT('Ctrl Pts',(-9.96641103905952,12.2,-4.26969063026913));
#270774=CARTESIAN_POINT('Ctrl Pts',(-9.96277439852244,12.2,-4.26932868602124));
#270775=CARTESIAN_POINT('Ctrl Pts',(-9.95913775748987,12.2,-4.26896674172404));
#270776=CARTESIAN_POINT('Ctrl Pts',(-9.95551705261475,12.2,-4.26860021032628));
#270777=CARTESIAN_POINT('Ctrl Pts',(-9.95191239069714,12.2,-4.26822919469466));
#270778=CARTESIAN_POINT('Ctrl Pts',(-9.94830772927065,12.2,-4.26785817911359));
#270779=CARTESIAN_POINT('Ctrl Pts',(-9.94471910794518,12.2,-4.26748267773156));
#270780=CARTESIAN_POINT('Ctrl Pts',(-9.9411466345018,12.2,-4.2671027935218));
#270781=CARTESIAN_POINT('Ctrl Pts',(-9.93668104233251,12.2,-4.26662793822077));
#270782=CARTESIAN_POINT('Ctrl Pts',(-9.93224068220688,12.2,-4.26614623688713));
#270783=CARTESIAN_POINT('Ctrl Pts',(-9.92782576033055,12.2,-4.26565789008193));
#270784=CARTESIAN_POINT('Ctrl Pts',(-9.92429382263698,12.2,-4.26526721261647));
#270785=CARTESIAN_POINT('Ctrl Pts',(-9.9207781666315,12.2,-4.26487228385883));
#270786=CARTESIAN_POINT('Ctrl Pts',(-9.91727889899741,12.2,-4.2644732082257));
#270787=CARTESIAN_POINT('Ctrl Pts',(-9.91377963184011,12.2,-4.26407413264694));
#270788=CARTESIAN_POINT('Ctrl Pts',(-9.91029675463041,12.2,-4.26367091152358));
#270789=CARTESIAN_POINT('Ctrl Pts',(-9.90683037446141,12.2,-4.2632636507591));
#270790=CARTESIAN_POINT('Ctrl Pts',(-9.9033639938201,12.2,-4.26285638993914));
#270791=CARTESIAN_POINT('Ctrl Pts',(-9.89991411150273,12.2,-4.26244509095004));
#270792=CARTESIAN_POINT('Ctrl Pts',(-9.89648083526114,12.2,-4.26202986148271));
#270793=CARTESIAN_POINT('Ctrl Pts',(-9.89304755948733,12.2,-4.26161463207195));
#270794=CARTESIAN_POINT('Ctrl Pts',(-9.88963089192687,12.2,-4.26119547374255));
#270795=CARTESIAN_POINT('Ctrl Pts',(-9.88623094081422,12.2,-4.26077249427752));
#270796=CARTESIAN_POINT('Ctrl Pts',(-9.88283098923834,12.2,-4.26034951475486));
#270797=CARTESIAN_POINT('Ctrl Pts',(-9.87944775677138,12.2,-4.25992271612239));
#270798=CARTESIAN_POINT('Ctrl Pts',(-9.87608135173937,12.2,-4.25949220870807));
#270799=CARTESIAN_POINT('Ctrl Pts',(-9.87271494716603,12.2,-4.25906170135241));
#270800=CARTESIAN_POINT('Ctrl Pts',(-9.86936537151861,12.2,-4.25862748709378));
#270801=CARTESIAN_POINT('Ctrl Pts',(-9.86603273634488,12.2,-4.25818967762994));
#270802=CARTESIAN_POINT('Ctrl Pts',(-9.86270010071707,12.2,-4.25775186810645));
#270803=CARTESIAN_POINT('Ctrl Pts',(-9.85938440543254,12.2,-4.25731046239373));
#270804=CARTESIAN_POINT('Ctrl Pts',(-9.85608576497498,12.2,-4.25686557875836));
#270805=CARTESIAN_POINT('Ctrl Pts',(-9.85196246462775,12.2,-4.25630947424447));
#270806=CARTESIAN_POINT('Ctrl Pts',(-9.84786581016064,12.2,-4.25574793036898));
#270807=CARTESIAN_POINT('Ctrl Pts',(-9.84379602423943,12.2,-4.25518117849139));
#270808=CARTESIAN_POINT('Ctrl Pts',(-9.83972623831823,12.2,-4.25461442661379));
#270809=CARTESIAN_POINT('Ctrl Pts',(-9.83568332359722,12.2,-4.25404246459586));
#270810=CARTESIAN_POINT('Ctrl Pts',(-9.83166750102918,12.2,-4.2534655252206));
#270811=CARTESIAN_POINT('Ctrl Pts',(-9.82765167846116,12.2,-4.25288858584534));
#270812=CARTESIAN_POINT('Ctrl Pts',(-9.82366294997854,12.2,-4.25230666850077));
#270813=CARTESIAN_POINT('Ctrl Pts',(-9.81970154400775,12.2,-4.2517200100283));
#270814=CARTESIAN_POINT('Ctrl Pts',(-9.81574013803695,12.2,-4.25113335155583));
#270815=CARTESIAN_POINT('Ctrl Pts',(-9.81180605415433,12.2,-4.25054195020015));
#270816=CARTESIAN_POINT('Ctrl Pts',(-9.807899520753,12.2,-4.24994604839436));
#270817=CARTESIAN_POINT('Ctrl Pts',(-9.80399298735167,12.2,-4.24935014658857));
#270818=CARTESIAN_POINT('Ctrl Pts',(-9.8001140056157,12.2,-4.2487497429881));
#270819=CARTESIAN_POINT('Ctrl Pts',(-9.79626280778635,12.2,-4.24814508288815));
#270820=CARTESIAN_POINT('Ctrl Pts',(-9.79241160995701,12.2,-4.24754042278821));
#270821=CARTESIAN_POINT('Ctrl Pts',(-9.78858819659571,12.2,-4.24693150449796));
#270822=CARTESIAN_POINT('Ctrl Pts',(-9.78479280152856,12.2,-4.24631857942819));
#270823=CARTESIAN_POINT('Ctrl Pts',(-9.7809974064614,12.2,-4.24570565435841));
#270824=CARTESIAN_POINT('Ctrl Pts',(-9.77723002954193,12.2,-4.24508871978581));
#270825=CARTESIAN_POINT('Ctrl Pts',(-9.77349091100259,12.2,-4.24446803145217));
#270826=CARTESIAN_POINT('Ctrl Pts',(-9.76975179287081,12.2,-4.24384734318619));
#270827=CARTESIAN_POINT('Ctrl Pts',(-9.7660409302215,12.2,-4.2432228994912));
#270828=CARTESIAN_POINT('Ctrl Pts',(-9.76235856402331,12.2,-4.24259496032382));
#270829=CARTESIAN_POINT('Ctrl Pts',(-9.75867619742375,12.2,-4.241967021088));
#270830=CARTESIAN_POINT('Ctrl Pts',(-9.75502232828207,12.2,-4.24133558456055));
#270831=CARTESIAN_POINT('Ctrl Pts',(-9.75139719918249,12.2,-4.24070091386637));
#270832=CARTESIAN_POINT('Ctrl Pts',(-9.74777207008294,12.2,-4.2400662431722));
#270833=CARTESIAN_POINT('Ctrl Pts',(-9.74417568140555,12.2,-4.23942833990622));
#270834=CARTESIAN_POINT('Ctrl Pts',(-9.74060827865587,12.2,-4.23878747008274));
#270835=CARTESIAN_POINT('Ctrl Pts',(-9.73704087590621,12.2,-4.23814660025926));
#270836=CARTESIAN_POINT('Ctrl Pts',(-9.73350245789784,12.2,-4.23750276470881));
#270837=CARTESIAN_POINT('Ctrl Pts',(-9.729993277688,12.2,-4.23685623575062));
#270838=CARTESIAN_POINT('Ctrl Pts',(-9.72648409747816,12.2,-4.23620970679243));
#270839=CARTESIAN_POINT('Ctrl Pts',(-9.72300415096625,12.2,-4.23556048506471));
#270840=CARTESIAN_POINT('Ctrl Pts',(-9.71955369270082,12.2,-4.23490884784262));
#270841=CARTESIAN_POINT('Ctrl Pts',(-9.7161032344354,12.2,-4.23425721062053));
#270842=CARTESIAN_POINT('Ctrl Pts',(-9.71268226287843,12.2,-4.23360315869224));
#270843=CARTESIAN_POINT('Ctrl Pts',(-9.70929103529349,12.2,-4.23294697480038));
#270844=CARTESIAN_POINT('Ctrl Pts',(-9.70589980770855,12.2,-4.23229079090851));
#270845=CARTESIAN_POINT('Ctrl Pts',(-9.70253832226108,12.2,-4.23163247609447));
#270846=CARTESIAN_POINT('Ctrl Pts',(-9.69920683823331,12.2,-4.23097231727502));
#270847=CARTESIAN_POINT('Ctrl Pts',(-9.69587535420553,12.2,-4.23031215845557));
#270848=CARTESIAN_POINT('Ctrl Pts',(-9.69257387279077,12.2,-4.22965015711379));
#270849=CARTESIAN_POINT('Ctrl Pts',(-9.6893026537482,12.2,-4.22898660745799));
#270850=CARTESIAN_POINT('Ctrl Pts',(-9.68537719103977,12.2,-4.22819034789997));
#270851=CARTESIAN_POINT('Ctrl Pts',(-9.68149530621348,12.2,-4.22739185813947));
#270852=CARTESIAN_POINT('Ctrl Pts',(-9.67765746143433,12.2,-4.22659165858529));
#270853=CARTESIAN_POINT('Ctrl Pts',(-9.67381961630657,12.2,-4.22579145895842));
#270854=CARTESIAN_POINT('Ctrl Pts',(-9.67002580960094,12.2,-4.22498954883965));
#270855=CARTESIAN_POINT('Ctrl Pts',(-9.66627650764965,12.2,-4.22418646212915));
#270856=CARTESIAN_POINT('Ctrl Pts',(-9.66252720603892,12.2,-4.22338337549158));
#270857=CARTESIAN_POINT('Ctrl Pts',(-9.65882241063247,12.2,-4.22257910981861));
#270858=CARTESIAN_POINT('Ctrl Pts',(-9.65516259326737,12.2,-4.22177421326448));
#270859=CARTESIAN_POINT('Ctrl Pts',(-9.65150277590228,12.2,-4.22096931671035));
#270860=CARTESIAN_POINT('Ctrl Pts',(-9.64788794090864,12.2,-4.22016378734798));
#270861=CARTESIAN_POINT('Ctrl Pts',(-9.64431856645303,12.2,-4.21935818404392));
#270862=CARTESIAN_POINT('Ctrl Pts',(-9.64074919199741,12.2,-4.21855258073986));
#270863=CARTESIAN_POINT('Ctrl Pts',(-9.63722528043084,12.2,-4.21774690530022));
#270864=CARTESIAN_POINT('Ctrl Pts',(-9.63374732280408,12.2,-4.21694172807945));
#270865=CARTESIAN_POINT('Ctrl Pts',(-9.6302693648614,12.2,-4.21613655078553));
#270866=CARTESIAN_POINT('Ctrl Pts',(-9.62683735939812,12.2,-4.21533187426664));
#270867=CARTESIAN_POINT('Ctrl Pts',(-9.62345180854899,12.2,-4.21452828222289));
#270868=CARTESIAN_POINT('Ctrl Pts',(-9.62006625800738,12.2,-4.21372469025214));
#270869=CARTESIAN_POINT('Ctrl Pts',(-9.61672715945526,12.2,-4.21292218647492));
#270870=CARTESIAN_POINT('Ctrl Pts',(-9.61343502397647,12.2,-4.21212136950038));
#270871=CARTESIAN_POINT('Ctrl Pts',(-9.61014288849769,12.2,-4.21132055252583));
#270872=CARTESIAN_POINT('Ctrl Pts',(-9.60689771440225,12.2,-4.21052142478306));
#270873=CARTESIAN_POINT('Ctrl Pts',(-9.60370002284853,12.2,-4.20972460356186));
#270874=CARTESIAN_POINT('Ctrl Pts',(-9.60050233100436,12.2,-4.20892778226828));
#270875=CARTESIAN_POINT('Ctrl Pts',(-9.59735211976474,12.2,-4.20813326644989));
#270876=CARTESIAN_POINT('Ctrl Pts',(-9.59424991709778,12.2,-4.20734169224021));
#270877=CARTESIAN_POINT('Ctrl Pts',(-9.59063068107566,12.2,-4.20641818910345));
#270878=CARTESIAN_POINT('Ctrl Pts',(-9.58707679118468,12.2,-4.20549868362322));
#270879=CARTESIAN_POINT('Ctrl Pts',(-9.58358910284248,12.2,-4.20458421777711));
#270880=CARTESIAN_POINT('Ctrl Pts',(-9.58059965534293,12.2,-4.20380038981747));
#270881=CARTESIAN_POINT('Ctrl Pts',(-9.57765884601473,12.2,-4.20302026229984));
#270882=CARTESIAN_POINT('Ctrl Pts',(-9.57476722835925,12.2,-4.20224450742441));
#270883=CARTESIAN_POINT('Ctrl Pts',(-9.57187561096643,12.2,-4.20146875261945));
#270884=CARTESIAN_POINT('Ctrl Pts',(-9.5690331816459,12.2,-4.200697371576));
#270885=CARTESIAN_POINT('Ctrl Pts',(-9.56624050723457,12.2,-4.19993105176702));
#270886=CARTESIAN_POINT('Ctrl Pts',(-9.56344783282325,12.2,-4.19916473195804));
#270887=CARTESIAN_POINT('Ctrl Pts',(-9.56070491039072,12.2,-4.19840347414696));
#270888=CARTESIAN_POINT('Ctrl Pts',(-9.55801231606847,12.2,-4.19764798759069));
#270889=CARTESIAN_POINT('Ctrl Pts',(-9.55531972150164,12.2,-4.19689250096579));
#270890=CARTESIAN_POINT('Ctrl Pts',(-9.55267745390051,12.2,-4.19614278658039));
#270891=CARTESIAN_POINT('Ctrl Pts',(-9.55008610146608,12.2,-4.19539957191979));
#270892=CARTESIAN_POINT('Ctrl Pts',(-9.54749474926703,12.2,-4.1946563573267));
#270893=CARTESIAN_POINT('Ctrl Pts',(-9.54495431257621,12.2,-4.1939196443235));
#270894=CARTESIAN_POINT('Ctrl Pts',(-9.54246538949996,12.2,-4.19319018001667));
#270895=CARTESIAN_POINT('Ctrl Pts',(-9.53997646642371,12.2,-4.19246071570983));
#270896=CARTESIAN_POINT('Ctrl Pts',(-9.53753905943302,12.2,-4.19173850167931));
#270897=CARTESIAN_POINT('Ctrl Pts',(-9.53515378023084,12.2,-4.19102431033578));
#270898=CARTESIAN_POINT('Ctrl Pts',(-9.532768500812,12.2,-4.19031011892737));
#270899=CARTESIAN_POINT('Ctrl Pts',(-9.53043534938044,12.2,-4.18960395015306));
#270900=CARTESIAN_POINT('Ctrl Pts',(-9.52815495700975,12.2,-4.18890659786566));
#270901=CARTESIAN_POINT('Ctrl Pts',(-9.52587456484618,12.2,-4.18820924564159));
#270902=CARTESIAN_POINT('Ctrl Pts',(-9.52364692716305,12.2,-4.18752071042808));
#270903=CARTESIAN_POINT('Ctrl Pts',(-9.52147269123231,12.2,-4.18684181128302));
#270904=CARTESIAN_POINT('Ctrl Pts',(-9.51929845530156,12.2,-4.18616291213796));
#270905=CARTESIAN_POINT('Ctrl Pts',(-9.51717761946508,12.2,-4.1854936485958));
#270906=CARTESIAN_POINT('Ctrl Pts',(-9.51511084262116,12.2,-4.18483486378594));
#270907=CARTESIAN_POINT('Ctrl Pts',(-9.51304406558951,12.2,-4.18417607891625));
#270908=CARTESIAN_POINT('Ctrl Pts',(-9.51103134861454,12.2,-4.18352777418118));
#270909=CARTESIAN_POINT('Ctrl Pts',(-9.50907336576156,12.2,-4.18289081914723));
#270910=CARTESIAN_POINT('Ctrl Pts',(-9.50711538308643,12.2,-4.18225386417116));
#270911=CARTESIAN_POINT('Ctrl Pts',(-9.50521213716328,12.2,-4.18162825895214));
#270912=CARTESIAN_POINT('Ctrl Pts',(-9.50336431839948,12.2,-4.18101490022495));
#270913=CARTESIAN_POINT('Ctrl Pts',(-9.5009094281732,12.2,-4.18020003224435));
#270914=CARTESIAN_POINT('Ctrl Pts',(-9.49855236068315,12.2,-4.17940677765138));
#270915=CARTESIAN_POINT('Ctrl Pts',(-9.49629481200006,12.2,-4.17863732200002));
#270916=CARTESIAN_POINT('Ctrl Pts',(-9.49629481200006,15.2,-4.17863732200002));
#270917=CARTESIAN_POINT('Ctrl Pts',(-9.49798593465032,15.2,-4.17921371881934));
#270918=CARTESIAN_POINT('Ctrl Pts',(-9.49973290438102,15.2,-4.17980347257967));
#270919=CARTESIAN_POINT('Ctrl Pts',(-9.50153500151926,15.2,-4.18040565840071));
#270920=CARTESIAN_POINT('Ctrl Pts',(-9.50334578928083,15.2,-4.18101074826615));
#270921=CARTESIAN_POINT('Ctrl Pts',(-9.5052122402571,15.2,-4.18162839186116));
#270922=CARTESIAN_POINT('Ctrl Pts',(-9.50713365521097,15.2,-4.1822576807609));
#270923=CARTESIAN_POINT('Ctrl Pts',(-9.50905506999029,15.2,-4.18288696960348));
#270924=CARTESIAN_POINT('Ctrl Pts',(-9.51103144900704,15.2,-4.18352790432366));
#270925=CARTESIAN_POINT('Ctrl Pts',(-9.51306211076662,15.2,-4.1841796053));
#270926=CARTESIAN_POINT('Ctrl Pts',(-9.5150927725262,15.2,-4.18483130627633));
#270927=CARTESIAN_POINT('Ctrl Pts',(-9.5171777169505,15.2,-4.18549377286806));
#270928=CARTESIAN_POINT('Ctrl Pts',(-9.51931627980988,15.2,-4.18616615495998));
#270929=CARTESIAN_POINT('Ctrl Pts',(-9.52145484286351,15.2,-4.18683853711298));
#270930=CARTESIAN_POINT('Ctrl Pts',(-9.5236470221604,15.2,-4.18752083260373));
#270931=CARTESIAN_POINT('Ctrl Pts',(-9.52589217403637,15.2,-4.18821221580869));
#270932=CARTESIAN_POINT('Ctrl Pts',(-9.52813732570841,15.2,-4.18890359895087));
#270933=CARTESIAN_POINT('Ctrl Pts',(-9.53043544305898,15.2,-4.18960406977284));
#270934=CARTESIAN_POINT('Ctrl Pts',(-9.53278589998437,15.2,-4.19031282325032));
#270935=CARTESIAN_POINT('Ctrl Pts',(-9.53513635690976,15.2,-4.1910215767278));
#270936=CARTESIAN_POINT('Ctrl Pts',(-9.53753914979115,15.2,-4.19173861702053));
#270937=CARTESIAN_POINT('Ctrl Pts',(-9.53999366086641,15.2,-4.19246316149388));
#270938=CARTESIAN_POINT('Ctrl Pts',(-9.54244817216462,15.2,-4.19318770603304));
#270939=CARTESIAN_POINT('Ctrl Pts',(-9.54495440171918,15.2,-4.1939197558398));
#270940=CARTESIAN_POINT('Ctrl Pts',(-9.54751174402873,15.2,-4.1946585525472));
#270941=CARTESIAN_POINT('Ctrl Pts',(-9.55006908610598,15.2,-4.1953973491875));
#270942=CARTESIAN_POINT('Ctrl Pts',(-9.55267754023118,15.2,-4.19614289582637));
#270943=CARTESIAN_POINT('Ctrl Pts',(-9.55533651838677,15.2,-4.19689445254932));
#270944=CARTESIAN_POINT('Ctrl Pts',(-9.5584386597293,15.2,-4.19777126877162));
#270945=CARTESIAN_POINT('Ctrl Pts',(-9.56160956564257,15.2,-4.19865626775237));
#270946=CARTESIAN_POINT('Ctrl Pts',(-9.5648483190859,15.2,-4.19954831685002));
#270947=CARTESIAN_POINT('Ctrl Pts',(-9.56762439332181,15.2,-4.2003129303226));
#270948=CARTESIAN_POINT('Ctrl Pts',(-9.57045031642585,15.2,-4.20108272011183));
#270949=CARTESIAN_POINT('Ctrl Pts',(-9.57332552165687,15.2,-4.20185699783389));
#270950=CARTESIAN_POINT('Ctrl Pts',(-9.57620072688789,15.2,-4.20263127555595));
#270951=CARTESIAN_POINT('Ctrl Pts',(-9.57912521616496,15.2,-4.20341004053597));
#270952=CARTESIAN_POINT('Ctrl Pts',(-9.5820984345548,15.2,-4.20419261550737));
#270953=CARTESIAN_POINT('Ctrl Pts',(-9.58507165294463,15.2,-4.20497519047877));
#270954=CARTESIAN_POINT('Ctrl Pts',(-9.58809360218851,15.2,-4.20576157844286));
#270955=CARTESIAN_POINT('Ctrl Pts',(-9.59116373765701,15.2,-4.20655112141395));
#270956=CARTESIAN_POINT('Ctrl Pts',(-9.59423387340437,15.2,-4.20734066445676));
#270957=CARTESIAN_POINT('Ctrl Pts',(-9.59735219801478,15.2,-4.20813336084157));
#270958=CARTESIAN_POINT('Ctrl Pts',(-9.60051817768938,15.2,-4.20892857480169));
#270959=CARTESIAN_POINT('Ctrl Pts',(-9.60368415707643,15.2,-4.20972378868958));
#270960=CARTESIAN_POINT('Ctrl Pts',(-9.60689779235132,15.2,-4.21052151836891));
#270961=CARTESIAN_POINT('Ctrl Pts',(-9.61015856181413,15.2,-4.21132113950644));
#270962=CARTESIAN_POINT('Ctrl Pts',(-9.61341933127693,15.2,-4.21212076064398));
#270963=CARTESIAN_POINT('Ctrl Pts',(-9.61672723454271,15.2,-4.2129222766751));
#270964=CARTESIAN_POINT('Ctrl Pts',(-9.62008176091767,15.2,-4.21372507597917));
#270965=CARTESIAN_POINT('Ctrl Pts',(-9.62343628759735,15.2,-4.21452787535618));
#270966=CARTESIAN_POINT('Ctrl Pts',(-9.62683743399816,15.2,-4.21533196143331));
#270967=CARTESIAN_POINT('Ctrl Pts',(-9.63028470168804,15.2,-4.21613673981054));
#270968=CARTESIAN_POINT('Ctrl Pts',(-9.6337319690648,15.2,-4.21694151811467));
#270969=CARTESIAN_POINT('Ctrl Pts',(-9.63722535415264,15.2,-4.21774698955026));
#270970=CARTESIAN_POINT('Ctrl Pts',(-9.64076436479004,15.2,-4.21855257777465));
#270971=CARTESIAN_POINT('Ctrl Pts',(-9.64430337542743,15.2,-4.21935816599903));
#270972=CARTESIAN_POINT('Ctrl Pts',(-9.64788801348929,15.2,-4.2201638697998));
#270973=CARTESIAN_POINT('Ctrl Pts',(-9.65151778835434,15.2,-4.22096912618724));
#270974=CARTESIAN_POINT('Ctrl Pts',(-9.65575252591672,15.2,-4.22190859202135));
#270975=CARTESIAN_POINT('Ctrl Pts',(-9.66004870645519,15.2,-4.22284744803079));
#270976=CARTESIAN_POINT('Ctrl Pts',(-9.66440556818162,15.2,-4.22378482329965));
#270977=CARTESIAN_POINT('Ctrl Pts',(-9.66814002089615,15.2,-4.22458828777411));
#270978=CARTESIAN_POINT('Ctrl Pts',(-9.67191905874185,15.2,-4.22539066415839));
#270979=CARTESIAN_POINT('Ctrl Pts',(-9.67574221059993,15.2,-4.2261914186294));
#270980=CARTESIAN_POINT('Ctrl Pts',(-9.67956536280529,15.2,-4.22699217317315));
#270981=CARTESIAN_POINT('Ctrl Pts',(-9.68343263213405,15.2,-4.22779130676898));
#270982=CARTESIAN_POINT('Ctrl Pts',(-9.68734355637842,15.2,-4.22858829460211));
#270983=CARTESIAN_POINT('Ctrl Pts',(-9.6906026597378,15.2,-4.22925245109352));
#270984=CARTESIAN_POINT('Ctrl Pts',(-9.69389207818172,15.2,-4.22991511941438));
#270985=CARTESIAN_POINT('Ctrl Pts',(-9.69721155068418,15.2,-4.23057600330313));
#270986=CARTESIAN_POINT('Ctrl Pts',(-9.70053102318663,15.2,-4.23123688719186));
#270987=CARTESIAN_POINT('Ctrl Pts',(-9.70388054947846,15.2,-4.23189598631391));
#270988=CARTESIAN_POINT('Ctrl Pts',(-9.70725987017534,15.2,-4.23255301103596));
#270989=CARTESIAN_POINT('Ctrl Pts',(-9.71063919050386,15.2,-4.23321003568639));
#270990=CARTESIAN_POINT('Ctrl Pts',(-9.71404830561634,15.2,-4.23386498646894));
#270991=CARTESIAN_POINT('Ctrl Pts',(-9.71748695780855,15.2,-4.23451757785633));
#270992=CARTESIAN_POINT('Ctrl Pts',(-9.72092561037556,15.2,-4.23517016931485));
#270993=CARTESIAN_POINT('Ctrl Pts',(-9.72439380244493,15.2,-4.23582040258733));
#270994=CARTESIAN_POINT('Ctrl Pts',(-9.72789127910919,15.2,-4.23646799744865));
#270995=CARTESIAN_POINT('Ctrl Pts',(-9.73138875577346,15.2,-4.23711559230997));
#270996=CARTESIAN_POINT('Ctrl Pts',(-9.73491551809502,15.2,-4.23776054943765));
#270997=CARTESIAN_POINT('Ctrl Pts',(-9.73847131660398,15.2,-4.23840259440048));
#270998=CARTESIAN_POINT('Ctrl Pts',(-9.74273827504728,15.2,-4.23917304839787));
#270999=CARTESIAN_POINT('Ctrl Pts',(-9.74704704402595,15.2,-4.23993930899185));
#271000=CARTESIAN_POINT('Ctrl Pts',(-9.75139719918249,15.2,-4.24070091386637));
#271001=CARTESIAN_POINT('Ctrl Pts',(-9.75502232828206,15.2,-4.24133558456055));
#271002=CARTESIAN_POINT('Ctrl Pts',(-9.75867619742377,15.2,-4.241967021088));
#271003=CARTESIAN_POINT('Ctrl Pts',(-9.76235856402332,15.2,-4.24259496032382));
#271004=CARTESIAN_POINT('Ctrl Pts',(-9.7660409302215,15.2,-4.2432228994912));
#271005=CARTESIAN_POINT('Ctrl Pts',(-9.76975179287081,15.2,-4.24384734318619));
#271006=CARTESIAN_POINT('Ctrl Pts',(-9.77349091100258,15.2,-4.24446803145217));
#271007=CARTESIAN_POINT('Ctrl Pts',(-9.77723002954193,15.2,-4.24508871978581));
#271008=CARTESIAN_POINT('Ctrl Pts',(-9.78099740646142,15.2,-4.24570565435842));
#271009=CARTESIAN_POINT('Ctrl Pts',(-9.78479280152856,15.2,-4.24631857942819));
#271010=CARTESIAN_POINT('Ctrl Pts',(-9.78858819659569,15.2,-4.24693150449795));
#271011=CARTESIAN_POINT('Ctrl Pts',(-9.792411609957,15.2,-4.24754042278821));
#271012=CARTESIAN_POINT('Ctrl Pts',(-9.79626280778635,15.2,-4.24814508288815));
#271013=CARTESIAN_POINT('Ctrl Pts',(-9.8001140056157,15.2,-4.2487497429881));
#271014=CARTESIAN_POINT('Ctrl Pts',(-9.80399298735165,15.2,-4.24935014658857));
#271015=CARTESIAN_POINT('Ctrl Pts',(-9.807899520753,15.2,-4.24994604839436));
#271016=CARTESIAN_POINT('Ctrl Pts',(-9.8125873610901,15.2,-4.25066113060029));
#271017=CARTESIAN_POINT('Ctrl Pts',(-9.8173148738238,15.2,-4.25136973113041));
#271018=CARTESIAN_POINT('Ctrl Pts',(-9.82208166525291,15.2,-4.25207143425151));
#271019=CARTESIAN_POINT('Ctrl Pts',(-9.82605399122733,15.2,-4.25265618682056));
#271020=CARTESIAN_POINT('Ctrl Pts',(-9.83005359423003,15.2,-4.25323615056453));
#271021=CARTESIAN_POINT('Ctrl Pts',(-9.83408024451002,15.2,-4.25381108980023));
#271022=CARTESIAN_POINT('Ctrl Pts',(-9.8381068943511,15.2,-4.25438602897326));
#271023=CARTESIAN_POINT('Ctrl Pts',(-9.84216059387434,15.2,-4.25495594343173));
#271024=CARTESIAN_POINT('Ctrl Pts',(-9.84624111773293,15.2,-4.25552060267617));
#271025=CARTESIAN_POINT('Ctrl Pts',(-9.8503216420363,15.2,-4.25608526198215));
#271026=CARTESIAN_POINT('Ctrl Pts',(-9.85442898980036,15.2,-4.25664466564936));
#271027=CARTESIAN_POINT('Ctrl Pts',(-9.85856294070094,15.2,-4.25719858738591));
#271028=CARTESIAN_POINT('Ctrl Pts',(-9.86187010160164,15.2,-4.25764172479931));
#271029=CARTESIAN_POINT('Ctrl Pts',(-9.86519428825217,15.2,-4.2580813537857));
#271030=CARTESIAN_POINT('Ctrl Pts',(-9.86853538672727,15.2,-4.25851735870032));
#271031=CARTESIAN_POINT('Ctrl Pts',(-9.87187648474714,15.2,-4.25895336355554));
#271032=CARTESIAN_POINT('Ctrl Pts',(-9.87523449661472,15.2,-4.25938574610627));
#271033=CARTESIAN_POINT('Ctrl Pts',(-9.87860930844822,15.2,-4.25981439223828));
#271034=CARTESIAN_POINT('Ctrl Pts',(-9.88198412074152,15.2,-4.26024303842869));
#271035=CARTESIAN_POINT('Ctrl Pts',(-9.88537573348923,15.2,-4.26066794827986));
#271036=CARTESIAN_POINT('Ctrl Pts',(-9.88878403650832,15.2,-4.26108901102503));
#271037=CARTESIAN_POINT('Ctrl Pts',(-9.8921923395274,15.2,-4.2615100737702));
#271038=CARTESIAN_POINT('Ctrl Pts',(-9.89561733290955,15.2,-4.26192728748992));
#271039=CARTESIAN_POINT('Ctrl Pts',(-9.89905890482103,15.2,-4.26234054506759));
#271040=CARTESIAN_POINT('Ctrl Pts',(-9.90250047626358,15.2,-4.26275380258896));
#271041=CARTESIAN_POINT('Ctrl Pts',(-9.90595862855205,15.2,-4.26316310312547));
#271042=CARTESIAN_POINT('Ctrl Pts',(-9.90943325100597,15.2,-4.26356833731642));
#271043=CARTESIAN_POINT('Ctrl Pts',(-9.9129078739333,15.2,-4.26397357156258));
#271044=CARTESIAN_POINT('Ctrl Pts',(-9.91639896647509,15.2,-4.26437473989929));
#271045=CARTESIAN_POINT('Ctrl Pts',(-9.91990642155681,15.2,-4.2647717360316));
#271046=CARTESIAN_POINT('Ctrl Pts',(-9.92341387616062,15.2,-4.26516873210983));
#271047=CARTESIAN_POINT('Ctrl Pts',(-9.92693769303174,15.2,-4.26556155464971));
#271048=CARTESIAN_POINT('Ctrl Pts',(-9.93047776368575,15.2,-4.26595009895156));
#271049=CARTESIAN_POINT('Ctrl Pts',(-9.93401783482209,15.2,-4.26633864330635));
#271050=CARTESIAN_POINT('Ctrl Pts',(-9.93757416057167,15.2,-4.26672290926028));
#271051=CARTESIAN_POINT('Ctrl Pts',(-9.9411466345018,15.2,-4.2671027935218));
#271052=CARTESIAN_POINT('Ctrl Pts',(-9.94471910794518,15.2,-4.26748267773156));
#271053=CARTESIAN_POINT('Ctrl Pts',(-9.94830772927064,15.2,-4.26785817911359));
#271054=CARTESIAN_POINT('Ctrl Pts',(-9.95191239069713,15.2,-4.26822919469466));
#271055=CARTESIAN_POINT('Ctrl Pts',(-9.95551705261475,15.2,-4.26860021032628));
#271056=CARTESIAN_POINT('Ctrl Pts',(-9.95913775748988,15.2,-4.26896674172404));
#271057=CARTESIAN_POINT('Ctrl Pts',(-9.96277439852244,15.2,-4.26932868602124));
#271058=CARTESIAN_POINT('Ctrl Pts',(-9.96641103905951,15.2,-4.26969063026913));
#271059=CARTESIAN_POINT('Ctrl Pts',(-9.970063615333,15.2,-4.27004798735964));
#271060=CARTESIAN_POINT('Ctrl Pts',(-9.97373202349277,15.2,-4.27040065768217));
#271061=CARTESIAN_POINT('Ctrl Pts',(-9.97740043215235,15.2,-4.27075332805274));
#271062=CARTESIAN_POINT('Ctrl Pts',(-9.98108467276382,15.2,-4.2711013117791));
#271063=CARTESIAN_POINT('Ctrl Pts',(-9.98478464124428,15.2,-4.27144450951971));
#271064=CARTESIAN_POINT('Ctrl Pts',(-9.98848460922063,15.2,-4.27178770721357));
#271065=CARTESIAN_POINT('Ctrl Pts',(-9.99220030512435,15.2,-4.27212612005838));
#271066=CARTESIAN_POINT('Ctrl Pts',(-9.99593162637327,15.2,-4.2724596484205));
#271067=CARTESIAN_POINT('Ctrl Pts',(-9.99966294813057,15.2,-4.27279317682806));
#271068=CARTESIAN_POINT('Ctrl Pts',(-10.0034098950776,15.2,-4.27312182422005));
#271069=CARTESIAN_POINT('Ctrl Pts',(-10.0071723642442,15.2,-4.27344549001692));
#271070=CARTESIAN_POINT('Ctrl Pts',(-10.0109348328982,15.2,-4.2737691557697));
#271071=CARTESIAN_POINT('Ctrl Pts',(-10.0147128244415,15.2,-4.27408784212387));
#271072=CARTESIAN_POINT('Ctrl Pts',(-10.0185062371298,15.2,-4.27440145443209));
#271073=CARTESIAN_POINT('Ctrl Pts',(-10.0222996503349,15.2,-4.27471506678303));
#271074=CARTESIAN_POINT('Ctrl Pts',(-10.0261084852055,15.2,-4.27502360426684));
#271075=CARTESIAN_POINT('Ctrl Pts',(-10.029932639025,15.2,-4.27532697328337));
#271076=CARTESIAN_POINT('Ctrl Pts',(-10.0337567928445,15.2,-4.2756303422999));
#271077=CARTESIAN_POINT('Ctrl Pts',(-10.0375962668992,15.2,-4.27592854345473));
#271078=CARTESIAN_POINT('Ctrl Pts',(-10.0414509613886,15.2,-4.27622148258126));
#271079=CARTESIAN_POINT('Ctrl Pts',(-10.0453056553528,15.2,-4.27651442166789));
#271080=CARTESIAN_POINT('Ctrl Pts',(-10.0491755684057,15.2,-4.2768020990494));
#271081=CARTESIAN_POINT('Ctrl Pts',(-10.0530606022724,15.2,-4.27708442524984));
#271082=CARTESIAN_POINT('Ctrl Pts',(-10.0569456366684,15.2,-4.27736675148875));
#271083=CARTESIAN_POINT('Ctrl Pts',(-10.0608457913308,15.2,-4.27764372328296));
#271084=CARTESIAN_POINT('Ctrl Pts',(-10.0647609666568,15.2,-4.27791525301943));
#271085=CARTESIAN_POINT('Ctrl Pts',(-10.0686761414494,15.2,-4.2781867827189));
#271086=CARTESIAN_POINT('Ctrl Pts',(-10.0726063385511,15.2,-4.27845286927185));
#271087=CARTESIAN_POINT('Ctrl Pts',(-10.0765514578943,15.2,-4.27871342369535));
#271088=CARTESIAN_POINT('Ctrl Pts',(-10.080496577775,15.2,-4.27897397815436));
#271089=CARTESIAN_POINT('Ctrl Pts',(-10.0844566198742,15.2,-4.27922900031341));
#271090=CARTESIAN_POINT('Ctrl Pts',(-10.0884314885685,15.2,-4.2794784020612));
#271091=CARTESIAN_POINT('Ctrl Pts',(-10.0924063567212,15.2,-4.279727803775));
#271092=CARTESIAN_POINT('Ctrl Pts',(-10.096396049365,15.2,-4.27997158488294));
#271093=CARTESIAN_POINT('Ctrl Pts',(-10.1004004706478,15.2,-4.28020965919719));
#271094=CARTESIAN_POINT('Ctrl Pts',(-10.1054059976604,15.2,-4.28050725211432));
#271095=CARTESIAN_POINT('Ctrl Pts',(-10.1104345373599,15.2,-4.280795926509));
#271096=CARTESIAN_POINT('Ctrl Pts',(-10.1154859011781,15.2,-4.28107551539837));
#271097=CARTESIAN_POINT('Ctrl Pts',(-10.1195269924529,15.2,-4.28129918652205));
#271098=CARTESIAN_POINT('Ctrl Pts',(-10.1235826926101,15.2,-4.2815170439367));
#271099=CARTESIAN_POINT('Ctrl Pts',(-10.1276529038329,15.2,-4.28172900055897));
#271100=CARTESIAN_POINT('Ctrl Pts',(-10.1317231145011,15.2,-4.28194095715237));
#271101=CARTESIAN_POINT('Ctrl Pts',(-10.1358078367674,15.2,-4.28214701488237));
#271102=CARTESIAN_POINT('Ctrl Pts',(-10.1399069769136,15.2,-4.28234708998764));
#271103=CARTESIAN_POINT('Ctrl Pts',(-10.1450309025152,15.2,-4.28259718388967));
#271104=CARTESIAN_POINT('Ctrl Pts',(-10.1501773539521,15.2,-4.28283792977325));
#271105=CARTESIAN_POINT('Ctrl Pts',(-10.1553461469371,15.2,-4.28306916546819));
#271106=CARTESIAN_POINT('Ctrl Pts',(-10.1594811815504,15.2,-4.28325415403423));
#271107=CARTESIAN_POINT('Ctrl Pts',(-10.1636305145293,15.2,-4.2834330567662));
#271108=CARTESIAN_POINT('Ctrl Pts',(-10.1677940530905,15.2,-4.28360579199743));
#271109=CARTESIAN_POINT('Ctrl Pts',(-10.1719575910844,15.2,-4.28377852720513));
#271110=CARTESIAN_POINT('Ctrl Pts',(-10.1761353339124,15.2,-4.28394509552296));
#271111=CARTESIAN_POINT('Ctrl Pts',(-10.1803271881668,15.2,-4.28410541601841));
#271112=CARTESIAN_POINT('Ctrl Pts',(-10.1855670064132,15.2,-4.2843058166541));
#271113=CARTESIAN_POINT('Ctrl Pts',(-10.1908288736391,15.2,-4.28449645575431));
#271114=CARTESIAN_POINT('Ctrl Pts',(-10.1961126098879,15.2,-4.28467717721316));
#271115=CARTESIAN_POINT('Ctrl Pts',(-10.2003395991174,15.2,-4.28482175438812));
#271116=CARTESIAN_POINT('Ctrl Pts',(-10.2045805838318,15.2,-4.2849599860651));
#271117=CARTESIAN_POINT('Ctrl Pts',(-10.208835472398,15.2,-4.28509179196076));
#271118=CARTESIAN_POINT('Ctrl Pts',(-10.2130903603844,15.2,-4.28522359783845));
#271119=CARTESIAN_POINT('Ctrl Pts',(-10.2173591515521,15.2,-4.28534897924708));
#271120=CARTESIAN_POINT('Ctrl Pts',(-10.221641755137,15.2,-4.28546785846609));
#271121=CARTESIAN_POINT('Ctrl Pts',(-10.2269950100557,15.2,-4.285616457502));
#271122=CARTESIAN_POINT('Ctrl Pts',(-10.2323698462372,15.2,-4.28575489680773));
#271123=CARTESIAN_POINT('Ctrl Pts',(-10.2377660858889,15.2,-4.2858830282666));
#271124=CARTESIAN_POINT('Ctrl Pts',(-10.2420830778455,15.2,-4.28598553343928));
#271125=CARTESIAN_POINT('Ctrl Pts',(-10.2464137683065,15.2,-4.28608144028063));
#271126=CARTESIAN_POINT('Ctrl Pts',(-10.2507580663219,15.2,-4.28617067550727));
#271127=CARTESIAN_POINT('Ctrl Pts',(-10.2551023637455,15.2,-4.28625991072176));
#271128=CARTESIAN_POINT('Ctrl Pts',(-10.2594602700253,15.2,-4.28634247359639));
#271129=CARTESIAN_POINT('Ctrl Pts',(-10.2638316936074,15.2,-4.286418290039));
#271130=CARTESIAN_POINT('Ctrl Pts',(-10.2692959735317,15.2,-4.28651306060003));
#271131=CARTESIAN_POINT('Ctrl Pts',(-10.2747813733467,15.2,-4.28659728756683));
#271132=CARTESIAN_POINT('Ctrl Pts',(-10.2802877236233,15.2,-4.28667083076183));
#271133=CARTESIAN_POINT('Ctrl Pts',(-10.2857940739,15.2,-4.28674437395684));
#271134=CARTESIAN_POINT('Ctrl Pts',(-10.2913213701106,15.2,-4.28680723204601));
#271135=CARTESIAN_POINT('Ctrl Pts',(-10.2968694391373,15.2,-4.28685926371324));
#271136=CARTESIAN_POINT('Ctrl Pts',(-10.3013078946005,15.2,-4.2869008890493));
#271137=CARTESIAN_POINT('Ctrl Pts',(-10.305759646986,15.2,-4.28693558648229));
#271138=CARTESIAN_POINT('Ctrl Pts',(-10.310224605898,15.2,-4.28696328376236));
#271139=CARTESIAN_POINT('Ctrl Pts',(-10.3135733247778,15.2,-4.28698405672052));
#271140=CARTESIAN_POINT('Ctrl Pts',(-10.3169294728717,15.2,-4.28700089251886));
#271141=CARTESIAN_POINT('Ctrl Pts',(-10.3202930125834,15.2,-4.28701376097638));
#271142=CARTESIAN_POINT('Ctrl Pts',(-10.3236565522952,15.2,-4.2870266294339));
#271143=CARTESIAN_POINT('Ctrl Pts',(-10.3270274840894,15.2,-4.28703553053356));
#271144=CARTESIAN_POINT('Ctrl Pts',(-10.3304057707583,15.2,-4.28704043499171));
#271145=CARTESIAN_POINT('Ctrl Pts',(-10.3337840574273,15.2,-4.28704533944986));
#271146=CARTESIAN_POINT('Ctrl Pts',(-10.3371696989875,15.2,-4.28704624758318));
#271147=CARTESIAN_POINT('Ctrl Pts',(-10.3405626591553,15.2,-4.28704313000032));
#271148=CARTESIAN_POINT('Ctrl Pts',(-10.3439556193231,15.2,-4.28704001241745));
#271149=CARTESIAN_POINT('Ctrl Pts',(-10.3473558971952,15.2,-4.28703286801852));
#271150=CARTESIAN_POINT('Ctrl Pts',(-10.3507634570741,15.2,-4.28702166947717));
#271151=CARTESIAN_POINT('Ctrl Pts',(-10.354171016953,15.2,-4.28701047093582));
#271152=CARTESIAN_POINT('Ctrl Pts',(-10.3575858588293,15.2,-4.28699521771966));
#271153=CARTESIAN_POINT('Ctrl Pts',(-10.3610079455373,15.2,-4.28697588072092));
#271154=CARTESIAN_POINT('Ctrl Pts',(-10.364430032867,15.2,-4.28695654371867));
#271155=CARTESIAN_POINT('Ctrl Pts',(-10.3678593656488,15.2,-4.2869331236986));
#271156=CARTESIAN_POINT('Ctrl Pts',(-10.3712959070242,15.2,-4.28690559073571));
#271157=CARTESIAN_POINT('Ctrl Pts',(-10.3758779611509,15.2,-4.28686888012685));
#271158=CARTESIAN_POINT('Ctrl Pts',(-10.3804728309398,15.2,-4.28682486137171));
#271159=CARTESIAN_POINT('Ctrl Pts',(-10.3850804303401,15.2,-4.28677346348751));
#271160=CARTESIAN_POINT('Ctrl Pts',(-10.3885361300473,15.2,-4.2867349150726));
#271161=CARTESIAN_POINT('Ctrl Pts',(-10.3919989904823,15.2,-4.28669221775923));
#271162=CARTESIAN_POINT('Ctrl Pts',(-10.3954689758204,15.2,-4.28664534275907));
#271163=CARTESIAN_POINT('Ctrl Pts',(-10.3989389611585,15.2,-4.28659846775892));
#271164=CARTESIAN_POINT('Ctrl Pts',(-10.4024160710514,15.2,-4.28654741552617));
#271165=CARTESIAN_POINT('Ctrl Pts',(-10.4059002692988,15.2,-4.28649215802875));
#271166=CARTESIAN_POINT('Ctrl Pts',(-10.4093844681792,15.2,-4.2864369005213));
#271167=CARTESIAN_POINT('Ctrl Pts',(-10.4128757560866,15.2,-4.28637743741266));
#271168=CARTESIAN_POINT('Ctrl Pts',(-10.416374096471,15.2,-4.28631374194449));
#271169=CARTESIAN_POINT('Ctrl Pts',(-10.4210385492576,15.2,-4.28622881467288));
#271170=CARTESIAN_POINT('Ctrl Pts',(-10.4257155408398,15.2,-4.28613636300781));
#271171=CARTESIAN_POINT('Ctrl Pts',(-10.4304049869001,15.2,-4.28603632351649));
#271172=CARTESIAN_POINT('Ctrl Pts',(-10.433922071605,15.2,-4.28596129389459));
#271173=CARTESIAN_POINT('Ctrl Pts',(-10.4374461613696,15.2,-4.28588199453348));
#271174=CARTESIAN_POINT('Ctrl Pts',(-10.4409772208336,15.2,-4.28579840003285));
#271175=CARTESIAN_POINT('Ctrl Pts',(-10.4445082802975,15.2,-4.28571480553221));
#271176=CARTESIAN_POINT('Ctrl Pts',(-10.4480463102736,15.2,-4.28562691523287));
#271177=CARTESIAN_POINT('Ctrl Pts',(-10.4515912749772,15.2,-4.28553470319514));
#271178=CARTESIAN_POINT('Ctrl Pts',(-10.4551362403248,15.2,-4.28544249114066));
#271179=CARTESIAN_POINT('Ctrl Pts',(-10.458688140191,15.2,-4.28534595605997));
#271180=CARTESIAN_POINT('Ctrl Pts',(-10.4622469395425,15.2,-4.28524507346138));
#271181=CARTESIAN_POINT('Ctrl Pts',(-10.4658057382475,15.2,-4.28514419088112));
#271182=CARTESIAN_POINT('Ctrl Pts',(-10.4693714358854,15.2,-4.28503895943442));
#271183=CARTESIAN_POINT('Ctrl Pts',(-10.4729439986312,15.2,-4.28492935297969));
#271184=CARTESIAN_POINT('Ctrl Pts',(-10.4777074154093,15.2,-4.28478321104668));
#271185=CARTESIAN_POINT('Ctrl Pts',(-10.4824830352626,15.2,-4.28462929291802));
#271186=CARTESIAN_POINT('Ctrl Pts',(-10.4872707759256,15.2,-4.28446753504316));
#271187=CARTESIAN_POINT('Ctrl Pts',(-10.4908615822381,15.2,-4.28434621660946));
#271188=CARTESIAN_POINT('Ctrl Pts',(-10.494459206711,15.2,-4.28422048939119));
#271189=CARTESIAN_POINT('Ctrl Pts',(-10.4980636140691,15.2,-4.284090326955));
#271190=CARTESIAN_POINT('Ctrl Pts',(-10.5028694894552,15.2,-4.28391677707949));
#271191=CARTESIAN_POINT('Ctrl Pts',(-10.5076874224697,15.2,-4.28373534306608));
#271192=CARTESIAN_POINT('Ctrl Pts',(-10.5125173337634,15.2,-4.28354596502517));
#271193=CARTESIAN_POINT('Ctrl Pts',(-10.5161397673982,15.2,-4.28340393148804));
#271194=CARTESIAN_POINT('Ctrl Pts',(-10.5197689368532,15.2,-4.28325742871055));
#271195=CARTESIAN_POINT('Ctrl Pts',(-10.5234048090538,15.2,-4.28310643179976));
#271196=CARTESIAN_POINT('Ctrl Pts',(-10.5270406812545,15.2,-4.28295543488898));
#271197=CARTESIAN_POINT('Ctrl Pts',(-10.530683256088,15.2,-4.28279994442849));
#271198=CARTESIAN_POINT('Ctrl Pts',(-10.5343324992461,15.2,-4.28263993501826));
#271199=CARTESIAN_POINT('Ctrl Pts',(-10.5379817430673,15.2,-4.28247992557895));
#271200=CARTESIAN_POINT('Ctrl Pts',(-10.5416376541653,15.2,-4.28231539797171));
#271201=CARTESIAN_POINT('Ctrl Pts',(-10.5453001995318,15.2,-4.28214632648818));
#271202=CARTESIAN_POINT('Ctrl Pts',(-10.5489627442329,15.2,-4.28197725503537));
#271203=CARTESIAN_POINT('Ctrl Pts',(-10.5526319228771,15.2,-4.28180363963515));
#271204=CARTESIAN_POINT('Ctrl Pts',(-10.5563077012613,15.2,-4.28162545671553));
#271205=CARTESIAN_POINT('Ctrl Pts',(-10.5599834796454,15.2,-4.28144727379591));
#271206=CARTESIAN_POINT('Ctrl Pts',(-10.5636658569023,15.2,-4.28126452353981));
#271207=CARTESIAN_POINT('Ctrl Pts',(-10.5673547996439,15.2,-4.28107717971288));
#271208=CARTESIAN_POINT('Ctrl Pts',(-10.5710437423854,15.2,-4.28088983588595));
#271209=CARTESIAN_POINT('Ctrl Pts',(-10.5747392502845,15.2,-4.28069790029291));
#271210=CARTESIAN_POINT('Ctrl Pts',(-10.578441290525,15.2,-4.28050134796672));
#271211=CARTESIAN_POINT('Ctrl Pts',(-10.5821433307655,15.2,-4.28030479564053));
#271212=CARTESIAN_POINT('Ctrl Pts',(-10.585851903114,15.2,-4.28010362866452));
#271213=CARTESIAN_POINT('Ctrl Pts',(-10.5895669738118,15.2,-4.27989782075574));
#271214=CARTESIAN_POINT('Ctrl Pts',(-10.5932820445096,15.2,-4.27969201284695));
#271215=CARTESIAN_POINT('Ctrl Pts',(-10.5970036129621,15.2,-4.27948156501067));
#271216=CARTESIAN_POINT('Ctrl Pts',(-10.6007316453038,15.2,-4.27926645254995));
#271217=CARTESIAN_POINT('Ctrl Pts',(-10.6044596776455,15.2,-4.27905134008923));
#271218=CARTESIAN_POINT('Ctrl Pts',(-10.6081941723546,15.2,-4.27883156294018));
#271219=CARTESIAN_POINT('Ctrl Pts',(-10.6119350967178,15.2,-4.27860709757398));
#271220=CARTESIAN_POINT('Ctrl Pts',(-10.6156760217606,15.2,-4.27838263216699));
#271221=CARTESIAN_POINT('Ctrl Pts',(-10.6194233779552,15.2,-4.27815347906703));
#271222=CARTESIAN_POINT('Ctrl Pts',(-10.6231771325433,15.2,-4.27791961719906));
#271223=CARTESIAN_POINT('Ctrl Pts',(-10.6269308864495,15.2,-4.27768575537358));
#271224=CARTESIAN_POINT('Ctrl Pts',(-10.6306910415803,15.2,-4.27744718588169));
#271225=CARTESIAN_POINT('Ctrl Pts',(-10.6344575621523,15.2,-4.27720388343178));
#271226=CARTESIAN_POINT('Ctrl Pts',(-10.6382240827244,15.2,-4.27696058098188));
#271227=CARTESIAN_POINT('Ctrl Pts',(-10.6419969666069,15.2,-4.27671254602513));
#271228=CARTESIAN_POINT('Ctrl Pts',(-10.6457761752368,15.2,-4.27645974949148));
#271229=CARTESIAN_POINT('Ctrl Pts',(-10.6495553838666,15.2,-4.27620695295783));
#271230=CARTESIAN_POINT('Ctrl Pts',(-10.6533409158171,15.2,-4.27594939275859));
#271231=CARTESIAN_POINT('Ctrl Pts',(-10.6571327397799,15.2,-4.27568705147528));
#271232=CARTESIAN_POINT('Ctrl Pts',(-10.6634524466141,15.2,-4.27524981598722));
#271233=CARTESIAN_POINT('Ctrl Pts',(-10.6697896272814,15.2,-4.27479929410113));
#271234=CARTESIAN_POINT('Ctrl Pts',(-10.6761442620001,15.2,-4.27433546900001));
#271235=CARTESIAN_POINT('Ctrl Pts',(-9.86852965800006,15.2,-3.20199116200001));
#271236=CARTESIAN_POINT('Ctrl Pts',(-9.86852965800006,11.6,-3.20199116200001));
#271237=CARTESIAN_POINT('Ctrl Pts',(-9.86869026600005,15.2,-3.20205902700001));
#271238=CARTESIAN_POINT('Ctrl Pts',(-9.86869026600005,11.6,-3.20205902700002));
#271239=CARTESIAN_POINT('Ctrl Pts',(-9.86901705900006,15.2,-3.20219720600001));
#271240=CARTESIAN_POINT('Ctrl Pts',(-9.86901705900006,11.6,-3.20219720600001));
#271241=CARTESIAN_POINT('Ctrl Pts',(-9.86951212500006,15.2,-3.20240682500001));
#271242=CARTESIAN_POINT('Ctrl Pts',(-9.86951212500006,11.6,-3.20240682500002));
#271243=CARTESIAN_POINT('Ctrl Pts',(-9.87017881200006,15.2,-3.20268969800001));
#271244=CARTESIAN_POINT('Ctrl Pts',(-9.87017881200006,11.6,-3.20268969800001));
#271245=CARTESIAN_POINT('Ctrl Pts',(-9.87102171700006,15.2,-3.20304833000002));
#271246=CARTESIAN_POINT('Ctrl Pts',(-9.87102171700006,11.6,-3.20304833000002));
#271247=CARTESIAN_POINT('Ctrl Pts',(-9.87187791600006,15.2,-3.20341363600001));
#271248=CARTESIAN_POINT('Ctrl Pts',(-9.87187791600006,11.6,-3.20341363600001));
#271249=CARTESIAN_POINT('Ctrl Pts',(-9.87274249600006,15.2,-3.20378354300002));
#271250=CARTESIAN_POINT('Ctrl Pts',(-9.87274249600006,11.6,-3.20378354300002));
#271251=CARTESIAN_POINT('Ctrl Pts',(-9.87361542500006,15.2,-3.20415805700001));
#271252=CARTESIAN_POINT('Ctrl Pts',(-9.87361542500006,11.6,-3.20415805700002));
#271253=CARTESIAN_POINT('Ctrl Pts',(-9.87449667000006,15.2,-3.20453718400001));
#271254=CARTESIAN_POINT('Ctrl Pts',(-9.87449667000006,11.6,-3.20453718400001));
#271255=CARTESIAN_POINT('Ctrl Pts',(-9.87538620100005,15.2,-3.20492093000002));
#271256=CARTESIAN_POINT('Ctrl Pts',(-9.87538620100005,11.6,-3.20492093000002));
#271257=CARTESIAN_POINT('Ctrl Pts',(-9.87628398500006,15.2,-3.20530930200002));
#271258=CARTESIAN_POINT('Ctrl Pts',(-9.87628398500006,11.6,-3.20530930200002));
#271259=CARTESIAN_POINT('Ctrl Pts',(-9.87718999100006,15.2,-3.20570230600001));
#271260=CARTESIAN_POINT('Ctrl Pts',(-9.87718999100006,11.6,-3.20570230600001));
#271261=CARTESIAN_POINT('Ctrl Pts',(-9.87810418900006,15.2,-3.20609994500002));
#271262=CARTESIAN_POINT('Ctrl Pts',(-9.87810418900006,11.6,-3.20609994500002));
#271263=CARTESIAN_POINT('Ctrl Pts',(-9.87902654600006,15.2,-3.20650222700001));
#271264=CARTESIAN_POINT('Ctrl Pts',(-9.87902654600006,11.6,-3.20650222700001));
#271265=CARTESIAN_POINT('Ctrl Pts',(-9.87995703200006,15.2,-3.20690915900002));
#271266=CARTESIAN_POINT('Ctrl Pts',(-9.87995703200006,11.6,-3.20690915900002));
#271267=CARTESIAN_POINT('Ctrl Pts',(-9.88089561700006,15.2,-3.20732074400001));
#271268=CARTESIAN_POINT('Ctrl Pts',(-9.88089561700006,11.6,-3.20732074400001));
#271269=CARTESIAN_POINT('Ctrl Pts',(-9.88184227000006,15.2,-3.20773698900001));
#271270=CARTESIAN_POINT('Ctrl Pts',(-9.88184227000006,11.6,-3.20773698900001));
#271271=CARTESIAN_POINT('Ctrl Pts',(-9.88279696000006,15.2,-3.20815790000001));
#271272=CARTESIAN_POINT('Ctrl Pts',(-9.88279696000006,11.6,-3.20815790000002));
#271273=CARTESIAN_POINT('Ctrl Pts',(-9.88375965700006,15.2,-3.20858348200002));
#271274=CARTESIAN_POINT('Ctrl Pts',(-9.88375965700006,11.6,-3.20858348200002));
#271275=CARTESIAN_POINT('Ctrl Pts',(-9.88473033100006,15.2,-3.20901374200002));
#271276=CARTESIAN_POINT('Ctrl Pts',(-9.88473033100006,11.6,-3.20901374200002));
#271277=CARTESIAN_POINT('Ctrl Pts',(-9.88570895100005,15.2,-3.20944868300002));
#271278=CARTESIAN_POINT('Ctrl Pts',(-9.88570895100005,11.6,-3.20944868300002));
#271279=CARTESIAN_POINT('Ctrl Pts',(-9.88669548900006,15.2,-3.20988831100002));
#271280=CARTESIAN_POINT('Ctrl Pts',(-9.88669548900006,11.6,-3.20988831100002));
#271281=CARTESIAN_POINT('Ctrl Pts',(-9.88768991400006,15.2,-3.21033263400002));
#271282=CARTESIAN_POINT('Ctrl Pts',(-9.88768991400006,11.6,-3.21033263400002));
#271283=CARTESIAN_POINT('Ctrl Pts',(-9.88869219600006,15.2,-3.21078165400001));
#271284=CARTESIAN_POINT('Ctrl Pts',(-9.88869219600006,11.6,-3.21078165400001));
#271285=CARTESIAN_POINT('Ctrl Pts',(-9.88970230600006,15.2,-3.21123537900001));
#271286=CARTESIAN_POINT('Ctrl Pts',(-9.88970230600006,11.6,-3.21123537900002));
#271287=CARTESIAN_POINT('Ctrl Pts',(-9.89072021400006,15.2,-3.21169381400002));
#271288=CARTESIAN_POINT('Ctrl Pts',(-9.89072021400006,11.6,-3.21169381400002));
#271289=CARTESIAN_POINT('Ctrl Pts',(-9.89174589300006,15.2,-3.21215696200001));
#271290=CARTESIAN_POINT('Ctrl Pts',(-9.89174589300006,11.6,-3.21215696200001));
#271291=CARTESIAN_POINT('Ctrl Pts',(-9.89277931200006,15.2,-3.21262483100002));
#271292=CARTESIAN_POINT('Ctrl Pts',(-9.89277931200006,11.6,-3.21262483100002));
#271293=CARTESIAN_POINT('Ctrl Pts',(-9.89382044300006,15.2,-3.21309742400001));
#271294=CARTESIAN_POINT('Ctrl Pts',(-9.89382044300006,11.6,-3.21309742400001));
#271295=CARTESIAN_POINT('Ctrl Pts',(-9.89486925600006,15.2,-3.21357474900001));
#271296=CARTESIAN_POINT('Ctrl Pts',(-9.89486925600006,11.6,-3.21357474900001));
#271297=CARTESIAN_POINT('Ctrl Pts',(-9.89592572400005,15.2,-3.21405680800002));
#271298=CARTESIAN_POINT('Ctrl Pts',(-9.89592572400005,11.6,-3.21405680800002));
#271299=CARTESIAN_POINT('Ctrl Pts',(-9.89698981700006,15.2,-3.21454360700002));
#271300=CARTESIAN_POINT('Ctrl Pts',(-9.89698981700006,11.6,-3.21454360700002));
#271301=CARTESIAN_POINT('Ctrl Pts',(-9.89806150700005,15.2,-3.21503515300002));
#271302=CARTESIAN_POINT('Ctrl Pts',(-9.89806150700005,11.6,-3.21503515300002));
#271303=CARTESIAN_POINT('Ctrl Pts',(-9.89914076600006,15.2,-3.21553144900002));
#271304=CARTESIAN_POINT('Ctrl Pts',(-9.89914076600006,11.6,-3.21553144900002));
#271305=CARTESIAN_POINT('Ctrl Pts',(-9.90022756600006,15.2,-3.21603250000001));
#271306=CARTESIAN_POINT('Ctrl Pts',(-9.90022756600006,11.6,-3.21603250000001));
#271307=CARTESIAN_POINT('Ctrl Pts',(-9.90132187900005,15.2,-3.21653831200001));
#271308=CARTESIAN_POINT('Ctrl Pts',(-9.90132187900005,11.6,-3.21653831200001));
#271309=CARTESIAN_POINT('Ctrl Pts',(-9.90242367500005,15.2,-3.21704889000001));
#271310=CARTESIAN_POINT('Ctrl Pts',(-9.90242367500005,11.6,-3.21704889000001));
#271311=CARTESIAN_POINT('Ctrl Pts',(-9.90353292900006,15.2,-3.21756423800001));
#271312=CARTESIAN_POINT('Ctrl Pts',(-9.90353292900006,11.6,-3.21756423800002));
#271313=CARTESIAN_POINT('Ctrl Pts',(-9.90464961300006,15.2,-3.21808436100001));
#271314=CARTESIAN_POINT('Ctrl Pts',(-9.90464961300006,11.6,-3.21808436100001));
#271315=CARTESIAN_POINT('Ctrl Pts',(-9.90577369800006,15.2,-3.21860926300001));
#271316=CARTESIAN_POINT('Ctrl Pts',(-9.90577369800006,11.6,-3.21860926300001));
#271317=CARTESIAN_POINT('Ctrl Pts',(-9.90690515800006,15.2,-3.21913895100002));
#271318=CARTESIAN_POINT('Ctrl Pts',(-9.90690515800006,11.6,-3.21913895100002));
#271319=CARTESIAN_POINT('Ctrl Pts',(-9.90804396400006,15.2,-3.21967342800002));
#271320=CARTESIAN_POINT('Ctrl Pts',(-9.90804396400006,11.6,-3.21967342800002));
#271321=CARTESIAN_POINT('Ctrl Pts',(-9.90919009200006,15.2,-3.22021269900001));
#271322=CARTESIAN_POINT('Ctrl Pts',(-9.90919009200006,11.6,-3.22021269900001));
#271323=CARTESIAN_POINT('Ctrl Pts',(-9.91034351100006,15.2,-3.22075677000001));
#271324=CARTESIAN_POINT('Ctrl Pts',(-9.91034351100006,11.6,-3.22075677000001));
#271325=CARTESIAN_POINT('Ctrl Pts',(-9.91150419600006,15.2,-3.22130564300001));
#271326=CARTESIAN_POINT('Ctrl Pts',(-9.91150419600006,11.6,-3.22130564300001));
#271327=CARTESIAN_POINT('Ctrl Pts',(-9.91267212100006,15.2,-3.22185932500001));
#271328=CARTESIAN_POINT('Ctrl Pts',(-9.91267212100006,11.6,-3.22185932500001));
#271329=CARTESIAN_POINT('Ctrl Pts',(-9.91384725800006,15.2,-3.22241781900001));
#271330=CARTESIAN_POINT('Ctrl Pts',(-9.91384725800006,11.6,-3.22241781900001));
#271331=CARTESIAN_POINT('Ctrl Pts',(-9.91502958100006,15.2,-3.22298113000001));
#271332=CARTESIAN_POINT('Ctrl Pts',(-9.91502958100006,11.6,-3.22298113000001));
#271333=CARTESIAN_POINT('Ctrl Pts',(-9.91621906300006,15.2,-3.22354926400001));
#271334=CARTESIAN_POINT('Ctrl Pts',(-9.91621906300006,11.6,-3.22354926400001));
#271335=CARTESIAN_POINT('Ctrl Pts',(-9.91741567800006,15.2,-3.22412222300001));
#271336=CARTESIAN_POINT('Ctrl Pts',(-9.91741567800006,11.6,-3.22412222300001));
#271337=CARTESIAN_POINT('Ctrl Pts',(-9.91861940000006,15.2,-3.22470001300001));
#271338=CARTESIAN_POINT('Ctrl Pts',(-9.91861940000006,11.6,-3.22470001300002));
#271339=CARTESIAN_POINT('Ctrl Pts',(-9.91983020200006,15.2,-3.22528263800002));
#271340=CARTESIAN_POINT('Ctrl Pts',(-9.91983020200006,11.6,-3.22528263800002));
#271341=CARTESIAN_POINT('Ctrl Pts',(-9.92104805900006,15.2,-3.22587010200001));
#271342=CARTESIAN_POINT('Ctrl Pts',(-9.92104805900006,11.6,-3.22587010200001));
#271343=CARTESIAN_POINT('Ctrl Pts',(-9.92227294400006,15.2,-3.22646241000001));
#271344=CARTESIAN_POINT('Ctrl Pts',(-9.92227294400006,11.6,-3.22646241000002));
#271345=CARTESIAN_POINT('Ctrl Pts',(-9.92350483300006,15.2,-3.22705956700001));
#271346=CARTESIAN_POINT('Ctrl Pts',(-9.92350483300006,11.6,-3.22705956700002));
#271347=CARTESIAN_POINT('Ctrl Pts',(-9.92474369700006,15.2,-3.22766157500002));
#271348=CARTESIAN_POINT('Ctrl Pts',(-9.92474369700006,11.6,-3.22766157500002));
#271349=CARTESIAN_POINT('Ctrl Pts',(-9.92598951400005,15.2,-3.22826844000002));
#271350=CARTESIAN_POINT('Ctrl Pts',(-9.92598951400005,11.6,-3.22826844000002));
#271351=CARTESIAN_POINT('Ctrl Pts',(-9.92724225800006,15.2,-3.22888016500002));
#271352=CARTESIAN_POINT('Ctrl Pts',(-9.92724225800006,11.6,-3.22888016500002));
#271353=CARTESIAN_POINT('Ctrl Pts',(-9.92850190000006,15.2,-3.22949675600002));
#271354=CARTESIAN_POINT('Ctrl Pts',(-9.92850190000006,11.6,-3.22949675600002));
#271355=CARTESIAN_POINT('Ctrl Pts',(-9.92976841900006,15.2,-3.23011821500002));
#271356=CARTESIAN_POINT('Ctrl Pts',(-9.92976841900006,11.6,-3.23011821500002));
#271357=CARTESIAN_POINT('Ctrl Pts',(-9.93104178800005,15.2,-3.23074454800001));
#271358=CARTESIAN_POINT('Ctrl Pts',(-9.93104178800005,11.6,-3.23074454800001));
#271359=CARTESIAN_POINT('Ctrl Pts',(-9.93232198100005,15.2,-3.23137575800001));
#271360=CARTESIAN_POINT('Ctrl Pts',(-9.93232198100005,11.6,-3.23137575800002));
#271361=CARTESIAN_POINT('Ctrl Pts',(-9.93360897600006,15.2,-3.23201184900002));
#271362=CARTESIAN_POINT('Ctrl Pts',(-9.93360897600006,11.6,-3.23201184900002));
#271363=CARTESIAN_POINT('Ctrl Pts',(-9.93490274500006,15.2,-3.23265282600001));
#271364=CARTESIAN_POINT('Ctrl Pts',(-9.93490274500006,11.6,-3.23265282600001));
#271365=CARTESIAN_POINT('Ctrl Pts',(-9.93620326500006,15.2,-3.23329869300002));
#271366=CARTESIAN_POINT('Ctrl Pts',(-9.93620326500006,11.6,-3.23329869300002));
#271367=CARTESIAN_POINT('Ctrl Pts',(-9.93751051000006,15.2,-3.23394945100001));
#271368=CARTESIAN_POINT('Ctrl Pts',(-9.93751051000006,11.6,-3.23394945100001));
#271369=CARTESIAN_POINT('Ctrl Pts',(-9.93882445700006,15.2,-3.23460510900001));
#271370=CARTESIAN_POINT('Ctrl Pts',(-9.93882445700006,11.6,-3.23460510900001));
#271371=CARTESIAN_POINT('Ctrl Pts',(-9.94014508100006,15.2,-3.23526566700002));
#271372=CARTESIAN_POINT('Ctrl Pts',(-9.94014508100006,11.6,-3.23526566700002));
#271373=CARTESIAN_POINT('Ctrl Pts',(-9.94147235700006,15.2,-3.23593113000001));
#271374=CARTESIAN_POINT('Ctrl Pts',(-9.94147235700006,11.6,-3.23593113000001));
#271375=CARTESIAN_POINT('Ctrl Pts',(-9.94280626000006,15.2,-3.23660150200002));
#271376=CARTESIAN_POINT('Ctrl Pts',(-9.94280626000006,11.6,-3.23660150200002));
#271377=CARTESIAN_POINT('Ctrl Pts',(-9.94414676800006,15.2,-3.23727678600001));
#271378=CARTESIAN_POINT('Ctrl Pts',(-9.94414676800006,11.6,-3.23727678600001));
#271379=CARTESIAN_POINT('Ctrl Pts',(-9.94549385600006,15.2,-3.23795698700001));
#271380=CARTESIAN_POINT('Ctrl Pts',(-9.94549385600006,11.6,-3.23795698700002));
#271381=CARTESIAN_POINT('Ctrl Pts',(-9.94684750000006,15.2,-3.23864211000001));
#271382=CARTESIAN_POINT('Ctrl Pts',(-9.94684750000006,11.6,-3.23864211000001));
#271383=CARTESIAN_POINT('Ctrl Pts',(-9.94820767500006,15.2,-3.23933215500002));
#271384=CARTESIAN_POINT('Ctrl Pts',(-9.94820767500006,11.6,-3.23933215500002));
#271385=CARTESIAN_POINT('Ctrl Pts',(-9.94957435800006,15.2,-3.24002712800001));
#271386=CARTESIAN_POINT('Ctrl Pts',(-9.94957435800006,11.6,-3.24002712800001));
#271387=CARTESIAN_POINT('Ctrl Pts',(-9.95094752700006,15.2,-3.24072703300001));
#271388=CARTESIAN_POINT('Ctrl Pts',(-9.95094752700006,11.6,-3.24072703300002));
#271389=CARTESIAN_POINT('Ctrl Pts',(-9.95232715600006,15.2,-3.24143187300002));
#271390=CARTESIAN_POINT('Ctrl Pts',(-9.95232715600006,11.6,-3.24143187300002));
#271391=CARTESIAN_POINT('Ctrl Pts',(-9.95371322300005,15.2,-3.24214165200001));
#271392=CARTESIAN_POINT('Ctrl Pts',(-9.95371322300005,11.6,-3.24214165200001));
#271393=CARTESIAN_POINT('Ctrl Pts',(-9.95510570200006,15.2,-3.24285637300001));
#271394=CARTESIAN_POINT('Ctrl Pts',(-9.95510570200006,11.6,-3.24285637300001));
#271395=CARTESIAN_POINT('Ctrl Pts',(-9.95650457300006,15.2,-3.24357604000001));
#271396=CARTESIAN_POINT('Ctrl Pts',(-9.95650457300006,11.6,-3.24357604000001));
#271397=CARTESIAN_POINT('Ctrl Pts',(-9.95790981200006,15.2,-3.24430065600001));
#271398=CARTESIAN_POINT('Ctrl Pts',(-9.95790981200006,11.6,-3.24430065600001));
#271399=CARTESIAN_POINT('Ctrl Pts',(-9.95932139400006,15.2,-3.24503022600001));
#271400=CARTESIAN_POINT('Ctrl Pts',(-9.95932139400006,11.6,-3.24503022600001));
#271401=CARTESIAN_POINT('Ctrl Pts',(-9.96073929800006,15.2,-3.24576475100002));
#271402=CARTESIAN_POINT('Ctrl Pts',(-9.96073929800006,11.6,-3.24576475100002));
#271403=CARTESIAN_POINT('Ctrl Pts',(-9.96216349900006,15.2,-3.24650423600001));
#271404=CARTESIAN_POINT('Ctrl Pts',(-9.96216349900006,11.6,-3.24650423600001));
#271405=CARTESIAN_POINT('Ctrl Pts',(-9.96359397600006,15.2,-3.24724868500001));
#271406=CARTESIAN_POINT('Ctrl Pts',(-9.96359397600006,11.6,-3.24724868500002));
#271407=CARTESIAN_POINT('Ctrl Pts',(-9.96503070500006,15.2,-3.24799810100002));
#271408=CARTESIAN_POINT('Ctrl Pts',(-9.96503070500006,11.6,-3.24799810100002));
#271409=CARTESIAN_POINT('Ctrl Pts',(-9.96647366400006,15.2,-3.24875248700002));
#271410=CARTESIAN_POINT('Ctrl Pts',(-9.96647366400006,11.6,-3.24875248700002));
#271411=CARTESIAN_POINT('Ctrl Pts',(-9.96792283000006,15.2,-3.24951184700002));
#271412=CARTESIAN_POINT('Ctrl Pts',(-9.96792283000006,11.6,-3.24951184700002));
#271413=CARTESIAN_POINT('Ctrl Pts',(-9.96937818100006,15.2,-3.25027618300001));
#271414=CARTESIAN_POINT('Ctrl Pts',(-9.96937818100006,11.6,-3.25027618300001));
#271415=CARTESIAN_POINT('Ctrl Pts',(-9.97083969300006,15.2,-3.25104549900002));
#271416=CARTESIAN_POINT('Ctrl Pts',(-9.97083969300006,11.6,-3.25104549900002));
#271417=CARTESIAN_POINT('Ctrl Pts',(-9.97230734500006,15.2,-3.25181979900002));
#271418=CARTESIAN_POINT('Ctrl Pts',(-9.97230734500006,11.6,-3.25181979900002));
#271419=CARTESIAN_POINT('Ctrl Pts',(-9.97378111500005,15.2,-3.25259908500001));
#271420=CARTESIAN_POINT('Ctrl Pts',(-9.97378111500005,11.6,-3.25259908500001));
#271421=CARTESIAN_POINT('Ctrl Pts',(-9.97526098000005,15.2,-3.25338336200002));
#271422=CARTESIAN_POINT('Ctrl Pts',(-9.97526098000005,11.6,-3.25338336200002));
#271423=CARTESIAN_POINT('Ctrl Pts',(-9.97674691800006,15.2,-3.25417263100002));
#271424=CARTESIAN_POINT('Ctrl Pts',(-9.97674691800006,11.6,-3.25417263100002));
#271425=CARTESIAN_POINT('Ctrl Pts',(-9.97823890700005,15.2,-3.25496689800001));
#271426=CARTESIAN_POINT('Ctrl Pts',(-9.97823890700005,11.6,-3.25496689800001));
#271427=CARTESIAN_POINT('Ctrl Pts',(-9.97973692500006,15.2,-3.25576616200001));
#271428=CARTESIAN_POINT('Ctrl Pts',(-9.97973692500006,11.6,-3.25576616200001));
#271429=CARTESIAN_POINT('Ctrl Pts',(-9.98124095000006,15.2,-3.25657043100001));
#271430=CARTESIAN_POINT('Ctrl Pts',(-9.98124095000006,11.6,-3.25657043100001));
#271431=CARTESIAN_POINT('Ctrl Pts',(-9.98275096100006,15.2,-3.25737970400001));
#271432=CARTESIAN_POINT('Ctrl Pts',(-9.98275096100006,11.6,-3.25737970400001));
#271433=CARTESIAN_POINT('Ctrl Pts',(-9.98426693400006,15.2,-3.25819398700002));
#271434=CARTESIAN_POINT('Ctrl Pts',(-9.98426693400006,11.6,-3.25819398700002));
#271435=CARTESIAN_POINT('Ctrl Pts',(-9.98578885000006,15.2,-3.25901328100001));
#271436=CARTESIAN_POINT('Ctrl Pts',(-9.98578885000006,11.6,-3.25901328100001));
#271437=CARTESIAN_POINT('Ctrl Pts',(-9.98731668700006,15.2,-3.25983759000001));
#271438=CARTESIAN_POINT('Ctrl Pts',(-9.98731668700006,11.6,-3.25983759000001));
#271439=CARTESIAN_POINT('Ctrl Pts',(-9.98885042200006,15.2,-3.26066691800001));
#271440=CARTESIAN_POINT('Ctrl Pts',(-9.98885042200006,11.6,-3.26066691800001));
#271441=CARTESIAN_POINT('Ctrl Pts',(-9.99039003500006,15.2,-3.26150126600002));
#271442=CARTESIAN_POINT('Ctrl Pts',(-9.99039003500006,11.6,-3.26150126600002));
#271443=CARTESIAN_POINT('Ctrl Pts',(-9.99193550400006,15.2,-3.26234063800001));
#271444=CARTESIAN_POINT('Ctrl Pts',(-9.99193550400006,11.6,-3.26234063800001));
#271445=CARTESIAN_POINT('Ctrl Pts',(-9.99348680900006,15.2,-3.26318503700001));
#271446=CARTESIAN_POINT('Ctrl Pts',(-9.99348680900006,11.6,-3.26318503700001));
#271447=CARTESIAN_POINT('Ctrl Pts',(-9.99504392600005,15.2,-3.26403446500001));
#271448=CARTESIAN_POINT('Ctrl Pts',(-9.99504392600005,11.6,-3.26403446500001));
#271449=CARTESIAN_POINT('Ctrl Pts',(-9.99660683700006,15.2,-3.26488892600001));
#271450=CARTESIAN_POINT('Ctrl Pts',(-9.99660683700006,11.6,-3.26488892600001));
#271451=CARTESIAN_POINT('Ctrl Pts',(-9.99817551900006,15.2,-3.26574842300001));
#271452=CARTESIAN_POINT('Ctrl Pts',(-9.99817551900006,11.6,-3.26574842300001));
#271453=CARTESIAN_POINT('Ctrl Pts',(-9.99974995100006,15.2,-3.26661295800001));
#271454=CARTESIAN_POINT('Ctrl Pts',(-9.99974995100006,11.6,-3.26661295800002));
#271455=CARTESIAN_POINT('Ctrl Pts',(-10.0013301140001,15.2,-3.26748253400002));
#271456=CARTESIAN_POINT('Ctrl Pts',(-10.0013301140001,11.6,-3.26748253400002));
#271457=CARTESIAN_POINT('Ctrl Pts',(-10.0029159850001,15.2,-3.26835715400001));
#271458=CARTESIAN_POINT('Ctrl Pts',(-10.0029159850001,11.6,-3.26835715400001));
#271459=CARTESIAN_POINT('Ctrl Pts',(-10.0045075450001,15.2,-3.26923682200002));
#271460=CARTESIAN_POINT('Ctrl Pts',(-10.0045075450001,11.6,-3.26923682200002));
#271461=CARTESIAN_POINT('Ctrl Pts',(-10.0061047720001,15.2,-3.27012153700001));
#271462=CARTESIAN_POINT('Ctrl Pts',(-10.0061047720001,11.6,-3.27012153700002));
#271463=CARTESIAN_POINT('Ctrl Pts',(-10.0077076460001,15.2,-3.27101130600001));
#271464=CARTESIAN_POINT('Ctrl Pts',(-10.0077076460001,11.6,-3.27101130600001));
#271465=CARTESIAN_POINT('Ctrl Pts',(-10.0093161470001,15.2,-3.27190613000001));
#271466=CARTESIAN_POINT('Ctrl Pts',(-10.0093161470001,11.6,-3.27190613000001));
#271467=CARTESIAN_POINT('Ctrl Pts',(-10.0109302540001,15.2,-3.27280601200002));
#271468=CARTESIAN_POINT('Ctrl Pts',(-10.0109302540001,11.6,-3.27280601200002));
#271469=CARTESIAN_POINT('Ctrl Pts',(-10.0125499470001,15.2,-3.27371095300002));
#271470=CARTESIAN_POINT('Ctrl Pts',(-10.0125499470001,11.6,-3.27371095300002));
#271471=CARTESIAN_POINT('Ctrl Pts',(-10.0141752040001,15.2,-3.27462095800001));
#271472=CARTESIAN_POINT('Ctrl Pts',(-10.0141752040001,11.6,-3.27462095800001));
#271473=CARTESIAN_POINT('Ctrl Pts',(-10.0158060070001,15.2,-3.27553602900001));
#271474=CARTESIAN_POINT('Ctrl Pts',(-10.0158060070001,11.6,-3.27553602900002));
#271475=CARTESIAN_POINT('Ctrl Pts',(-10.0174423360001,15.2,-3.27645616800002));
#271476=CARTESIAN_POINT('Ctrl Pts',(-10.0174423360001,11.6,-3.27645616800002));
#271477=CARTESIAN_POINT('Ctrl Pts',(-10.0190841680001,15.2,-3.27738137700001));
#271478=CARTESIAN_POINT('Ctrl Pts',(-10.0190841680001,11.6,-3.27738137700001));
#271479=CARTESIAN_POINT('Ctrl Pts',(-10.0207314860001,15.2,-3.27831166000002));
#271480=CARTESIAN_POINT('Ctrl Pts',(-10.0207314860001,11.6,-3.27831166000002));
#271481=CARTESIAN_POINT('Ctrl Pts',(-10.0223842680001,15.2,-3.27924701900002));
#271482=CARTESIAN_POINT('Ctrl Pts',(-10.0223842680001,11.6,-3.27924701900002));
#271483=CARTESIAN_POINT('Ctrl Pts',(-10.0240424950001,15.2,-3.28018745500001));
#271484=CARTESIAN_POINT('Ctrl Pts',(-10.0240424950001,11.6,-3.28018745500001));
#271485=CARTESIAN_POINT('Ctrl Pts',(-10.0257061490001,15.2,-3.28113297400002));
#271486=CARTESIAN_POINT('Ctrl Pts',(-10.0257061490001,11.6,-3.28113297400002));
#271487=CARTESIAN_POINT('Ctrl Pts',(-10.0273752060001,15.2,-3.28208357600001));
#271488=CARTESIAN_POINT('Ctrl Pts',(-10.0273752060001,11.6,-3.28208357600001));
#271489=CARTESIAN_POINT('Ctrl Pts',(-10.0290496500001,15.2,-3.28303926300002));
#271490=CARTESIAN_POINT('Ctrl Pts',(-10.0290496500001,11.6,-3.28303926300002));
#271491=CARTESIAN_POINT('Ctrl Pts',(-10.0307294600001,15.2,-3.28400003900001));
#271492=CARTESIAN_POINT('Ctrl Pts',(-10.0307294600001,11.6,-3.28400003900002));
#271493=CARTESIAN_POINT('Ctrl Pts',(-10.0324146170001,15.2,-3.28496590500002));
#271494=CARTESIAN_POINT('Ctrl Pts',(-10.0324146170001,11.6,-3.28496590500002));
#271495=CARTESIAN_POINT('Ctrl Pts',(-10.0341051000001,15.2,-3.28593686500001));
#271496=CARTESIAN_POINT('Ctrl Pts',(-10.0341051000001,11.6,-3.28593686500001));
#271497=CARTESIAN_POINT('Ctrl Pts',(-10.0358008910001,15.2,-3.28691292000002));
#271498=CARTESIAN_POINT('Ctrl Pts',(-10.0358008910001,11.6,-3.28691292000002));
#271499=CARTESIAN_POINT('Ctrl Pts',(-10.0375019710001,15.2,-3.28789407300001));
#271500=CARTESIAN_POINT('Ctrl Pts',(-10.0375019710001,11.6,-3.28789407300001));
#271501=CARTESIAN_POINT('Ctrl Pts',(-10.0392083190001,15.2,-3.28888032700001));
#271502=CARTESIAN_POINT('Ctrl Pts',(-10.0392083190001,11.6,-3.28888032700001));
#271503=CARTESIAN_POINT('Ctrl Pts',(-10.0409199180001,15.2,-3.28987168200001));
#271504=CARTESIAN_POINT('Ctrl Pts',(-10.0409199180001,11.6,-3.28987168200001));
#271505=CARTESIAN_POINT('Ctrl Pts',(-10.0426367470001,15.2,-3.29086814300001));
#271506=CARTESIAN_POINT('Ctrl Pts',(-10.0426367470001,11.6,-3.29086814300001));
#271507=CARTESIAN_POINT('Ctrl Pts',(-10.0443587870001,15.2,-3.29186971100001));
#271508=CARTESIAN_POINT('Ctrl Pts',(-10.0443587870001,11.6,-3.29186971100001));
#271509=CARTESIAN_POINT('Ctrl Pts',(-10.0460860200001,15.2,-3.29287638800002));
#271510=CARTESIAN_POINT('Ctrl Pts',(-10.0460860200001,11.6,-3.29287638800002));
#271511=CARTESIAN_POINT('Ctrl Pts',(-10.0478184260001,15.2,-3.29388817600002));
#271512=CARTESIAN_POINT('Ctrl Pts',(-10.0478184260001,11.6,-3.29388817600002));
#271513=CARTESIAN_POINT('Ctrl Pts',(-10.0495559880001,15.2,-3.29490507900001));
#271514=CARTESIAN_POINT('Ctrl Pts',(-10.0495559880001,11.6,-3.29490507900001));
#271515=CARTESIAN_POINT('Ctrl Pts',(-10.0512986840001,15.2,-3.29592709700002));
#271516=CARTESIAN_POINT('Ctrl Pts',(-10.0512986840001,11.6,-3.29592709700002));
#271517=CARTESIAN_POINT('Ctrl Pts',(-10.0530464980001,15.2,-3.29695423400001));
#271518=CARTESIAN_POINT('Ctrl Pts',(-10.0530464980001,11.6,-3.29695423400001));
#271519=CARTESIAN_POINT('Ctrl Pts',(-10.0547994090001,15.2,-3.29798649200002));
#271520=CARTESIAN_POINT('Ctrl Pts',(-10.0547994090001,11.6,-3.29798649200002));
#271521=CARTESIAN_POINT('Ctrl Pts',(-10.0565574010001,15.2,-3.29902387100002));
#271522=CARTESIAN_POINT('Ctrl Pts',(-10.0565574010001,11.6,-3.29902387100002));
#271523=CARTESIAN_POINT('Ctrl Pts',(-10.0583204520001,15.2,-3.30006637500002));
#271524=CARTESIAN_POINT('Ctrl Pts',(-10.0583204520001,11.6,-3.30006637500002));
#271525=CARTESIAN_POINT('Ctrl Pts',(-10.0600885460001,15.2,-3.30111400600002));
#271526=CARTESIAN_POINT('Ctrl Pts',(-10.0600885460001,11.6,-3.30111400600002));
#271527=CARTESIAN_POINT('Ctrl Pts',(-10.0618616650001,15.2,-3.30216676600001));
#271528=CARTESIAN_POINT('Ctrl Pts',(-10.0618616650001,11.6,-3.30216676600001));
#271529=CARTESIAN_POINT('Ctrl Pts',(-10.0636397890001,15.2,-3.30322465600001));
#271530=CARTESIAN_POINT('Ctrl Pts',(-10.0636397890001,11.6,-3.30322465600001));
#271531=CARTESIAN_POINT('Ctrl Pts',(-10.0654229000001,15.2,-3.30428768000001));
#271532=CARTESIAN_POINT('Ctrl Pts',(-10.0654229000001,11.6,-3.30428768000001));
#271533=CARTESIAN_POINT('Ctrl Pts',(-10.0672109790001,15.2,-3.30535583800001));
#271534=CARTESIAN_POINT('Ctrl Pts',(-10.0672109790001,11.6,-3.30535583800002));
#271535=CARTESIAN_POINT('Ctrl Pts',(-10.0690040090001,15.2,-3.30642913300002));
#271536=CARTESIAN_POINT('Ctrl Pts',(-10.0690040090001,11.6,-3.30642913300002));
#271537=CARTESIAN_POINT('Ctrl Pts',(-10.0708019710001,15.2,-3.30750756800001));
#271538=CARTESIAN_POINT('Ctrl Pts',(-10.0708019710001,11.6,-3.30750756800001));
#271539=CARTESIAN_POINT('Ctrl Pts',(-10.0726048470001,15.2,-3.30859114400001));
#271540=CARTESIAN_POINT('Ctrl Pts',(-10.0726048470001,11.6,-3.30859114400001));
#271541=CARTESIAN_POINT('Ctrl Pts',(-10.0744126190001,15.2,-3.30967986200001));
#271542=CARTESIAN_POINT('Ctrl Pts',(-10.0744126190001,11.6,-3.30967986200001));
#271543=CARTESIAN_POINT('Ctrl Pts',(-10.0762252700001,15.2,-3.31077372500001));
#271544=CARTESIAN_POINT('Ctrl Pts',(-10.0762252700001,11.6,-3.31077372500001));
#271545=CARTESIAN_POINT('Ctrl Pts',(-10.0780427800001,15.2,-3.31187273500001));
#271546=CARTESIAN_POINT('Ctrl Pts',(-10.0780427800001,11.6,-3.31187273500001));
#271547=CARTESIAN_POINT('Ctrl Pts',(-10.0798651330001,15.2,-3.31297689300001));
#271548=CARTESIAN_POINT('Ctrl Pts',(-10.0798651330001,11.6,-3.31297689300001));
#271549=CARTESIAN_POINT('Ctrl Pts',(-10.0816923090001,15.2,-3.31408620300001));
#271550=CARTESIAN_POINT('Ctrl Pts',(-10.0816923090001,11.6,-3.31408620300001));
#271551=CARTESIAN_POINT('Ctrl Pts',(-10.0835242930001,15.2,-3.31520066400001));
#271552=CARTESIAN_POINT('Ctrl Pts',(-10.0835242930001,11.6,-3.31520066400001));
#271553=CARTESIAN_POINT('Ctrl Pts',(-10.0853610650001,15.2,-3.31632027900001));
#271554=CARTESIAN_POINT('Ctrl Pts',(-10.0853610650001,11.6,-3.31632027900001));
#271555=CARTESIAN_POINT('Ctrl Pts',(-10.0872026080001,15.2,-3.31744505100001));
#271556=CARTESIAN_POINT('Ctrl Pts',(-10.0872026080001,11.6,-3.31744505100001));
#271557=CARTESIAN_POINT('Ctrl Pts',(-10.0890489030001,15.2,-3.31857498100002));
#271558=CARTESIAN_POINT('Ctrl Pts',(-10.0890489030001,11.6,-3.31857498100002));
#271559=CARTESIAN_POINT('Ctrl Pts',(-10.0908999360001,15.2,-3.31971007100002));
#271560=CARTESIAN_POINT('Ctrl Pts',(-10.0908999360001,11.6,-3.31971007100002));
#271561=CARTESIAN_POINT('Ctrl Pts',(-10.0927556870001,15.2,-3.32085032200002));
#271562=CARTESIAN_POINT('Ctrl Pts',(-10.0927556870001,11.6,-3.32085032200002));
#271563=CARTESIAN_POINT('Ctrl Pts',(-10.0946161380001,15.2,-3.32199573500001));
#271564=CARTESIAN_POINT('Ctrl Pts',(-10.0946161380001,11.6,-3.32199573500001));
#271565=CARTESIAN_POINT('Ctrl Pts',(-10.0964812720001,15.2,-3.32314631500001));
#271566=CARTESIAN_POINT('Ctrl Pts',(-10.0964812720001,11.6,-3.32314631500001));
#271567=CARTESIAN_POINT('Ctrl Pts',(-10.0983510720001,15.2,-3.32430206100002));
#271568=CARTESIAN_POINT('Ctrl Pts',(-10.0983510720001,11.6,-3.32430206100002));
#271569=CARTESIAN_POINT('Ctrl Pts',(-10.1002255210001,15.2,-3.32546297600001));
#271570=CARTESIAN_POINT('Ctrl Pts',(-10.1002255210001,11.6,-3.32546297600001));
#271571=CARTESIAN_POINT('Ctrl Pts',(-10.1021046020001,15.2,-3.32662906000001));
#271572=CARTESIAN_POINT('Ctrl Pts',(-10.1021046020001,11.6,-3.32662906000001));
#271573=CARTESIAN_POINT('Ctrl Pts',(-10.1039882970001,15.2,-3.32780031700001));
#271574=CARTESIAN_POINT('Ctrl Pts',(-10.1039882970001,11.6,-3.32780031700001));
#271575=CARTESIAN_POINT('Ctrl Pts',(-10.1058765880001,15.2,-3.32897674700002));
#271576=CARTESIAN_POINT('Ctrl Pts',(-10.1058765880001,11.6,-3.32897674700002));
#271577=CARTESIAN_POINT('Ctrl Pts',(-10.1077694590001,15.2,-3.33015835100001));
#271578=CARTESIAN_POINT('Ctrl Pts',(-10.1077694590001,11.6,-3.33015835100001));
#271579=CARTESIAN_POINT('Ctrl Pts',(-10.1096668940001,15.2,-3.33134513300001));
#271580=CARTESIAN_POINT('Ctrl Pts',(-10.1096668940001,11.6,-3.33134513300001));
#271581=CARTESIAN_POINT('Ctrl Pts',(-10.1115688740001,15.2,-3.33253709300001));
#271582=CARTESIAN_POINT('Ctrl Pts',(-10.1115688740001,11.6,-3.33253709300001));
#271583=CARTESIAN_POINT('Ctrl Pts',(-10.1134753840001,15.2,-3.33373423300001));
#271584=CARTESIAN_POINT('Ctrl Pts',(-10.1134753840001,11.6,-3.33373423300001));
#271585=CARTESIAN_POINT('Ctrl Pts',(-10.1153864040001,15.2,-3.33493655500002));
#271586=CARTESIAN_POINT('Ctrl Pts',(-10.1153864040001,11.6,-3.33493655500002));
#271587=CARTESIAN_POINT('Ctrl Pts',(-10.1173019210001,15.2,-3.33614406000001));
#271588=CARTESIAN_POINT('Ctrl Pts',(-10.1173019210001,11.6,-3.33614406000002));
#271589=CARTESIAN_POINT('Ctrl Pts',(-10.1192219160001,15.2,-3.33735675000002));
#271590=CARTESIAN_POINT('Ctrl Pts',(-10.1192219160001,11.6,-3.33735675000002));
#271591=CARTESIAN_POINT('Ctrl Pts',(-10.1211463720001,15.2,-3.33857462500001));
#271592=CARTESIAN_POINT('Ctrl Pts',(-10.1211463720001,11.6,-3.33857462500002));
#271593=CARTESIAN_POINT('Ctrl Pts',(-10.1230752720001,15.2,-3.33979768900001));
#271594=CARTESIAN_POINT('Ctrl Pts',(-10.1230752720001,11.6,-3.33979768900001));
#271595=CARTESIAN_POINT('Ctrl Pts',(-10.1250086010001,15.2,-3.34102594200001));
#271596=CARTESIAN_POINT('Ctrl Pts',(-10.1250086010001,11.6,-3.34102594200001));
#271597=CARTESIAN_POINT('Ctrl Pts',(-10.1269463420001,15.2,-3.34225938500001));
#271598=CARTESIAN_POINT('Ctrl Pts',(-10.1269463420001,11.6,-3.34225938500001));
#271599=CARTESIAN_POINT('Ctrl Pts',(-10.1288884770001,15.2,-3.34349802000002));
#271600=CARTESIAN_POINT('Ctrl Pts',(-10.1288884770001,11.6,-3.34349802000002));
#271601=CARTESIAN_POINT('Ctrl Pts',(-10.1308349920001,15.2,-3.34474185000001));
#271602=CARTESIAN_POINT('Ctrl Pts',(-10.1308349920001,11.6,-3.34474185000001));
#271603=CARTESIAN_POINT('Ctrl Pts',(-10.1327858680001,15.2,-3.34599087400001));
#271604=CARTESIAN_POINT('Ctrl Pts',(-10.1327858680001,11.6,-3.34599087400001));
#271605=CARTESIAN_POINT('Ctrl Pts',(-10.1347410890001,15.2,-3.34724509500001));
#271606=CARTESIAN_POINT('Ctrl Pts',(-10.1347410890001,11.6,-3.34724509500001));
#271607=CARTESIAN_POINT('Ctrl Pts',(-10.1367006410001,15.2,-3.34850451400001));
#271608=CARTESIAN_POINT('Ctrl Pts',(-10.1367006410001,11.6,-3.34850451400001));
#271609=CARTESIAN_POINT('Ctrl Pts',(-10.1386645040001,15.2,-3.34976913200002));
#271610=CARTESIAN_POINT('Ctrl Pts',(-10.1386645040001,11.6,-3.34976913200002));
#271611=CARTESIAN_POINT('Ctrl Pts',(-10.1406326650001,15.2,-3.35103895100001));
#271612=CARTESIAN_POINT('Ctrl Pts',(-10.1406326650001,11.6,-3.35103895100001));
#271613=CARTESIAN_POINT('Ctrl Pts',(-10.1426051060001,15.2,-3.35231397200001));
#271614=CARTESIAN_POINT('Ctrl Pts',(-10.1426051060001,11.6,-3.35231397200001));
#271615=CARTESIAN_POINT('Ctrl Pts',(-10.1445818110001,15.2,-3.35359419500001));
#271616=CARTESIAN_POINT('Ctrl Pts',(-10.1445818110001,11.6,-3.35359419500001));
#271617=CARTESIAN_POINT('Ctrl Pts',(-10.1465627640001,15.2,-3.35487962500002));
#271618=CARTESIAN_POINT('Ctrl Pts',(-10.1465627640001,11.6,-3.35487962500002));
#271619=CARTESIAN_POINT('Ctrl Pts',(-10.1485479490001,15.2,-3.35617026000001));
#271620=CARTESIAN_POINT('Ctrl Pts',(-10.1485479490001,11.6,-3.35617026000001));
#271621=CARTESIAN_POINT('Ctrl Pts',(-10.1505373510001,15.2,-3.35746610300002));
#271622=CARTESIAN_POINT('Ctrl Pts',(-10.1505373510001,11.6,-3.35746610300002));
#271623=CARTESIAN_POINT('Ctrl Pts',(-10.1525309520001,15.2,-3.35876715300001));
#271624=CARTESIAN_POINT('Ctrl Pts',(-10.1525309520001,11.6,-3.35876715300001));
#271625=CARTESIAN_POINT('Ctrl Pts',(-10.1545287380001,15.2,-3.36007341400002));
#271626=CARTESIAN_POINT('Ctrl Pts',(-10.1545287380001,11.6,-3.36007341400002));
#271627=CARTESIAN_POINT('Ctrl Pts',(-10.1565306900001,15.2,-3.36138488700001));
#271628=CARTESIAN_POINT('Ctrl Pts',(-10.1565306900001,11.6,-3.36138488700001));
#271629=CARTESIAN_POINT('Ctrl Pts',(-10.1585367960001,15.2,-3.36270157200001));
#271630=CARTESIAN_POINT('Ctrl Pts',(-10.1585367960001,11.6,-3.36270157200001));
#271631=CARTESIAN_POINT('Ctrl Pts',(-10.1605470380001,15.2,-3.36402347000002));
#271632=CARTESIAN_POINT('Ctrl Pts',(-10.1605470380001,11.6,-3.36402347000002));
#271633=CARTESIAN_POINT('Ctrl Pts',(-10.1625614000001,15.2,-3.36535058300001));
#271634=CARTESIAN_POINT('Ctrl Pts',(-10.1625614000001,11.6,-3.36535058300001));
#271635=CARTESIAN_POINT('Ctrl Pts',(-10.1645798690001,15.2,-3.36668291200001));
#271636=CARTESIAN_POINT('Ctrl Pts',(-10.1645798690001,11.6,-3.36668291200001));
#271637=CARTESIAN_POINT('Ctrl Pts',(-10.1666024250001,15.2,-3.36802045800002));
#271638=CARTESIAN_POINT('Ctrl Pts',(-10.1666024250001,11.6,-3.36802045800002));
#271639=CARTESIAN_POINT('Ctrl Pts',(-10.1686290550001,15.2,-3.36936322300001));
#271640=CARTESIAN_POINT('Ctrl Pts',(-10.1686290550001,11.6,-3.36936322300002));
#271641=CARTESIAN_POINT('Ctrl Pts',(-10.1706597440001,15.2,-3.37071120800001));
#271642=CARTESIAN_POINT('Ctrl Pts',(-10.1706597440001,11.6,-3.37071120800002));
#271643=CARTESIAN_POINT('Ctrl Pts',(-10.1726944750001,15.2,-3.37206441300001));
#271644=CARTESIAN_POINT('Ctrl Pts',(-10.1726944750001,11.6,-3.37206441300001));
#271645=CARTESIAN_POINT('Ctrl Pts',(-10.1747332320001,15.2,-3.37342284000002));
#271646=CARTESIAN_POINT('Ctrl Pts',(-10.1747332320001,11.6,-3.37342284000002));
#271647=CARTESIAN_POINT('Ctrl Pts',(-10.1767760010001,15.2,-3.37478649100001));
#271648=CARTESIAN_POINT('Ctrl Pts',(-10.1767760010001,11.6,-3.37478649100001));
#271649=CARTESIAN_POINT('Ctrl Pts',(-10.1788227660001,15.2,-3.37615536500001));
#271650=CARTESIAN_POINT('Ctrl Pts',(-10.1788227660001,11.6,-3.37615536500001));
#271651=CARTESIAN_POINT('Ctrl Pts',(-10.1808735120001,15.2,-3.37752946400002));
#271652=CARTESIAN_POINT('Ctrl Pts',(-10.1808735120001,11.6,-3.37752946400002));
#271653=CARTESIAN_POINT('Ctrl Pts',(-10.1829282230001,15.2,-3.37890879000001));
#271654=CARTESIAN_POINT('Ctrl Pts',(-10.1829282230001,11.6,-3.37890879000002));
#271655=CARTESIAN_POINT('Ctrl Pts',(-10.1849868840001,15.2,-3.38029334300002));
#271656=CARTESIAN_POINT('Ctrl Pts',(-10.1849868840001,11.6,-3.38029334300002));
#271657=CARTESIAN_POINT('Ctrl Pts',(-10.1870494800001,15.2,-3.38168312400001));
#271658=CARTESIAN_POINT('Ctrl Pts',(-10.1870494800001,11.6,-3.38168312400001));
#271659=CARTESIAN_POINT('Ctrl Pts',(-10.1891159950001,15.2,-3.38307813400001));
#271660=CARTESIAN_POINT('Ctrl Pts',(-10.1891159950001,11.6,-3.38307813400002));
#271661=CARTESIAN_POINT('Ctrl Pts',(-10.1911864150001,15.2,-3.38447837600001));
#271662=CARTESIAN_POINT('Ctrl Pts',(-10.1911864150001,11.6,-3.38447837600001));
#271663=CARTESIAN_POINT('Ctrl Pts',(-10.1932607240001,15.2,-3.38588384800001));
#271664=CARTESIAN_POINT('Ctrl Pts',(-10.1932607240001,11.6,-3.38588384800001));
#271665=CARTESIAN_POINT('Ctrl Pts',(-10.1953389060001,15.2,-3.38729455300002));
#271666=CARTESIAN_POINT('Ctrl Pts',(-10.1953389060001,11.6,-3.38729455300002));
#271667=CARTESIAN_POINT('Ctrl Pts',(-10.1974209480001,15.2,-3.38871049100002));
#271668=CARTESIAN_POINT('Ctrl Pts',(-10.1974209480001,11.6,-3.38871049100002));
#271669=CARTESIAN_POINT('Ctrl Pts',(-10.1995068350001,15.2,-3.39013166400001));
#271670=CARTESIAN_POINT('Ctrl Pts',(-10.1995068350001,11.6,-3.39013166400001));
#271671=CARTESIAN_POINT('Ctrl Pts',(-10.2015965500001,15.2,-3.39155807200001));
#271672=CARTESIAN_POINT('Ctrl Pts',(-10.2015965500001,11.6,-3.39155807200001));
#271673=CARTESIAN_POINT('Ctrl Pts',(-10.2036900790001,15.2,-3.39298971600002));
#271674=CARTESIAN_POINT('Ctrl Pts',(-10.2036900790001,11.6,-3.39298971600002));
#271675=CARTESIAN_POINT('Ctrl Pts',(-10.2057874080001,15.2,-3.39442659900001));
#271676=CARTESIAN_POINT('Ctrl Pts',(-10.2057874080001,11.6,-3.39442659900001));
#271677=CARTESIAN_POINT('Ctrl Pts',(-10.2078885200001,15.2,-3.39586871800002));
#271678=CARTESIAN_POINT('Ctrl Pts',(-10.2078885200001,11.6,-3.39586871800002));
#271679=CARTESIAN_POINT('Ctrl Pts',(-10.2099934030001,15.2,-3.39731607600001));
#271680=CARTESIAN_POINT('Ctrl Pts',(-10.2099934030001,11.6,-3.39731607600001));
#271681=CARTESIAN_POINT('Ctrl Pts',(-10.2121020400001,15.2,-3.39876867400001));
#271682=CARTESIAN_POINT('Ctrl Pts',(-10.2121020400001,11.6,-3.39876867400001));
#271683=CARTESIAN_POINT('Ctrl Pts',(-10.2142144180001,15.2,-3.40022651400002));
#271684=CARTESIAN_POINT('Ctrl Pts',(-10.2142144180001,11.6,-3.40022651400002));
#271685=CARTESIAN_POINT('Ctrl Pts',(-10.2163305200001,15.2,-3.40168959500001));
#271686=CARTESIAN_POINT('Ctrl Pts',(-10.2163305200001,11.6,-3.40168959500002));
#271687=CARTESIAN_POINT('Ctrl Pts',(-10.2184503330001,15.2,-3.40315791800001));
#271688=CARTESIAN_POINT('Ctrl Pts',(-10.2184503330001,11.6,-3.40315791800002));
#271689=CARTESIAN_POINT('Ctrl Pts',(-10.2205738430001,15.2,-3.40463148500001));
#271690=CARTESIAN_POINT('Ctrl Pts',(-10.2205738430001,11.6,-3.40463148500001));
#271691=CARTESIAN_POINT('Ctrl Pts',(-10.2227010340001,15.2,-3.40611029600002));
#271692=CARTESIAN_POINT('Ctrl Pts',(-10.2227010340001,11.6,-3.40611029600002));
#271693=CARTESIAN_POINT('Ctrl Pts',(-10.2248318930001,15.2,-3.40759435200002));
#271694=CARTESIAN_POINT('Ctrl Pts',(-10.2248318930001,11.6,-3.40759435200002));
#271695=CARTESIAN_POINT('Ctrl Pts',(-10.2269664030001,15.2,-3.40908365300002));
#271696=CARTESIAN_POINT('Ctrl Pts',(-10.2269664030001,11.6,-3.40908365300002));
#271697=CARTESIAN_POINT('Ctrl Pts',(-10.2291045510001,15.2,-3.41057820100001));
#271698=CARTESIAN_POINT('Ctrl Pts',(-10.2291045510001,11.6,-3.41057820100001));
#271699=CARTESIAN_POINT('Ctrl Pts',(-10.2312463240001,15.2,-3.41207799600001));
#271700=CARTESIAN_POINT('Ctrl Pts',(-10.2312463240001,11.6,-3.41207799600001));
#271701=CARTESIAN_POINT('Ctrl Pts',(-10.2333917050001,15.2,-3.41358304000002));
#271702=CARTESIAN_POINT('Ctrl Pts',(-10.2333917050001,11.6,-3.41358304000002));
#271703=CARTESIAN_POINT('Ctrl Pts',(-10.2355406810001,15.2,-3.41509333200001));
#271704=CARTESIAN_POINT('Ctrl Pts',(-10.2355406810001,11.6,-3.41509333200001));
#271705=CARTESIAN_POINT('Ctrl Pts',(-10.2376932380001,15.2,-3.41660887400002));
#271706=CARTESIAN_POINT('Ctrl Pts',(-10.2376932380001,11.6,-3.41660887400002));
#271707=CARTESIAN_POINT('Ctrl Pts',(-10.2398493600001,15.2,-3.41812966500001));
#271708=CARTESIAN_POINT('Ctrl Pts',(-10.2398493600001,11.6,-3.41812966500001));
#271709=CARTESIAN_POINT('Ctrl Pts',(-10.2420090360001,15.2,-3.41965571000001));
#271710=CARTESIAN_POINT('Ctrl Pts',(-10.2420090360001,11.6,-3.41965571000001));
#271711=CARTESIAN_POINT('Ctrl Pts',(-10.2441722480001,15.2,-3.42118700400002));
#271712=CARTESIAN_POINT('Ctrl Pts',(-10.2441722480001,11.6,-3.42118700400002));
#271713=CARTESIAN_POINT('Ctrl Pts',(-10.2463389840001,15.2,-3.42272355100001));
#271714=CARTESIAN_POINT('Ctrl Pts',(-10.2463389840001,11.6,-3.42272355100001));
#271715=CARTESIAN_POINT('Ctrl Pts',(-10.2485092300001,15.2,-3.42426535100001));
#271716=CARTESIAN_POINT('Ctrl Pts',(-10.2485092300001,11.6,-3.42426535100001));
#271717=CARTESIAN_POINT('Ctrl Pts',(-10.2506829710001,15.2,-3.42581240500001));
#271718=CARTESIAN_POINT('Ctrl Pts',(-10.2506829710001,11.6,-3.42581240500001));
#271719=CARTESIAN_POINT('Ctrl Pts',(-10.2528601940001,15.2,-3.42736471300002));
#271720=CARTESIAN_POINT('Ctrl Pts',(-10.2528601940001,11.6,-3.42736471300002));
#271721=CARTESIAN_POINT('Ctrl Pts',(-10.2550408840001,15.2,-3.42892227700001));
#271722=CARTESIAN_POINT('Ctrl Pts',(-10.2550408840001,11.6,-3.42892227700002));
#271723=CARTESIAN_POINT('Ctrl Pts',(-10.2572250270001,15.2,-3.43048509600001));
#271724=CARTESIAN_POINT('Ctrl Pts',(-10.2572250270001,11.6,-3.43048509600001));
#271725=CARTESIAN_POINT('Ctrl Pts',(-10.2594126090001,15.2,-3.43205317100002));
#271726=CARTESIAN_POINT('Ctrl Pts',(-10.2594126090001,11.6,-3.43205317100002));
#271727=CARTESIAN_POINT('Ctrl Pts',(-10.2616036170001,15.2,-3.43362650300001));
#271728=CARTESIAN_POINT('Ctrl Pts',(-10.2616036170001,11.6,-3.43362650300001));
#271729=CARTESIAN_POINT('Ctrl Pts',(-10.2637980370001,15.2,-3.43520509300001));
#271730=CARTESIAN_POINT('Ctrl Pts',(-10.2637980370001,11.6,-3.43520509300001));
#271731=CARTESIAN_POINT('Ctrl Pts',(-10.2659958540001,15.2,-3.43678894100002));
#271732=CARTESIAN_POINT('Ctrl Pts',(-10.2659958540001,11.6,-3.43678894100002));
#271733=CARTESIAN_POINT('Ctrl Pts',(-10.2681970550001,15.2,-3.43837804700001));
#271734=CARTESIAN_POINT('Ctrl Pts',(-10.2681970550001,11.6,-3.43837804700002));
#271735=CARTESIAN_POINT('Ctrl Pts',(-10.2704016260001,15.2,-3.43997241200002));
#271736=CARTESIAN_POINT('Ctrl Pts',(-10.2704016260001,11.6,-3.43997241200002));
#271737=CARTESIAN_POINT('Ctrl Pts',(-10.2726095530001,15.2,-3.44157203700002));
#271738=CARTESIAN_POINT('Ctrl Pts',(-10.2726095530001,11.6,-3.44157203700002));
#271739=CARTESIAN_POINT('Ctrl Pts',(-10.2748208240001,15.2,-3.44317692300002));
#271740=CARTESIAN_POINT('Ctrl Pts',(-10.2748208240001,11.6,-3.44317692300002));
#271741=CARTESIAN_POINT('Ctrl Pts',(-10.2770354230001,15.2,-3.44478706900002));
#271742=CARTESIAN_POINT('Ctrl Pts',(-10.2770354230001,11.6,-3.44478706900002));
#271743=CARTESIAN_POINT('Ctrl Pts',(-10.2792533370001,15.2,-3.44640247600001));
#271744=CARTESIAN_POINT('Ctrl Pts',(-10.2792533370001,11.6,-3.44640247600001));
#271745=CARTESIAN_POINT('Ctrl Pts',(-10.2814745530001,15.2,-3.44802314500001));
#271746=CARTESIAN_POINT('Ctrl Pts',(-10.2814745530001,11.6,-3.44802314500001));
#271747=CARTESIAN_POINT('Ctrl Pts',(-10.2836990580001,15.2,-3.44964907700001));
#271748=CARTESIAN_POINT('Ctrl Pts',(-10.2836990580001,11.6,-3.44964907700001));
#271749=CARTESIAN_POINT('Ctrl Pts',(-10.2859268370001,15.2,-3.45128027200001));
#271750=CARTESIAN_POINT('Ctrl Pts',(-10.2859268370001,11.6,-3.45128027200001));
#271751=CARTESIAN_POINT('Ctrl Pts',(-10.2881578770001,15.2,-3.45291672900002));
#271752=CARTESIAN_POINT('Ctrl Pts',(-10.2881578770001,11.6,-3.45291672900002));
#271753=CARTESIAN_POINT('Ctrl Pts',(-10.2903921640001,15.2,-3.45455845000001));
#271754=CARTESIAN_POINT('Ctrl Pts',(-10.2903921640001,11.6,-3.45455845000001));
#271755=CARTESIAN_POINT('Ctrl Pts',(-10.2926296860001,15.2,-3.45620543600001));
#271756=CARTESIAN_POINT('Ctrl Pts',(-10.2926296860001,11.6,-3.45620543600001));
#271757=CARTESIAN_POINT('Ctrl Pts',(-10.2948704290001,15.2,-3.45785768600001));
#271758=CARTESIAN_POINT('Ctrl Pts',(-10.2948704290001,11.6,-3.45785768600001));
#271759=CARTESIAN_POINT('Ctrl Pts',(-10.2971143780001,15.2,-3.45951520100002));
#271760=CARTESIAN_POINT('Ctrl Pts',(-10.2971143780001,11.6,-3.45951520100002));
#271761=CARTESIAN_POINT('Ctrl Pts',(-10.2993615220001,15.2,-3.46117798000002));
#271762=CARTESIAN_POINT('Ctrl Pts',(-10.2993615220001,11.6,-3.46117798000002));
#271763=CARTESIAN_POINT('Ctrl Pts',(-10.3016118470001,15.2,-3.46284602700001));
#271764=CARTESIAN_POINT('Ctrl Pts',(-10.3016118470001,11.6,-3.46284602700001));
#271765=CARTESIAN_POINT('Ctrl Pts',(-10.3038653390001,15.2,-3.46451933900001));
#271766=CARTESIAN_POINT('Ctrl Pts',(-10.3038653390001,11.6,-3.46451933900001));
#271767=CARTESIAN_POINT('Ctrl Pts',(-10.3061219850001,15.2,-3.46619791800002));
#271768=CARTESIAN_POINT('Ctrl Pts',(-10.3061219850001,11.6,-3.46619791800002));
#271769=CARTESIAN_POINT('Ctrl Pts',(-10.3083817730001,15.2,-3.46788176400001));
#271770=CARTESIAN_POINT('Ctrl Pts',(-10.3083817730001,11.6,-3.46788176400001));
#271771=CARTESIAN_POINT('Ctrl Pts',(-10.3106446870001,15.2,-3.46957087800002));
#271772=CARTESIAN_POINT('Ctrl Pts',(-10.3106446870001,11.6,-3.46957087800002));
#271773=CARTESIAN_POINT('Ctrl Pts',(-10.3129107160001,15.2,-3.47126525800002));
#271774=CARTESIAN_POINT('Ctrl Pts',(-10.3129107160001,11.6,-3.47126525800002));
#271775=CARTESIAN_POINT('Ctrl Pts',(-10.3151798480001,15.2,-3.47296490700002));
#271776=CARTESIAN_POINT('Ctrl Pts',(-10.3151798480001,11.6,-3.47296490700002));
#271777=CARTESIAN_POINT('Ctrl Pts',(-10.3174520670001,15.2,-3.47466982400002));
#271778=CARTESIAN_POINT('Ctrl Pts',(-10.3174520670001,11.6,-3.47466982400002));
#271779=CARTESIAN_POINT('Ctrl Pts',(-10.3197273620001,15.2,-3.47638001000002));
#271780=CARTESIAN_POINT('Ctrl Pts',(-10.3197273620001,11.6,-3.47638001000002));
#271781=CARTESIAN_POINT('Ctrl Pts',(-10.3220057200001,15.2,-3.47809546500002));
#271782=CARTESIAN_POINT('Ctrl Pts',(-10.3220057200001,11.6,-3.47809546500002));
#271783=CARTESIAN_POINT('Ctrl Pts',(-10.3242871260001,15.2,-3.47981618900001));
#271784=CARTESIAN_POINT('Ctrl Pts',(-10.3242871260001,11.6,-3.47981618900001));
#271785=CARTESIAN_POINT('Ctrl Pts',(-10.3265715690001,15.2,-3.48154218200001));
#271786=CARTESIAN_POINT('Ctrl Pts',(-10.3265715690001,11.6,-3.48154218200001));
#271787=CARTESIAN_POINT('Ctrl Pts',(-10.3288590360001,15.2,-3.48327344600001));
#271788=CARTESIAN_POINT('Ctrl Pts',(-10.3288590360001,11.6,-3.48327344600001));
#271789=CARTESIAN_POINT('Ctrl Pts',(-10.3311495120001,15.2,-3.48500997900001));
#271790=CARTESIAN_POINT('Ctrl Pts',(-10.3311495120001,11.6,-3.48500997900001));
#271791=CARTESIAN_POINT('Ctrl Pts',(-10.3334429860001,15.2,-3.48675178300001));
#271792=CARTESIAN_POINT('Ctrl Pts',(-10.3334429860001,11.6,-3.48675178300002));
#271793=CARTESIAN_POINT('Ctrl Pts',(-10.3357394460001,15.2,-3.48849885700002));
#271794=CARTESIAN_POINT('Ctrl Pts',(-10.3357394460001,11.6,-3.48849885700002));
#271795=CARTESIAN_POINT('Ctrl Pts',(-10.3380388780001,15.2,-3.49025120200002));
#271796=CARTESIAN_POINT('Ctrl Pts',(-10.3380388780001,11.6,-3.49025120200002));
#271797=CARTESIAN_POINT('Ctrl Pts',(-10.3403412680001,15.2,-3.49200881800002));
#271798=CARTESIAN_POINT('Ctrl Pts',(-10.3403412680001,11.6,-3.49200881800002));
#271799=CARTESIAN_POINT('Ctrl Pts',(-10.3426466050001,15.2,-3.49377170500001));
#271800=CARTESIAN_POINT('Ctrl Pts',(-10.3426466050001,11.6,-3.49377170500001));
#271801=CARTESIAN_POINT('Ctrl Pts',(-10.3449548750001,15.2,-3.49553986400001));
#271802=CARTESIAN_POINT('Ctrl Pts',(-10.3449548750001,11.6,-3.49553986400002));
#271803=CARTESIAN_POINT('Ctrl Pts',(-10.3472660680001,15.2,-3.49731329400001));
#271804=CARTESIAN_POINT('Ctrl Pts',(-10.3472660680001,11.6,-3.49731329400001));
#271805=CARTESIAN_POINT('Ctrl Pts',(-10.3495801680001,15.2,-3.49909199600001));
#271806=CARTESIAN_POINT('Ctrl Pts',(-10.3495801680001,11.6,-3.49909199600001));
#271807=CARTESIAN_POINT('Ctrl Pts',(-10.3518971640001,15.2,-3.50087597000002));
#271808=CARTESIAN_POINT('Ctrl Pts',(-10.3518971640001,11.6,-3.50087597000002));
#271809=CARTESIAN_POINT('Ctrl Pts',(-10.3542170430001,15.2,-3.50266521600001));
#271810=CARTESIAN_POINT('Ctrl Pts',(-10.3542170430001,11.6,-3.50266521600001));
#271811=CARTESIAN_POINT('Ctrl Pts',(-10.3565397920001,15.2,-3.50445973500001));
#271812=CARTESIAN_POINT('Ctrl Pts',(-10.3565397920001,11.6,-3.50445973500001));
#271813=CARTESIAN_POINT('Ctrl Pts',(-10.3588654000001,15.2,-3.50625952500002));
#271814=CARTESIAN_POINT('Ctrl Pts',(-10.3588654000001,11.6,-3.50625952500002));
#271815=CARTESIAN_POINT('Ctrl Pts',(-10.3611938520001,15.2,-3.50806458800001));
#271816=CARTESIAN_POINT('Ctrl Pts',(-10.3611938520001,11.6,-3.50806458800002));
#271817=CARTESIAN_POINT('Ctrl Pts',(-10.3635251390001,15.2,-3.50987492500002));
#271818=CARTESIAN_POINT('Ctrl Pts',(-10.3635251390001,11.6,-3.50987492500002));
#271819=CARTESIAN_POINT('Ctrl Pts',(-10.3658592460001,15.2,-3.51169053400001));
#271820=CARTESIAN_POINT('Ctrl Pts',(-10.3658592460001,11.6,-3.51169053400001));
#271821=CARTESIAN_POINT('Ctrl Pts',(-10.3681961610001,15.2,-3.51351141600002));
#271822=CARTESIAN_POINT('Ctrl Pts',(-10.3681961610001,11.6,-3.51351141600002));
#271823=CARTESIAN_POINT('Ctrl Pts',(-10.3705358710001,15.2,-3.51533757000002));
#271824=CARTESIAN_POINT('Ctrl Pts',(-10.3705358710001,11.6,-3.51533757000002));
#271825=CARTESIAN_POINT('Ctrl Pts',(-10.3728783650001,15.2,-3.51716899900001));
#271826=CARTESIAN_POINT('Ctrl Pts',(-10.3728783650001,11.6,-3.51716899900001));
#271827=CARTESIAN_POINT('Ctrl Pts',(-10.3752236290001,15.2,-3.51900569900002));
#271828=CARTESIAN_POINT('Ctrl Pts',(-10.3752236290001,11.6,-3.51900569900002));
#271829=CARTESIAN_POINT('Ctrl Pts',(-10.3775716530001,15.2,-3.52084767400001));
#271830=CARTESIAN_POINT('Ctrl Pts',(-10.3775716530001,11.6,-3.52084767400001));
#271831=CARTESIAN_POINT('Ctrl Pts',(-10.3799224230001,15.2,-3.52269492200001));
#271832=CARTESIAN_POINT('Ctrl Pts',(-10.3799224230001,11.6,-3.52269492200001));
#271833=CARTESIAN_POINT('Ctrl Pts',(-10.3822759270001,15.2,-3.52454744300001));
#271834=CARTESIAN_POINT('Ctrl Pts',(-10.3822759270001,11.6,-3.52454744300001));
#271835=CARTESIAN_POINT('Ctrl Pts',(-10.3846321520001,15.2,-3.52640523800002));
#271836=CARTESIAN_POINT('Ctrl Pts',(-10.3846321520001,11.6,-3.52640523800002));
#271837=CARTESIAN_POINT('Ctrl Pts',(-10.3869910880001,15.2,-3.52826830500002));
#271838=CARTESIAN_POINT('Ctrl Pts',(-10.3869910880001,11.6,-3.52826830500002));
#271839=CARTESIAN_POINT('Ctrl Pts',(-10.3893527210001,15.2,-3.53013664700002));
#271840=CARTESIAN_POINT('Ctrl Pts',(-10.3893527210001,11.6,-3.53013664700002));
#271841=CARTESIAN_POINT('Ctrl Pts',(-10.3917170390001,15.2,-3.53201026100002));
#271842=CARTESIAN_POINT('Ctrl Pts',(-10.3917170390001,11.6,-3.53201026100002));
#271843=CARTESIAN_POINT('Ctrl Pts',(-10.3940840300001,15.2,-3.53388914800002));
#271844=CARTESIAN_POINT('Ctrl Pts',(-10.3940840300001,11.6,-3.53388914800002));
#271845=CARTESIAN_POINT('Ctrl Pts',(-10.3964536830001,15.2,-3.53577331000002));
#271846=CARTESIAN_POINT('Ctrl Pts',(-10.3964536830001,11.6,-3.53577331000002));
#271847=CARTESIAN_POINT('Ctrl Pts',(-10.3988259850001,15.2,-3.53766274500002));
#271848=CARTESIAN_POINT('Ctrl Pts',(-10.3988259850001,11.6,-3.53766274500002));
#271849=CARTESIAN_POINT('Ctrl Pts',(-10.4012009230001,15.2,-3.53955745300001));
#271850=CARTESIAN_POINT('Ctrl Pts',(-10.4012009230001,11.6,-3.53955745300001));
#271851=CARTESIAN_POINT('Ctrl Pts',(-10.4035784870001,15.2,-3.54145743400001));
#271852=CARTESIAN_POINT('Ctrl Pts',(-10.4035784870001,11.6,-3.54145743400002));
#271853=CARTESIAN_POINT('Ctrl Pts',(-10.4059586630001,15.2,-3.54336268900001));
#271854=CARTESIAN_POINT('Ctrl Pts',(-10.4059586630001,11.6,-3.54336268900001));
#271855=CARTESIAN_POINT('Ctrl Pts',(-10.4083414410001,15.2,-3.54527321700001));
#271856=CARTESIAN_POINT('Ctrl Pts',(-10.4083414410001,11.6,-3.54527321700001));
#271857=CARTESIAN_POINT('Ctrl Pts',(-10.4107268080001,15.2,-3.54718901800001));
#271858=CARTESIAN_POINT('Ctrl Pts',(-10.4107268080001,11.6,-3.54718901800001));
#271859=CARTESIAN_POINT('Ctrl Pts',(-10.4131147520001,15.2,-3.54911009300002));
#271860=CARTESIAN_POINT('Ctrl Pts',(-10.4131147520001,11.6,-3.54911009300002));
#271861=CARTESIAN_POINT('Ctrl Pts',(-10.4155052600001,15.2,-3.55103644000001));
#271862=CARTESIAN_POINT('Ctrl Pts',(-10.4155052600001,11.6,-3.55103644000002));
#271863=CARTESIAN_POINT('Ctrl Pts',(-10.4178983230001,15.2,-3.55296805900001));
#271864=CARTESIAN_POINT('Ctrl Pts',(-10.4178983230001,11.6,-3.55296805900001));
#271865=CARTESIAN_POINT('Ctrl Pts',(-10.4202939270001,15.2,-3.55490495200002));
#271866=CARTESIAN_POINT('Ctrl Pts',(-10.4202939270001,11.6,-3.55490495200002));
#271867=CARTESIAN_POINT('Ctrl Pts',(-10.4226920610001,15.2,-3.55684711800001));
#271868=CARTESIAN_POINT('Ctrl Pts',(-10.4226920610001,11.6,-3.55684711800001));
#271869=CARTESIAN_POINT('Ctrl Pts',(-10.4250927130001,15.2,-3.55879455600002));
#271870=CARTESIAN_POINT('Ctrl Pts',(-10.4250927130001,11.6,-3.55879455600002));
#271871=CARTESIAN_POINT('Ctrl Pts',(-10.4274958710001,15.2,-3.56074726700002));
#271872=CARTESIAN_POINT('Ctrl Pts',(-10.4274958710001,11.6,-3.56074726700002));
#271873=CARTESIAN_POINT('Ctrl Pts',(-10.4299015240001,15.2,-3.56270525000001));
#271874=CARTESIAN_POINT('Ctrl Pts',(-10.4299015240001,11.6,-3.56270525000001));
#271875=CARTESIAN_POINT('Ctrl Pts',(-10.4323096600001,15.2,-3.56466850500002));
#271876=CARTESIAN_POINT('Ctrl Pts',(-10.4323096600001,11.6,-3.56466850500002));
#271877=CARTESIAN_POINT('Ctrl Pts',(-10.4347202660001,15.2,-3.56663703300002));
#271878=CARTESIAN_POINT('Ctrl Pts',(-10.4347202660001,11.6,-3.56663703300002));
#271879=CARTESIAN_POINT('Ctrl Pts',(-10.4371333320001,15.2,-3.56861083100001));
#271880=CARTESIAN_POINT('Ctrl Pts',(-10.4371333320001,11.6,-3.56861083100001));
#271881=CARTESIAN_POINT('Ctrl Pts',(-10.4395488460001,15.2,-3.57058990100001));
#271882=CARTESIAN_POINT('Ctrl Pts',(-10.4395488460001,11.6,-3.57058990100001));
#271883=CARTESIAN_POINT('Ctrl Pts',(-10.4419667960001,15.2,-3.57257424500002));
#271884=CARTESIAN_POINT('Ctrl Pts',(-10.4419667960001,11.6,-3.57257424500002));
#271885=CARTESIAN_POINT('Ctrl Pts',(-10.4443871710001,15.2,-3.57456385800001));
#271886=CARTESIAN_POINT('Ctrl Pts',(-10.4443871710001,11.6,-3.57456385800001));
#271887=CARTESIAN_POINT('Ctrl Pts',(-10.4468099580001,15.2,-3.57655874200002));
#271888=CARTESIAN_POINT('Ctrl Pts',(-10.4468099580001,11.6,-3.57655874200002));
#271889=CARTESIAN_POINT('Ctrl Pts',(-10.4492351490001,15.2,-3.57855889700001));
#271890=CARTESIAN_POINT('Ctrl Pts',(-10.4492351490001,11.6,-3.57855889700002));
#271891=CARTESIAN_POINT('Ctrl Pts',(-10.4516627280001,15.2,-3.58056432300002));
#271892=CARTESIAN_POINT('Ctrl Pts',(-10.4516627280001,11.6,-3.58056432300002));
#271893=CARTESIAN_POINT('Ctrl Pts',(-10.4540926860001,15.2,-3.58257502100002));
#271894=CARTESIAN_POINT('Ctrl Pts',(-10.4540926860001,11.6,-3.58257502100002));
#271895=CARTESIAN_POINT('Ctrl Pts',(-10.4565250110001,15.2,-3.58459098700001));
#271896=CARTESIAN_POINT('Ctrl Pts',(-10.4565250110001,11.6,-3.58459098700001));
#271897=CARTESIAN_POINT('Ctrl Pts',(-10.4589596920001,15.2,-3.58661222400002));
#271898=CARTESIAN_POINT('Ctrl Pts',(-10.4589596920001,11.6,-3.58661222400002));
#271899=CARTESIAN_POINT('Ctrl Pts',(-10.4613967180001,15.2,-3.58863873100002));
#271900=CARTESIAN_POINT('Ctrl Pts',(-10.4613967180001,11.6,-3.58863873100002));
#271901=CARTESIAN_POINT('Ctrl Pts',(-10.4638360760001,15.2,-3.59067050700002));
#271902=CARTESIAN_POINT('Ctrl Pts',(-10.4638360760001,11.6,-3.59067050700002));
#271903=CARTESIAN_POINT('Ctrl Pts',(-10.4662777560001,15.2,-3.59270755200002));
#271904=CARTESIAN_POINT('Ctrl Pts',(-10.4662777560001,11.6,-3.59270755200002));
#271905=CARTESIAN_POINT('Ctrl Pts',(-10.4687217460001,15.2,-3.59474986700001));
#271906=CARTESIAN_POINT('Ctrl Pts',(-10.4687217460001,11.6,-3.59474986700001));
#271907=CARTESIAN_POINT('Ctrl Pts',(-10.4711680340001,15.2,-3.59679744900001));
#271908=CARTESIAN_POINT('Ctrl Pts',(-10.4711680340001,11.6,-3.59679744900001));
#271909=CARTESIAN_POINT('Ctrl Pts',(-10.4736166110001,15.2,-3.59885030100001));
#271910=CARTESIAN_POINT('Ctrl Pts',(-10.4736166110001,11.6,-3.59885030100001));
#271911=CARTESIAN_POINT('Ctrl Pts',(-10.4760674640001,15.2,-3.60090842000002));
#271912=CARTESIAN_POINT('Ctrl Pts',(-10.4760674640001,11.6,-3.60090842000002));
#271913=CARTESIAN_POINT('Ctrl Pts',(-10.4785205830001,15.2,-3.60297180700002));
#271914=CARTESIAN_POINT('Ctrl Pts',(-10.4785205830001,11.6,-3.60297180700002));
#271915=CARTESIAN_POINT('Ctrl Pts',(-10.4809759550001,15.2,-3.60504046200001));
#271916=CARTESIAN_POINT('Ctrl Pts',(-10.4809759550001,11.6,-3.60504046200001));
#271917=CARTESIAN_POINT('Ctrl Pts',(-10.4834335690001,15.2,-3.60711438300001));
#271918=CARTESIAN_POINT('Ctrl Pts',(-10.4834335690001,11.6,-3.60711438300001));
#271919=CARTESIAN_POINT('Ctrl Pts',(-10.4858934160001,15.2,-3.60919357300002));
#271920=CARTESIAN_POINT('Ctrl Pts',(-10.4858934160001,11.6,-3.60919357300002));
#271921=CARTESIAN_POINT('Ctrl Pts',(-10.4883554830001,15.2,-3.61127802800001));
#271922=CARTESIAN_POINT('Ctrl Pts',(-10.4883554830001,11.6,-3.61127802800001));
#271923=CARTESIAN_POINT('Ctrl Pts',(-10.4908197590001,15.2,-3.61336774900002));
#271924=CARTESIAN_POINT('Ctrl Pts',(-10.4908197590001,11.6,-3.61336774900002));
#271925=CARTESIAN_POINT('Ctrl Pts',(-10.4932862330001,15.2,-3.61546273600001));
#271926=CARTESIAN_POINT('Ctrl Pts',(-10.4932862330001,11.6,-3.61546273600002));
#271927=CARTESIAN_POINT('Ctrl Pts',(-10.4957548950001,15.2,-3.61756298900001));
#271928=CARTESIAN_POINT('Ctrl Pts',(-10.4957548950001,11.6,-3.61756298900001));
#271929=CARTESIAN_POINT('Ctrl Pts',(-10.4982257320001,15.2,-3.61966850600002));
#271930=CARTESIAN_POINT('Ctrl Pts',(-10.4982257320001,11.6,-3.61966850600002));
#271931=CARTESIAN_POINT('Ctrl Pts',(-10.5006987350001,15.2,-3.62177928800001));
#271932=CARTESIAN_POINT('Ctrl Pts',(-10.5006987350001,11.6,-3.62177928800001));
#271933=CARTESIAN_POINT('Ctrl Pts',(-10.5031738910001,15.2,-3.62389533400002));
#271934=CARTESIAN_POINT('Ctrl Pts',(-10.5031738910001,11.6,-3.62389533400002));
#271935=CARTESIAN_POINT('Ctrl Pts',(-10.5056511920001,15.2,-3.62601664500001));
#271936=CARTESIAN_POINT('Ctrl Pts',(-10.5056511920001,11.6,-3.62601664500001));
#271937=CARTESIAN_POINT('Ctrl Pts',(-10.5081306230001,15.2,-3.62814321800002));
#271938=CARTESIAN_POINT('Ctrl Pts',(-10.5081306230001,11.6,-3.62814321800002));
#271939=CARTESIAN_POINT('Ctrl Pts',(-10.5106121760001,15.2,-3.63027505600002));
#271940=CARTESIAN_POINT('Ctrl Pts',(-10.5106121760001,11.6,-3.63027505600002));
#271941=CARTESIAN_POINT('Ctrl Pts',(-10.5130958400001,15.2,-3.63241215500001));
#271942=CARTESIAN_POINT('Ctrl Pts',(-10.5130958400001,11.6,-3.63241215500001));
#271943=CARTESIAN_POINT('Ctrl Pts',(-10.5155816020001,15.2,-3.63455451700001));
#271944=CARTESIAN_POINT('Ctrl Pts',(-10.5155816020001,11.6,-3.63455451700002));
#271945=CARTESIAN_POINT('Ctrl Pts',(-10.5180694530001,15.2,-3.63670214000001));
#271946=CARTESIAN_POINT('Ctrl Pts',(-10.5180694530001,11.6,-3.63670214000001));
#271947=CARTESIAN_POINT('Ctrl Pts',(-10.5205593820001,15.2,-3.63885502500001));
#271948=CARTESIAN_POINT('Ctrl Pts',(-10.5205593820001,11.6,-3.63885502500001));
#271949=CARTESIAN_POINT('Ctrl Pts',(-10.5230513770001,15.2,-3.64101317100001));
#271950=CARTESIAN_POINT('Ctrl Pts',(-10.5230513770001,11.6,-3.64101317100001));
#271951=CARTESIAN_POINT('Ctrl Pts',(-10.5255454300001,15.2,-3.64317657700001));
#271952=CARTESIAN_POINT('Ctrl Pts',(-10.5255454300001,11.6,-3.64317657700001));
#271953=CARTESIAN_POINT('Ctrl Pts',(-10.5280415260001,15.2,-3.64534524300002));
#271954=CARTESIAN_POINT('Ctrl Pts',(-10.5280415260001,11.6,-3.64534524300002));
#271955=CARTESIAN_POINT('Ctrl Pts',(-10.5305396570001,15.2,-3.64751916900001));
#271956=CARTESIAN_POINT('Ctrl Pts',(-10.5305396570001,11.6,-3.64751916900001));
#271957=CARTESIAN_POINT('Ctrl Pts',(-10.5330398120001,15.2,-3.64969835300001));
#271958=CARTESIAN_POINT('Ctrl Pts',(-10.5330398120001,11.6,-3.64969835300002));
#271959=CARTESIAN_POINT('Ctrl Pts',(-10.5355419810001,15.2,-3.65188279700002));
#271960=CARTESIAN_POINT('Ctrl Pts',(-10.5355419810001,11.6,-3.65188279700002));
#271961=CARTESIAN_POINT('Ctrl Pts',(-10.5380461510001,15.2,-3.65407249800001));
#271962=CARTESIAN_POINT('Ctrl Pts',(-10.5380461510001,11.6,-3.65407249800001));
#271963=CARTESIAN_POINT('Ctrl Pts',(-10.5405523130001,15.2,-3.65626745600002));
#271964=CARTESIAN_POINT('Ctrl Pts',(-10.5405523130001,11.6,-3.65626745600002));
#271965=CARTESIAN_POINT('Ctrl Pts',(-10.5430604560001,15.2,-3.65846767300001));
#271966=CARTESIAN_POINT('Ctrl Pts',(-10.5430604560001,11.6,-3.65846767300001));
#271967=CARTESIAN_POINT('Ctrl Pts',(-10.5455705700001,15.2,-3.66067314500001));
#271968=CARTESIAN_POINT('Ctrl Pts',(-10.5455705700001,11.6,-3.66067314500001));
#271969=CARTESIAN_POINT('Ctrl Pts',(-10.5480826430001,15.2,-3.66288387400001));
#271970=CARTESIAN_POINT('Ctrl Pts',(-10.5480826430001,11.6,-3.66288387400001));
#271971=CARTESIAN_POINT('Ctrl Pts',(-10.5505966660001,15.2,-3.66509985700001));
#271972=CARTESIAN_POINT('Ctrl Pts',(-10.5505966660001,11.6,-3.66509985700001));
#271973=CARTESIAN_POINT('Ctrl Pts',(-10.5531126260001,15.2,-3.66732109700001));
#271974=CARTESIAN_POINT('Ctrl Pts',(-10.5531126260001,11.6,-3.66732109700001));
#271975=CARTESIAN_POINT('Ctrl Pts',(-10.5556305150001,15.2,-3.66954758900001));
#271976=CARTESIAN_POINT('Ctrl Pts',(-10.5556305150001,11.6,-3.66954758900001));
#271977=CARTESIAN_POINT('Ctrl Pts',(-10.5581503220001,15.2,-3.67177933600002));
#271978=CARTESIAN_POINT('Ctrl Pts',(-10.5581503220001,11.6,-3.67177933600002));
#271979=CARTESIAN_POINT('Ctrl Pts',(-10.5606720350001,15.2,-3.67401633600001));
#271980=CARTESIAN_POINT('Ctrl Pts',(-10.5606720350001,11.6,-3.67401633600001));
#271981=CARTESIAN_POINT('Ctrl Pts',(-10.5631956460001,15.2,-3.67625858900002));
#271982=CARTESIAN_POINT('Ctrl Pts',(-10.5631956460001,11.6,-3.67625858900002));
#271983=CARTESIAN_POINT('Ctrl Pts',(-10.5657211420001,15.2,-3.67850609400001));
#271984=CARTESIAN_POINT('Ctrl Pts',(-10.5657211420001,11.6,-3.67850609400001));
#271985=CARTESIAN_POINT('Ctrl Pts',(-10.5682485140001,15.2,-3.68075885100001));
#271986=CARTESIAN_POINT('Ctrl Pts',(-10.5682485140001,11.6,-3.68075885100001));
#271987=CARTESIAN_POINT('Ctrl Pts',(-10.5707777510001,15.2,-3.68301685800001));
#271988=CARTESIAN_POINT('Ctrl Pts',(-10.5707777510001,11.6,-3.68301685800001));
#271989=CARTESIAN_POINT('Ctrl Pts',(-10.5733088430001,15.2,-3.68528011600001));
#271990=CARTESIAN_POINT('Ctrl Pts',(-10.5733088430001,11.6,-3.68528011600001));
#271991=CARTESIAN_POINT('Ctrl Pts',(-10.5758417790001,15.2,-3.68754862400001));
#271992=CARTESIAN_POINT('Ctrl Pts',(-10.5758417790001,11.6,-3.68754862400001));
#271993=CARTESIAN_POINT('Ctrl Pts',(-10.5783765500001,15.2,-3.68982238000001));
#271994=CARTESIAN_POINT('Ctrl Pts',(-10.5783765500001,11.6,-3.68982238000001));
#271995=CARTESIAN_POINT('Ctrl Pts',(-10.5809131450001,15.2,-3.69210138500002));
#271996=CARTESIAN_POINT('Ctrl Pts',(-10.5809131450001,11.6,-3.69210138500002));
#271997=CARTESIAN_POINT('Ctrl Pts',(-10.5834515520001,15.2,-3.69438563900002));
#271998=CARTESIAN_POINT('Ctrl Pts',(-10.5834515520001,11.6,-3.69438563900002));
#271999=CARTESIAN_POINT('Ctrl Pts',(-10.5859917630001,15.2,-3.69667513900001));
#272000=CARTESIAN_POINT('Ctrl Pts',(-10.5859917630001,11.6,-3.69667513900001));
#272001=CARTESIAN_POINT('Ctrl Pts',(-10.5885337670001,15.2,-3.69896988600001));
#272002=CARTESIAN_POINT('Ctrl Pts',(-10.5885337670001,11.6,-3.69896988600001));
#272003=CARTESIAN_POINT('Ctrl Pts',(-10.5910775530001,15.2,-3.70126987800001));
#272004=CARTESIAN_POINT('Ctrl Pts',(-10.5910775530001,11.6,-3.70126987800001));
#272005=CARTESIAN_POINT('Ctrl Pts',(-10.5936231110001,15.2,-3.70357511600002));
#272006=CARTESIAN_POINT('Ctrl Pts',(-10.5936231110001,11.6,-3.70357511600002));
#272007=CARTESIAN_POINT('Ctrl Pts',(-10.5961704330001,15.2,-3.70588560000002));
#272008=CARTESIAN_POINT('Ctrl Pts',(-10.5961704330001,11.6,-3.70588560000002));
#272009=CARTESIAN_POINT('Ctrl Pts',(-10.5987195050001,15.2,-3.70820132600001));
#272010=CARTESIAN_POINT('Ctrl Pts',(-10.5987195050001,11.6,-3.70820132600001));
#272011=CARTESIAN_POINT('Ctrl Pts',(-10.6012703200001,15.2,-3.71052229700001));
#272012=CARTESIAN_POINT('Ctrl Pts',(-10.6012703200001,11.6,-3.71052229700001));
#272013=CARTESIAN_POINT('Ctrl Pts',(-10.6038228660001,15.2,-3.71284850900001));
#272014=CARTESIAN_POINT('Ctrl Pts',(-10.6038228660001,11.6,-3.71284850900001));
#272015=CARTESIAN_POINT('Ctrl Pts',(-10.6063771330001,15.2,-3.71517996400001));
#272016=CARTESIAN_POINT('Ctrl Pts',(-10.6063771330001,11.6,-3.71517996400002));
#272017=CARTESIAN_POINT('Ctrl Pts',(-10.6089331120001,15.2,-3.71751666000002));
#272018=CARTESIAN_POINT('Ctrl Pts',(-10.6089331120001,11.6,-3.71751666000002));
#272019=CARTESIAN_POINT('Ctrl Pts',(-10.6114907930001,15.2,-3.71985859600001));
#272020=CARTESIAN_POINT('Ctrl Pts',(-10.6114907930001,11.6,-3.71985859600001));
#272021=CARTESIAN_POINT('Ctrl Pts',(-10.6140501650001,15.2,-3.72220577200002));
#272022=CARTESIAN_POINT('Ctrl Pts',(-10.6140501650001,11.6,-3.72220577200002));
#272023=CARTESIAN_POINT('Ctrl Pts',(-10.6166112170001,15.2,-3.72455818700002));
#272024=CARTESIAN_POINT('Ctrl Pts',(-10.6166112170001,11.6,-3.72455818700002));
#272025=CARTESIAN_POINT('Ctrl Pts',(-10.6191739410001,15.2,-3.72691584200001));
#272026=CARTESIAN_POINT('Ctrl Pts',(-10.6191739410001,11.6,-3.72691584200001));
#272027=CARTESIAN_POINT('Ctrl Pts',(-10.6217383260001,15.2,-3.72927873300001));
#272028=CARTESIAN_POINT('Ctrl Pts',(-10.6217383260001,11.6,-3.72927873300001));
#272029=CARTESIAN_POINT('Ctrl Pts',(-10.6243043610001,15.2,-3.73164686100001));
#272030=CARTESIAN_POINT('Ctrl Pts',(-10.6243043610001,11.6,-3.73164686100001));
#272031=CARTESIAN_POINT('Ctrl Pts',(-10.6268720380001,15.2,-3.73402022600001));
#272032=CARTESIAN_POINT('Ctrl Pts',(-10.6268720380001,11.6,-3.73402022600001));
#272033=CARTESIAN_POINT('Ctrl Pts',(-10.6294413450001,15.2,-3.73639882600001));
#272034=CARTESIAN_POINT('Ctrl Pts',(-10.6294413450001,11.6,-3.73639882600001));
#272035=CARTESIAN_POINT('Ctrl Pts',(-10.6320122750001,15.2,-3.73878266000002));
#272036=CARTESIAN_POINT('Ctrl Pts',(-10.6320122750001,11.6,-3.73878266000002));
#272037=CARTESIAN_POINT('Ctrl Pts',(-10.6345848160001,15.2,-3.74117172800001));
#272038=CARTESIAN_POINT('Ctrl Pts',(-10.6345848160001,11.6,-3.74117172800001));
#272039=CARTESIAN_POINT('Ctrl Pts',(-10.6371589570001,15.2,-3.74356603100002));
#272040=CARTESIAN_POINT('Ctrl Pts',(-10.6371589570001,11.6,-3.74356603100002));
#272041=CARTESIAN_POINT('Ctrl Pts',(-10.6397346900001,15.2,-3.74596556400002));
#272042=CARTESIAN_POINT('Ctrl Pts',(-10.6397346900001,11.6,-3.74596556400002));
#272043=CARTESIAN_POINT('Ctrl Pts',(-10.6423120040001,15.2,-3.74837033000002));
#272044=CARTESIAN_POINT('Ctrl Pts',(-10.6423120040001,11.6,-3.74837033000002));
#272045=CARTESIAN_POINT('Ctrl Pts',(-10.6448908910001,15.2,-3.75078032600001));
#272046=CARTESIAN_POINT('Ctrl Pts',(-10.6448908910001,11.6,-3.75078032600001));
#272047=CARTESIAN_POINT('Ctrl Pts',(-10.6474713390001,15.2,-3.75319555200001));
#272048=CARTESIAN_POINT('Ctrl Pts',(-10.6474713390001,11.6,-3.75319555200001));
#272049=CARTESIAN_POINT('Ctrl Pts',(-10.6500533400001,15.2,-3.75561600800001));
#272050=CARTESIAN_POINT('Ctrl Pts',(-10.6500533400001,11.6,-3.75561600800001));
#272051=CARTESIAN_POINT('Ctrl Pts',(-10.6526368820001,15.2,-3.75804169200002));
#272052=CARTESIAN_POINT('Ctrl Pts',(-10.6526368820001,11.6,-3.75804169200002));
#272053=CARTESIAN_POINT('Ctrl Pts',(-10.6552219570001,15.2,-3.76047260400002));
#272054=CARTESIAN_POINT('Ctrl Pts',(-10.6552219570001,11.6,-3.76047260400002));
#272055=CARTESIAN_POINT('Ctrl Pts',(-10.6578085550001,15.2,-3.76290874200001));
#272056=CARTESIAN_POINT('Ctrl Pts',(-10.6578085550001,11.6,-3.76290874200001));
#272057=CARTESIAN_POINT('Ctrl Pts',(-10.6603966660001,15.2,-3.76535010600001));
#272058=CARTESIAN_POINT('Ctrl Pts',(-10.6603966660001,11.6,-3.76535010600001));
#272059=CARTESIAN_POINT('Ctrl Pts',(-10.6629862800001,15.2,-3.76779669600001));
#272060=CARTESIAN_POINT('Ctrl Pts',(-10.6629862800001,11.6,-3.76779669600001));
#272061=CARTESIAN_POINT('Ctrl Pts',(-10.6655773880001,15.2,-3.77024850900002));
#272062=CARTESIAN_POINT('Ctrl Pts',(-10.6655773880001,11.6,-3.77024850900002));
#272063=CARTESIAN_POINT('Ctrl Pts',(-10.6681699790001,15.2,-3.77270554500001));
#272064=CARTESIAN_POINT('Ctrl Pts',(-10.6681699790001,11.6,-3.77270554500001));
#272065=CARTESIAN_POINT('Ctrl Pts',(-10.6707640450001,15.2,-3.77516780500001));
#272066=CARTESIAN_POINT('Ctrl Pts',(-10.6707640450001,11.6,-3.77516780500002));
#272067=CARTESIAN_POINT('Ctrl Pts',(-10.6733595760001,15.2,-3.77763528600001));
#272068=CARTESIAN_POINT('Ctrl Pts',(-10.6733595760001,11.6,-3.77763528600001));
#272069=CARTESIAN_POINT('Ctrl Pts',(-10.6759565610001,15.2,-3.78010798800001));
#272070=CARTESIAN_POINT('Ctrl Pts',(-10.6759565610001,11.6,-3.78010798800001));
#272071=CARTESIAN_POINT('Ctrl Pts',(-10.6785549920001,15.2,-3.78258590900002));
#272072=CARTESIAN_POINT('Ctrl Pts',(-10.6785549920001,11.6,-3.78258590900002));
#272073=CARTESIAN_POINT('Ctrl Pts',(-10.6811548570001,15.2,-3.78506905000001));
#272074=CARTESIAN_POINT('Ctrl Pts',(-10.6811548570001,11.6,-3.78506905000001));
#272075=CARTESIAN_POINT('Ctrl Pts',(-10.6837561510001,15.2,-3.78755740900001));
#272076=CARTESIAN_POINT('Ctrl Pts',(-10.6837561510001,11.6,-3.78755740900001));
#272077=CARTESIAN_POINT('Ctrl Pts',(-10.6863588600001,15.2,-3.79005098500001));
#272078=CARTESIAN_POINT('Ctrl Pts',(-10.6863588600001,11.6,-3.79005098500001));
#272079=CARTESIAN_POINT('Ctrl Pts',(-10.6889629760001,15.2,-3.79254977800001));
#272080=CARTESIAN_POINT('Ctrl Pts',(-10.6889629760001,11.6,-3.79254977800001));
#272081=CARTESIAN_POINT('Ctrl Pts',(-10.6915684890001,15.2,-3.79505378600001));
#272082=CARTESIAN_POINT('Ctrl Pts',(-10.6915684890001,11.6,-3.79505378600001));
#272083=CARTESIAN_POINT('Ctrl Pts',(-10.6941753910001,15.2,-3.79756300900001));
#272084=CARTESIAN_POINT('Ctrl Pts',(-10.6941753910001,11.6,-3.79756300900001));
#272085=CARTESIAN_POINT('Ctrl Pts',(-10.6967836710001,15.2,-3.80007744500002));
#272086=CARTESIAN_POINT('Ctrl Pts',(-10.6967836710001,11.6,-3.80007744500002));
#272087=CARTESIAN_POINT('Ctrl Pts',(-10.6993933200001,15.2,-3.80259709400002));
#272088=CARTESIAN_POINT('Ctrl Pts',(-10.6993933200001,11.6,-3.80259709400002));
#272089=CARTESIAN_POINT('Ctrl Pts',(-10.7020043290001,15.2,-3.80512195600001));
#272090=CARTESIAN_POINT('Ctrl Pts',(-10.7020043290001,11.6,-3.80512195600002));
#272091=CARTESIAN_POINT('Ctrl Pts',(-10.7046166880001,15.2,-3.80765202700001));
#272092=CARTESIAN_POINT('Ctrl Pts',(-10.7046166880001,11.6,-3.80765202700002));
#272093=CARTESIAN_POINT('Ctrl Pts',(-10.7072303880001,15.2,-3.81018730900001));
#272094=CARTESIAN_POINT('Ctrl Pts',(-10.7072303880001,11.6,-3.81018730900002));
#272095=CARTESIAN_POINT('Ctrl Pts',(-10.7098454180001,15.2,-3.81272780000002));
#272096=CARTESIAN_POINT('Ctrl Pts',(-10.7098454180001,11.6,-3.81272780000002));
#272097=CARTESIAN_POINT('Ctrl Pts',(-10.7124617720001,15.2,-3.81527349900002));
#272098=CARTESIAN_POINT('Ctrl Pts',(-10.7124617720001,11.6,-3.81527349900002));
#272099=CARTESIAN_POINT('Ctrl Pts',(-10.7150794370001,15.2,-3.81782440400002));
#272100=CARTESIAN_POINT('Ctrl Pts',(-10.7150794370001,11.6,-3.81782440400002));
#272101=CARTESIAN_POINT('Ctrl Pts',(-10.7176984060001,15.2,-3.82038051600002));
#272102=CARTESIAN_POINT('Ctrl Pts',(-10.7176984060001,11.6,-3.82038051600002));
#272103=CARTESIAN_POINT('Ctrl Pts',(-10.7203186690001,15.2,-3.82294183300001));
#272104=CARTESIAN_POINT('Ctrl Pts',(-10.7203186690001,11.6,-3.82294183300001));
#272105=CARTESIAN_POINT('Ctrl Pts',(-10.7229402150001,15.2,-3.82550835400002));
#272106=CARTESIAN_POINT('Ctrl Pts',(-10.7229402150001,11.6,-3.82550835400002));
#272107=CARTESIAN_POINT('Ctrl Pts',(-10.7255630380001,15.2,-3.82808007900001));
#272108=CARTESIAN_POINT('Ctrl Pts',(-10.7255630380001,11.6,-3.82808007900001));
#272109=CARTESIAN_POINT('Ctrl Pts',(-10.7281871270001,15.2,-3.83065700500001));
#272110=CARTESIAN_POINT('Ctrl Pts',(-10.7281871270001,11.6,-3.83065700500001));
#272111=CARTESIAN_POINT('Ctrl Pts',(-10.7308124710001,15.2,-3.83323913300002));
#272112=CARTESIAN_POINT('Ctrl Pts',(-10.7308124710001,11.6,-3.83323913300002));
#272113=CARTESIAN_POINT('Ctrl Pts',(-10.7334390640001,15.2,-3.83582646100002));
#272114=CARTESIAN_POINT('Ctrl Pts',(-10.7334390640001,11.6,-3.83582646100002));
#272115=CARTESIAN_POINT('Ctrl Pts',(-10.7360668940001,15.2,-3.83841898800001));
#272116=CARTESIAN_POINT('Ctrl Pts',(-10.7360668940001,11.6,-3.83841898800001));
#272117=CARTESIAN_POINT('Ctrl Pts',(-10.7386959530001,15.2,-3.84101671300002));
#272118=CARTESIAN_POINT('Ctrl Pts',(-10.7386959530001,11.6,-3.84101671300002));
#272119=CARTESIAN_POINT('Ctrl Pts',(-10.7413262330001,15.2,-3.84361963500002));
#272120=CARTESIAN_POINT('Ctrl Pts',(-10.7413262330001,11.6,-3.84361963500002));
#272121=CARTESIAN_POINT('Ctrl Pts',(-10.7439577220001,15.2,-3.84622775400001));
#272122=CARTESIAN_POINT('Ctrl Pts',(-10.7439577220001,11.6,-3.84622775400001));
#272123=CARTESIAN_POINT('Ctrl Pts',(-10.7465904140001,15.2,-3.84884106800001));
#272124=CARTESIAN_POINT('Ctrl Pts',(-10.7465904140001,11.6,-3.84884106800001));
#272125=CARTESIAN_POINT('Ctrl Pts',(-10.7492242980001,15.2,-3.85145957500002));
#272126=CARTESIAN_POINT('Ctrl Pts',(-10.7492242980001,11.6,-3.85145957500002));
#272127=CARTESIAN_POINT('Ctrl Pts',(-10.7518593670001,15.2,-3.85408327600001));
#272128=CARTESIAN_POINT('Ctrl Pts',(-10.7518593670001,11.6,-3.85408327600001));
#272129=CARTESIAN_POINT('Ctrl Pts',(-10.7544956090001,15.2,-3.85671216900001));
#272130=CARTESIAN_POINT('Ctrl Pts',(-10.7544956090001,11.6,-3.85671216900001));
#272131=CARTESIAN_POINT('Ctrl Pts',(-10.7571330160001,15.2,-3.85934625200001));
#272132=CARTESIAN_POINT('Ctrl Pts',(-10.7571330160001,11.6,-3.85934625200001));
#272133=CARTESIAN_POINT('Ctrl Pts',(-10.7597715780001,15.2,-3.86198552600002));
#272134=CARTESIAN_POINT('Ctrl Pts',(-10.7597715780001,11.6,-3.86198552600002));
#272135=CARTESIAN_POINT('Ctrl Pts',(-10.7624112860001,15.2,-3.86462998800001));
#272136=CARTESIAN_POINT('Ctrl Pts',(-10.7624112860001,11.6,-3.86462998800001));
#272137=CARTESIAN_POINT('Ctrl Pts',(-10.7650521310001,15.2,-3.86727963800002));
#272138=CARTESIAN_POINT('Ctrl Pts',(-10.7650521310001,11.6,-3.86727963800002));
#272139=CARTESIAN_POINT('Ctrl Pts',(-10.7676941040001,15.2,-3.86993447500001));
#272140=CARTESIAN_POINT('Ctrl Pts',(-10.7676941040001,11.6,-3.86993447500001));
#272141=CARTESIAN_POINT('Ctrl Pts',(-10.7703371960001,15.2,-3.87259449700001));
#272142=CARTESIAN_POINT('Ctrl Pts',(-10.7703371960001,11.6,-3.87259449700002));
#272143=CARTESIAN_POINT('Ctrl Pts',(-10.7729813980001,15.2,-3.87525970300001));
#272144=CARTESIAN_POINT('Ctrl Pts',(-10.7729813980001,11.6,-3.87525970300001));
#272145=CARTESIAN_POINT('Ctrl Pts',(-10.7756267050001,15.2,-3.87793009300001));
#272146=CARTESIAN_POINT('Ctrl Pts',(-10.7756267050001,11.6,-3.87793009300002));
#272147=CARTESIAN_POINT('Ctrl Pts',(-10.7782731050001,15.2,-3.88060566600001));
#272148=CARTESIAN_POINT('Ctrl Pts',(-10.7782731050001,11.6,-3.88060566600001));
#272149=CARTESIAN_POINT('Ctrl Pts',(-10.7809205920001,15.2,-3.88328642000001));
#272150=CARTESIAN_POINT('Ctrl Pts',(-10.7809205920001,11.6,-3.88328642000001));
#272151=CARTESIAN_POINT('Ctrl Pts',(-10.7835691560001,15.2,-3.88597235400002));
#272152=CARTESIAN_POINT('Ctrl Pts',(-10.7835691560001,11.6,-3.88597235400002));
#272153=CARTESIAN_POINT('Ctrl Pts',(-10.7862187870001,15.2,-3.88866346700001));
#272154=CARTESIAN_POINT('Ctrl Pts',(-10.7862187870001,11.6,-3.88866346700001));
#272155=CARTESIAN_POINT('Ctrl Pts',(-10.7888694730001,15.2,-3.89135975900002));
#272156=CARTESIAN_POINT('Ctrl Pts',(-10.7888694730001,11.6,-3.89135975900002));
#272157=CARTESIAN_POINT('Ctrl Pts',(-10.7915212030001,15.2,-3.89406122600001));
#272158=CARTESIAN_POINT('Ctrl Pts',(-10.7915212030001,11.6,-3.89406122600001));
#272159=CARTESIAN_POINT('Ctrl Pts',(-10.7941739680001,15.2,-3.89676786900001));
#272160=CARTESIAN_POINT('Ctrl Pts',(-10.7941739680001,11.6,-3.89676786900001));
#272161=CARTESIAN_POINT('Ctrl Pts',(-10.7968277560001,15.2,-3.89947968500001));
#272162=CARTESIAN_POINT('Ctrl Pts',(-10.7968277560001,11.6,-3.89947968500001));
#272163=CARTESIAN_POINT('Ctrl Pts',(-10.7994825590001,15.2,-3.90219667400002));
#272164=CARTESIAN_POINT('Ctrl Pts',(-10.7994825590001,11.6,-3.90219667400002));
#272165=CARTESIAN_POINT('Ctrl Pts',(-10.8021383740001,15.2,-3.90491883400002));
#272166=CARTESIAN_POINT('Ctrl Pts',(-10.8021383740001,11.6,-3.90491883400002));
#272167=CARTESIAN_POINT('Ctrl Pts',(-10.8047951940001,15.2,-3.90764616700002));
#272168=CARTESIAN_POINT('Ctrl Pts',(-10.8047951940001,11.6,-3.90764616700002));
#272169=CARTESIAN_POINT('Ctrl Pts',(-10.8074530190001,15.2,-3.91037866900001));
#272170=CARTESIAN_POINT('Ctrl Pts',(-10.8074530190001,11.6,-3.91037866900001));
#272171=CARTESIAN_POINT('Ctrl Pts',(-10.8095800800001,15.2,-3.91256880900002));
#272172=CARTESIAN_POINT('Ctrl Pts',(-10.8095800800001,11.6,-3.91256880900002));
#272173=CARTESIAN_POINT('Ctrl Pts',(-10.8111758270001,15.2,-3.91421373900001));
#272174=CARTESIAN_POINT('Ctrl Pts',(-10.8111758270001,11.6,-3.91421373900001));
#272175=CARTESIAN_POINT('Ctrl Pts',(-10.8122398590001,15.2,-3.91531139400001));
#272176=CARTESIAN_POINT('Ctrl Pts',(-10.8122398590001,11.6,-3.91531139400001));
#272177=CARTESIAN_POINT('Ctrl Pts',(-10.8127719260001,15.2,-3.91586047900002));
#272178=CARTESIAN_POINT('Ctrl Pts',(-10.8127719260001,11.6,-3.91586047900002));
#272179=CARTESIAN_POINT('Ctrl Pts',(-9.86852965800006,15.2,-3.20199116200001));
#272180=CARTESIAN_POINT('Ctrl Pts',(-9.87017542455281,15.2,-3.20268658157505));
#272181=CARTESIAN_POINT('Ctrl Pts',(-9.87187175388031,15.2,-3.20340918512851));
#272182=CARTESIAN_POINT('Ctrl Pts',(-9.87361750383377,15.2,-3.20415921016782));
#272183=CARTESIAN_POINT('Ctrl Pts',(-9.87537167267595,15.2,-3.204912852207));
#272184=CARTESIAN_POINT('Ctrl Pts',(-9.87717574023296,15.2,-3.20569417462551));
#272185=CARTESIAN_POINT('Ctrl Pts',(-9.87902857842933,15.2,-3.20650338954498));
#272186=CARTESIAN_POINT('Ctrl Pts',(-9.88088141645739,15.2,-3.20731260439096));
#272187=CARTESIAN_POINT('Ctrl Pts',(-9.88278302851245,15.2,-3.2081497105564));
#272188=CARTESIAN_POINT('Ctrl Pts',(-9.88473231752497,15.2,-3.20901491227497));
#272189=CARTESIAN_POINT('Ctrl Pts',(-9.88668160653749,15.2,-3.20988011399353));
#272190=CARTESIAN_POINT('Ctrl Pts',(-9.88867857432724,15.1999999999999,
-3.21077340827496));
#272191=CARTESIAN_POINT('Ctrl Pts',(-9.89072215651906,15.2,-3.21169499220255));
#272192=CARTESIAN_POINT('Ctrl Pts',(-9.89276573889652,15.2,-3.21261657621385));
#272193=CARTESIAN_POINT('Ctrl Pts',(-9.89485593802995,15.2,-3.21356644793468));
#272194=CARTESIAN_POINT('Ctrl Pts',(-9.89699171648278,15.2,-3.21454479382328));
#272195=CARTESIAN_POINT('Ctrl Pts',(-9.89912749474164,15.2,-3.21552313962301));
#272196=CARTESIAN_POINT('Ctrl Pts',(-9.90130885331331,15.2,-3.21652996002495));
#272197=CARTESIAN_POINT('Ctrl Pts',(-9.90353478649266,15.2,-3.2175654317421));
#272198=CARTESIAN_POINT('Ctrl Pts',(-9.90576071967203,15.2,-3.21860090345925));
#272199=CARTESIAN_POINT('Ctrl Pts',(-9.90803122770171,15.2,-3.21966502577316));
#272200=CARTESIAN_POINT('Ctrl Pts',(-9.91034532736571,15.2,-3.22075797048219));
#272201=CARTESIAN_POINT('Ctrl Pts',(-9.91265942723992,15.2,-3.22185091529049));
#272202=CARTESIAN_POINT('Ctrl Pts',(-9.91501712228624,15.2,-3.22297268096072));
#272203=CARTESIAN_POINT('Ctrl Pts',(-9.91741745500329,15.2,-3.22412343085873));
#272204=CARTESIAN_POINT('Ctrl Pts',(-9.91981778750232,15.2,-3.22527418065224));
#272205=CARTESIAN_POINT('Ctrl Pts',(-9.92226075844071,15.2,-3.22645391558363));
#272206=CARTESIAN_POINT('Ctrl Pts',(-9.92474543535224,15.2,-3.22766278929097));
#272207=CARTESIAN_POINT('Ctrl Pts',(-9.92723011226377,15.2,-3.22887166299831));
#272208=CARTESIAN_POINT('Ctrl Pts',(-9.92975649757194,15.2,-3.23010967648666));
#272209=CARTESIAN_POINT('Ctrl Pts',(-9.93232368131025,15.2,-3.23137697818935));
#272210=CARTESIAN_POINT('Ctrl Pts',(-9.93489086504854,15.2,-3.23264427989204));
#272211=CARTESIAN_POINT('Ctrl Pts',(-9.937498847977,15.2,-3.23394087139731));
#272212=CARTESIAN_POINT('Ctrl Pts',(-9.94014674371137,15.2,-3.2352668930971));
#272213=CARTESIAN_POINT('Ctrl Pts',(-9.94279463968627,15.2,-3.23659291491734));
#272214=CARTESIAN_POINT('Ctrl Pts',(-9.94548244775676,15.2,-3.2379483681488));
#272215=CARTESIAN_POINT('Ctrl Pts',(-9.9482093021571,15.2,-3.23933338705891));
#272216=CARTESIAN_POINT('Ctrl Pts',(-9.95093615630974,15.2,-3.24071840584321));
#272217=CARTESIAN_POINT('Ctrl Pts',(-9.95370205916299,15.2,-3.24213299364531));
#272218=CARTESIAN_POINT('Ctrl Pts',(-9.95650616499038,15.2,-3.24357727726597));
#272219=CARTESIAN_POINT('Ctrl Pts',(-9.95931027081778,15.2,-3.24502156088664));
#272220=CARTESIAN_POINT('Ctrl Pts',(-9.96215257803497,15.2,-3.24649554081774));
#272221=CARTESIAN_POINT('Ctrl Pts',(-9.96503226217778,15.2,-3.24799934334439));
#272222=CARTESIAN_POINT('Ctrl Pts',(-9.96791194658215,15.2,-3.24950314600764));
#272223=CARTESIAN_POINT('Ctrl Pts',(-9.97082900750689,15.2,-3.25103676921545));
#272224=CARTESIAN_POINT('Ctrl Pts',(-9.97378263891945,15.2,-3.25260033280197));
#272225=CARTESIAN_POINT('Ctrl Pts',(-9.97673627006372,15.2,-3.25416389624646));
#272226=CARTESIAN_POINT('Ctrl Pts',(-9.9797264712199,15.2,-3.2557573999259));
#272227=CARTESIAN_POINT('Ctrl Pts',(-9.98275245154029,15.2,-3.25738095645756));
#272228=CARTESIAN_POINT('Ctrl Pts',(-9.9857784318607,15.2,-3.25900451298922));
#272229=CARTESIAN_POINT('Ctrl Pts',(-9.98884019241067,15.2,-3.26065812320466));
#272230=CARTESIAN_POINT('Ctrl Pts',(-9.99193696262913,15.2,-3.2623418945581));
#272231=CARTESIAN_POINT('Ctrl Pts',(-9.99503373312888,15.2,-3.26402566606449));
#272232=CARTESIAN_POINT('Ctrl Pts',(-9.998165510507,15.2,-3.26573959840982));
#272233=CARTESIAN_POINT('Ctrl Pts',(-10.0013315413397,15.2,-3.2674837951771));
#272234=CARTESIAN_POINT('Ctrl Pts',(-10.0044975718848,15.2,-3.26922799178594));
#272235=CARTESIAN_POINT('Ctrl Pts',(-10.0076978541008,15.2,-3.27100245334886));
#272236=CARTESIAN_POINT('Ctrl Pts',(-10.0109316504833,15.2,-3.27280727678329));
#272237=CARTESIAN_POINT('Ctrl Pts',(-10.0141654468658,15.2,-3.27461210021773));
#272238=CARTESIAN_POINT('Ctrl Pts',(-10.0174327550794,15.2,-3.27644728653758));
#272239=CARTESIAN_POINT('Ctrl Pts',(-10.0207328517058,15.2,-3.27831292881123));
#272240=CARTESIAN_POINT('Ctrl Pts',(-10.024032948632,15.2,-3.28017857125434));
#272241=CARTESIAN_POINT('Ctrl Pts',(-10.0273658332479,15.2,-3.28207466921122));
#272242=CARTESIAN_POINT('Ctrl Pts',(-10.0307307971001,15.2,-3.28400131173497));
#272243=CARTESIAN_POINT('Ctrl Pts',(-10.0340957606467,15.2,-3.28592795408372));
#272244=CARTESIAN_POINT('Ctrl Pts',(-10.0374928009605,15.2,-3.28788514203065));
#272245=CARTESIAN_POINT('Ctrl Pts',(-10.0409212255182,15.2,-3.28987295846753));
#272246=CARTESIAN_POINT('Ctrl Pts',(-10.044349650076,15.2,-3.29186077490442));
#272247=CARTESIAN_POINT('Ctrl Pts',(-10.0478094564797,15.2,-3.29387922119752));
#272248=CARTESIAN_POINT('Ctrl Pts',(-10.0512999632682,15.2,-3.29592837662175));
#272249=CARTESIAN_POINT('Ctrl Pts',(-10.054208719031,15.2,-3.29763600620398));
#272250=CARTESIAN_POINT('Ctrl Pts',(-10.0571387938471,15.2,-3.29936496208675));
#272251=CARTESIAN_POINT('Ctrl Pts',(-10.0600898020405,15.2,-3.30111528812729));
#272252=CARTESIAN_POINT('Ctrl Pts',(-10.0630408102338,15.2,-3.30286561416783));
#272253=CARTESIAN_POINT('Ctrl Pts',(-10.0660127512293,15.2,-3.30463730936312));
#272254=CARTESIAN_POINT('Ctrl Pts',(-10.0690052420067,15.2,-3.30643041798232));
#272255=CARTESIAN_POINT('Ctrl Pts',(-10.0719977327841,15.2,-3.30822352660152));
#272256=CARTESIAN_POINT('Ctrl Pts',(-10.07501077405,15.2,-3.31003804834439));
#272257=CARTESIAN_POINT('Ctrl Pts',(-10.0780439907167,15.2,-3.31187402202496));
#272258=CARTESIAN_POINT('Ctrl Pts',(-10.0810772073834,15.2,-3.31370999570553));
#272259=CARTESIAN_POINT('Ctrl Pts',(-10.0841305999877,15.2,-3.31556742195907));
#272260=CARTESIAN_POINT('Ctrl Pts',(-10.0872037960433,15.2,-3.31744634050932));
#272261=CARTESIAN_POINT('Ctrl Pts',(-10.090276992099,15.2,-3.31932525905957));
#272262=CARTESIAN_POINT('Ctrl Pts',(-10.0933699960638,15.2,-3.32122566818577));
#272263=CARTESIAN_POINT('Ctrl Pts',(-10.0964824387037,15.2,-3.32314760665912));
#272264=CARTESIAN_POINT('Ctrl Pts',(-10.0995948813436,15.2,-3.32506954513246));
#272265=CARTESIAN_POINT('Ctrl Pts',(-10.1027267670941,15.2,-3.32701301197191));
#272266=CARTESIAN_POINT('Ctrl Pts',(-10.1058777332062,15.2,-3.32897804065361));
#272267=CARTESIAN_POINT('Ctrl Pts',(-10.1090286993183,15.2,-3.3309430693353));
#272268=CARTESIAN_POINT('Ctrl Pts',(-10.1121987497985,15.2,-3.33292966151468));
#272269=CARTESIAN_POINT('Ctrl Pts',(-10.1153875285702,15.2,-3.33493785099149));
#272270=CARTESIAN_POINT('Ctrl Pts',(-10.1185763073419,15.2,-3.3369460404683));
#272271=CARTESIAN_POINT('Ctrl Pts',(-10.121783815176,15.2,-3.3389758262332));
#272272=CARTESIAN_POINT('Ctrl Pts',(-10.1250097044136,15.2,-3.34102723977663));
#272273=CARTESIAN_POINT('Ctrl Pts',(-10.1282355936513,15.2,-3.34307865332005));
#272274=CARTESIAN_POINT('Ctrl Pts',(-10.131479863653,15.2,-3.3451516946333));
#272275=CARTESIAN_POINT('Ctrl Pts',(-10.1347421721267,15.2,-3.34724639477395));
#272276=CARTESIAN_POINT('Ctrl Pts',(-10.1380044802448,15.2,-3.34934109468628));
#272277=CARTESIAN_POINT('Ctrl Pts',(-10.1412848268184,15.2,-3.35145745227179));
#272278=CARTESIAN_POINT('Ctrl Pts',(-10.1445828725686,15.2,-3.35359549641198));
#272279=CARTESIAN_POINT('Ctrl Pts',(-10.1478809186783,15.2,-3.35573354078522));
#272280=CARTESIAN_POINT('Ctrl Pts',(-10.1511966662766,15.2,-3.35789327163863));
#272281=CARTESIAN_POINT('Ctrl Pts',(-10.1545297791224,15.2,-3.3600747167063));
#272282=CARTESIAN_POINT('Ctrl Pts',(-10.1578628919682,15.2,-3.36225616177396));
#272283=CARTESIAN_POINT('Ctrl Pts',(-10.1612133718276,15.2,-3.36445931992739));
#272284=CARTESIAN_POINT('Ctrl Pts',(-10.1645808903679,15.2,-3.36668421596729));
#272285=CARTESIAN_POINT('Ctrl Pts',(-10.1679484089082,15.2,-3.36890911200718));
#272286=CARTESIAN_POINT('Ctrl Pts',(-10.1713329648365,15.2,-3.37115574719711));
#272287=CARTESIAN_POINT('Ctrl Pts',(-10.1747342345886,15.2,-3.37342414571171));
#272288=CARTESIAN_POINT('Ctrl Pts',(-10.1781355043407,15.2,-3.37569254422632));
#272289=CARTESIAN_POINT('Ctrl Pts',(-10.1815534888375,15.2,-3.37798270471114));
#272290=CARTESIAN_POINT('Ctrl Pts',(-10.1849878675172,15.2,-3.38029464984889));
#272291=CARTESIAN_POINT('Ctrl Pts',(-10.1891091221574,15.2,-3.3830689841654));
#272292=CARTESIAN_POINT('Ctrl Pts',(-10.1932539831256,15.2,-3.38587468871912));
#272293=CARTESIAN_POINT('Ctrl Pts',(-10.1974219096877,15.2,-3.38871180004254));
#272294=CARTESIAN_POINT('Ctrl Pts',(-10.2002005270171,15.2,-3.39060320733379));
#272295=CARTESIAN_POINT('Ctrl Pts',(-10.2029893949504,15.2,-3.39250857353023));
#272296=CARTESIAN_POINT('Ctrl Pts',(-10.2057883537898,15.2,-3.39442790804865));
#272297=CARTESIAN_POINT('Ctrl Pts',(-10.2085873130105,15.2,-3.39634724282858));
#272298=CARTESIAN_POINT('Ctrl Pts',(-10.2113963643396,15.2,-3.39828054381079));
#272299=CARTESIAN_POINT('Ctrl Pts',(-10.2142153494943,15.2,-3.40022782458501));
#272300=CARTESIAN_POINT('Ctrl Pts',(-10.2170343342648,15.2,-3.40217510509392));
#272301=CARTESIAN_POINT('Ctrl Pts',(-10.2198632526341,15.2,-3.40413636252046));
#272302=CARTESIAN_POINT('Ctrl Pts',(-10.2227019507347,15.2,-3.40611160708028));
#272303=CARTESIAN_POINT('Ctrl Pts',(-10.2255406492221,15.2,-3.40808685190924));
#272304=CARTESIAN_POINT('Ctrl Pts',(-10.2283891251487,15.2,-3.4100760822497));
#272305=CARTESIAN_POINT('Ctrl Pts',(-10.2312472264481,15.2,-3.41207930851572));
#272306=CARTESIAN_POINT('Ctrl Pts',(-10.2341053273581,15.2,-3.4140825345088));
#272307=CARTESIAN_POINT('Ctrl Pts',(-10.2369730513868,15.2,-3.41609975441768));
#272308=CARTESIAN_POINT('Ctrl Pts',(-10.2398502482066,15.2,-3.4181309782507));
#272309=CARTESIAN_POINT('Ctrl Pts',(-10.2427274454183,15.2,-3.42016220236048));
#272310=CARTESIAN_POINT('Ctrl Pts',(-10.2456141140673,15.2,-3.42220742849139));
#272311=CARTESIAN_POINT('Ctrl Pts',(-10.2485101040035,15.2,-3.4242666646601));
#272312=CARTESIAN_POINT('Ctrl Pts',(-10.2514060935452,15.2,-3.42632590054824));
#272313=CARTESIAN_POINT('Ctrl Pts',(-10.2543114045956,15.2,-3.42839914698696));
#272314=CARTESIAN_POINT('Ctrl Pts',(-10.2572258863355,15.2,-3.43048640969716));
#272315=CARTESIAN_POINT('Ctrl Pts',(-10.2601403684725,15.2,-3.43257367269175));
#272316=CARTESIAN_POINT('Ctrl Pts',(-10.2630640229044,15.2,-3.43467495284292));
#272317=CARTESIAN_POINT('Ctrl Pts',(-10.2659967002315,15.2,-3.43679025568135));
#272318=CARTESIAN_POINT('Ctrl Pts',(-10.268929377159,15.2,-3.43890555823157));
#272319=CARTESIAN_POINT('Ctrl Pts',(-10.2718710773958,15.2,-3.44103488317618));
#272320=CARTESIAN_POINT('Ctrl Pts',(-10.2748216555426,15.2,-3.44317823766619));
#272321=CARTESIAN_POINT('Ctrl Pts',(-10.2785098785276,15.2,-3.44585743099772));
#272322=CARTESIAN_POINT('Ctrl Pts',(-10.2822119710007,15.2,-3.44855854367164));
#272323=CARTESIAN_POINT('Ctrl Pts',(-10.2859276518104,15.2,-3.45128158720893));
#272324=CARTESIAN_POINT('Ctrl Pts',(-10.2889001966201,15.2,-3.45346002215749));
#272325=CARTESIAN_POINT('Ctrl Pts',(-10.2918814373921,15.2,-3.45565249229263));
#272326=CARTESIAN_POINT('Ctrl Pts',(-10.2948712307779,15.2,-3.45785900241381));
#272327=CARTESIAN_POINT('Ctrl Pts',(-10.2978610237562,15.2,-3.46006551223434));
#272328=CARTESIAN_POINT('Ctrl Pts',(-10.3008593699856,15.2,-3.46228606144095));
#272329=CARTESIAN_POINT('Ctrl Pts',(-10.3038661270168,15.2,-3.46452065536794));
#272330=CARTESIAN_POINT('Ctrl Pts',(-10.3068728844575,15.2,-3.4667552495994));
#272331=CARTESIAN_POINT('Ctrl Pts',(-10.3098880524291,15.2,-3.46900388897341));
#272332=CARTESIAN_POINT('Ctrl Pts',(-10.3129114917188,15.2,-3.47126657521817));
#272333=CARTESIAN_POINT('Ctrl Pts',(-10.3159349305965,15.2,-3.47352926115465));
#272334=CARTESIAN_POINT('Ctrl Pts',(-10.3189666405635,15.2,-3.47580599606413));
#272335=CARTESIAN_POINT('Ctrl Pts',(-10.3220064815363,15.2,-3.47809678187542));
#272336=CARTESIAN_POINT('Ctrl Pts',(-10.3250463229234,15.2,-3.48038756799883));
#272337=CARTESIAN_POINT('Ctrl Pts',(-10.3280942959362,15.2,-3.48269240520968));
#272338=CARTESIAN_POINT('Ctrl Pts',(-10.3311502614917,15.2,-3.48501129672495));
#272339=CARTESIAN_POINT('Ctrl Pts',(-10.3342062270471,15.2,-3.48733018824023));
#272340=CARTESIAN_POINT('Ctrl Pts',(-10.3372701884479,15.2,-3.48966313395713));
#272341=CARTESIAN_POINT('Ctrl Pts',(-10.3403420052273,15.2,-3.49201013614203));
#272342=CARTESIAN_POINT('Ctrl Pts',(-10.3434138215881,15.2,-3.49435713800716));
#272343=CARTESIAN_POINT('Ctrl Pts',(-10.3464934962197,15.2,-3.49671819684843));
#272344=CARTESIAN_POINT('Ctrl Pts',(-10.3495808919813,15.2,-3.49909331399834));
#272345=CARTESIAN_POINT('Ctrl Pts',(-10.3526682881635,15.2,-3.50146843147186));
#272346=CARTESIAN_POINT('Ctrl Pts',(-10.3557634060541,15.2,-3.50385760800215));
#272347=CARTESIAN_POINT('Ctrl Pts',(-10.3588661115573,15.2,-3.50626084363456));
#272348=CARTESIAN_POINT('Ctrl Pts',(-10.3619688166378,15.2,-3.50866407893954));
#272349=CARTESIAN_POINT('Ctrl Pts',(-10.3650791111006,15.2,-3.5110813765899));
#272350=CARTESIAN_POINT('Ctrl Pts',(-10.3681968595119,15.2,-3.51351273383466));
#272351=CARTESIAN_POINT('Ctrl Pts',(-10.371314608348,15.2,-3.5159440914107));
#272352=CARTESIAN_POINT('Ctrl Pts',(-10.3744398117545,15.2,-3.51838951047657));
#272353=CARTESIAN_POINT('Ctrl Pts',(-10.3775723399713,15.2,-3.52084899262359));
#272354=CARTESIAN_POINT('Ctrl Pts',(-10.3807048677612,15.2,-3.52330847443551));
#272355=CARTESIAN_POINT('Ctrl Pts',(-10.3838447177117,15.2,-3.52578201770102));
#272356=CARTESIAN_POINT('Ctrl Pts',(-10.3869917620095,15.2,-3.52826962349673));
#272357=CARTESIAN_POINT('Ctrl Pts',(-10.3901388067361,15.2,-3.53075722963138));
#272358=CARTESIAN_POINT('Ctrl Pts',(-10.3932930434469,15.2,-3.53325889711217));
#272359=CARTESIAN_POINT('Ctrl Pts',(-10.3964543455085,15.2,-3.53577462847242));
#272360=CARTESIAN_POINT('Ctrl Pts',(-10.3996156471394,15.2,-3.53829035948991));
#272361=CARTESIAN_POINT('Ctrl Pts',(-10.4027840118273,15.2,-3.540820151774));
#272362=CARTESIAN_POINT('Ctrl Pts',(-10.4059593129559,15.2,-3.54336400684238));
#272363=CARTESIAN_POINT('Ctrl Pts',(-10.4091346145171,15.2,-3.54590786225736));
#272364=CARTESIAN_POINT('Ctrl Pts',(-10.4123168524667,15.2,-3.54846578042204));
#272365=CARTESIAN_POINT('Ctrl Pts',(-10.4155058987105,15.2,-3.55103775801838));
#272366=CARTESIAN_POINT('Ctrl Pts',(-10.4186949445199,15.2,-3.55360973526429));
#272367=CARTESIAN_POINT('Ctrl Pts',(-10.421890800525,15.2,-3.55619577468885));
#272368=CARTESIAN_POINT('Ctrl Pts',(-10.4250933389847,15.2,-3.55879587380818));
#272369=CARTESIAN_POINT('Ctrl Pts',(-10.4282958778808,15.2,-3.56139597328176));
#272370=CARTESIAN_POINT('Ctrl Pts',(-10.431505100697,15.2,-3.5640101331206));
#272371=CARTESIAN_POINT('Ctrl Pts',(-10.4347208809834,15.2,-3.56663835054162));
#272372=CARTESIAN_POINT('Ctrl Pts',(-10.4379366612697,15.2,-3.56926656796264));
#272373=CARTESIAN_POINT('Ctrl Pts',(-10.441159000893,15.2,-3.57190884457696));
#272374=CARTESIAN_POINT('Ctrl Pts',(-10.4443877745696,15.2,-3.57456517616761));
#272375=CARTESIAN_POINT('Ctrl Pts',(-10.4476165478063,15.2,-3.57722150739633));
#272376=CARTESIAN_POINT('Ctrl Pts',(-10.4508517572842,15.2,-3.57989189565267));
#272377=CARTESIAN_POINT('Ctrl Pts',(-10.4540932777562,15.2,-3.58257633805647));
#272378=CARTESIAN_POINT('Ctrl Pts',(-10.4573347986697,15.2,-3.58526078082602));
#272379=CARTESIAN_POINT('Ctrl Pts',(-10.4605826327263,15.2,-3.58795927716365));
#272380=CARTESIAN_POINT('Ctrl Pts',(-10.4638366570154,15.2,-3.5906718247018));
#272381=CARTESIAN_POINT('Ctrl Pts',(-10.4670906808611,15.2,-3.59338437187037));
#272382=CARTESIAN_POINT('Ctrl Pts',(-10.4703508946366,15.2,-3.59611097056212));
#272383=CARTESIAN_POINT('Ctrl Pts',(-10.4736171797581,15.2,-3.59885161755938));
#272384=CARTESIAN_POINT('Ctrl Pts',(-10.4768834653246,15.2,-3.60159226493005));
#272385=CARTESIAN_POINT('Ctrl Pts',(-10.4801558212383,15.2,-3.6043469596919));
#272386=CARTESIAN_POINT('Ctrl Pts',(-10.4834341276924,15.2,-3.60711570059347));
#272387=CARTESIAN_POINT('Ctrl Pts',(-10.4867124336999,15.2,-3.60988444111779));
#272388=CARTESIAN_POINT('Ctrl Pts',(-10.4899966905866,15.2,-3.61266722592879));
#272389=CARTESIAN_POINT('Ctrl Pts',(-10.4932867797061,15.2,-3.61546405225478));
#272390=CARTESIAN_POINT('Ctrl Pts',(-10.4965768692739,15.2,-3.61826087896184));
#272391=CARTESIAN_POINT('Ctrl Pts',(-10.4998727905591,15.2,-3.62107174573727));
#272392=CARTESIAN_POINT('Ctrl Pts',(-10.5031744274617,15.2,-3.6238966504477));
#272393=CARTESIAN_POINT('Ctrl Pts',(-10.5064760639143,15.2,-3.62672155477323));
#272394=CARTESIAN_POINT('Ctrl Pts',(-10.509783414714,15.2,-3.62956049639464));
#272395=CARTESIAN_POINT('Ctrl Pts',(-10.5130963640527,15.2,-3.63241347030272));
#272396=CARTESIAN_POINT('Ctrl Pts',(-10.5164093138427,15.2,-3.63526644459952));
#272397=CARTESIAN_POINT('Ctrl Pts',(-10.5197278608097,15.2,-3.6381334514749));
#272398=CARTESIAN_POINT('Ctrl Pts',(-10.5230518917135,15.2,-3.64101448624395));
#272399=CARTESIAN_POINT('Ctrl Pts',(-10.5263759221644,15.2,-3.64389552062046));
#272400=CARTESIAN_POINT('Ctrl Pts',(-10.5297054338141,15.2,-3.64679058244413));
#272401=CARTESIAN_POINT('Ctrl Pts',(-10.5330403149298,15.2,-3.64969966748266));
#272402=CARTESIAN_POINT('Ctrl Pts',(-10.5363751964999,15.2,-3.65260875291756));
#272403=CARTESIAN_POINT('Ctrl Pts',(-10.5397154450937,15.2,-3.65553186073961));
#272404=CARTESIAN_POINT('Ctrl Pts',(-10.5430609487356,15.2,-3.65846898680196));
#272405=CARTESIAN_POINT('Ctrl Pts',(-10.5464064519218,15.2,-3.66140611246413));
#272406=CARTESIAN_POINT('Ctrl Pts',(-10.5497572096734,15.2,-3.6643572552701));
#272407=CARTESIAN_POINT('Ctrl Pts',(-10.5531131076764,15.2,-3.66732240958183));
#272408=CARTESIAN_POINT('Ctrl Pts',(-10.5556300317501,15.2,-3.66954627582062));
#272409=CARTESIAN_POINT('Ctrl Pts',(-10.5581498485163,15.2,-3.67177802294497));
#272410=CARTESIAN_POINT('Ctrl Pts',(-10.5606725100083,15.2,-3.67401764972987));
#272411=CARTESIAN_POINT('Ctrl Pts',(-10.563195171042,15.2,-3.67625727610791));
#272412=CARTESIAN_POINT('Ctrl Pts',(-10.5657206770006,15.2,-3.67850478189386));
#272413=CARTESIAN_POINT('Ctrl Pts',(-10.568248980534,15.2,-3.68076016377093));
#272414=CARTESIAN_POINT('Ctrl Pts',(-10.5707772840674,15.2,-3.68301554564799));
#272415=CARTESIAN_POINT('Ctrl Pts',(-10.5733083851495,15.2,-3.68527880414086));
#272416=CARTESIAN_POINT('Ctrl Pts',(-10.5758422377357,15.2,-3.68754993602703));
#272417=CARTESIAN_POINT('Ctrl Pts',(-10.5783760903218,15.2,-3.68982106791319));
#272418=CARTESIAN_POINT('Ctrl Pts',(-10.5809126948451,15.2,-3.69210007368729));
#272419=CARTESIAN_POINT('Ctrl Pts',(-10.5834520029727,15.2,-3.69438695053122));
#272420=CARTESIAN_POINT('Ctrl Pts',(-10.5868377474504,15.2,-3.69743611993342));
#272421=CARTESIAN_POINT('Ctrl Pts',(-10.5902283002085,15.2,-3.70049928002284));
#272422=CARTESIAN_POINT('Ctrl Pts',(-10.5936235525052,15.2,-3.70357642796975));
#272423=CARTESIAN_POINT('Ctrl Pts',(-10.5961699914963,15.2,-3.7058842887203));
#272424=CARTESIAN_POINT('Ctrl Pts',(-10.598719073554,15.2,-3.70820001622045));
#272425=CARTESIAN_POINT('Ctrl Pts',(-10.6012707530449,15.2,-3.71052360755336));
#272426=CARTESIAN_POINT('Ctrl Pts',(-10.6038224325357,15.2,-3.71284719888628));
#272427=CARTESIAN_POINT('Ctrl Pts',(-10.6063767084503,15.2,-3.71517865412643));
#272428=CARTESIAN_POINT('Ctrl Pts',(-10.608933537494,15.2,-3.71751797001042));
#272429=CARTESIAN_POINT('Ctrl Pts',(-10.6114903665377,15.2,-3.7198572858944));
#272430=CARTESIAN_POINT('Ctrl Pts',(-10.6140497478458,15.2,-3.72220446215606));
#272431=CARTESIAN_POINT('Ctrl Pts',(-10.6166116349727,15.2,-3.72455949695616));
#272432=CARTESIAN_POINT('Ctrl Pts',(-10.6191735220996,15.2,-3.72691453175626));
#272433=CARTESIAN_POINT('Ctrl Pts',(-10.6217379161138,15.2,-3.72927742364517));
#272434=CARTESIAN_POINT('Ctrl Pts',(-10.624304771187,15.2,-3.73164816997501));
#272435=CARTESIAN_POINT('Ctrl Pts',(-10.6268716262601,15.2,-3.73401891630486));
#272436=CARTESIAN_POINT('Ctrl Pts',(-10.6294409427498,15.2,-3.73639751703417));
#272437=CARTESIAN_POINT('Ctrl Pts',(-10.6320126771977,15.2,-3.73878396798805));
#272438=CARTESIAN_POINT('Ctrl Pts',(-10.6345844121128,15.2,-3.74117041937548));
#272439=CARTESIAN_POINT('Ctrl Pts',(-10.6371585627536,15.2,-3.74356472287346));
#272440=CARTESIAN_POINT('Ctrl Pts',(-10.6397350858367,15.2,-3.74596687272364));
#272441=CARTESIAN_POINT('Ctrl Pts',(-10.6423116084518,15.2,-3.74836902213742));
#272442=CARTESIAN_POINT('Ctrl Pts',(-10.644890504014,15.2,-3.75077901900063));
#272443=CARTESIAN_POINT('Ctrl Pts',(-10.6474717277161,15.2,-3.75319685995116));
#272444=CARTESIAN_POINT('Ctrl Pts',(-10.6500529514182,15.2,-3.75561470090168));
#272445=CARTESIAN_POINT('Ctrl Pts',(-10.652636502459,15.2,-3.75804038595309));
#272446=CARTESIAN_POINT('Ctrl Pts',(-10.6552223380319,15.2,-3.76047391078201));
#272447=CARTESIAN_POINT('Ctrl Pts',(-10.6578081736048,15.2,-3.76290743561094));
#272448=CARTESIAN_POINT('Ctrl Pts',(-10.6603962934108,15.2,-3.76534880048895));
#272449=CARTESIAN_POINT('Ctrl Pts',(-10.6629866534834,15.2,-3.76779800177495));
#272450=CARTESIAN_POINT('Ctrl Pts',(-10.6655770135559,15.2,-3.77024720306095));
#272451=CARTESIAN_POINT('Ctrl Pts',(-10.6681696134284,15.2,-3.77270423972167));
#272452=CARTESIAN_POINT('Ctrl Pts',(-10.6707644109589,15.2,-3.77516911000642));
#272453=CARTESIAN_POINT('Ctrl Pts',(-10.6733592084894,15.2,-3.77763398029118));
#272454=CARTESIAN_POINT('Ctrl Pts',(-10.6759562027948,15.2,-3.78010668256707));
#272455=CARTESIAN_POINT('Ctrl Pts',(-10.6785553499918,15.2,-3.78258721343421));
#272456=CARTESIAN_POINT('Ctrl Pts',(-10.6811544976609,15.2,-3.78506774475199));
#272457=CARTESIAN_POINT('Ctrl Pts',(-10.6837558001723,15.2,-3.78755610499696));
#272458=CARTESIAN_POINT('Ctrl Pts',(-10.6863592123009,15.2,-3.79005228977747));
#272459=CARTESIAN_POINT('Ctrl Pts',(-10.6889626239566,15.2,-3.7925484741045));
#272460=CARTESIAN_POINT('Ctrl Pts',(-10.6915681458188,15.2,-3.79505248330087));
#272461=CARTESIAN_POINT('Ctrl Pts',(-10.6941757360212,15.2,-3.79756431275268));
#272462=CARTESIAN_POINT('Ctrl Pts',(-10.6967833262237,15.2,-3.80007614220449));
#272463=CARTESIAN_POINT('Ctrl Pts',(-10.6993929836795,15.2,-3.80259579225008));
#272464=CARTESIAN_POINT('Ctrl Pts',(-10.7020046667931,15.2,-3.80512325857559));
#272465=CARTESIAN_POINT('Ctrl Pts',(-10.7046163499067,15.2,-3.8076507249011));
#272466=CARTESIAN_POINT('Ctrl Pts',(-10.7072300578284,15.2,-3.81018600720901));
#272467=CARTESIAN_POINT('Ctrl Pts',(-10.7098457489417,15.2,-3.81272910199162));
#272468=CARTESIAN_POINT('Ctrl Pts',(-10.712461440055,15.2,-3.81527219677424));
#272469=CARTESIAN_POINT('Ctrl Pts',(-10.7150791141766,15.2,-3.81782310269817));
#272470=CARTESIAN_POINT('Ctrl Pts',(-10.7176987292062,15.2,-3.82038181697953));
#272471=CARTESIAN_POINT('Ctrl Pts',(-10.721191549563,15.2,-3.82379343633122));
#272472=CARTESIAN_POINT('Ctrl Pts',(-10.7246878198781,15.2,-3.82721893633585));
#272473=CARTESIAN_POINT('Ctrl Pts',(-10.7281874412995,15.2,-3.83065830597411));
#272474=CARTESIAN_POINT('Ctrl Pts',(-10.7308121571272,15.2,-3.83323783296851));
#272475=CARTESIAN_POINT('Ctrl Pts',(-10.7334387577986,15.2,-3.8358251619599));
#272476=CARTESIAN_POINT('Ctrl Pts',(-10.7360672015366,15.2,-3.83842028778296));
#272477=CARTESIAN_POINT('Ctrl Pts',(-10.7386956452746,15.2,-3.84101541360602));
#272478=CARTESIAN_POINT('Ctrl Pts',(-10.7413259330123,15.2,-3.84361833651148));
#272479=CARTESIAN_POINT('Ctrl Pts',(-10.7439580227084,15.2,-3.84622905274996));
#272480=CARTESIAN_POINT('Ctrl Pts',(-10.7474674759552,15.2,-3.84971000805078));
#272481=CARTESIAN_POINT('Ctrl Pts',(-10.7509801356163,15.2,-3.85320481629488));
#272482=CARTESIAN_POINT('Ctrl Pts',(-10.7544959008082,15.2,-3.85671346709863));
#272483=CARTESIAN_POINT('Ctrl Pts',(-10.7580116655211,15.2,-3.86022211742432));
#272484=CARTESIAN_POINT('Ctrl Pts',(-10.7615305356029,15.2,-3.8637446105123));
#272485=CARTESIAN_POINT('Ctrl Pts',(-10.7650524129976,15.2,-3.86728093473922));
#272486=CARTESIAN_POINT('Ctrl Pts',(-10.7676938211637,15.2,-3.86993317802986));
#272487=CARTESIAN_POINT('Ctrl Pts',(-10.770336920208,15.2,-3.87259320084024));
#272488=CARTESIAN_POINT('Ctrl Pts',(-10.7729816739035,15.2,-3.87526099870097));
#272489=CARTESIAN_POINT('Ctrl Pts',(-10.7756264275989,15.2,-3.87792879656169));
#272490=CARTESIAN_POINT('Ctrl Pts',(-10.7782728361025,15.2,-3.88060437059689));
#272491=CARTESIAN_POINT('Ctrl Pts',(-10.7809208606728,15.2,-3.883287714415));
#272492=CARTESIAN_POINT('Ctrl Pts',(-10.7835688857241,15.2,-3.88597105872058));
#272493=CARTESIAN_POINT('Ctrl Pts',(-10.7862185270425,15.2,-3.88866217361171));
#272494=CARTESIAN_POINT('Ctrl Pts',(-10.7888697345947,15.2,-3.89136105337999));
#272495=CARTESIAN_POINT('Ctrl Pts',(-10.7915209416652,15.2,-3.89405993265798));
#272496=CARTESIAN_POINT('Ctrl Pts',(-10.7941737152272,15.2,-3.89676657630398));
#272497=CARTESIAN_POINT('Ctrl Pts',(-10.7968280103053,15.2,-3.89948097875854));
#272498=CARTESIAN_POINT('Ctrl Pts',(-10.7994823053833,15.2,-3.9021953812131));
#272499=CARTESIAN_POINT('Ctrl Pts',(-10.802138123266,15.2,-3.9049175422178));
#272500=CARTESIAN_POINT('Ctrl Pts',(-10.8047954455073,15.2,-3.90764745961307));
#272501=CARTESIAN_POINT('Ctrl Pts',(-10.8074527677486,15.2,-3.91037737700834));
#272502=CARTESIAN_POINT('Ctrl Pts',(-10.8101115924531,15.2,-3.91311505550024));
#272503=CARTESIAN_POINT('Ctrl Pts',(-10.8127719255158,15.2,-3.91586047850026));
#272504=CARTESIAN_POINT('Ctrl Pts',(-9.86852965800006,12.2,-3.20199116200001));
#272505=CARTESIAN_POINT('Ctrl Pts',(-9.87017542455281,12.2,-3.20268658157505));
#272506=CARTESIAN_POINT('Ctrl Pts',(-9.87187175388031,12.2,-3.2034091851285));
#272507=CARTESIAN_POINT('Ctrl Pts',(-9.87361750383377,12.2,-3.20415921016783));
#272508=CARTESIAN_POINT('Ctrl Pts',(-9.87537167267595,12.2,-3.204912852207));
#272509=CARTESIAN_POINT('Ctrl Pts',(-9.87717574023296,12.2,-3.20569417462551));
#272510=CARTESIAN_POINT('Ctrl Pts',(-9.87902857842933,12.2,-3.20650338954498));
#272511=CARTESIAN_POINT('Ctrl Pts',(-9.88088141645739,12.2,-3.20731260439096));
#272512=CARTESIAN_POINT('Ctrl Pts',(-9.88278302851245,12.2,-3.2081497105564));
#272513=CARTESIAN_POINT('Ctrl Pts',(-9.88473231752497,12.2,-3.20901491227497));
#272514=CARTESIAN_POINT('Ctrl Pts',(-9.88668160653749,12.2,-3.20988011399353));
#272515=CARTESIAN_POINT('Ctrl Pts',(-9.88867857432724,12.2,-3.21077340827496));
#272516=CARTESIAN_POINT('Ctrl Pts',(-9.89072215651907,12.2,-3.21169499220255));
#272517=CARTESIAN_POINT('Ctrl Pts',(-9.89276573889652,12.2,-3.21261657621385));
#272518=CARTESIAN_POINT('Ctrl Pts',(-9.89485593802995,12.2,-3.21356644793469));
#272519=CARTESIAN_POINT('Ctrl Pts',(-9.89699171648278,12.2,-3.21454479382328));
#272520=CARTESIAN_POINT('Ctrl Pts',(-9.89912749474163,12.2,-3.21552313962301));
#272521=CARTESIAN_POINT('Ctrl Pts',(-9.90130885331331,12.2,-3.21652996002495));
#272522=CARTESIAN_POINT('Ctrl Pts',(-9.90353478649266,12.2,-3.2175654317421));
#272523=CARTESIAN_POINT('Ctrl Pts',(-9.90576071967203,12.2,-3.21860090345926));
#272524=CARTESIAN_POINT('Ctrl Pts',(-9.90803122770171,12.2,-3.21966502577315));
#272525=CARTESIAN_POINT('Ctrl Pts',(-9.91034532736571,12.2,-3.22075797048219));
#272526=CARTESIAN_POINT('Ctrl Pts',(-9.91265942723992,12.2,-3.22185091529049));
#272527=CARTESIAN_POINT('Ctrl Pts',(-9.91501712228624,12.2,-3.22297268096071));
#272528=CARTESIAN_POINT('Ctrl Pts',(-9.91741745500329,12.2,-3.22412343085874));
#272529=CARTESIAN_POINT('Ctrl Pts',(-9.91981778750232,12.2,-3.22527418065224));
#272530=CARTESIAN_POINT('Ctrl Pts',(-9.92226075844071,12.2,-3.22645391558362));
#272531=CARTESIAN_POINT('Ctrl Pts',(-9.92474543535223,12.2,-3.22766278929097));
#272532=CARTESIAN_POINT('Ctrl Pts',(-9.92723011226377,12.2,-3.22887166299831));
#272533=CARTESIAN_POINT('Ctrl Pts',(-9.92975649757194,12.2,-3.23010967648667));
#272534=CARTESIAN_POINT('Ctrl Pts',(-9.93232368131025,12.2,-3.23137697818935));
#272535=CARTESIAN_POINT('Ctrl Pts',(-9.93489086504854,12.2,-3.23264427989204));
#272536=CARTESIAN_POINT('Ctrl Pts',(-9.937498847977,12.2,-3.23394087139731));
#272537=CARTESIAN_POINT('Ctrl Pts',(-9.94014674371137,12.2,-3.2352668930971));
#272538=CARTESIAN_POINT('Ctrl Pts',(-9.94279463968627,12.2,-3.23659291491734));
#272539=CARTESIAN_POINT('Ctrl Pts',(-9.94548244775676,12.2,-3.2379483681488));
#272540=CARTESIAN_POINT('Ctrl Pts',(-9.9482093021571,12.2,-3.23933338705891));
#272541=CARTESIAN_POINT('Ctrl Pts',(-9.95093615630974,12.2,-3.24071840584321));
#272542=CARTESIAN_POINT('Ctrl Pts',(-9.953702059163,12.2,-3.24213299364531));
#272543=CARTESIAN_POINT('Ctrl Pts',(-9.95650616499039,12.2,-3.24357727726598));
#272544=CARTESIAN_POINT('Ctrl Pts',(-9.95931027081779,12.2,-3.24502156088664));
#272545=CARTESIAN_POINT('Ctrl Pts',(-9.96215257803497,12.2,-3.24649554081773));
#272546=CARTESIAN_POINT('Ctrl Pts',(-9.96503226217778,12.2,-3.24799934334439));
#272547=CARTESIAN_POINT('Ctrl Pts',(-9.96791194658215,12.2,-3.24950314600764));
#272548=CARTESIAN_POINT('Ctrl Pts',(-9.97082900750689,12.2,-3.25103676921545));
#272549=CARTESIAN_POINT('Ctrl Pts',(-9.97378263891945,12.2,-3.25260033280197));
#272550=CARTESIAN_POINT('Ctrl Pts',(-9.97673627006372,12.2,-3.25416389624646));
#272551=CARTESIAN_POINT('Ctrl Pts',(-9.97972647121991,12.2,-3.25575739992591));
#272552=CARTESIAN_POINT('Ctrl Pts',(-9.9827524515403,12.2,-3.25738095645757));
#272553=CARTESIAN_POINT('Ctrl Pts',(-9.98577843186071,12.2,-3.25900451298923));
#272554=CARTESIAN_POINT('Ctrl Pts',(-9.98884019241067,12.2,-3.26065812320466));
#272555=CARTESIAN_POINT('Ctrl Pts',(-9.99193696262912,12.2,-3.26234189455811));
#272556=CARTESIAN_POINT('Ctrl Pts',(-9.99503373312888,12.2,-3.26402566606449));
#272557=CARTESIAN_POINT('Ctrl Pts',(-9.99816551050701,12.2,-3.26573959840983));
#272558=CARTESIAN_POINT('Ctrl Pts',(-10.0013315413397,12.2,-3.2674837951771));
#272559=CARTESIAN_POINT('Ctrl Pts',(-10.0044975718848,12.2,-3.26922799178594));
#272560=CARTESIAN_POINT('Ctrl Pts',(-10.0076978541008,12.2,-3.27100245334886));
#272561=CARTESIAN_POINT('Ctrl Pts',(-10.0109316504833,12.2,-3.27280727678329));
#272562=CARTESIAN_POINT('Ctrl Pts',(-10.0141654468658,12.2,-3.27461210021773));
#272563=CARTESIAN_POINT('Ctrl Pts',(-10.0174327550794,12.2,-3.27644728653758));
#272564=CARTESIAN_POINT('Ctrl Pts',(-10.0207328517058,12.2,-3.27831292881123));
#272565=CARTESIAN_POINT('Ctrl Pts',(-10.024032948632,12.2,-3.28017857125434));
#272566=CARTESIAN_POINT('Ctrl Pts',(-10.0273658332478,12.2,-3.28207466921121));
#272567=CARTESIAN_POINT('Ctrl Pts',(-10.0307307971001,12.2,-3.28400131173497));
#272568=CARTESIAN_POINT('Ctrl Pts',(-10.0340957606467,12.2,-3.28592795408371));
#272569=CARTESIAN_POINT('Ctrl Pts',(-10.0374928009605,12.2,-3.28788514203065));
#272570=CARTESIAN_POINT('Ctrl Pts',(-10.0409212255182,12.2,-3.28987295846753));
#272571=CARTESIAN_POINT('Ctrl Pts',(-10.044349650076,12.2,-3.29186077490442));
#272572=CARTESIAN_POINT('Ctrl Pts',(-10.0478094564797,12.2,-3.29387922119753));
#272573=CARTESIAN_POINT('Ctrl Pts',(-10.0512999632682,12.2,-3.29592837662175));
#272574=CARTESIAN_POINT('Ctrl Pts',(-10.054208719031,12.2,-3.29763600620398));
#272575=CARTESIAN_POINT('Ctrl Pts',(-10.0571387938471,12.2,-3.29936496208675));
#272576=CARTESIAN_POINT('Ctrl Pts',(-10.0600898020405,12.2,-3.30111528812729));
#272577=CARTESIAN_POINT('Ctrl Pts',(-10.0630408102338,12.2,-3.30286561416783));
#272578=CARTESIAN_POINT('Ctrl Pts',(-10.0660127512293,12.2,-3.30463730936312));
#272579=CARTESIAN_POINT('Ctrl Pts',(-10.0690052420067,12.2,-3.30643041798232));
#272580=CARTESIAN_POINT('Ctrl Pts',(-10.0719977327841,12.2,-3.30822352660152));
#272581=CARTESIAN_POINT('Ctrl Pts',(-10.07501077405,12.2,-3.31003804834439));
#272582=CARTESIAN_POINT('Ctrl Pts',(-10.0780439907167,12.2,-3.31187402202496));
#272583=CARTESIAN_POINT('Ctrl Pts',(-10.0810772073834,12.2,-3.31370999570553));
#272584=CARTESIAN_POINT('Ctrl Pts',(-10.0841305999877,12.2,-3.31556742195907));
#272585=CARTESIAN_POINT('Ctrl Pts',(-10.0872037960433,12.2,-3.31744634050932));
#272586=CARTESIAN_POINT('Ctrl Pts',(-10.090276992099,12.2,-3.31932525905957));
#272587=CARTESIAN_POINT('Ctrl Pts',(-10.0933699960638,12.2,-3.32122566818577));
#272588=CARTESIAN_POINT('Ctrl Pts',(-10.0964824387037,12.2,-3.32314760665912));
#272589=CARTESIAN_POINT('Ctrl Pts',(-10.0995948813436,12.2,-3.32506954513246));
#272590=CARTESIAN_POINT('Ctrl Pts',(-10.1027267670941,12.2,-3.32701301197191));
#272591=CARTESIAN_POINT('Ctrl Pts',(-10.1058777332062,12.2,-3.32897804065361));
#272592=CARTESIAN_POINT('Ctrl Pts',(-10.1090286993183,12.2,-3.3309430693353));
#272593=CARTESIAN_POINT('Ctrl Pts',(-10.1121987497985,12.2,-3.33292966151467));
#272594=CARTESIAN_POINT('Ctrl Pts',(-10.1153875285702,12.2,-3.33493785099149));
#272595=CARTESIAN_POINT('Ctrl Pts',(-10.1185763073419,12.2,-3.3369460404683));
#272596=CARTESIAN_POINT('Ctrl Pts',(-10.121783815176,12.2,-3.3389758262332));
#272597=CARTESIAN_POINT('Ctrl Pts',(-10.1250097044136,12.2,-3.34102723977662));
#272598=CARTESIAN_POINT('Ctrl Pts',(-10.1282355936512,12.2,-3.34307865332006));
#272599=CARTESIAN_POINT('Ctrl Pts',(-10.131479863653,12.2,-3.3451516946333));
#272600=CARTESIAN_POINT('Ctrl Pts',(-10.1347421721267,12.2,-3.34724639477395));
#272601=CARTESIAN_POINT('Ctrl Pts',(-10.1380044802448,12.2,-3.34934109468629));
#272602=CARTESIAN_POINT('Ctrl Pts',(-10.1412848268184,12.2,-3.35145745227179));
#272603=CARTESIAN_POINT('Ctrl Pts',(-10.1445828725686,12.2,-3.35359549641198));
#272604=CARTESIAN_POINT('Ctrl Pts',(-10.1485405281159,12.2,-3.35616114979969));
#272605=CARTESIAN_POINT('Ctrl Pts',(-10.152523672949,12.2,-3.35875803192372));
#272606=CARTESIAN_POINT('Ctrl Pts',(-10.1565317286685,12.2,-3.36138619015165));
#272607=CARTESIAN_POINT('Ctrl Pts',(-10.1598717749195,12.2,-3.36357632188889));
#272608=CARTESIAN_POINT('Ctrl Pts',(-10.1632291239811,12.2,-3.36578817017837));
#272609=CARTESIAN_POINT('Ctrl Pts',(-10.1666034437041,12.2,-3.36802176288784));
#272610=CARTESIAN_POINT('Ctrl Pts',(-10.1699777634272,12.2,-3.3702553555973));
#272611=CARTESIAN_POINT('Ctrl Pts',(-10.1733690573854,12.2,-3.37251069268799));
#272612=CARTESIAN_POINT('Ctrl Pts',(-10.176777000404,12.2,-3.37478779703937));
#272613=CARTESIAN_POINT('Ctrl Pts',(-10.1801849434227,12.2,-3.37706490139075));
#272614=CARTESIAN_POINT('Ctrl Pts',(-10.1836095364654,12.2,-3.37936377212395));
#272615=CARTESIAN_POINT('Ctrl Pts',(-10.1870504602168,12.2,-3.38168443157018));
#272616=CARTESIAN_POINT('Ctrl Pts',(-10.1898031989928,12.2,-3.3835409589754));
#272617=CARTESIAN_POINT('Ctrl Pts',(-10.192566389873,12.2,-3.38541143248989));
#272618=CARTESIAN_POINT('Ctrl Pts',(-10.1953398707567,12.2,-3.38729586111271));
#272619=CARTESIAN_POINT('Ctrl Pts',(-10.1988067221448,12.2,-3.38965139708379));
#272620=CARTESIAN_POINT('Ctrl Pts',(-10.2022896549545,12.2,-3.3920287397045));
#272621=CARTESIAN_POINT('Ctrl Pts',(-10.2057883537898,12.2,-3.39442790804865));
#272622=CARTESIAN_POINT('Ctrl Pts',(-10.2085873130105,12.2,-3.39634724282858));
#272623=CARTESIAN_POINT('Ctrl Pts',(-10.2113963643396,12.2,-3.39828054381079));
#272624=CARTESIAN_POINT('Ctrl Pts',(-10.2142153494943,12.2,-3.40022782458501));
#272625=CARTESIAN_POINT('Ctrl Pts',(-10.2170343342648,12.2,-3.40217510509392));
#272626=CARTESIAN_POINT('Ctrl Pts',(-10.2198632526341,12.2,-3.40413636252046));
#272627=CARTESIAN_POINT('Ctrl Pts',(-10.2227019507347,12.2,-3.40611160708028));
#272628=CARTESIAN_POINT('Ctrl Pts',(-10.2255406492221,12.2,-3.40808685190924));
#272629=CARTESIAN_POINT('Ctrl Pts',(-10.2283891251487,12.2,-3.4100760822497));
#272630=CARTESIAN_POINT('Ctrl Pts',(-10.2312472264481,12.2,-3.41207930851572));
#272631=CARTESIAN_POINT('Ctrl Pts',(-10.2341053273581,12.2,-3.4140825345088));
#272632=CARTESIAN_POINT('Ctrl Pts',(-10.2369730513868,12.2,-3.41609975441768));
#272633=CARTESIAN_POINT('Ctrl Pts',(-10.2398502482066,12.2,-3.41813097825071));
#272634=CARTESIAN_POINT('Ctrl Pts',(-10.2427274454183,12.2,-3.42016220236049));
#272635=CARTESIAN_POINT('Ctrl Pts',(-10.2456141140673,12.2,-3.42220742849139));
#272636=CARTESIAN_POINT('Ctrl Pts',(-10.2485101040035,12.2,-3.4242666646601));
#272637=CARTESIAN_POINT('Ctrl Pts',(-10.2514060935452,12.2,-3.42632590054824));
#272638=CARTESIAN_POINT('Ctrl Pts',(-10.2543114045956,12.2,-3.42839914698696));
#272639=CARTESIAN_POINT('Ctrl Pts',(-10.2572258863355,12.2,-3.43048640969716));
#272640=CARTESIAN_POINT('Ctrl Pts',(-10.2601403684725,12.2,-3.43257367269174));
#272641=CARTESIAN_POINT('Ctrl Pts',(-10.2630640229044,12.2,-3.43467495284292));
#272642=CARTESIAN_POINT('Ctrl Pts',(-10.2659967002315,12.2,-3.43679025568135));
#272643=CARTESIAN_POINT('Ctrl Pts',(-10.268929377159,12.2,-3.43890555823157));
#272644=CARTESIAN_POINT('Ctrl Pts',(-10.2718710773958,12.2,-3.44103488317619));
#272645=CARTESIAN_POINT('Ctrl Pts',(-10.2748216555426,12.2,-3.4431782376662));
#272646=CARTESIAN_POINT('Ctrl Pts',(-10.2777722340914,12.2,-3.44532159244823));
#272647=CARTESIAN_POINT('Ctrl Pts',(-10.2807316885656,12.2,-3.4474789746704));
#272648=CARTESIAN_POINT('Ctrl Pts',(-10.2836998765187,12.2,-3.44965039274311));
#272649=CARTESIAN_POINT('Ctrl Pts',(-10.2866680640674,12.2,-3.45182181051995));
#272650=CARTESIAN_POINT('Ctrl Pts',(-10.2896449826096,12.2,-3.45400726117158));
#272651=CARTESIAN_POINT('Ctrl Pts',(-10.2926304907536,12.2,-3.45620675165702));
#272652=CARTESIAN_POINT('Ctrl Pts',(-10.2956159993043,12.2,-3.45840624244214));
#272653=CARTESIAN_POINT('Ctrl Pts',(-10.2986100954281,12.2,-3.46061977055912));
#272654=CARTESIAN_POINT('Ctrl Pts',(-10.3016126387584,12.2,-3.46284734329163));
#272655=CARTESIAN_POINT('Ctrl Pts',(-10.3046151820887,12.2,-3.46507491602413));
#272656=CARTESIAN_POINT('Ctrl Pts',(-10.3076261720144,12.2,-3.46731653206384));
#272657=CARTESIAN_POINT('Ctrl Pts',(-10.3106454662354,12.2,-3.46957219491044));
#272658=CARTESIAN_POINT('Ctrl Pts',(-10.3136647600449,12.2,-3.4718278574497));
#272659=CARTESIAN_POINT('Ctrl Pts',(-10.3166923608546,12.2,-3.47409756675812));
#272660=CARTESIAN_POINT('Ctrl Pts',(-10.3197281277313,12.2,-3.47638132724841));
#272661=CARTESIAN_POINT('Ctrl Pts',(-10.3227638950216,12.2,-3.47866508804986));
#272662=CARTESIAN_POINT('Ctrl Pts',(-10.3258078280596,12.2,-3.48096289886718));
#272663=CARTESIAN_POINT('Ctrl Pts',(-10.3288597887824,12.2,-3.48327476366129));
#272664=CARTESIAN_POINT('Ctrl Pts',(-10.3319117490892,12.2,-3.4855866281404));
#272665=CARTESIAN_POINT('Ctrl Pts',(-10.3349717375812,12.2,-3.48791254575102));
#272666=CARTESIAN_POINT('Ctrl Pts',(-10.3380396172743,12.2,-3.4902525195588));
#272667=CARTESIAN_POINT('Ctrl Pts',(-10.3411074973854,12.2,-3.49259249368541));
#272668=CARTESIAN_POINT('Ctrl Pts',(-10.3441832677497,12.2,-3.49494652403118));
#272669=CARTESIAN_POINT('Ctrl Pts',(-10.3472667952392,12.2,-3.49731461233533));
#272670=CARTESIAN_POINT('Ctrl Pts',(-10.3503503223085,12.2,-3.49968270031683));
#272671=CARTESIAN_POINT('Ctrl Pts',(-10.3534416034951,12.2,-3.50206484678435));
#272672=CARTESIAN_POINT('Ctrl Pts',(-10.3565405064634,12.2,-3.50446105258753));
#272673=CARTESIAN_POINT('Ctrl Pts',(-10.359639409854,12.2,-3.5068572587172));
#272674=CARTESIAN_POINT('Ctrl Pts',(-10.3627459347984,12.2,-3.50926752496524));
#272675=CARTESIAN_POINT('Ctrl Pts',(-10.3658599482463,12.2,-3.51169185243161));
#272676=CARTESIAN_POINT('Ctrl Pts',(-10.36897396127,12.2,-3.51411617956767));
#272677=CARTESIAN_POINT('Ctrl Pts',(-10.3720954612795,12.2,-3.51655456731226));
#272678=CARTESIAN_POINT('Ctrl Pts',(-10.3752243185127,12.2,-3.51900701734417));
#272679=CARTESIAN_POINT('Ctrl Pts',(-10.3783531761722,12.2,-3.52145946771024));
#272680=CARTESIAN_POINT('Ctrl Pts',(-10.3814893904686,12.2,-3.52392598138622));
#272681=CARTESIAN_POINT('Ctrl Pts',(-10.3846328299737,12.2,-3.52640655624455));
#272682=CARTESIAN_POINT('Ctrl Pts',(-10.3877762690506,12.2,-3.5288871307649));
#272683=CARTESIAN_POINT('Ctrl Pts',(-10.3909269338926,12.2,-3.53138176717965));
#272684=CARTESIAN_POINT('Ctrl Pts',(-10.3940846949671,12.2,-3.53389046630646));
#272685=CARTESIAN_POINT('Ctrl Pts',(-10.3972424564718,12.2,-3.53639916577509));
#272686=CARTESIAN_POINT('Ctrl Pts',(-10.4004073145271,12.2,-3.53892192834503));
#272687=CARTESIAN_POINT('Ctrl Pts',(-10.4035791400333,12.2,-3.54145875248328));
#272688=CARTESIAN_POINT('Ctrl Pts',(-10.4067509655395,12.2,-3.54399557662153));
#272689=CARTESIAN_POINT('Ctrl Pts',(-10.4099297599355,12.2,-3.54654646340589));
#272690=CARTESIAN_POINT('Ctrl Pts',(-10.4131153935542,12.2,-3.549111411436));
#272691=CARTESIAN_POINT('Ctrl Pts',(-10.4163010267389,12.2,-3.55167635911664));
#272692=CARTESIAN_POINT('Ctrl Pts',(-10.4194935014115,12.2,-3.55425536688178));
#272693=CARTESIAN_POINT('Ctrl Pts',(-10.4226926904979,12.2,-3.55684843601486));
#272694=CARTESIAN_POINT('Ctrl Pts',(-10.42589188002,12.2,-3.55944150550125));
#272695=CARTESIAN_POINT('Ctrl Pts',(-10.4290977844856,12.2,-3.56204863494535));
#272696=CARTESIAN_POINT('Ctrl Pts',(-10.4323102780503,12.2,-3.5646698236452));
#272697=CARTESIAN_POINT('Ctrl Pts',(-10.4355227711772,12.2,-3.56729101198792));
#272698=CARTESIAN_POINT('Ctrl Pts',(-10.4387418535672,12.2,-3.56992625780935));
#272699=CARTESIAN_POINT('Ctrl Pts',(-10.4419674019697,12.2,-3.57257556209185));
#272700=CARTESIAN_POINT('Ctrl Pts',(-10.4459993378026,12.2,-3.5758871927157));
#272701=CARTESIAN_POINT('Ctrl Pts',(-10.450041376835,12.2,-3.5792207847774));
#272702=CARTESIAN_POINT('Ctrl Pts',(-10.4540932777562,12.2,-3.58257633805647));
#272703=CARTESIAN_POINT('Ctrl Pts',(-10.4573347986697,12.2,-3.58526078082602));
#272704=CARTESIAN_POINT('Ctrl Pts',(-10.4605826327263,12.2,-3.58795927716365));
#272705=CARTESIAN_POINT('Ctrl Pts',(-10.4638366570154,12.2,-3.5906718247018));
#272706=CARTESIAN_POINT('Ctrl Pts',(-10.4670906808611,12.2,-3.59338437187037));
#272707=CARTESIAN_POINT('Ctrl Pts',(-10.4703508946366,12.2,-3.59611097056212));
#272708=CARTESIAN_POINT('Ctrl Pts',(-10.4736171797581,12.2,-3.59885161755938));
#272709=CARTESIAN_POINT('Ctrl Pts',(-10.4768834653246,12.2,-3.60159226493005));
#272710=CARTESIAN_POINT('Ctrl Pts',(-10.4801558212383,12.2,-3.60434695969191));
#272711=CARTESIAN_POINT('Ctrl Pts',(-10.4834341276924,12.2,-3.60711570059347));
#272712=CARTESIAN_POINT('Ctrl Pts',(-10.4867124336999,12.2,-3.60988444111779));
#272713=CARTESIAN_POINT('Ctrl Pts',(-10.4899966905866,12.2,-3.61266722592879));
#272714=CARTESIAN_POINT('Ctrl Pts',(-10.4932867797061,12.2,-3.61546405225478));
#272715=CARTESIAN_POINT('Ctrl Pts',(-10.4965768692739,12.2,-3.61826087896184));
#272716=CARTESIAN_POINT('Ctrl Pts',(-10.4998727905591,12.2,-3.62107174573727));
#272717=CARTESIAN_POINT('Ctrl Pts',(-10.5031744274617,12.2,-3.6238966504477));
#272718=CARTESIAN_POINT('Ctrl Pts',(-10.5064760639143,12.2,-3.62672155477323));
#272719=CARTESIAN_POINT('Ctrl Pts',(-10.509783414714,12.2,-3.62956049639464));
#272720=CARTESIAN_POINT('Ctrl Pts',(-10.5130963640527,12.2,-3.63241347030272));
#272721=CARTESIAN_POINT('Ctrl Pts',(-10.5164093138427,12.2,-3.63526644459952));
#272722=CARTESIAN_POINT('Ctrl Pts',(-10.5197278608097,12.2,-3.6381334514749));
#272723=CARTESIAN_POINT('Ctrl Pts',(-10.5230518917135,12.2,-3.64101448624395));
#272724=CARTESIAN_POINT('Ctrl Pts',(-10.5263759221644,12.2,-3.64389552062046));
#272725=CARTESIAN_POINT('Ctrl Pts',(-10.529705433814,12.2,-3.64679058244413));
#272726=CARTESIAN_POINT('Ctrl Pts',(-10.5330403149298,12.2,-3.64969966748266));
#272727=CARTESIAN_POINT('Ctrl Pts',(-10.5363751964999,12.2,-3.65260875291756));
#272728=CARTESIAN_POINT('Ctrl Pts',(-10.5397154450937,12.2,-3.65553186073961));
#272729=CARTESIAN_POINT('Ctrl Pts',(-10.5430609487356,12.2,-3.65846898680196));
#272730=CARTESIAN_POINT('Ctrl Pts',(-10.5464064519218,12.2,-3.66140611246413));
#272731=CARTESIAN_POINT('Ctrl Pts',(-10.5497572096734,12.2,-3.66435725527011));
#272732=CARTESIAN_POINT('Ctrl Pts',(-10.5531131076764,12.2,-3.66732240958183));
#272733=CARTESIAN_POINT('Ctrl Pts',(-10.5556300317501,12.2,-3.66954627582063));
#272734=CARTESIAN_POINT('Ctrl Pts',(-10.5581498485163,12.2,-3.67177802294497));
#272735=CARTESIAN_POINT('Ctrl Pts',(-10.5606725100083,12.2,-3.67401764972988));
#272736=CARTESIAN_POINT('Ctrl Pts',(-10.5631951710421,12.2,-3.67625727610791));
#272737=CARTESIAN_POINT('Ctrl Pts',(-10.5657206770006,12.2,-3.67850478189387));
#272738=CARTESIAN_POINT('Ctrl Pts',(-10.568248980534,12.2,-3.68076016377093));
#272739=CARTESIAN_POINT('Ctrl Pts',(-10.5707772840674,12.2,-3.68301554564799));
#272740=CARTESIAN_POINT('Ctrl Pts',(-10.5733083851495,12.2,-3.68527880414086));
#272741=CARTESIAN_POINT('Ctrl Pts',(-10.5758422377357,12.2,-3.68754993602703));
#272742=CARTESIAN_POINT('Ctrl Pts',(-10.5783760903218,12.2,-3.68982106791319));
#272743=CARTESIAN_POINT('Ctrl Pts',(-10.5809126948451,12.2,-3.69210007368729));
#272744=CARTESIAN_POINT('Ctrl Pts',(-10.5834520029727,12.2,-3.69438695053122));
#272745=CARTESIAN_POINT('Ctrl Pts',(-10.5859913111003,12.2,-3.69667382737515));
#272746=CARTESIAN_POINT('Ctrl Pts',(-10.5885333245821,12.2,-3.69896857428344));
#272747=CARTESIAN_POINT('Ctrl Pts',(-10.5910779957394,12.2,-3.70127118924078));
#272748=CARTESIAN_POINT('Ctrl Pts',(-10.5936226668967,12.2,-3.70357380419811));
#272749=CARTESIAN_POINT('Ctrl Pts',(-10.5961699975372,12.2,-3.70588428831321));
#272750=CARTESIAN_POINT('Ctrl Pts',(-10.5987199401525,12.2,-3.70820263668624));
#272751=CARTESIAN_POINT('Ctrl Pts',(-10.6012698832311,12.2,-3.71052098548043));
#272752=CARTESIAN_POINT('Ctrl Pts',(-10.6038224389687,12.2,-3.71284719905183));
#272753=CARTESIAN_POINT('Ctrl Pts',(-10.6063775615487,12.2,-3.71518127476713));
#272754=CARTESIAN_POINT('Ctrl Pts',(-10.6089326836646,12.2,-3.7175153500584));
#272755=CARTESIAN_POINT('Ctrl Pts',(-10.6114903742769,12.2,-3.7198572866884));
#272756=CARTESIAN_POINT('Ctrl Pts',(-10.6140505855204,12.2,-3.72220708222133));
#272757=CARTESIAN_POINT('Ctrl Pts',(-10.6166107967639,12.2,-3.72455687775426));
#272758=CARTESIAN_POINT('Ctrl Pts',(-10.6191735296894,12.2,-3.7269145330432));
#272759=CARTESIAN_POINT('Ctrl Pts',(-10.6217387388047,12.2,-3.7292800424996));
#272760=CARTESIAN_POINT('Ctrl Pts',(-10.62430394792,12.2,-3.73164555195599));
#272761=CARTESIAN_POINT('Ctrl Pts',(-10.6268716330934,12.2,-3.73401891763647));
#272762=CARTESIAN_POINT('Ctrl Pts',(-10.6294417507084,12.2,-3.73640013450829));
#272763=CARTESIAN_POINT('Ctrl Pts',(-10.6320118683233,12.2,-3.73878135138012));
#272764=CARTESIAN_POINT('Ctrl Pts',(-10.6345844185798,12.2,-3.7411704204766));
#272765=CARTESIAN_POINT('Ctrl Pts',(-10.6371593546944,12.2,-3.74356733830549));
#272766=CARTESIAN_POINT('Ctrl Pts',(-10.639734290809,12.2,-3.74596425613438));
#272767=CARTESIAN_POINT('Ctrl Pts',(-10.6423116140828,12.2,-3.74836902200129));
#272768=CARTESIAN_POINT('Ctrl Pts',(-10.6448912807843,12.2,-3.75078163303326));
#272769=CARTESIAN_POINT('Ctrl Pts',(-10.6474709474858,12.2,-3.75319424406522));
#272770=CARTESIAN_POINT('Ctrl Pts',(-10.6500529570142,12.2,-3.75561470062656));
#272771=CARTESIAN_POINT('Ctrl Pts',(-10.65263726467,12.2,-3.75804299845393));
#272772=CARTESIAN_POINT('Ctrl Pts',(-10.6552215727953,12.2,-3.76047129672244));
#272773=CARTESIAN_POINT('Ctrl Pts',(-10.6578081802379,12.2,-3.7629074357765));
#272774=CARTESIAN_POINT('Ctrl Pts',(-10.6603970423227,12.2,-3.76535141300775));
#272775=CARTESIAN_POINT('Ctrl Pts',(-10.6638488576521,12.2,-3.76861004857612));
#272776=CARTESIAN_POINT('Ctrl Pts',(-10.6673046810753,12.2,-3.77188261644268));
#272777=CARTESIAN_POINT('Ctrl Pts',(-10.6707644109589,12.2,-3.77516911000642));
#272778=CARTESIAN_POINT('Ctrl Pts',(-10.6733592084894,12.2,-3.77763398029118));
#272779=CARTESIAN_POINT('Ctrl Pts',(-10.6759562027948,12.2,-3.78010668256707));
#272780=CARTESIAN_POINT('Ctrl Pts',(-10.6785553499918,12.2,-3.78258721343421));
#272781=CARTESIAN_POINT('Ctrl Pts',(-10.6811544976609,12.2,-3.78506774475199));
#272782=CARTESIAN_POINT('Ctrl Pts',(-10.6837558001723,12.2,-3.78755610499696));
#272783=CARTESIAN_POINT('Ctrl Pts',(-10.6863592123009,12.2,-3.79005228977747));
#272784=CARTESIAN_POINT('Ctrl Pts',(-10.6906982314118,12.2,-3.79421259668688));
#272785=CARTESIAN_POINT('Ctrl Pts',(-10.6950431128834,12.2,-3.79839463823787));
#272786=CARTESIAN_POINT('Ctrl Pts',(-10.6993936594227,12.2,-3.80259839666678));
#272787=CARTESIAN_POINT('Ctrl Pts',(-10.7020039880101,12.2,-3.80512065236562));
#272788=CARTESIAN_POINT('Ctrl Pts',(-10.7046163564398,12.2,-3.80765072506667));
#272789=CARTESIAN_POINT('Ctrl Pts',(-10.7072307211116,12.2,-3.81018861181157));
#272790=CARTESIAN_POINT('Ctrl Pts',(-10.7098450853086,12.2,-3.81272649809541));
#272791=CARTESIAN_POINT('Ctrl Pts',(-10.7124614470638,12.2,-3.81527219763719));
#272792=CARTESIAN_POINT('Ctrl Pts',(-10.7150797632605,12.2,-3.81782570600342));
#272793=CARTESIAN_POINT('Ctrl Pts',(-10.7176980794572,12.2,-3.82037921436965));
#272794=CARTESIAN_POINT('Ctrl Pts',(-10.7203183505024,12.2,-3.82294053218393));
#272795=CARTESIAN_POINT('Ctrl Pts',(-10.7229405342108,12.2,-3.8255096549773));
#272796=CARTESIAN_POINT('Ctrl Pts',(-10.7255627179191,12.2,-3.82807877777066));
#272797=CARTESIAN_POINT('Ctrl Pts',(-10.7281868155311,12.2,-3.83065570521315));
#272798=CARTESIAN_POINT('Ctrl Pts',(-10.7308127831977,12.2,-3.83324043300595));
#272799=CARTESIAN_POINT('Ctrl Pts',(-10.7334387508642,12.2,-3.83582516079875));
#272800=CARTESIAN_POINT('Ctrl Pts',(-10.7360665893591,12.2,-3.83841768861181));
#272801=CARTESIAN_POINT('Ctrl Pts',(-10.7386962579301,12.2,-3.84101801197499));
#272802=CARTESIAN_POINT('Ctrl Pts',(-10.7413259265011,12.2,-3.84361833533817));
#272803=CARTESIAN_POINT('Ctrl Pts',(-10.7439574243052,12.2,-3.84622645534246));
#272804=CARTESIAN_POINT('Ctrl Pts',(-10.7465907114593,12.2,-3.8488423657047));
#272805=CARTESIAN_POINT('Ctrl Pts',(-10.7492239990918,12.2,-3.85145827654216));
#272806=CARTESIAN_POINT('Ctrl Pts',(-10.7518590766748,12.2,-3.8540819787568));
#272807=CARTESIAN_POINT('Ctrl Pts',(-10.7544959008082,12.2,-3.85671346709864));
#272808=CARTESIAN_POINT('Ctrl Pts',(-10.7580116655211,12.2,-3.86022211742433));
#272809=CARTESIAN_POINT('Ctrl Pts',(-10.7615305356029,12.2,-3.86374461051231));
#272810=CARTESIAN_POINT('Ctrl Pts',(-10.7650524129976,12.2,-3.86728093473922));
#272811=CARTESIAN_POINT('Ctrl Pts',(-10.7676938211637,12.2,-3.86993317802987));
#272812=CARTESIAN_POINT('Ctrl Pts',(-10.770336920208,12.2,-3.87259320084024));
#272813=CARTESIAN_POINT('Ctrl Pts',(-10.7729816739035,12.2,-3.87526099870097));
#272814=CARTESIAN_POINT('Ctrl Pts',(-10.7756264275989,12.2,-3.87792879656169));
#272815=CARTESIAN_POINT('Ctrl Pts',(-10.7782728361025,12.2,-3.88060437059689));
#272816=CARTESIAN_POINT('Ctrl Pts',(-10.7809208606728,12.2,-3.883287714415));
#272817=CARTESIAN_POINT('Ctrl Pts',(-10.7835688857241,12.2,-3.88597105872058));
#272818=CARTESIAN_POINT('Ctrl Pts',(-10.7862185270425,12.2,-3.88866217361171));
#272819=CARTESIAN_POINT('Ctrl Pts',(-10.7888697345947,12.2,-3.89136105337999));
#272820=CARTESIAN_POINT('Ctrl Pts',(-10.7915209416652,12.2,-3.89405993265798));
#272821=CARTESIAN_POINT('Ctrl Pts',(-10.7941737152272,12.2,-3.89676657630398));
#272822=CARTESIAN_POINT('Ctrl Pts',(-10.7968280103053,12.2,-3.89948097875854));
#272823=CARTESIAN_POINT('Ctrl Pts',(-10.7994823053833,12.2,-3.9021953812131));
#272824=CARTESIAN_POINT('Ctrl Pts',(-10.802138123266,12.2,-3.9049175422178));
#272825=CARTESIAN_POINT('Ctrl Pts',(-10.8047954455073,12.2,-3.90764745961308));
#272826=CARTESIAN_POINT('Ctrl Pts',(-10.8074527677486,12.2,-3.91037737700835));
#272827=CARTESIAN_POINT('Ctrl Pts',(-10.8101115924531,12.2,-3.91311505550024));
#272828=CARTESIAN_POINT('Ctrl Pts',(-10.8127719255158,12.2,-3.91586047850026));
#272829=CARTESIAN_POINT('Origin',(-5.66257110645729E-14,15.2,-1.77635683940025E-14));
#272830=CARTESIAN_POINT('',(-9.31239140042914,15.2,-4.57383771138038));
#272831=CARTESIAN_POINT('',(-9.31239140042914,12.2,-4.57383771138038));
#272832=CARTESIAN_POINT('',(-9.31239140000006,15.2,-4.57383771100002));
#272833=CARTESIAN_POINT('Origin',(-5.66257110645729E-14,12.2,-1.77635683940025E-14));
#272834=CARTESIAN_POINT('Origin',(-5.66257110645729E-14,15.2,-1.77635683940025E-14));
#272835=CARTESIAN_POINT('Origin',(-5.66257110645729E-14,15.2,-1.77635683940025E-14));
#272836=CARTESIAN_POINT('',(-10.1454284470001,15.2,-5.41482055400001));
#272837=CARTESIAN_POINT('',(-9.95917514600006,15.2,-5.75020264100001));
#272838=CARTESIAN_POINT('Origin',(-5.66257110645729E-14,15.2,-1.77635683940025E-14));
#272839=CARTESIAN_POINT('',(-9.95917514600006,12.2,-5.75020264100001));
#272840=CARTESIAN_POINT('',(-9.95917514600006,15.2,-5.75020264100001));
#272841=CARTESIAN_POINT('',(-10.1454284470001,12.2,-5.41482055400001));
#272842=CARTESIAN_POINT('Origin',(-5.66257110645729E-14,12.2,-1.77635683940025E-14));
#272843=CARTESIAN_POINT('',(-10.1454284470001,15.2,-5.41482055400001));
#272844=CARTESIAN_POINT('Ctrl Pts',(-9.31239140100006,15.2,-4.57383771200002));
#272845=CARTESIAN_POINT('Ctrl Pts',(-9.31239140100006,11.6,-4.57383771200002));
#272846=CARTESIAN_POINT('Ctrl Pts',(-9.31254071700006,15.2,-4.57392774200001));
#272847=CARTESIAN_POINT('Ctrl Pts',(-9.31254071700006,11.6,-4.57392774200002));
#272848=CARTESIAN_POINT('Ctrl Pts',(-9.31284451800006,15.2,-4.57411102300001));
#272849=CARTESIAN_POINT('Ctrl Pts',(-9.31284451800006,11.6,-4.57411102300001));
#272850=CARTESIAN_POINT('Ctrl Pts',(-9.31330471300006,15.2,-4.57438896200001));
#272851=CARTESIAN_POINT('Ctrl Pts',(-9.31330471300006,11.6,-4.57438896200001));
#272852=CARTESIAN_POINT('Ctrl Pts',(-9.31392435800005,15.2,-4.57476383600001));
#272853=CARTESIAN_POINT('Ctrl Pts',(-9.31392435800005,11.6,-4.57476383600001));
#272854=CARTESIAN_POINT('Ctrl Pts',(-9.31470764300006,15.2,-4.57523877600002));
#272855=CARTESIAN_POINT('Ctrl Pts',(-9.31470764300006,11.6,-4.57523877600002));
#272856=CARTESIAN_POINT('Ctrl Pts',(-9.31550313900006,15.2,-4.57572221300001));
#272857=CARTESIAN_POINT('Ctrl Pts',(-9.31550313900006,11.6,-4.57572221300001));
#272858=CARTESIAN_POINT('Ctrl Pts',(-9.31630627600006,15.2,-4.57621139800001));
#272859=CARTESIAN_POINT('Ctrl Pts',(-9.31630627600006,11.6,-4.57621139800001));
#272860=CARTESIAN_POINT('Ctrl Pts',(-9.31711702100005,15.2,-4.57670633100001));
#272861=CARTESIAN_POINT('Ctrl Pts',(-9.31711702100005,11.6,-4.57670633100001));
#272862=CARTESIAN_POINT('Ctrl Pts',(-9.31793534100006,15.2,-4.57720701200001));
#272863=CARTESIAN_POINT('Ctrl Pts',(-9.31793534100006,11.6,-4.57720701200001));
#272864=CARTESIAN_POINT('Ctrl Pts',(-9.31876120500006,15.2,-4.57771344700001));
#272865=CARTESIAN_POINT('Ctrl Pts',(-9.31876120500006,11.6,-4.57771344700001));
#272866=CARTESIAN_POINT('Ctrl Pts',(-9.31959457900006,15.2,-4.57822563400001));
#272867=CARTESIAN_POINT('Ctrl Pts',(-9.31959457900006,11.6,-4.57822563400002));
#272868=CARTESIAN_POINT('Ctrl Pts',(-9.32043543400006,15.2,-4.57874357400001));
#272869=CARTESIAN_POINT('Ctrl Pts',(-9.32043543400006,11.6,-4.57874357400002));
#272870=CARTESIAN_POINT('Ctrl Pts',(-9.32128373600005,15.2,-4.57926727100002));
#272871=CARTESIAN_POINT('Ctrl Pts',(-9.32128373600005,11.6,-4.57926727100002));
#272872=CARTESIAN_POINT('Ctrl Pts',(-9.32213945400006,15.2,-4.57979672400001));
#272873=CARTESIAN_POINT('Ctrl Pts',(-9.32213945400006,11.6,-4.57979672400001));
#272874=CARTESIAN_POINT('Ctrl Pts',(-9.32300255700006,15.2,-4.58033193400002));
#272875=CARTESIAN_POINT('Ctrl Pts',(-9.32300255700006,11.6,-4.58033193400002));
#272876=CARTESIAN_POINT('Ctrl Pts',(-9.32387301400006,15.2,-4.58087290600002));
#272877=CARTESIAN_POINT('Ctrl Pts',(-9.32387301400006,11.6,-4.58087290600002));
#272878=CARTESIAN_POINT('Ctrl Pts',(-9.32475079300006,15.2,-4.58141963700001));
#272879=CARTESIAN_POINT('Ctrl Pts',(-9.32475079300006,11.6,-4.58141963700002));
#272880=CARTESIAN_POINT('Ctrl Pts',(-9.32563586400006,15.2,-4.58197212900001));
#272881=CARTESIAN_POINT('Ctrl Pts',(-9.32563586400006,11.6,-4.58197212900001));
#272882=CARTESIAN_POINT('Ctrl Pts',(-9.32652819500005,15.2,-4.58253038500001));
#272883=CARTESIAN_POINT('Ctrl Pts',(-9.32652819500005,11.6,-4.58253038500002));
#272884=CARTESIAN_POINT('Ctrl Pts',(-9.32742775700006,15.2,-4.58309440600001));
#272885=CARTESIAN_POINT('Ctrl Pts',(-9.32742775700006,11.6,-4.58309440600001));
#272886=CARTESIAN_POINT('Ctrl Pts',(-9.32833451800006,15.2,-4.58366419300001));
#272887=CARTESIAN_POINT('Ctrl Pts',(-9.32833451800006,11.6,-4.58366419300001));
#272888=CARTESIAN_POINT('Ctrl Pts',(-9.32924844800005,15.2,-4.58423974600001));
#272889=CARTESIAN_POINT('Ctrl Pts',(-9.32924844800005,11.6,-4.58423974600001));
#272890=CARTESIAN_POINT('Ctrl Pts',(-9.33016951800006,15.2,-4.58482106700002));
#272891=CARTESIAN_POINT('Ctrl Pts',(-9.33016951800006,11.6,-4.58482106700002));
#272892=CARTESIAN_POINT('Ctrl Pts',(-9.33109769500006,15.2,-4.58540815700001));
#272893=CARTESIAN_POINT('Ctrl Pts',(-9.33109769500006,11.6,-4.58540815700002));
#272894=CARTESIAN_POINT('Ctrl Pts',(-9.33203295300006,15.2,-4.58600101800001));
#272895=CARTESIAN_POINT('Ctrl Pts',(-9.33203295300006,11.6,-4.58600101800002));
#272896=CARTESIAN_POINT('Ctrl Pts',(-9.33297525900005,15.2,-4.58659964900002));
#272897=CARTESIAN_POINT('Ctrl Pts',(-9.33297525900005,11.6,-4.58659964900002));
#272898=CARTESIAN_POINT('Ctrl Pts',(-9.33392458400006,15.2,-4.58720405300001));
#272899=CARTESIAN_POINT('Ctrl Pts',(-9.33392458400006,11.6,-4.58720405300001));
#272900=CARTESIAN_POINT('Ctrl Pts',(-9.33488090000005,15.2,-4.58781423000001));
#272901=CARTESIAN_POINT('Ctrl Pts',(-9.33488090000005,11.6,-4.58781423000001));
#272902=CARTESIAN_POINT('Ctrl Pts',(-9.33584417700006,15.2,-4.58843018200001));
#272903=CARTESIAN_POINT('Ctrl Pts',(-9.33584417700006,11.6,-4.58843018200001));
#272904=CARTESIAN_POINT('Ctrl Pts',(-9.33681438400006,15.2,-4.58905190900001));
#272905=CARTESIAN_POINT('Ctrl Pts',(-9.33681438400006,11.6,-4.58905190900001));
#272906=CARTESIAN_POINT('Ctrl Pts',(-9.33779149400005,15.2,-4.58967941300001));
#272907=CARTESIAN_POINT('Ctrl Pts',(-9.33779149400005,11.6,-4.58967941300001));
#272908=CARTESIAN_POINT('Ctrl Pts',(-9.33877547800006,15.2,-4.59031269400001));
#272909=CARTESIAN_POINT('Ctrl Pts',(-9.33877547800006,11.6,-4.59031269400001));
#272910=CARTESIAN_POINT('Ctrl Pts',(-9.33976630500006,15.2,-4.59095175300002));
#272911=CARTESIAN_POINT('Ctrl Pts',(-9.33976630500006,11.6,-4.59095175300002));
#272912=CARTESIAN_POINT('Ctrl Pts',(-9.34076394800006,15.2,-4.59159659300001));
#272913=CARTESIAN_POINT('Ctrl Pts',(-9.34076394800006,11.6,-4.59159659300001));
#272914=CARTESIAN_POINT('Ctrl Pts',(-9.34176837900005,15.2,-4.59224721100002));
#272915=CARTESIAN_POINT('Ctrl Pts',(-9.34176837900005,11.6,-4.59224721100002));
#272916=CARTESIAN_POINT('Ctrl Pts',(-9.34277956900005,15.2,-4.59290361300001));
#272917=CARTESIAN_POINT('Ctrl Pts',(-9.34277956900005,11.6,-4.59290361300001));
#272918=CARTESIAN_POINT('Ctrl Pts',(-9.34379748800006,15.2,-4.59356579500001));
#272919=CARTESIAN_POINT('Ctrl Pts',(-9.34379748800006,11.6,-4.59356579500002));
#272920=CARTESIAN_POINT('Ctrl Pts',(-9.34482211000006,15.2,-4.59423376000001));
#272921=CARTESIAN_POINT('Ctrl Pts',(-9.34482211000006,11.6,-4.59423376000002));
#272922=CARTESIAN_POINT('Ctrl Pts',(-9.34585340600006,15.2,-4.59490751000001));
#272923=CARTESIAN_POINT('Ctrl Pts',(-9.34585340600006,11.6,-4.59490751000002));
#272924=CARTESIAN_POINT('Ctrl Pts',(-9.34689134900006,15.2,-4.59558704400001));
#272925=CARTESIAN_POINT('Ctrl Pts',(-9.34689134900006,11.6,-4.59558704400001));
#272926=CARTESIAN_POINT('Ctrl Pts',(-9.34793590900006,15.2,-4.59627236300001));
#272927=CARTESIAN_POINT('Ctrl Pts',(-9.34793590900006,11.6,-4.59627236300001));
#272928=CARTESIAN_POINT('Ctrl Pts',(-9.34898706000006,15.2,-4.59696346900001));
#272929=CARTESIAN_POINT('Ctrl Pts',(-9.34898706000006,11.6,-4.59696346900001));
#272930=CARTESIAN_POINT('Ctrl Pts',(-9.35004477500006,15.2,-4.59766036300001));
#272931=CARTESIAN_POINT('Ctrl Pts',(-9.35004477500006,11.6,-4.59766036300001));
#272932=CARTESIAN_POINT('Ctrl Pts',(-9.35110902500006,15.2,-4.59836304300001));
#272933=CARTESIAN_POINT('Ctrl Pts',(-9.35110902500006,11.6,-4.59836304300001));
#272934=CARTESIAN_POINT('Ctrl Pts',(-9.35217978400006,15.2,-4.59907151300001));
#272935=CARTESIAN_POINT('Ctrl Pts',(-9.35217978400006,11.6,-4.59907151300001));
#272936=CARTESIAN_POINT('Ctrl Pts',(-9.35325702300006,15.2,-4.59978577200001));
#272937=CARTESIAN_POINT('Ctrl Pts',(-9.35325702300006,11.6,-4.59978577200001));
#272938=CARTESIAN_POINT('Ctrl Pts',(-9.35434071700006,15.2,-4.60050582100001));
#272939=CARTESIAN_POINT('Ctrl Pts',(-9.35434071700006,11.6,-4.60050582100001));
#272940=CARTESIAN_POINT('Ctrl Pts',(-9.35543083700006,15.2,-4.60123166100002));
#272941=CARTESIAN_POINT('Ctrl Pts',(-9.35543083700006,11.6,-4.60123166100002));
#272942=CARTESIAN_POINT('Ctrl Pts',(-9.35652735900005,15.2,-4.60196329200001));
#272943=CARTESIAN_POINT('Ctrl Pts',(-9.35652735900005,11.6,-4.60196329200001));
#272944=CARTESIAN_POINT('Ctrl Pts',(-9.35763025400006,15.2,-4.60270071600001));
#272945=CARTESIAN_POINT('Ctrl Pts',(-9.35763025400006,11.6,-4.60270071600002));
#272946=CARTESIAN_POINT('Ctrl Pts',(-9.35873949500006,15.2,-4.60344393200002));
#272947=CARTESIAN_POINT('Ctrl Pts',(-9.35873949500006,11.6,-4.60344393200002));
#272948=CARTESIAN_POINT('Ctrl Pts',(-9.35985505600006,15.2,-4.60419294200001));
#272949=CARTESIAN_POINT('Ctrl Pts',(-9.35985505600006,11.6,-4.60419294200001));
#272950=CARTESIAN_POINT('Ctrl Pts',(-9.36097691300006,15.2,-4.60494774600001));
#272951=CARTESIAN_POINT('Ctrl Pts',(-9.36097691300006,11.6,-4.60494774600001));
#272952=CARTESIAN_POINT('Ctrl Pts',(-9.36210503700006,15.2,-4.60570834500002));
#272953=CARTESIAN_POINT('Ctrl Pts',(-9.36210503700006,11.6,-4.60570834500002));
#272954=CARTESIAN_POINT('Ctrl Pts',(-9.36323940100005,15.2,-4.60647473800002));
#272955=CARTESIAN_POINT('Ctrl Pts',(-9.36323940100005,11.6,-4.60647473800002));
#272956=CARTESIAN_POINT('Ctrl Pts',(-9.36437998200006,15.2,-4.60724692800001));
#272957=CARTESIAN_POINT('Ctrl Pts',(-9.36437998200006,11.6,-4.60724692800001));
#272958=CARTESIAN_POINT('Ctrl Pts',(-9.36552675200006,15.2,-4.60802491300001));
#272959=CARTESIAN_POINT('Ctrl Pts',(-9.36552675200006,11.6,-4.60802491300001));
#272960=CARTESIAN_POINT('Ctrl Pts',(-9.36667968600006,15.2,-4.60880869700001));
#272961=CARTESIAN_POINT('Ctrl Pts',(-9.36667968600006,11.6,-4.60880869700001));
#272962=CARTESIAN_POINT('Ctrl Pts',(-9.36783875800005,15.2,-4.60959827800002));
#272963=CARTESIAN_POINT('Ctrl Pts',(-9.36783875800005,11.6,-4.60959827800002));
#272964=CARTESIAN_POINT('Ctrl Pts',(-9.36900394300006,15.2,-4.61039365500001));
#272965=CARTESIAN_POINT('Ctrl Pts',(-9.36900394300006,11.6,-4.61039365500001));
#272966=CARTESIAN_POINT('Ctrl Pts',(-9.37017521400006,15.2,-4.61119483300001));
#272967=CARTESIAN_POINT('Ctrl Pts',(-9.37017521400006,11.6,-4.61119483300001));
#272968=CARTESIAN_POINT('Ctrl Pts',(-9.37135254700006,15.2,-4.61200180900001));
#272969=CARTESIAN_POINT('Ctrl Pts',(-9.37135254700006,11.6,-4.61200180900002));
#272970=CARTESIAN_POINT('Ctrl Pts',(-9.37253591600006,15.2,-4.61281458400002));
#272971=CARTESIAN_POINT('Ctrl Pts',(-9.37253591600006,11.6,-4.61281458400002));
#272972=CARTESIAN_POINT('Ctrl Pts',(-9.37372529600006,15.2,-4.61363315900002));
#272973=CARTESIAN_POINT('Ctrl Pts',(-9.37372529600006,11.6,-4.61363315900002));
#272974=CARTESIAN_POINT('Ctrl Pts',(-9.37492066200006,15.2,-4.61445753500001));
#272975=CARTESIAN_POINT('Ctrl Pts',(-9.37492066200006,11.6,-4.61445753500001));
#272976=CARTESIAN_POINT('Ctrl Pts',(-9.37612198900006,15.2,-4.61528771100001));
#272977=CARTESIAN_POINT('Ctrl Pts',(-9.37612198900006,11.6,-4.61528771100001));
#272978=CARTESIAN_POINT('Ctrl Pts',(-9.37732925200006,15.2,-4.61612368800001));
#272979=CARTESIAN_POINT('Ctrl Pts',(-9.37732925200006,11.6,-4.61612368800001));
#272980=CARTESIAN_POINT('Ctrl Pts',(-9.37854242600006,15.2,-4.61696546600002));
#272981=CARTESIAN_POINT('Ctrl Pts',(-9.37854242600006,11.6,-4.61696546600002));
#272982=CARTESIAN_POINT('Ctrl Pts',(-9.37976148700006,15.2,-4.61781304700001));
#272983=CARTESIAN_POINT('Ctrl Pts',(-9.37976148700006,11.6,-4.61781304700002));
#272984=CARTESIAN_POINT('Ctrl Pts',(-9.38098641000006,15.2,-4.61866643000001));
#272985=CARTESIAN_POINT('Ctrl Pts',(-9.38098641000006,11.6,-4.61866643000001));
#272986=CARTESIAN_POINT('Ctrl Pts',(-9.38221717000006,15.2,-4.61952561600001));
#272987=CARTESIAN_POINT('Ctrl Pts',(-9.38221717000006,11.6,-4.61952561600001));
#272988=CARTESIAN_POINT('Ctrl Pts',(-9.38345374400006,15.2,-4.62039060400001));
#272989=CARTESIAN_POINT('Ctrl Pts',(-9.38345374400006,11.6,-4.62039060400001));
#272990=CARTESIAN_POINT('Ctrl Pts',(-9.38469610600006,15.2,-4.62126139500001));
#272991=CARTESIAN_POINT('Ctrl Pts',(-9.38469610600006,11.6,-4.62126139500001));
#272992=CARTESIAN_POINT('Ctrl Pts',(-9.38594423300006,15.2,-4.62213799100001));
#272993=CARTESIAN_POINT('Ctrl Pts',(-9.38594423300006,11.6,-4.62213799100002));
#272994=CARTESIAN_POINT('Ctrl Pts',(-9.38719810100006,15.2,-4.62302038900001));
#272995=CARTESIAN_POINT('Ctrl Pts',(-9.38719810100006,11.6,-4.62302038900001));
#272996=CARTESIAN_POINT('Ctrl Pts',(-9.38845768500006,15.2,-4.62390859300001));
#272997=CARTESIAN_POINT('Ctrl Pts',(-9.38845768500006,11.6,-4.62390859300002));
#272998=CARTESIAN_POINT('Ctrl Pts',(-9.38972296200006,15.2,-4.62480260000001));
#272999=CARTESIAN_POINT('Ctrl Pts',(-9.38972296200006,11.6,-4.62480260000001));
#273000=CARTESIAN_POINT('Ctrl Pts',(-9.39099390900006,15.2,-4.62570241200002));
#273001=CARTESIAN_POINT('Ctrl Pts',(-9.39099390900006,11.6,-4.62570241200002));
#273002=CARTESIAN_POINT('Ctrl Pts',(-9.39227050100006,15.2,-4.62660802900002));
#273003=CARTESIAN_POINT('Ctrl Pts',(-9.39227050100006,11.6,-4.62660802900002));
#273004=CARTESIAN_POINT('Ctrl Pts',(-9.39355271300006,15.2,-4.62751945000001));
#273005=CARTESIAN_POINT('Ctrl Pts',(-9.39355271300006,11.6,-4.62751945000001));
#273006=CARTESIAN_POINT('Ctrl Pts',(-9.39484052500006,15.2,-4.62843667700001));
#273007=CARTESIAN_POINT('Ctrl Pts',(-9.39484052500006,11.6,-4.62843667700001));
#273008=CARTESIAN_POINT('Ctrl Pts',(-9.39613391000006,15.2,-4.62935971000002));
#273009=CARTESIAN_POINT('Ctrl Pts',(-9.39613391000006,11.6,-4.62935971000002));
#273010=CARTESIAN_POINT('Ctrl Pts',(-9.39743284800005,15.2,-4.63028854700001));
#273011=CARTESIAN_POINT('Ctrl Pts',(-9.39743284800005,11.6,-4.63028854700002));
#273012=CARTESIAN_POINT('Ctrl Pts',(-9.39873731400005,15.2,-4.63122319200002));
#273013=CARTESIAN_POINT('Ctrl Pts',(-9.39873731400005,11.6,-4.63122319200002));
#273014=CARTESIAN_POINT('Ctrl Pts',(-9.40004728400006,15.2,-4.63216364100001));
#273015=CARTESIAN_POINT('Ctrl Pts',(-9.40004728400006,11.6,-4.63216364100001));
#273016=CARTESIAN_POINT('Ctrl Pts',(-9.40136273700006,15.2,-4.63310989700001));
#273017=CARTESIAN_POINT('Ctrl Pts',(-9.40136273700006,11.6,-4.63310989700001));
#273018=CARTESIAN_POINT('Ctrl Pts',(-9.40268364800006,15.2,-4.63406195800002));
#273019=CARTESIAN_POINT('Ctrl Pts',(-9.40268364800006,11.6,-4.63406195800002));
#273020=CARTESIAN_POINT('Ctrl Pts',(-9.40400999600006,15.2,-4.63501982600001));
#273021=CARTESIAN_POINT('Ctrl Pts',(-9.40400999600006,11.6,-4.63501982600001));
#273022=CARTESIAN_POINT('Ctrl Pts',(-9.40534175600006,15.2,-4.63598350100002));
#273023=CARTESIAN_POINT('Ctrl Pts',(-9.40534175600006,11.6,-4.63598350100002));
#273024=CARTESIAN_POINT('Ctrl Pts',(-9.40667890800006,15.2,-4.63695298200001));
#273025=CARTESIAN_POINT('Ctrl Pts',(-9.40667890800006,11.6,-4.63695298200001));
#273026=CARTESIAN_POINT('Ctrl Pts',(-9.40802142700005,15.2,-4.63792826900002));
#273027=CARTESIAN_POINT('Ctrl Pts',(-9.40802142700005,11.6,-4.63792826900002));
#273028=CARTESIAN_POINT('Ctrl Pts',(-9.40936929200006,15.2,-4.63890936200002));
#273029=CARTESIAN_POINT('Ctrl Pts',(-9.40936929200006,11.6,-4.63890936200002));
#273030=CARTESIAN_POINT('Ctrl Pts',(-9.41072247900006,15.2,-4.63989626300001));
#273031=CARTESIAN_POINT('Ctrl Pts',(-9.41072247900006,11.6,-4.63989626300001));
#273032=CARTESIAN_POINT('Ctrl Pts',(-9.41208096700005,15.2,-4.64088897000002));
#273033=CARTESIAN_POINT('Ctrl Pts',(-9.41208096700005,11.6,-4.64088897000002));
#273034=CARTESIAN_POINT('Ctrl Pts',(-9.41344473500006,15.2,-4.64188748400002));
#273035=CARTESIAN_POINT('Ctrl Pts',(-9.41344473500006,11.6,-4.64188748400002));
#273036=CARTESIAN_POINT('Ctrl Pts',(-9.41481375700005,15.2,-4.64289180400002));
#273037=CARTESIAN_POINT('Ctrl Pts',(-9.41481375700005,11.6,-4.64289180400002));
#273038=CARTESIAN_POINT('Ctrl Pts',(-9.41618801500006,15.2,-4.64390193100002));
#273039=CARTESIAN_POINT('Ctrl Pts',(-9.41618801500006,11.6,-4.64390193100002));
#273040=CARTESIAN_POINT('Ctrl Pts',(-9.41756748400006,15.2,-4.64491786400002));
#273041=CARTESIAN_POINT('Ctrl Pts',(-9.41756748400006,11.6,-4.64491786400002));
#273042=CARTESIAN_POINT('Ctrl Pts',(-9.41895214300006,15.2,-4.64593960400002));
#273043=CARTESIAN_POINT('Ctrl Pts',(-9.41895214300006,11.6,-4.64593960400002));
#273044=CARTESIAN_POINT('Ctrl Pts',(-9.42034197000006,15.2,-4.64696715000001));
#273045=CARTESIAN_POINT('Ctrl Pts',(-9.42034197000006,11.6,-4.64696715000002));
#273046=CARTESIAN_POINT('Ctrl Pts',(-9.42173694400006,15.2,-4.64800050400001));
#273047=CARTESIAN_POINT('Ctrl Pts',(-9.42173694400006,11.6,-4.64800050400001));
#273048=CARTESIAN_POINT('Ctrl Pts',(-9.42313704200006,15.2,-4.64903966200001));
#273049=CARTESIAN_POINT('Ctrl Pts',(-9.42313704200006,11.6,-4.64903966200001));
#273050=CARTESIAN_POINT('Ctrl Pts',(-9.42454224400005,15.2,-4.65008462800002));
#273051=CARTESIAN_POINT('Ctrl Pts',(-9.42454224400005,11.6,-4.65008462800002));
#273052=CARTESIAN_POINT('Ctrl Pts',(-9.42595252800006,15.2,-4.65113539900001));
#273053=CARTESIAN_POINT('Ctrl Pts',(-9.42595252800006,11.6,-4.65113539900001));
#273054=CARTESIAN_POINT('Ctrl Pts',(-9.42736787200005,15.2,-4.65219197700002));
#273055=CARTESIAN_POINT('Ctrl Pts',(-9.42736787200005,11.6,-4.65219197700002));
#273056=CARTESIAN_POINT('Ctrl Pts',(-9.42878825300006,15.2,-4.65325436100001));
#273057=CARTESIAN_POINT('Ctrl Pts',(-9.42878825300006,11.6,-4.65325436100002));
#273058=CARTESIAN_POINT('Ctrl Pts',(-9.43021365300006,15.2,-4.65432255000001));
#273059=CARTESIAN_POINT('Ctrl Pts',(-9.43021365300006,11.6,-4.65432255000001));
#273060=CARTESIAN_POINT('Ctrl Pts',(-9.43164405000006,15.2,-4.65539654500001));
#273061=CARTESIAN_POINT('Ctrl Pts',(-9.43164405000006,11.6,-4.65539654500002));
#273062=CARTESIAN_POINT('Ctrl Pts',(-9.43307942100006,15.2,-4.65647634500002));
#273063=CARTESIAN_POINT('Ctrl Pts',(-9.43307942100006,11.6,-4.65647634500002));
#273064=CARTESIAN_POINT('Ctrl Pts',(-9.43451974600006,15.2,-4.65756195100001));
#273065=CARTESIAN_POINT('Ctrl Pts',(-9.43451974600006,11.6,-4.65756195100001));
#273066=CARTESIAN_POINT('Ctrl Pts',(-9.43596500400006,15.2,-4.65865336200002));
#273067=CARTESIAN_POINT('Ctrl Pts',(-9.43596500400006,11.6,-4.65865336200002));
#273068=CARTESIAN_POINT('Ctrl Pts',(-9.43741517400005,15.2,-4.65975057700001));
#273069=CARTESIAN_POINT('Ctrl Pts',(-9.43741517400005,11.6,-4.65975057700002));
#273070=CARTESIAN_POINT('Ctrl Pts',(-9.43887023600006,15.2,-4.66085359800001));
#273071=CARTESIAN_POINT('Ctrl Pts',(-9.43887023600006,11.6,-4.66085359800002));
#273072=CARTESIAN_POINT('Ctrl Pts',(-9.44033016700006,15.2,-4.66196242300001));
#273073=CARTESIAN_POINT('Ctrl Pts',(-9.44033016700006,11.6,-4.66196242300002));
#273074=CARTESIAN_POINT('Ctrl Pts',(-9.44179495000006,15.2,-4.66307705300002));
#273075=CARTESIAN_POINT('Ctrl Pts',(-9.44179495000006,11.6,-4.66307705300002));
#273076=CARTESIAN_POINT('Ctrl Pts',(-9.44326456000006,15.2,-4.66419748500002));
#273077=CARTESIAN_POINT('Ctrl Pts',(-9.44326456000006,11.6,-4.66419748500002));
#273078=CARTESIAN_POINT('Ctrl Pts',(-9.44473898000006,15.2,-4.66532372300001));
#273079=CARTESIAN_POINT('Ctrl Pts',(-9.44473898000006,11.6,-4.66532372300002));
#273080=CARTESIAN_POINT('Ctrl Pts',(-9.44621818800006,15.2,-4.66645576400001));
#273081=CARTESIAN_POINT('Ctrl Pts',(-9.44621818800006,11.6,-4.66645576400001));
#273082=CARTESIAN_POINT('Ctrl Pts',(-9.44770216400006,15.2,-4.66759360700001));
#273083=CARTESIAN_POINT('Ctrl Pts',(-9.44770216400006,11.6,-4.66759360700001));
#273084=CARTESIAN_POINT('Ctrl Pts',(-9.44919088600006,15.2,-4.66873725400001));
#273085=CARTESIAN_POINT('Ctrl Pts',(-9.44919088600006,11.6,-4.66873725400002));
#273086=CARTESIAN_POINT('Ctrl Pts',(-9.45068433700006,15.2,-4.66988670300001));
#273087=CARTESIAN_POINT('Ctrl Pts',(-9.45068433700006,11.6,-4.66988670300002));
#273088=CARTESIAN_POINT('Ctrl Pts',(-9.45218249400006,15.2,-4.67104195400001));
#273089=CARTESIAN_POINT('Ctrl Pts',(-9.45218249400006,11.6,-4.67104195400002));
#273090=CARTESIAN_POINT('Ctrl Pts',(-9.45368533800006,15.2,-4.67220300800001));
#273091=CARTESIAN_POINT('Ctrl Pts',(-9.45368533800006,11.6,-4.67220300800001));
#273092=CARTESIAN_POINT('Ctrl Pts',(-9.45519284900006,15.2,-4.67336986400001));
#273093=CARTESIAN_POINT('Ctrl Pts',(-9.45519284900006,11.6,-4.67336986400001));
#273094=CARTESIAN_POINT('Ctrl Pts',(-9.45670500700006,15.2,-4.67454252000001));
#273095=CARTESIAN_POINT('Ctrl Pts',(-9.45670500700006,11.6,-4.67454252000001));
#273096=CARTESIAN_POINT('Ctrl Pts',(-9.45822179200006,15.2,-4.67572097700002));
#273097=CARTESIAN_POINT('Ctrl Pts',(-9.45822179200006,11.6,-4.67572097700002));
#273098=CARTESIAN_POINT('Ctrl Pts',(-9.45974318400006,15.2,-4.67690523600002));
#273099=CARTESIAN_POINT('Ctrl Pts',(-9.45974318400006,11.6,-4.67690523600002));
#273100=CARTESIAN_POINT('Ctrl Pts',(-9.46126916300006,15.2,-4.67809529500002));
#273101=CARTESIAN_POINT('Ctrl Pts',(-9.46126916300006,11.6,-4.67809529500002));
#273102=CARTESIAN_POINT('Ctrl Pts',(-9.46279971000006,15.2,-4.67929115300001));
#273103=CARTESIAN_POINT('Ctrl Pts',(-9.46279971000006,11.6,-4.67929115300001));
#273104=CARTESIAN_POINT('Ctrl Pts',(-9.46433480500006,15.2,-4.68049281000001));
#273105=CARTESIAN_POINT('Ctrl Pts',(-9.46433480500006,11.6,-4.68049281000001));
#273106=CARTESIAN_POINT('Ctrl Pts',(-9.46587442900006,15.2,-4.68170026700002));
#273107=CARTESIAN_POINT('Ctrl Pts',(-9.46587442900006,11.6,-4.68170026700002));
#273108=CARTESIAN_POINT('Ctrl Pts',(-9.46741856000006,15.2,-4.68291352200001));
#273109=CARTESIAN_POINT('Ctrl Pts',(-9.46741856000006,11.6,-4.68291352200001));
#273110=CARTESIAN_POINT('Ctrl Pts',(-9.46896718300006,15.2,-4.68413257500002));
#273111=CARTESIAN_POINT('Ctrl Pts',(-9.46896718300006,11.6,-4.68413257500002));
#273112=CARTESIAN_POINT('Ctrl Pts',(-9.47052027400006,15.2,-4.68535742600002));
#273113=CARTESIAN_POINT('Ctrl Pts',(-9.47052027400006,11.6,-4.68535742600002));
#273114=CARTESIAN_POINT('Ctrl Pts',(-9.47207781800006,15.2,-4.68658807500002));
#273115=CARTESIAN_POINT('Ctrl Pts',(-9.47207781800006,11.6,-4.68658807500002));
#273116=CARTESIAN_POINT('Ctrl Pts',(-9.47363979200006,15.2,-4.68782452000001));
#273117=CARTESIAN_POINT('Ctrl Pts',(-9.47363979200006,11.6,-4.68782452000002));
#273118=CARTESIAN_POINT('Ctrl Pts',(-9.47520617900006,15.2,-4.68906676100001));
#273119=CARTESIAN_POINT('Ctrl Pts',(-9.47520617900006,11.6,-4.68906676100001));
#273120=CARTESIAN_POINT('Ctrl Pts',(-9.47677695900006,15.2,-4.69031479900002));
#273121=CARTESIAN_POINT('Ctrl Pts',(-9.47677695900006,11.6,-4.69031479900002));
#273122=CARTESIAN_POINT('Ctrl Pts',(-9.47835211500006,15.2,-4.69156863100002));
#273123=CARTESIAN_POINT('Ctrl Pts',(-9.47835211500006,11.6,-4.69156863100002));
#273124=CARTESIAN_POINT('Ctrl Pts',(-9.47993162400006,15.2,-4.69282825900001));
#273125=CARTESIAN_POINT('Ctrl Pts',(-9.47993162400006,11.6,-4.69282825900002));
#273126=CARTESIAN_POINT('Ctrl Pts',(-9.48151547100006,15.2,-4.69409368000001));
#273127=CARTESIAN_POINT('Ctrl Pts',(-9.48151547100006,11.6,-4.69409368000001));
#273128=CARTESIAN_POINT('Ctrl Pts',(-9.48310363400006,15.2,-4.69536489600001));
#273129=CARTESIAN_POINT('Ctrl Pts',(-9.48310363400006,11.6,-4.69536489600001));
#273130=CARTESIAN_POINT('Ctrl Pts',(-9.48469609800006,15.2,-4.69664190500001));
#273131=CARTESIAN_POINT('Ctrl Pts',(-9.48469609800006,11.6,-4.69664190500001));
#273132=CARTESIAN_POINT('Ctrl Pts',(-9.48629284000006,15.2,-4.69792470600002));
#273133=CARTESIAN_POINT('Ctrl Pts',(-9.48629284000006,11.6,-4.69792470600002));
#273134=CARTESIAN_POINT('Ctrl Pts',(-9.48789384500006,15.2,-4.69921330000002));
#273135=CARTESIAN_POINT('Ctrl Pts',(-9.48789384500006,11.6,-4.69921330000002));
#273136=CARTESIAN_POINT('Ctrl Pts',(-9.48949909200006,15.2,-4.70050768500001));
#273137=CARTESIAN_POINT('Ctrl Pts',(-9.48949909200006,11.6,-4.70050768500002));
#273138=CARTESIAN_POINT('Ctrl Pts',(-9.49110856400005,15.2,-4.70180786200002));
#273139=CARTESIAN_POINT('Ctrl Pts',(-9.49110856400005,11.6,-4.70180786200002));
#273140=CARTESIAN_POINT('Ctrl Pts',(-9.49272224000006,15.2,-4.70311382800002));
#273141=CARTESIAN_POINT('Ctrl Pts',(-9.49272224000006,11.6,-4.70311382800002));
#273142=CARTESIAN_POINT('Ctrl Pts',(-9.49434010600006,15.2,-4.70442558400002));
#273143=CARTESIAN_POINT('Ctrl Pts',(-9.49434010600006,11.6,-4.70442558400002));
#273144=CARTESIAN_POINT('Ctrl Pts',(-9.49596213900006,15.2,-4.70574313000002));
#273145=CARTESIAN_POINT('Ctrl Pts',(-9.49596213900006,11.6,-4.70574313000002));
#273146=CARTESIAN_POINT('Ctrl Pts',(-9.49758832300006,15.2,-4.70706646400001));
#273147=CARTESIAN_POINT('Ctrl Pts',(-9.49758832300006,11.6,-4.70706646400001));
#273148=CARTESIAN_POINT('Ctrl Pts',(-9.49921864000006,15.2,-4.70839558600002));
#273149=CARTESIAN_POINT('Ctrl Pts',(-9.49921864000006,11.6,-4.70839558600002));
#273150=CARTESIAN_POINT('Ctrl Pts',(-9.50085307100006,15.2,-4.70973049600001));
#273151=CARTESIAN_POINT('Ctrl Pts',(-9.50085307100006,11.6,-4.70973049600001));
#273152=CARTESIAN_POINT('Ctrl Pts',(-9.50249159800006,15.2,-4.71107119200001));
#273153=CARTESIAN_POINT('Ctrl Pts',(-9.50249159800006,11.6,-4.71107119200001));
#273154=CARTESIAN_POINT('Ctrl Pts',(-9.50413420300006,15.2,-4.71241767400001));
#273155=CARTESIAN_POINT('Ctrl Pts',(-9.50413420300006,11.6,-4.71241767400001));
#273156=CARTESIAN_POINT('Ctrl Pts',(-9.50578086900006,15.2,-4.71376994100002));
#273157=CARTESIAN_POINT('Ctrl Pts',(-9.50578086900006,11.6,-4.71376994100002));
#273158=CARTESIAN_POINT('Ctrl Pts',(-9.50743157600006,15.2,-4.71512799400001));
#273159=CARTESIAN_POINT('Ctrl Pts',(-9.50743157600006,11.6,-4.71512799400002));
#273160=CARTESIAN_POINT('Ctrl Pts',(-9.50908630800006,15.2,-4.71649183000002));
#273161=CARTESIAN_POINT('Ctrl Pts',(-9.50908630800006,11.6,-4.71649183000002));
#273162=CARTESIAN_POINT('Ctrl Pts',(-9.51074504700006,15.2,-4.71786145000001));
#273163=CARTESIAN_POINT('Ctrl Pts',(-9.51074504700006,11.6,-4.71786145000001));
#273164=CARTESIAN_POINT('Ctrl Pts',(-9.51240777300006,15.2,-4.71923685200001));
#273165=CARTESIAN_POINT('Ctrl Pts',(-9.51240777300006,11.6,-4.71923685200002));
#273166=CARTESIAN_POINT('Ctrl Pts',(-9.51407447200006,15.2,-4.72061803600001));
#273167=CARTESIAN_POINT('Ctrl Pts',(-9.51407447200006,11.6,-4.72061803600001));
#273168=CARTESIAN_POINT('Ctrl Pts',(-9.51574512200006,15.2,-4.72200500100001));
#273169=CARTESIAN_POINT('Ctrl Pts',(-9.51574512200006,11.6,-4.72200500100001));
#273170=CARTESIAN_POINT('Ctrl Pts',(-9.51741970900006,15.2,-4.72339774700002));
#273171=CARTESIAN_POINT('Ctrl Pts',(-9.51741970900006,11.6,-4.72339774700002));
#273172=CARTESIAN_POINT('Ctrl Pts',(-9.51909821500006,15.2,-4.72479627200002));
#273173=CARTESIAN_POINT('Ctrl Pts',(-9.51909821500006,11.6,-4.72479627200002));
#273174=CARTESIAN_POINT('Ctrl Pts',(-9.52078062000006,15.2,-4.72620057600002));
#273175=CARTESIAN_POINT('Ctrl Pts',(-9.52078062000006,11.6,-4.72620057600002));
#273176=CARTESIAN_POINT('Ctrl Pts',(-9.52246690900006,15.2,-4.72761065900002));
#273177=CARTESIAN_POINT('Ctrl Pts',(-9.52246690900006,11.6,-4.72761065900002));
#273178=CARTESIAN_POINT('Ctrl Pts',(-9.52415706300006,15.2,-4.72902651900001));
#273179=CARTESIAN_POINT('Ctrl Pts',(-9.52415706300006,11.6,-4.72902651900002));
#273180=CARTESIAN_POINT('Ctrl Pts',(-9.52585106700005,15.2,-4.73044815500002));
#273181=CARTESIAN_POINT('Ctrl Pts',(-9.52585106700005,11.6,-4.73044815500002));
#273182=CARTESIAN_POINT('Ctrl Pts',(-9.52754890100006,15.2,-4.73187556700001));
#273183=CARTESIAN_POINT('Ctrl Pts',(-9.52754890100006,11.6,-4.73187556700002));
#273184=CARTESIAN_POINT('Ctrl Pts',(-9.52925054900006,15.2,-4.73330875500002));
#273185=CARTESIAN_POINT('Ctrl Pts',(-9.52925054900006,11.6,-4.73330875500002));
#273186=CARTESIAN_POINT('Ctrl Pts',(-9.53095599400006,15.2,-4.73474771700001));
#273187=CARTESIAN_POINT('Ctrl Pts',(-9.53095599400006,11.6,-4.73474771700001));
#273188=CARTESIAN_POINT('Ctrl Pts',(-9.53266521800006,15.2,-4.73619245200001));
#273189=CARTESIAN_POINT('Ctrl Pts',(-9.53266521800006,11.6,-4.73619245200002));
#273190=CARTESIAN_POINT('Ctrl Pts',(-9.53437820600006,15.2,-4.73764296000001));
#273191=CARTESIAN_POINT('Ctrl Pts',(-9.53437820600006,11.6,-4.73764296000002));
#273192=CARTESIAN_POINT('Ctrl Pts',(-9.53609493900006,15.2,-4.73909923900001));
#273193=CARTESIAN_POINT('Ctrl Pts',(-9.53609493900006,11.6,-4.73909923900001));
#273194=CARTESIAN_POINT('Ctrl Pts',(-9.53781539900006,15.2,-4.74056129000001));
#273195=CARTESIAN_POINT('Ctrl Pts',(-9.53781539900006,11.6,-4.74056129000001));
#273196=CARTESIAN_POINT('Ctrl Pts',(-9.53953957300006,15.2,-4.74202911000001));
#273197=CARTESIAN_POINT('Ctrl Pts',(-9.53953957300006,11.6,-4.74202911000001));
#273198=CARTESIAN_POINT('Ctrl Pts',(-9.54126744000006,15.2,-4.74350270000001));
#273199=CARTESIAN_POINT('Ctrl Pts',(-9.54126744000006,11.6,-4.74350270000001));
#273200=CARTESIAN_POINT('Ctrl Pts',(-9.54299898700006,15.2,-4.74498205800002));
#273201=CARTESIAN_POINT('Ctrl Pts',(-9.54299898700006,11.6,-4.74498205800002));
#273202=CARTESIAN_POINT('Ctrl Pts',(-9.54473419400006,15.2,-4.74646718400002));
#273203=CARTESIAN_POINT('Ctrl Pts',(-9.54473419400006,11.6,-4.74646718400002));
#273204=CARTESIAN_POINT('Ctrl Pts',(-9.54647304600006,15.2,-4.74795807600001));
#273205=CARTESIAN_POINT('Ctrl Pts',(-9.54647304600006,11.6,-4.74795807600001));
#273206=CARTESIAN_POINT('Ctrl Pts',(-9.54821552600006,15.2,-4.74945473400001));
#273207=CARTESIAN_POINT('Ctrl Pts',(-9.54821552600006,11.6,-4.74945473400001));
#273208=CARTESIAN_POINT('Ctrl Pts',(-9.54996161700005,15.2,-4.75095715700002));
#273209=CARTESIAN_POINT('Ctrl Pts',(-9.54996161700005,11.6,-4.75095715700002));
#273210=CARTESIAN_POINT('Ctrl Pts',(-9.55171130400006,15.2,-4.75246534400001));
#273211=CARTESIAN_POINT('Ctrl Pts',(-9.55171130400006,11.6,-4.75246534400002));
#273212=CARTESIAN_POINT('Ctrl Pts',(-9.55346456800006,15.2,-4.75397929300001));
#273213=CARTESIAN_POINT('Ctrl Pts',(-9.55346456800006,11.6,-4.75397929300002));
#273214=CARTESIAN_POINT('Ctrl Pts',(-9.55522139400006,15.2,-4.75549900500001));
#273215=CARTESIAN_POINT('Ctrl Pts',(-9.55522139400006,11.6,-4.75549900500001));
#273216=CARTESIAN_POINT('Ctrl Pts',(-9.55698176600006,15.2,-4.75702447800002));
#273217=CARTESIAN_POINT('Ctrl Pts',(-9.55698176600006,11.6,-4.75702447800002));
#273218=CARTESIAN_POINT('Ctrl Pts',(-9.55874566600006,15.2,-4.75855571100002));
#273219=CARTESIAN_POINT('Ctrl Pts',(-9.55874566600006,11.6,-4.75855571100002));
#273220=CARTESIAN_POINT('Ctrl Pts',(-9.56051308000006,15.2,-4.76009270400001));
#273221=CARTESIAN_POINT('Ctrl Pts',(-9.56051308000006,11.6,-4.76009270400001));
#273222=CARTESIAN_POINT('Ctrl Pts',(-9.56228398900006,15.2,-4.76163545400001));
#273223=CARTESIAN_POINT('Ctrl Pts',(-9.56228398900006,11.6,-4.76163545400001));
#273224=CARTESIAN_POINT('Ctrl Pts',(-9.56405838000006,15.2,-4.76318396200002));
#273225=CARTESIAN_POINT('Ctrl Pts',(-9.56405838000006,11.6,-4.76318396200002));
#273226=CARTESIAN_POINT('Ctrl Pts',(-9.56583623400006,15.2,-4.76473822600001));
#273227=CARTESIAN_POINT('Ctrl Pts',(-9.56583623400006,11.6,-4.76473822600001));
#273228=CARTESIAN_POINT('Ctrl Pts',(-9.56761753700006,15.2,-4.76629824700002));
#273229=CARTESIAN_POINT('Ctrl Pts',(-9.56761753700006,11.6,-4.76629824700002));
#273230=CARTESIAN_POINT('Ctrl Pts',(-9.56940227100005,15.2,-4.76786402000001));
#273231=CARTESIAN_POINT('Ctrl Pts',(-9.56940227100005,11.6,-4.76786402000002));
#273232=CARTESIAN_POINT('Ctrl Pts',(-9.57119042200006,15.2,-4.76943554800001));
#273233=CARTESIAN_POINT('Ctrl Pts',(-9.57119042200006,11.6,-4.76943554800001));
#273234=CARTESIAN_POINT('Ctrl Pts',(-9.57298197200006,15.2,-4.77101282700001));
#273235=CARTESIAN_POINT('Ctrl Pts',(-9.57298197200006,11.6,-4.77101282700001));
#273236=CARTESIAN_POINT('Ctrl Pts',(-9.57477690700006,15.2,-4.77259585800001));
#273237=CARTESIAN_POINT('Ctrl Pts',(-9.57477690700006,11.6,-4.77259585800002));
#273238=CARTESIAN_POINT('Ctrl Pts',(-9.57657520800005,15.2,-4.77418463900001));
#273239=CARTESIAN_POINT('Ctrl Pts',(-9.57657520800005,11.6,-4.77418463900001));
#273240=CARTESIAN_POINT('Ctrl Pts',(-9.57837686400006,15.2,-4.77577917000001));
#273241=CARTESIAN_POINT('Ctrl Pts',(-9.57837686400006,11.6,-4.77577917000001));
#273242=CARTESIAN_POINT('Ctrl Pts',(-9.58018185400006,15.2,-4.77737944900001));
#273243=CARTESIAN_POINT('Ctrl Pts',(-9.58018185400006,11.6,-4.77737944900001));
#273244=CARTESIAN_POINT('Ctrl Pts',(-9.58199016700006,15.2,-4.77898547400001));
#273245=CARTESIAN_POINT('Ctrl Pts',(-9.58199016700006,11.6,-4.77898547400002));
#273246=CARTESIAN_POINT('Ctrl Pts',(-9.58380178400006,15.2,-4.78059724600001));
#273247=CARTESIAN_POINT('Ctrl Pts',(-9.58380178400006,11.6,-4.78059724600001));
#273248=CARTESIAN_POINT('Ctrl Pts',(-9.58561669100006,15.2,-4.78221476300002));
#273249=CARTESIAN_POINT('Ctrl Pts',(-9.58561669100006,11.6,-4.78221476300002));
#273250=CARTESIAN_POINT('Ctrl Pts',(-9.58743487200006,15.2,-4.78383802400002));
#273251=CARTESIAN_POINT('Ctrl Pts',(-9.58743487200006,11.6,-4.78383802400002));
#273252=CARTESIAN_POINT('Ctrl Pts',(-9.58925631100006,15.2,-4.78546702800001));
#273253=CARTESIAN_POINT('Ctrl Pts',(-9.58925631100006,11.6,-4.78546702800002));
#273254=CARTESIAN_POINT('Ctrl Pts',(-9.59108099300006,15.2,-4.78710177400002));
#273255=CARTESIAN_POINT('Ctrl Pts',(-9.59108099300006,11.6,-4.78710177400002));
#273256=CARTESIAN_POINT('Ctrl Pts',(-9.59290890200006,15.2,-4.78874226000002));
#273257=CARTESIAN_POINT('Ctrl Pts',(-9.59290890200006,11.6,-4.78874226000002));
#273258=CARTESIAN_POINT('Ctrl Pts',(-9.59474002200006,15.2,-4.79038848600001));
#273259=CARTESIAN_POINT('Ctrl Pts',(-9.59474002200006,11.6,-4.79038848600002));
#273260=CARTESIAN_POINT('Ctrl Pts',(-9.59657434000006,15.2,-4.79204045100001));
#273261=CARTESIAN_POINT('Ctrl Pts',(-9.59657434000006,11.6,-4.79204045100001));
#273262=CARTESIAN_POINT('Ctrl Pts',(-9.59841183800006,15.2,-4.79369815300001));
#273263=CARTESIAN_POINT('Ctrl Pts',(-9.59841183800006,11.6,-4.79369815300002));
#273264=CARTESIAN_POINT('Ctrl Pts',(-9.60025250300006,15.2,-4.79536159100002));
#273265=CARTESIAN_POINT('Ctrl Pts',(-9.60025250300006,11.6,-4.79536159100002));
#273266=CARTESIAN_POINT('Ctrl Pts',(-9.60209631800006,15.2,-4.79703076500002));
#273267=CARTESIAN_POINT('Ctrl Pts',(-9.60209631800006,11.6,-4.79703076500002));
#273268=CARTESIAN_POINT('Ctrl Pts',(-9.60394326800006,15.2,-4.79870567200001));
#273269=CARTESIAN_POINT('Ctrl Pts',(-9.60394326800006,11.6,-4.79870567200001));
#273270=CARTESIAN_POINT('Ctrl Pts',(-9.60579333900006,15.2,-4.80038631200001));
#273271=CARTESIAN_POINT('Ctrl Pts',(-9.60579333900006,11.6,-4.80038631200001));
#273272=CARTESIAN_POINT('Ctrl Pts',(-9.60764651500006,15.2,-4.80207268400001));
#273273=CARTESIAN_POINT('Ctrl Pts',(-9.60764651500006,11.6,-4.80207268400001));
#273274=CARTESIAN_POINT('Ctrl Pts',(-9.60950278100006,15.2,-4.80376478600002));
#273275=CARTESIAN_POINT('Ctrl Pts',(-9.60950278100006,11.6,-4.80376478600002));
#273276=CARTESIAN_POINT('Ctrl Pts',(-9.61136212100006,15.2,-4.80546261800002));
#273277=CARTESIAN_POINT('Ctrl Pts',(-9.61136212100006,11.6,-4.80546261800002));
#273278=CARTESIAN_POINT('Ctrl Pts',(-9.61322452200006,15.2,-4.80716617800002));
#273279=CARTESIAN_POINT('Ctrl Pts',(-9.61322452200006,11.6,-4.80716617800002));
#273280=CARTESIAN_POINT('Ctrl Pts',(-9.61508996800006,15.2,-4.80887546500002));
#273281=CARTESIAN_POINT('Ctrl Pts',(-9.61508996800006,11.6,-4.80887546500002));
#273282=CARTESIAN_POINT('Ctrl Pts',(-9.61695844300005,15.2,-4.81059047700001));
#273283=CARTESIAN_POINT('Ctrl Pts',(-9.61695844300005,11.6,-4.81059047700001));
#273284=CARTESIAN_POINT('Ctrl Pts',(-9.61882993500006,15.2,-4.81231121400001));
#273285=CARTESIAN_POINT('Ctrl Pts',(-9.61882993500006,11.6,-4.81231121400001));
#273286=CARTESIAN_POINT('Ctrl Pts',(-9.62070442700006,15.2,-4.81403767400002));
#273287=CARTESIAN_POINT('Ctrl Pts',(-9.62070442700006,11.6,-4.81403767400002));
#273288=CARTESIAN_POINT('Ctrl Pts',(-9.62258190400006,15.2,-4.81576985800002));
#273289=CARTESIAN_POINT('Ctrl Pts',(-9.62258190400006,11.6,-4.81576985800002));
#273290=CARTESIAN_POINT('Ctrl Pts',(-9.62446235200006,15.2,-4.81750776100001));
#273291=CARTESIAN_POINT('Ctrl Pts',(-9.62446235200006,11.6,-4.81750776100002));
#273292=CARTESIAN_POINT('Ctrl Pts',(-9.62634575600006,15.2,-4.81925138300001));
#273293=CARTESIAN_POINT('Ctrl Pts',(-9.62634575600006,11.6,-4.81925138300001));
#273294=CARTESIAN_POINT('Ctrl Pts',(-9.62823210200006,15.2,-4.82100072500002));
#273295=CARTESIAN_POINT('Ctrl Pts',(-9.62823210200006,11.6,-4.82100072500002));
#273296=CARTESIAN_POINT('Ctrl Pts',(-9.63012137400005,15.2,-4.82275578400001));
#273297=CARTESIAN_POINT('Ctrl Pts',(-9.63012137400005,11.6,-4.82275578400001));
#273298=CARTESIAN_POINT('Ctrl Pts',(-9.63201355900006,15.2,-4.82451655900002));
#273299=CARTESIAN_POINT('Ctrl Pts',(-9.63201355900006,11.6,-4.82451655900002));
#273300=CARTESIAN_POINT('Ctrl Pts',(-9.63390864200005,15.2,-4.82628304800001));
#273301=CARTESIAN_POINT('Ctrl Pts',(-9.63390864200005,11.6,-4.82628304800001));
#273302=CARTESIAN_POINT('Ctrl Pts',(-9.63580660800006,15.2,-4.82805525200002));
#273303=CARTESIAN_POINT('Ctrl Pts',(-9.63580660800006,11.6,-4.82805525200002));
#273304=CARTESIAN_POINT('Ctrl Pts',(-9.63770744300006,15.2,-4.82983316700001));
#273305=CARTESIAN_POINT('Ctrl Pts',(-9.63770744300006,11.6,-4.82983316700001));
#273306=CARTESIAN_POINT('Ctrl Pts',(-9.63961113100006,15.2,-4.83161679200002));
#273307=CARTESIAN_POINT('Ctrl Pts',(-9.63961113100006,11.6,-4.83161679200002));
#273308=CARTESIAN_POINT('Ctrl Pts',(-9.64151766000005,15.2,-4.83340612800002));
#273309=CARTESIAN_POINT('Ctrl Pts',(-9.64151766000005,11.6,-4.83340612800002));
#273310=CARTESIAN_POINT('Ctrl Pts',(-9.64342701400006,15.2,-4.83520117200001));
#273311=CARTESIAN_POINT('Ctrl Pts',(-9.64342701400006,11.6,-4.83520117200001));
#273312=CARTESIAN_POINT('Ctrl Pts',(-9.64533918000006,15.2,-4.83700192200001));
#273313=CARTESIAN_POINT('Ctrl Pts',(-9.64533918000006,11.6,-4.83700192200002));
#273314=CARTESIAN_POINT('Ctrl Pts',(-9.64725414300006,15.2,-4.83880837900001));
#273315=CARTESIAN_POINT('Ctrl Pts',(-9.64725414300006,11.6,-4.83880837900002));
#273316=CARTESIAN_POINT('Ctrl Pts',(-9.64917188800005,15.2,-4.84062054000002));
#273317=CARTESIAN_POINT('Ctrl Pts',(-9.64917188800005,11.6,-4.84062054000002));
#273318=CARTESIAN_POINT('Ctrl Pts',(-9.65109240200006,15.2,-4.84243840400001));
#273319=CARTESIAN_POINT('Ctrl Pts',(-9.65109240200006,11.6,-4.84243840400001));
#273320=CARTESIAN_POINT('Ctrl Pts',(-9.65301567100006,15.2,-4.84426196900001));
#273321=CARTESIAN_POINT('Ctrl Pts',(-9.65301567100006,11.6,-4.84426196900001));
#273322=CARTESIAN_POINT('Ctrl Pts',(-9.65494167900006,15.2,-4.84609123600002));
#273323=CARTESIAN_POINT('Ctrl Pts',(-9.65494167900006,11.6,-4.84609123600002));
#273324=CARTESIAN_POINT('Ctrl Pts',(-9.65687041400006,15.2,-4.84792620100002));
#273325=CARTESIAN_POINT('Ctrl Pts',(-9.65687041400006,11.6,-4.84792620100002));
#273326=CARTESIAN_POINT('Ctrl Pts',(-9.65880186100006,15.2,-4.84976686400001));
#273327=CARTESIAN_POINT('Ctrl Pts',(-9.65880186100006,11.6,-4.84976686400001));
#273328=CARTESIAN_POINT('Ctrl Pts',(-9.66073600600006,15.2,-4.85161322300002));
#273329=CARTESIAN_POINT('Ctrl Pts',(-9.66073600600006,11.6,-4.85161322300002));
#273330=CARTESIAN_POINT('Ctrl Pts',(-9.66267283500006,15.2,-4.85346527800001));
#273331=CARTESIAN_POINT('Ctrl Pts',(-9.66267283500006,11.6,-4.85346527800001));
#273332=CARTESIAN_POINT('Ctrl Pts',(-9.66461233400006,15.2,-4.85532302500001));
#273333=CARTESIAN_POINT('Ctrl Pts',(-9.66461233400006,11.6,-4.85532302500001));
#273334=CARTESIAN_POINT('Ctrl Pts',(-9.66655449000006,15.2,-4.85718646500001));
#273335=CARTESIAN_POINT('Ctrl Pts',(-9.66655449000006,11.6,-4.85718646500001));
#273336=CARTESIAN_POINT('Ctrl Pts',(-9.66849928800006,15.2,-4.85905559500001));
#273337=CARTESIAN_POINT('Ctrl Pts',(-9.66849928800006,11.6,-4.85905559500001));
#273338=CARTESIAN_POINT('Ctrl Pts',(-9.67044671500006,15.2,-4.86093041600002));
#273339=CARTESIAN_POINT('Ctrl Pts',(-9.67044671500006,11.6,-4.86093041600002));
#273340=CARTESIAN_POINT('Ctrl Pts',(-9.67239675600006,15.2,-4.86281092400001));
#273341=CARTESIAN_POINT('Ctrl Pts',(-9.67239675600006,11.6,-4.86281092400001));
#273342=CARTESIAN_POINT('Ctrl Pts',(-9.67434939900006,15.2,-4.86469711900002));
#273343=CARTESIAN_POINT('Ctrl Pts',(-9.67434939900006,11.6,-4.86469711900002));
#273344=CARTESIAN_POINT('Ctrl Pts',(-9.67630462800006,15.2,-4.86658900000001));
#273345=CARTESIAN_POINT('Ctrl Pts',(-9.67630462800006,11.6,-4.86658900000002));
#273346=CARTESIAN_POINT('Ctrl Pts',(-9.67826243300006,15.2,-4.86848656300001));
#273347=CARTESIAN_POINT('Ctrl Pts',(-9.67826243300006,11.6,-4.86848656300001));
#273348=CARTESIAN_POINT('Ctrl Pts',(-9.68022279600006,15.2,-4.87038981000001));
#273349=CARTESIAN_POINT('Ctrl Pts',(-9.68022279600006,11.6,-4.87038981000001));
#273350=CARTESIAN_POINT('Ctrl Pts',(-9.68218570600006,15.2,-4.87229873800001));
#273351=CARTESIAN_POINT('Ctrl Pts',(-9.68218570600006,11.6,-4.87229873800001));
#273352=CARTESIAN_POINT('Ctrl Pts',(-9.68415114900005,15.2,-4.87421334500001));
#273353=CARTESIAN_POINT('Ctrl Pts',(-9.68415114900005,11.6,-4.87421334500001));
#273354=CARTESIAN_POINT('Ctrl Pts',(-9.68611911100006,15.2,-4.87613363000001));
#273355=CARTESIAN_POINT('Ctrl Pts',(-9.68611911100006,11.6,-4.87613363000001));
#273356=CARTESIAN_POINT('Ctrl Pts',(-9.68808957900006,15.2,-4.87805959100001));
#273357=CARTESIAN_POINT('Ctrl Pts',(-9.68808957900006,11.6,-4.87805959100002));
#273358=CARTESIAN_POINT('Ctrl Pts',(-9.69006253900006,15.2,-4.87999122800002));
#273359=CARTESIAN_POINT('Ctrl Pts',(-9.69006253900006,11.6,-4.87999122800002));
#273360=CARTESIAN_POINT('Ctrl Pts',(-9.69203797800006,15.2,-4.88192854000001));
#273361=CARTESIAN_POINT('Ctrl Pts',(-9.69203797800006,11.6,-4.88192854000001));
#273362=CARTESIAN_POINT('Ctrl Pts',(-9.69401588300006,15.2,-4.88387152300001));
#273363=CARTESIAN_POINT('Ctrl Pts',(-9.69401588300006,11.6,-4.88387152300001));
#273364=CARTESIAN_POINT('Ctrl Pts',(-9.69599623900006,15.2,-4.88582017700002));
#273365=CARTESIAN_POINT('Ctrl Pts',(-9.69599623900006,11.6,-4.88582017700002));
#273366=CARTESIAN_POINT('Ctrl Pts',(-9.69797903400006,15.2,-4.88777450000002));
#273367=CARTESIAN_POINT('Ctrl Pts',(-9.69797903400006,11.6,-4.88777450000002));
#273368=CARTESIAN_POINT('Ctrl Pts',(-9.69996425500005,15.2,-4.88973449200001));
#273369=CARTESIAN_POINT('Ctrl Pts',(-9.69996425500005,11.6,-4.88973449200001));
#273370=CARTESIAN_POINT('Ctrl Pts',(-9.70195188800006,15.2,-4.89170014900001));
#273371=CARTESIAN_POINT('Ctrl Pts',(-9.70195188800006,11.6,-4.89170014900001));
#273372=CARTESIAN_POINT('Ctrl Pts',(-9.70394191900006,15.2,-4.89367147200001));
#273373=CARTESIAN_POINT('Ctrl Pts',(-9.70394191900006,11.6,-4.89367147200001));
#273374=CARTESIAN_POINT('Ctrl Pts',(-9.70593433700006,15.2,-4.89564845700002));
#273375=CARTESIAN_POINT('Ctrl Pts',(-9.70593433700006,11.6,-4.89564845700002));
#273376=CARTESIAN_POINT('Ctrl Pts',(-9.70792912700006,15.2,-4.89763110500002));
#273377=CARTESIAN_POINT('Ctrl Pts',(-9.70792912700006,11.6,-4.89763110500002));
#273378=CARTESIAN_POINT('Ctrl Pts',(-9.70992627600006,15.2,-4.89961941300002));
#273379=CARTESIAN_POINT('Ctrl Pts',(-9.70992627600006,11.6,-4.89961941300002));
#273380=CARTESIAN_POINT('Ctrl Pts',(-9.71192577300006,15.2,-4.90161338000001));
#273381=CARTESIAN_POINT('Ctrl Pts',(-9.71192577300006,11.6,-4.90161338000001));
#273382=CARTESIAN_POINT('Ctrl Pts',(-9.71392760200006,15.2,-4.90361300400001));
#273383=CARTESIAN_POINT('Ctrl Pts',(-9.71392760200006,11.6,-4.90361300400001));
#273384=CARTESIAN_POINT('Ctrl Pts',(-9.71593175100006,15.2,-4.90561828400002));
#273385=CARTESIAN_POINT('Ctrl Pts',(-9.71593175100006,11.6,-4.90561828400002));
#273386=CARTESIAN_POINT('Ctrl Pts',(-9.71793820800006,15.2,-4.90762921800002));
#273387=CARTESIAN_POINT('Ctrl Pts',(-9.71793820800006,11.6,-4.90762921800002));
#273388=CARTESIAN_POINT('Ctrl Pts',(-9.71994695800005,15.2,-4.90964580500002));
#273389=CARTESIAN_POINT('Ctrl Pts',(-9.71994695800005,11.6,-4.90964580500002));
#273390=CARTESIAN_POINT('Ctrl Pts',(-9.72195799100006,15.2,-4.91166804200001));
#273391=CARTESIAN_POINT('Ctrl Pts',(-9.72195799100006,11.6,-4.91166804200002));
#273392=CARTESIAN_POINT('Ctrl Pts',(-9.72397129100005,15.2,-4.91369593000002));
#273393=CARTESIAN_POINT('Ctrl Pts',(-9.72397129100005,11.6,-4.91369593000002));
#273394=CARTESIAN_POINT('Ctrl Pts',(-9.72598684800005,15.2,-4.91572946500002));
#273395=CARTESIAN_POINT('Ctrl Pts',(-9.72598684800005,11.6,-4.91572946500002));
#273396=CARTESIAN_POINT('Ctrl Pts',(-9.72800464700006,15.2,-4.91776864800002));
#273397=CARTESIAN_POINT('Ctrl Pts',(-9.72800464700006,11.6,-4.91776864800002));
#273398=CARTESIAN_POINT('Ctrl Pts',(-9.73002467500006,15.2,-4.91981347400001));
#273399=CARTESIAN_POINT('Ctrl Pts',(-9.73002467500006,11.6,-4.91981347400001));
#273400=CARTESIAN_POINT('Ctrl Pts',(-9.73204692100006,15.2,-4.92186394400001));
#273401=CARTESIAN_POINT('Ctrl Pts',(-9.73204692100006,11.6,-4.92186394400001));
#273402=CARTESIAN_POINT('Ctrl Pts',(-9.73407137000006,15.2,-4.92392005600002));
#273403=CARTESIAN_POINT('Ctrl Pts',(-9.73407137000006,11.6,-4.92392005600002));
#273404=CARTESIAN_POINT('Ctrl Pts',(-9.73609801200006,15.2,-4.92598180800002));
#273405=CARTESIAN_POINT('Ctrl Pts',(-9.73609801200006,11.6,-4.92598180800002));
#273406=CARTESIAN_POINT('Ctrl Pts',(-9.73812683300006,15.2,-4.92804919800002));
#273407=CARTESIAN_POINT('Ctrl Pts',(-9.73812683300006,11.6,-4.92804919800002));
#273408=CARTESIAN_POINT('Ctrl Pts',(-9.74015782000006,15.2,-4.93012222600001));
#273409=CARTESIAN_POINT('Ctrl Pts',(-9.74015782000006,11.6,-4.93012222600001));
#273410=CARTESIAN_POINT('Ctrl Pts',(-9.74219096100006,15.2,-4.93220088800001));
#273411=CARTESIAN_POINT('Ctrl Pts',(-9.74219096100006,11.6,-4.93220088800001));
#273412=CARTESIAN_POINT('Ctrl Pts',(-9.74422624200006,15.2,-4.93428518400002));
#273413=CARTESIAN_POINT('Ctrl Pts',(-9.74422624200006,11.6,-4.93428518400002));
#273414=CARTESIAN_POINT('Ctrl Pts',(-9.74626365300006,15.2,-4.93637511300001));
#273415=CARTESIAN_POINT('Ctrl Pts',(-9.74626365300006,11.6,-4.93637511300001));
#273416=CARTESIAN_POINT('Ctrl Pts',(-9.74830317900006,15.2,-4.93847067000001));
#273417=CARTESIAN_POINT('Ctrl Pts',(-9.74830317900006,11.6,-4.93847067000001));
#273418=CARTESIAN_POINT('Ctrl Pts',(-9.75034480900005,15.2,-4.94057185800001));
#273419=CARTESIAN_POINT('Ctrl Pts',(-9.75034480900005,11.6,-4.94057185800001));
#273420=CARTESIAN_POINT('Ctrl Pts',(-9.75238852900006,15.2,-4.94267867300001));
#273421=CARTESIAN_POINT('Ctrl Pts',(-9.75238852900006,11.6,-4.94267867300001));
#273422=CARTESIAN_POINT('Ctrl Pts',(-9.75443432900006,15.2,-4.94479111400001));
#273423=CARTESIAN_POINT('Ctrl Pts',(-9.75443432900006,11.6,-4.94479111400001));
#273424=CARTESIAN_POINT('Ctrl Pts',(-9.75648219500006,15.2,-4.94690917700002));
#273425=CARTESIAN_POINT('Ctrl Pts',(-9.75648219500006,11.6,-4.94690917700002));
#273426=CARTESIAN_POINT('Ctrl Pts',(-9.75853211400005,15.2,-4.94903286300001));
#273427=CARTESIAN_POINT('Ctrl Pts',(-9.75853211400005,11.6,-4.94903286300001));
#273428=CARTESIAN_POINT('Ctrl Pts',(-9.76058407400006,15.2,-4.95116217000001));
#273429=CARTESIAN_POINT('Ctrl Pts',(-9.76058407400006,11.6,-4.95116217000002));
#273430=CARTESIAN_POINT('Ctrl Pts',(-9.76263806400006,15.2,-4.95329709600002));
#273431=CARTESIAN_POINT('Ctrl Pts',(-9.76263806400006,11.6,-4.95329709600002));
#273432=CARTESIAN_POINT('Ctrl Pts',(-9.76469407100006,15.2,-4.95543763800002));
#273433=CARTESIAN_POINT('Ctrl Pts',(-9.76469407100006,11.6,-4.95543763800002));
#273434=CARTESIAN_POINT('Ctrl Pts',(-9.76675208200006,15.2,-4.95758379600002));
#273435=CARTESIAN_POINT('Ctrl Pts',(-9.76675208200006,11.6,-4.95758379600002));
#273436=CARTESIAN_POINT('Ctrl Pts',(-9.76881208600006,15.2,-4.95973556900001));
#273437=CARTESIAN_POINT('Ctrl Pts',(-9.76881208600006,11.6,-4.95973556900002));
#273438=CARTESIAN_POINT('Ctrl Pts',(-9.77087406900005,15.2,-4.96189295300002));
#273439=CARTESIAN_POINT('Ctrl Pts',(-9.77087406900005,11.6,-4.96189295300002));
#273440=CARTESIAN_POINT('Ctrl Pts',(-9.77293802100006,15.2,-4.96405594800001));
#273441=CARTESIAN_POINT('Ctrl Pts',(-9.77293802100006,11.6,-4.96405594800002));
#273442=CARTESIAN_POINT('Ctrl Pts',(-9.77500392800006,15.2,-4.96622455100002));
#273443=CARTESIAN_POINT('Ctrl Pts',(-9.77500392800006,11.6,-4.96622455100002));
#273444=CARTESIAN_POINT('Ctrl Pts',(-9.77707178000006,15.2,-4.96839876200001));
#273445=CARTESIAN_POINT('Ctrl Pts',(-9.77707178000006,11.6,-4.96839876200002));
#273446=CARTESIAN_POINT('Ctrl Pts',(-9.77914156200006,15.2,-4.97057857700002));
#273447=CARTESIAN_POINT('Ctrl Pts',(-9.77914156200006,11.6,-4.97057857700002));
#273448=CARTESIAN_POINT('Ctrl Pts',(-9.78121326400006,15.2,-4.97276399700001));
#273449=CARTESIAN_POINT('Ctrl Pts',(-9.78121326400006,11.6,-4.97276399700001));
#273450=CARTESIAN_POINT('Ctrl Pts',(-9.78328687400005,15.2,-4.97495501800001));
#273451=CARTESIAN_POINT('Ctrl Pts',(-9.78328687400005,11.6,-4.97495501800001));
#273452=CARTESIAN_POINT('Ctrl Pts',(-9.78536237900006,15.2,-4.97715164000001));
#273453=CARTESIAN_POINT('Ctrl Pts',(-9.78536237900006,11.6,-4.97715164000002));
#273454=CARTESIAN_POINT('Ctrl Pts',(-9.78743976900006,15.2,-4.97935386100002));
#273455=CARTESIAN_POINT('Ctrl Pts',(-9.78743976900006,11.6,-4.97935386100002));
#273456=CARTESIAN_POINT('Ctrl Pts',(-9.78951902900006,15.2,-4.98156167700001));
#273457=CARTESIAN_POINT('Ctrl Pts',(-9.78951902900006,11.6,-4.98156167700001));
#273458=CARTESIAN_POINT('Ctrl Pts',(-9.79160014900006,15.2,-4.98377508900001));
#273459=CARTESIAN_POINT('Ctrl Pts',(-9.79160014900006,11.6,-4.98377508900001));
#273460=CARTESIAN_POINT('Ctrl Pts',(-9.79368311700006,15.2,-4.98599409400001));
#273461=CARTESIAN_POINT('Ctrl Pts',(-9.79368311700006,11.6,-4.98599409400002));
#273462=CARTESIAN_POINT('Ctrl Pts',(-9.79576792100006,15.2,-4.98821869000002));
#273463=CARTESIAN_POINT('Ctrl Pts',(-9.79576792100006,11.6,-4.98821869000002));
#273464=CARTESIAN_POINT('Ctrl Pts',(-9.79785454900006,15.2,-4.99044887600002));
#273465=CARTESIAN_POINT('Ctrl Pts',(-9.79785454900006,11.6,-4.99044887600002));
#273466=CARTESIAN_POINT('Ctrl Pts',(-9.79994298800005,15.2,-4.99268465100001));
#273467=CARTESIAN_POINT('Ctrl Pts',(-9.79994298800005,11.6,-4.99268465100002));
#273468=CARTESIAN_POINT('Ctrl Pts',(-9.80203322900006,15.2,-4.99492601000001));
#273469=CARTESIAN_POINT('Ctrl Pts',(-9.80203322900006,11.6,-4.99492601000001));
#273470=CARTESIAN_POINT('Ctrl Pts',(-9.80412525900006,15.2,-4.99717295500002));
#273471=CARTESIAN_POINT('Ctrl Pts',(-9.80412525900006,11.6,-4.99717295500002));
#273472=CARTESIAN_POINT('Ctrl Pts',(-9.80621906500006,15.2,-4.99942548300002));
#273473=CARTESIAN_POINT('Ctrl Pts',(-9.80621906500006,11.6,-4.99942548300002));
#273474=CARTESIAN_POINT('Ctrl Pts',(-9.80831463700006,15.2,-5.00168359100002));
#273475=CARTESIAN_POINT('Ctrl Pts',(-9.80831463700006,11.6,-5.00168359100002));
#273476=CARTESIAN_POINT('Ctrl Pts',(-9.81041196200006,15.2,-5.00394727800002));
#273477=CARTESIAN_POINT('Ctrl Pts',(-9.81041196200006,11.6,-5.00394727800002));
#273478=CARTESIAN_POINT('Ctrl Pts',(-9.81251102900006,15.2,-5.00621654300001));
#273479=CARTESIAN_POINT('Ctrl Pts',(-9.81251102900006,11.6,-5.00621654300001));
#273480=CARTESIAN_POINT('Ctrl Pts',(-9.81461182700006,15.2,-5.00849138200001));
#273481=CARTESIAN_POINT('Ctrl Pts',(-9.81461182700006,11.6,-5.00849138200001));
#273482=CARTESIAN_POINT('Ctrl Pts',(-9.81671434400005,15.2,-5.01077179600002));
#273483=CARTESIAN_POINT('Ctrl Pts',(-9.81671434400005,11.6,-5.01077179600002));
#273484=CARTESIAN_POINT('Ctrl Pts',(-9.81881856700005,15.2,-5.01305778200001));
#273485=CARTESIAN_POINT('Ctrl Pts',(-9.81881856700005,11.6,-5.01305778200001));
#273486=CARTESIAN_POINT('Ctrl Pts',(-9.82092448700006,15.2,-5.01534933700002));
#273487=CARTESIAN_POINT('Ctrl Pts',(-9.82092448700006,11.6,-5.01534933700002));
#273488=CARTESIAN_POINT('Ctrl Pts',(-9.82303209100006,15.2,-5.01764646100002));
#273489=CARTESIAN_POINT('Ctrl Pts',(-9.82303209100006,11.6,-5.01764646100002));
#273490=CARTESIAN_POINT('Ctrl Pts',(-9.82514136700006,15.2,-5.01994915000001));
#273491=CARTESIAN_POINT('Ctrl Pts',(-9.82514136700006,11.6,-5.01994915000001));
#273492=CARTESIAN_POINT('Ctrl Pts',(-9.82725230400006,15.2,-5.02225740500001));
#273493=CARTESIAN_POINT('Ctrl Pts',(-9.82725230400006,11.6,-5.02225740500001));
#273494=CARTESIAN_POINT('Ctrl Pts',(-9.82936489100006,15.2,-5.02457122300001));
#273495=CARTESIAN_POINT('Ctrl Pts',(-9.82936489100006,11.6,-5.02457122300001));
#273496=CARTESIAN_POINT('Ctrl Pts',(-9.83147911800006,15.2,-5.02689060100002));
#273497=CARTESIAN_POINT('Ctrl Pts',(-9.83147911800006,11.6,-5.02689060100002));
#273498=CARTESIAN_POINT('Ctrl Pts',(-9.83359497000006,15.2,-5.02921553800002));
#273499=CARTESIAN_POINT('Ctrl Pts',(-9.83359497000006,11.6,-5.02921553800002));
#273500=CARTESIAN_POINT('Ctrl Pts',(-9.83571243900006,15.2,-5.03154603200001));
#273501=CARTESIAN_POINT('Ctrl Pts',(-9.83571243900006,11.6,-5.03154603200001));
#273502=CARTESIAN_POINT('Ctrl Pts',(-9.83783151200005,15.2,-5.03388208200001));
#273503=CARTESIAN_POINT('Ctrl Pts',(-9.83783151200005,11.6,-5.03388208200001));
#273504=CARTESIAN_POINT('Ctrl Pts',(-9.83995217700006,15.2,-5.03622368500002));
#273505=CARTESIAN_POINT('Ctrl Pts',(-9.83995217700006,11.6,-5.03622368500002));
#273506=CARTESIAN_POINT('Ctrl Pts',(-9.84207442500006,15.2,-5.03857084000002));
#273507=CARTESIAN_POINT('Ctrl Pts',(-9.84207442500006,11.6,-5.03857084000002));
#273508=CARTESIAN_POINT('Ctrl Pts',(-9.84419824200006,15.2,-5.04092354500001));
#273509=CARTESIAN_POINT('Ctrl Pts',(-9.84419824200006,11.6,-5.04092354500001));
#273510=CARTESIAN_POINT('Ctrl Pts',(-9.84632361900006,15.2,-5.04328179700002));
#273511=CARTESIAN_POINT('Ctrl Pts',(-9.84632361900006,11.6,-5.04328179700002));
#273512=CARTESIAN_POINT('Ctrl Pts',(-9.84845054500006,15.2,-5.04564559600002));
#273513=CARTESIAN_POINT('Ctrl Pts',(-9.84845054500006,11.6,-5.04564559600002));
#273514=CARTESIAN_POINT('Ctrl Pts',(-9.85057900700006,15.2,-5.04801493900001));
#273515=CARTESIAN_POINT('Ctrl Pts',(-9.85057900700006,11.6,-5.04801493900001));
#273516=CARTESIAN_POINT('Ctrl Pts',(-9.85270899400006,15.2,-5.05038982300002));
#273517=CARTESIAN_POINT('Ctrl Pts',(-9.85270899400006,11.6,-5.05038982300002));
#273518=CARTESIAN_POINT('Ctrl Pts',(-9.85484049700006,15.2,-5.05277024800002));
#273519=CARTESIAN_POINT('Ctrl Pts',(-9.85484049700006,11.6,-5.05277024800002));
#273520=CARTESIAN_POINT('Ctrl Pts',(-9.85697350300006,15.2,-5.05515621100002));
#273521=CARTESIAN_POINT('Ctrl Pts',(-9.85697350300006,11.6,-5.05515621100002));
#273522=CARTESIAN_POINT('Ctrl Pts',(-9.85910800200006,15.2,-5.05754771100001));
#273523=CARTESIAN_POINT('Ctrl Pts',(-9.85910800200006,11.6,-5.05754771100001));
#273524=CARTESIAN_POINT('Ctrl Pts',(-9.86124398100005,15.2,-5.05994474600001));
#273525=CARTESIAN_POINT('Ctrl Pts',(-9.86124398100005,11.6,-5.05994474600001));
#273526=CARTESIAN_POINT('Ctrl Pts',(-9.86338143200006,15.2,-5.06234731400002));
#273527=CARTESIAN_POINT('Ctrl Pts',(-9.86338143200006,11.6,-5.06234731400002));
#273528=CARTESIAN_POINT('Ctrl Pts',(-9.86552034100006,15.2,-5.06475541200002));
#273529=CARTESIAN_POINT('Ctrl Pts',(-9.86552034100006,11.6,-5.06475541200002));
#273530=CARTESIAN_POINT('Ctrl Pts',(-9.86766069800005,15.2,-5.06716903800001));
#273531=CARTESIAN_POINT('Ctrl Pts',(-9.86766069800005,11.6,-5.06716903800001));
#273532=CARTESIAN_POINT('Ctrl Pts',(-9.86980249400006,15.2,-5.06958819300001));
#273533=CARTESIAN_POINT('Ctrl Pts',(-9.86980249400006,11.6,-5.06958819300001));
#273534=CARTESIAN_POINT('Ctrl Pts',(-9.87194571500006,15.2,-5.07201287100001));
#273535=CARTESIAN_POINT('Ctrl Pts',(-9.87194571500006,11.6,-5.07201287100001));
#273536=CARTESIAN_POINT('Ctrl Pts',(-9.87409035200006,15.2,-5.07444307400001));
#273537=CARTESIAN_POINT('Ctrl Pts',(-9.87409035200006,11.6,-5.07444307400001));
#273538=CARTESIAN_POINT('Ctrl Pts',(-9.87623639400006,15.2,-5.07687879700002));
#273539=CARTESIAN_POINT('Ctrl Pts',(-9.87623639400006,11.6,-5.07687879700002));
#273540=CARTESIAN_POINT('Ctrl Pts',(-9.87838382900006,15.2,-5.07932003900001));
#273541=CARTESIAN_POINT('Ctrl Pts',(-9.87838382900006,11.6,-5.07932003900001));
#273542=CARTESIAN_POINT('Ctrl Pts',(-9.88053264700006,15.2,-5.08176679900001));
#273543=CARTESIAN_POINT('Ctrl Pts',(-9.88053264700006,11.6,-5.08176679900001));
#273544=CARTESIAN_POINT('Ctrl Pts',(-9.88268283700006,15.2,-5.08421907400002));
#273545=CARTESIAN_POINT('Ctrl Pts',(-9.88268283700006,11.6,-5.08421907400002));
#273546=CARTESIAN_POINT('Ctrl Pts',(-9.88483438900005,15.2,-5.08667686300001));
#273547=CARTESIAN_POINT('Ctrl Pts',(-9.88483438900005,11.6,-5.08667686300001));
#273548=CARTESIAN_POINT('Ctrl Pts',(-9.88698729100006,15.2,-5.08914016200002));
#273549=CARTESIAN_POINT('Ctrl Pts',(-9.88698729100006,11.6,-5.08914016200002));
#273550=CARTESIAN_POINT('Ctrl Pts',(-9.88914153400006,15.2,-5.09160897000001));
#273551=CARTESIAN_POINT('Ctrl Pts',(-9.88914153400006,11.6,-5.09160897000001));
#273552=CARTESIAN_POINT('Ctrl Pts',(-9.89129710500006,15.2,-5.09408328800002));
#273553=CARTESIAN_POINT('Ctrl Pts',(-9.89129710500006,11.6,-5.09408328800002));
#273554=CARTESIAN_POINT('Ctrl Pts',(-9.89345399500005,15.2,-5.09656310900001));
#273555=CARTESIAN_POINT('Ctrl Pts',(-9.89345399500005,11.6,-5.09656310900001));
#273556=CARTESIAN_POINT('Ctrl Pts',(-9.89561219300005,15.2,-5.09904843500002));
#273557=CARTESIAN_POINT('Ctrl Pts',(-9.89561219300005,11.6,-5.09904843500002));
#273558=CARTESIAN_POINT('Ctrl Pts',(-9.89777168700006,15.2,-5.10153926100001));
#273559=CARTESIAN_POINT('Ctrl Pts',(-9.89777168700006,11.6,-5.10153926100001));
#273560=CARTESIAN_POINT('Ctrl Pts',(-9.89993246800006,15.2,-5.10403558800002));
#273561=CARTESIAN_POINT('Ctrl Pts',(-9.89993246800006,11.6,-5.10403558800002));
#273562=CARTESIAN_POINT('Ctrl Pts',(-9.90209452500006,15.2,-5.10653741200001));
#273563=CARTESIAN_POINT('Ctrl Pts',(-9.90209452500006,11.6,-5.10653741200001));
#273564=CARTESIAN_POINT('Ctrl Pts',(-9.90425784700006,15.2,-5.10904473100001));
#273565=CARTESIAN_POINT('Ctrl Pts',(-9.90425784700006,11.6,-5.10904473100001));
#273566=CARTESIAN_POINT('Ctrl Pts',(-9.90642242400006,15.2,-5.11155754400002));
#273567=CARTESIAN_POINT('Ctrl Pts',(-9.90642242400006,11.6,-5.11155754400002));
#273568=CARTESIAN_POINT('Ctrl Pts',(-9.90858824500006,15.2,-5.11407584900001));
#273569=CARTESIAN_POINT('Ctrl Pts',(-9.90858824500006,11.6,-5.11407584900001));
#273570=CARTESIAN_POINT('Ctrl Pts',(-9.91075529900005,15.2,-5.11659964200001));
#273571=CARTESIAN_POINT('Ctrl Pts',(-9.91075529900005,11.6,-5.11659964200001));
#273572=CARTESIAN_POINT('Ctrl Pts',(-9.91292357700006,15.2,-5.11912892300002));
#273573=CARTESIAN_POINT('Ctrl Pts',(-9.91292357700006,11.6,-5.11912892300002));
#273574=CARTESIAN_POINT('Ctrl Pts',(-9.91509306700006,15.2,-5.12166369100001));
#273575=CARTESIAN_POINT('Ctrl Pts',(-9.91509306700006,11.6,-5.12166369100001));
#273576=CARTESIAN_POINT('Ctrl Pts',(-9.91726376000006,15.2,-5.12420394000001));
#273577=CARTESIAN_POINT('Ctrl Pts',(-9.91726376000006,11.6,-5.12420394000001));
#273578=CARTESIAN_POINT('Ctrl Pts',(-9.91943564400006,15.2,-5.12674967200001));
#273579=CARTESIAN_POINT('Ctrl Pts',(-9.91943564400006,11.6,-5.12674967200001));
#273580=CARTESIAN_POINT('Ctrl Pts',(-9.92160871100005,15.2,-5.12930088300001));
#273581=CARTESIAN_POINT('Ctrl Pts',(-9.92160871100005,11.6,-5.12930088300001));
#273582=CARTESIAN_POINT('Ctrl Pts',(-9.92378294700006,15.2,-5.13185757200001));
#273583=CARTESIAN_POINT('Ctrl Pts',(-9.92378294700006,11.6,-5.13185757200001));
#273584=CARTESIAN_POINT('Ctrl Pts',(-9.92595834500005,15.2,-5.13441973500001));
#273585=CARTESIAN_POINT('Ctrl Pts',(-9.92595834500005,11.6,-5.13441973500001));
#273586=CARTESIAN_POINT('Ctrl Pts',(-9.92813489300006,15.2,-5.13698737200002));
#273587=CARTESIAN_POINT('Ctrl Pts',(-9.92813489300006,11.6,-5.13698737200002));
#273588=CARTESIAN_POINT('Ctrl Pts',(-9.93031258000006,15.2,-5.13956048000002));
#273589=CARTESIAN_POINT('Ctrl Pts',(-9.93031258000006,11.6,-5.13956048000002));
#273590=CARTESIAN_POINT('Ctrl Pts',(-9.93249139800006,15.2,-5.14213905700001));
#273591=CARTESIAN_POINT('Ctrl Pts',(-9.93249139800006,11.6,-5.14213905700001));
#273592=CARTESIAN_POINT('Ctrl Pts',(-9.93467133500006,15.2,-5.14472310100002));
#273593=CARTESIAN_POINT('Ctrl Pts',(-9.93467133500006,11.6,-5.14472310100002));
#273594=CARTESIAN_POINT('Ctrl Pts',(-9.93685238200005,15.2,-5.14731261100001));
#273595=CARTESIAN_POINT('Ctrl Pts',(-9.93685238200005,11.6,-5.14731261100001));
#273596=CARTESIAN_POINT('Ctrl Pts',(-9.93903452600006,15.2,-5.14990758300002));
#273597=CARTESIAN_POINT('Ctrl Pts',(-9.93903452600006,11.6,-5.14990758300002));
#273598=CARTESIAN_POINT('Ctrl Pts',(-9.94121776000006,15.2,-5.15250801600001));
#273599=CARTESIAN_POINT('Ctrl Pts',(-9.94121776000006,11.6,-5.15250801600001));
#273600=CARTESIAN_POINT('Ctrl Pts',(-9.94340207300005,15.2,-5.15511390800001));
#273601=CARTESIAN_POINT('Ctrl Pts',(-9.94340207300005,11.6,-5.15511390800001));
#273602=CARTESIAN_POINT('Ctrl Pts',(-9.94558745400006,15.2,-5.15772525700001));
#273603=CARTESIAN_POINT('Ctrl Pts',(-9.94558745400006,11.6,-5.15772525700001));
#273604=CARTESIAN_POINT('Ctrl Pts',(-9.94777389400006,15.2,-5.16034206000001));
#273605=CARTESIAN_POINT('Ctrl Pts',(-9.94777389400006,11.6,-5.16034206000001));
#273606=CARTESIAN_POINT('Ctrl Pts',(-9.94996138000005,15.2,-5.16296431600002));
#273607=CARTESIAN_POINT('Ctrl Pts',(-9.94996138000005,11.6,-5.16296431600002));
#273608=CARTESIAN_POINT('Ctrl Pts',(-9.95214990600006,15.2,-5.16559202200002));
#273609=CARTESIAN_POINT('Ctrl Pts',(-9.95214990600006,11.6,-5.16559202200002));
#273610=CARTESIAN_POINT('Ctrl Pts',(-9.95433945900006,15.2,-5.16822517700001));
#273611=CARTESIAN_POINT('Ctrl Pts',(-9.95433945900006,11.6,-5.16822517700001));
#273612=CARTESIAN_POINT('Ctrl Pts',(-9.95653003000006,15.2,-5.17086377700001));
#273613=CARTESIAN_POINT('Ctrl Pts',(-9.95653003000006,11.6,-5.17086377700001));
#273614=CARTESIAN_POINT('Ctrl Pts',(-9.95872160900005,15.2,-5.17350782200001));
#273615=CARTESIAN_POINT('Ctrl Pts',(-9.95872160900005,11.6,-5.17350782200001));
#273616=CARTESIAN_POINT('Ctrl Pts',(-9.96091418600006,15.2,-5.17615730900001));
#273617=CARTESIAN_POINT('Ctrl Pts',(-9.96091418600006,11.6,-5.17615730900001));
#273618=CARTESIAN_POINT('Ctrl Pts',(-9.96310775000006,15.2,-5.17881223600002));
#273619=CARTESIAN_POINT('Ctrl Pts',(-9.96310775000006,11.6,-5.17881223600002));
#273620=CARTESIAN_POINT('Ctrl Pts',(-9.96530229300006,15.2,-5.18147260100001));
#273621=CARTESIAN_POINT('Ctrl Pts',(-9.96530229300006,11.6,-5.18147260100001));
#273622=CARTESIAN_POINT('Ctrl Pts',(-9.96749780300006,15.2,-5.18413840100001));
#273623=CARTESIAN_POINT('Ctrl Pts',(-9.96749780300006,11.6,-5.18413840100001));
#273624=CARTESIAN_POINT('Ctrl Pts',(-9.96969427100005,15.2,-5.18680963500001));
#273625=CARTESIAN_POINT('Ctrl Pts',(-9.96969427100005,11.6,-5.18680963500001));
#273626=CARTESIAN_POINT('Ctrl Pts',(-9.97189168800006,15.2,-5.18948630000001));
#273627=CARTESIAN_POINT('Ctrl Pts',(-9.97189168800006,11.6,-5.18948630000001));
#273628=CARTESIAN_POINT('Ctrl Pts',(-9.97409004300006,15.2,-5.19216839600002));
#273629=CARTESIAN_POINT('Ctrl Pts',(-9.97409004300006,11.6,-5.19216839600002));
#273630=CARTESIAN_POINT('Ctrl Pts',(-9.97628932500006,15.2,-5.19485591700001));
#273631=CARTESIAN_POINT('Ctrl Pts',(-9.97628932500006,11.6,-5.19485591700001));
#273632=CARTESIAN_POINT('Ctrl Pts',(-9.97848952700006,15.2,-5.19754886400001));
#273633=CARTESIAN_POINT('Ctrl Pts',(-9.97848952700006,11.6,-5.19754886400001));
#273634=CARTESIAN_POINT('Ctrl Pts',(-9.98069063600006,15.2,-5.20024723400001));
#273635=CARTESIAN_POINT('Ctrl Pts',(-9.98069063600006,11.6,-5.20024723400001));
#273636=CARTESIAN_POINT('Ctrl Pts',(-9.98289264400006,15.2,-5.20295102400001));
#273637=CARTESIAN_POINT('Ctrl Pts',(-9.98289264400006,11.6,-5.20295102400001));
#273638=CARTESIAN_POINT('Ctrl Pts',(-9.98509554200006,15.2,-5.20566023400002));
#273639=CARTESIAN_POINT('Ctrl Pts',(-9.98509554200006,11.6,-5.20566023400002));
#273640=CARTESIAN_POINT('Ctrl Pts',(-9.98729931800005,15.2,-5.20837486000001));
#273641=CARTESIAN_POINT('Ctrl Pts',(-9.98729931800005,11.6,-5.20837486000001));
#273642=CARTESIAN_POINT('Ctrl Pts',(-9.98950396400006,15.2,-5.21109489900001));
#273643=CARTESIAN_POINT('Ctrl Pts',(-9.98950396400006,11.6,-5.21109489900001));
#273644=CARTESIAN_POINT('Ctrl Pts',(-9.99170947000006,15.2,-5.21382035100002));
#273645=CARTESIAN_POINT('Ctrl Pts',(-9.99170947000006,11.6,-5.21382035100002));
#273646=CARTESIAN_POINT('Ctrl Pts',(-9.99391582600006,15.2,-5.21655121300002));
#273647=CARTESIAN_POINT('Ctrl Pts',(-9.99391582600006,11.6,-5.21655121300002));
#273648=CARTESIAN_POINT('Ctrl Pts',(-9.99612302200006,15.2,-5.21928748300001));
#273649=CARTESIAN_POINT('Ctrl Pts',(-9.99612302200006,11.6,-5.21928748300001));
#273650=CARTESIAN_POINT('Ctrl Pts',(-9.99833104800006,15.2,-5.22202915700001));
#273651=CARTESIAN_POINT('Ctrl Pts',(-9.99833104800006,11.6,-5.22202915700001));
#273652=CARTESIAN_POINT('Ctrl Pts',(-10.0005398960001,15.2,-5.22477623700001));
#273653=CARTESIAN_POINT('Ctrl Pts',(-10.0005398960001,11.6,-5.22477623700001));
#273654=CARTESIAN_POINT('Ctrl Pts',(-10.0027495550001,15.2,-5.22752871700002));
#273655=CARTESIAN_POINT('Ctrl Pts',(-10.0027495550001,11.6,-5.22752871700002));
#273656=CARTESIAN_POINT('Ctrl Pts',(-10.0049600160001,15.2,-5.23028659500001));
#273657=CARTESIAN_POINT('Ctrl Pts',(-10.0049600160001,11.6,-5.23028659500001));
#273658=CARTESIAN_POINT('Ctrl Pts',(-10.0071712680001,15.2,-5.23304987100001));
#273659=CARTESIAN_POINT('Ctrl Pts',(-10.0071712680001,11.6,-5.23304987100001));
#273660=CARTESIAN_POINT('Ctrl Pts',(-10.0093833030001,15.2,-5.23581854200001));
#273661=CARTESIAN_POINT('Ctrl Pts',(-10.0093833030001,11.6,-5.23581854200001));
#273662=CARTESIAN_POINT('Ctrl Pts',(-10.0115961110001,15.2,-5.23859260400001));
#273663=CARTESIAN_POINT('Ctrl Pts',(-10.0115961110001,11.6,-5.23859260400001));
#273664=CARTESIAN_POINT('Ctrl Pts',(-10.0138096830001,15.2,-5.24137205800002));
#273665=CARTESIAN_POINT('Ctrl Pts',(-10.0138096830001,11.6,-5.24137205800002));
#273666=CARTESIAN_POINT('Ctrl Pts',(-10.0160240080001,15.2,-5.24415689900001));
#273667=CARTESIAN_POINT('Ctrl Pts',(-10.0160240080001,11.6,-5.24415689900001));
#273668=CARTESIAN_POINT('Ctrl Pts',(-10.0182390770001,15.2,-5.24694712600001));
#273669=CARTESIAN_POINT('Ctrl Pts',(-10.0182390770001,11.6,-5.24694712600001));
#273670=CARTESIAN_POINT('Ctrl Pts',(-10.0204548810001,15.2,-5.24974273600002));
#273671=CARTESIAN_POINT('Ctrl Pts',(-10.0204548810001,11.6,-5.24974273600002));
#273672=CARTESIAN_POINT('Ctrl Pts',(-10.0226714120001,15.2,-5.25254372800001));
#273673=CARTESIAN_POINT('Ctrl Pts',(-10.0226714120001,11.6,-5.25254372800001));
#273674=CARTESIAN_POINT('Ctrl Pts',(-10.0248886580001,15.2,-5.25535009900001));
#273675=CARTESIAN_POINT('Ctrl Pts',(-10.0248886580001,11.6,-5.25535009900001));
#273676=CARTESIAN_POINT('Ctrl Pts',(-10.0271066100001,15.2,-5.25816184700002));
#273677=CARTESIAN_POINT('Ctrl Pts',(-10.0271066100001,11.6,-5.25816184700002));
#273678=CARTESIAN_POINT('Ctrl Pts',(-10.0293252590001,15.2,-5.26097897000001));
#273679=CARTESIAN_POINT('Ctrl Pts',(-10.0293252590001,11.6,-5.26097897000001));
#273680=CARTESIAN_POINT('Ctrl Pts',(-10.0315445970001,15.2,-5.26380146500002));
#273681=CARTESIAN_POINT('Ctrl Pts',(-10.0315445970001,11.6,-5.26380146500002));
#273682=CARTESIAN_POINT('Ctrl Pts',(-10.0337646130001,15.2,-5.26662933100001));
#273683=CARTESIAN_POINT('Ctrl Pts',(-10.0337646130001,11.6,-5.26662933100001));
#273684=CARTESIAN_POINT('Ctrl Pts',(-10.0359852980001,15.2,-5.26946256500001));
#273685=CARTESIAN_POINT('Ctrl Pts',(-10.0359852980001,11.6,-5.26946256500001));
#273686=CARTESIAN_POINT('Ctrl Pts',(-10.0382066420001,15.2,-5.27230116500002));
#273687=CARTESIAN_POINT('Ctrl Pts',(-10.0382066420001,11.6,-5.27230116500002));
#273688=CARTESIAN_POINT('Ctrl Pts',(-10.0404286360001,15.2,-5.27514512700002));
#273689=CARTESIAN_POINT('Ctrl Pts',(-10.0404286360001,11.6,-5.27514512700002));
#273690=CARTESIAN_POINT('Ctrl Pts',(-10.0426512720001,15.2,-5.27799445100001));
#273691=CARTESIAN_POINT('Ctrl Pts',(-10.0426512720001,11.6,-5.27799445100001));
#273692=CARTESIAN_POINT('Ctrl Pts',(-10.0448745390001,15.2,-5.28084913400001));
#273693=CARTESIAN_POINT('Ctrl Pts',(-10.0448745390001,11.6,-5.28084913400001));
#273694=CARTESIAN_POINT('Ctrl Pts',(-10.0470984300001,15.2,-5.28370917400002));
#273695=CARTESIAN_POINT('Ctrl Pts',(-10.0470984300001,11.6,-5.28370917400002));
#273696=CARTESIAN_POINT('Ctrl Pts',(-10.0493229330001,15.2,-5.28657456900001));
#273697=CARTESIAN_POINT('Ctrl Pts',(-10.0493229330001,11.6,-5.28657456900001));
#273698=CARTESIAN_POINT('Ctrl Pts',(-10.0515480410001,15.2,-5.28944531500001));
#273699=CARTESIAN_POINT('Ctrl Pts',(-10.0515480410001,11.6,-5.28944531500001));
#273700=CARTESIAN_POINT('Ctrl Pts',(-10.0537737430001,15.2,-5.29232141200001));
#273701=CARTESIAN_POINT('Ctrl Pts',(-10.0537737430001,11.6,-5.29232141200001));
#273702=CARTESIAN_POINT('Ctrl Pts',(-10.0560000300001,15.2,-5.29520285700002));
#273703=CARTESIAN_POINT('Ctrl Pts',(-10.0560000300001,11.6,-5.29520285700002));
#273704=CARTESIAN_POINT('Ctrl Pts',(-10.0582268940001,15.2,-5.29808964700001));
#273705=CARTESIAN_POINT('Ctrl Pts',(-10.0582268940001,11.6,-5.29808964700001));
#273706=CARTESIAN_POINT('Ctrl Pts',(-10.0604543260001,15.2,-5.30098178000001));
#273707=CARTESIAN_POINT('Ctrl Pts',(-10.0604543260001,11.6,-5.30098178000001));
#273708=CARTESIAN_POINT('Ctrl Pts',(-10.0626823150001,15.2,-5.30387925400001));
#273709=CARTESIAN_POINT('Ctrl Pts',(-10.0626823150001,11.6,-5.30387925400001));
#273710=CARTESIAN_POINT('Ctrl Pts',(-10.0649108540001,15.2,-5.30678206600002));
#273711=CARTESIAN_POINT('Ctrl Pts',(-10.0649108540001,11.6,-5.30678206600002));
#273712=CARTESIAN_POINT('Ctrl Pts',(-10.0671399330001,15.2,-5.30969021500002));
#273713=CARTESIAN_POINT('Ctrl Pts',(-10.0671399330001,11.6,-5.30969021500002));
#273714=CARTESIAN_POINT('Ctrl Pts',(-10.0693695420001,15.2,-5.31260369700002));
#273715=CARTESIAN_POINT('Ctrl Pts',(-10.0693695420001,11.6,-5.31260369700002));
#273716=CARTESIAN_POINT('Ctrl Pts',(-10.0715996740001,15.2,-5.31552251300001));
#273717=CARTESIAN_POINT('Ctrl Pts',(-10.0715996740001,11.6,-5.31552251300001));
#273718=CARTESIAN_POINT('Ctrl Pts',(-10.0738303190001,15.2,-5.31844665600001));
#273719=CARTESIAN_POINT('Ctrl Pts',(-10.0738303190001,11.6,-5.31844665600001));
#273720=CARTESIAN_POINT('Ctrl Pts',(-10.0760614660001,15.2,-5.32137612700001));
#273721=CARTESIAN_POINT('Ctrl Pts',(-10.0760614660001,11.6,-5.32137612700001));
#273722=CARTESIAN_POINT('Ctrl Pts',(-10.0782931080001,15.2,-5.32431092300001));
#273723=CARTESIAN_POINT('Ctrl Pts',(-10.0782931080001,11.6,-5.32431092300001));
#273724=CARTESIAN_POINT('Ctrl Pts',(-10.0805252360001,15.2,-5.32725104100002));
#273725=CARTESIAN_POINT('Ctrl Pts',(-10.0805252360001,11.6,-5.32725104100002));
#273726=CARTESIAN_POINT('Ctrl Pts',(-10.0827578410001,15.2,-5.33019648000002));
#273727=CARTESIAN_POINT('Ctrl Pts',(-10.0827578410001,11.6,-5.33019648000002));
#273728=CARTESIAN_POINT('Ctrl Pts',(-10.0849909120001,15.2,-5.33314723600002));
#273729=CARTESIAN_POINT('Ctrl Pts',(-10.0849909120001,11.6,-5.33314723600002));
#273730=CARTESIAN_POINT('Ctrl Pts',(-10.0872244440001,15.2,-5.33610330700002));
#273731=CARTESIAN_POINT('Ctrl Pts',(-10.0872244440001,11.6,-5.33610330700002));
#273732=CARTESIAN_POINT('Ctrl Pts',(-10.0894584250001,15.2,-5.33906469200002));
#273733=CARTESIAN_POINT('Ctrl Pts',(-10.0894584250001,11.6,-5.33906469200002));
#273734=CARTESIAN_POINT('Ctrl Pts',(-10.0916928480001,15.2,-5.34203138700001));
#273735=CARTESIAN_POINT('Ctrl Pts',(-10.0916928480001,11.6,-5.34203138700001));
#273736=CARTESIAN_POINT('Ctrl Pts',(-10.0939277020001,15.2,-5.34500339300001));
#273737=CARTESIAN_POINT('Ctrl Pts',(-10.0939277020001,11.6,-5.34500339300001));
#273738=CARTESIAN_POINT('Ctrl Pts',(-10.0961629820001,15.2,-5.34798070300001));
#273739=CARTESIAN_POINT('Ctrl Pts',(-10.0961629820001,11.6,-5.34798070300001));
#273740=CARTESIAN_POINT('Ctrl Pts',(-10.0983986740001,15.2,-5.35096331800001));
#273741=CARTESIAN_POINT('Ctrl Pts',(-10.0983986740001,11.6,-5.35096331800001));
#273742=CARTESIAN_POINT('Ctrl Pts',(-10.1006347720001,15.2,-5.35395123400002));
#273743=CARTESIAN_POINT('Ctrl Pts',(-10.1006347720001,11.6,-5.35395123400002));
#273744=CARTESIAN_POINT('Ctrl Pts',(-10.1028712650001,15.2,-5.35694444900002));
#273745=CARTESIAN_POINT('Ctrl Pts',(-10.1028712650001,11.6,-5.35694444900002));
#273746=CARTESIAN_POINT('Ctrl Pts',(-10.1051081460001,15.2,-5.35994296100001));
#273747=CARTESIAN_POINT('Ctrl Pts',(-10.1051081460001,11.6,-5.35994296100001));
#273748=CARTESIAN_POINT('Ctrl Pts',(-10.1073454040001,15.2,-5.36294676700001));
#273749=CARTESIAN_POINT('Ctrl Pts',(-10.1073454040001,11.6,-5.36294676700001));
#273750=CARTESIAN_POINT('Ctrl Pts',(-10.1095830330001,15.2,-5.36595586500002));
#273751=CARTESIAN_POINT('Ctrl Pts',(-10.1095830330001,11.6,-5.36595586500002));
#273752=CARTESIAN_POINT('Ctrl Pts',(-10.1118210230001,15.2,-5.36897025200001));
#273753=CARTESIAN_POINT('Ctrl Pts',(-10.1118210230001,11.6,-5.36897025200001));
#273754=CARTESIAN_POINT('Ctrl Pts',(-10.1140593680001,15.2,-5.37198992800001));
#273755=CARTESIAN_POINT('Ctrl Pts',(-10.1140593680001,11.6,-5.37198992800001));
#273756=CARTESIAN_POINT('Ctrl Pts',(-10.1162980580001,15.2,-5.37501489000002));
#273757=CARTESIAN_POINT('Ctrl Pts',(-10.1162980580001,11.6,-5.37501489000002));
#273758=CARTESIAN_POINT('Ctrl Pts',(-10.1185370870001,15.2,-5.37804513400001));
#273759=CARTESIAN_POINT('Ctrl Pts',(-10.1185370870001,11.6,-5.37804513400001));
#273760=CARTESIAN_POINT('Ctrl Pts',(-10.1207764440001,15.2,-5.38108065900001));
#273761=CARTESIAN_POINT('Ctrl Pts',(-10.1207764440001,11.6,-5.38108065900001));
#273762=CARTESIAN_POINT('Ctrl Pts',(-10.1230161200001,15.2,-5.38412146200002));
#273763=CARTESIAN_POINT('Ctrl Pts',(-10.1230161200001,11.6,-5.38412146200002));
#273764=CARTESIAN_POINT('Ctrl Pts',(-10.1252561030001,15.2,-5.38716754100002));
#273765=CARTESIAN_POINT('Ctrl Pts',(-10.1252561030001,11.6,-5.38716754100002));
#273766=CARTESIAN_POINT('Ctrl Pts',(-10.1274963840001,15.2,-5.39021889200002));
#273767=CARTESIAN_POINT('Ctrl Pts',(-10.1274963840001,11.6,-5.39021889200002));
#273768=CARTESIAN_POINT('Ctrl Pts',(-10.1297369520001,15.2,-5.39327551300001));
#273769=CARTESIAN_POINT('Ctrl Pts',(-10.1297369520001,11.6,-5.39327551300001));
#273770=CARTESIAN_POINT('Ctrl Pts',(-10.1319777960001,15.2,-5.39633740000002));
#273771=CARTESIAN_POINT('Ctrl Pts',(-10.1319777960001,11.6,-5.39633740000002));
#273772=CARTESIAN_POINT('Ctrl Pts',(-10.1342189100001,15.2,-5.39940455200002));
#273773=CARTESIAN_POINT('Ctrl Pts',(-10.1342189100001,11.6,-5.39940455200002));
#273774=CARTESIAN_POINT('Ctrl Pts',(-10.1364602890001,15.2,-5.40247696800002));
#273775=CARTESIAN_POINT('Ctrl Pts',(-10.1364602890001,11.6,-5.40247696800002));
#273776=CARTESIAN_POINT('Ctrl Pts',(-10.1387019270001,15.2,-5.40555464300001));
#273777=CARTESIAN_POINT('Ctrl Pts',(-10.1387019270001,11.6,-5.40555464300001));
#273778=CARTESIAN_POINT('Ctrl Pts',(-10.1409438220001,15.2,-5.40863758200001));
#273779=CARTESIAN_POINT('Ctrl Pts',(-10.1409438220001,11.6,-5.40863758200001));
#273780=CARTESIAN_POINT('Ctrl Pts',(-10.1427375440001,15.2,-5.41110814000001));
#273781=CARTESIAN_POINT('Ctrl Pts',(-10.1427375440001,11.6,-5.41110814000001));
#273782=CARTESIAN_POINT('Ctrl Pts',(-10.1440829500001,15.2,-5.41296342600001));
#273783=CARTESIAN_POINT('Ctrl Pts',(-10.1440829500001,11.6,-5.41296342600001));
#273784=CARTESIAN_POINT('Ctrl Pts',(-10.1449799400001,15.2,-5.41420133600001));
#273785=CARTESIAN_POINT('Ctrl Pts',(-10.1449799400001,11.6,-5.41420133600001));
#273786=CARTESIAN_POINT('Ctrl Pts',(-10.1454284470001,15.2,-5.41482055400001));
#273787=CARTESIAN_POINT('Ctrl Pts',(-10.1454284470001,11.6,-5.41482055400001));
#273788=CARTESIAN_POINT('Ctrl Pts',(-9.31239140100006,15.2,-4.57383771200002));
#273789=CARTESIAN_POINT('Ctrl Pts',(-9.31392145135453,15.2,-4.5747602550189));
#273790=CARTESIAN_POINT('Ctrl Pts',(-9.31549767328181,15.2,-4.5757169317027));
#273791=CARTESIAN_POINT('Ctrl Pts',(-9.31711891458909,15.2,-4.57670776794144));
#273792=CARTESIAN_POINT('Ctrl Pts',(-9.31874797434146,15.2,-4.57770338249336));
#273793=CARTESIAN_POINT('Ctrl Pts',(-9.32042248440092,15.2,-4.57873349977316));
#273794=CARTESIAN_POINT('Ctrl Pts',(-9.32214130041636,15.2,-4.57979816338637));
#273795=CARTESIAN_POINT('Ctrl Pts',(-9.32386011627568,15.2,-4.58086282690287));
#273796=CARTESIAN_POINT('Ctrl Pts',(-9.32562323899895,15.2,-4.58196203944949));
#273797=CARTESIAN_POINT('Ctrl Pts',(-9.32742955676663,15.2,-4.58309584749161));
#273798=CARTESIAN_POINT('Ctrl Pts',(-9.32923587453431,15.2,-4.58422965553373));
#273799=CARTESIAN_POINT('Ctrl Pts',(-9.33108538730214,15.1999999999999,
-4.5853980568443));
#273800=CARTESIAN_POINT('Ctrl Pts',(-9.33297701357543,15.2,-4.58660109210866));
#273801=CARTESIAN_POINT('Ctrl Pts',(-9.33486864002055,15.2,-4.5878041274823));
#273802=CARTESIAN_POINT('Ctrl Pts',(-9.3368023827215,15.2,-4.58904179825028));
#273803=CARTESIAN_POINT('Ctrl Pts',(-9.33877718899858,15.2,-4.59031413865532));
#273804=CARTESIAN_POINT('Ctrl Pts',(-9.3407519950963,15.2,-4.59158647894478));
#273805=CARTESIAN_POINT('Ctrl Pts',(-9.34276786524956,15.2,-4.59289349118482));
#273806=CARTESIAN_POINT('Ctrl Pts',(-9.34482377851759,15.2,-4.59423520622557));
#273807=CARTESIAN_POINT('Ctrl Pts',(-9.34687969178564,15.2,-4.59557692126631));
#273808=CARTESIAN_POINT('Ctrl Pts',(-9.34897564777141,15.2,-4.59695334018431));
#273809=CARTESIAN_POINT('Ctrl Pts',(-9.3511106521088,15.2,-4.59836449038153));
#273810=CARTESIAN_POINT('Ctrl Pts',(-9.35324565664012,15.2,-4.59977564070692));
#273811=CARTESIAN_POINT('Ctrl Pts',(-9.35541970904296,15.2,-4.60122152401996));
#273812=CARTESIAN_POINT('Ctrl Pts',(-9.35763184074945,15.2,-4.60270216418635));
#273813=CARTESIAN_POINT('Ctrl Pts',(-9.35984397225501,15.2,-4.60418280421825));
#273814=CARTESIAN_POINT('Ctrl Pts',(-9.36209418289796,15.2,-4.60569820177273));
#273815=CARTESIAN_POINT('Ctrl Pts',(-9.36438152939981,15.2,-4.60724837688458));
#273816=CARTESIAN_POINT('Ctrl Pts',(-9.36666887590164,15.2,-4.60879855199643));
#273817=CARTESIAN_POINT('Ctrl Pts',(-9.36899335821715,15.2,-4.61038350755551));
#273818=CARTESIAN_POINT('Ctrl Pts',(-9.37135405587983,15.2,-4.61200325866183));
#273819=CARTESIAN_POINT('Ctrl Pts',(-9.3737147535425,15.2,-4.61362300976815));
#273820=CARTESIAN_POINT('Ctrl Pts',(-9.37611166665067,15.2,-4.61527755752124));
#273821=CARTESIAN_POINT('Ctrl Pts',(-9.37854389747655,15.2,-4.61696691654082));
#273822=CARTESIAN_POINT('Ctrl Pts',(-9.38097612852336,15.2,-4.61865627571385));
#273823=CARTESIAN_POINT('Ctrl Pts',(-9.38344367732367,15.2,-4.62038044747359));
#273824=CARTESIAN_POINT('Ctrl Pts',(-9.38594566837816,15.2,-4.6221394416543));
#273825=CARTESIAN_POINT('Ctrl Pts',(-9.38844765920541,15.2,-4.62389843567523));
#273826=CARTESIAN_POINT('Ctrl Pts',(-9.39098409293896,15.2,-4.62569225337402));
#273827=CARTESIAN_POINT('Ctrl Pts',(-9.3935541129405,15.2,-4.62752090148246));
#273828=CARTESIAN_POINT('Ctrl Pts',(-9.39612413294204,15.2,-4.62934954959089));
#273829=CARTESIAN_POINT('Ctrl Pts',(-9.39872774117737,15.2,-4.63121303114775));
#273830=CARTESIAN_POINT('Ctrl Pts',(-9.40136410124598,15.2,-4.63311134807638));
#273831=CARTESIAN_POINT('Ctrl Pts',(-9.40400046155406,15.2,-4.63500966517743));
#273832=CARTESIAN_POINT('Ctrl Pts',(-9.40666957427374,15.2,-4.63694281996525));
#273833=CARTESIAN_POINT('Ctrl Pts',(-9.40937062267234,15.2,-4.63891081407403));
#273834=CARTESIAN_POINT('Ctrl Pts',(-9.4120716708256,15.2,-4.64087880800404));
#273835=CARTESIAN_POINT('Ctrl Pts',(-9.4148046571617,15.2,-4.64288164279723));
#273836=CARTESIAN_POINT('Ctrl Pts',(-9.41756878149041,15.2,-4.64491931573237));
#273837=CARTESIAN_POINT('Ctrl Pts',(-9.42033290581914,15.2,-4.64695698866751));
#273838=CARTESIAN_POINT('Ctrl Pts',(-9.42312816853842,15.2,-4.64902950149088));
#273839=CARTESIAN_POINT('Ctrl Pts',(-9.42595379268368,15.2,-4.65113685049526));
#273840=CARTESIAN_POINT('Ctrl Pts',(-9.42877941708561,15.2,-4.65324419969107));
#273841=CARTESIAN_POINT('Ctrl Pts',(-9.4316353997261,15.2,-4.65538638539788));
#273842=CARTESIAN_POINT('Ctrl Pts',(-9.43452097952922,15.2,-4.65756340246064));
#273843=CARTESIAN_POINT('Ctrl Pts',(-9.43740655907024,15.2,-4.65974041932565));
#273844=CARTESIAN_POINT('Ctrl Pts',(-9.44032173581531,15.2,-4.66195226643992));
#273845=CARTESIAN_POINT('Ctrl Pts',(-9.44326576245833,15.2,-4.66419893644161));
#273846=CARTESIAN_POINT('Ctrl Pts',(-9.44620978910137,15.2,-4.66644560644331));
#273847=CARTESIAN_POINT('Ctrl Pts',(-9.4491826676622,15.2,-4.66872709947977));
#273848=CARTESIAN_POINT('Ctrl Pts',(-9.45218366545143,15.2,-4.6710434045093));
#273849=CARTESIAN_POINT('Ctrl Pts',(-9.45518466351327,15.2,-4.67335970974922));
#273850=CARTESIAN_POINT('Ctrl Pts',(-9.45821378240637,15.2,-4.67571082796929));
#273851=CARTESIAN_POINT('Ctrl Pts',(-9.46127030532485,15.2,-4.67809674501836));
#273852=CARTESIAN_POINT('Ctrl Pts',(-9.46432682796567,15.2,-4.68048266185072));
#273853=CARTESIAN_POINT('Ctrl Pts',(-9.46741075545025,15.2,-4.68290337572906));
#273854=CARTESIAN_POINT('Ctrl Pts',(-9.47052138718476,15.2,-4.68535887548441));
#273855=CARTESIAN_POINT('Ctrl Pts',(-9.47363201891927,15.2,-4.68781437523976));
#273856=CARTESIAN_POINT('Ctrl Pts',(-9.47676935546881,15.2,-4.69030465833076));
#273857=CARTESIAN_POINT('Ctrl Pts',(-9.47993270826938,15.2,-4.69282970715415));
#273858=CARTESIAN_POINT('Ctrl Pts',(-9.48256883569898,15.2,-4.69493391458343));
#273859=CARTESIAN_POINT('Ctrl Pts',(-9.48522303133183,15.2,-4.69706226520502));
#273860=CARTESIAN_POINT('Ctrl Pts',(-9.48789490535871,15.2,-4.69921474763433));
#273861=CARTESIAN_POINT('Ctrl Pts',(-9.49056677938559,15.2,-4.70136723006365));
#273862=CARTESIAN_POINT('Ctrl Pts',(-9.49325633158075,15.2,-4.70354384381107));
#273863=CARTESIAN_POINT('Ctrl Pts',(-9.49596317673188,15.2,-4.70574457701543));
#273864=CARTESIAN_POINT('Ctrl Pts',(-9.498670021883,15.2,-4.70794531021979));
#273865=CARTESIAN_POINT('Ctrl Pts',(-9.50139416162778,15.2,-4.71017016276661));
#273866=CARTESIAN_POINT('Ctrl Pts',(-9.50413521822501,15.2,-4.71241912026661));
#273867=CARTESIAN_POINT('Ctrl Pts',(-9.50687627482223,15.2,-4.71466807776662));
#273868=CARTESIAN_POINT('Ctrl Pts',(-9.50963424783888,15.2,-4.71694114255182));
#273869=CARTESIAN_POINT('Ctrl Pts',(-9.51240876618487,15.2,-4.71923829749288));
#273870=CARTESIAN_POINT('Ctrl Pts',(-9.51518328453086,15.2,-4.72153545243395));
#273871=CARTESIAN_POINT('Ctrl Pts',(-9.51797434851064,15.2,-4.72385669852445));
#273872=CARTESIAN_POINT('Ctrl Pts',(-9.52078159115037,15.2,-4.72620202088682));
#273873=CARTESIAN_POINT('Ctrl Pts',(-9.52358883379011,15.2,-4.72854734324919));
#273874=CARTESIAN_POINT('Ctrl Pts',(-9.52641225669053,15.2,-4.73091674053871));
#273875=CARTESIAN_POINT('Ctrl Pts',(-9.52925149842746,15.2,-4.73331019866496));
#273876=CARTESIAN_POINT('Ctrl Pts',(-9.53209074016441,15.2,-4.73570365679122));
#273877=CARTESIAN_POINT('Ctrl Pts',(-9.53494580164996,15.2,-4.7381211734154));
#273878=CARTESIAN_POINT('Ctrl Pts',(-9.53781632776663,15.2,-4.7405627325668));
#273879=CARTESIAN_POINT('Ctrl Pts',(-9.54068685388331,15.2,-4.7430042917182));
#273880=CARTESIAN_POINT('Ctrl Pts',(-9.54357284573936,15.2,-4.74546989288476));
#273881=CARTESIAN_POINT('Ctrl Pts',(-9.54647395337948,15.2,-4.74795951781727));
#273882=CARTESIAN_POINT('Ctrl Pts',(-9.54937506101962,15.2,-4.75044914274978));
#273883=CARTESIAN_POINT('Ctrl Pts',(-9.55229128489328,15.2,-4.7529627916299));
#273884=CARTESIAN_POINT('Ctrl Pts',(-9.55522228086673,15.2,-4.75550044559022));
#273885=CARTESIAN_POINT('Ctrl Pts',(-9.55815327652072,15.2,-4.75803809927393));
#273886=CARTESIAN_POINT('Ctrl Pts',(-9.56109904385334,15.2,-4.76059975770666));
#273887=CARTESIAN_POINT('Ctrl Pts',(-9.5640592454045,15.2,-4.76318540068676));
#273888=CARTESIAN_POINT('Ctrl Pts',(-9.56701944727832,15.2,-4.7657710439487));
#273889=CARTESIAN_POINT('Ctrl Pts',(-9.56999408261026,15.2,-4.76838067303523));
#273890=CARTESIAN_POINT('Ctrl Pts',(-9.57298281781743,15.2,-4.77101426463048));
#273891=CARTESIAN_POINT('Ctrl Pts',(-9.57597155302458,15.2,-4.77364785622573));
#273892=CARTESIAN_POINT('Ctrl Pts',(-9.57897438660657,15.2,-4.77630541294561));
#273893=CARTESIAN_POINT('Ctrl Pts',(-9.58199099264712,15.2,-4.77898691037422));
#273894=CARTESIAN_POINT('Ctrl Pts',(-9.58561092009308,15.2,-4.78220470746392));
#273895=CARTESIAN_POINT('Ctrl Pts',(-9.58925067816236,15.2,-4.78545698304766));
#273896=CARTESIAN_POINT('Ctrl Pts',(-9.59290970512903,15.2,-4.78874369530966));
#273897=CARTESIAN_POINT('Ctrl Pts',(-9.59595889410176,15.2,-4.79148262204539));
#273898=CARTESIAN_POINT('Ctrl Pts',(-9.59902146667348,15.2,-4.79424546467918));
#273899=CARTESIAN_POINT('Ctrl Pts',(-9.60209710216066,15.2,-4.79703219863947));
#273900=CARTESIAN_POINT('Ctrl Pts',(-9.60455761034924,15.2,-4.79926158562544));
#273901=CARTESIAN_POINT('Ctrl Pts',(-9.6070264804701,15.2,-4.80150626259555));
#273902=CARTESIAN_POINT('Ctrl Pts',(-9.6095035493226,15.2,-4.80376621829868));
#273903=CARTESIAN_POINT('Ctrl Pts',(-9.61198061851259,15.2,-4.80602617430972));
#273904=CARTESIAN_POINT('Ctrl Pts',(-9.61446588758684,15.2,-4.80830140910293));
#273905=CARTESIAN_POINT('Ctrl Pts',(-9.6169591975702,15.2,-4.81059190856574));
#273906=CARTESIAN_POINT('Ctrl Pts',(-9.61945250721385,15.2,-4.81288240771646));
#273907=CARTESIAN_POINT('Ctrl Pts',(-9.62195385795338,15.2,-4.8151881740372));
#273908=CARTESIAN_POINT('Ctrl Pts',(-9.62446309080331,15.2,-4.81750919056869));
#273909=CARTESIAN_POINT('Ctrl Pts',(-9.62697232399511,15.2,-4.81983020741642));
#273910=CARTESIAN_POINT('Ctrl Pts',(-9.62948943990175,15.2,-4.82216647831043));
#273911=CARTESIAN_POINT('Ctrl Pts',(-9.6320142837065,15.2,-4.82451798771733));
#273912=CARTESIAN_POINT('Ctrl Pts',(-9.63453912716724,15.2,-4.82686949680385));
#273913=CARTESIAN_POINT('Ctrl Pts',(-9.63707169781845,15.2,-4.82923624555923));
#273914=CARTESIAN_POINT('Ctrl Pts',(-9.63961184084815,15.2,-4.83161821937107));
#273915=CARTESIAN_POINT('Ctrl Pts',(-9.64215198422393,15.2,-4.83400019350745));
#273916=CARTESIAN_POINT('Ctrl Pts',(-9.6446997014748,15.2,-4.83639739330373));
#273917=CARTESIAN_POINT('Ctrl Pts',(-9.64725483872565,15.2,-4.83880980521398));
#273918=CARTESIAN_POINT('Ctrl Pts',(-9.64980997562837,15.2,-4.84122221679555));
#273919=CARTESIAN_POINT('Ctrl Pts',(-9.65237253334902,15.2,-4.84364983922404));
#273920=CARTESIAN_POINT('Ctrl Pts',(-9.65494236030487,15.2,-4.84609266013389));
#273921=CARTESIAN_POINT('Ctrl Pts',(-9.65751218761084,15.2,-4.84853548137659));
#273922=CARTESIAN_POINT('Ctrl Pts',(-9.66008928519087,15.2,-4.85099349973058));
#273923=CARTESIAN_POINT('Ctrl Pts',(-9.66267350251012,15.2,-4.85346670104331));
#273924=CARTESIAN_POINT('Ctrl Pts',(-9.66525771947728,15.2,-4.85593990201906));
#273925=CARTESIAN_POINT('Ctrl Pts',(-9.66784905781333,15.2,-4.85842828513574));
#273926=CARTESIAN_POINT('Ctrl Pts',(-9.67044736810021,15.2,-4.86093183737397));
#273927=CARTESIAN_POINT('Ctrl Pts',(-9.6730456787411,15.2,-4.8634353899533));
#273928=CARTESIAN_POINT('Ctrl Pts',(-9.67565096202709,15.2,-4.86595411054239));
#273929=CARTESIAN_POINT('Ctrl Pts',(-9.67826307255836,15.2,-4.86848798395828));
#273930=CARTESIAN_POINT('Ctrl Pts',(-9.68087518308964,15.2,-4.87102185737418));
#273931=CARTESIAN_POINT('Ctrl Pts',(-9.68349411927721,15.2,-4.87357088540569));
#273932=CARTESIAN_POINT('Ctrl Pts',(-9.68611973792099,15.2,-4.87613504943587));
#273933=CARTESIAN_POINT('Ctrl Pts',(-9.68874535620702,15.2,-4.87869921311667));
#273934=CARTESIAN_POINT('Ctrl Pts',(-9.69137765681035,15.2,-4.88127851637635));
#273935=CARTESIAN_POINT('Ctrl Pts',(-9.69401649577323,15.2,-4.88387294073152));
#273936=CARTESIAN_POINT('Ctrl Pts',(-9.69665533509566,15.2,-4.88646736544018));
#273937=CARTESIAN_POINT('Ctrl Pts',(-9.69930071320232,15.2,-4.88907691257618));
#273938=CARTESIAN_POINT('Ctrl Pts',(-9.70195248795859,15.2,-4.89170156588742));
#273939=CARTESIAN_POINT('Ctrl Pts',(-9.70460426235357,15.2,-4.89432621884106));
#273940=CARTESIAN_POINT('Ctrl Pts',(-9.70726243379217,15.2,-4.89696597790942));
#273941=CARTESIAN_POINT('Ctrl Pts',(-9.70992686274061,15.2,-4.89962082752473));
#273942=CARTESIAN_POINT('Ctrl Pts',(-9.71259129205207,15.2,-4.90227567750177));
#273943=CARTESIAN_POINT('Ctrl Pts',(-9.71526197812224,15.2,-4.90494561756343));
#273944=CARTESIAN_POINT('Ctrl Pts',(-9.71793878168015,15.2,-4.90763063162299));
#273945=CARTESIAN_POINT('Ctrl Pts',(-9.72128478594518,15.2,-4.91098689901451));
#273946=CARTESIAN_POINT('Ctrl Pts',(-9.7246403505394,15.2,-4.91436671868765));
#273947=CARTESIAN_POINT('Ctrl Pts',(-9.72800520470683,15.2,-4.91777005924512));
#273948=CARTESIAN_POINT('Ctrl Pts',(-9.73137005887425,15.2,-4.9211733998026));
#273949=CARTESIAN_POINT('Ctrl Pts',(-9.73474420335293,15.2,-4.92460025986046));
#273950=CARTESIAN_POINT('Ctrl Pts',(-9.73812737495089,15.2,-4.92805060791794));
#273951=CARTESIAN_POINT('Ctrl Pts',(-9.74083391200801,15.2,-4.93081088613827));
#273952=CARTESIAN_POINT('Ctrl Pts',(-9.74354622543582,15.2,-4.93358619639133));
#273953=CARTESIAN_POINT('Ctrl Pts',(-9.74626418178152,15.2,-4.93637652006472));
#273954=CARTESIAN_POINT('Ctrl Pts',(-9.74898213849753,15.2,-4.9391668441183));
#273955=CARTESIAN_POINT('Ctrl Pts',(-9.75170573663861,15.2,-4.94197218401417));
#273956=CARTESIAN_POINT('Ctrl Pts',(-9.75443484595458,15.2,-4.94479252000276));
#273957=CARTESIAN_POINT('Ctrl Pts',(-9.75716395489872,15.2,-4.94761285560708));
#273958=CARTESIAN_POINT('Ctrl Pts',(-9.75989857169488,15.2,-4.95044818819274));
#273959=CARTESIAN_POINT('Ctrl Pts',(-9.76263856802609,15.2,-4.95329849979209));
#273960=CARTESIAN_POINT('Ctrl Pts',(-9.76537856473063,15.2,-4.95614881177979));
#273961=CARTESIAN_POINT('Ctrl Pts',(-9.76812393932808,15.2,-4.95901410334082));
#273962=CARTESIAN_POINT('Ctrl Pts',(-9.77087456161587,15.2,-4.96189435614299));
#273963=CARTESIAN_POINT('Ctrl Pts',(-9.77362518352887,15.2,-4.96477460855272));
#273964=CARTESIAN_POINT('Ctrl Pts',(-9.77638105387264,15.2,-4.96766982170941));
#273965=CARTESIAN_POINT('Ctrl Pts',(-9.77914204175771,15.2,-4.97057997797052));
#273966=CARTESIAN_POINT('Ctrl Pts',(-9.78190303001894,15.2,-4.97349013462814));
#273967=CARTESIAN_POINT('Ctrl Pts',(-9.78466913800581,15.2,-4.9764152353709));
#273968=CARTESIAN_POINT('Ctrl Pts',(-9.78744023676829,15.2,-4.97935526003212));
#273969=CARTESIAN_POINT('Ctrl Pts',(-9.79021133515321,15.2,-4.98229528429275));
#273970=CARTESIAN_POINT('Ctrl Pts',(-9.79298742348709,15.2,-4.98525023270316));
#273971=CARTESIAN_POINT('Ctrl Pts',(-9.79576837653703,15.2,-4.9882200870144));
#273972=CARTESIAN_POINT('Ctrl Pts',(-9.79854932996587,15.2,-4.99118994173029));
#273973=CARTESIAN_POINT('Ctrl Pts',(-9.80133514680659,15.2,-4.9941747022415));
#273974=CARTESIAN_POINT('Ctrl Pts',(-9.80412570302694,15.2,-4.99717435075201));
#273975=CARTESIAN_POINT('Ctrl Pts',(-9.80691625886708,15.2,-5.00017399885381));
#273976=CARTESIAN_POINT('Ctrl Pts',(-9.80971155279107,15.2,-5.0031885337955));
#273977=CARTESIAN_POINT('Ctrl Pts',(-9.81251146128392,15.2,-5.00621793604632));
#273978=CARTESIAN_POINT('Ctrl Pts',(-9.81531137015826,15.2,-5.0092473387099));
#273979=CARTESIAN_POINT('Ctrl Pts',(-9.81811589324418,15.2,-5.01229160993879));
#273980=CARTESIAN_POINT('Ctrl Pts',(-9.82092490800837,15.2,-5.01535072921662));
#273981=CARTESIAN_POINT('Ctrl Pts',(-9.82373392277256,15.2,-5.01840984849443));
#273982=CARTESIAN_POINT('Ctrl Pts',(-9.82654742665396,15.2,-5.02148381624067));
#273983=CARTESIAN_POINT('Ctrl Pts',(-9.8293653014191,15.2,-5.02457261352165));
#273984=CARTESIAN_POINT('Ctrl Pts',(-9.8321831758003,15.2,-5.02766141038177));
#273985=CARTESIAN_POINT('Ctrl Pts',(-9.83500541940801,15.2,-5.0307650353942));
#273986=CARTESIAN_POINT('Ctrl Pts',(-9.83783191002311,15.2,-5.0338834702645));
#273987=CARTESIAN_POINT('Ctrl Pts',(-9.84065840102332,15.2,-5.03700190555969));
#273988=CARTESIAN_POINT('Ctrl Pts',(-9.84348913920863,15.2,-5.04013515023326));
#273989=CARTESIAN_POINT('Ctrl Pts',(-9.84632400669687,15.2,-5.04328318423967));
#273990=CARTESIAN_POINT('Ctrl Pts',(-9.84915887379886,15.2,-5.04643121781715));
#273991=CARTESIAN_POINT('Ctrl Pts',(-9.85199786805311,15.2,-5.04959404073994));
#273992=CARTESIAN_POINT('Ctrl Pts',(-9.85484087254266,15.2,-5.052771632257));
#273993=CARTESIAN_POINT('Ctrl Pts',(-9.85768387741957,15.2,-5.055949224207));
#273994=CARTESIAN_POINT('Ctrl Pts',(-9.86053089131561,15.2,-5.05914158624857));
#273995=CARTESIAN_POINT('Ctrl Pts',(-9.86338179694708,15.2,-5.06234869697374));
#273996=CARTESIAN_POINT('Ctrl Pts',(-9.86694542879219,15.2,-5.06635758516173));
#273997=CARTESIAN_POINT('Ctrl Pts',(-9.87051513947279,15.2,-5.07038951664512));
#273998=CARTESIAN_POINT('Ctrl Pts',(-9.8740907037094,15.2,-5.07444445456368));
#273999=CARTESIAN_POINT('Ctrl Pts',(-9.87695115486483,15.2,-5.07768840463335));
#274000=CARTESIAN_POINT('Ctrl Pts',(-9.87981535070587,15.2,-5.08094707675383));
#274001=CARTESIAN_POINT('Ctrl Pts',(-9.88268317724897,15.2,-5.0842204522075));
#274002=CARTESIAN_POINT('Ctrl Pts',(-9.88555100418281,15.2,-5.08749382810716));
#274003=CARTESIAN_POINT('Ctrl Pts',(-9.88842246196105,15.2,-5.09078190490244));
#274004=CARTESIAN_POINT('Ctrl Pts',(-9.89129743515057,15.2,-5.09408466430429));
#274005=CARTESIAN_POINT('Ctrl Pts',(-9.89417240794838,15.2,-5.09738742325614));
#274006=CARTESIAN_POINT('Ctrl Pts',(-9.89705089622251,15.2,-5.10070486193438));
#274007=CARTESIAN_POINT('Ctrl Pts',(-9.89993278676448,15.2,-5.10403696199437));
#274008=CARTESIAN_POINT('Ctrl Pts',(-9.90281467769911,15.2,-5.10736906250835));
#274009=CARTESIAN_POINT('Ctrl Pts',(-9.90569997112302,15.2,-5.11071582267962));
#274010=CARTESIAN_POINT('Ctrl Pts',(-9.90858855350288,15.2,-5.11407722130822));
#274011=CARTESIAN_POINT('Ctrl Pts',(-9.91147713548918,15.2,-5.11743861947884));
#274012=CARTESIAN_POINT('Ctrl Pts',(-9.91436900723339,15.2,-5.1208146564282));
#274013=CARTESIAN_POINT('Ctrl Pts',(-9.91726405736331,15.2,-5.12420531020803));
#274014=CARTESIAN_POINT('Ctrl Pts',(-9.91943534505935,15.2,-5.1267483006584));
#274015=CARTESIAN_POINT('Ctrl Pts',(-9.92160842085518,15.2,-5.12929951423611));
#274016=CARTESIAN_POINT('Ctrl Pts',(-9.92378323698427,15.2,-5.13185893997534));
#274017=CARTESIAN_POINT('Ctrl Pts',(-9.92595805350845,15.2,-5.13441836617954));
#274018=CARTESIAN_POINT('Ctrl Pts',(-9.9281346112081,15.2,-5.13698600510269));
#274019=CARTESIAN_POINT('Ctrl Pts',(-9.93031286319157,15.2,-5.1395618478115));
#274020=CARTESIAN_POINT('Ctrl Pts',(-9.93249111477933,15.2,-5.14213769005236));
#274021=CARTESIAN_POINT('Ctrl Pts',(-9.93467106195033,15.2,-5.14472173610946));
#274022=CARTESIAN_POINT('Ctrl Pts',(-9.93685265653787,15.2,-5.14731397680765));
#274023=CARTESIAN_POINT('Ctrl Pts',(-9.93903425112541,15.2,-5.14990621750584));
#274024=CARTESIAN_POINT('Ctrl Pts',(-9.94121749392148,15.2,-5.15250665203523));
#274025=CARTESIAN_POINT('Ctrl Pts',(-9.9434023400187,15.2,-5.155115272244));
#274026=CARTESIAN_POINT('Ctrl Pts',(-9.94558718611591,15.2,-5.15772389245277));
#274027=CARTESIAN_POINT('Ctrl Pts',(-9.94777363480096,15.2,-5.1603406977644));
#274028=CARTESIAN_POINT('Ctrl Pts',(-9.94996163993972,15.2,-5.16296567851424));
#274029=CARTESIAN_POINT('Ctrl Pts',(-9.95214964507848,15.2,-5.16559065926408));
#274030=CARTESIAN_POINT('Ctrl Pts',(-9.95433920767431,15.2,-5.16822381565886));
#274031=CARTESIAN_POINT('Ctrl Pts',(-9.95653028176125,15.2,-5.17086513793719));
#274032=CARTESIAN_POINT('Ctrl Pts',(-9.95872135584818,15.2,-5.17350646021553));
#274033=CARTESIAN_POINT('Ctrl Pts',(-9.96091394165166,15.2,-5.17615594921828));
#274034=CARTESIAN_POINT('Ctrl Pts',(-9.96310799423841,15.2,-5.17881359491226));
#274035=CARTESIAN_POINT('Ctrl Pts',(-9.96530204722373,15.2,-5.18147124108905));
#274036=CARTESIAN_POINT('Ctrl Pts',(-9.96749756672617,15.2,-5.18413704359317));
#274037=CARTESIAN_POINT('Ctrl Pts',(-9.96969450871231,15.2,-5.18681099335788));
#274038=CARTESIAN_POINT('Ctrl Pts',(-9.97189145029933,15.2,-5.18948494263682));
#274039=CARTESIAN_POINT('Ctrl Pts',(-9.97408981417886,15.2,-5.19216704003293));
#274040=CARTESIAN_POINT('Ctrl Pts',(-9.97628955537565,15.2,-5.1948572739872));
#274041=CARTESIAN_POINT('Ctrl Pts',(-9.97995579083685,15.2,-5.1993409974072));
#274042=CARTESIAN_POINT('Ctrl Pts',(-9.98362585221359,15.2,-5.20384732657383));
#274043=CARTESIAN_POINT('Ctrl Pts',(-9.9872995359639,15.2,-5.20837621386734));
#274044=CARTESIAN_POINT('Ctrl Pts',(-9.989503746134,15.2,-5.21109354614473));
#274045=CARTESIAN_POINT('Ctrl Pts',(-9.99170926115401,15.2,-5.21381899963));
#274046=CARTESIAN_POINT('Ctrl Pts',(-9.99391603624061,15.2,-5.21655256528139));
#274047=CARTESIAN_POINT('Ctrl Pts',(-9.9961228113272,15.2,-5.21928613093277));
#274048=CARTESIAN_POINT('Ctrl Pts',(-9.9983308461723,15.2,-5.22202780745652));
#274049=CARTESIAN_POINT('Ctrl Pts',(-10.0005400987687,15.2,-5.22477758703579));
#274050=CARTESIAN_POINT('Ctrl Pts',(-10.0027493513651,15.2,-5.22752736661506));
#274051=CARTESIAN_POINT('Ctrl Pts',(-10.0049598210517,15.2,-5.23028524661876));
#274052=CARTESIAN_POINT('Ctrl Pts',(-10.0071714637314,15.2,-5.23305121973911));
#274053=CARTESIAN_POINT('Ctrl Pts',(-10.0093831064111,15.2,-5.23581719285947));
#274054=CARTESIAN_POINT('Ctrl Pts',(-10.0115959234393,15.2,-5.23859125733195));
#274055=CARTESIAN_POINT('Ctrl Pts',(-10.0138098710254,15.2,-5.24137340448017));
#274056=CARTESIAN_POINT('Ctrl Pts',(-10.0160238186115,15.2,-5.24415555162838));
#274057=CARTESIAN_POINT('Ctrl Pts',(-10.0182388956476,15.2,-5.24694578014271));
#274058=CARTESIAN_POINT('Ctrl Pts',(-10.0204550622336,15.2,-5.24974408087327));
#274059=CARTESIAN_POINT('Ctrl Pts',(-10.0226712292222,15.2,-5.25254238211218));
#274060=CARTESIAN_POINT('Ctrl Pts',(-10.0248884846278,15.2,-5.25534875565338));
#274061=CARTESIAN_POINT('Ctrl Pts',(-10.027106784742,15.2,-5.25816319135518));
#274062=CARTESIAN_POINT('Ctrl Pts',(-10.0293250844532,15.2,-5.26097762654569));
#274063=CARTESIAN_POINT('Ctrl Pts',(-10.031544430856,15.2,-5.26380012362741));
#274064=CARTESIAN_POINT('Ctrl Pts',(-10.0337647804838,15.2,-5.26663067331696));
#274065=CARTESIAN_POINT('Ctrl Pts',(-10.0359851301115,15.2,-5.2694612230065));
#274066=CARTESIAN_POINT('Ctrl Pts',(-10.0382064823394,15.2,-5.27229982469302));
#274067=CARTESIAN_POINT('Ctrl Pts',(-10.0404287964771,15.2,-5.27514646747755));
#274068=CARTESIAN_POINT('Ctrl Pts',(-10.0426511106147,15.2,-5.27799311026207));
#274069=CARTESIAN_POINT('Ctrl Pts',(-10.0448743869021,15.2,-5.28084779557175));
#274070=CARTESIAN_POINT('Ctrl Pts',(-10.0470985830397,15.2,-5.28371051273069));
#274071=CARTESIAN_POINT('Ctrl Pts',(-10.0500641781592,15.2,-5.28752746928932));
#274072=CARTESIAN_POINT('Ctrl Pts',(-10.0530314081763,15.2,-5.29135870395377));
#274073=CARTESIAN_POINT('Ctrl Pts',(-10.0560001747271,15.2,-5.29520419388704));
#274074=CARTESIAN_POINT('Ctrl Pts',(-10.058226749438,15.2,-5.29808831107501));
#274075=CARTESIAN_POINT('Ctrl Pts',(-10.0604541895072,15.2,-5.30098044610422));
#274076=CARTESIAN_POINT('Ctrl Pts',(-10.0626824527179,15.2,-5.30388058883287));
#274077=CARTESIAN_POINT('Ctrl Pts',(-10.0649107159287,15.2,-5.30678073156153));
#274078=CARTESIAN_POINT('Ctrl Pts',(-10.0671398030063,15.2,-5.30968888177863));
#274079=CARTESIAN_POINT('Ctrl Pts',(-10.0693696727271,15.2,-5.31260503043594));
#274080=CARTESIAN_POINT('Ctrl Pts',(-10.0715995424479,15.2,-5.31552117909326));
#274081=CARTESIAN_POINT('Ctrl Pts',(-10.073830195969,15.2,-5.31844532509055));
#274082=CARTESIAN_POINT('Ctrl Pts',(-10.0760615897314,15.2,-5.3213774582473));
#274083=CARTESIAN_POINT('Ctrl Pts',(-10.0782929834937,15.2,-5.32430959140405));
#274084=CARTESIAN_POINT('Ctrl Pts',(-10.0805251200545,15.2,-5.32724971180322));
#274085=CARTESIAN_POINT('Ctrl Pts',(-10.0827579573067,15.2,-5.33019780894542));
#274086=CARTESIAN_POINT('Ctrl Pts',(-10.0849907945588,15.2,-5.33314590608762));
#274087=CARTESIAN_POINT('Ctrl Pts',(-10.0872243338109,15.2,-5.33610197912926));
#274088=CARTESIAN_POINT('Ctrl Pts',(-10.0894585349797,15.2,-5.33906601889547));
#274089=CARTESIAN_POINT('Ctrl Pts',(-10.0916927365543,15.2,-5.34203005920015));
#274090=CARTESIAN_POINT('Ctrl Pts',(-10.0939276000624,15.2,-5.34500206704876));
#274091=CARTESIAN_POINT('Ctrl Pts',(-10.0961630855541,15.2,-5.34798202985793));
#274092=CARTESIAN_POINT('Ctrl Pts',(-10.0991437321994,15.2,-5.35195531270122));
#274093=CARTESIAN_POINT('Ctrl Pts',(-10.1021254821311,15.2,-5.355942739759));
#274094=CARTESIAN_POINT('Ctrl Pts',(-10.1051082402897,15.2,-5.35994428450557));
#274095=CARTESIAN_POINT('Ctrl Pts',(-10.1073453090102,15.2,-5.3629454432018));
#274096=CARTESIAN_POINT('Ctrl Pts',(-10.1095829447208,15.2,-5.36595454263154));
#274097=CARTESIAN_POINT('Ctrl Pts',(-10.1118211114728,15.2,-5.36897157389624));
#274098=CARTESIAN_POINT('Ctrl Pts',(-10.1140592782247,15.2,-5.37198860516093));
#274099=CARTESIAN_POINT('Ctrl Pts',(-10.1162979764433,15.2,-5.37501356935007));
#274100=CARTESIAN_POINT('Ctrl Pts',(-10.1185371685286,15.2,-5.37804645357213));
#274101=CARTESIAN_POINT('Ctrl Pts',(-10.1207763610206,15.2,-5.38107933834516));
#274102=CARTESIAN_POINT('Ctrl Pts',(-10.1230160464794,15.2,-5.3841201444871));
#274103=CARTESIAN_POINT('Ctrl Pts',(-10.1252561779717,15.2,-5.38716885968126));
#274104=CARTESIAN_POINT('Ctrl Pts',(-10.1274963090571,15.2,-5.39021757432157));
#274105=CARTESIAN_POINT('Ctrl Pts',(-10.1297368853697,15.2,-5.3932741973836));
#274106=CARTESIAN_POINT('Ctrl Pts',(-10.131977863942,15.2,-5.39633871684295));
#274107=CARTESIAN_POINT('Ctrl Pts',(-10.1342188425142,15.2,-5.3994032363023));
#274108=CARTESIAN_POINT('Ctrl Pts',(-10.1364602251632,15.2,-5.40247565238601));
#274109=CARTESIAN_POINT('Ctrl Pts',(-10.1387019915142,15.2,-5.40555595924693));
#274110=CARTESIAN_POINT('Ctrl Pts',(-10.1409437578652,15.2,-5.40863626610785));
#274111=CARTESIAN_POINT('Ctrl Pts',(-10.1431859115927,15.2,-5.41172446343756));
#274112=CARTESIAN_POINT('Ctrl Pts',(-10.1454284470001,15.2,-5.41482055400001));
#274113=CARTESIAN_POINT('Ctrl Pts',(-9.31239140100006,12.2,-4.57383771200002));
#274114=CARTESIAN_POINT('Ctrl Pts',(-9.31392145135453,12.2,-4.5747602550189));
#274115=CARTESIAN_POINT('Ctrl Pts',(-9.31549767328181,12.2,-4.5757169317027));
#274116=CARTESIAN_POINT('Ctrl Pts',(-9.31711891458909,12.2,-4.57670776794144));
#274117=CARTESIAN_POINT('Ctrl Pts',(-9.31874797434146,12.2,-4.57770338249336));
#274118=CARTESIAN_POINT('Ctrl Pts',(-9.32042248440092,12.2,-4.57873349977316));
#274119=CARTESIAN_POINT('Ctrl Pts',(-9.32214130041636,12.2,-4.57979816338637));
#274120=CARTESIAN_POINT('Ctrl Pts',(-9.32386011627568,12.2,-4.58086282690287));
#274121=CARTESIAN_POINT('Ctrl Pts',(-9.32562323899895,12.2,-4.58196203944949));
#274122=CARTESIAN_POINT('Ctrl Pts',(-9.32742955676663,12.2,-4.58309584749161));
#274123=CARTESIAN_POINT('Ctrl Pts',(-9.32923587453431,12.2,-4.58422965553373));
#274124=CARTESIAN_POINT('Ctrl Pts',(-9.33108538730214,12.2,-4.5853980568443));
#274125=CARTESIAN_POINT('Ctrl Pts',(-9.33297701357543,12.2,-4.58660109210866));
#274126=CARTESIAN_POINT('Ctrl Pts',(-9.33486864002055,12.2,-4.5878041274823));
#274127=CARTESIAN_POINT('Ctrl Pts',(-9.3368023827215,12.2,-4.58904179825028));
#274128=CARTESIAN_POINT('Ctrl Pts',(-9.33877718899858,12.2,-4.59031413865532));
#274129=CARTESIAN_POINT('Ctrl Pts',(-9.3407519950963,12.2,-4.59158647894478));
#274130=CARTESIAN_POINT('Ctrl Pts',(-9.34276786524956,12.2,-4.59289349118482));
#274131=CARTESIAN_POINT('Ctrl Pts',(-9.34482377851759,12.2,-4.59423520622557));
#274132=CARTESIAN_POINT('Ctrl Pts',(-9.34687969178564,12.2,-4.59557692126631));
#274133=CARTESIAN_POINT('Ctrl Pts',(-9.34897564777141,12.2,-4.59695334018431));
#274134=CARTESIAN_POINT('Ctrl Pts',(-9.3511106521088,12.2,-4.59836449038153));
#274135=CARTESIAN_POINT('Ctrl Pts',(-9.35324565664012,12.2,-4.59977564070692));
#274136=CARTESIAN_POINT('Ctrl Pts',(-9.35541970904296,12.2,-4.60122152401996));
#274137=CARTESIAN_POINT('Ctrl Pts',(-9.35763184074945,12.2,-4.60270216418635));
#274138=CARTESIAN_POINT('Ctrl Pts',(-9.35984397225501,12.2,-4.60418280421825));
#274139=CARTESIAN_POINT('Ctrl Pts',(-9.36209418289797,12.2,-4.60569820177273));
#274140=CARTESIAN_POINT('Ctrl Pts',(-9.36438152939981,12.2,-4.60724837688458));
#274141=CARTESIAN_POINT('Ctrl Pts',(-9.36666887590164,12.2,-4.60879855199643));
#274142=CARTESIAN_POINT('Ctrl Pts',(-9.36899335821715,12.2,-4.61038350755551));
#274143=CARTESIAN_POINT('Ctrl Pts',(-9.37135405587982,12.2,-4.61200325866183));
#274144=CARTESIAN_POINT('Ctrl Pts',(-9.3737147535425,12.2,-4.61362300976815));
#274145=CARTESIAN_POINT('Ctrl Pts',(-9.37611166665068,12.2,-4.61527755752125));
#274146=CARTESIAN_POINT('Ctrl Pts',(-9.37854389747655,12.2,-4.61696691654082));
#274147=CARTESIAN_POINT('Ctrl Pts',(-9.38097612852336,12.2,-4.61865627571385));
#274148=CARTESIAN_POINT('Ctrl Pts',(-9.38344367732366,12.2,-4.62038044747359));
#274149=CARTESIAN_POINT('Ctrl Pts',(-9.38594566837816,12.2,-4.6221394416543));
#274150=CARTESIAN_POINT('Ctrl Pts',(-9.38844765920541,12.2,-4.62389843567522));
#274151=CARTESIAN_POINT('Ctrl Pts',(-9.39098409293896,12.2,-4.62569225337401));
#274152=CARTESIAN_POINT('Ctrl Pts',(-9.39355411294049,12.2,-4.62752090148245));
#274153=CARTESIAN_POINT('Ctrl Pts',(-9.39612413294203,12.2,-4.62934954959089));
#274154=CARTESIAN_POINT('Ctrl Pts',(-9.39872774117737,12.2,-4.63121303114775));
#274155=CARTESIAN_POINT('Ctrl Pts',(-9.40136410124598,12.2,-4.63311134807638));
#274156=CARTESIAN_POINT('Ctrl Pts',(-9.40400046155406,12.2,-4.63500966517744));
#274157=CARTESIAN_POINT('Ctrl Pts',(-9.40666957427374,12.2,-4.63694281996525));
#274158=CARTESIAN_POINT('Ctrl Pts',(-9.40937062267235,12.2,-4.63891081407403));
#274159=CARTESIAN_POINT('Ctrl Pts',(-9.4120716708256,12.2,-4.64087880800404));
#274160=CARTESIAN_POINT('Ctrl Pts',(-9.4148046571617,12.2,-4.64288164279723));
#274161=CARTESIAN_POINT('Ctrl Pts',(-9.41756878149041,12.2,-4.64491931573237));
#274162=CARTESIAN_POINT('Ctrl Pts',(-9.42033290581914,12.2,-4.64695698866751));
#274163=CARTESIAN_POINT('Ctrl Pts',(-9.42312816853842,12.2,-4.64902950149087));
#274164=CARTESIAN_POINT('Ctrl Pts',(-9.42595379268368,12.2,-4.65113685049526));
#274165=CARTESIAN_POINT('Ctrl Pts',(-9.42877941708561,12.2,-4.65324419969107));
#274166=CARTESIAN_POINT('Ctrl Pts',(-9.4316353997261,12.2,-4.65538638539789));
#274167=CARTESIAN_POINT('Ctrl Pts',(-9.43452097952923,12.2,-4.65756340246064));
#274168=CARTESIAN_POINT('Ctrl Pts',(-9.43740655907025,12.2,-4.65974041932565));
#274169=CARTESIAN_POINT('Ctrl Pts',(-9.44032173581533,12.2,-4.66195226643993));
#274170=CARTESIAN_POINT('Ctrl Pts',(-9.44326576245835,12.2,-4.66419893644163));
#274171=CARTESIAN_POINT('Ctrl Pts',(-9.44620978910138,12.2,-4.66644560644333));
#274172=CARTESIAN_POINT('Ctrl Pts',(-9.4491826676622,12.2,-4.66872709947977));
#274173=CARTESIAN_POINT('Ctrl Pts',(-9.45218366545143,12.2,-4.6710434045093));
#274174=CARTESIAN_POINT('Ctrl Pts',(-9.45518466351327,12.2,-4.67335970974922));
#274175=CARTESIAN_POINT('Ctrl Pts',(-9.45821378240637,12.2,-4.67571082796928));
#274176=CARTESIAN_POINT('Ctrl Pts',(-9.46127030532485,12.2,-4.67809674501836));
#274177=CARTESIAN_POINT('Ctrl Pts',(-9.46432682796567,12.2,-4.68048266185072));
#274178=CARTESIAN_POINT('Ctrl Pts',(-9.46741075545025,12.2,-4.68290337572907));
#274179=CARTESIAN_POINT('Ctrl Pts',(-9.47052138718476,12.2,-4.68535887548441));
#274180=CARTESIAN_POINT('Ctrl Pts',(-9.47363201891927,12.2,-4.68781437523976));
#274181=CARTESIAN_POINT('Ctrl Pts',(-9.4767693554688,12.2,-4.69030465833076));
#274182=CARTESIAN_POINT('Ctrl Pts',(-9.47993270826938,12.2,-4.69282970715415));
#274183=CARTESIAN_POINT('Ctrl Pts',(-9.48256883569897,12.2,-4.69493391458342));
#274184=CARTESIAN_POINT('Ctrl Pts',(-9.48522303133183,12.2,-4.69706226520502));
#274185=CARTESIAN_POINT('Ctrl Pts',(-9.48789490535872,12.2,-4.69921474763433));
#274186=CARTESIAN_POINT('Ctrl Pts',(-9.49056677938559,12.2,-4.70136723006365));
#274187=CARTESIAN_POINT('Ctrl Pts',(-9.49325633158075,12.2,-4.70354384381107));
#274188=CARTESIAN_POINT('Ctrl Pts',(-9.49596317673188,12.2,-4.70574457701543));
#274189=CARTESIAN_POINT('Ctrl Pts',(-9.498670021883,12.2,-4.70794531021979));
#274190=CARTESIAN_POINT('Ctrl Pts',(-9.50139416162778,12.2,-4.71017016276662));
#274191=CARTESIAN_POINT('Ctrl Pts',(-9.50413521822501,12.2,-4.71241912026662));
#274192=CARTESIAN_POINT('Ctrl Pts',(-9.50687627482223,12.2,-4.71466807776662));
#274193=CARTESIAN_POINT('Ctrl Pts',(-9.50963424783887,12.2,-4.71694114255181));
#274194=CARTESIAN_POINT('Ctrl Pts',(-9.51240876618487,12.2,-4.71923829749288));
#274195=CARTESIAN_POINT('Ctrl Pts',(-9.51518328453086,12.2,-4.72153545243394));
#274196=CARTESIAN_POINT('Ctrl Pts',(-9.51797434851064,12.2,-4.72385669852444));
#274197=CARTESIAN_POINT('Ctrl Pts',(-9.52078159115037,12.2,-4.72620202088682));
#274198=CARTESIAN_POINT('Ctrl Pts',(-9.52358883379011,12.2,-4.72854734324919));
#274199=CARTESIAN_POINT('Ctrl Pts',(-9.52641225669053,12.2,-4.73091674053871));
#274200=CARTESIAN_POINT('Ctrl Pts',(-9.52925149842746,12.2,-4.73331019866497));
#274201=CARTESIAN_POINT('Ctrl Pts',(-9.53209074016441,12.2,-4.73570365679122));
#274202=CARTESIAN_POINT('Ctrl Pts',(-9.53494580164996,12.2,-4.7381211734154));
#274203=CARTESIAN_POINT('Ctrl Pts',(-9.53781632776663,12.2,-4.7405627325668));
#274204=CARTESIAN_POINT('Ctrl Pts',(-9.54068685388331,12.2,-4.7430042917182));
#274205=CARTESIAN_POINT('Ctrl Pts',(-9.54357284573936,12.2,-4.74546989288476));
#274206=CARTESIAN_POINT('Ctrl Pts',(-9.54647395337949,12.2,-4.74795951781727));
#274207=CARTESIAN_POINT('Ctrl Pts',(-9.54937506101962,12.2,-4.75044914274978));
#274208=CARTESIAN_POINT('Ctrl Pts',(-9.55229128489328,12.2,-4.7529627916299));
#274209=CARTESIAN_POINT('Ctrl Pts',(-9.55522228086673,12.2,-4.75550044559022));
#274210=CARTESIAN_POINT('Ctrl Pts',(-9.55815327652072,12.2,-4.75803809927394));
#274211=CARTESIAN_POINT('Ctrl Pts',(-9.56109904385334,12.2,-4.76059975770666));
#274212=CARTESIAN_POINT('Ctrl Pts',(-9.5640592454045,12.2,-4.76318540068676));
#274213=CARTESIAN_POINT('Ctrl Pts',(-9.56701944727832,12.2,-4.7657710439487));
#274214=CARTESIAN_POINT('Ctrl Pts',(-9.56999408261026,12.2,-4.76838067303523));
#274215=CARTESIAN_POINT('Ctrl Pts',(-9.57298281781743,12.2,-4.77101426463048));
#274216=CARTESIAN_POINT('Ctrl Pts',(-9.57597155302458,12.2,-4.77364785622573));
#274217=CARTESIAN_POINT('Ctrl Pts',(-9.57897438660656,12.2,-4.7763054129456));
#274218=CARTESIAN_POINT('Ctrl Pts',(-9.58199099264712,12.2,-4.77898691037422));
#274219=CARTESIAN_POINT('Ctrl Pts',(-9.58500759868768,12.2,-4.78166840780283));
#274220=CARTESIAN_POINT('Ctrl Pts',(-9.58803797563447,12.2,-4.78437384870405));
#274221=CARTESIAN_POINT('Ctrl Pts',(-9.59108179939673,12.2,-4.78710320869987));
#274222=CARTESIAN_POINT('Ctrl Pts',(-9.59412562315899,12.2,-4.78983256869569));
#274223=CARTESIAN_POINT('Ctrl Pts',(-9.59718289253887,12.2,-4.79258584833639));
#274224=CARTESIAN_POINT('Ctrl Pts',(-9.60025329031597,12.2,-4.79536302479347));
#274225=CARTESIAN_POINT('Ctrl Pts',(-9.60332368809306,12.2,-4.79814020125056));
#274226=CARTESIAN_POINT('Ctrl Pts',(-9.60640721300385,12.2,-4.80094127343883));
#274227=CARTESIAN_POINT('Ctrl Pts',(-9.6095035493226,12.2,-4.80376621829868));
#274228=CARTESIAN_POINT('Ctrl Pts',(-9.6119806185126,12.2,-4.80602617430972));
#274229=CARTESIAN_POINT('Ctrl Pts',(-9.61446588758683,12.2,-4.80830140910293));
#274230=CARTESIAN_POINT('Ctrl Pts',(-9.61695919757019,12.2,-4.81059190856574));
#274231=CARTESIAN_POINT('Ctrl Pts',(-9.61945250721385,12.2,-4.81288240771646));
#274232=CARTESIAN_POINT('Ctrl Pts',(-9.62195385795338,12.2,-4.8151881740372));
#274233=CARTESIAN_POINT('Ctrl Pts',(-9.6244630908033,12.2,-4.81750919056869));
#274234=CARTESIAN_POINT('Ctrl Pts',(-9.62697232399511,12.2,-4.81983020741642));
#274235=CARTESIAN_POINT('Ctrl Pts',(-9.62948943990175,12.2,-4.82216647831043));
#274236=CARTESIAN_POINT('Ctrl Pts',(-9.6320142837065,12.2,-4.82451798771733));
#274237=CARTESIAN_POINT('Ctrl Pts',(-9.63453912716724,12.2,-4.82686949680385));
#274238=CARTESIAN_POINT('Ctrl Pts',(-9.63707169781845,12.2,-4.82923624555923));
#274239=CARTESIAN_POINT('Ctrl Pts',(-9.63961184084815,12.2,-4.83161821937107));
#274240=CARTESIAN_POINT('Ctrl Pts',(-9.64215198422393,12.2,-4.83400019350745));
#274241=CARTESIAN_POINT('Ctrl Pts',(-9.6446997014748,12.2,-4.83639739330373));
#274242=CARTESIAN_POINT('Ctrl Pts',(-9.64725483872565,12.2,-4.83880980521398));
#274243=CARTESIAN_POINT('Ctrl Pts',(-9.64980997562837,12.2,-4.84122221679555));
#274244=CARTESIAN_POINT('Ctrl Pts',(-9.65237253334902,12.2,-4.84364983922403));
#274245=CARTESIAN_POINT('Ctrl Pts',(-9.65494236030486,12.2,-4.84609266013389));
#274246=CARTESIAN_POINT('Ctrl Pts',(-9.65751218761083,12.2,-4.84853548137658));
#274247=CARTESIAN_POINT('Ctrl Pts',(-9.66008928519087,12.2,-4.85099349973058));
#274248=CARTESIAN_POINT('Ctrl Pts',(-9.66267350251012,12.2,-4.85346670104331));
#274249=CARTESIAN_POINT('Ctrl Pts',(-9.66525771947728,12.2,-4.85593990201906));
#274250=CARTESIAN_POINT('Ctrl Pts',(-9.66784905781333,12.2,-4.85842828513574));
#274251=CARTESIAN_POINT('Ctrl Pts',(-9.67044736810021,12.2,-4.86093183737397));
#274252=CARTESIAN_POINT('Ctrl Pts',(-9.6730456787411,12.2,-4.8634353899533));
#274253=CARTESIAN_POINT('Ctrl Pts',(-9.67565096202709,12.2,-4.86595411054239));
#274254=CARTESIAN_POINT('Ctrl Pts',(-9.67826307255836,12.2,-4.86848798395828));
#274255=CARTESIAN_POINT('Ctrl Pts',(-9.68087518308964,12.2,-4.87102185737418));
#274256=CARTESIAN_POINT('Ctrl Pts',(-9.68349411927721,12.2,-4.87357088540569));
#274257=CARTESIAN_POINT('Ctrl Pts',(-9.68611973792099,12.2,-4.87613504943587));
#274258=CARTESIAN_POINT('Ctrl Pts',(-9.68874535620702,12.2,-4.87869921311667));
#274259=CARTESIAN_POINT('Ctrl Pts',(-9.69137765681035,12.2,-4.88127851637635));
#274260=CARTESIAN_POINT('Ctrl Pts',(-9.69401649577323,12.2,-4.88387294073152));
#274261=CARTESIAN_POINT('Ctrl Pts',(-9.69665533509566,12.2,-4.88646736544018));
#274262=CARTESIAN_POINT('Ctrl Pts',(-9.69930071320232,12.2,-4.88907691257618));
#274263=CARTESIAN_POINT('Ctrl Pts',(-9.70195248795859,12.2,-4.89170156588742));
#274264=CARTESIAN_POINT('Ctrl Pts',(-9.70460426235357,12.2,-4.89432621884106));
#274265=CARTESIAN_POINT('Ctrl Pts',(-9.70726243379217,12.2,-4.89696597790942));
#274266=CARTESIAN_POINT('Ctrl Pts',(-9.70992686274061,12.2,-4.89962082752473));
#274267=CARTESIAN_POINT('Ctrl Pts',(-9.71259129205207,12.2,-4.90227567750177));
#274268=CARTESIAN_POINT('Ctrl Pts',(-9.71526197812224,12.2,-4.90494561756343));
#274269=CARTESIAN_POINT('Ctrl Pts',(-9.71793878168015,12.2,-4.90763063162299));
#274270=CARTESIAN_POINT('Ctrl Pts',(-9.72061558487334,12.2,-4.9103156453167));
#274271=CARTESIAN_POINT('Ctrl Pts',(-9.72329850607269,12.2,-4.91301573183997));
#274272=CARTESIAN_POINT('Ctrl Pts',(-9.72598740829694,12.2,-4.91573087672814));
#274273=CARTESIAN_POINT('Ctrl Pts',(-9.72867631088753,12.2,-4.91844602198624));
#274274=CARTESIAN_POINT('Ctrl Pts',(-9.73137119228999,12.2,-4.92117622362949));
#274275=CARTESIAN_POINT('Ctrl Pts',(-9.73407191843753,12.2,-4.92392146622452));
#274276=CARTESIAN_POINT('Ctrl Pts',(-9.73677264421712,12.2,-4.9266667084455));
#274277=CARTESIAN_POINT('Ctrl Pts',(-9.73947921572654,12.2,-4.92942699090073));
#274278=CARTESIAN_POINT('Ctrl Pts',(-9.74219149563983,12.2,-4.932202296089));
#274279=CARTESIAN_POINT('Ctrl Pts',(-9.74490377592268,12.2,-4.93497760165539));
#274280=CARTESIAN_POINT('Ctrl Pts',(-9.74762176627394,12.2,-4.93776792979501));
#274281=CARTESIAN_POINT('Ctrl Pts',(-9.75034533175607,12.2,-4.94057326500444));
#274282=CARTESIAN_POINT('Ctrl Pts',(-9.75306889686712,12.2,-4.94337859983163));
#274283=CARTESIAN_POINT('Ctrl Pts',(-9.75579803931316,12.2,-4.94619893957527));
#274284=CARTESIAN_POINT('Ctrl Pts',(-9.75853262381126,12.2,-4.94903426778638));
#274285=CARTESIAN_POINT('Ctrl Pts',(-9.76126720868195,12.2,-4.95186959638382));
#274286=CARTESIAN_POINT('Ctrl Pts',(-9.76400723812036,12.2,-4.95471991250215));
#274287=CARTESIAN_POINT('Ctrl Pts',(-9.7667525802269,12.2,-4.95758519972691));
#274288=CARTESIAN_POINT('Ctrl Pts',(-9.76949792195939,12.2,-4.96045048656128));
#274289=CARTESIAN_POINT('Ctrl Pts',(-9.77224857603917,12.2,-4.96333074362037));
#274290=CARTESIAN_POINT('Ctrl Pts',(-9.77500441375779,12.2,-4.96622595249326));
#274291=CARTESIAN_POINT('Ctrl Pts',(-9.77776025185188,12.2,-4.96912116176063));
#274292=CARTESIAN_POINT('Ctrl Pts',(-9.78052127223538,12.2,-4.97203132285163));
#274293=CARTESIAN_POINT('Ctrl Pts',(-9.78328734777504,12.2,-4.97495641823329));
#274294=CARTESIAN_POINT('Ctrl Pts',(-9.78743646070764,12.2,-4.97934406090722));
#274295=CARTESIAN_POINT('Ctrl Pts',(-9.79159694677267,12.2,-4.98376530534521));
#274296=CARTESIAN_POINT('Ctrl Pts',(-9.79576837653703,12.2,-4.9882200870144));
#274297=CARTESIAN_POINT('Ctrl Pts',(-9.79854932996587,12.2,-4.99118994173029));
#274298=CARTESIAN_POINT('Ctrl Pts',(-9.80133514680659,12.2,-4.9941747022415));
#274299=CARTESIAN_POINT('Ctrl Pts',(-9.80412570302694,12.2,-4.997174350752));
#274300=CARTESIAN_POINT('Ctrl Pts',(-9.80691625886708,12.2,-5.00017399885381));
#274301=CARTESIAN_POINT('Ctrl Pts',(-9.80971155279107,12.2,-5.0031885337955));
#274302=CARTESIAN_POINT('Ctrl Pts',(-9.81251146128392,12.2,-5.00621793604632));
#274303=CARTESIAN_POINT('Ctrl Pts',(-9.81531137015826,12.2,-5.0092473387099));
#274304=CARTESIAN_POINT('Ctrl Pts',(-9.81811589324418,12.2,-5.01229160993879));
#274305=CARTESIAN_POINT('Ctrl Pts',(-9.82092490800837,12.2,-5.01535072921662));
#274306=CARTESIAN_POINT('Ctrl Pts',(-9.82373392277256,12.2,-5.01840984849443));
#274307=CARTESIAN_POINT('Ctrl Pts',(-9.82654742665396,12.2,-5.02148381624067));
#274308=CARTESIAN_POINT('Ctrl Pts',(-9.8293653014191,12.2,-5.02457261352165));
#274309=CARTESIAN_POINT('Ctrl Pts',(-9.8321831758003,12.2,-5.02766141038177));
#274310=CARTESIAN_POINT('Ctrl Pts',(-9.83500541940801,12.2,-5.0307650353942));
#274311=CARTESIAN_POINT('Ctrl Pts',(-9.83783191002311,12.2,-5.0338834702645));
#274312=CARTESIAN_POINT('Ctrl Pts',(-9.84065840102332,12.2,-5.03700190555969));
#274313=CARTESIAN_POINT('Ctrl Pts',(-9.84348913920863,12.2,-5.04013515023326));
#274314=CARTESIAN_POINT('Ctrl Pts',(-9.84632400669687,12.2,-5.04328318423967));
#274315=CARTESIAN_POINT('Ctrl Pts',(-9.84915887379886,12.2,-5.04643121781715));
#274316=CARTESIAN_POINT('Ctrl Pts',(-9.85199786805311,12.2,-5.04959404073994));
#274317=CARTESIAN_POINT('Ctrl Pts',(-9.85484087254266,12.2,-5.052771632257));
#274318=CARTESIAN_POINT('Ctrl Pts',(-9.85839462844512,12.2,-5.05674362197803));
#274319=CARTESIAN_POINT('Ctrl Pts',(-9.86195464930968,12.2,-5.06073869074068));
#274320=CARTESIAN_POINT('Ctrl Pts',(-9.86552070300643,12.2,-5.06475679402278));
#274321=CARTESIAN_POINT('Ctrl Pts',(-9.86837354611931,12.2,-5.06797127682365));
#274322=CARTESIAN_POINT('Ctrl Pts',(-9.87123025216421,12.2,-5.07120050405204));
#274323=CARTESIAN_POINT('Ctrl Pts',(-9.8740907037094,12.2,-5.07444445456368));
#274324=CARTESIAN_POINT('Ctrl Pts',(-9.87695115486483,12.2,-5.07768840463335));
#274325=CARTESIAN_POINT('Ctrl Pts',(-9.87981535070587,12.2,-5.08094707675383));
#274326=CARTESIAN_POINT('Ctrl Pts',(-9.88268317724897,12.2,-5.0842204522075));
#274327=CARTESIAN_POINT('Ctrl Pts',(-9.88555100418281,12.2,-5.08749382810716));
#274328=CARTESIAN_POINT('Ctrl Pts',(-9.88842246196105,12.2,-5.09078190490244));
#274329=CARTESIAN_POINT('Ctrl Pts',(-9.89129743515057,12.2,-5.09408466430429));
#274330=CARTESIAN_POINT('Ctrl Pts',(-9.89417240794838,12.2,-5.09738742325614));
#274331=CARTESIAN_POINT('Ctrl Pts',(-9.89705089622251,12.2,-5.10070486193438));
#274332=CARTESIAN_POINT('Ctrl Pts',(-9.89993278676448,12.2,-5.10403696199437));
#274333=CARTESIAN_POINT('Ctrl Pts',(-9.90281467769911,12.2,-5.10736906250835));
#274334=CARTESIAN_POINT('Ctrl Pts',(-9.90569997112302,12.2,-5.11071582267963));
#274335=CARTESIAN_POINT('Ctrl Pts',(-9.90858855350289,12.2,-5.11407722130823));
#274336=CARTESIAN_POINT('Ctrl Pts',(-9.91147713548918,12.2,-5.11743861947885));
#274337=CARTESIAN_POINT('Ctrl Pts',(-9.91436900723339,12.2,-5.1208146564282));
#274338=CARTESIAN_POINT('Ctrl Pts',(-9.91726405736331,12.2,-5.12420531020803));
#274339=CARTESIAN_POINT('Ctrl Pts',(-9.91943534505935,12.2,-5.1267483006584));
#274340=CARTESIAN_POINT('Ctrl Pts',(-9.92160842085518,12.2,-5.12929951423611));
#274341=CARTESIAN_POINT('Ctrl Pts',(-9.92378323698427,12.2,-5.13185893997534));
#274342=CARTESIAN_POINT('Ctrl Pts',(-9.92595805350845,12.2,-5.13441836617954));
#274343=CARTESIAN_POINT('Ctrl Pts',(-9.9281346112081,12.2,-5.13698600510269));
#274344=CARTESIAN_POINT('Ctrl Pts',(-9.93031286319157,12.2,-5.1395618478115));
#274345=CARTESIAN_POINT('Ctrl Pts',(-9.93249111477933,12.2,-5.14213769005236));
#274346=CARTESIAN_POINT('Ctrl Pts',(-9.93467106195033,12.2,-5.14472173610946));
#274347=CARTESIAN_POINT('Ctrl Pts',(-9.93685265653787,12.2,-5.14731397680765));
#274348=CARTESIAN_POINT('Ctrl Pts',(-9.93903425112541,12.2,-5.14990621750584));
#274349=CARTESIAN_POINT('Ctrl Pts',(-9.94121749392148,12.2,-5.15250665203523));
#274350=CARTESIAN_POINT('Ctrl Pts',(-9.9434023400187,12.2,-5.155115272244));
#274351=CARTESIAN_POINT('Ctrl Pts',(-9.94558718611591,12.2,-5.15772389245277));
#274352=CARTESIAN_POINT('Ctrl Pts',(-9.94777363480096,12.2,-5.1603406977644));
#274353=CARTESIAN_POINT('Ctrl Pts',(-9.94996163993972,12.2,-5.16296567851424));
#274354=CARTESIAN_POINT('Ctrl Pts',(-9.95214964507848,12.2,-5.16559065926408));
#274355=CARTESIAN_POINT('Ctrl Pts',(-9.95433920767431,12.2,-5.16822381565886));
#274356=CARTESIAN_POINT('Ctrl Pts',(-9.95653028176125,12.2,-5.17086513793719));
#274357=CARTESIAN_POINT('Ctrl Pts',(-9.95872135584819,12.2,-5.17350646021553));
#274358=CARTESIAN_POINT('Ctrl Pts',(-9.96091394165166,12.2,-5.17615594921828));
#274359=CARTESIAN_POINT('Ctrl Pts',(-9.96310799423841,12.2,-5.17881359491226));
#274360=CARTESIAN_POINT('Ctrl Pts',(-9.96530204722373,12.2,-5.18147124108905));
#274361=CARTESIAN_POINT('Ctrl Pts',(-9.96749756672617,12.2,-5.18413704359317));
#274362=CARTESIAN_POINT('Ctrl Pts',(-9.96969450871231,12.2,-5.18681099335788));
#274363=CARTESIAN_POINT('Ctrl Pts',(-9.97189145029933,12.2,-5.18948494263682));
#274364=CARTESIAN_POINT('Ctrl Pts',(-9.97408981417886,12.2,-5.19216704003294));
#274365=CARTESIAN_POINT('Ctrl Pts',(-9.97628955537566,12.2,-5.1948572739872));
#274366=CARTESIAN_POINT('Ctrl Pts',(-9.97995579083685,12.2,-5.1993409974072));
#274367=CARTESIAN_POINT('Ctrl Pts',(-9.98362585221359,12.2,-5.20384732657383));
#274368=CARTESIAN_POINT('Ctrl Pts',(-9.9872995359639,12.2,-5.20837621386734));
#274369=CARTESIAN_POINT('Ctrl Pts',(-9.989503746134,12.2,-5.21109354614473));
#274370=CARTESIAN_POINT('Ctrl Pts',(-9.99170926115401,12.2,-5.21381899963));
#274371=CARTESIAN_POINT('Ctrl Pts',(-9.99391603624061,12.2,-5.21655256528139));
#274372=CARTESIAN_POINT('Ctrl Pts',(-9.9961228113272,12.2,-5.21928613093277));
#274373=CARTESIAN_POINT('Ctrl Pts',(-9.9983308461723,12.2,-5.22202780745652));
#274374=CARTESIAN_POINT('Ctrl Pts',(-10.0005400987687,12.2,-5.22477758703579));
#274375=CARTESIAN_POINT('Ctrl Pts',(-10.0027493513651,12.2,-5.22752736661506));
#274376=CARTESIAN_POINT('Ctrl Pts',(-10.0049598210517,12.2,-5.23028524661876));
#274377=CARTESIAN_POINT('Ctrl Pts',(-10.0071714637314,12.2,-5.23305121973911));
#274378=CARTESIAN_POINT('Ctrl Pts',(-10.0093831064111,12.2,-5.23581719285947));
#274379=CARTESIAN_POINT('Ctrl Pts',(-10.0115959234393,12.2,-5.23859125733195));
#274380=CARTESIAN_POINT('Ctrl Pts',(-10.0138098710254,12.2,-5.24137340448017));
#274381=CARTESIAN_POINT('Ctrl Pts',(-10.0160238186115,12.2,-5.24415555162838));
#274382=CARTESIAN_POINT('Ctrl Pts',(-10.0182388956476,12.2,-5.24694578014271));
#274383=CARTESIAN_POINT('Ctrl Pts',(-10.0204550622336,12.2,-5.24974408087327));
#274384=CARTESIAN_POINT('Ctrl Pts',(-10.0226712292222,12.2,-5.25254238211218));
#274385=CARTESIAN_POINT('Ctrl Pts',(-10.0248884846278,12.2,-5.25534875565338));
#274386=CARTESIAN_POINT('Ctrl Pts',(-10.027106784742,12.2,-5.25816319135518));
#274387=CARTESIAN_POINT('Ctrl Pts',(-10.0293250844532,12.2,-5.26097762654569));
#274388=CARTESIAN_POINT('Ctrl Pts',(-10.031544430856,12.2,-5.26380012362741));
#274389=CARTESIAN_POINT('Ctrl Pts',(-10.0337647804838,12.2,-5.26663067331696));
#274390=CARTESIAN_POINT('Ctrl Pts',(-10.0359851301115,12.2,-5.26946122300651));
#274391=CARTESIAN_POINT('Ctrl Pts',(-10.0382064823394,12.2,-5.27229982469302));
#274392=CARTESIAN_POINT('Ctrl Pts',(-10.0404287964771,12.2,-5.27514646747755));
#274393=CARTESIAN_POINT('Ctrl Pts',(-10.0433918818594,12.2,-5.27894199101787));
#274394=CARTESIAN_POINT('Ctrl Pts',(-10.046356677641,12.2,-5.28275181269434));
#274395=CARTESIAN_POINT('Ctrl Pts',(-10.0493230837317,12.2,-5.28657590615806));
#274396=CARTESIAN_POINT('Ctrl Pts',(-10.0515478888049,12.2,-5.28944397690714));
#274397=CARTESIAN_POINT('Ctrl Pts',(-10.0537735996117,12.2,-5.29232007617512));
#274398=CARTESIAN_POINT('Ctrl Pts',(-10.0560001747271,12.2,-5.29520419388704));
#274399=CARTESIAN_POINT('Ctrl Pts',(-10.058226749438,12.2,-5.29808831107501));
#274400=CARTESIAN_POINT('Ctrl Pts',(-10.0604541895072,12.2,-5.30098044610422));
#274401=CARTESIAN_POINT('Ctrl Pts',(-10.0626824527179,12.2,-5.30388058883287));
#274402=CARTESIAN_POINT('Ctrl Pts',(-10.0649107159287,12.2,-5.30678073156153));
#274403=CARTESIAN_POINT('Ctrl Pts',(-10.0671398030063,12.2,-5.30968888177863));
#274404=CARTESIAN_POINT('Ctrl Pts',(-10.0693696727271,12.2,-5.31260503043594));
#274405=CARTESIAN_POINT('Ctrl Pts',(-10.0715995424479,12.2,-5.31552117909327));
#274406=CARTESIAN_POINT('Ctrl Pts',(-10.073830195969,12.2,-5.31844532509055));
#274407=CARTESIAN_POINT('Ctrl Pts',(-10.0760615897314,12.2,-5.3213774582473));
#274408=CARTESIAN_POINT('Ctrl Pts',(-10.0782929834937,12.2,-5.32430959140405));
#274409=CARTESIAN_POINT('Ctrl Pts',(-10.0805251200545,12.2,-5.32724971180322));
#274410=CARTESIAN_POINT('Ctrl Pts',(-10.0827579573067,12.2,-5.33019780894542));
#274411=CARTESIAN_POINT('Ctrl Pts',(-10.0849907945588,12.2,-5.33314590608762));
#274412=CARTESIAN_POINT('Ctrl Pts',(-10.0872243338109,12.2,-5.33610197912926));
#274413=CARTESIAN_POINT('Ctrl Pts',(-10.0894585349797,12.2,-5.33906601889547));
#274414=CARTESIAN_POINT('Ctrl Pts',(-10.0916927365543,12.2,-5.34203005920015));
#274415=CARTESIAN_POINT('Ctrl Pts',(-10.0939276000624,12.2,-5.34500206704876));
#274416=CARTESIAN_POINT('Ctrl Pts',(-10.0961630855541,12.2,-5.34798202985793));
#274417=CARTESIAN_POINT('Ctrl Pts',(-10.0991437321994,12.2,-5.35195531270122));
#274418=CARTESIAN_POINT('Ctrl Pts',(-10.1021254821311,12.2,-5.355942739759));
#274419=CARTESIAN_POINT('Ctrl Pts',(-10.1051082402897,12.2,-5.35994428450557));
#274420=CARTESIAN_POINT('Ctrl Pts',(-10.1073453090102,12.2,-5.3629454432018));
#274421=CARTESIAN_POINT('Ctrl Pts',(-10.1095829447208,12.2,-5.36595454263154));
#274422=CARTESIAN_POINT('Ctrl Pts',(-10.1118211114728,12.2,-5.36897157389624));
#274423=CARTESIAN_POINT('Ctrl Pts',(-10.1140592782247,12.2,-5.37198860516093));
#274424=CARTESIAN_POINT('Ctrl Pts',(-10.1162979764433,12.2,-5.37501356935007));
#274425=CARTESIAN_POINT('Ctrl Pts',(-10.1185371685286,12.2,-5.37804645357213));
#274426=CARTESIAN_POINT('Ctrl Pts',(-10.1207763610206,12.2,-5.38107933834517));
#274427=CARTESIAN_POINT('Ctrl Pts',(-10.1230160464794,12.2,-5.3841201444871));
#274428=CARTESIAN_POINT('Ctrl Pts',(-10.1252561779717,12.2,-5.38716885968126));
#274429=CARTESIAN_POINT('Ctrl Pts',(-10.1274963090571,12.2,-5.39021757432157));
#274430=CARTESIAN_POINT('Ctrl Pts',(-10.1297368853697,12.2,-5.3932741973836));
#274431=CARTESIAN_POINT('Ctrl Pts',(-10.131977863942,12.2,-5.39633871684295));
#274432=CARTESIAN_POINT('Ctrl Pts',(-10.1342188425142,12.2,-5.3994032363023));
#274433=CARTESIAN_POINT('Ctrl Pts',(-10.1364602251632,12.2,-5.40247565238601));
#274434=CARTESIAN_POINT('Ctrl Pts',(-10.1387019915142,12.2,-5.40555595924693));
#274435=CARTESIAN_POINT('Ctrl Pts',(-10.1409437578652,12.2,-5.40863626610785));
#274436=CARTESIAN_POINT('Ctrl Pts',(-10.1431859115927,12.2,-5.41172446343756));
#274437=CARTESIAN_POINT('Ctrl Pts',(-10.1454284470001,12.2,-5.41482055400001));
#274438=CARTESIAN_POINT('Ctrl Pts',(-9.95917514600006,15.2,-5.75020264100001));
#274439=CARTESIAN_POINT('Ctrl Pts',(-9.95917514600006,11.6,-5.75020264100001));
#274440=CARTESIAN_POINT('Ctrl Pts',(-9.95841243100006,15.2,-5.75014921000002));
#274441=CARTESIAN_POINT('Ctrl Pts',(-9.95841243100006,11.6,-5.75014921000002));
#274442=CARTESIAN_POINT('Ctrl Pts',(-9.95688746000006,15.2,-5.75004209300002));
#274443=CARTESIAN_POINT('Ctrl Pts',(-9.95688746000006,11.6,-5.75004209300002));
#274444=CARTESIAN_POINT('Ctrl Pts',(-9.95460138500006,15.2,-5.74988064700002));
#274445=CARTESIAN_POINT('Ctrl Pts',(-9.95460138500006,11.6,-5.74988064700002));
#274446=CARTESIAN_POINT('Ctrl Pts',(-9.95155604400006,15.2,-5.74966384900002));
#274447=CARTESIAN_POINT('Ctrl Pts',(-9.95155604400006,11.6,-5.74966384900002));
#274448=CARTESIAN_POINT('Ctrl Pts',(-9.94775397000006,15.2,-5.74939029000002));
#274449=CARTESIAN_POINT('Ctrl Pts',(-9.94775397000006,11.6,-5.74939029000002));
#274450=CARTESIAN_POINT('Ctrl Pts',(-9.94395649900006,15.2,-5.74911416700001));
#274451=CARTESIAN_POINT('Ctrl Pts',(-9.94395649900006,11.6,-5.74911416700001));
#274452=CARTESIAN_POINT('Ctrl Pts',(-9.94016363100006,15.2,-5.74883548400001));
#274453=CARTESIAN_POINT('Ctrl Pts',(-9.94016363100006,11.6,-5.74883548400001));
#274454=CARTESIAN_POINT('Ctrl Pts',(-9.93637537100006,15.2,-5.74855424400001));
#274455=CARTESIAN_POINT('Ctrl Pts',(-9.93637537100006,11.6,-5.74855424400001));
#274456=CARTESIAN_POINT('Ctrl Pts',(-9.93259172200006,15.2,-5.74827044900001));
#274457=CARTESIAN_POINT('Ctrl Pts',(-9.93259172200006,11.6,-5.74827044900001));
#274458=CARTESIAN_POINT('Ctrl Pts',(-9.92881269100006,15.2,-5.74798410500001));
#274459=CARTESIAN_POINT('Ctrl Pts',(-9.92881269100006,11.6,-5.74798410500001));
#274460=CARTESIAN_POINT('Ctrl Pts',(-9.92503828400006,15.2,-5.74769522000001));
#274461=CARTESIAN_POINT('Ctrl Pts',(-9.92503828400006,11.6,-5.74769522000001));
#274462=CARTESIAN_POINT('Ctrl Pts',(-9.92126851000006,15.2,-5.74740380100002));
#274463=CARTESIAN_POINT('Ctrl Pts',(-9.92126851000006,11.6,-5.74740380100002));
#274464=CARTESIAN_POINT('Ctrl Pts',(-9.91750337600006,15.2,-5.74710985300002));
#274465=CARTESIAN_POINT('Ctrl Pts',(-9.91750337600006,11.6,-5.74710985300002));
#274466=CARTESIAN_POINT('Ctrl Pts',(-9.91374289200006,15.2,-5.74681338700002));
#274467=CARTESIAN_POINT('Ctrl Pts',(-9.91374289200006,11.6,-5.74681338700002));
#274468=CARTESIAN_POINT('Ctrl Pts',(-9.90998706400006,15.2,-5.74651440900002));
#274469=CARTESIAN_POINT('Ctrl Pts',(-9.90998706400006,11.6,-5.74651440900002));
#274470=CARTESIAN_POINT('Ctrl Pts',(-9.90623590000006,15.2,-5.74621292500002));
#274471=CARTESIAN_POINT('Ctrl Pts',(-9.90623590000006,11.6,-5.74621292500002));
#274472=CARTESIAN_POINT('Ctrl Pts',(-9.90248940500006,15.2,-5.74590894100002));
#274473=CARTESIAN_POINT('Ctrl Pts',(-9.90248940500006,11.6,-5.74590894100002));
#274474=CARTESIAN_POINT('Ctrl Pts',(-9.89874758700006,15.2,-5.74560246200001));
#274475=CARTESIAN_POINT('Ctrl Pts',(-9.89874758700006,11.6,-5.74560246200001));
#274476=CARTESIAN_POINT('Ctrl Pts',(-9.89501045000006,15.2,-5.74529349400001));
#274477=CARTESIAN_POINT('Ctrl Pts',(-9.89501045000006,11.6,-5.74529349400001));
#274478=CARTESIAN_POINT('Ctrl Pts',(-9.89127800100006,15.2,-5.74498204400002));
#274479=CARTESIAN_POINT('Ctrl Pts',(-9.89127800100006,11.6,-5.74498204400002));
#274480=CARTESIAN_POINT('Ctrl Pts',(-9.88755024700006,15.2,-5.74466811600002));
#274481=CARTESIAN_POINT('Ctrl Pts',(-9.88755024700006,11.6,-5.74466811600002));
#274482=CARTESIAN_POINT('Ctrl Pts',(-9.88382719300006,15.2,-5.74435171600002));
#274483=CARTESIAN_POINT('Ctrl Pts',(-9.88382719300006,11.6,-5.74435171600002));
#274484=CARTESIAN_POINT('Ctrl Pts',(-9.88010884700006,15.2,-5.74403285200002));
#274485=CARTESIAN_POINT('Ctrl Pts',(-9.88010884700006,11.6,-5.74403285200002));
#274486=CARTESIAN_POINT('Ctrl Pts',(-9.87639521400006,15.2,-5.74371152900002));
#274487=CARTESIAN_POINT('Ctrl Pts',(-9.87639521400006,11.6,-5.74371152900002));
#274488=CARTESIAN_POINT('Ctrl Pts',(-9.87268630300006,15.2,-5.74338775400002));
#274489=CARTESIAN_POINT('Ctrl Pts',(-9.87268630300006,11.6,-5.74338775400002));
#274490=CARTESIAN_POINT('Ctrl Pts',(-9.86898212000006,15.2,-5.74306153500002));
#274491=CARTESIAN_POINT('Ctrl Pts',(-9.86898212000006,11.6,-5.74306153500002));
#274492=CARTESIAN_POINT('Ctrl Pts',(-9.86528267300006,15.2,-5.74273287600001));
#274493=CARTESIAN_POINT('Ctrl Pts',(-9.86528267300006,11.6,-5.74273287600001));
#274494=CARTESIAN_POINT('Ctrl Pts',(-9.86158796700006,15.2,-5.74240178400002));
#274495=CARTESIAN_POINT('Ctrl Pts',(-9.86158796700006,11.6,-5.74240178400002));
#274496=CARTESIAN_POINT('Ctrl Pts',(-9.85789800900006,15.2,-5.74206826700002));
#274497=CARTESIAN_POINT('Ctrl Pts',(-9.85789800900006,11.6,-5.74206826700002));
#274498=CARTESIAN_POINT('Ctrl Pts',(-9.85421280700006,15.2,-5.74173232900002));
#274499=CARTESIAN_POINT('Ctrl Pts',(-9.85421280700006,11.6,-5.74173232900002));
#274500=CARTESIAN_POINT('Ctrl Pts',(-9.85053236600006,15.2,-5.74139397800002));
#274501=CARTESIAN_POINT('Ctrl Pts',(-9.85053236600006,11.6,-5.74139397800002));
#274502=CARTESIAN_POINT('Ctrl Pts',(-9.84685669200006,15.2,-5.74105321800002));
#274503=CARTESIAN_POINT('Ctrl Pts',(-9.84685669200006,11.6,-5.74105321800002));
#274504=CARTESIAN_POINT('Ctrl Pts',(-9.84318579500006,15.2,-5.74071005800001));
#274505=CARTESIAN_POINT('Ctrl Pts',(-9.84318579500006,11.6,-5.74071005800001));
#274506=CARTESIAN_POINT('Ctrl Pts',(-9.83951967700006,15.2,-5.74036450400002));
#274507=CARTESIAN_POINT('Ctrl Pts',(-9.83951967700006,11.6,-5.74036450400002));
#274508=CARTESIAN_POINT('Ctrl Pts',(-9.83585834900006,15.2,-5.74001656000001));
#274509=CARTESIAN_POINT('Ctrl Pts',(-9.83585834900006,11.6,-5.74001656000001));
#274510=CARTESIAN_POINT('Ctrl Pts',(-9.83220181500006,15.2,-5.73966623600001));
#274511=CARTESIAN_POINT('Ctrl Pts',(-9.83220181500006,11.6,-5.73966623600001));
#274512=CARTESIAN_POINT('Ctrl Pts',(-9.82855008400006,15.2,-5.73931353600001));
#274513=CARTESIAN_POINT('Ctrl Pts',(-9.82855008400006,11.6,-5.73931353600001));
#274514=CARTESIAN_POINT('Ctrl Pts',(-9.82490316100006,15.2,-5.73895846600001));
#274515=CARTESIAN_POINT('Ctrl Pts',(-9.82490316100006,11.6,-5.73895846600001));
#274516=CARTESIAN_POINT('Ctrl Pts',(-9.82126105300006,15.2,-5.73860103500002));
#274517=CARTESIAN_POINT('Ctrl Pts',(-9.82126105300006,11.6,-5.73860103500002));
#274518=CARTESIAN_POINT('Ctrl Pts',(-9.81762376700006,15.2,-5.73824124900002));
#274519=CARTESIAN_POINT('Ctrl Pts',(-9.81762376700006,11.6,-5.73824124900002));
#274520=CARTESIAN_POINT('Ctrl Pts',(-9.81399131100006,15.2,-5.73787911300002));
#274521=CARTESIAN_POINT('Ctrl Pts',(-9.81399131100006,11.6,-5.73787911300002));
#274522=CARTESIAN_POINT('Ctrl Pts',(-9.81036369000006,15.2,-5.73751463500002));
#274523=CARTESIAN_POINT('Ctrl Pts',(-9.81036369000006,11.6,-5.73751463500002));
#274524=CARTESIAN_POINT('Ctrl Pts',(-9.80674091100006,15.2,-5.73714781900001));
#274525=CARTESIAN_POINT('Ctrl Pts',(-9.80674091100006,11.6,-5.73714781900001));
#274526=CARTESIAN_POINT('Ctrl Pts',(-9.80312298100005,15.2,-5.73677867600002));
#274527=CARTESIAN_POINT('Ctrl Pts',(-9.80312298100005,11.6,-5.73677867600002));
#274528=CARTESIAN_POINT('Ctrl Pts',(-9.79950990800005,15.2,-5.73640720800002));
#274529=CARTESIAN_POINT('Ctrl Pts',(-9.79950990800005,11.6,-5.73640720800002));
#274530=CARTESIAN_POINT('Ctrl Pts',(-9.79590169600005,15.2,-5.73603342500002));
#274531=CARTESIAN_POINT('Ctrl Pts',(-9.79590169600005,11.6,-5.73603342500002));
#274532=CARTESIAN_POINT('Ctrl Pts',(-9.79229835500006,15.2,-5.73565733100001));
#274533=CARTESIAN_POINT('Ctrl Pts',(-9.79229835500006,11.6,-5.73565733100001));
#274534=CARTESIAN_POINT('Ctrl Pts',(-9.78869989000006,15.2,-5.73527893500002));
#274535=CARTESIAN_POINT('Ctrl Pts',(-9.78869989000006,11.6,-5.73527893500002));
#274536=CARTESIAN_POINT('Ctrl Pts',(-9.78510630800006,15.2,-5.73489824300002));
#274537=CARTESIAN_POINT('Ctrl Pts',(-9.78510630800006,11.6,-5.73489824300002));
#274538=CARTESIAN_POINT('Ctrl Pts',(-9.78151761600006,15.2,-5.73451526100002));
#274539=CARTESIAN_POINT('Ctrl Pts',(-9.78151761600006,11.6,-5.73451526100002));
#274540=CARTESIAN_POINT('Ctrl Pts',(-9.77793382100005,15.2,-5.73412999600002));
#274541=CARTESIAN_POINT('Ctrl Pts',(-9.77793382100005,11.6,-5.73412999600002));
#274542=CARTESIAN_POINT('Ctrl Pts',(-9.77435492900005,15.2,-5.73374245400001));
#274543=CARTESIAN_POINT('Ctrl Pts',(-9.77435492900005,11.6,-5.73374245400001));
#274544=CARTESIAN_POINT('Ctrl Pts',(-9.77078094800006,15.2,-5.73335264400002));
#274545=CARTESIAN_POINT('Ctrl Pts',(-9.77078094800006,11.6,-5.73335264400002));
#274546=CARTESIAN_POINT('Ctrl Pts',(-9.76721188400006,15.2,-5.73296057000002));
#274547=CARTESIAN_POINT('Ctrl Pts',(-9.76721188400006,11.6,-5.73296057000002));
#274548=CARTESIAN_POINT('Ctrl Pts',(-9.76364774500006,15.2,-5.73256624100001));
#274549=CARTESIAN_POINT('Ctrl Pts',(-9.76364774500006,11.6,-5.73256624100001));
#274550=CARTESIAN_POINT('Ctrl Pts',(-9.76008853600005,15.2,-5.73216966200001));
#274551=CARTESIAN_POINT('Ctrl Pts',(-9.76008853600005,11.6,-5.73216966200001));
#274552=CARTESIAN_POINT('Ctrl Pts',(-9.75653426500006,15.2,-5.73177084100001));
#274553=CARTESIAN_POINT('Ctrl Pts',(-9.75653426500006,11.6,-5.73177084100001));
#274554=CARTESIAN_POINT('Ctrl Pts',(-9.75298493900006,15.2,-5.73136978400001));
#274555=CARTESIAN_POINT('Ctrl Pts',(-9.75298493900006,11.6,-5.73136978400001));
#274556=CARTESIAN_POINT('Ctrl Pts',(-9.74944056500006,15.2,-5.73096650000001));
#274557=CARTESIAN_POINT('Ctrl Pts',(-9.74944056500006,11.6,-5.73096650000001));
#274558=CARTESIAN_POINT('Ctrl Pts',(-9.74590115000005,15.2,-5.73056099200001));
#274559=CARTESIAN_POINT('Ctrl Pts',(-9.74590115000005,11.6,-5.73056099200001));
#274560=CARTESIAN_POINT('Ctrl Pts',(-9.74236669900005,15.2,-5.73015327100002));
#274561=CARTESIAN_POINT('Ctrl Pts',(-9.74236669900005,11.6,-5.73015327100002));
#274562=CARTESIAN_POINT('Ctrl Pts',(-9.73883722100006,15.2,-5.72974334100002));
#274563=CARTESIAN_POINT('Ctrl Pts',(-9.73883722100006,11.6,-5.72974334100002));
#274564=CARTESIAN_POINT('Ctrl Pts',(-9.73531272200006,15.2,-5.72933121000001));
#274565=CARTESIAN_POINT('Ctrl Pts',(-9.73531272200006,11.6,-5.72933121000001));
#274566=CARTESIAN_POINT('Ctrl Pts',(-9.73179320900006,15.2,-5.72891688500002));
#274567=CARTESIAN_POINT('Ctrl Pts',(-9.73179320900006,11.6,-5.72891688500002));
#274568=CARTESIAN_POINT('Ctrl Pts',(-9.72827869000006,15.2,-5.72850037300002));
#274569=CARTESIAN_POINT('Ctrl Pts',(-9.72827869000006,11.6,-5.72850037300002));
#274570=CARTESIAN_POINT('Ctrl Pts',(-9.72476917000006,15.2,-5.72808168000002));
#274571=CARTESIAN_POINT('Ctrl Pts',(-9.72476917000006,11.6,-5.72808168000002));
#274572=CARTESIAN_POINT('Ctrl Pts',(-9.72126465700006,15.2,-5.72766081300002));
#274573=CARTESIAN_POINT('Ctrl Pts',(-9.72126465700006,11.6,-5.72766081300002));
#274574=CARTESIAN_POINT('Ctrl Pts',(-9.71776515900006,15.2,-5.72723778200002));
#274575=CARTESIAN_POINT('Ctrl Pts',(-9.71776515900006,11.6,-5.72723778200002));
#274576=CARTESIAN_POINT('Ctrl Pts',(-9.71427068100006,15.2,-5.72681259100002));
#274577=CARTESIAN_POINT('Ctrl Pts',(-9.71427068100006,11.6,-5.72681259100002));
#274578=CARTESIAN_POINT('Ctrl Pts',(-9.71078123000006,15.2,-5.72638524700002));
#274579=CARTESIAN_POINT('Ctrl Pts',(-9.71078123000006,11.6,-5.72638524700002));
#274580=CARTESIAN_POINT('Ctrl Pts',(-9.70729681500006,15.2,-5.72595575900002));
#274581=CARTESIAN_POINT('Ctrl Pts',(-9.70729681500006,11.6,-5.72595575900002));
#274582=CARTESIAN_POINT('Ctrl Pts',(-9.70381744100006,15.2,-5.72552413200001));
#274583=CARTESIAN_POINT('Ctrl Pts',(-9.70381744100006,11.6,-5.72552413200001));
#274584=CARTESIAN_POINT('Ctrl Pts',(-9.70034311500006,15.2,-5.72509037400001));
#274585=CARTESIAN_POINT('Ctrl Pts',(-9.70034311500006,11.6,-5.72509037400001));
#274586=CARTESIAN_POINT('Ctrl Pts',(-9.69687384600006,15.2,-5.72465449300001));
#274587=CARTESIAN_POINT('Ctrl Pts',(-9.69687384600006,11.6,-5.72465449300001));
#274588=CARTESIAN_POINT('Ctrl Pts',(-9.69340963900006,15.2,-5.72421649500002));
#274589=CARTESIAN_POINT('Ctrl Pts',(-9.69340963900006,11.6,-5.72421649500002));
#274590=CARTESIAN_POINT('Ctrl Pts',(-9.68995050200006,15.2,-5.72377638700001));
#274591=CARTESIAN_POINT('Ctrl Pts',(-9.68995050200006,11.6,-5.72377638700001));
#274592=CARTESIAN_POINT('Ctrl Pts',(-9.68649644100006,15.2,-5.72333417800002));
#274593=CARTESIAN_POINT('Ctrl Pts',(-9.68649644100006,11.6,-5.72333417800002));
#274594=CARTESIAN_POINT('Ctrl Pts',(-9.68304746500005,15.2,-5.72288987300002));
#274595=CARTESIAN_POINT('Ctrl Pts',(-9.68304746500005,11.6,-5.72288987300002));
#274596=CARTESIAN_POINT('Ctrl Pts',(-9.67960357800006,15.2,-5.72244348100002));
#274597=CARTESIAN_POINT('Ctrl Pts',(-9.67960357800006,11.6,-5.72244348100002));
#274598=CARTESIAN_POINT('Ctrl Pts',(-9.67616479000006,15.2,-5.72199500700002));
#274599=CARTESIAN_POINT('Ctrl Pts',(-9.67616479000006,11.6,-5.72199500700002));
#274600=CARTESIAN_POINT('Ctrl Pts',(-9.67273110700006,15.2,-5.72154446000001));
#274601=CARTESIAN_POINT('Ctrl Pts',(-9.67273110700006,11.6,-5.72154446000001));
#274602=CARTESIAN_POINT('Ctrl Pts',(-9.66930253400006,15.2,-5.72109184700002));
#274603=CARTESIAN_POINT('Ctrl Pts',(-9.66930253400006,11.6,-5.72109184700002));
#274604=CARTESIAN_POINT('Ctrl Pts',(-9.66587908100006,15.2,-5.72063717600001));
#274605=CARTESIAN_POINT('Ctrl Pts',(-9.66587908100006,11.6,-5.72063717600001));
#274606=CARTESIAN_POINT('Ctrl Pts',(-9.66246075400005,15.2,-5.72018045200001));
#274607=CARTESIAN_POINT('Ctrl Pts',(-9.66246075400005,11.6,-5.72018045200001));
#274608=CARTESIAN_POINT('Ctrl Pts',(-9.65904756000005,15.2,-5.71972168500002));
#274609=CARTESIAN_POINT('Ctrl Pts',(-9.65904756000005,11.6,-5.71972168500002));
#274610=CARTESIAN_POINT('Ctrl Pts',(-9.65563950500006,15.2,-5.71926088000002));
#274611=CARTESIAN_POINT('Ctrl Pts',(-9.65563950500006,11.6,-5.71926088000002));
#274612=CARTESIAN_POINT('Ctrl Pts',(-9.65223659800006,15.2,-5.71879804700002));
#274613=CARTESIAN_POINT('Ctrl Pts',(-9.65223659800006,11.6,-5.71879804700002));
#274614=CARTESIAN_POINT('Ctrl Pts',(-9.64883884500006,15.2,-5.71833319000002));
#274615=CARTESIAN_POINT('Ctrl Pts',(-9.64883884500006,11.6,-5.71833319000002));
#274616=CARTESIAN_POINT('Ctrl Pts',(-9.64544625400006,15.2,-5.71786632000002));
#274617=CARTESIAN_POINT('Ctrl Pts',(-9.64544625400006,11.6,-5.71786632000002));
#274618=CARTESIAN_POINT('Ctrl Pts',(-9.64205883100006,15.2,-5.71739744100002));
#274619=CARTESIAN_POINT('Ctrl Pts',(-9.64205883100006,11.6,-5.71739744100002));
#274620=CARTESIAN_POINT('Ctrl Pts',(-9.63867658300006,15.2,-5.71692656400002));
#274621=CARTESIAN_POINT('Ctrl Pts',(-9.63867658300006,11.6,-5.71692656400002));
#274622=CARTESIAN_POINT('Ctrl Pts',(-9.63529951700006,15.2,-5.71645369400001));
#274623=CARTESIAN_POINT('Ctrl Pts',(-9.63529951700006,11.6,-5.71645369400001));
#274624=CARTESIAN_POINT('Ctrl Pts',(-9.63192764200006,15.2,-5.71597884000001));
#274625=CARTESIAN_POINT('Ctrl Pts',(-9.63192764200006,11.6,-5.71597884000001));
#274626=CARTESIAN_POINT('Ctrl Pts',(-9.62856096400006,15.2,-5.71550200700001));
#274627=CARTESIAN_POINT('Ctrl Pts',(-9.62856096400006,11.6,-5.71550200700001));
#274628=CARTESIAN_POINT('Ctrl Pts',(-9.62519948900006,15.2,-5.71502320500001));
#274629=CARTESIAN_POINT('Ctrl Pts',(-9.62519948900006,11.6,-5.71502320500001));
#274630=CARTESIAN_POINT('Ctrl Pts',(-9.62184322600006,15.2,-5.71454244100002));
#274631=CARTESIAN_POINT('Ctrl Pts',(-9.62184322600006,11.6,-5.71454244100002));
#274632=CARTESIAN_POINT('Ctrl Pts',(-9.61849218000006,15.2,-5.71405972200001));
#274633=CARTESIAN_POINT('Ctrl Pts',(-9.61849218000006,11.6,-5.71405972200001));
#274634=CARTESIAN_POINT('Ctrl Pts',(-9.61514636100006,15.2,-5.71357505700002));
#274635=CARTESIAN_POINT('Ctrl Pts',(-9.61514636100006,11.6,-5.71357505700002));
#274636=CARTESIAN_POINT('Ctrl Pts',(-9.61180577400006,15.2,-5.71308845100001));
#274637=CARTESIAN_POINT('Ctrl Pts',(-9.61180577400006,11.6,-5.71308845100001));
#274638=CARTESIAN_POINT('Ctrl Pts',(-9.60847042700006,15.2,-5.71259991300002));
#274639=CARTESIAN_POINT('Ctrl Pts',(-9.60847042700006,11.6,-5.71259991300002));
#274640=CARTESIAN_POINT('Ctrl Pts',(-9.60514032600006,15.2,-5.71210945300002));
#274641=CARTESIAN_POINT('Ctrl Pts',(-9.60514032600006,11.6,-5.71210945300002));
#274642=CARTESIAN_POINT('Ctrl Pts',(-9.60181548000006,15.2,-5.71161707400002));
#274643=CARTESIAN_POINT('Ctrl Pts',(-9.60181548000006,11.6,-5.71161707400002));
#274644=CARTESIAN_POINT('Ctrl Pts',(-9.59849589600006,15.2,-5.71112278700002));
#274645=CARTESIAN_POINT('Ctrl Pts',(-9.59849589600006,11.6,-5.71112278700002));
#274646=CARTESIAN_POINT('Ctrl Pts',(-9.59518158000006,15.2,-5.71062660000001));
#274647=CARTESIAN_POINT('Ctrl Pts',(-9.59518158000006,11.6,-5.71062660000001));
#274648=CARTESIAN_POINT('Ctrl Pts',(-9.59187253900006,15.2,-5.71012851800001));
#274649=CARTESIAN_POINT('Ctrl Pts',(-9.59187253900006,11.6,-5.71012851800001));
#274650=CARTESIAN_POINT('Ctrl Pts',(-9.58856878200006,15.2,-5.70962855200002));
#274651=CARTESIAN_POINT('Ctrl Pts',(-9.58856878200006,11.6,-5.70962855200002));
#274652=CARTESIAN_POINT('Ctrl Pts',(-9.58527031500006,15.2,-5.70912670700002));
#274653=CARTESIAN_POINT('Ctrl Pts',(-9.58527031500006,11.6,-5.70912670700002));
#274654=CARTESIAN_POINT('Ctrl Pts',(-9.58197714700006,15.2,-5.70862299200002));
#274655=CARTESIAN_POINT('Ctrl Pts',(-9.58197714700006,11.6,-5.70862299200002));
#274656=CARTESIAN_POINT('Ctrl Pts',(-9.57868928200006,15.2,-5.70811741500002));
#274657=CARTESIAN_POINT('Ctrl Pts',(-9.57868928200006,11.6,-5.70811741500002));
#274658=CARTESIAN_POINT('Ctrl Pts',(-9.57540672900006,15.2,-5.70760998400001));
#274659=CARTESIAN_POINT('Ctrl Pts',(-9.57540672900006,11.6,-5.70760998400001));
#274660=CARTESIAN_POINT('Ctrl Pts',(-9.57212949600006,15.2,-5.70710070600001));
#274661=CARTESIAN_POINT('Ctrl Pts',(-9.57212949600006,11.6,-5.70710070600001));
#274662=CARTESIAN_POINT('Ctrl Pts',(-9.56885759000006,15.2,-5.70658959000002));
#274663=CARTESIAN_POINT('Ctrl Pts',(-9.56885759000006,11.6,-5.70658959000002));
#274664=CARTESIAN_POINT('Ctrl Pts',(-9.56559101700006,15.2,-5.70607664300002));
#274665=CARTESIAN_POINT('Ctrl Pts',(-9.56559101700006,11.6,-5.70607664300002));
#274666=CARTESIAN_POINT('Ctrl Pts',(-9.56232978500006,15.2,-5.70556187300002));
#274667=CARTESIAN_POINT('Ctrl Pts',(-9.56232978500006,11.6,-5.70556187300002));
#274668=CARTESIAN_POINT('Ctrl Pts',(-9.55907390200006,15.2,-5.70504528800001));
#274669=CARTESIAN_POINT('Ctrl Pts',(-9.55907390200006,11.6,-5.70504528800001));
#274670=CARTESIAN_POINT('Ctrl Pts',(-9.55582337400006,15.2,-5.70452689600002));
#274671=CARTESIAN_POINT('Ctrl Pts',(-9.55582337400006,11.6,-5.70452689600002));
#274672=CARTESIAN_POINT('Ctrl Pts',(-9.55257821000006,15.2,-5.70400670700002));
#274673=CARTESIAN_POINT('Ctrl Pts',(-9.55257821000006,11.6,-5.70400670700002));
#274674=CARTESIAN_POINT('Ctrl Pts',(-9.54933841600005,15.2,-5.70348472500001));
#274675=CARTESIAN_POINT('Ctrl Pts',(-9.54933841600005,11.6,-5.70348472500001));
#274676=CARTESIAN_POINT('Ctrl Pts',(-9.54610400000006,15.2,-5.70296096100002));
#274677=CARTESIAN_POINT('Ctrl Pts',(-9.54610400000006,11.6,-5.70296096100002));
#274678=CARTESIAN_POINT('Ctrl Pts',(-9.54287496800006,15.2,-5.70243542200001));
#274679=CARTESIAN_POINT('Ctrl Pts',(-9.54287496800006,11.6,-5.70243542200001));
#274680=CARTESIAN_POINT('Ctrl Pts',(-9.53965133000005,15.2,-5.70190811700002));
#274681=CARTESIAN_POINT('Ctrl Pts',(-9.53965133000005,11.6,-5.70190811700002));
#274682=CARTESIAN_POINT('Ctrl Pts',(-9.53643309000006,15.2,-5.70137905200002));
#274683=CARTESIAN_POINT('Ctrl Pts',(-9.53643309000006,11.6,-5.70137905200002));
#274684=CARTESIAN_POINT('Ctrl Pts',(-9.53322025900006,15.2,-5.70084823700002));
#274685=CARTESIAN_POINT('Ctrl Pts',(-9.53322025900006,11.6,-5.70084823700002));
#274686=CARTESIAN_POINT('Ctrl Pts',(-9.53001284100005,15.2,-5.70031568100001));
#274687=CARTESIAN_POINT('Ctrl Pts',(-9.53001284100005,11.6,-5.70031568100001));
#274688=CARTESIAN_POINT('Ctrl Pts',(-9.52681084500006,15.2,-5.69978139000002));
#274689=CARTESIAN_POINT('Ctrl Pts',(-9.52681084500006,11.6,-5.69978139000002));
#274690=CARTESIAN_POINT('Ctrl Pts',(-9.52361428000006,15.2,-5.69924537200002));
#274691=CARTESIAN_POINT('Ctrl Pts',(-9.52361428000006,11.6,-5.69924537200002));
#274692=CARTESIAN_POINT('Ctrl Pts',(-9.52042315000006,15.2,-5.69870763800001));
#274693=CARTESIAN_POINT('Ctrl Pts',(-9.52042315000006,11.6,-5.69870763800001));
#274694=CARTESIAN_POINT('Ctrl Pts',(-9.51723746400006,15.2,-5.69816819400002));
#274695=CARTESIAN_POINT('Ctrl Pts',(-9.51723746400006,11.6,-5.69816819400002));
#274696=CARTESIAN_POINT('Ctrl Pts',(-9.51405723100006,15.2,-5.69762704800001));
#274697=CARTESIAN_POINT('Ctrl Pts',(-9.51405723100006,11.6,-5.69762704800001));
#274698=CARTESIAN_POINT('Ctrl Pts',(-9.51088245600006,15.2,-5.69708421000002));
#274699=CARTESIAN_POINT('Ctrl Pts',(-9.51088245600006,11.6,-5.69708421000002));
#274700=CARTESIAN_POINT('Ctrl Pts',(-9.50771314700006,15.2,-5.69653968700001));
#274701=CARTESIAN_POINT('Ctrl Pts',(-9.50771314700006,11.6,-5.69653968700001));
#274702=CARTESIAN_POINT('Ctrl Pts',(-9.50454931300006,15.2,-5.69599348800002));
#274703=CARTESIAN_POINT('Ctrl Pts',(-9.50454931300006,11.6,-5.69599348800002));
#274704=CARTESIAN_POINT('Ctrl Pts',(-9.50139095800006,15.2,-5.69544562100001));
#274705=CARTESIAN_POINT('Ctrl Pts',(-9.50139095800006,11.6,-5.69544562100001));
#274706=CARTESIAN_POINT('Ctrl Pts',(-9.49823809300005,15.2,-5.69489609400001));
#274707=CARTESIAN_POINT('Ctrl Pts',(-9.49823809300005,11.6,-5.69489609400001));
#274708=CARTESIAN_POINT('Ctrl Pts',(-9.49509072500006,15.2,-5.69434491500001));
#274709=CARTESIAN_POINT('Ctrl Pts',(-9.49509072500006,11.6,-5.69434491500001));
#274710=CARTESIAN_POINT('Ctrl Pts',(-9.49194886000006,15.2,-5.69379209500001));
#274711=CARTESIAN_POINT('Ctrl Pts',(-9.49194886000006,11.6,-5.69379209500001));
#274712=CARTESIAN_POINT('Ctrl Pts',(-9.48881250600006,15.2,-5.69323764000002));
#274713=CARTESIAN_POINT('Ctrl Pts',(-9.48881250600006,11.6,-5.69323764000002));
#274714=CARTESIAN_POINT('Ctrl Pts',(-9.48568167200006,15.2,-5.69268155900001));
#274715=CARTESIAN_POINT('Ctrl Pts',(-9.48568167200006,11.6,-5.69268155900001));
#274716=CARTESIAN_POINT('Ctrl Pts',(-9.48255636300006,15.2,-5.69212386100002));
#274717=CARTESIAN_POINT('Ctrl Pts',(-9.48255636300006,11.6,-5.69212386100002));
#274718=CARTESIAN_POINT('Ctrl Pts',(-9.47943658800006,15.2,-5.69156455400002));
#274719=CARTESIAN_POINT('Ctrl Pts',(-9.47943658800006,11.6,-5.69156455400002));
#274720=CARTESIAN_POINT('Ctrl Pts',(-9.47632235400006,15.2,-5.69100364700001));
#274721=CARTESIAN_POINT('Ctrl Pts',(-9.47632235400006,11.6,-5.69100364700001));
#274722=CARTESIAN_POINT('Ctrl Pts',(-9.47321366800006,15.2,-5.69044114700001));
#274723=CARTESIAN_POINT('Ctrl Pts',(-9.47321366800006,11.6,-5.69044114700001));
#274724=CARTESIAN_POINT('Ctrl Pts',(-9.47011053900006,15.2,-5.68987706500002));
#274725=CARTESIAN_POINT('Ctrl Pts',(-9.47011053900006,11.6,-5.68987706500002));
#274726=CARTESIAN_POINT('Ctrl Pts',(-9.46701297400006,15.2,-5.68931140800002));
#274727=CARTESIAN_POINT('Ctrl Pts',(-9.46701297400006,11.6,-5.68931140800002));
#274728=CARTESIAN_POINT('Ctrl Pts',(-9.46392098000005,15.2,-5.68874418700001));
#274729=CARTESIAN_POINT('Ctrl Pts',(-9.46392098000005,11.6,-5.68874418700001));
#274730=CARTESIAN_POINT('Ctrl Pts',(-9.46083456600006,15.2,-5.68817540700002));
#274731=CARTESIAN_POINT('Ctrl Pts',(-9.46083456600006,11.6,-5.68817540700002));
#274732=CARTESIAN_POINT('Ctrl Pts',(-9.45775373800006,15.2,-5.68760507900001));
#274733=CARTESIAN_POINT('Ctrl Pts',(-9.45775373800006,11.6,-5.68760507900001));
#274734=CARTESIAN_POINT('Ctrl Pts',(-9.45467850400006,15.2,-5.68703321000001));
#274735=CARTESIAN_POINT('Ctrl Pts',(-9.45467850400006,11.6,-5.68703321000001));
#274736=CARTESIAN_POINT('Ctrl Pts',(-9.45160887200006,15.2,-5.68645981100002));
#274737=CARTESIAN_POINT('Ctrl Pts',(-9.45160887200006,11.6,-5.68645981100002));
#274738=CARTESIAN_POINT('Ctrl Pts',(-9.44854485000005,15.2,-5.68588488900001));
#274739=CARTESIAN_POINT('Ctrl Pts',(-9.44854485000005,11.6,-5.68588488900001));
#274740=CARTESIAN_POINT('Ctrl Pts',(-9.44548644300006,15.2,-5.68530845500002));
#274741=CARTESIAN_POINT('Ctrl Pts',(-9.44548644300006,11.6,-5.68530845500002));
#274742=CARTESIAN_POINT('Ctrl Pts',(-9.44243366200006,15.2,-5.68473051500002));
#274743=CARTESIAN_POINT('Ctrl Pts',(-9.44243366200006,11.6,-5.68473051500002));
#274744=CARTESIAN_POINT('Ctrl Pts',(-9.43938651300006,15.2,-5.68415107900002));
#274745=CARTESIAN_POINT('Ctrl Pts',(-9.43938651300006,11.6,-5.68415107900002));
#274746=CARTESIAN_POINT('Ctrl Pts',(-9.43634500500006,15.2,-5.68357015700002));
#274747=CARTESIAN_POINT('Ctrl Pts',(-9.43634500500006,11.6,-5.68357015700002));
#274748=CARTESIAN_POINT('Ctrl Pts',(-9.43330914300006,15.2,-5.68298775600002));
#274749=CARTESIAN_POINT('Ctrl Pts',(-9.43330914300006,11.6,-5.68298775600002));
#274750=CARTESIAN_POINT('Ctrl Pts',(-9.43027893700006,15.2,-5.68240388600002));
#274751=CARTESIAN_POINT('Ctrl Pts',(-9.43027893700006,11.6,-5.68240388600002));
#274752=CARTESIAN_POINT('Ctrl Pts',(-9.42725439400006,15.2,-5.68181855600002));
#274753=CARTESIAN_POINT('Ctrl Pts',(-9.42725439400006,11.6,-5.68181855600002));
#274754=CARTESIAN_POINT('Ctrl Pts',(-9.42423552100006,15.2,-5.68123177400001));
#274755=CARTESIAN_POINT('Ctrl Pts',(-9.42423552100006,11.6,-5.68123177400001));
#274756=CARTESIAN_POINT('Ctrl Pts',(-9.42122232700006,15.2,-5.68064355000002));
#274757=CARTESIAN_POINT('Ctrl Pts',(-9.42122232700006,11.6,-5.68064355000002));
#274758=CARTESIAN_POINT('Ctrl Pts',(-9.41821481900006,15.2,-5.68005389300002));
#274759=CARTESIAN_POINT('Ctrl Pts',(-9.41821481900006,11.6,-5.68005389300002));
#274760=CARTESIAN_POINT('Ctrl Pts',(-9.41521300400006,15.2,-5.67946281100002));
#274761=CARTESIAN_POINT('Ctrl Pts',(-9.41521300400006,11.6,-5.67946281100002));
#274762=CARTESIAN_POINT('Ctrl Pts',(-9.41221689100006,15.2,-5.67887031500002));
#274763=CARTESIAN_POINT('Ctrl Pts',(-9.41221689100006,11.6,-5.67887031500002));
#274764=CARTESIAN_POINT('Ctrl Pts',(-9.40922648700005,15.2,-5.67827641200001));
#274765=CARTESIAN_POINT('Ctrl Pts',(-9.40922648700005,11.6,-5.67827641200001));
#274766=CARTESIAN_POINT('Ctrl Pts',(-9.40624180100006,15.2,-5.67768111200002));
#274767=CARTESIAN_POINT('Ctrl Pts',(-9.40624180100006,11.6,-5.67768111200002));
#274768=CARTESIAN_POINT('Ctrl Pts',(-9.40326283700006,15.2,-5.67708442400002));
#274769=CARTESIAN_POINT('Ctrl Pts',(-9.40326283700006,11.6,-5.67708442400002));
#274770=CARTESIAN_POINT('Ctrl Pts',(-9.40028960800005,15.2,-5.67648635800002));
#274771=CARTESIAN_POINT('Ctrl Pts',(-9.40028960800005,11.6,-5.67648635800002));
#274772=CARTESIAN_POINT('Ctrl Pts',(-9.39732211800006,15.2,-5.67588692100002));
#274773=CARTESIAN_POINT('Ctrl Pts',(-9.39732211800006,11.6,-5.67588692100002));
#274774=CARTESIAN_POINT('Ctrl Pts',(-9.39436037700006,15.2,-5.67528612600002));
#274775=CARTESIAN_POINT('Ctrl Pts',(-9.39436037700006,11.6,-5.67528612600002));
#274776=CARTESIAN_POINT('Ctrl Pts',(-9.39140439200006,15.2,-5.67468397800001));
#274777=CARTESIAN_POINT('Ctrl Pts',(-9.39140439200006,11.6,-5.67468397800001));
#274778=CARTESIAN_POINT('Ctrl Pts',(-9.38845417000006,15.2,-5.67408048900001));
#274779=CARTESIAN_POINT('Ctrl Pts',(-9.38845417000006,11.6,-5.67408048900001));
#274780=CARTESIAN_POINT('Ctrl Pts',(-9.38550971900005,15.2,-5.67347566700001));
#274781=CARTESIAN_POINT('Ctrl Pts',(-9.38550971900005,11.6,-5.67347566700001));
#274782=CARTESIAN_POINT('Ctrl Pts',(-9.38257104800006,15.2,-5.67286952400002));
#274783=CARTESIAN_POINT('Ctrl Pts',(-9.38257104800006,11.6,-5.67286952400002));
#274784=CARTESIAN_POINT('Ctrl Pts',(-9.37963816300006,15.2,-5.67226206500001));
#274785=CARTESIAN_POINT('Ctrl Pts',(-9.37963816300006,11.6,-5.67226206500001));
#274786=CARTESIAN_POINT('Ctrl Pts',(-9.37671107500006,15.2,-5.67165330200002));
#274787=CARTESIAN_POINT('Ctrl Pts',(-9.37671107500006,11.6,-5.67165330200002));
#274788=CARTESIAN_POINT('Ctrl Pts',(-9.37378978800006,15.2,-5.67104324400002));
#274789=CARTESIAN_POINT('Ctrl Pts',(-9.37378978800006,11.6,-5.67104324400002));
#274790=CARTESIAN_POINT('Ctrl Pts',(-9.37087431300006,15.2,-5.67043190100001));
#274791=CARTESIAN_POINT('Ctrl Pts',(-9.37087431300006,11.6,-5.67043190100001));
#274792=CARTESIAN_POINT('Ctrl Pts',(-9.36796465500005,15.2,-5.66981928200001));
#274793=CARTESIAN_POINT('Ctrl Pts',(-9.36796465500005,11.6,-5.66981928200001));
#274794=CARTESIAN_POINT('Ctrl Pts',(-9.36506082600006,15.2,-5.66920539600002));
#274795=CARTESIAN_POINT('Ctrl Pts',(-9.36506082600006,11.6,-5.66920539600002));
#274796=CARTESIAN_POINT('Ctrl Pts',(-9.36216282900006,15.2,-5.66859025300002));
#274797=CARTESIAN_POINT('Ctrl Pts',(-9.36216282900006,11.6,-5.66859025300002));
#274798=CARTESIAN_POINT('Ctrl Pts',(-9.35927067600005,15.2,-5.66797386300002));
#274799=CARTESIAN_POINT('Ctrl Pts',(-9.35927067600005,11.6,-5.66797386300002));
#274800=CARTESIAN_POINT('Ctrl Pts',(-9.35638437300006,15.2,-5.66735623400002));
#274801=CARTESIAN_POINT('Ctrl Pts',(-9.35638437300006,11.6,-5.66735623400002));
#274802=CARTESIAN_POINT('Ctrl Pts',(-9.35350392700006,15.2,-5.66673737800001));
#274803=CARTESIAN_POINT('Ctrl Pts',(-9.35350392700006,11.6,-5.66673737800001));
#274804=CARTESIAN_POINT('Ctrl Pts',(-9.35062934800006,15.2,-5.66611730200002));
#274805=CARTESIAN_POINT('Ctrl Pts',(-9.35062934800006,11.6,-5.66611730200002));
#274806=CARTESIAN_POINT('Ctrl Pts',(-9.34776064400006,15.2,-5.66549601900002));
#274807=CARTESIAN_POINT('Ctrl Pts',(-9.34776064400006,11.6,-5.66549601900002));
#274808=CARTESIAN_POINT('Ctrl Pts',(-9.34489782000006,15.2,-5.66487353500002));
#274809=CARTESIAN_POINT('Ctrl Pts',(-9.34489782000006,11.6,-5.66487353500002));
#274810=CARTESIAN_POINT('Ctrl Pts',(-9.34204088800006,15.2,-5.66424986100002));
#274811=CARTESIAN_POINT('Ctrl Pts',(-9.34204088800006,11.6,-5.66424986100002));
#274812=CARTESIAN_POINT('Ctrl Pts',(-9.33918985300006,15.2,-5.66362500900001));
#274813=CARTESIAN_POINT('Ctrl Pts',(-9.33918985300006,11.6,-5.66362500900001));
#274814=CARTESIAN_POINT('Ctrl Pts',(-9.33634472400006,15.2,-5.66299898600001));
#274815=CARTESIAN_POINT('Ctrl Pts',(-9.33634472400006,11.6,-5.66299898600001));
#274816=CARTESIAN_POINT('Ctrl Pts',(-9.33350550900006,15.2,-5.66237180200002));
#274817=CARTESIAN_POINT('Ctrl Pts',(-9.33350550900006,11.6,-5.66237180200002));
#274818=CARTESIAN_POINT('Ctrl Pts',(-9.33067221700006,15.2,-5.66174346800001));
#274819=CARTESIAN_POINT('Ctrl Pts',(-9.33067221700006,11.6,-5.66174346800001));
#274820=CARTESIAN_POINT('Ctrl Pts',(-9.32784485500006,15.2,-5.66111399300001));
#274821=CARTESIAN_POINT('Ctrl Pts',(-9.32784485500006,11.6,-5.66111399300001));
#274822=CARTESIAN_POINT('Ctrl Pts',(-9.32502343100006,15.2,-5.66048338800002));
#274823=CARTESIAN_POINT('Ctrl Pts',(-9.32502343100006,11.6,-5.66048338800002));
#274824=CARTESIAN_POINT('Ctrl Pts',(-9.32220795200006,15.2,-5.65985166300001));
#274825=CARTESIAN_POINT('Ctrl Pts',(-9.32220795200006,11.6,-5.65985166300001));
#274826=CARTESIAN_POINT('Ctrl Pts',(-9.31939842900006,15.2,-5.65921882600002));
#274827=CARTESIAN_POINT('Ctrl Pts',(-9.31939842900006,11.6,-5.65921882600002));
#274828=CARTESIAN_POINT('Ctrl Pts',(-9.31659486700006,15.2,-5.65858488800002));
#274829=CARTESIAN_POINT('Ctrl Pts',(-9.31659486700006,11.6,-5.65858488800002));
#274830=CARTESIAN_POINT('Ctrl Pts',(-9.31379727700006,15.2,-5.65794986000002));
#274831=CARTESIAN_POINT('Ctrl Pts',(-9.31379727700006,11.6,-5.65794986000002));
#274832=CARTESIAN_POINT('Ctrl Pts',(-9.31100566500006,15.2,-5.65731375100002));
#274833=CARTESIAN_POINT('Ctrl Pts',(-9.31100566500006,11.6,-5.65731375100002));
#274834=CARTESIAN_POINT('Ctrl Pts',(-9.30822003900006,15.2,-5.65667657100001));
#274835=CARTESIAN_POINT('Ctrl Pts',(-9.30822003900006,11.6,-5.65667657100001));
#274836=CARTESIAN_POINT('Ctrl Pts',(-9.30544040900006,15.2,-5.65603833100001));
#274837=CARTESIAN_POINT('Ctrl Pts',(-9.30544040900006,11.6,-5.65603833100001));
#274838=CARTESIAN_POINT('Ctrl Pts',(-9.30266678100006,15.2,-5.65539904000002));
#274839=CARTESIAN_POINT('Ctrl Pts',(-9.30266678100006,11.6,-5.65539904000002));
#274840=CARTESIAN_POINT('Ctrl Pts',(-9.29989916500006,15.2,-5.65475871000002));
#274841=CARTESIAN_POINT('Ctrl Pts',(-9.29989916500006,11.6,-5.65475871000002));
#274842=CARTESIAN_POINT('Ctrl Pts',(-9.29713756800006,15.2,-5.65411734800002));
#274843=CARTESIAN_POINT('Ctrl Pts',(-9.29713756800006,11.6,-5.65411734800002));
#274844=CARTESIAN_POINT('Ctrl Pts',(-9.29438199800006,15.2,-5.65347496700002));
#274845=CARTESIAN_POINT('Ctrl Pts',(-9.29438199800006,11.6,-5.65347496700002));
#274846=CARTESIAN_POINT('Ctrl Pts',(-9.29163246500006,15.2,-5.65283157600001));
#274847=CARTESIAN_POINT('Ctrl Pts',(-9.29163246500006,11.6,-5.65283157600001));
#274848=CARTESIAN_POINT('Ctrl Pts',(-9.28888897500006,15.2,-5.65218718600002));
#274849=CARTESIAN_POINT('Ctrl Pts',(-9.28888897500006,11.6,-5.65218718600002));
#274850=CARTESIAN_POINT('Ctrl Pts',(-9.28615153700006,15.2,-5.65154180700001));
#274851=CARTESIAN_POINT('Ctrl Pts',(-9.28615153700006,11.6,-5.65154180700001));
#274852=CARTESIAN_POINT('Ctrl Pts',(-9.28342015900006,15.2,-5.65089545000002));
#274853=CARTESIAN_POINT('Ctrl Pts',(-9.28342015900006,11.6,-5.65089545000002));
#274854=CARTESIAN_POINT('Ctrl Pts',(-9.28069485100006,15.2,-5.65024812400001));
#274855=CARTESIAN_POINT('Ctrl Pts',(-9.28069485100006,11.6,-5.65024812400001));
#274856=CARTESIAN_POINT('Ctrl Pts',(-9.27797561900006,15.2,-5.64959984000001));
#274857=CARTESIAN_POINT('Ctrl Pts',(-9.27797561900006,11.6,-5.64959984000001));
#274858=CARTESIAN_POINT('Ctrl Pts',(-9.27526247200005,15.2,-5.64895060900001));
#274859=CARTESIAN_POINT('Ctrl Pts',(-9.27526247200005,11.6,-5.64895060900001));
#274860=CARTESIAN_POINT('Ctrl Pts',(-9.27255541900006,15.2,-5.64830044000002));
#274861=CARTESIAN_POINT('Ctrl Pts',(-9.27255541900006,11.6,-5.64830044000002));
#274862=CARTESIAN_POINT('Ctrl Pts',(-9.26985446700006,15.2,-5.64764934600001));
#274863=CARTESIAN_POINT('Ctrl Pts',(-9.26985446700006,11.6,-5.64764934600001));
#274864=CARTESIAN_POINT('Ctrl Pts',(-9.26715962600005,15.2,-5.64699733600001));
#274865=CARTESIAN_POINT('Ctrl Pts',(-9.26715962600005,11.6,-5.64699733600001));
#274866=CARTESIAN_POINT('Ctrl Pts',(-9.26447090200006,15.2,-5.64634441900001));
#274867=CARTESIAN_POINT('Ctrl Pts',(-9.26447090200006,11.6,-5.64634441900001));
#274868=CARTESIAN_POINT('Ctrl Pts',(-9.26178830500006,15.2,-5.64569061000002));
#274869=CARTESIAN_POINT('Ctrl Pts',(-9.26178830500006,11.6,-5.64569061000002));
#274870=CARTESIAN_POINT('Ctrl Pts',(-9.25911184300006,15.2,-5.64503591500001));
#274871=CARTESIAN_POINT('Ctrl Pts',(-9.25911184300006,11.6,-5.64503591500001));
#274872=CARTESIAN_POINT('Ctrl Pts',(-9.25644152500006,15.2,-5.64438034700002));
#274873=CARTESIAN_POINT('Ctrl Pts',(-9.25644152500006,11.6,-5.64438034700002));
#274874=CARTESIAN_POINT('Ctrl Pts',(-9.25377735900006,15.2,-5.64372391600001));
#274875=CARTESIAN_POINT('Ctrl Pts',(-9.25377735900006,11.6,-5.64372391600001));
#274876=CARTESIAN_POINT('Ctrl Pts',(-9.25111935200006,15.2,-5.64306663200002));
#274877=CARTESIAN_POINT('Ctrl Pts',(-9.25111935200006,11.6,-5.64306663200002));
#274878=CARTESIAN_POINT('Ctrl Pts',(-9.24846751400005,15.2,-5.64240850900001));
#274879=CARTESIAN_POINT('Ctrl Pts',(-9.24846751400005,11.6,-5.64240850900001));
#274880=CARTESIAN_POINT('Ctrl Pts',(-9.24582185200006,15.2,-5.64174955400001));
#274881=CARTESIAN_POINT('Ctrl Pts',(-9.24582185200006,11.6,-5.64174955400001));
#274882=CARTESIAN_POINT('Ctrl Pts',(-9.24318237700006,15.2,-5.64108978000001));
#274883=CARTESIAN_POINT('Ctrl Pts',(-9.24318237700006,11.6,-5.64108978000001));
#274884=CARTESIAN_POINT('Ctrl Pts',(-9.24054909400006,15.2,-5.64042919800002));
#274885=CARTESIAN_POINT('Ctrl Pts',(-9.24054909400006,11.6,-5.64042919800002));
#274886=CARTESIAN_POINT('Ctrl Pts',(-9.23792201400006,15.2,-5.63976781700001));
#274887=CARTESIAN_POINT('Ctrl Pts',(-9.23792201400006,11.6,-5.63976781700001));
#274888=CARTESIAN_POINT('Ctrl Pts',(-9.23530114500006,15.2,-5.63910565000001));
#274889=CARTESIAN_POINT('Ctrl Pts',(-9.23530114500006,11.6,-5.63910565000001));
#274890=CARTESIAN_POINT('Ctrl Pts',(-9.23268649500006,15.2,-5.63844270600002));
#274891=CARTESIAN_POINT('Ctrl Pts',(-9.23268649500006,11.6,-5.63844270600002));
#274892=CARTESIAN_POINT('Ctrl Pts',(-9.23007807100005,15.2,-5.63777899800002));
#274893=CARTESIAN_POINT('Ctrl Pts',(-9.23007807100005,11.6,-5.63777899800002));
#274894=CARTESIAN_POINT('Ctrl Pts',(-9.22747588600006,15.2,-5.63711453700002));
#274895=CARTESIAN_POINT('Ctrl Pts',(-9.22747588600006,11.6,-5.63711453700002));
#274896=CARTESIAN_POINT('Ctrl Pts',(-9.22487994400005,15.2,-5.63644933100001));
#274897=CARTESIAN_POINT('Ctrl Pts',(-9.22487994400005,11.6,-5.63644933100001));
#274898=CARTESIAN_POINT('Ctrl Pts',(-9.22229025500006,15.2,-5.63578339500001));
#274899=CARTESIAN_POINT('Ctrl Pts',(-9.22229025500006,11.6,-5.63578339500001));
#274900=CARTESIAN_POINT('Ctrl Pts',(-9.21970682800006,15.2,-5.63511673800001));
#274901=CARTESIAN_POINT('Ctrl Pts',(-9.21970682800006,11.6,-5.63511673800001));
#274902=CARTESIAN_POINT('Ctrl Pts',(-9.21712967100006,15.2,-5.63444937200002));
#274903=CARTESIAN_POINT('Ctrl Pts',(-9.21712967100006,11.6,-5.63444937200002));
#274904=CARTESIAN_POINT('Ctrl Pts',(-9.21455879300006,15.2,-5.63378130700002));
#274905=CARTESIAN_POINT('Ctrl Pts',(-9.21455879300006,11.6,-5.63378130700002));
#274906=CARTESIAN_POINT('Ctrl Pts',(-9.21199420300006,15.2,-5.63311255500002));
#274907=CARTESIAN_POINT('Ctrl Pts',(-9.21199420300006,11.6,-5.63311255500002));
#274908=CARTESIAN_POINT('Ctrl Pts',(-9.20943590900006,15.2,-5.63244312900002));
#274909=CARTESIAN_POINT('Ctrl Pts',(-9.20943590900006,11.6,-5.63244312900002));
#274910=CARTESIAN_POINT('Ctrl Pts',(-9.20688391900006,15.2,-5.63177303700002));
#274911=CARTESIAN_POINT('Ctrl Pts',(-9.20688391900006,11.6,-5.63177303700002));
#274912=CARTESIAN_POINT('Ctrl Pts',(-9.20433824200006,15.2,-5.63110229300001));
#274913=CARTESIAN_POINT('Ctrl Pts',(-9.20433824200006,11.6,-5.63110229300001));
#274914=CARTESIAN_POINT('Ctrl Pts',(-9.20179888700006,15.2,-5.63043090700001));
#274915=CARTESIAN_POINT('Ctrl Pts',(-9.20179888700006,11.6,-5.63043090700001));
#274916=CARTESIAN_POINT('Ctrl Pts',(-9.19926586300006,15.2,-5.62975889100001));
#274917=CARTESIAN_POINT('Ctrl Pts',(-9.19926586300006,11.6,-5.62975889100001));
#274918=CARTESIAN_POINT('Ctrl Pts',(-9.19673917800005,15.2,-5.62908625600001));
#274919=CARTESIAN_POINT('Ctrl Pts',(-9.19673917800005,11.6,-5.62908625600001));
#274920=CARTESIAN_POINT('Ctrl Pts',(-9.19421884100006,15.2,-5.62841301400002));
#274921=CARTESIAN_POINT('Ctrl Pts',(-9.19421884100006,11.6,-5.62841301400002));
#274922=CARTESIAN_POINT('Ctrl Pts',(-9.19170486100005,15.2,-5.62773917700001));
#274923=CARTESIAN_POINT('Ctrl Pts',(-9.19170486100005,11.6,-5.62773917700001));
#274924=CARTESIAN_POINT('Ctrl Pts',(-9.18919724600006,15.2,-5.62706475600002));
#274925=CARTESIAN_POINT('Ctrl Pts',(-9.18919724600006,11.6,-5.62706475600002));
#274926=CARTESIAN_POINT('Ctrl Pts',(-9.18669600500006,15.2,-5.62638976200001));
#274927=CARTESIAN_POINT('Ctrl Pts',(-9.18669600500006,11.6,-5.62638976200001));
#274928=CARTESIAN_POINT('Ctrl Pts',(-9.18420114700006,15.2,-5.62571420700001));
#274929=CARTESIAN_POINT('Ctrl Pts',(-9.18420114700006,11.6,-5.62571420700001));
#274930=CARTESIAN_POINT('Ctrl Pts',(-9.18171268000006,15.2,-5.62503810300001));
#274931=CARTESIAN_POINT('Ctrl Pts',(-9.18171268000006,11.6,-5.62503810300001));
#274932=CARTESIAN_POINT('Ctrl Pts',(-9.17923061300005,15.2,-5.62436146200001));
#274933=CARTESIAN_POINT('Ctrl Pts',(-9.17923061300005,11.6,-5.62436146200001));
#274934=CARTESIAN_POINT('Ctrl Pts',(-9.17675495600006,15.2,-5.62368429500001));
#274935=CARTESIAN_POINT('Ctrl Pts',(-9.17675495600006,11.6,-5.62368429500001));
#274936=CARTESIAN_POINT('Ctrl Pts',(-9.17428571800006,15.2,-5.62300661500001));
#274937=CARTESIAN_POINT('Ctrl Pts',(-9.17428571800006,11.6,-5.62300661500001));
#274938=CARTESIAN_POINT('Ctrl Pts',(-9.17182290500006,15.2,-5.62232843300002));
#274939=CARTESIAN_POINT('Ctrl Pts',(-9.17182290500006,11.6,-5.62232843300002));
#274940=CARTESIAN_POINT('Ctrl Pts',(-9.16936652800005,15.2,-5.62164975900002));
#274941=CARTESIAN_POINT('Ctrl Pts',(-9.16936652800005,11.6,-5.62164975900002));
#274942=CARTESIAN_POINT('Ctrl Pts',(-9.16691659500006,15.2,-5.62097060900001));
#274943=CARTESIAN_POINT('Ctrl Pts',(-9.16691659500006,11.6,-5.62097060900001));
#274944=CARTESIAN_POINT('Ctrl Pts',(-9.16447311600006,15.2,-5.62029099200001));
#274945=CARTESIAN_POINT('Ctrl Pts',(-9.16447311600006,11.6,-5.62029099200001));
#274946=CARTESIAN_POINT('Ctrl Pts',(-9.16203609900006,15.2,-5.61961092000002));
#274947=CARTESIAN_POINT('Ctrl Pts',(-9.16203609900006,11.6,-5.61961092000002));
#274948=CARTESIAN_POINT('Ctrl Pts',(-9.15960555200006,15.2,-5.61893040700001));
#274949=CARTESIAN_POINT('Ctrl Pts',(-9.15960555200006,11.6,-5.61893040700001));
#274950=CARTESIAN_POINT('Ctrl Pts',(-9.15718148700006,15.2,-5.61824946300002));
#274951=CARTESIAN_POINT('Ctrl Pts',(-9.15718148700006,11.6,-5.61824946300002));
#274952=CARTESIAN_POINT('Ctrl Pts',(-9.15476390900006,15.2,-5.61756810200002));
#274953=CARTESIAN_POINT('Ctrl Pts',(-9.15476390900006,11.6,-5.61756810200002));
#274954=CARTESIAN_POINT('Ctrl Pts',(-9.15235283000005,15.2,-5.61688633300002));
#274955=CARTESIAN_POINT('Ctrl Pts',(-9.15235283000005,11.6,-5.61688633300002));
#274956=CARTESIAN_POINT('Ctrl Pts',(-9.14994825800006,15.2,-5.61620417200002));
#274957=CARTESIAN_POINT('Ctrl Pts',(-9.14994825800006,11.6,-5.61620417200002));
#274958=CARTESIAN_POINT('Ctrl Pts',(-9.14755020200005,15.2,-5.61552162900002));
#274959=CARTESIAN_POINT('Ctrl Pts',(-9.14755020200005,11.6,-5.61552162900002));
#274960=CARTESIAN_POINT('Ctrl Pts',(-9.14515866900006,15.2,-5.61483871700001));
#274961=CARTESIAN_POINT('Ctrl Pts',(-9.14515866900006,11.6,-5.61483871700001));
#274962=CARTESIAN_POINT('Ctrl Pts',(-9.14277367200006,15.2,-5.61415544800001));
#274963=CARTESIAN_POINT('Ctrl Pts',(-9.14277367200006,11.6,-5.61415544800001));
#274964=CARTESIAN_POINT('Ctrl Pts',(-9.14039521600006,15.2,-5.61347183400001));
#274965=CARTESIAN_POINT('Ctrl Pts',(-9.14039521600006,11.6,-5.61347183400001));
#274966=CARTESIAN_POINT('Ctrl Pts',(-9.13802331300005,15.2,-5.61278788800001));
#274967=CARTESIAN_POINT('Ctrl Pts',(-9.13802331300005,11.6,-5.61278788800001));
#274968=CARTESIAN_POINT('Ctrl Pts',(-9.13565797000006,15.2,-5.61210362300002));
#274969=CARTESIAN_POINT('Ctrl Pts',(-9.13565797000006,11.6,-5.61210362300002));
#274970=CARTESIAN_POINT('Ctrl Pts',(-9.13329919900006,15.2,-5.61141905000001));
#274971=CARTESIAN_POINT('Ctrl Pts',(-9.13329919900006,11.6,-5.61141905000001));
#274972=CARTESIAN_POINT('Ctrl Pts',(-9.13094700500006,15.2,-5.61073418300001));
#274973=CARTESIAN_POINT('Ctrl Pts',(-9.13094700500006,11.6,-5.61073418300001));
#274974=CARTESIAN_POINT('Ctrl Pts',(-9.12860140000006,15.2,-5.61004903300002));
#274975=CARTESIAN_POINT('Ctrl Pts',(-9.12860140000006,11.6,-5.61004903300002));
#274976=CARTESIAN_POINT('Ctrl Pts',(-9.12626239200005,15.2,-5.60936361300001));
#274977=CARTESIAN_POINT('Ctrl Pts',(-9.12626239200005,11.6,-5.60936361300001));
#274978=CARTESIAN_POINT('Ctrl Pts',(-9.12392999100006,15.2,-5.60867793700002));
#274979=CARTESIAN_POINT('Ctrl Pts',(-9.12392999100006,11.6,-5.60867793700002));
#274980=CARTESIAN_POINT('Ctrl Pts',(-9.12160420500006,15.2,-5.60799201600001));
#274981=CARTESIAN_POINT('Ctrl Pts',(-9.12160420500006,11.6,-5.60799201600001));
#274982=CARTESIAN_POINT('Ctrl Pts',(-9.11928504400005,15.2,-5.60730586400001));
#274983=CARTESIAN_POINT('Ctrl Pts',(-9.11928504400005,11.6,-5.60730586400001));
#274984=CARTESIAN_POINT('Ctrl Pts',(-9.11697251700006,15.2,-5.60661949300002));
#274985=CARTESIAN_POINT('Ctrl Pts',(-9.11697251700006,11.6,-5.60661949300002));
#274986=CARTESIAN_POINT('Ctrl Pts',(-9.11466663400006,15.2,-5.60593291600001));
#274987=CARTESIAN_POINT('Ctrl Pts',(-9.11466663400006,11.6,-5.60593291600001));
#274988=CARTESIAN_POINT('Ctrl Pts',(-9.11236740200006,15.2,-5.60524614600002));
#274989=CARTESIAN_POINT('Ctrl Pts',(-9.11236740200006,11.6,-5.60524614600002));
#274990=CARTESIAN_POINT('Ctrl Pts',(-9.11007483200006,15.2,-5.60455919500002));
#274991=CARTESIAN_POINT('Ctrl Pts',(-9.11007483200006,11.6,-5.60455919500002));
#274992=CARTESIAN_POINT('Ctrl Pts',(-9.10778893400006,15.2,-5.60387207800002));
#274993=CARTESIAN_POINT('Ctrl Pts',(-9.10778893400006,11.6,-5.60387207800002));
#274994=CARTESIAN_POINT('Ctrl Pts',(-9.10550971500006,15.2,-5.60318480500001));
#274995=CARTESIAN_POINT('Ctrl Pts',(-9.10550971500006,11.6,-5.60318480500001));
#274996=CARTESIAN_POINT('Ctrl Pts',(-9.10323718600005,15.2,-5.60249739200001));
#274997=CARTESIAN_POINT('Ctrl Pts',(-9.10323718600005,11.6,-5.60249739200001));
#274998=CARTESIAN_POINT('Ctrl Pts',(-9.10097135600006,15.2,-5.60180985000001));
#274999=CARTESIAN_POINT('Ctrl Pts',(-9.10097135600006,11.6,-5.60180985000001));
#275000=CARTESIAN_POINT('Ctrl Pts',(-9.09871223500006,15.2,-5.60112219300001));
#275001=CARTESIAN_POINT('Ctrl Pts',(-9.09871223500006,11.6,-5.60112219300001));
#275002=CARTESIAN_POINT('Ctrl Pts',(-9.09645983100006,15.2,-5.60043443500001));
#275003=CARTESIAN_POINT('Ctrl Pts',(-9.09645983100006,11.6,-5.60043443500001));
#275004=CARTESIAN_POINT('Ctrl Pts',(-9.09421415200006,15.2,-5.59974658700002));
#275005=CARTESIAN_POINT('Ctrl Pts',(-9.09421415200006,11.6,-5.59974658700002));
#275006=CARTESIAN_POINT('Ctrl Pts',(-9.09197521100005,15.2,-5.59905866400001));
#275007=CARTESIAN_POINT('Ctrl Pts',(-9.09197521100005,11.6,-5.59905866400001));
#275008=CARTESIAN_POINT('Ctrl Pts',(-9.08974301600006,15.2,-5.59837067900002));
#275009=CARTESIAN_POINT('Ctrl Pts',(-9.08974301600006,11.6,-5.59837067900002));
#275010=CARTESIAN_POINT('Ctrl Pts',(-9.08751757500006,15.2,-5.59768264400001));
#275011=CARTESIAN_POINT('Ctrl Pts',(-9.08751757500006,11.6,-5.59768264400001));
#275012=CARTESIAN_POINT('Ctrl Pts',(-9.08529889900005,15.2,-5.59699457500002));
#275013=CARTESIAN_POINT('Ctrl Pts',(-9.08529889900005,11.6,-5.59699457500002));
#275014=CARTESIAN_POINT('Ctrl Pts',(-9.08308699800006,15.2,-5.59630648300002));
#275015=CARTESIAN_POINT('Ctrl Pts',(-9.08308699800006,11.6,-5.59630648300002));
#275016=CARTESIAN_POINT('Ctrl Pts',(-9.08088188000006,15.2,-5.59561838200001));
#275017=CARTESIAN_POINT('Ctrl Pts',(-9.08088188000006,11.6,-5.59561838200001));
#275018=CARTESIAN_POINT('Ctrl Pts',(-9.07868355400005,15.2,-5.59493028700001));
#275019=CARTESIAN_POINT('Ctrl Pts',(-9.07868355400005,11.6,-5.59493028700001));
#275020=CARTESIAN_POINT('Ctrl Pts',(-9.07649203200006,15.2,-5.59424221100001));
#275021=CARTESIAN_POINT('Ctrl Pts',(-9.07649203200006,11.6,-5.59424221100001));
#275022=CARTESIAN_POINT('Ctrl Pts',(-9.07430732100006,15.2,-5.59355416500001));
#275023=CARTESIAN_POINT('Ctrl Pts',(-9.07430732100006,11.6,-5.59355416500001));
#275024=CARTESIAN_POINT('Ctrl Pts',(-9.07212943200006,15.2,-5.59286616700001));
#275025=CARTESIAN_POINT('Ctrl Pts',(-9.07212943200006,11.6,-5.59286616700001));
#275026=CARTESIAN_POINT('Ctrl Pts',(-9.06995837500006,15.2,-5.59217822700001));
#275027=CARTESIAN_POINT('Ctrl Pts',(-9.06995837500006,11.6,-5.59217822700001));
#275028=CARTESIAN_POINT('Ctrl Pts',(-9.06779415800005,15.2,-5.59149036100001));
#275029=CARTESIAN_POINT('Ctrl Pts',(-9.06779415800005,11.6,-5.59149036100001));
#275030=CARTESIAN_POINT('Ctrl Pts',(-9.06563679200006,15.2,-5.59080258200002));
#275031=CARTESIAN_POINT('Ctrl Pts',(-9.06563679200006,11.6,-5.59080258200002));
#275032=CARTESIAN_POINT('Ctrl Pts',(-9.06348628500006,15.2,-5.59011490300001));
#275033=CARTESIAN_POINT('Ctrl Pts',(-9.06348628500006,11.6,-5.59011490300001));
#275034=CARTESIAN_POINT('Ctrl Pts',(-9.06134264800006,15.2,-5.58942734000002));
#275035=CARTESIAN_POINT('Ctrl Pts',(-9.06134264800006,11.6,-5.58942734000002));
#275036=CARTESIAN_POINT('Ctrl Pts',(-9.05920589100005,15.2,-5.58873990500001));
#275037=CARTESIAN_POINT('Ctrl Pts',(-9.05920589100005,11.6,-5.58873990500001));
#275038=CARTESIAN_POINT('Ctrl Pts',(-9.05707602300006,15.2,-5.58805261300002));
#275039=CARTESIAN_POINT('Ctrl Pts',(-9.05707602300006,11.6,-5.58805261300002));
#275040=CARTESIAN_POINT('Ctrl Pts',(-9.05495305400006,15.2,-5.58736547900001));
#275041=CARTESIAN_POINT('Ctrl Pts',(-9.05495305400006,11.6,-5.58736547900001));
#275042=CARTESIAN_POINT('Ctrl Pts',(-9.05283699300006,15.2,-5.58667851400001));
#275043=CARTESIAN_POINT('Ctrl Pts',(-9.05283699300006,11.6,-5.58667851400001));
#275044=CARTESIAN_POINT('Ctrl Pts',(-9.05072785100005,15.2,-5.58599173500001));
#275045=CARTESIAN_POINT('Ctrl Pts',(-9.05072785100005,11.6,-5.58599173500001));
#275046=CARTESIAN_POINT('Ctrl Pts',(-9.04862563600006,15.2,-5.58530515500001));
#275047=CARTESIAN_POINT('Ctrl Pts',(-9.04862563600006,11.6,-5.58530515500001));
#275048=CARTESIAN_POINT('Ctrl Pts',(-9.04653036000006,15.2,-5.58461878900002));
#275049=CARTESIAN_POINT('Ctrl Pts',(-9.04653036000006,11.6,-5.58461878900002));
#275050=CARTESIAN_POINT('Ctrl Pts',(-9.04444203100006,15.2,-5.58393265000001));
#275051=CARTESIAN_POINT('Ctrl Pts',(-9.04444203100006,11.6,-5.58393265000001));
#275052=CARTESIAN_POINT('Ctrl Pts',(-9.04236066000006,15.2,-5.58324675400002));
#275053=CARTESIAN_POINT('Ctrl Pts',(-9.04236066000006,11.6,-5.58324675400002));
#275054=CARTESIAN_POINT('Ctrl Pts',(-9.04028625700006,15.2,-5.58256111400001));
#275055=CARTESIAN_POINT('Ctrl Pts',(-9.04028625700006,11.6,-5.58256111400001));
#275056=CARTESIAN_POINT('Ctrl Pts',(-9.03821883100006,15.2,-5.58187574600002));
#275057=CARTESIAN_POINT('Ctrl Pts',(-9.03821883100006,11.6,-5.58187574600002));
#275058=CARTESIAN_POINT('Ctrl Pts',(-9.03615839200006,15.2,-5.58119066200002));
#275059=CARTESIAN_POINT('Ctrl Pts',(-9.03615839200006,11.6,-5.58119066200002));
#275060=CARTESIAN_POINT('Ctrl Pts',(-9.03410494900006,15.2,-5.58050587900001));
#275061=CARTESIAN_POINT('Ctrl Pts',(-9.03410494900006,11.6,-5.58050587900001));
#275062=CARTESIAN_POINT('Ctrl Pts',(-9.03205851500006,15.2,-5.57982141200001));
#275063=CARTESIAN_POINT('Ctrl Pts',(-9.03205851500006,11.6,-5.57982141200001));
#275064=CARTESIAN_POINT('Ctrl Pts',(-9.03001909700006,15.2,-5.57913727300001));
#275065=CARTESIAN_POINT('Ctrl Pts',(-9.03001909700006,11.6,-5.57913727300001));
#275066=CARTESIAN_POINT('Ctrl Pts',(-9.02798670700006,15.2,-5.57845347800002));
#275067=CARTESIAN_POINT('Ctrl Pts',(-9.02798670700006,11.6,-5.57845347800002));
#275068=CARTESIAN_POINT('Ctrl Pts',(-9.02596135300006,15.2,-5.57777004200001));
#275069=CARTESIAN_POINT('Ctrl Pts',(-9.02596135300006,11.6,-5.57777004200001));
#275070=CARTESIAN_POINT('Ctrl Pts',(-9.02394304700006,15.2,-5.57708698000001));
#275071=CARTESIAN_POINT('Ctrl Pts',(-9.02394304700006,11.6,-5.57708698000001));
#275072=CARTESIAN_POINT('Ctrl Pts',(-9.02193179700006,15.2,-5.57640430700001));
#275073=CARTESIAN_POINT('Ctrl Pts',(-9.02193179700006,11.6,-5.57640430700001));
#275074=CARTESIAN_POINT('Ctrl Pts',(-9.01992761500006,15.2,-5.57572203700001));
#275075=CARTESIAN_POINT('Ctrl Pts',(-9.01992761500006,11.6,-5.57572203700001));
#275076=CARTESIAN_POINT('Ctrl Pts',(-9.01793051100006,15.2,-5.57504018600001));
#275077=CARTESIAN_POINT('Ctrl Pts',(-9.01793051100006,11.6,-5.57504018600001));
#275078=CARTESIAN_POINT('Ctrl Pts',(-9.01594049400006,15.2,-5.57435876800001));
#275079=CARTESIAN_POINT('Ctrl Pts',(-9.01594049400006,11.6,-5.57435876800001));
#275080=CARTESIAN_POINT('Ctrl Pts',(-9.01395757400006,15.2,-5.57367779900002));
#275081=CARTESIAN_POINT('Ctrl Pts',(-9.01395757400006,11.6,-5.57367779900002));
#275082=CARTESIAN_POINT('Ctrl Pts',(-9.01198176300005,15.2,-5.57299729300002));
#275083=CARTESIAN_POINT('Ctrl Pts',(-9.01198176300005,11.6,-5.57299729300002));
#275084=CARTESIAN_POINT('Ctrl Pts',(-9.01001306900006,15.2,-5.57231726600001));
#275085=CARTESIAN_POINT('Ctrl Pts',(-9.01001306900006,11.6,-5.57231726600001));
#275086=CARTESIAN_POINT('Ctrl Pts',(-9.00805150400006,15.2,-5.57163773500001));
#275087=CARTESIAN_POINT('Ctrl Pts',(-9.00805150400006,11.6,-5.57163773500001));
#275088=CARTESIAN_POINT('Ctrl Pts',(-9.00609707700006,15.2,-5.57095871100001));
#275089=CARTESIAN_POINT('Ctrl Pts',(-9.00609707700006,11.6,-5.57095871100001));
#275090=CARTESIAN_POINT('Ctrl Pts',(-9.00414979900006,15.2,-5.57028021300002));
#275091=CARTESIAN_POINT('Ctrl Pts',(-9.00414979900006,11.6,-5.57028021300002));
#275092=CARTESIAN_POINT('Ctrl Pts',(-9.00220967900006,15.2,-5.56960225700001));
#275093=CARTESIAN_POINT('Ctrl Pts',(-9.00220967900006,11.6,-5.56960225700001));
#275094=CARTESIAN_POINT('Ctrl Pts',(-9.00027673000006,15.2,-5.56892485600001));
#275095=CARTESIAN_POINT('Ctrl Pts',(-9.00027673000006,11.6,-5.56892485600001));
#275096=CARTESIAN_POINT('Ctrl Pts',(-8.99835095900006,15.2,-5.56824802500001));
#275097=CARTESIAN_POINT('Ctrl Pts',(-8.99835095900006,11.6,-5.56824802500001));
#275098=CARTESIAN_POINT('Ctrl Pts',(-8.99643237900005,15.2,-5.56757178200002));
#275099=CARTESIAN_POINT('Ctrl Pts',(-8.99643237900005,11.6,-5.56757178200002));
#275100=CARTESIAN_POINT('Ctrl Pts',(-8.99452100000006,15.2,-5.56689614200002));
#275101=CARTESIAN_POINT('Ctrl Pts',(-8.99452100000006,11.6,-5.56689614200002));
#275102=CARTESIAN_POINT('Ctrl Pts',(-8.99261683100006,15.2,-5.56622112000001));
#275103=CARTESIAN_POINT('Ctrl Pts',(-8.99261683100006,11.6,-5.56622112000001));
#275104=CARTESIAN_POINT('Ctrl Pts',(-8.99071988300006,15.2,-5.56554673300001));
#275105=CARTESIAN_POINT('Ctrl Pts',(-8.99071988300006,11.6,-5.56554673300001));
#275106=CARTESIAN_POINT('Ctrl Pts',(-8.98883016700006,15.2,-5.56487299500001));
#275107=CARTESIAN_POINT('Ctrl Pts',(-8.98883016700006,11.6,-5.56487299500001));
#275108=CARTESIAN_POINT('Ctrl Pts',(-8.98694769300005,15.2,-5.56419992300001));
#275109=CARTESIAN_POINT('Ctrl Pts',(-8.98694769300005,11.6,-5.56419992300001));
#275110=CARTESIAN_POINT('Ctrl Pts',(-8.98507247200006,15.2,-5.56352753400001));
#275111=CARTESIAN_POINT('Ctrl Pts',(-8.98507247200006,11.6,-5.56352753400001));
#275112=CARTESIAN_POINT('Ctrl Pts',(-8.98320451500006,15.2,-5.56285584200001));
#275113=CARTESIAN_POINT('Ctrl Pts',(-8.98320451500006,11.6,-5.56285584200001));
#275114=CARTESIAN_POINT('Ctrl Pts',(-8.98134383200006,15.2,-5.56218486400001));
#275115=CARTESIAN_POINT('Ctrl Pts',(-8.98134383200006,11.6,-5.56218486400001));
#275116=CARTESIAN_POINT('Ctrl Pts',(-8.97949043200006,15.2,-5.56151461700002));
#275117=CARTESIAN_POINT('Ctrl Pts',(-8.97949043200006,11.6,-5.56151461700002));
#275118=CARTESIAN_POINT('Ctrl Pts',(-8.97764432800006,15.2,-5.56084511500002));
#275119=CARTESIAN_POINT('Ctrl Pts',(-8.97764432800006,11.6,-5.56084511500002));
#275120=CARTESIAN_POINT('Ctrl Pts',(-8.97580552900006,15.2,-5.56017637700001));
#275121=CARTESIAN_POINT('Ctrl Pts',(-8.97580552900006,11.6,-5.56017637700001));
#275122=CARTESIAN_POINT('Ctrl Pts',(-8.97397404700006,15.2,-5.55950841800001));
#275123=CARTESIAN_POINT('Ctrl Pts',(-8.97397404700006,11.6,-5.55950841800001));
#275124=CARTESIAN_POINT('Ctrl Pts',(-8.97214989200006,15.2,-5.55884125300001));
#275125=CARTESIAN_POINT('Ctrl Pts',(-8.97214989200006,11.6,-5.55884125300001));
#275126=CARTESIAN_POINT('Ctrl Pts',(-8.97033307400006,15.2,-5.55817490100001));
#275127=CARTESIAN_POINT('Ctrl Pts',(-8.97033307400006,11.6,-5.55817490100001));
#275128=CARTESIAN_POINT('Ctrl Pts',(-8.96852360500005,15.2,-5.55750937700001));
#275129=CARTESIAN_POINT('Ctrl Pts',(-8.96852360500005,11.6,-5.55750937700001));
#275130=CARTESIAN_POINT('Ctrl Pts',(-8.96672149500005,15.2,-5.55684469700001));
#275131=CARTESIAN_POINT('Ctrl Pts',(-8.96672149500005,11.6,-5.55684469700001));
#275132=CARTESIAN_POINT('Ctrl Pts',(-8.96492675600006,15.2,-5.55618088000001));
#275133=CARTESIAN_POINT('Ctrl Pts',(-8.96492675600006,11.6,-5.55618088000001));
#275134=CARTESIAN_POINT('Ctrl Pts',(-8.96313939700006,15.2,-5.55551794000001));
#275135=CARTESIAN_POINT('Ctrl Pts',(-8.96313939700006,11.6,-5.55551794000001));
#275136=CARTESIAN_POINT('Ctrl Pts',(-8.96135943000005,15.2,-5.55485589600002));
#275137=CARTESIAN_POINT('Ctrl Pts',(-8.96135943000005,11.6,-5.55485589600002));
#275138=CARTESIAN_POINT('Ctrl Pts',(-8.95958686500006,15.2,-5.55419476300001));
#275139=CARTESIAN_POINT('Ctrl Pts',(-8.95958686500006,11.6,-5.55419476300001));
#275140=CARTESIAN_POINT('Ctrl Pts',(-8.95782171400005,15.2,-5.55353456000002));
#275141=CARTESIAN_POINT('Ctrl Pts',(-8.95782171400005,11.6,-5.55353456000002));
#275142=CARTESIAN_POINT('Ctrl Pts',(-8.95606398700006,15.2,-5.55287530100002));
#275143=CARTESIAN_POINT('Ctrl Pts',(-8.95606398700006,11.6,-5.55287530100002));
#275144=CARTESIAN_POINT('Ctrl Pts',(-8.95431369600006,15.2,-5.55221700600002));
#275145=CARTESIAN_POINT('Ctrl Pts',(-8.95431369600006,11.6,-5.55221700600002));
#275146=CARTESIAN_POINT('Ctrl Pts',(-8.95257085100006,15.2,-5.55155969100001));
#275147=CARTESIAN_POINT('Ctrl Pts',(-8.95257085100006,11.6,-5.55155969100001));
#275148=CARTESIAN_POINT('Ctrl Pts',(-8.95083546400006,15.2,-5.55090337200001));
#275149=CARTESIAN_POINT('Ctrl Pts',(-8.95083546400006,11.6,-5.55090337200001));
#275150=CARTESIAN_POINT('Ctrl Pts',(-8.94910754500006,15.2,-5.55024806800001));
#275151=CARTESIAN_POINT('Ctrl Pts',(-8.94910754500006,11.6,-5.55024806800001));
#275152=CARTESIAN_POINT('Ctrl Pts',(-8.94738710500006,15.2,-5.54959379500001));
#275153=CARTESIAN_POINT('Ctrl Pts',(-8.94738710500006,11.6,-5.54959379500001));
#275154=CARTESIAN_POINT('Ctrl Pts',(-8.94567415700006,15.2,-5.54894057200002));
#275155=CARTESIAN_POINT('Ctrl Pts',(-8.94567415700006,11.6,-5.54894057200002));
#275156=CARTESIAN_POINT('Ctrl Pts',(-8.94396871000006,15.2,-5.54828841500001));
#275157=CARTESIAN_POINT('Ctrl Pts',(-8.94396871000006,11.6,-5.54828841500001));
#275158=CARTESIAN_POINT('Ctrl Pts',(-8.94227077600006,15.2,-5.54763734200002));
#275159=CARTESIAN_POINT('Ctrl Pts',(-8.94227077600006,11.6,-5.54763734200002));
#275160=CARTESIAN_POINT('Ctrl Pts',(-8.94058036500006,15.2,-5.54698737000002));
#275161=CARTESIAN_POINT('Ctrl Pts',(-8.94058036500006,11.6,-5.54698737000002));
#275162=CARTESIAN_POINT('Ctrl Pts',(-8.93889749100006,15.2,-5.54633851800002));
#275163=CARTESIAN_POINT('Ctrl Pts',(-8.93889749100006,11.6,-5.54633851800002));
#275164=CARTESIAN_POINT('Ctrl Pts',(-8.93722216300005,15.2,-5.54569080200002));
#275165=CARTESIAN_POINT('Ctrl Pts',(-8.93722216300005,11.6,-5.54569080200002));
#275166=CARTESIAN_POINT('Ctrl Pts',(-8.93555439300006,15.2,-5.54504424100001));
#275167=CARTESIAN_POINT('Ctrl Pts',(-8.93555439300006,11.6,-5.54504424100001));
#275168=CARTESIAN_POINT('Ctrl Pts',(-8.93389419300006,15.2,-5.54439885300001));
#275169=CARTESIAN_POINT('Ctrl Pts',(-8.93389419300006,11.6,-5.54439885300001));
#275170=CARTESIAN_POINT('Ctrl Pts',(-8.93224157200006,15.2,-5.54375465500001));
#275171=CARTESIAN_POINT('Ctrl Pts',(-8.93224157200006,11.6,-5.54375465500001));
#275172=CARTESIAN_POINT('Ctrl Pts',(-8.93059654400006,15.2,-5.54311166500002));
#275173=CARTESIAN_POINT('Ctrl Pts',(-8.93059654400006,11.6,-5.54311166500002));
#275174=CARTESIAN_POINT('Ctrl Pts',(-8.92895911900006,15.2,-5.54246990200001));
#275175=CARTESIAN_POINT('Ctrl Pts',(-8.92895911900006,11.6,-5.54246990200001));
#275176=CARTESIAN_POINT('Ctrl Pts',(-8.92732930900005,15.2,-5.54182938400002));
#275177=CARTESIAN_POINT('Ctrl Pts',(-8.92732930900005,11.6,-5.54182938400002));
#275178=CARTESIAN_POINT('Ctrl Pts',(-8.92570712400006,15.2,-5.54119012900002));
#275179=CARTESIAN_POINT('Ctrl Pts',(-8.92570712400006,11.6,-5.54119012900002));
#275180=CARTESIAN_POINT('Ctrl Pts',(-8.92409257800006,15.2,-5.54055215500001));
#275181=CARTESIAN_POINT('Ctrl Pts',(-8.92409257800006,11.6,-5.54055215500001));
#275182=CARTESIAN_POINT('Ctrl Pts',(-8.92248568200005,15.2,-5.53991548100001));
#275183=CARTESIAN_POINT('Ctrl Pts',(-8.92248568200005,11.6,-5.53991548100001));
#275184=CARTESIAN_POINT('Ctrl Pts',(-8.92088644600006,15.2,-5.53928012400001));
#275185=CARTESIAN_POINT('Ctrl Pts',(-8.92088644600006,11.6,-5.53928012400001));
#275186=CARTESIAN_POINT('Ctrl Pts',(-8.91929488200006,15.2,-5.53864610500002));
#275187=CARTESIAN_POINT('Ctrl Pts',(-8.91929488200006,11.6,-5.53864610500002));
#275188=CARTESIAN_POINT('Ctrl Pts',(-8.91771100300006,15.2,-5.53801344000002));
#275189=CARTESIAN_POINT('Ctrl Pts',(-8.91771100300006,11.6,-5.53801344000002));
#275190=CARTESIAN_POINT('Ctrl Pts',(-8.91613481900006,15.2,-5.53738215000001));
#275191=CARTESIAN_POINT('Ctrl Pts',(-8.91613481900006,11.6,-5.53738215000001));
#275192=CARTESIAN_POINT('Ctrl Pts',(-8.91456634200006,15.2,-5.53675225200001));
#275193=CARTESIAN_POINT('Ctrl Pts',(-8.91456634200006,11.6,-5.53675225200001));
#275194=CARTESIAN_POINT('Ctrl Pts',(-8.91300558500006,15.2,-5.53612376600002));
#275195=CARTESIAN_POINT('Ctrl Pts',(-8.91300558500006,11.6,-5.53612376600002));
#275196=CARTESIAN_POINT('Ctrl Pts',(-8.91145255900006,15.2,-5.53549671000001));
#275197=CARTESIAN_POINT('Ctrl Pts',(-8.91145255900006,11.6,-5.53549671000001));
#275198=CARTESIAN_POINT('Ctrl Pts',(-8.90990727500006,15.2,-5.53487110500001));
#275199=CARTESIAN_POINT('Ctrl Pts',(-8.90990727500006,11.6,-5.53487110500001));
#275200=CARTESIAN_POINT('Ctrl Pts',(-8.90836974600006,15.2,-5.53424696600001));
#275201=CARTESIAN_POINT('Ctrl Pts',(-8.90836974600006,11.6,-5.53424696600001));
#275202=CARTESIAN_POINT('Ctrl Pts',(-8.90683998400006,15.2,-5.53362431600001));
#275203=CARTESIAN_POINT('Ctrl Pts',(-8.90683998400006,11.6,-5.53362431600001));
#275204=CARTESIAN_POINT('Ctrl Pts',(-8.90531800000005,15.2,-5.53300317300002));
#275205=CARTESIAN_POINT('Ctrl Pts',(-8.90531800000005,11.6,-5.53300317300002));
#275206=CARTESIAN_POINT('Ctrl Pts',(-8.90380380500006,15.2,-5.53238355600001));
#275207=CARTESIAN_POINT('Ctrl Pts',(-8.90380380500006,11.6,-5.53238355600001));
#275208=CARTESIAN_POINT('Ctrl Pts',(-8.90229741300006,15.2,-5.53176548500002));
#275209=CARTESIAN_POINT('Ctrl Pts',(-8.90229741300006,11.6,-5.53176548500002));
#275210=CARTESIAN_POINT('Ctrl Pts',(-8.90079883600006,15.2,-5.53114897800001));
#275211=CARTESIAN_POINT('Ctrl Pts',(-8.90079883600006,11.6,-5.53114897800001));
#275212=CARTESIAN_POINT('Ctrl Pts',(-8.89930808500005,15.2,-5.53053405700001));
#275213=CARTESIAN_POINT('Ctrl Pts',(-8.89930808500005,11.6,-5.53053405700001));
#275214=CARTESIAN_POINT('Ctrl Pts',(-8.89782517200005,15.2,-5.52992073900001));
#275215=CARTESIAN_POINT('Ctrl Pts',(-8.89782517200005,11.6,-5.52992073900001));
#275216=CARTESIAN_POINT('Ctrl Pts',(-8.89635011000006,15.2,-5.52930904500001));
#275217=CARTESIAN_POINT('Ctrl Pts',(-8.89635011000006,11.6,-5.52930904500001));
#275218=CARTESIAN_POINT('Ctrl Pts',(-8.89488291000006,15.2,-5.52869899600001));
#275219=CARTESIAN_POINT('Ctrl Pts',(-8.89488291000006,11.6,-5.52869899600001));
#275220=CARTESIAN_POINT('Ctrl Pts',(-8.89342358400006,15.2,-5.52809061000001));
#275221=CARTESIAN_POINT('Ctrl Pts',(-8.89342358400006,11.6,-5.52809061000001));
#275222=CARTESIAN_POINT('Ctrl Pts',(-8.89197214600006,15.2,-5.52748390800001));
#275223=CARTESIAN_POINT('Ctrl Pts',(-8.89197214600006,11.6,-5.52748390800001));
#275224=CARTESIAN_POINT('Ctrl Pts',(-8.89052860700006,15.2,-5.52687890900001));
#275225=CARTESIAN_POINT('Ctrl Pts',(-8.89052860700006,11.6,-5.52687890900001));
#275226=CARTESIAN_POINT('Ctrl Pts',(-8.88909298100005,15.2,-5.52627563500002));
#275227=CARTESIAN_POINT('Ctrl Pts',(-8.88909298100005,11.6,-5.52627563500002));
#275228=CARTESIAN_POINT('Ctrl Pts',(-8.88766527700006,15.2,-5.52567410500002));
#275229=CARTESIAN_POINT('Ctrl Pts',(-8.88766527700006,11.6,-5.52567410500002));
#275230=CARTESIAN_POINT('Ctrl Pts',(-8.88624550900006,15.2,-5.52507434000002));
#275231=CARTESIAN_POINT('Ctrl Pts',(-8.88624550900006,11.6,-5.52507434000002));
#275232=CARTESIAN_POINT('Ctrl Pts',(-8.88483369100006,15.2,-5.52447635900001));
#275233=CARTESIAN_POINT('Ctrl Pts',(-8.88483369100006,11.6,-5.52447635900001));
#275234=CARTESIAN_POINT('Ctrl Pts',(-8.88342983400005,15.2,-5.52388018300002));
#275235=CARTESIAN_POINT('Ctrl Pts',(-8.88342983400005,11.6,-5.52388018300002));
#275236=CARTESIAN_POINT('Ctrl Pts',(-8.88203395000006,15.2,-5.52328583400001));
#275237=CARTESIAN_POINT('Ctrl Pts',(-8.88203395000006,11.6,-5.52328583400001));
#275238=CARTESIAN_POINT('Ctrl Pts',(-8.88064605300006,15.2,-5.52269333100002));
#275239=CARTESIAN_POINT('Ctrl Pts',(-8.88064605300006,11.6,-5.52269333100002));
#275240=CARTESIAN_POINT('Ctrl Pts',(-8.87926615400006,15.2,-5.52210269500002));
#275241=CARTESIAN_POINT('Ctrl Pts',(-8.87926615400006,11.6,-5.52210269500002));
#275242=CARTESIAN_POINT('Ctrl Pts',(-8.87789426600006,15.2,-5.52151394800001));
#275243=CARTESIAN_POINT('Ctrl Pts',(-8.87789426600006,11.6,-5.52151394800001));
#275244=CARTESIAN_POINT('Ctrl Pts',(-8.87653040200006,15.2,-5.52092711100002));
#275245=CARTESIAN_POINT('Ctrl Pts',(-8.87653040200006,11.6,-5.52092711100002));
#275246=CARTESIAN_POINT('Ctrl Pts',(-8.87517457600006,15.2,-5.52034220400001));
#275247=CARTESIAN_POINT('Ctrl Pts',(-8.87517457600006,11.6,-5.52034220400001));
#275248=CARTESIAN_POINT('Ctrl Pts',(-8.87382679800006,15.2,-5.51975924800002));
#275249=CARTESIAN_POINT('Ctrl Pts',(-8.87382679800006,11.6,-5.51975924800002));
#275250=CARTESIAN_POINT('Ctrl Pts',(-8.87248708300006,15.2,-5.51917826500001));
#275251=CARTESIAN_POINT('Ctrl Pts',(-8.87248708300006,11.6,-5.51917826500001));
#275252=CARTESIAN_POINT('Ctrl Pts',(-8.87115544200006,15.2,-5.51859927600002));
#275253=CARTESIAN_POINT('Ctrl Pts',(-8.87115544200006,11.6,-5.51859927600002));
#275254=CARTESIAN_POINT('Ctrl Pts',(-8.86983189000006,15.2,-5.51802230200002));
#275255=CARTESIAN_POINT('Ctrl Pts',(-8.86983189000006,11.6,-5.51802230200002));
#275256=CARTESIAN_POINT('Ctrl Pts',(-8.86851643800006,15.2,-5.51744736600002));
#275257=CARTESIAN_POINT('Ctrl Pts',(-8.86851643800006,11.6,-5.51744736600002));
#275258=CARTESIAN_POINT('Ctrl Pts',(-8.86720910000006,15.2,-5.51687448900001));
#275259=CARTESIAN_POINT('Ctrl Pts',(-8.86720910000006,11.6,-5.51687448900001));
#275260=CARTESIAN_POINT('Ctrl Pts',(-8.86590988800006,15.2,-5.51630369100002));
#275261=CARTESIAN_POINT('Ctrl Pts',(-8.86590988800006,11.6,-5.51630369100002));
#275262=CARTESIAN_POINT('Ctrl Pts',(-8.86461881500006,15.2,-5.51573499500002));
#275263=CARTESIAN_POINT('Ctrl Pts',(-8.86461881500006,11.6,-5.51573499500002));
#275264=CARTESIAN_POINT('Ctrl Pts',(-8.86333589600006,15.2,-5.51516842500002));
#275265=CARTESIAN_POINT('Ctrl Pts',(-8.86333589600006,11.6,-5.51516842500002));
#275266=CARTESIAN_POINT('Ctrl Pts',(-8.86206114200006,15.2,-5.51460399900002));
#275267=CARTESIAN_POINT('Ctrl Pts',(-8.86206114200006,11.6,-5.51460399900002));
#275268=CARTESIAN_POINT('Ctrl Pts',(-8.86079456700006,15.2,-5.51404174200002));
#275269=CARTESIAN_POINT('Ctrl Pts',(-8.86079456700006,11.6,-5.51404174200002));
#275270=CARTESIAN_POINT('Ctrl Pts',(-8.85953618500006,15.2,-5.51348167500001));
#275271=CARTESIAN_POINT('Ctrl Pts',(-8.85953618500006,11.6,-5.51348167500001));
#275272=CARTESIAN_POINT('Ctrl Pts',(-8.85828600800006,15.2,-5.51292382200002));
#275273=CARTESIAN_POINT('Ctrl Pts',(-8.85828600800006,11.6,-5.51292382200002));
#275274=CARTESIAN_POINT('Ctrl Pts',(-8.85704404900006,15.2,-5.51236820300002));
#275275=CARTESIAN_POINT('Ctrl Pts',(-8.85704404900006,11.6,-5.51236820300002));
#275276=CARTESIAN_POINT('Ctrl Pts',(-8.85581032300006,15.2,-5.51181484300002));
#275277=CARTESIAN_POINT('Ctrl Pts',(-8.85581032300006,11.6,-5.51181484300002));
#275278=CARTESIAN_POINT('Ctrl Pts',(-8.85458484100005,15.2,-5.51126376300001));
#275279=CARTESIAN_POINT('Ctrl Pts',(-8.85458484100005,11.6,-5.51126376300001));
#275280=CARTESIAN_POINT('Ctrl Pts',(-8.85336761800006,15.2,-5.51071498500002));
#275281=CARTESIAN_POINT('Ctrl Pts',(-8.85336761800006,11.6,-5.51071498500002));
#275282=CARTESIAN_POINT('Ctrl Pts',(-8.85215866800005,15.2,-5.51016853300001));
#275283=CARTESIAN_POINT('Ctrl Pts',(-8.85215866800005,11.6,-5.51016853300001));
#275284=CARTESIAN_POINT('Ctrl Pts',(-8.85095800400006,15.2,-5.50962443100001));
#275285=CARTESIAN_POINT('Ctrl Pts',(-8.85095800400006,11.6,-5.50962443100001));
#275286=CARTESIAN_POINT('Ctrl Pts',(-8.84976563900005,15.2,-5.50908269900001));
#275287=CARTESIAN_POINT('Ctrl Pts',(-8.84976563900005,11.6,-5.50908269900001));
#275288=CARTESIAN_POINT('Ctrl Pts',(-8.84858158700006,15.2,-5.50854336400001));
#275289=CARTESIAN_POINT('Ctrl Pts',(-8.84858158700006,11.6,-5.50854336400001));
#275290=CARTESIAN_POINT('Ctrl Pts',(-8.84740586100006,15.2,-5.50800644600002));
#275291=CARTESIAN_POINT('Ctrl Pts',(-8.84740586100006,11.6,-5.50800644600002));
#275292=CARTESIAN_POINT('Ctrl Pts',(-8.84623847600006,15.2,-5.50747197000002));
#275293=CARTESIAN_POINT('Ctrl Pts',(-8.84623847600006,11.6,-5.50747197000002));
#275294=CARTESIAN_POINT('Ctrl Pts',(-8.84507944500006,15.2,-5.50693996000001));
#275295=CARTESIAN_POINT('Ctrl Pts',(-8.84507944500006,11.6,-5.50693996000001));
#275296=CARTESIAN_POINT('Ctrl Pts',(-8.84392878100006,15.2,-5.50641043700002));
#275297=CARTESIAN_POINT('Ctrl Pts',(-8.84392878100006,11.6,-5.50641043700002));
#275298=CARTESIAN_POINT('Ctrl Pts',(-8.84278650000006,15.2,-5.50588342700001));
#275299=CARTESIAN_POINT('Ctrl Pts',(-8.84278650000006,11.6,-5.50588342700001));
#275300=CARTESIAN_POINT('Ctrl Pts',(-8.84165261400006,15.2,-5.50535895400001));
#275301=CARTESIAN_POINT('Ctrl Pts',(-8.84165261400006,11.6,-5.50535895400001));
#275302=CARTESIAN_POINT('Ctrl Pts',(-8.84052713700006,15.2,-5.50483704100001));
#275303=CARTESIAN_POINT('Ctrl Pts',(-8.84052713700006,11.6,-5.50483704100001));
#275304=CARTESIAN_POINT('Ctrl Pts',(-8.83941008400006,15.2,-5.50431771200001));
#275305=CARTESIAN_POINT('Ctrl Pts',(-8.83941008400006,11.6,-5.50431771200001));
#275306=CARTESIAN_POINT('Ctrl Pts',(-8.83830146800006,15.2,-5.50380099200002));
#275307=CARTESIAN_POINT('Ctrl Pts',(-8.83830146800006,11.6,-5.50380099200002));
#275308=CARTESIAN_POINT('Ctrl Pts',(-8.83720130500006,15.2,-5.50328690400002));
#275309=CARTESIAN_POINT('Ctrl Pts',(-8.83720130500006,11.6,-5.50328690400002));
#275310=CARTESIAN_POINT('Ctrl Pts',(-8.83610960700006,15.2,-5.50277547300002));
#275311=CARTESIAN_POINT('Ctrl Pts',(-8.83610960700006,11.6,-5.50277547300002));
#275312=CARTESIAN_POINT('Ctrl Pts',(-8.83502638900006,15.2,-5.50226672400001));
#275313=CARTESIAN_POINT('Ctrl Pts',(-8.83502638900006,11.6,-5.50226672400001));
#275314=CARTESIAN_POINT('Ctrl Pts',(-8.83395166600006,15.2,-5.50176068100001));
#275315=CARTESIAN_POINT('Ctrl Pts',(-8.83395166600006,11.6,-5.50176068100001));
#275316=CARTESIAN_POINT('Ctrl Pts',(-8.83288545200006,15.2,-5.50125736900001));
#275317=CARTESIAN_POINT('Ctrl Pts',(-8.83288545200006,11.6,-5.50125736900001));
#275318=CARTESIAN_POINT('Ctrl Pts',(-8.83182776000006,15.2,-5.50075681300001));
#275319=CARTESIAN_POINT('Ctrl Pts',(-8.83182776000006,11.6,-5.50075681300001));
#275320=CARTESIAN_POINT('Ctrl Pts',(-8.83077860600006,15.2,-5.50025903800002));
#275321=CARTESIAN_POINT('Ctrl Pts',(-8.83077860600006,11.6,-5.50025903800002));
#275322=CARTESIAN_POINT('Ctrl Pts',(-8.82973800300006,15.2,-5.49976406800001));
#275323=CARTESIAN_POINT('Ctrl Pts',(-8.82973800300006,11.6,-5.49976406800001));
#275324=CARTESIAN_POINT('Ctrl Pts',(-8.82870596800006,15.2,-5.49927193100002));
#275325=CARTESIAN_POINT('Ctrl Pts',(-8.82870596800006,11.6,-5.49927193100002));
#275326=CARTESIAN_POINT('Ctrl Pts',(-8.82768251300006,15.2,-5.49878264900002));
#275327=CARTESIAN_POINT('Ctrl Pts',(-8.82768251300006,11.6,-5.49878264900002));
#275328=CARTESIAN_POINT('Ctrl Pts',(-8.82666765400005,15.2,-5.49829625000001));
#275329=CARTESIAN_POINT('Ctrl Pts',(-8.82666765400005,11.6,-5.49829625000001));
#275330=CARTESIAN_POINT('Ctrl Pts',(-8.82566140500006,15.2,-5.49781275800001));
#275331=CARTESIAN_POINT('Ctrl Pts',(-8.82566140500006,11.6,-5.49781275800001));
#275332=CARTESIAN_POINT('Ctrl Pts',(-8.82466378100006,15.2,-5.49733219900002));
#275333=CARTESIAN_POINT('Ctrl Pts',(-8.82466378100006,11.6,-5.49733219900002));
#275334=CARTESIAN_POINT('Ctrl Pts',(-8.82367479800006,15.2,-5.49685460000001));
#275335=CARTESIAN_POINT('Ctrl Pts',(-8.82367479800006,11.6,-5.49685460000001));
#275336=CARTESIAN_POINT('Ctrl Pts',(-8.82269446900006,15.2,-5.49637998700002));
#275337=CARTESIAN_POINT('Ctrl Pts',(-8.82269446900006,11.6,-5.49637998700002));
#275338=CARTESIAN_POINT('Ctrl Pts',(-8.82172281000006,15.2,-5.49590838500002));
#275339=CARTESIAN_POINT('Ctrl Pts',(-8.82172281000006,11.6,-5.49590838500002));
#275340=CARTESIAN_POINT('Ctrl Pts',(-8.82075983700006,15.2,-5.49543981900001));
#275341=CARTESIAN_POINT('Ctrl Pts',(-8.82075983700006,11.6,-5.49543981900001));
#275342=CARTESIAN_POINT('Ctrl Pts',(-8.81980556200006,15.2,-5.49497431900001));
#275343=CARTESIAN_POINT('Ctrl Pts',(-8.81980556200006,11.6,-5.49497431900001));
